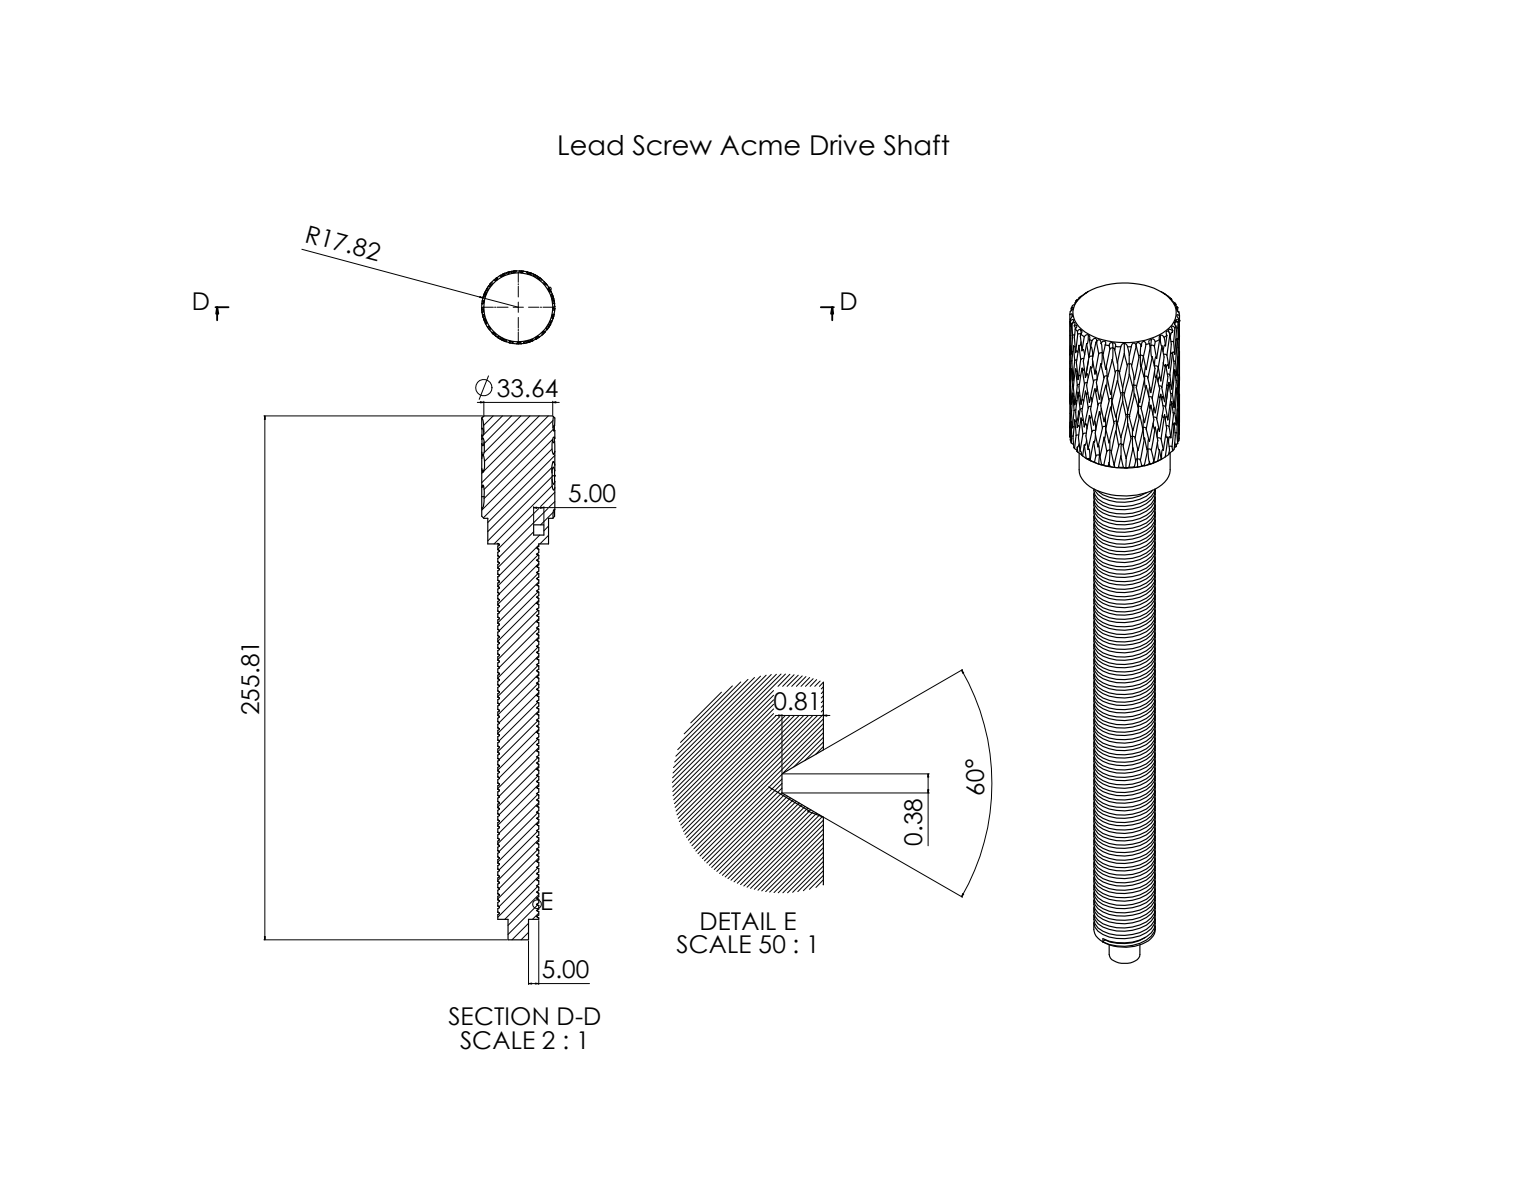
ISO-10303-21;
HEADER;
FILE_DESCRIPTION (('STEP AP214'),
    '1' );
FILE_NAME ('Lead Screw Acme Drive Shaft.step',
    '2026-10-24T22:31:37',
    ( '' ),
    ( '' ),
    'SwSTEP 2.0',
    'SolidWorks 2025',
    '' );
FILE_SCHEMA (( 'AUTOMOTIVE_DESIGN' ));
ENDSEC;

DATA;
#2=EDGE_CURVE ( 'NONE', #71353, #27127, #17244, .T. ) ;
#5=CARTESIAN_POINT ( 'NONE',  ( 165.5065167046122099, 285.3186853228385758, 0.5240180121679646197 ) ) ;
#6=CARTESIAN_POINT ( 'NONE',  ( 181.3318829485781976, 258.8378521386378566, -10.46588027007283017 ) ) ;
#8=ORIENTED_EDGE ( 'NONE', *, *, #76052, .F. ) ;
#9=CARTESIAN_POINT ( 'NONE',  ( 192.4853974341616549, 296.6629111496555424, 11.26379224701618398 ) ) ;
#12=CARTESIAN_POINT ( 'NONE',  ( 201.3053499423511425, 281.9759013948520874, -16.75960365258566398 ) ) ;
#15=CARTESIAN_POINT ( 'NONE',  ( 199.8044370756099966, 266.7412756917946695, 4.662294411209313871 ) ) ;
#16=CARTESIAN_POINT ( 'NONE',  ( 202.7688273210276293, 274.1343011241658587, 13.26872680179261366 ) ) ;
#19=CARTESIAN_POINT ( 'NONE',  ( 199.0151342380902406, 265.3454304162409585, 1.621217956766562551 ) ) ;
#20=CARTESIAN_POINT ( 'NONE',  ( 154.6973317394036940, 271.0068791071395253, 14.01324914462427174 ) ) ;
#21=VERTEX_POINT ( 'NONE', #91655 ) ;
#22=CARTESIAN_POINT ( 'NONE',  ( 146.8195026170398023, 276.3481572557323034, 4.765869558735466249 ) ) ;
#23=CARTESIAN_POINT ( 'NONE',  ( 202.2773826701151165, 280.2922913237452462, 16.62862787739668846 ) ) ;
#24=CARTESIAN_POINT ( 'NONE',  ( 164.2578067403839555, 246.1441285162624126, -2.322300236470859591 ) ) ;
#26=B_SPLINE_CURVE_WITH_KNOTS ( 'NONE', 3,
 ( #42002, #50106, #43488, #81061 ),
 .UNSPECIFIED., .F., .F.,
 ( 4, 4 ),
 ( 0.04462388129695979422, 0.04887120950165262795 ),
 .UNSPECIFIED. ) ;
#29=CARTESIAN_POINT ( 'NONE',  ( 171.0277932295235814, 274.5471866711665712, 17.25980421070102366 ) ) ;
#32=CARTESIAN_POINT ( 'NONE',  ( -22.42236680055709641, 157.8615022471902591, 0.000000000000000000 ) ) ;
#33=CARTESIAN_POINT ( 'NONE',  ( 149.7543087857887656, 247.2677522451417929, -5.000000000000041744 ) ) ;
#34=CARTESIAN_POINT ( 'NONE',  ( 82.20432729060253507, 208.2677522451417929, -5.000000000000041744 ) ) ;
#35=VERTEX_POINT ( 'NONE', #22220 ) ;
#41=CARTESIAN_POINT ( 'NONE',  ( 20.25662117580333899, 176.3768266524159856, -9.188101187500093303 ) ) ;
#42=FACE_OUTER_BOUND ( 'NONE', #88886, .T. ) ;
#43=ADVANCED_FACE ( 'NONE', ( #53119 ), #78501, .F. ) ;
#44=CARTESIAN_POINT ( 'NONE',  ( 181.8933809143826466, 275.6627081342313090, -16.43118812148207653 ) ) ;
#46=CARTESIAN_POINT ( 'NONE',  ( 119.5854454918513170, 251.3967562850347122, -4.648177544792955347E-16 ) ) ;
#48=DIRECTION ( 'NONE',  ( -0.8660254037844387076, -0.4999999999999998890, -0.000000000000000000 ) ) ;
#49=CARTESIAN_POINT ( 'NONE',  ( 176.0471099249906217, 252.5555583919553726, -3.347364798285545895 ) ) ;
#50=CARTESIAN_POINT ( 'NONE',  ( 190.7726985512088049, 261.9670508072832718, -0.9699378005772294475 ) ) ;
#51=CARTESIAN_POINT ( 'NONE',  ( 182.4467602783141729, 295.3384606270356585, 1.016252470355397008 ) ) ;
#52=CARTESIAN_POINT ( 'NONE',  ( 71.10837680816226225, 221.8615022471903160, 5.000000000000046185 ) ) ;
#55=CARTESIAN_POINT ( 'NONE',  ( 36.00728465925030974, 191.5958772461660544, -9.188101187500095079 ) ) ;
#57=ADVANCED_FACE ( 'NONE', ( #26227 ), #57103, .T. ) ;
#59=CARTESIAN_POINT ( 'NONE',  ( 72.04657099559547362, 205.7365022471902023, -10.00000000000009237 ) ) ;
#60=CARTESIAN_POINT ( 'NONE',  ( 198.6894790592683080, 286.5067226703918095, -17.06774375037124614 ) ) ;
#61=CARTESIAN_POINT ( 'NONE',  ( 164.2600772519394923, 246.1401958748887182, -2.110785484364219311 ) ) ;
#63=CARTESIAN_POINT ( 'NONE',  ( 159.8708946529933996, 278.4983629143405324, -9.843749539283454197 ) ) ;
#64=CARTESIAN_POINT ( 'NONE',  ( 160.1967185059513383, 280.0836358635930310, 9.265555704265979742 ) ) ;
#66=FACE_OUTER_BOUND ( 'NONE', #40596, .T. ) ;
#68=CARTESIAN_POINT ( 'NONE',  ( 188.9056787950111413, 270.0514309397178181, -14.11362088196558773 ) ) ;
#73=CARTESIAN_POINT ( 'NONE',  ( -4.101579717973121930, 179.9860189848785694, -2.679491924311240503 ) ) ;
#75=EDGE_LOOP ( 'NONE', ( #46929, #82112, #52955, #6832 ) ) ;
#79=CARTESIAN_POINT ( 'NONE',  ( 180.4501283053277803, 256.5846271277198412, -7.835696842545695873 ) ) ;
#81=ORIENTED_EDGE ( 'NONE', *, *, #67086, .T. ) ;
#83=ORIENTED_EDGE ( 'NONE', *, *, #17750, .F. ) ;
#84=CARTESIAN_POINT ( 'NONE',  ( 190.9907605556751093, 299.8412942717858414, 8.799173206188184437 ) ) ;
#85=DIRECTION ( 'NONE',  ( 0.4999999999999992784, -0.8660254037844390407, 0.000000000000000000 ) ) ;
#89=CARTESIAN_POINT ( 'NONE',  ( 148.3280470635002928, 273.7352816289870248, 9.058704604771318003 ) ) ;
#90=CARTESIAN_POINT ( 'NONE',  ( 196.4783028304046013, 290.3365922432724346, -16.37291435488387492 ) ) ;
#91=CARTESIAN_POINT ( 'NONE',  ( 173.2337249902883798, 270.7486416191997023, 17.82094672905207133 ) ) ;
#94=CARTESIAN_POINT ( 'NONE',  ( 159.3297396961336290, 265.7340194281295567, 16.79158499271843041 ) ) ;
#97=CARTESIAN_POINT ( 'NONE',  ( 149.4491471355718772, 271.7934793437897270, 11.43912701239353780 ) ) ;
#101=CARTESIAN_POINT ( 'NONE',  ( 159.7595800023532320, 255.3516961917271999, 16.21405881663931936 ) ) ;
#104=VERTEX_POINT ( 'NONE', #18635 ) ;
#106=CARTESIAN_POINT ( 'NONE',  ( 190.9402756120810523, 299.5005484933402613, 5.898581097966179243 ) ) ;
#108=CARTESIAN_POINT ( 'NONE',  ( 189.8480911035503880, 301.8204558191226283, -0.8992086515915015399 ) ) ;
#109=CARTESIAN_POINT ( 'NONE',  ( 190.2389970918280540, 301.1433867864428748, 4.601241515604689525 ) ) ;
#110=CARTESIAN_POINT ( 'NONE',  ( 173.6269293304046357, 276.7763204810394200, -15.65584202761720611 ) ) ;
#111=CARTESIAN_POINT ( 'NONE',  ( 146.5086121934486982, 276.8866352649785654, -0.04230388357226919777 ) ) ;
#113=CARTESIAN_POINT ( 'NONE',  ( 192.8011239859581849, 296.7056528303708660, -11.79847971295421694 ) ) ;
#114=CARTESIAN_POINT ( 'NONE',  ( 161.7445750920071816, 256.8061939151814386, 15.71254058960433397 ) ) ;
#116=DIRECTION ( 'NONE',  ( -0.8660254037844387076, -0.4999999999999998890, -0.000000000000000000 ) ) ;
#120=CARTESIAN_POINT ( 'NONE',  ( 105.9391831106087380, 219.7202760586659736, -5.415160957724236172E-17 ) ) ;
#122=CARTESIAN_POINT ( 'NONE',  ( 149.0943192338760070, 272.4080592974699471, -12.87526400066115606 ) ) ;
#126=CARTESIAN_POINT ( 'NONE',  ( 180.5399386764078997, 283.1336537301233420, -15.18944844307240238 ) ) ;
#130=VERTEX_POINT ( 'NONE', #94659 ) ;
#131=CARTESIAN_POINT ( 'NONE',  ( 163.0056347026689707, 248.3129541054019569, -11.27842346302751508 ) ) ;
#133=CARTESIAN_POINT ( 'NONE',  ( 45.39824762976388683, 187.0177522451417929, 5.000000000000051514 ) ) ;
#134=CARTESIAN_POINT ( 'NONE',  ( 124.5040820605901217, 248.8149278399160949, -9.188101187500095079 ) ) ;
#135=CARTESIAN_POINT ( 'NONE',  ( 180.7770252323854834, 294.0936096853982349, -2.952313513407788026 ) ) ;
#137=CARTESIAN_POINT ( 'NONE',  ( 157.6673516573649181, 257.5591315650518141, 16.79781451397666103 ) ) ;
#138=CARTESIAN_POINT ( 'NONE',  ( 175.3042518086594441, 253.4457403629180021, -3.880823026268251930 ) ) ;
#139=CARTESIAN_POINT ( 'NONE',  ( 46.23738328933649200, 191.3768266524159856, -9.188101187500091527 ) ) ;
#145=CARTESIAN_POINT ( 'NONE',  ( 146.8358616138309571, 276.3198226421291679, 4.054088818585255716 ) ) ;
#148=CARTESIAN_POINT ( 'NONE',  ( 17.25242200676963833, 170.7677522451417929, -5.000000000000041744 ) ) ;
#149=CARTESIAN_POINT ( 'NONE',  ( 102.9889369814289921, 240.2677522451419065, -5.000000000000047962 ) ) ;
#151=CARTESIAN_POINT ( 'NONE',  ( 163.3854574543125580, 247.6550818016845597, 10.82482370245618775 ) ) ;
#152=CARTESIAN_POINT ( 'NONE',  ( 163.3939361803663246, 247.6403962173759226, -10.78041711314006790 ) ) ;
#153=EDGE_CURVE ( 'NONE', #73023, #47320, #41466, .T. ) ;
#154=CARTESIAN_POINT ( 'NONE',  ( 29.56604717072103483, 194.0024278399160949, 9.188101187500095079 ) ) ;
#156=CARTESIAN_POINT ( 'NONE',  ( 195.4765535648738535, 273.5335777180424657, 14.55181105716135903 ) ) ;
#159=CARTESIAN_POINT ( 'NONE',  ( 194.7274671941087831, 275.0520795863097305, -15.83285290351333785 ) ) ;
#160=CARTESIAN_POINT ( 'NONE',  ( 69.07880331415105957, 204.5643266524160140, 9.188101187500095079 ) ) ;
#161=EDGE_CURVE ( 'NONE', #56410, #9864, #92298, .T. ) ;
#162=CARTESIAN_POINT ( 'NONE',  ( 161.4396252346964218, 251.0253620690641299, 14.51972485405798885 ) ) ;
#167=( BOUNDED_CURVE ( )  B_SPLINE_CURVE ( 2, ( #94120, #92619, #24674, #32772, #7471, #38365, #3886, #40856, #18091 ),
 .UNSPECIFIED., .F., .T. ) 
 B_SPLINE_CURVE_WITH_KNOTS ( ( 3, 2, 2, 2, 3 ),
 ( 0.1330645161290322509, 0.1344086021505376261, 0.1370967741935483764, 0.1397849462365591267, 0.1411290322580645296 ),
 .UNSPECIFIED. ) 
 CURVE ( )  GEOMETRIC_REPRESENTATION_ITEM ( )  RATIONAL_B_SPLINE_CURVE ( ( 0.9330127018922194093, 0.9330127018922194093, 1.000000000000000000, 0.8660254037844387076, 1.000000000000000000, 0.8660254037844387076, 1.000000000000000000, 0.9330127018922187432, 0.9330127018922194093 ) ) 
 REPRESENTATION_ITEM ( '' )  );
#168=CARTESIAN_POINT ( 'NONE',  ( 165.4887069070615269, 269.3414653546907402, 17.07898631664743405 ) ) ;
#169=CARTESIAN_POINT ( 'NONE',  ( 29.10614472461701752, 187.6115022471902591, 10.00000000000009592 ) ) ;
#170=CARTESIAN_POINT ( 'NONE',  ( 208.2175703429120688, 270.0035844679667889, 2.257951022351344150 ) ) ;
#171=CARTESIAN_POINT ( 'NONE',  ( -1.394013918807642360, 163.8768266524159856, 9.188101187500098632 ) ) ;
#173=CARTESIAN_POINT ( 'NONE',  ( 167.7163553651179768, 262.5077956943969753, -16.64284935447819791 ) ) ;
#175=CARTESIAN_POINT ( 'NONE',  ( 185.3704253846254346, 260.3657602090070782, 6.355839938251095944 ) ) ;
#176=CARTESIAN_POINT ( 'NONE',  ( 206.0627831668701901, 273.7357853363691902, 10.14454147593459687 ) ) ;
#181=CARTESIAN_POINT ( 'NONE',  ( 208.2813134324037492, 269.8931781983357041, -0.4511785827856357178 ) ) ;
#188=CARTESIAN_POINT ( 'NONE',  ( 84.96478326871331888, 219.8615022471902591, -10.00000000000009592 ) ) ;
#189=CARTESIAN_POINT ( 'NONE',  ( 173.0837253472800796, 264.8280141993791972, 17.07053884509587860 ) ) ;
#190=CARTESIAN_POINT ( 'NONE',  ( 162.6541320028305506, 248.9217746405196294, -10.16950121496441817 ) ) ;
#197=ORIENTED_EDGE ( 'NONE', *, *, #54268, .F. ) ;
#202=CARTESIAN_POINT ( 'NONE',  ( 171.2743479101317234, 254.4242377521371736, -11.94796457435898951 ) ) ;
#203=CARTESIAN_POINT ( 'NONE',  ( 164.2712161151136172, 246.1209027979328710, 7.276091357954241445 ) ) ;
#206=CARTESIAN_POINT ( 'NONE',  ( 155.6989589471585020, 260.9684877483775267, 17.28906573347438425 ) ) ;
#207=CARTESIAN_POINT ( 'NONE',  ( 151.2455280670316711, 268.6820563007532314, 14.35914944935941229 ) ) ;
#214=CARTESIAN_POINT ( 'NONE',  ( 159.9635946688021022, 268.7707599091479551, -17.14635356962945778 ) ) ;
#217=ORIENTED_EDGE ( 'NONE', *, *, #97229, .F. ) ;
#219=CARTESIAN_POINT ( 'NONE',  ( 207.5792673731680793, 271.1091576421853233, 2.359198794924813214 ) ) ;
#221=CARTESIAN_POINT ( 'NONE',  ( 167.3703162778506055, 281.6204983129350694, 11.41617640160279024 ) ) ;
#222=CARTESIAN_POINT ( 'NONE',  ( 194.9220242159064185, 293.0321458743159724, -14.92681063007793263 ) ) ;
#225=ADVANCED_FACE ( 'NONE', ( #75832 ), #98127, .T. ) ;
#228=CARTESIAN_POINT ( 'NONE',  ( 198.4408884114532725, 277.4403926908931908, -15.34803116808097023 ) ) ;
#232=EDGE_CURVE ( 'NONE', #38319, #90439, #71654, .T. ) ;
#233=CARTESIAN_POINT ( 'NONE',  ( 147.2256490141643042, 275.6446910606013603, -4.110658582098289493 ) ) ;
#236=CARTESIAN_POINT ( 'NONE',  ( 206.3018347371251195, 273.3217358710584790, -9.309724106897926177 ) ) ;
#239=CARTESIAN_POINT ( 'NONE',  ( 171.8224262749942852, 254.8926688302297521, 11.02064826558146748 ) ) ;
#240=CARTESIAN_POINT ( 'NONE',  ( 157.5687383428415274, 281.7222027203141579, 1.387399794590924440 ) ) ;
#242=CARTESIAN_POINT ( 'NONE',  ( 194.3044832453722677, 294.1017582110366106, -14.10778293554018603 ) ) ;
#244=CARTESIAN_POINT ( 'NONE',  ( 141.2767884429413243, 240.8262482093457777, 3.021315404115420679E-15 ) ) ;
#245=CARTESIAN_POINT ( 'NONE',  ( -0.9341114727036189391, 170.2677522451418781, 10.00000000000009592 ) ) ;
#246=CARTESIAN_POINT ( 'NONE',  ( 94.73480590126506229, 219.3768266524160140, 9.188101187500096856 ) ) ;
#247=CARTESIAN_POINT ( 'NONE',  ( 195.8651621160345542, 269.3302623707359658, -10.80388373675355851 ) ) ;
#250=CARTESIAN_POINT ( 'NONE',  ( 170.2105851965358738, 280.7371124046519526, -14.06690082814746390 ) ) ;
#252=CARTESIAN_POINT ( 'NONE',  ( 17.27983239817682559, 168.5327760586659736, 1.948934522072303157E-15 ) ) ;
#254=CARTESIAN_POINT ( 'NONE',  ( 200.4592688079413847, 283.4413569069752725, 18.39277739746426832 ) ) ;
#255=ORIENTED_EDGE ( 'NONE', *, *, #28716, .T. ) ;
#256=ORIENTED_EDGE ( 'NONE', *, *, #59561, .F. ) ;
#257=CARTESIAN_POINT ( 'NONE',  ( 167.4700212936181458, 285.1112495945437786, 9.221858443278774686 ) ) ;
#259=CARTESIAN_POINT ( 'NONE',  ( 157.8159121039657293, 257.3018173235443555, -17.05074702406642118 ) ) ;
#261=CARTESIAN_POINT ( 'NONE',  ( 201.9437967514558920, 280.8700790835527528, -16.67046097481324196 ) ) ;
#262=CARTESIAN_POINT ( 'NONE',  ( 113.9506338607584723, 225.0494855054051868, -2.679491924311248496 ) ) ;
#264=CARTESIAN_POINT ( 'NONE',  ( 23.34166312890287998, 184.2833772461660544, -9.188101187500095079 ) ) ;
#265=CARTESIAN_POINT ( 'NONE',  ( 130.0524911732904343, 236.7048013555409796, 4.594050593750051981 ) ) ;
#266=CARTESIAN_POINT ( 'NONE',  ( 183.1279196651564973, 257.7771318069471249, -2.489900343309737529 ) ) ;
#267=ORIENTED_EDGE ( 'NONE', *, *, #37270, .F. ) ;
#268=CARTESIAN_POINT ( 'NONE',  ( 179.8888715531147682, 274.4711782159853328, -17.82026667163308531 ) ) ;
#269=CARTESIAN_POINT ( 'NONE',  ( -8.863483026448420787, 159.5643266524160140, 9.188101187500095079 ) ) ;
#271=CARTESIAN_POINT ( 'NONE',  ( 194.5047661587782386, 293.7548580291293092, 14.86680123054176583 ) ) ;
#272=CARTESIAN_POINT ( 'NONE',  ( 177.2183068813167495, 256.3290312667157309, -10.31296860541032423 ) ) ;
#273=CARTESIAN_POINT ( 'NONE',  ( 190.1462790299653420, 284.8797699240140560, 17.00550891877788473 ) ) ;
#274=CARTESIAN_POINT ( 'NONE',  ( 147.6508870500795467, 274.9081571770856272, -8.950912509993816712 ) ) ;
#275=CARTESIAN_POINT ( 'NONE',  ( 189.2224370172964143, 262.6230431603515854, 8.075317388220659254 ) ) ;
#276=CARTESIAN_POINT ( 'NONE',  ( 167.7174649547847309, 278.2620246372183601, 14.62053864993239216 ) ) ;
#279=CARTESIAN_POINT ( 'NONE',  ( 148.3707431749605234, 273.6613297946520902, 8.912574527564540716 ) ) ;
#281=ORIENTED_EDGE ( 'NONE', *, *, #67790, .T. ) ;
#283=CARTESIAN_POINT ( 'NONE',  ( 184.9437015084479299, 269.6468049839930927, 15.52015019358652204 ) ) ;
#284=CARTESIAN_POINT ( 'NONE',  ( 109.0781781035623226, 233.7833772461660544, -9.188101187500095079 ) ) ;
#286=CARTESIAN_POINT ( 'NONE',  ( 190.9907605556751093, 299.8412942717858414, 8.799173206188184437 ) ) ;
#288=CYLINDRICAL_SURFACE ( 'NONE', #48455, 17.82106496071139645 ) ;
#290=CARTESIAN_POINT ( 'NONE',  ( 195.5685147139090816, 278.4936960503050045, 16.53693894814080423 ) ) ;
#291=CARTESIAN_POINT ( 'NONE',  ( 201.3138726815416817, 270.7303338844035352, -9.934698065831957692 ) ) ;
#292=CARTESIAN_POINT ( 'NONE',  ( 163.2031704490160848, 279.2514240946757695, 12.88724473550253258 ) ) ;
#293=CARTESIAN_POINT ( 'NONE',  ( 137.7719789713245291, 261.8967562850346553, -4.648177544792955347E-16 ) ) ;
#298=CARTESIAN_POINT ( 'NONE',  ( 163.8995163580303256, 256.4334289116373498, -14.90821826893867730 ) ) ;
#302=CARTESIAN_POINT ( 'NONE',  ( 149.5390997184345281, 271.6376768999995761, -11.52989534384373016 ) ) ;
#305=B_SPLINE_SURFACE_WITH_KNOTS ( 'NONE', 3, 1, ( 
 ( #12840, #43700 ),
 ( #74643, #5218 ),
 ( #82762, #13328 ),
 ( #36596, #67500 ),
 ( #98432, #29023 ),
 ( #59894, #44684 ),
 ( #39075, #60879 ),
 ( #91339, #6708 ),
 ( #61389, #92343 ),
 ( #76606, #22402 ),
 ( #37586, #53297 ),
 ( #7698, #46696 ),
 ( #602, #22892 ),
 ( #14308, #91841 ),
 ( #8206, #99420 ),
 ( #45194, #69988 ),
 ( #69496, #23889 ),
 ( #99915, #7192 ),
 ( #68496, #84250 ),
 ( #92834, #15789 ),
 ( #38077, #54790 ),
 ( #14798, #21899 ),
 ( #68004, #53777 ),
 ( #38590, #77621 ),
 ( #31486, #84740 ),
 ( #76133, #45680 ),
 ( #62378, #29997 ),
 ( #68990, #93335 ),
 ( #109, #85769 ),
 ( #30501, #15281 ),
 ( #46176, #77096 ),
 ( #83745, #30994 ),
 ( #61879, #16297 ),
 ( #23385, #54275 ) ),
 .UNSPECIFIED., .T., .F., .F.,
 ( 4, 2, 2, 2, 2, 2, 2, 2, 2, 2, 2, 2, 2, 2, 2, 2, 4 ),
 ( 2, 2 ),
 ( 0.000000000000000000, 0.06250000000000000000, 0.1250000000000000000, 0.1875000000000000000, 0.2500000000000000000, 0.3125000000000000000, 0.3750000000000000000, 0.4375000000000000000, 0.5000000000000000000, 0.5625000000000000000, 0.6250000000000000000, 0.6875000000000000000, 0.7500000000000000000, 0.8125000000000000000, 0.8750000000000000000, 0.9375000000000000000, 1.000000000000000000 ),
 ( 0.000000000000000000, 1.000000000000000000 ),
 .UNSPECIFIED. ) ;
#309=CARTESIAN_POINT ( 'NONE',  ( 183.6798712561491982, 264.4388490002158960, -13.51192819117503596 ) ) ;
#311=CARTESIAN_POINT ( 'NONE',  ( 152.6845319923753834, 266.1896283897672220, 17.20844521882669653 ) ) ;
#312=VERTEX_POINT ( 'NONE', #28205 ) ;
#316=CARTESIAN_POINT ( 'NONE',  ( 167.5102911960937320, 249.8330499937025309, 6.951336391313942542 ) ) ;
#318=B_SPLINE_CURVE_WITH_KNOTS ( 'NONE', 3,
 ( #32597, #24493, #55372, #7801 ),
 .UNSPECIFIED., .F., .F.,
 ( 4, 4 ),
 ( 0.02854077651451781411, 0.03771323773808555463 ),
 .UNSPECIFIED. ) ;
#321=CARTESIAN_POINT ( 'NONE',  ( 158.9773147466768819, 255.2902089383236159, 17.46634807813732237 ) ) ;
#322=CARTESIAN_POINT ( 'NONE',  ( 192.9115332263593814, 296.5144184163711429, -13.56440505672942898 ) ) ;
#323=CARTESIAN_POINT ( 'NONE',  ( 163.1062016187225936, 254.8584145212696228, 15.52417137768656019 ) ) ;
#327=ORIENTED_EDGE ( 'NONE', *, *, #3828, .T. ) ;
#328=CARTESIAN_POINT ( 'NONE',  ( 195.4130005142917241, 291.0508895501969846, 16.15472393341080348 ) ) ;
#331=ORIENTED_EDGE ( 'NONE', *, *, #16780, .F. ) ;
#332=CARTESIAN_POINT ( 'NONE',  ( 171.7871149756895761, 270.4574563033415870, 16.48193621075655102 ) ) ;
#334=EDGE_CURVE ( 'NONE', #85237, #99635, #55991, .T. ) ;
#338=CARTESIAN_POINT ( 'NONE',  ( 196.1025787785897307, 284.4507243824010629, -17.50425523595241017 ) ) ;
#340=CARTESIAN_POINT ( 'NONE',  ( 167.6634616256541790, 249.2278186638985744, -5.457181400944699057 ) ) ;
#341=DIRECTION ( 'NONE',  ( -0.8660254037844387076, -0.4999999999999998890, -0.000000000000000000 ) ) ;
#343=CARTESIAN_POINT ( 'NONE',  ( 186.8073520874924611, 287.1005927419247996, -15.84640929283254174 ) ) ;
#344=ADVANCED_FACE ( 'NONE', ( #31678 ), #99228, .T. ) ;
#345=CARTESIAN_POINT ( 'NONE',  ( 119.1457234225564008, 239.5958772461660544, -9.188101187500095079 ) ) ;
#346=VERTEX_POINT ( 'NONE', #7914 ) ;
#349=CARTESIAN_POINT ( 'NONE',  ( 189.4928799553373437, 274.7536700704093846, 17.18705487055967396 ) ) ;
#350=ORIENTED_EDGE ( 'NONE', *, *, #95990, .T. ) ;
#352=ORIENTED_EDGE ( 'NONE', *, *, #17619, .T. ) ;
#356=CARTESIAN_POINT ( 'NONE',  ( 171.0928659016861673, 287.7346803495887002, -4.756451642342891972 ) ) ;
#359=CARTESIAN_POINT ( 'NONE',  ( 153.1961624462112752, 265.3034584490234806, -16.19494717845262954 ) ) ;
#360=CARTESIAN_POINT ( 'NONE',  ( 177.2362443690770135, 288.8424983797139021, -9.276591687040479428 ) ) ;
#363=CARTESIAN_POINT ( 'NONE',  ( 164.5340810747928515, 246.5053760637088658, 4.244836759601243514 ) ) ;
#364=ORIENTED_EDGE ( 'NONE', *, *, #82612, .F. ) ;
#365=CARTESIAN_POINT ( 'NONE',  ( 147.9791529310278122, 274.3395839928920168, -7.789432462804474433 ) ) ;
#368=CARTESIAN_POINT ( 'NONE',  ( 188.2054311839045226, 266.2807901288332459, -11.82779421608511150 ) ) ;
#369=CARTESIAN_POINT ( 'NONE',  ( 156.9836120038223726, 276.6206255467238293, 10.24398227673275841 ) ) ;
#370=CARTESIAN_POINT ( 'NONE',  ( 195.6984238921373560, 265.3498530178097212, 4.338345965406653626 ) ) ;
#371=CARTESIAN_POINT ( 'NONE',  ( 179.8888715531147682, 274.4711782159853328, -17.82026667163308531 ) ) ;
#373=CARTESIAN_POINT ( 'NONE',  ( 153.4529711877194131, 270.0553744293359841, 14.23171068006870854 ) ) ;
#375=CARTESIAN_POINT ( 'NONE',  ( 200.7484899876179441, 282.9404111291507888, -16.88964748465601673 ) ) ;
#376=ORIENTED_EDGE ( 'NONE', *, *, #23774, .F. ) ;
#377=CARTESIAN_POINT ( 'NONE',  ( 147.4963928429778264, 275.1757489932608109, 4.929816573182678852 ) ) ;
#379=CARTESIAN_POINT ( 'NONE',  ( 187.3693387071396046, 263.1408467955632204, -9.037621127357647666 ) ) ;
#381=CARTESIAN_POINT ( 'NONE',  ( 173.8665542827094725, 250.6399523573830095, -0.9454928766311748722 ) ) ;
#382=B_SPLINE_CURVE_WITH_KNOTS ( 'NONE', 3,
 ( #16996, #47885, #78827, #78323 ),
 .UNSPECIFIED., .F., .F.,
 ( 4, 4 ),
 ( 0.003697259335896347244, 0.01166702794401381499 ),
 .UNSPECIFIED. ) ;
#383=CARTESIAN_POINT ( 'NONE',  ( 184.7157775894015117, 297.3647472220100099, -4.497232409310948142 ) ) ;
#386=CARTESIAN_POINT ( 'NONE',  ( 155.2419697281468416, 261.7600162942170527, 18.58580762350309357 ) ) ;
#387=CARTESIAN_POINT ( 'NONE',  ( 191.1424450985878138, 283.3691956586972083, -16.58317466969614173 ) ) ;
#389=CARTESIAN_POINT ( 'NONE',  ( 84.82981389336303835, 207.5327760586659167, 1.948934522072303157E-15 ) ) ;
#394=CARTESIAN_POINT ( 'NONE',  ( 202.8535267948003593, 279.2943804273081696, -15.36804658072946062 ) ) ;
#395=DIRECTION ( 'NONE',  ( 0.4999999999999992784, -0.8660254037844390407, 0.000000000000000000 ) ) ;
#397=CARTESIAN_POINT ( 'NONE',  ( 48.76667776935668996, 187.4155109091896065, 2.679491924311254714 ) ) ;
#400=FACE_OUTER_BOUND ( 'NONE', #98699, .T. ) ;
#401=CARTESIAN_POINT ( 'NONE',  ( 166.1592670111344887, 249.7066296865716311, -9.087955240109561572 ) ) ;
#402=CARTESIAN_POINT ( 'NONE',  ( 205.5338712131946863, 274.6518877128656868, -12.59077173197751343 ) ) ;
#403=CARTESIAN_POINT ( 'NONE',  ( 195.8248271798537417, 291.4684452715354155, 17.35175160929494709 ) ) ;
#404=CARTESIAN_POINT ( 'NONE',  ( 167.9211111253673323, 249.4040118433879627, 8.061254949035708606 ) ) ;
#405=CARTESIAN_POINT ( 'NONE',  ( 207.5785076975260779, 271.1104734389944042, -6.824813054587777650 ) ) ;
#406=CARTESIAN_POINT ( 'NONE',  ( 43.09804120061789945, 189.5643266524160140, 9.188101187500095079 ) ) ;
#407=CARTESIAN_POINT ( 'NONE',  ( 56.16917826928300883, 212.4244531367911577, -4.594050593750046652 ) ) ;
#408=CARTESIAN_POINT ( 'NONE',  ( 185.8626946602280441, 259.3471889805154547, 7.308832903665572367 ) ) ;
#411=CARTESIAN_POINT ( 'NONE',  ( 163.8983913010820572, 258.1275895590765685, 15.54516205773220250 ) ) ;
#412=CARTESIAN_POINT ( 'NONE',  ( -3.441976700948088386, 155.4865022471901455, 1.119607411625061291E-15 ) ) ;
#416=CARTESIAN_POINT ( 'NONE',  ( 132.8668134119921547, 247.5177522451418497, -10.00000000000009592 ) ) ;
#419=CARTESIAN_POINT ( 'NONE',  ( 70.29673831216418023, 202.2048013555409796, 4.594050593750051981 ) ) ;
#421=CARTESIAN_POINT ( 'NONE',  ( 155.2193237801463113, 261.7992402267395846, -18.58295809893692407 ) ) ;
#422=CARTESIAN_POINT ( 'NONE',  ( 159.6978881494930249, 254.0421391940632532, 15.34888828951022610 ) ) ;
#424=CARTESIAN_POINT ( 'NONE',  ( 153.3576077035983758, 276.7962943880863804, 7.310696788985877603 ) ) ;
#426=B_SPLINE_CURVE_WITH_KNOTS ( 'NONE', 3,
 ( #1225, #30627, #55888, #713 ),
 .UNSPECIFIED., .F., .F.,
 ( 4, 4 ),
 ( 0.04422796245080886507, 0.04887120950165270428 ),
 .UNSPECIFIED. ) ;
#427=EDGE_CURVE ( 'NONE', #15755, #20151, #43801, .T. ) ;
#429=CARTESIAN_POINT ( 'NONE',  ( 113.4714528099510744, 242.9865022471902876, -10.00000000000009415 ) ) ;
#430=CARTESIAN_POINT ( 'NONE',  ( 200.8828793852583203, 282.7076418644388696, 17.90302398138411633 ) ) ;
#431=CARTESIAN_POINT ( 'NONE',  ( 164.4440639631384045, 245.8215215431751233, -2.910115319305802029 ) ) ;
#432=ORIENTED_EDGE ( 'NONE', *, *, #46720, .F. ) ;
#436=CARTESIAN_POINT ( 'NONE',  ( 206.1405152101578437, 273.6011494880188479, -9.618815605734603480 ) ) ;
#437=CARTESIAN_POINT ( 'NONE',  ( 190.3113039736807934, 278.6935773923744364, -16.50932879894303085 ) ) ;
#439=EDGE_LOOP ( 'NONE', ( #58462, #85908, #2245, #41062 ) ) ;
#440=CARTESIAN_POINT ( 'NONE',  ( 173.3330552357551824, 251.5762317818503959, 0.1350323028907620126 ) ) ;
#441=VERTEX_POINT ( 'NONE', #51248 ) ;
#443=CARTESIAN_POINT ( 'NONE',  ( 147.8308140999695866, 274.5965143850199865, -7.866624397492971710 ) ) ;
#446=ORIENTED_EDGE ( 'NONE', *, *, #42908, .T. ) ;
#454=CARTESIAN_POINT ( 'NONE',  ( 206.7680519836501958, 272.5142239127119979, -10.57935479673322021 ) ) ;
#455=ORIENTED_EDGE ( 'NONE', *, *, #60528, .T. ) ;
#456=CARTESIAN_POINT ( 'NONE',  ( 174.8047606067528363, 286.1344884131184472, 10.79450168243746688 ) ) ;
#457=EDGE_CURVE ( 'NONE', #20349, #15680, #60827, .T. ) ;
#458=CARTESIAN_POINT ( 'NONE',  ( 162.5887743522035294, 284.9919049736276975, -2.844505511527740005 ) ) ;
#460=CARTESIAN_POINT ( 'NONE',  ( 163.4218292706009095, 247.5920839679097014, -10.44611490715852042 ) ) ;
#461=CARTESIAN_POINT ( 'NONE',  ( 204.9103773355753617, 275.7318107871104189, 13.62808820451859937 ) ) ;
#462=CARTESIAN_POINT ( 'NONE',  ( 185.4002507578896086, 292.6011188852542091, -10.72436994641770269 ) ) ;
#463=CARTESIAN_POINT ( 'NONE',  ( 164.3112807403088595, 265.7596940169248683, -17.57772941833111346 ) ) ;
#464=CARTESIAN_POINT ( 'NONE',  ( 141.8249372320439647, 246.5643266524160140, 9.188101187500095079 ) ) ;
#465=CARTESIAN_POINT ( 'NONE',  ( 165.2663344650013642, 263.6115507486170486, 17.68040007492823662 ) ) ;
#467=CARTESIAN_POINT ( 'NONE',  ( 181.8478599454992661, 260.3285582005539709, 9.484317556428793594 ) ) ;
#468=CARTESIAN_POINT ( 'NONE',  ( 71.08131351252005459, 211.8458772461660544, 9.188101187500095079 ) ) ;
#469=VERTEX_POINT ( 'NONE', #18019 ) ;
#470=CARTESIAN_POINT ( 'NONE',  ( 191.0900422946452011, 299.6693332556258724, 8.872191398975367349 ) ) ;
#473=CARTESIAN_POINT ( 'NONE',  ( 196.0559066898898379, 291.0682038195648715, -16.90522961251436485 ) ) ;
#474=ORIENTED_EDGE ( 'NONE', *, *, #73314, .T. ) ;
#476=EDGE_CURVE ( 'NONE', #86658, #66772, #15991, .T. ) ;
#480=CARTESIAN_POINT ( 'NONE',  ( 56.79295721098551297, 192.0494855054051868, -2.679491924311248496 ) ) ;
#481=CARTESIAN_POINT ( 'NONE',  ( 162.4279131726858623, 249.3135971479585464, 10.85034575916916921 ) ) ;
#482=CARTESIAN_POINT ( 'NONE',  ( 87.75264963113552596, 209.2202760586659167, -5.415160957724236172E-17 ) ) ;
#483=VERTEX_POINT ( 'NONE', #71220 ) ;
#487=CARTESIAN_POINT ( 'NONE',  ( 161.3271158790198001, 251.2202339894231216, -13.00083852162470244 ) ) ;
#490=CARTESIAN_POINT ( 'NONE',  ( 184.0117498620529659, 275.1892951444139612, 16.37277468287277671 ) ) ;
#491=ADVANCED_FACE ( 'NONE', ( #88467 ), #10916, .T. ) ;
#492=CARTESIAN_POINT ( 'NONE',  ( 206.4695239676918845, 273.0312896038346366, 10.41704154450801667 ) ) ;
#493=CARTESIAN_POINT ( 'NONE',  ( 161.9109773315472012, 284.6651530195127293, 0.5383145704399616704 ) ) ;
#495=CARTESIAN_POINT ( 'NONE',  ( 162.8949375270381665, 261.5393056731645061, 17.17550692532979895 ) ) ;
#499=CARTESIAN_POINT ( 'NONE',  ( 152.9251141908703175, 265.7729277985770864, -16.20110192949203309 ) ) ;
#503=CARTESIAN_POINT ( 'NONE',  ( 195.7907645185857461, 265.4364973583962524, 4.438536951565118294 ) ) ;
#504=CARTESIAN_POINT ( 'NONE',  ( 98.80083580102480312, 239.3967562850347122, -4.648177544792955347E-16 ) ) ;
#506=CARTESIAN_POINT ( 'NONE',  ( 187.8986993795193428, 266.2277010579576881, -11.94388868202539911 ) ) ;
#507=CARTESIAN_POINT ( 'NONE',  ( 198.6368176188399275, 266.0031191539155770, 1.462458297540865537 ) ) ;
#510=B_SPLINE_CURVE_WITH_KNOTS ( 'NONE', 3,
 ( #45409, #38802, #46912, #7929 ),
 .UNSPECIFIED., .F., .F.,
 ( 4, 4 ),
 ( 0.02277490244884483594, 0.03199231217593029308 ),
 .UNSPECIFIED. ) ;
#513=CARTESIAN_POINT ( 'NONE',  ( 202.5511585997265911, 279.8180975037686835, 17.12781264818056925 ) ) ;
#514=DIRECTION ( 'NONE',  ( -0.8660254037844359321, -0.5000000000000051070, -0.000000000000000000 ) ) ;
#517=CARTESIAN_POINT ( 'NONE',  ( 176.1295626651131556, 285.2769818187388751, -12.16386616229632800 ) ) ;
#520=CARTESIAN_POINT ( 'NONE',  ( 168.9255865893414921, 272.9744073663551376, 15.96626197445653261 ) ) ;
#522=CARTESIAN_POINT ( 'NONE',  ( 176.3945350884862933, 261.0281843545697029, -14.71337765310037504 ) ) ;
#523=CARTESIAN_POINT ( 'NONE',  ( 188.2324206269368858, 260.8148967101335529, 3.170919259758945952 ) ) ;
#524=CARTESIAN_POINT ( 'NONE',  ( 12.40843950188935629, 165.7202760586659736, -5.415160957724236172E-17 ) ) ;
#528=CARTESIAN_POINT ( 'NONE',  ( -22.42236680055709641, 157.8615022471902591, 0.000000000000000000 ) ) ;
#531=CARTESIAN_POINT ( 'NONE',  ( 25.61497981383703149, 185.5958772461660544, -9.188101187500095079 ) ) ;
#535=CARTESIAN_POINT ( 'NONE',  ( 191.7247331938518187, 298.5700163710982338, -9.650650827884682315 ) ) ;
#536=CARTESIAN_POINT ( 'NONE',  ( 142.5294721856450053, 241.5494855054051584, -2.679491924311248496 ) ) ;
#537=B_SPLINE_SURFACE_WITH_KNOTS ( 'NONE', 3, 1, ( 
 ( #25794, #64786 ),
 ( #41970, #96714 ),
 ( #10586, #19203 ),
 ( #57158, #3497 ),
 ( #88139, #43459 ),
 ( #50560, #42940 ),
 ( #41459, #81030 ),
 ( #96214, #56670 ),
 ( #73879, #4472 ),
 ( #26777, #57658 ),
 ( #11593, #11095 ),
 ( #34855, #82013 ),
 ( #66275, #97210 ),
 ( #89625, #74400 ),
 ( #87655, #49084 ),
 ( #80017, #72402 ),
 ( #3009, #33901 ),
 ( #95732, #26284 ),
 ( #18685, #49568 ),
 ( #72907, #14572 ),
 ( #75892, #28768 ),
 ( #22162, #29274 ),
 ( #15043, #76853 ),
 ( #5967, #43950 ),
 ( #98186, #30258 ),
 ( #82527, #74889 ),
 ( #84500, #22668 ),
 ( #59650, #97693 ),
 ( #98692, #37349 ),
 ( #28262, #45448 ),
 ( #90621, #44952 ),
 ( #92116, #36356 ),
 ( #76381, #21185 ),
 ( #14066, #60636 ) ),
 .UNSPECIFIED., .T., .F., .F.,
 ( 4, 2, 2, 2, 2, 2, 2, 2, 2, 2, 2, 2, 2, 2, 2, 2, 4 ),
 ( 2, 2 ),
 ( 0.000000000000000000, 0.06250000000000000000, 0.1250000000000000000, 0.1875000000000000000, 0.2500000000000000000, 0.3125000000000000000, 0.3750000000000000000, 0.4375000000000000000, 0.5000000000000000000, 0.5625000000000000000, 0.6250000000000000000, 0.6875000000000000000, 0.7500000000000000000, 0.8125000000000000000, 0.8750000000000000000, 0.9375000000000000000, 1.000000000000000000 ),
 ( 0.000000000000000000, 1.000000000000000000 ),
 .UNSPECIFIED. ) ;
#539=CARTESIAN_POINT ( 'NONE',  ( 174.3697573357644899, 277.1653490889620457, -17.12727634137145571 ) ) ;
#541=EDGE_CURVE ( 'NONE', #2236, #46058, #2271, .T. ) ;
#542=CARTESIAN_POINT ( 'NONE',  ( 183.0713581288837304, 295.8141884393991745, 1.453977782348063963 ) ) ;
#543=CARTESIAN_POINT ( 'NONE',  ( 64.97403019802248991, 214.9865022471903160, 10.00000000000009237 ) ) ;
#545=CARTESIAN_POINT ( 'NONE',  ( 205.7559715084180425, 271.1536124878838336, 6.114938359024117531 ) ) ;
#546=EDGE_CURVE ( 'NONE', #4549, #55003, #44142, .T. ) ;
#547=CARTESIAN_POINT ( 'NONE',  ( 24.66750420662404508, 194.2369531367911293, -4.594050593750048428 ) ) ;
#549=EDGE_CURVE ( 'NONE', #7391, #22636, #70359, .T. ) ;
#550=CARTESIAN_POINT ( 'NONE',  ( 73.72680694775513643, 201.8262482093457777, 3.021315404115420679E-15 ) ) ;
#551=CARTESIAN_POINT ( 'NONE',  ( 198.8570476668614049, 286.2164853282868080, -17.01721544293231858 ) ) ;
#554=CARTESIAN_POINT ( 'NONE',  ( 159.9770076892122006, 278.5918188642896212, -9.796288430209179054 ) ) ;
#556=SHAPE_DEFINITION_REPRESENTATION ( #17576, #88422 ) ;
#558=CARTESIAN_POINT ( 'NONE',  ( 190.5444288681022442, 300.6143634316900943, -1.000014190476072873 ) ) ;
#559=CARTESIAN_POINT ( 'NONE',  ( 100.0535195437283988, 240.1199935810941213, 2.679491924311251605 ) ) ;
#562=CARTESIAN_POINT ( 'NONE',  ( 185.5148080131019412, 290.8628339942631555, 13.12244952321606206 ) ) ;
#565=CARTESIAN_POINT ( 'NONE',  ( -3.532187684056978583, 178.7677522451419350, -5.000000000000047962 ) ) ;
#567=CARTESIAN_POINT ( 'NONE',  ( 174.1456200854750023, 291.7975269716956177, -2.042136877227955782 ) ) ;
#569=CARTESIAN_POINT ( 'NONE',  ( 150.8167050463783312, 269.4247995599803289, 14.38040671671637938 ) ) ;
#570=CARTESIAN_POINT ( 'NONE',  ( 180.2008674086625888, 256.3788900776044102, -7.862092545524210330 ) ) ;
#573=CARTESIAN_POINT ( 'NONE',  ( 189.0587110057432483, 273.8589833282692325, -15.65961006902252883 ) ) ;
#576=CARTESIAN_POINT ( 'NONE',  ( 191.3375250863502970, 299.2406804863936145, 8.828791580707859410 ) ) ;
#580=CARTESIAN_POINT ( 'NONE',  ( 190.5154909595809727, 300.6644853595138329, -0.04129855346138300298 ) ) ;
#584=CARTESIAN_POINT ( 'NONE',  ( 161.8159150606452670, 267.0902596021308568, 16.49972241951906327 ) ) ;
#585=ORIENTED_EDGE ( 'NONE', *, *, #42908, .F. ) ;
#587=CARTESIAN_POINT ( 'NONE',  ( 149.5593209768671841, 271.6026526530012575, 11.55487339793564949 ) ) ;
#592=CARTESIAN_POINT ( 'NONE',  ( 150.2494575935072874, 270.4073009688167986, 14.61449051812962985 ) ) ;
#598=AXIS2_PLACEMENT_3D ( 'NONE', #72578, #77279, #80192 ) ;
#600=CARTESIAN_POINT ( 'NONE',  ( 190.5444288681022442, 300.6143634316900943, -1.000014190476072873 ) ) ;
#602=CARTESIAN_POINT ( 'NONE',  ( 190.6023073677431512, 300.5141149296460981, 3.174888932019753973 ) ) ;
#603=CARTESIAN_POINT ( 'NONE',  ( 132.5758265486178971, 258.8967562850347122, -4.648177544792955347E-16 ) ) ;
#604=CARTESIAN_POINT ( 'NONE',  ( 191.0739205222354258, 299.6972569845476073, 8.800115285385583519 ) ) ;
#605=CARTESIAN_POINT ( 'NONE',  ( 147.4323331177958494, 275.2867036919951147, -5.064030047414062707 ) ) ;
#607=CARTESIAN_POINT ( 'NONE',  ( 163.5023530932012079, 257.7703811534142346, 15.52546879389397461 ) ) ;
#610=CARTESIAN_POINT ( 'NONE',  ( 205.7576124508049418, 274.2643565215761328, 10.88614016733041545 ) ) ;
#614=CARTESIAN_POINT ( 'NONE',  ( 115.2218061334819623, 228.1423013555409796, -4.594050593750043987 ) ) ;
#615=ORIENTED_EDGE ( 'NONE', *, *, #63474, .T. ) ;
#616=CARTESIAN_POINT ( 'NONE',  ( 190.0576675296552764, 301.4574588010404455, -4.282990501740621347 ) ) ;
#619=CARTESIAN_POINT ( 'NONE',  ( 203.1705638993064156, 278.7452560544191442, -15.08126533799095093 ) ) ;
#621=CARTESIAN_POINT ( 'NONE',  ( 192.6159067191336476, 296.6392389330721926, 11.36185169173896448 ) ) ;
#623=CARTESIAN_POINT ( 'NONE',  ( 198.6444633007815810, 284.5846922512318997, -17.80363864581810418 ) ) ;
#624=ORIENTED_EDGE ( 'NONE', *, *, #90672, .T. ) ;
#625=CARTESIAN_POINT ( 'NONE',  ( 162.9383752892161397, 248.4294508267893491, -11.25953730674605957 ) ) ;
#628=CARTESIAN_POINT ( 'NONE',  ( 206.3009434829942279, 272.9081483067511158, 8.547891559723822752 ) ) ;
#629=CARTESIAN_POINT ( 'NONE',  ( 124.8827946268633298, 255.1589784336661069, -6.496448406907676862E-16 ) ) ;
#630=CARTESIAN_POINT ( 'NONE',  ( 190.2913651263166628, 294.6875229615724265, -12.30047797060472803 ) ) ;
#632=CARTESIAN_POINT ( 'NONE',  ( 196.2609093297512857, 290.7131288316392670, 16.03897268885959448 ) ) ;
#635=CARTESIAN_POINT ( 'NONE',  ( 57.73936995728981714, 194.9548013555410080, -4.594050593750042211 ) ) ;
#637=ORIENTED_EDGE ( 'NONE', *, *, #87810, .T. ) ;
#640=CARTESIAN_POINT ( 'NONE',  ( 21.31191609055706593, 183.1115022471902591, 10.00000000000009592 ) ) ;
#641=CARTESIAN_POINT ( 'NONE',  ( 174.4676371989123140, 262.1820789082375995, 14.34376349448554144 ) ) ;
#643=CARTESIAN_POINT ( 'NONE',  ( 154.9528145190857344, 262.2608478075840708, -17.26679351315302213 ) ) ;
#644=CARTESIAN_POINT ( 'NONE',  ( 178.2689201652922861, 261.3463682195790625, 12.89043557696258979 ) ) ;
#645=CARTESIAN_POINT ( 'NONE',  ( 100.3908607700756619, 238.7677522451419065, -5.000000000000047962 ) ) ;
#647=ORIENTED_EDGE ( 'NONE', *, *, #96875, .T. ) ;
#648=CARTESIAN_POINT ( 'NONE',  ( 202.6070187115982719, 279.7213449518906145, 15.56322169823762280 ) ) ;
#650=CARTESIAN_POINT ( 'NONE',  ( 29.48529115882250551, 178.6423013555409796, -4.594050593750043987 ) ) ;
#655=CARTESIAN_POINT ( 'NONE',  ( 174.4019427205360842, 268.6781143085732992, 17.66204038257215458 ) ) ;
#656=CARTESIAN_POINT ( 'NONE',  ( 67.50895872190925218, 209.7833772461660544, -9.188101187500095079 ) ) ;
#657=CARTESIAN_POINT ( 'NONE',  ( 164.4817765375028102, 245.7562014482918755, -6.334578229142199035 ) ) ;
#659=CARTESIAN_POINT ( 'NONE',  ( 45.37789370152431445, 208.5530062829863027, -4.648177544792955347E-16 ) ) ;
#661=ORIENTED_EDGE ( 'NONE', *, *, #87113, .F. ) ;
#663=CARTESIAN_POINT ( 'NONE',  ( 164.0312634879877294, 268.4089602666911105, 16.55773273759760400 ) ) ;
#664=CARTESIAN_POINT ( 'NONE',  ( 22.68312297988236992, 197.2365022471903444, 2.944929066748280225E-16 ) ) ;
#665=CARTESIAN_POINT ( 'NONE',  ( 163.1008115941903895, 248.1481028935802442, 11.25332017433677834 ) ) ;
#666=CARTESIAN_POINT ( 'NONE',  ( -4.614459115189767147, 158.9548013555409796, -4.594050593750042211 ) ) ;
#668=CARTESIAN_POINT ( 'NONE',  ( 164.4039089034689027, 259.8557547647841943, -16.35869283172417710 ) ) ;
#669=CARTESIAN_POINT ( 'NONE',  ( 170.1430290936755227, 263.5485301713791841, 15.83574950237116141 ) ) ;
#671=CARTESIAN_POINT ( 'NONE',  ( 185.5569508314414406, 260.4628387231232409, 6.337775543338724837 ) ) ;
#672=CARTESIAN_POINT ( 'NONE',  ( 206.0691053506789387, 273.7248349927971844, 11.70564474658248422 ) ) ;
#674=CARTESIAN_POINT ( 'NONE',  ( 183.8314122675164981, 256.5947891462430448, -1.876126292579811894 ) ) ;
#677=CARTESIAN_POINT ( 'NONE',  ( 135.2899281637556896, 260.4637435831425023, 2.679491924311251605 ) ) ;
#679=CARTESIAN_POINT ( 'NONE',  ( 181.7952694153465245, 287.8449457046345970, 13.56394578825295305 ) ) ;
#680=CARTESIAN_POINT ( 'NONE',  ( 196.2127072044743272, 290.0836373517121274, 16.37479000986071398 ) ) ;
#682=ORIENTED_EDGE ( 'NONE', *, *, #27159, .T. ) ;
#683=CARTESIAN_POINT ( 'NONE',  ( 160.3856437025401931, 252.8509116329982191, 16.19741910828728493 ) ) ;
#684=CARTESIAN_POINT ( 'NONE',  ( 157.3029956111992362, 258.1902147490555421, -18.22269824972649843 ) ) ;
#686=CARTESIAN_POINT ( 'NONE',  ( 207.6477529416552557, 270.9905371579805546, 7.447146952410988341 ) ) ;
#687=CARTESIAN_POINT ( 'NONE',  ( 185.2057911854575138, 276.7165103822673586, 17.80337911918299909 ) ) ;
#688=CARTESIAN_POINT ( 'NONE',  ( 163.0056347026689707, 248.3129541054019569, -11.27842346302751508 ) ) ;
#689=CARTESIAN_POINT ( 'NONE',  ( 153.0444155045374544, 265.5662918618958201, -16.15173036748435109 ) ) ;
#690=VERTEX_POINT ( 'NONE', #63350 ) ;
#691=CARTESIAN_POINT ( 'NONE',  ( 190.8932553518572206, 280.9403775647153338, 16.64665765453319679 ) ) ;
#699=CARTESIAN_POINT ( 'NONE',  ( 149.7072529793668707, 271.3464269086063041, -11.98883662638834657 ) ) ;
#702=CARTESIAN_POINT ( 'NONE',  ( 200.6129772034685175, 283.1751261563724142, 18.36811917402039640 ) ) ;
#704=CARTESIAN_POINT ( 'NONE',  ( 151.2591548104722108, 274.8925958778597192, -8.633445779095369588 ) ) ;
#705=VERTEX_POINT ( 'NONE', #23335 ) ;
#711=ORIENTED_EDGE ( 'NONE', *, *, #24354, .F. ) ;
#712=CARTESIAN_POINT ( 'NONE',  ( 207.5215400641004351, 271.2091442744748520, 2.886080616848571534 ) ) ;
#713=CARTESIAN_POINT ( 'NONE',  ( 198.7045056313791633, 284.4806958840320021, 17.79791830837532274 ) ) ;
#715=CARTESIAN_POINT ( 'NONE',  ( 148.3025927079438304, 273.7793698660844939, -8.046026357031887954 ) ) ;
#716=CARTESIAN_POINT ( 'NONE',  ( 175.1828650004762267, 290.0278138422783627, 6.199890812727518075 ) ) ;
#721=CARTESIAN_POINT ( 'NONE',  ( 198.3666213183647926, 277.3917214242281375, -15.34159264812408452 ) ) ;
#723=CARTESIAN_POINT ( 'NONE',  ( 193.0512205562391159, 275.6825563886401369, -16.88465587640301280 ) ) ;
#725=CARTESIAN_POINT ( 'NONE',  ( 191.1159732739488106, 299.6244194819818745, 5.816361631709846769 ) ) ;
#727=CARTESIAN_POINT ( 'NONE',  ( 159.4491226731523454, 254.4730136382542582, -15.39140229921534520 ) ) ;
#732=CARTESIAN_POINT ( 'NONE',  ( 200.4116241316243645, 283.5238799070667142, 18.37703770054986663 ) ) ;
#734=VERTEX_POINT ( 'NONE', #24355 ) ;
#735=CARTESIAN_POINT ( 'NONE',  ( 193.8687075137383999, 294.8565439189318340, -14.51137100490168486 ) ) ;
#736=LINE ( 'NONE', #24036, #27376 ) ;
#737=EDGE_CURVE ( 'NONE', #53287, #48247, #79529, .T. ) ;
#738=CARTESIAN_POINT ( 'NONE',  ( 15.88121511744428282, 166.6427522451417644, 1.119607411625061291E-15 ) ) ;
#739=CARTESIAN_POINT ( 'NONE',  ( 85.91165145656357538, 232.6589784336661353, -6.496448406907676862E-16 ) ) ;
#741=CYLINDRICAL_SURFACE ( 'NONE', #85952, 17.82106496071139645 ) ;
#742=CARTESIAN_POINT ( 'NONE',  ( 166.9577072416738019, 278.1838835069849551, -13.42963054343457863 ) ) ;
#744=CARTESIAN_POINT ( 'NONE',  ( 9.079046938504149011, 185.2369531367911293, -4.594050593750048428 ) ) ;
#746=CARTESIAN_POINT ( 'NONE',  ( 161.4025183475459073, 251.0896330829197041, 14.50747140106038735 ) ) ;
#748=UNCERTAINTY_MEASURE_WITH_UNIT (LENGTH_MEASURE( 1.000000000000000082E-05 ), #95770, 'distance_accuracy_value', 'NONE');
#751=CARTESIAN_POINT ( 'NONE',  ( 197.6375537770108792, 265.0377995068387804, -2.979366280021975122 ) ) ;
#753=CARTESIAN_POINT ( 'NONE',  ( 202.6448056009234904, 279.6558961397194594, -17.13147024041661126 ) ) ;
#754=( BOUNDED_CURVE ( )  B_SPLINE_CURVE ( 2, ( #51590, #82036, #12612, #50581, #74420, #81531, #96236, #65295, #83027 ),
 .UNSPECIFIED., .F., .T. ) 
 B_SPLINE_CURVE_WITH_KNOTS ( ( 3, 2, 2, 2, 3 ),
 ( 0.3266129032258064391, 0.3279569892473118142, 0.3306451612903225645, 0.3333333333333333148, 0.3346774193548386900 ),
 .UNSPECIFIED. ) 
 CURVE ( )  GEOMETRIC_REPRESENTATION_ITEM ( )  RATIONAL_B_SPLINE_CURVE ( ( 0.9330127018922194093, 0.9330127018922194093, 1.000000000000000000, 0.8660254037844387076, 1.000000000000000000, 0.8660254037844387076, 1.000000000000000000, 0.9330127018922194093, 0.9330127018922194093 ) ) 
 REPRESENTATION_ITEM ( '' )  );
#755=CARTESIAN_POINT ( 'NONE',  ( 113.3812418268423414, 226.2677522451417929, -5.000000000000041744 ) ) ;
#757=CARTESIAN_POINT ( 'NONE',  ( 24.36989474801440636, 191.0024278399161233, 9.188101187500095079 ) ) ;
#758=CARTESIAN_POINT ( 'NONE',  ( 197.6585140451727511, 276.4987611936116423, 15.20518655683599896 ) ) ;
#759=VERTEX_POINT ( 'NONE', #25344 ) ;
#761=CARTESIAN_POINT ( 'NONE',  ( 182.6096789788834087, 260.7894769810658318, -10.76918927552311622 ) ) ;
#765=CARTESIAN_POINT ( 'NONE',  ( 59.77787777531585789, 211.9865022471903160, 10.00000000000009415 ) ) ;
#766=CARTESIAN_POINT ( 'NONE',  ( 186.1370921618058674, 283.3846817430978149, 17.26256540491417368 ) ) ;
#767=CARTESIAN_POINT ( 'NONE',  ( 194.2389208611690492, 294.2153155915419802, -15.75132567904764791 ) ) ;
#769=CARTESIAN_POINT ( 'NONE',  ( 192.5078993207126814, 265.1470235889372589, 7.748826881858292381 ) ) ;
#770=CARTESIAN_POINT ( 'NONE',  ( 168.9579038699606315, 279.3139280689009070, 15.08363371378442608 ) ) ;
#772=CARTESIAN_POINT ( 'NONE',  ( 146.8859094598974480, 276.2331372299326517, -0.7994986043261681496 ) ) ;
#773=CARTESIAN_POINT ( 'NONE',  ( 148.3997536239841679, 273.6110822229926498, 8.713694244701960301 ) ) ;
#776=CARTESIAN_POINT ( 'NONE',  ( 188.7267243920021542, 295.1910411013678299, 11.79826141631466463 ) ) ;
#777=CARTESIAN_POINT ( 'NONE',  ( 9.548404355818409073, 182.9865022471903160, -10.00000000000009592 ) ) ;
#778=CARTESIAN_POINT ( 'NONE',  ( 115.8441751185107478, 231.5643266524159856, 9.188101187500095079 ) ) ;
#780=CARTESIAN_POINT ( 'NONE',  ( -13.83428154636143503, 169.4865022471903160, -10.00000000000009592 ) ) ;
#781=EDGE_CURVE ( 'NONE', #55876, #18677, #11467, .T. ) ;
#784=CARTESIAN_POINT ( 'NONE',  ( 195.1938325246360364, 279.1028983798199761, 16.30285934901647238 ) ) ;
#785=CARTESIAN_POINT ( 'NONE',  ( 150.4341052900205682, 270.0874817769553147, -15.18648472748443368 ) ) ;
#786=CARTESIAN_POINT ( 'NONE',  ( 190.4856830296963039, 261.1280128588217622, -4.649057565560686278 ) ) ;
#787=CARTESIAN_POINT ( 'NONE',  ( 149.8050492866161392, 271.5723974896224604, -11.69608657949948061 ) ) ;
#788=CARTESIAN_POINT ( 'NONE',  ( 113.8864233123832577, 229.8927522451418213, 10.00000000000009948 ) ) ;
#789=CARTESIAN_POINT ( 'NONE',  ( 132.0211419364472363, 235.4824982072973683, 3.021315404115420679E-15 ) ) ;
#792=CARTESIAN_POINT ( 'NONE',  ( 192.9767279769529864, 266.9258724154651645, 11.43531444180136347 ) ) ;
#793=CARTESIAN_POINT ( 'NONE',  ( 178.9040352719350722, 280.8175526911114162, 16.40818605171233813 ) ) ;
#794=CARTESIAN_POINT ( 'NONE',  ( 199.8193483442802005, 270.0841922650383822, 9.248294916842718649 ) ) ;
#799=( GEOMETRIC_REPRESENTATION_CONTEXT ( 3 ) GLOBAL_UNCERTAINTY_ASSIGNED_CONTEXT ( ( #748 ) ) GLOBAL_UNIT_ASSIGNED_CONTEXT ( ( #95770, #27323, #35406 ) ) REPRESENTATION_CONTEXT ( 'NONE', 'WORKASPACE' ) );
#800=CARTESIAN_POINT ( 'NONE',  ( 182.6461938784695747, 263.4785373306806378, -13.90739657620127190 ) ) ;
#804=CARTESIAN_POINT ( 'NONE',  ( 187.3992198486085385, 278.8856332353482230, 17.56695100383910102 ) ) ;
#805=B_SPLINE_SURFACE_WITH_KNOTS ( 'NONE', 3, 1, ( 
 ( #39651, #16380 ),
 ( #76687, #85852 ),
 ( #46781, #683 ),
 ( #77179, #92421 ),
 ( #60970, #69577 ),
 ( #53858, #21983 ),
 ( #84821, #76212 ),
 ( #60465, #22971 ),
 ( #6788, #91420 ),
 ( #99503, #8286 ),
 ( #39152, #100002 ),
 ( #47271, #15359 ),
 ( #30586, #31068 ),
 ( #84329, #70065 ),
 ( #62455, #93422 ),
 ( #23973, #61959 ),
 ( #61473, #54353 ),
 ( #52877, #83828 ),
 ( #45764, #91930 ),
 ( #15871, #22485 ),
 ( #14875, #95446 ),
 ( #94418, #33589 ),
 ( #55848, #40665 ),
 ( #9805, #47760 ),
 ( #16875, #40161 ),
 ( #71602, #71103 ),
 ( #86843, #78699 ),
 ( #17899, #79233 ),
 ( #2698, #1701 ),
 ( #87852, #56868 ),
 ( #72610, #17378 ),
 ( #24971, #25997 ),
 ( #64485, #2198 ),
 ( #33081, #63481 ) ),
 .UNSPECIFIED., .T., .F., .F.,
 ( 4, 2, 2, 2, 2, 2, 2, 2, 2, 2, 2, 2, 2, 2, 2, 2, 4 ),
 ( 2, 2 ),
 ( 0.000000000000000000, 0.06250000000000000000, 0.1250000000000000000, 0.1875000000000000000, 0.2500000000000000000, 0.3125000000000000000, 0.3750000000000000000, 0.4375000000000000000, 0.5000000000000000000, 0.5625000000000000000, 0.6250000000000000000, 0.6875000000000000000, 0.7500000000000000000, 0.8125000000000000000, 0.8750000000000000000, 0.9375000000000000000, 1.000000000000000000 ),
 ( 0.000000000000000000, 1.000000000000000000 ),
 .UNSPECIFIED. ) ;
#807=ORIENTED_EDGE ( 'NONE', *, *, #26966, .F. ) ;
#808=B_SPLINE_CURVE_WITH_KNOTS ( 'NONE', 3,
 ( #93246, #8616, #85674, #37500, #16211, #70408, #16709, #68407, #29915, #60785, #91750, #22313, #53216, #84167, #2530, #71426, #19242, #65308, #78530, #33412, #95269, #18222, #32901, #2016, #17202, #49603, #70927, #56193, #64818, #94250, #49116, #80053, #3531, #94743, #1532, #48624, #10620, #55682, #86669, #41498, #42006, #32413, #63308, #72439, #3045, #48104, #26320, #34408, #79047, #57194 ),
 .UNSPECIFIED., .F., .F.,
 ( 4, 2, 2, 2, 2, 2, 2, 2, 2, 2, 2, 2, 2, 2, 2, 2, 2, 2, 2, 2, 2, 2, 2, 2, 4 ),
 ( 0.0001456936475078258835, 0.001156712366743216369, 0.001662221726360948787, 0.001788599066265381945, 0.001914976406169814887, 0.002041353746074247612, 0.002167731085978680770, 0.002420485765787583950, 0.002673240445596487564, 0.003178749805214391069, 0.004189768524450103969, 0.005200787243685817303, 0.005706296603303709532, 0.005959051283112655646, 0.006211805962921601761, 0.006274994632873879055, 0.006338183302826156350, 0.006401371972778433644, 0.006464560642730710939, 0.006717315322539938946, 0.007222824682158399297, 0.007475579361967629038, 0.007728334041776859648, 0.007981088721586090257, 0.008233843401395319131 ),
 .UNSPECIFIED. ) ;
#810=CARTESIAN_POINT ( 'NONE',  ( 147.8819534105757043, 274.5079385007862811, -9.338341377131436971 ) ) ;
#811=CARTESIAN_POINT ( 'NONE',  ( 156.7854950622006527, 259.0865519928661911, 18.17819951099994213 ) ) ;
#815=CARTESIAN_POINT ( 'NONE',  ( 205.9381235462180655, 273.9517021329910449, 12.32333910181129788 ) ) ;
#817=CARTESIAN_POINT ( 'NONE',  ( -22.42236680055709641, 157.8615022471902591, 0.000000000000000000 ) ) ;
#818=B_SPLINE_CURVE_WITH_KNOTS ( 'NONE', 3,
 ( #71729, #81351, #33203, #2834, #64103, #49904, #57488, #95053, #56499, #27618, #95568, #64613, #80862, #4294, #35196, #25614, #18022, #66102, #26113, #40781, #56991, #58484, #89460, #87973, #20015, #49403, #19032, #80351, #10921, #3332, #34210, #42288, #51391, #53382, #51903, #75711, #21021, #58967, #98011, #29109, #45282, #82844, #89937, #83331, #99507, #66599, #13415, #74728, #12417, #5793, #44284, #52388, #6792, #43284 ),
 .UNSPECIFIED., .F., .F.,
 ( 4, 2, 2, 2, 2, 2, 2, 2, 2, 2, 2, 2, 2, 2, 2, 2, 2, 2, 2, 2, 2, 2, 2, 2, 2, 2, 4 ),
 ( 0.0007884837803721018784, 0.0009911425274972654638, 0.001092471901059910953, 0.001193801274622556009, 0.001295130648185201499, 0.001396460021747846555, 0.001599118768873064025, 0.002004436263123498315, 0.002409753757373932822, 0.003220388745874802703, 0.004031023734375672150, 0.004841658722876542899, 0.005246976217126939242, 0.005449634964252138281, 0.005550964337814701804, 0.005601629024595986168, 0.005652293711377270533, 0.005702958398158554897, 0.005753623084939839261, 0.005854952458502437479, 0.006057611205627632181, 0.006260269952752827750, 0.006462928699878023320, 0.006665587447003218889, 0.006868246194128413591, 0.007070904941253609161, 0.007273563688378803863 ),
 .UNSPECIFIED. ) ;
#821=CARTESIAN_POINT ( 'NONE',  ( 121.6288370910339864, 229.4824982072973398, 3.021315404115420679E-15 ) ) ;
#823=ORIENTED_EDGE ( 'NONE', *, *, #34079, .T. ) ;
#825=CARTESIAN_POINT ( 'NONE',  ( 175.1988826894065312, 258.4881829066944192, 12.95490576022639928 ) ) ;
#828=ORIENTED_EDGE ( 'NONE', *, *, #42263, .F. ) ;
#829=CARTESIAN_POINT ( 'NONE',  ( 169.4845393771928173, 269.1455624229661225, 17.04989631985375453 ) ) ;
#834=CARTESIAN_POINT ( 'NONE',  ( 190.0226014859668453, 301.5181949703289774, 3.835066345245774500 ) ) ;
#835=CARTESIAN_POINT ( 'NONE',  ( 195.0987748510856647, 262.8777892843546056, 0.5876111608821336096 ) ) ;
#836=CARTESIAN_POINT ( 'NONE',  ( 171.4762298308916968, 250.4071321773194256, -5.778962900379556622 ) ) ;
#837=CARTESIAN_POINT ( 'NONE',  ( 44.24123536260515976, 207.8967562850346837, -4.648177544792955347E-16 ) ) ;
#838=CARTESIAN_POINT ( 'NONE',  ( 202.6998011068605194, 275.8073517492424571, -14.46034972092035531 ) ) ;
#839=CARTESIAN_POINT ( 'NONE',  ( 127.4544149619371609, 235.2048013555409796, 4.594050593750051981 ) ) ;
#842=ORIENTED_EDGE ( 'NONE', *, *, #99346, .F. ) ;
#846=ORIENTED_EDGE ( 'NONE', *, *, #5709, .T. ) ;
#847=CARTESIAN_POINT ( 'NONE',  ( 203.6154480045567254, 276.2142138887539886, 13.33356564682453893 ) ) ;
#848=CARTESIAN_POINT ( 'NONE',  ( 177.5663600863603904, 253.5925114390991553, 1.368723437027021594 ) ) ;
#850=CARTESIAN_POINT ( 'NONE',  ( 165.4781454232152953, 246.0304399151612245, -2.837517270351797016 ) ) ;
#851=DIRECTION ( 'NONE',  ( -0.8660254037844359321, -0.5000000000000051070, -0.000000000000000000 ) ) ;
#853=CARTESIAN_POINT ( 'NONE',  ( 153.2283961777204695, 265.2476279883323400, -17.66880461074566000 ) ) ;
#854=CARTESIAN_POINT ( 'NONE',  ( 174.2107584283791937, 288.2982359596526294, -10.05413864759180775 ) ) ;
#855=CARTESIAN_POINT ( 'NONE',  ( 173.2798715285074991, 281.8114527337138497, 15.08241540710736750 ) ) ;
#858=B_SPLINE_CURVE_WITH_KNOTS ( 'NONE', 3,
 ( #9139, #88196, #40012, #86692 ),
 .UNSPECIFIED., .F., .F.,
 ( 4, 4 ),
 ( 0.01500120671162206987, 0.02374886763876108906 ),
 .UNSPECIFIED. ) ;
#859=CARTESIAN_POINT ( 'NONE',  ( 194.9385458806846430, 293.0035295114944347, -15.70518692812489192 ) ) ;
#860=CARTESIAN_POINT ( 'NONE',  ( 152.7606255379852485, 273.9024957846719417, 12.20944343624798201 ) ) ;
#862=CARTESIAN_POINT ( 'NONE',  ( 190.7462944391682527, 267.5255109591399787, -12.03952247946680565 ) ) ;
#863=EDGE_CURVE ( 'NONE', #22269, #42801, #98193, .T. ) ;
#864=CARTESIAN_POINT ( 'NONE',  ( 159.4675140783279801, 279.0638630585228270, 10.93816975955046544 ) ) ;
#865=CARTESIAN_POINT ( 'NONE',  ( 194.1886218511698985, 264.4780071475063892, 4.425547236910387205 ) ) ;
#867=CARTESIAN_POINT ( 'NONE',  ( 6.290725127440143893, 185.9860189848785126, -2.679491924311252493 ) ) ;
#868=CARTESIAN_POINT ( 'NONE',  ( 164.7214155129279902, 283.9927988242368428, -6.830869372685311802 ) ) ;
#869=CARTESIAN_POINT ( 'NONE',  ( 160.8351940225509793, 281.7148115565385638, 6.356997412616704146 ) ) ;
#870=CARTESIAN_POINT ( 'NONE',  ( 200.6680263064462792, 283.0797783131037022, -17.21821073473145347 ) ) ;
#872=CARTESIAN_POINT ( 'NONE',  ( 204.7752845747214110, 272.8046689790122628, -9.561809439462201965 ) ) ;
#873=CARTESIAN_POINT ( 'NONE',  ( 190.3857086002435324, 265.7052621535535195, -12.18680232436801170 ) ) ;
#874=CARTESIAN_POINT ( 'NONE',  ( 188.8588437571793008, 263.8686956098205769, -9.115312588253704718 ) ) ;
#875=CARTESIAN_POINT ( 'NONE',  ( 191.8098186646358272, 275.3759357196170185, -15.83273902380079257 ) ) ;
#876=CARTESIAN_POINT ( 'NONE',  ( 33.29424590502123493, 178.4824982072973683, 3.021315404115420679E-15 ) ) ;
#878=CARTESIAN_POINT ( 'NONE',  ( 184.9851449735395192, 296.8426758125457354, -4.344182660386399775 ) ) ;
#881=CARTESIAN_POINT ( 'NONE',  ( 153.1745822862813498, 265.3408363824576668, 16.18092354043443493 ) ) ;
#884=CARTESIAN_POINT ( 'NONE',  ( 34.75566377745538205, 179.3262482093457493, 3.021315404115420679E-15 ) ) ;
#885=CARTESIAN_POINT ( 'NONE',  ( -2.801305199957352166, 163.0643266524160140, -9.188101187500093303 ) ) ;
#886=CARTESIAN_POINT ( 'NONE',  ( 88.99704050542813150, 228.3149278399160664, 9.188101187500093303 ) ) ;
#888=CARTESIAN_POINT ( 'NONE',  ( 147.2567621633200474, 275.5908015054806128, -3.647191014543873955 ) ) ;
#889=CARTESIAN_POINT ( 'NONE',  ( 187.7710022618638277, 277.0665775429750397, -17.72351784843695555 ) ) ;
#894=CARTESIAN_POINT ( 'NONE',  ( 158.3585752585947262, 263.3710999200782226, 17.79390465796247156 ) ) ;
#898=CARTESIAN_POINT ( 'NONE',  ( 161.8357418099448353, 250.3392680350139869, 14.17480975207680061 ) ) ;
#900=CARTESIAN_POINT ( 'NONE',  ( 169.4976558230340231, 251.7484151835147657, -9.940267045083754027 ) ) ;
#901=CARTESIAN_POINT ( 'NONE',  ( 161.8566033897550085, 252.0880471315855686, 14.23877116480228544 ) ) ;
#902=CARTESIAN_POINT ( 'NONE',  ( 157.6335212189247557, 257.6177276032722716, 16.76495363836117036 ) ) ;
#903=CARTESIAN_POINT ( 'NONE',  ( -22.42236680055709641, 157.8615022471902591, 0.000000000000000000 ) ) ;
#906=CARTESIAN_POINT ( 'NONE',  ( 37.36027580478099708, 198.5024278399160664, 9.188101187500095079 ) ) ;
#907=CARTESIAN_POINT ( 'NONE',  ( 78.84873917453550973, 207.1423013555409796, -4.594050593750043987 ) ) ;
#911=CARTESIAN_POINT ( 'NONE',  ( 167.2464745708191458, 259.8228882802526982, 16.05418551386606651 ) ) ;
#912=CARTESIAN_POINT ( 'NONE',  ( 147.5623555321158165, 249.8768266524159856, -9.188101187500091527 ) ) ;
#917=EDGE_CURVE ( 'NONE', #66866, #86172, #60293, .T. ) ;
#919=CARTESIAN_POINT ( 'NONE',  ( 150.7133245577828689, 269.6038598187387834, -14.58664962216439598 ) ) ;
#920=CARTESIAN_POINT ( 'NONE',  ( 196.2630260332681189, 290.7094625936034049, -17.43112004684450866 ) ) ;
#922=CARTESIAN_POINT ( 'NONE',  ( 68.13167480270307408, 200.9548013555409796, -4.594050593750042211 ) ) ;
#924=CARTESIAN_POINT ( 'NONE',  ( 203.1044072055706806, 278.8598428092302584, -16.67109798570195878 ) ) ;
#925=CARTESIAN_POINT ( 'NONE',  ( 198.5966822647444587, 286.6674514332866579, 17.25284514431582750 ) ) ;
#927=CARTESIAN_POINT ( 'NONE',  ( 153.3890631498689743, 264.9693446294729711, 16.84838431772464773 ) ) ;
#928=ADVANCED_FACE ( 'NONE', ( #98768 ), #28850, .T. ) ;
#929=AXIS2_PLACEMENT_3D ( 'NONE', #31113, #92953, #30634 ) ;
#931=CARTESIAN_POINT ( 'NONE',  ( 103.0791479645378104, 236.9865022471902876, -10.00000000000009415 ) ) ;
#932=CARTESIAN_POINT ( 'NONE',  ( 200.8769374536528858, 282.7179335918746688, 17.26928237494566787 ) ) ;
#933=CARTESIAN_POINT ( 'NONE',  ( 164.4781197247689306, 245.7625352337404649, -1.511762618280499515 ) ) ;
#936=CARTESIAN_POINT ( 'NONE',  ( 184.6950506501621021, 271.1962962339267165, 16.22049766843658603 ) ) ;
#938=CARTESIAN_POINT ( 'NONE',  ( 206.6912923161529818, 272.6471755567893638, -9.325620632947922317 ) ) ;
#939=CARTESIAN_POINT ( 'NONE',  ( 193.9232833982383113, 293.2909642926495621, 15.00674244883364139 ) ) ;
#941=VERTEX_POINT ( 'NONE', #98260 ) ;
#945=CARTESIAN_POINT ( 'NONE',  ( 194.3011251241114508, 294.1075746476782342, -14.76047579547631905 ) ) ;
#947=VERTEX_POINT ( 'NONE', #91178 ) ;
#951=CARTESIAN_POINT ( 'NONE',  ( 30.24280306353621128, 178.2677522451417929, -5.000000000000041744 ) ) ;
#955=CARTESIAN_POINT ( 'NONE',  ( 159.7132918459648181, 254.0154592091499239, -16.90058287995827158 ) ) ;
#957=ORIENTED_EDGE ( 'NONE', *, *, #62143, .T. ) ;
#958=CARTESIAN_POINT ( 'NONE',  ( 174.8110114269580606, 286.1294775324029160, 11.21431686804888983 ) ) ;
#959=CARTESIAN_POINT ( 'NONE',  ( 163.2766929973646484, 283.7647176037089594, -3.009406773168611604 ) ) ;
#962=CARTESIAN_POINT ( 'NONE',  ( 194.1493756275458793, 294.3704124857528655, 13.94613522129020744 ) ) ;
#964=CARTESIAN_POINT ( 'NONE',  ( 157.1539462478114615, 258.4483758192793061, -17.96006278656275867 ) ) ;
#965=CARTESIAN_POINT ( 'NONE',  ( 138.6852480475602931, 257.0024278399160949, 9.188101187500095079 ) ) ;
#966=CARTESIAN_POINT ( 'NONE',  ( 206.3049127377101968, 270.5357785998967870, 2.445900227168405383 ) ) ;
#967=CARTESIAN_POINT ( 'NONE',  ( 179.2020837305335306, 258.4857288146945962, 9.693322143454775386 ) ) ;
#968=CARTESIAN_POINT ( 'NONE',  ( 80.33678646758374953, 223.3149278399160949, -9.188101187500095079 ) ) ;
#970=CARTESIAN_POINT ( 'NONE',  ( 151.4327733764141612, 268.3577379114237829, 14.90862905801242100 ) ) ;
#972=EDGE_LOOP ( 'NONE', ( #1245, #99515, #43357, #14062, #15878 ) ) ;
#973=CARTESIAN_POINT ( 'NONE',  ( 157.2072737763903945, 258.3560098303381096, -16.87862088075553402 ) ) ;
#975=ORIENTED_EDGE ( 'NONE', *, *, #37146, .F. ) ;
#978=CARTESIAN_POINT ( 'NONE',  ( 146.6138605399200117, 276.7043397814778132, -0.5394499176159462950 ) ) ;
#979=CARTESIAN_POINT ( 'NONE',  ( 149.3545991938273971, 273.9572411826421217, -10.14243178476390028 ) ) ;
#982=CARTESIAN_POINT ( 'NONE',  ( 90.35072584248885619, 210.7202760586659736, -5.415160957724236172E-17 ) ) ;
#983=VERTEX_POINT ( 'NONE', #22234 ) ;
#985=CARTESIAN_POINT ( 'NONE',  ( 112.9278751967105450, 247.5530062829863311, -4.648177544792955347E-16 ) ) ;
#986=CARTESIAN_POINT ( 'NONE',  ( 161.2518619042614034, 251.3505776971759360, -13.56582882383257349 ) ) ;
#990=CARTESIAN_POINT ( 'NONE',  ( 183.6463619201787481, 275.7299020814296568, 17.02459170948687373 ) ) ;
#993=CARTESIAN_POINT ( 'NONE',  ( 155.8152618860606538, 260.7670451491295012, 0.000000000000000000 ) ) ;
#998=CARTESIAN_POINT ( 'NONE',  ( 185.2745384195171141, 260.2690603060960370, 6.274088207539249673 ) ) ;
#1000=CARTESIAN_POINT ( 'NONE',  ( 200.7694952279801157, 282.9040289856181403, -17.94628235092568502 ) ) ;
#1002=VECTOR ( 'NONE', #51820, 1000.000000000000000 ) ;
#1004=EDGE_CURVE ( 'NONE', #12032, #15116, #42515, .T. ) ;
#1007=CARTESIAN_POINT ( 'NONE',  ( 186.6806167748573273, 293.5666024053780916, -12.22359308779079079 ) ) ;
#1008=CARTESIAN_POINT ( 'NONE',  ( 200.8828793852583203, 282.7076418644388696, 17.90302398138411633 ) ) ;
#1010=CARTESIAN_POINT ( 'NONE',  ( 169.7276834213985239, 251.0855122629868106, 6.971127372306837877 ) ) ;
#1012=CARTESIAN_POINT ( 'NONE',  ( 156.9258225138436842, 272.6371026541438596, 14.45601229042061675 ) ) ;
#1013=CARTESIAN_POINT ( 'NONE',  ( 162.7561251957091031, 248.7451172484279027, 11.07313294959361194 ) ) ;
#1014=B_SPLINE_CURVE_WITH_KNOTS ( 'NONE', 3,
 ( #94462, #9852, #87416, #64532 ),
 .UNSPECIFIED., .F., .F.,
 ( 4, 4 ),
 ( 0.02269137219855666548, 0.03190570623119325794 ),
 .UNSPECIFIED. ) ;
#1017=CARTESIAN_POINT ( 'NONE',  ( 194.4889937320412230, 293.7821766735966662, 14.99892588346621380 ) ) ;
#1019=CARTESIAN_POINT ( 'NONE',  ( 200.1528453280087945, 282.4639923692292314, -16.67548112269998128 ) ) ;
#1021=CARTESIAN_POINT ( 'NONE',  ( 168.3381296007061678, 273.6507282997970947, 16.34367694402899573 ) ) ;
#1025=CARTESIAN_POINT ( 'NONE',  ( 188.8970709661001592, 261.1830301768237632, 2.866754512114129128 ) ) ;
#1026=CARTESIAN_POINT ( 'NONE',  ( 194.9663593620817892, 265.9656423931795644, -7.350908074652497071 ) ) ;
#1028=CARTESIAN_POINT ( 'NONE',  ( -6.184650803196579893, 176.4244531367911293, -4.594050593750046652 ) ) ;
#1029=CARTESIAN_POINT ( 'NONE',  ( 154.6982851380984130, 273.6571292083216349, -13.42362762759460892 ) ) ;
#1031=CARTESIAN_POINT ( 'NONE',  ( 161.1018488054811542, 253.0685122771756994, -14.87691902254530696 ) ) ;
#1032=ADVANCED_FACE ( 'NONE', ( #74961 ), #37422, .T. ) ;
#1034=CARTESIAN_POINT ( 'NONE',  ( 164.6063343576543048, 274.4739709976624908, 16.17759516952312637 ) ) ;
#1035=CARTESIAN_POINT ( 'NONE',  ( 22.47598482088345406, 171.5327760586659451, 1.948934522072302763E-15 ) ) ;
#1036=CARTESIAN_POINT ( 'NONE',  ( 71.24475614018626857, 200.3932355074535963, -2.679491924311248496 ) ) ;
#1038=CARTESIAN_POINT ( 'NONE',  ( 129.9981042655041392, 235.8615022471901739, 5.000000000000051514 ) ) ;
#1039=B_SPLINE_CURVE_WITH_KNOTS ( 'NONE', 3,
 ( #8432, #70727, #7943, #24129, #38316, #68726, #92091, #16026, #78345, #39300, #69722, #86490, #100153, #85996 ),
 .UNSPECIFIED., .F., .F.,
 ( 4, 2, 2, 2, 2, 2, 4 ),
 ( 0.000000000000000000, 0.0004397231552390210105, 0.0008794463104780420211, 0.001099307888097552418, 0.001319169465717063032, 0.001539031043336573645, 0.001758892620956084042 ),
 .UNSPECIFIED. ) ;
#1040=CARTESIAN_POINT ( 'NONE',  ( 173.3440299427151388, 273.3511298303828312, -17.59202441768653102 ) ) ;
#1041=CARTESIAN_POINT ( 'NONE',  ( 13.97105408662886461, 167.3262482093458061, -5.229199737892075682E-14 ) ) ;
#1043=DIRECTION ( 'NONE',  ( 0.8660254037844395958, 0.4999999999999985567, 0.000000000000000000 ) ) ;
#1044=CARTESIAN_POINT ( 'NONE',  ( 150.3996455637841621, 270.1471677736116703, 15.13740740754872327 ) ) ;
#1045=CARTESIAN_POINT ( 'NONE',  ( 64.10800479423805598, 214.4865022471902876, -10.00000000000009415 ) ) ;
#1049=CARTESIAN_POINT ( 'NONE',  ( 36.95476026646328194, 182.9548013555409796, -4.594050593750042211 ) ) ;
#1053=CARTESIAN_POINT ( 'NONE',  ( 199.1526122334580862, 285.7045524820243259, -17.32174362185583050 ) ) ;
#1056=CARTESIAN_POINT ( 'NONE',  ( 202.2006020915977729, 279.2500615382859905, -15.85648173203151323 ) ) ;
#1057=CARTESIAN_POINT ( 'NONE',  ( 163.9073938094922767, 282.0100812378155410, 10.03296392472801024 ) ) ;
#1059=CARTESIAN_POINT ( 'NONE',  ( 202.7599932440484451, 279.4563852894229967, 15.58249343055423353 ) ) ;
#1060=CARTESIAN_POINT ( 'NONE',  ( 100.8238734719678860, 239.0177522451419350, 5.000000000000046185 ) ) ;
#1062=CARTESIAN_POINT ( 'NONE',  ( 175.2559942677915785, 257.1225370724986874, 11.81907156814548365 ) ) ;
#1063=ORIENTED_EDGE ( 'NONE', *, *, #73652, .T. ) ;
#1070=( BOUNDED_CURVE ( )  B_SPLINE_CURVE ( 2, ( #26741, #78974, #33868, #55617, #95188, #32338, #25759, #50042, #86600 ),
 .UNSPECIFIED., .F., .T. ) 
 B_SPLINE_CURVE_WITH_KNOTS ( ( 3, 2, 2, 2, 3 ),
 ( 0.3588709677419354982, 0.3602150537634408733, 0.3629032258064516236, 0.3655913978494623739, 0.3669354838709677491 ),
 .UNSPECIFIED. ) 
 CURVE ( )  GEOMETRIC_REPRESENTATION_ITEM ( )  RATIONAL_B_SPLINE_CURVE ( ( 0.9330127018922194093, 0.9330127018922194093, 1.000000000000000000, 0.8660254037844387076, 1.000000000000000000, 0.8660254037844387076, 1.000000000000000000, 0.9330127018922194093, 0.9330127018922194093 ) ) 
 REPRESENTATION_ITEM ( '' )  );
#1071=CARTESIAN_POINT ( 'NONE',  ( 32.27361296988652128, 177.8932355074535678, -2.679491924311248496 ) ) ;
#1073=VECTOR ( 'NONE', #13467, 1000.000000000000000 ) ;
#1076=ORIENTED_EDGE ( 'NONE', *, *, #83228, .T. ) ;
#1077=VERTEX_POINT ( 'NONE', #76454 ) ;
#1078=DIRECTION ( 'NONE',  ( 0.4999999999999998890, -0.8660254037844385966, 0.000000000000000000 ) ) ;
#1081=CARTESIAN_POINT ( 'NONE',  ( 191.5766842709549280, 298.8264446275616137, 8.039910086100929831 ) ) ;
#1083=CYLINDRICAL_SURFACE ( 'NONE', #77437, 17.82106496071139645 ) ;
#1086=CARTESIAN_POINT ( 'NONE',  ( 147.6220714307702622, 274.9580672937808572, 8.392894244419288441 ) ) ;
#1087=CARTESIAN_POINT ( 'NONE',  ( 148.9194629746633893, 272.7109192224475009, -12.27648025871169679 ) ) ;
#1088=CARTESIAN_POINT ( 'NONE',  ( 180.5747241553744686, 287.0254358638467806, -13.54112932651550416 ) ) ;
#1089=ORIENTED_EDGE ( 'NONE', *, *, #73411, .F. ) ;
#1092=CARTESIAN_POINT ( 'NONE',  ( 161.9493756838661511, 266.9722091390776768, 16.54811282007660012 ) ) ;
#1093=ORIENTED_EDGE ( 'NONE', *, *, #65996, .T. ) ;
#1095=CARTESIAN_POINT ( 'NONE',  ( 157.1289238671306805, 259.1523436189365270, 17.02785937198905941 ) ) ;
#1097=CARTESIAN_POINT ( 'NONE',  ( 58.68649846873780263, 198.5643266524160140, 9.188101187500095079 ) ) ;
#1106=CARTESIAN_POINT ( 'NONE',  ( 190.1607982559816890, 301.2788311432216233, -4.972636536415983244 ) ) ;
#1107=CARTESIAN_POINT ( 'NONE',  ( 147.6207754342248961, 274.9603120256437592, 8.795690793376332195 ) ) ;
#1108=VERTEX_POINT ( 'NONE', #37915 ) ;
#1109=CARTESIAN_POINT ( 'NONE',  ( 175.3538927705540686, 261.0322813687463395, -14.65776196239626650 ) ) ;
#1110=CARTESIAN_POINT ( 'NONE',  ( 171.9695299662907360, 276.3046275190319534, -16.98996149290084645 ) ) ;
#1111=CARTESIAN_POINT ( 'NONE',  ( 207.8792014703394671, 270.5896565469619759, -5.780233892547864905 ) ) ;
#1112=CARTESIAN_POINT ( 'NONE',  ( 193.1169444172380167, 296.1586357973259283, -13.13373377033755318 ) ) ;
#1113=CARTESIAN_POINT ( 'NONE',  ( 163.8566702472313921, 257.1696457478908542, 15.67296822151954849 ) ) ;
#1114=CARTESIAN_POINT ( 'NONE',  ( 176.9230647991562364, 269.9553266851162334, 16.63264067541030755 ) ) ;
#1119=CARTESIAN_POINT ( 'NONE',  ( 109.2403843188893831, 240.0024278399160949, -9.188101187500093303 ) ) ;
#1121=CARTESIAN_POINT ( 'NONE',  ( 191.1000148935602567, 299.6520602076213891, -9.462302242170249400 ) ) ;
#1123=CARTESIAN_POINT ( 'NONE',  ( 155.6535436963908694, 261.0471492701456668, -17.87366571046205976 ) ) ;
#1124=EDGE_CURVE ( 'NONE', #7185, #31220, #63203, .T. ) ;
#1125=CARTESIAN_POINT ( 'NONE',  ( 192.3862142521138878, 296.3260726571497798, 12.05156688669263687 ) ) ;
#1127=CYLINDRICAL_SURFACE ( 'NONE', #11083, 17.82106496071139645 ) ;
#1133=CARTESIAN_POINT ( 'NONE',  ( 206.7044739906782809, 272.6243442267827959, -10.28926534613781030 ) ) ;
#1134=CARTESIAN_POINT ( 'NONE',  ( 126.4254891512956220, 252.9869531367911009, 4.594050593750046652 ) ) ;
#1135=CARTESIAN_POINT ( 'NONE',  ( 151.1126408083691501, 268.9122237844355254, -15.82705194100464396 ) ) ;
#1136=CARTESIAN_POINT ( 'NONE',  ( 185.5783427554117395, 297.2518047243089541, 4.097492125301632093 ) ) ;
#1138=CARTESIAN_POINT ( 'NONE',  ( 187.5093160991869752, 281.3588210269506931, -17.01637650260816059 ) ) ;
#1140=CARTESIAN_POINT ( 'NONE',  ( 46.39958950466356669, 197.5958772461660544, -9.188101187500095079 ) ) ;
#1145=CARTESIAN_POINT ( 'NONE',  ( 161.9461893331167914, 280.9078031139047198, -10.53061385661272276 ) ) ;
#1146=B_SPLINE_SURFACE_WITH_KNOTS ( 'NONE', 3, 1, ( 
 ( #89996, #5855 ),
 ( #51958, #82898 ),
 ( #84381, #98579 ),
 ( #52440, #59026 ),
 ( #83388, #20572 ),
 ( #13953, #22044 ),
 ( #44836, #83892 ),
 ( #37727, #15933 ),
 ( #92477, #45818 ),
 ( #23024, #38730 ),
 ( #92967, #93981 ),
 ( #47330, #76742 ),
 ( #1760, #77240 ),
 ( #242, #7335 ),
 ( #23521, #53917 ),
 ( #54412, #40216 ),
 ( #46838, #61534 ),
 ( #8344, #77761 ),
 ( #38217, #85387 ),
 ( #78256, #70122 ),
 ( #31123, #8836 ),
 ( #735, #25031 ),
 ( #24533, #55910 ),
 ( #39215, #32639 ),
 ( #69633, #100062 ),
 ( #7846, #31619 ),
 ( #86398, #69132 ),
 ( #63535, #84879 ),
 ( #62516, #93479 ),
 ( #62015, #15419 ),
 ( #55414, #1246 ),
 ( #94477, #24032 ),
 ( #54932, #30649 ),
 ( #85909, #16436 ) ),
 .UNSPECIFIED., .T., .F., .F.,
 ( 4, 2, 2, 2, 2, 2, 2, 2, 2, 2, 2, 2, 2, 2, 2, 2, 4 ),
 ( 2, 2 ),
 ( 0.000000000000000000, 0.06250000000000000000, 0.1250000000000000000, 0.1875000000000000000, 0.2500000000000000000, 0.3125000000000000000, 0.3750000000000000000, 0.4375000000000000000, 0.5000000000000000000, 0.5625000000000000000, 0.6250000000000000000, 0.6875000000000000000, 0.7500000000000000000, 0.8125000000000000000, 0.8750000000000000000, 0.9375000000000000000, 1.000000000000000000 ),
 ( 0.000000000000000000, 1.000000000000000000 ),
 .UNSPECIFIED. ) ;
#1148=CARTESIAN_POINT ( 'NONE',  ( 174.7088583562716053, 261.8961954955167357, 14.25351817334065530 ) ) ;
#1149=CARTESIAN_POINT ( 'NONE',  ( 151.2840067701813780, 278.5577605986394474, -1.687242923209387735 ) ) ;
#1151=CARTESIAN_POINT ( 'NONE',  ( 17.82181404068577635, 169.5494855054051868, -2.679491924311248496 ) ) ;
#1154=CARTESIAN_POINT ( 'NONE',  ( 119.0825757350898755, 232.8927522451418213, 10.00000000000009592 ) ) ;
#1155=CARTESIAN_POINT ( 'NONE',  ( 194.6014564220333511, 293.2009624057436099, -14.62462923522720715 ) ) ;
#1157=CARTESIAN_POINT ( 'NONE',  ( 147.6430623265936219, 274.9217099957185155, 8.258152514891218487 ) ) ;
#1158=CYLINDRICAL_SURFACE ( 'NONE', #83638, 10.00000000000010658 ) ;
#1159=CARTESIAN_POINT ( 'NONE',  ( 34.24843087963692767, 181.3923013555409796, 4.594050593750050204 ) ) ;
#1165=CARTESIAN_POINT ( 'NONE',  ( 55.05949644674294774, 214.8464784336661637, 1.353441290958777327E-15 ) ) ;
#1166=CARTESIAN_POINT ( 'NONE',  ( 172.5743551997954910, 287.3686559151746565, 7.484598097167019404 ) ) ;
#1167=CARTESIAN_POINT ( 'NONE',  ( 184.7346430054644770, 257.4289713573899689, 1.391138223594709178 ) ) ;
#1168=CARTESIAN_POINT ( 'NONE',  ( 204.6470611188870521, 276.1878878528713130, -13.02652554726987866 ) ) ;
#1171=CARTESIAN_POINT ( 'NONE',  ( 179.4155677608637802, 294.8372702107813552, 1.080509646882094721 ) ) ;
#1172=CARTESIAN_POINT ( 'NONE',  ( 33.07542782529571923, 183.2365022471902023, -10.00000000000009059 ) ) ;
#1175=CARTESIAN_POINT ( 'NONE',  ( 162.7644741734472120, 248.7306563947940958, 9.865755277559742353 ) ) ;
#1176=CARTESIAN_POINT ( 'NONE',  ( -5.724140937729833567, 161.3768266524159856, -9.188101187500091527 ) ) ;
#1179=CARTESIAN_POINT ( 'NONE',  ( 200.3640505997411481, 282.4509422428217249, 17.04400613106654561 ) ) ;
#1180=CARTESIAN_POINT ( 'NONE',  ( 185.7885272225882147, 259.4715261277827949, 7.392998191279108511 ) ) ;
#1181=CARTESIAN_POINT ( 'NONE',  ( 164.3090168944849836, 246.0554299274959931, 2.641760039552302430 ) ) ;
#1185=CARTESIAN_POINT ( 'NONE',  ( 177.8941590232256829, 264.7610587325321490, 16.13327920565182438 ) ) ;
#1187=CARTESIAN_POINT ( 'NONE',  ( 177.8185504528716194, 286.5248637125107507, 13.46785215458145935 ) ) ;
#1188=CARTESIAN_POINT ( 'NONE',  ( 167.1765958872485669, 286.3533408718084843, 0.5009160953947644490 ) ) ;
#1190=DIRECTION ( 'NONE',  ( -0.8660254037844387076, -0.4999999999999998890, -0.000000000000000000 ) ) ;
#1191=CARTESIAN_POINT ( 'NONE',  ( 206.0930919633010774, 273.6832889610345774, -9.866500005465628220 ) ) ;
#1192=CARTESIAN_POINT ( 'NONE',  ( 152.6656396574222754, 266.2223508737794759, 17.04346597795114349 ) ) ;
#1193=DIRECTION ( 'NONE',  ( 0.4999999999999992784, -0.8660254037844390407, 0.000000000000000000 ) ) ;
#1194=CARTESIAN_POINT ( 'NONE',  ( 191.3509382880371561, 298.5884961055737108, 8.308752174519279166 ) ) ;
#1195=CARTESIAN_POINT ( 'NONE',  ( 162.6257765080958677, 248.9708877980734485, -10.42859054881151160 ) ) ;
#1196=CARTESIAN_POINT ( 'NONE',  ( 155.2695601165254402, 261.7122283397445131, 16.98599069618989077 ) ) ;
#1198=ORIENTED_EDGE ( 'NONE', *, *, #96350, .T. ) ;
#1201=ORIENTED_EDGE ( 'NONE', *, *, #26302, .F. ) ;
#1207=CARTESIAN_POINT ( 'NONE',  ( 197.0226655822963551, 289.3937282992477549, -17.28982543158101493 ) ) ;
#1211=CARTESIAN_POINT ( 'NONE',  ( 203.1289230791707325, 278.8173800705629901, 16.48573034889792766 ) ) ;
#1212=AXIS2_PLACEMENT_3D ( 'NONE', #50050, #11070, #88611 ) ;
#1213=CARTESIAN_POINT ( 'NONE',  ( 179.7896684074626705, 294.5542936293851994, 4.419446707887151327 ) ) ;
#1214=CARTESIAN_POINT ( 'NONE',  ( 151.1926529451685326, 268.7736386982768408, 14.30343427984827365 ) ) ;
#1215=CARTESIAN_POINT ( 'NONE',  ( 170.8865616681041786, 262.8912071418242817, 16.88624067591380040 ) ) ;
#1222=ORIENTED_EDGE ( 'NONE', *, *, #62050, .F. ) ;
#1223=CARTESIAN_POINT ( 'NONE',  ( 164.4989226152910646, 245.7265035704120351, -6.575810094723514965 ) ) ;
#1225=CARTESIAN_POINT ( 'NONE',  ( 194.3413770922408617, 282.8930799310762723, 17.82077676852630077 ) ) ;
#1226=CARTESIAN_POINT ( 'NONE',  ( 167.8168677204402286, 281.0867839191200233, 11.63333370205274164 ) ) ;
#1227=CARTESIAN_POINT ( 'NONE',  ( 194.8708600166808651, 293.1207648669033006, -14.79199694356877970 ) ) ;
#1232=CARTESIAN_POINT ( 'NONE',  ( 198.5175125801355023, 277.4849542247185923, -15.35271413496788284 ) ) ;
#1233=CARTESIAN_POINT ( 'NONE',  ( 191.2828038517077687, 298.6283140572585921, -8.265843987895989287 ) ) ;
#1234=CARTESIAN_POINT ( 'NONE',  ( 159.3169041484411537, 254.7020228407560580, 16.67170756419672628 ) ) ;
#1236=CARTESIAN_POINT ( 'NONE',  ( 147.4638118793037336, 275.2321808777038541, -3.319864518316978597 ) ) ;
#1237=CARTESIAN_POINT ( 'NONE',  ( 168.5649949959667424, 256.9588418996493715, -14.86446260810648567 ) ) ;
#1238=CARTESIAN_POINT ( 'NONE',  ( 206.7408728089182546, 272.5612996242556960, -10.63134519248043475 ) ) ;
#1242=CARTESIAN_POINT ( 'NONE',  ( 200.4403816905005158, 283.4740703539914648, 16.81798557643505987 ) ) ;
#1244=CARTESIAN_POINT ( 'NONE',  ( 115.1800009256237729, 225.7592609112380160, 2.679491924311254714 ) ) ;
#1245=ORIENTED_EDGE ( 'NONE', *, *, #53442, .T. ) ;
#1246=CARTESIAN_POINT ( 'NONE',  ( 155.2417138354696817, 261.7604595133352063, -18.54054473025617966 ) ) ;
#1248=CARTESIAN_POINT ( 'NONE',  ( 128.6323578686148892, 256.6199935810940929, 2.679491924311251605 ) ) ;
#1250=CARTESIAN_POINT ( 'NONE',  ( 141.9699493749754140, 259.7505386000626686, -7.968025677899344572 ) ) ;
#1251=EDGE_CURVE ( 'NONE', #65280, #58155, #20847, .T. ) ;
#1252=CARTESIAN_POINT ( 'NONE',  ( 14.65434579541627969, 179.2677522451418497, 10.00000000000009592 ) ) ;
#1253=CARTESIAN_POINT ( 'NONE',  ( 94.11243691623624841, 215.9548013555409796, -4.594050593750042211 ) ) ;
#1255=CARTESIAN_POINT ( 'NONE',  ( 174.6020076113873358, 282.3130386525841686, -14.36087153468174904 ) ) ;
#1256=B_SPLINE_CURVE_WITH_KNOTS ( 'NONE', 3,
 ( #89072, #19623, #50977, #66193 ),
 .UNSPECIFIED., .F., .F.,
 ( 4, 4 ),
 ( 0.03792759114226184475, 0.04649815087312540729 ),
 .UNSPECIFIED. ) ;
#1258=CARTESIAN_POINT ( 'NONE',  ( 6.480970727150832111, 183.7369531367911009, -4.594050593750048428 ) ) ;
#1260=CARTESIAN_POINT ( 'NONE',  ( 200.6129772034685175, 283.1751261563724142, 18.36811917402039640 ) ) ;
#1263=CARTESIAN_POINT ( 'NONE',  ( 147.7840666256145425, 276.6774833857293174, 0.9737628777943441172 ) ) ;
#1264=CARTESIAN_POINT ( 'NONE',  ( 189.0469464145041911, 261.1622915045712148, -6.157471025067191128 ) ) ;
#1267=CARTESIAN_POINT ( 'NONE',  ( 207.7320178805681508, 270.8445860024863237, -5.379955943374661764 ) ) ;
#1268=CARTESIAN_POINT ( 'NONE',  ( 86.26382137438992004, 230.6115022471902876, -5.000000000000047962 ) ) ;
#1270=CARTESIAN_POINT ( 'NONE',  ( 30.10766014385131939, 182.0643266524160424, 9.188101187500095079 ) ) ;
#1271=CARTESIAN_POINT ( 'NONE',  ( 82.63733999249467388, 228.5177522451419350, 5.000000000000046185 ) ) ;
#1273=CARTESIAN_POINT ( 'NONE',  ( 199.5360113197090186, 277.4446805320934004, 15.14791943599612445 ) ) ;
#1275=CARTESIAN_POINT ( 'NONE',  ( 194.9499559406243918, 279.5747724307917679, 17.51673600049429780 ) ) ;
#1276=CARTESIAN_POINT ( 'NONE',  ( 182.5651185885155598, 260.5800487877630758, -10.89712475207159592 ) ) ;
#1278=CARTESIAN_POINT ( 'NONE',  ( 151.2671975087473015, 270.6445237267302559, 14.15418255155509542 ) ) ;
#1279=CARTESIAN_POINT ( 'NONE',  ( 157.1606030646430554, 258.4368458743103361, 17.96998724893680688 ) ) ;
#1282=LINE ( 'NONE', #32166, #20635 ) ;
#1283=CARTESIAN_POINT ( 'NONE',  ( 186.5814202129567434, 282.6718092406691767, 16.17431581196632706 ) ) ;
#1284=CARTESIAN_POINT ( 'NONE',  ( 194.7576540903134799, 293.3168432830895540, -14.62421624641040196 ) ) ;
#1285=CARTESIAN_POINT ( 'NONE',  ( 190.1907070792632624, 262.6060493502955637, 8.341994654895554362 ) ) ;
#1286=CARTESIAN_POINT ( 'NONE',  ( 163.7239493340838123, 247.0687966679708438, 6.286946239157660266 ) ) ;
#1287=CARTESIAN_POINT ( 'NONE',  ( 26.96143514339544467, 174.8262482093457777, 3.021315404115420679E-15 ) ) ;
#1289=CARTESIAN_POINT ( 'NONE',  ( 147.7978300115112233, 274.6536445020713018, 7.902890709649431855 ) ) ;
#1291=FACE_OUTER_BOUND ( 'NONE', #71938, .T. ) ;
#1292=AXIS2_PLACEMENT_3D ( 'NONE', #79941, #10501, #47984 ) ;
#1293=CARTESIAN_POINT ( 'NONE',  ( 162.0012282828890022, 251.8624688453083422, -14.05248242572528738 ) ) ;
#1294=CARTESIAN_POINT ( 'NONE',  ( 105.1810637865323628, 231.5333772461660828, 9.188101187500095079 ) ) ;
#1299=CARTESIAN_POINT ( 'NONE',  ( 196.2609093297512857, 290.7131288316392670, 16.03897268885959448 ) ) ;
#1301=CARTESIAN_POINT ( 'NONE',  ( 191.1669730766547275, 299.5360852325191559, -7.933564783864602177 ) ) ;
#1302=CARTESIAN_POINT ( 'NONE',  ( 190.2490083984490354, 261.0793145204391976, -4.628088261293119565 ) ) ;
#1305=CARTESIAN_POINT ( 'NONE',  ( 46.95533697774293103, 209.4637435831424455, 2.679491924311303119 ) ) ;
#1306=CARTESIAN_POINT ( 'NONE',  ( 146.9700173529739970, 276.0874580858064746, -5.099093031535578469 ) ) ;
#1309=CARTESIAN_POINT ( 'NONE',  ( -22.42236680055709641, 157.8615022471902591, 0.000000000000000000 ) ) ;
#1311=CARTESIAN_POINT ( 'NONE',  ( 199.9158968934949598, 270.1292180026705410, 9.240553224730840398 ) ) ;
#1312=ORIENTED_EDGE ( 'NONE', *, *, #9305, .T. ) ;
#1315=CARTESIAN_POINT ( 'NONE',  ( 180.9962514683335257, 255.6518059654043782, 5.281628127585873855 ) ) ;
#1317=CARTESIAN_POINT ( 'NONE',  ( 183.2138347319267950, 296.5967044714456620, -4.168135968712713968 ) ) ;
#1318=FACE_OUTER_BOUND ( 'NONE', #30711, .T. ) ;
#1325=CARTESIAN_POINT ( 'NONE',  ( 165.6005443753849420, 279.9182785130287243, 11.76136245517345991 ) ) ;
#1326=ADVANCED_FACE ( 'NONE', ( #76214 ), #13894, .T. ) ;
#1329=ORIENTED_EDGE ( 'NONE', *, *, #21958, .F. ) ;
#1331=CARTESIAN_POINT ( 'NONE',  ( 134.6192181478005523, 236.9824982072973967, 3.021315404115420679E-15 ) ) ;
#1332=CARTESIAN_POINT ( 'NONE',  ( 163.7729086741176161, 246.9839966035275438, 6.099406794390714204 ) ) ;
#1335=FACE_OUTER_BOUND ( 'NONE', #59028, .T. ) ;
#1338=CARTESIAN_POINT ( 'NONE',  ( 175.4214522509338678, 258.5208151414564668, 13.04691889165856011 ) ) ;
#1341=VERTEX_POINT ( 'NONE', #60468 ) ;
#1342=CARTESIAN_POINT ( 'NONE',  ( 173.3891276806938322, 270.4835184475072651, 17.26558241125811222 ) ) ;
#1345=CARTESIAN_POINT ( 'NONE',  ( 182.7854418666322545, 280.3108875730028444, -16.10961360330436065 ) ) ;
#1346=CARTESIAN_POINT ( 'NONE',  ( 164.2877295051262934, 246.0923007674255416, -1.726861278304287373 ) ) ;
#1347=CARTESIAN_POINT ( 'NONE',  ( 147.5830093564496224, 275.0257247911527543, -7.422490571551428218 ) ) ;
#1348=CARTESIAN_POINT ( 'NONE',  ( 186.1630411436486554, 296.9614825196608194, -7.488375694256206749 ) ) ;
#1351=CARTESIAN_POINT ( 'NONE',  ( 167.6436438581388870, 249.1749608028844705, -5.378307912567069415 ) ) ;
#1354=CARTESIAN_POINT ( 'NONE',  ( 154.0314627544081816, 279.5640916383285912, 2.169601216685385303 ) ) ;
#1355=CARTESIAN_POINT ( 'NONE',  ( 129.5380282679697075, 245.5958772461660544, -9.188101187500095079 ) ) ;
#1356=CARTESIAN_POINT ( 'NONE',  ( 186.6422722926715778, 262.8257398156653153, -9.173408779546029734 ) ) ;
#1364=CARTESIAN_POINT ( 'NONE',  ( 180.8417871952999860, 256.1704575049583354, 0.9644184763862307941 ) ) ;
#1365=CARTESIAN_POINT ( 'NONE',  ( 174.3162989310297633, 290.4431585964500755, -4.830845372109453528 ) ) ;
#1366=CARTESIAN_POINT ( 'NONE',  ( 192.2537778369132582, 297.6536841698438138, 12.51786810291793550 ) ) ;
#1370=CARTESIAN_POINT ( 'NONE',  ( 153.6596595523362794, 266.9882342533689439, 16.60685250298524807 ) ) ;
#1372=( BOUNDED_CURVE ( )  B_SPLINE_CURVE ( 1, ( #51079, #12106 ),
 .UNSPECIFIED., .F., .T. ) 
 B_SPLINE_CURVE_WITH_KNOTS ( ( 2, 2 ),
 ( 0.000000000000000000, 0.0003750000000000086272 ),
 .UNSPECIFIED. ) 
 CURVE ( )  GEOMETRIC_REPRESENTATION_ITEM ( )  RATIONAL_B_SPLINE_CURVE ( ( 0.9368410486966849415, 0.9368410486966849415 ) ) 
 REPRESENTATION_ITEM ( '' )  );
#1373=ORIENTED_EDGE ( 'NONE', *, *, #91745, .T. ) ;
#1374=CARTESIAN_POINT ( 'NONE',  ( 194.5252985417586729, 293.7192948986070178, -14.54632727629426370 ) ) ;
#1378=CARTESIAN_POINT ( 'NONE',  ( 191.0752600067845037, 266.8597520346529564, -12.80755884565359892 ) ) ;
#1381=CARTESIAN_POINT ( 'NONE',  ( 160.2722201351343472, 278.9910888498445729, 10.57498524561427367 ) ) ;
#1382=CARTESIAN_POINT ( 'NONE',  ( 151.9042993347139827, 267.5410309945612539, -16.88973072590943403 ) ) ;
#1383=CARTESIAN_POINT ( 'NONE',  ( 190.7862358025146534, 300.1955415356651429, 3.573119809004446257 ) ) ;
#1384=CARTESIAN_POINT ( 'NONE',  ( 204.7544901219449969, 272.8412540040631029, -10.83433605784845355 ) ) ;
#1385=CARTESIAN_POINT ( 'NONE',  ( 152.9741103202414081, 270.0357790464439063, 14.04803099111643760 ) ) ;
#1386=CARTESIAN_POINT ( 'NONE',  ( 160.8742158466989736, 281.6452003631559364, 6.228587064600521472 ) ) ;
#1387=CARTESIAN_POINT ( 'NONE',  ( 152.6621968174709991, 266.2283140474973493, -17.02835521334403168 ) ) ;
#1388=ORIENTED_EDGE ( 'NONE', *, *, #48703, .F. ) ;
#1389=CARTESIAN_POINT ( 'NONE',  ( 190.2648877593310317, 301.0985428348857340, -4.426259207433023590 ) ) ;
#1390=B_SPLINE_SURFACE_WITH_KNOTS ( 'NONE', 3, 1, ( 
 ( #13898, #71857 ),
 ( #79977, #98016 ),
 ( #41420, #36683 ),
 ( #67592, #59475 ),
 ( #80483, #34336 ),
 ( #2970, #2454 ),
 ( #33336, #96176 ),
 ( #70074, #45771 ),
 ( #83837, #37190 ),
 ( #100010, #91940 ),
 ( #22493, #6299 ),
 ( #39161, #84828 ),
 ( #30595, #22978 ),
 ( #14881, #61481 ),
 ( #7286, #689 ),
 ( #77710, #99510 ),
 ( #85334, #61964 ),
 ( #6795, #30094 ),
 ( #31571, #23982 ),
 ( #76219, #62463 ),
 ( #46265, #84336 ),
 ( #8296, #15367 ),
 ( #68092, #93429 ),
 ( #99013, #76693 ),
 ( #92431, #29600 ),
 ( #60472, #69085 ),
 ( #46790, #54879 ),
 ( #91429, #37676 ),
 ( #92917, #85860 ),
 ( #15877, #68587 ),
 ( #45285, #44778 ),
 ( #53867, #54361 ),
 ( #77186, #75714 ),
 ( #21992, #69583 ) ),
 .UNSPECIFIED., .T., .F., .F.,
 ( 4, 2, 2, 2, 2, 2, 2, 2, 2, 2, 2, 2, 2, 2, 2, 2, 4 ),
 ( 2, 2 ),
 ( 0.000000000000000000, 0.06250000000000000000, 0.1250000000000000000, 0.1875000000000000000, 0.2500000000000000000, 0.3125000000000000000, 0.3750000000000000000, 0.4375000000000000000, 0.5000000000000000000, 0.5625000000000000000, 0.6250000000000000000, 0.6875000000000000000, 0.7500000000000000000, 0.8125000000000000000, 0.8750000000000000000, 0.9375000000000000000, 1.000000000000000000 ),
 ( 0.000000000000000000, 1.000000000000000000 ),
 .UNSPECIFIED. ) ;
#1392=CARTESIAN_POINT ( 'NONE',  ( 128.5366863930700276, 235.0177522451417929, 5.000000000000051514 ) ) ;
#1393=CARTESIAN_POINT ( 'NONE',  ( 196.0587100571994483, 289.0633482449420626, -17.27351923437598913 ) ) ;
#1394=CARTESIAN_POINT ( 'NONE',  ( 199.1713105229414964, 278.4797133870983430, -16.65774537300400837 ) ) ;
#1396=CARTESIAN_POINT ( 'NONE',  ( 193.9204722154232741, 294.7668848255750049, 15.43855698596013859 ) ) ;
#1399=CARTESIAN_POINT ( 'NONE',  ( -12.00317221093202136, 170.0024278399160949, 9.188101187500095079 ) ) ;
#1400=CARTESIAN_POINT ( 'NONE',  ( 84.42325706775034178, 228.7369531367911293, -4.594050593750048428 ) ) ;
#1402=CARTESIAN_POINT ( 'NONE',  ( 146.7944005049231180, 276.3916353892955726, -4.243051111306586520 ) ) ;
#1403=CARTESIAN_POINT ( 'NONE',  ( 182.7907705717913416, 294.2845485110142363, -8.010541978009545261 ) ) ;
#1404=B_SPLINE_CURVE_WITH_KNOTS ( 'NONE', 3,
 ( #51844, #89875, #97463, #67524, #6224, #81777, #42715, #73650, #37120, #43720, #4230, #51321, #82288, #13349 ),
 .UNSPECIFIED., .F., .F.,
 ( 4, 2, 2, 2, 2, 2, 4 ),
 ( 8.079268757097385768E-15, 0.0005064305305122302706, 0.001012861061016381284, 0.001266076326268456790, 0.001519291591520532296, 0.001772506856772607803, 0.002025722122024683526 ),
 .UNSPECIFIED. ) ;
#1412=CARTESIAN_POINT ( 'NONE',  ( 161.9966032734278940, 250.0606478072812706, 13.86476480043075199 ) ) ;
#1413=CARTESIAN_POINT ( 'NONE',  ( 192.1779685593947420, 266.1842805242176269, 11.64530923862864142 ) ) ;
#1414=CARTESIAN_POINT ( 'NONE',  ( 161.5601416284384584, 251.9944088100220085, 13.91020052908825733 ) ) ;
#1417=CARTESIAN_POINT ( 'NONE',  ( 161.2133744761260061, 251.4172398781588811, -14.30368667312104058 ) ) ;
#1418=CARTESIAN_POINT ( 'NONE',  ( 39.09232661234986494, 199.5024278399160664, -9.188101187500093303 ) ) ;
#1419=CARTESIAN_POINT ( 'NONE',  ( 75.81765026128996965, 205.3923013555409796, 4.594050593750050204 ) ) ;
#1422=AXIS2_PLACEMENT_3D ( 'NONE', #52734, #21363, #76084 ) ;
#1423=CARTESIAN_POINT ( 'NONE',  ( 96.31878499345593525, 237.9637435831424739, 2.679491924311251605 ) ) ;
#1424=CARTESIAN_POINT ( 'NONE',  ( 198.2912749888956512, 286.5204237852628353, -17.12625248512345166 ) ) ;
#1426=AXIS2_PLACEMENT_3D ( 'NONE', #48202, #77624, #47685 ) ;
#1427=CARTESIAN_POINT ( 'NONE',  ( 196.5306890327151734, 269.6898905632888273, -10.81324570519863748 ) ) ;
#1430=CARTESIAN_POINT ( 'NONE',  ( 198.4522155198218059, 286.9176751754968109, -17.57438352224490075 ) ) ;
#1433=CARTESIAN_POINT ( 'NONE',  ( 65.88516108981343677, 208.8458772461660544, 9.188101187500095079 ) ) ;
#1435=CARTESIAN_POINT ( 'NONE',  ( 203.2369479875374623, 278.6302754407888074, -16.66242713208754367 ) ) ;
#1437=CARTESIAN_POINT ( 'NONE',  ( 197.8822014719394531, 287.9049684674569676, 17.88172308374019792 ) ) ;
#1439=CARTESIAN_POINT ( 'NONE',  ( 153.8601318185219782, 264.1534297615118021, 16.57777867432794139 ) ) ;
#1440=ADVANCED_FACE ( 'NONE', ( #52883 ), #76689, .T. ) ;
#1443=CARTESIAN_POINT ( 'NONE',  ( 104.4503548538631890, 231.1115022471902307, 10.00000000000009592 ) ) ;
#1444=CARTESIAN_POINT ( 'NONE',  ( 200.9111546617170916, 282.6586676490145464, 17.66063511622358106 ) ) ;
#1445=CARTESIAN_POINT ( 'NONE',  ( 207.4826643481121664, 271.2764789897469768, 7.783310782367018454 ) ) ;
#1448=CARTESIAN_POINT ( 'NONE',  ( 185.8974605661406940, 271.6370272364711127, 16.87882237039100275 ) ) ;
#1449=ORIENTED_EDGE ( 'NONE', *, *, #86391, .F. ) ;
#1450=CARTESIAN_POINT ( 'NONE',  ( 159.8732321751776624, 253.7384344327741132, -15.51998349828054202 ) ) ;
#1451=CARTESIAN_POINT ( 'NONE',  ( 189.2360998237118963, 278.0599140720760829, -16.51445267049493282 ) ) ;
#1452=EDGE_CURVE ( 'NONE', #483, #4766, #99437, .T. ) ;
#1456=VERTEX_POINT ( 'NONE', #82843 ) ;
#1458=CARTESIAN_POINT ( 'NONE',  ( 162.7595241543376972, 265.1439861438755088, -17.82152945942356226 ) ) ;
#1462=CARTESIAN_POINT ( 'NONE',  ( -27.42236680055714260, 166.5217562850347406, 1.224646799147364892E-15 ) ) ;
#1465=ORIENTED_EDGE ( 'NONE', *, *, #2974, .T. ) ;
#1469=EDGE_LOOP ( 'NONE', ( #89103, #33769, #36814, #35601 ) ) ;
#1470=CARTESIAN_POINT ( 'NONE',  ( 171.2347629857892457, 284.6507891007374269, 10.77592557674535279 ) ) ;
#1474=CARTESIAN_POINT ( 'NONE',  ( 155.5204415533959548, 261.2776889444089647, 17.19127227448963424 ) ) ;
#1475=CARTESIAN_POINT ( 'NONE',  ( 185.3860032077430162, 292.5766161388369255, -10.74141587811191911 ) ) ;
#1476=CARTESIAN_POINT ( 'NONE',  ( 157.1269483542914998, 258.4951375425532092, -17.15328932028234377 ) ) ;
#1477=CARTESIAN_POINT ( 'NONE',  ( 134.1114646098825176, 257.4244531367911577, -4.594050593750046652 ) ) ;
#1478=CARTESIAN_POINT ( 'NONE',  ( 205.3498812800093276, 270.0116018477241369, 2.442032521302731851 ) ) ;
#1480=CARTESIAN_POINT ( 'NONE',  ( 93.67942421434402434, 215.7048013555409796, 4.594050593750051981 ) ) ;
#1482=CARTESIAN_POINT ( 'NONE',  ( 151.4281781455628675, 268.3656970847310390, 15.24742929158552585 ) ) ;
#1485=CARTESIAN_POINT ( 'NONE',  ( 182.7264905230827878, 296.4309396610331078, 3.745374670362856762 ) ) ;
#1486=ORIENTED_EDGE ( 'NONE', *, *, #95684, .F. ) ;
#1490=CARTESIAN_POINT ( 'NONE',  ( 146.6834825911944620, 276.5837508513432681, 0.6716460511724984261 ) ) ;
#1492=CARTESIAN_POINT ( 'NONE',  ( 171.9695299662907360, 276.3046275190319534, -16.98996149290084645 ) ) ;
#1493=CARTESIAN_POINT ( 'NONE',  ( 207.5603179267596374, 271.1419790461399089, 2.162348062361596490 ) ) ;
#1494=CARTESIAN_POINT ( 'NONE',  ( 81.04025856027610075, 229.8464784336661353, 1.353441290958777327E-15 ) ) ;
#1498=CARTESIAN_POINT ( 'NONE',  ( 162.9111474110223412, 248.4766108952035211, -9.702990628959184960 ) ) ;
#1502=ADVANCED_FACE ( 'NONE', ( #1704 ), #40670, .T. ) ;
#1505=CARTESIAN_POINT ( 'NONE',  ( 162.2205785505892948, 283.9195354534895728, 0.5141653453796740658 ) ) ;
#1506=CARTESIAN_POINT ( 'NONE',  ( 186.2214199329484074, 263.1771180729978710, -12.06840420414929937 ) ) ;
#1511=CARTESIAN_POINT ( 'NONE',  ( 185.1628174925895678, 260.2253205732822039, 6.313110411375027375 ) ) ;
#1512=CARTESIAN_POINT ( 'NONE',  ( 206.3423291502491566, 273.2515974901050413, -10.76717883871977577 ) ) ;
#1514=CARTESIAN_POINT ( 'NONE',  ( 199.3359313799735162, 277.8054090533971134, 16.38672730308284997 ) ) ;
#1515=CARTESIAN_POINT ( 'NONE',  ( 174.6702674810315159, 283.6871151125846495, 13.51636394462591895 ) ) ;
#1516=CARTESIAN_POINT ( 'NONE',  ( -22.42236680055709641, 157.8615022471902591, 0.000000000000000000 ) ) ;
#1518=ORIENTED_EDGE ( 'NONE', *, *, #11686, .T. ) ;
#1519=CARTESIAN_POINT ( 'NONE',  ( -2.408111037970082968, 180.9637435831425307, 2.679491924311264039 ) ) ;
#1521=CARTESIAN_POINT ( 'NONE',  ( 161.1884843536000744, 251.4603508349806873, 13.21272898143761942 ) ) ;
#1523=CARTESIAN_POINT ( 'NONE',  ( 171.6205452999947738, 251.3949250676056977, 7.279205862586061393 ) ) ;
#1524=CARTESIAN_POINT ( 'NONE',  ( 198.8472845770790229, 265.6353728642903889, 1.646580097172975155 ) ) ;
#1525=CARTESIAN_POINT ( 'NONE',  ( 177.2779740990669666, 290.8998969752722701, -6.149525471840052937 ) ) ;
#1526=CARTESIAN_POINT ( 'NONE',  ( 153.4465587549918837, 270.2984085571182504, 14.02096340496593108 ) ) ;
#1528=FACE_OUTER_BOUND ( 'NONE', #61023, .T. ) ;
#1529=B_SPLINE_CURVE_WITH_KNOTS ( 'NONE', 3,
 ( #96845, #49698, #64407, #3141, #26909, #50685, #4601, #80651, #87781, #27413, #66398, #72019, #97325, #19817, #11229, #48719, #3621, #18317, #42095, #89268, #79650, #80149, #10715, #10216 ),
 .UNSPECIFIED., .F., .F.,
 ( 4, 2, 2, 2, 2, 2, 2, 2, 2, 2, 2, 4 ),
 ( 0.0002170125375182288085, 0.0007842342920218860289, 0.001067845169273751692, 0.001138747888586716644, 0.001174199248243124093, 0.001209650607899531542, 0.001245101967555938991, 0.001280553327212346441, 0.001351456046525128813, 0.001918677801027586635, 0.002202288678278833435, 0.002485899555530080886 ),
 .UNSPECIFIED. ) ;
#1532=CARTESIAN_POINT ( 'NONE',  ( 180.6402368737672646, 266.9317641007265252, -14.80827112732728779 ) ) ;
#1536=CARTESIAN_POINT ( 'NONE',  ( 170.0966408101324703, 273.6447761240920613, 15.99755975640291084 ) ) ;
#1537=CARTESIAN_POINT ( 'NONE',  ( 163.3213225887255078, 283.7535443778070317, -3.395488904438747735 ) ) ;
#1539=CARTESIAN_POINT ( 'NONE',  ( 188.8136734414513001, 259.8025127425751180, 3.692511016432421744 ) ) ;
#1540=CARTESIAN_POINT ( 'NONE',  ( 194.8451752635450021, 266.1831273802821443, -7.490151361129687935 ) ) ;
#1541=CARTESIAN_POINT ( 'NONE',  ( 2.557053438076354990, 172.2833772461660828, -9.188101187500095079 ) ) ;
#1543=VERTEX_POINT ( 'NONE', #85856 ) ;
#1544=CARTESIAN_POINT ( 'NONE',  ( 160.2740869459746023, 254.0686150970925610, -15.36085255641610914 ) ) ;
#1547=CARTESIAN_POINT ( 'NONE',  ( 198.7501991201633018, 286.4015524398827779, -18.58948563601804693 ) ) ;
#1548=CARTESIAN_POINT ( 'NONE',  ( 24.58674819472551931, 178.8768266524160140, 9.188101187500096856 ) ) ;
#1551=CARTESIAN_POINT ( 'NONE',  ( 180.8890834033174713, 294.3766012452771861, 6.559837412958372305 ) ) ;
#1552=CARTESIAN_POINT ( 'NONE',  ( 191.8000917695741805, 298.4394914891611847, -9.452573400474340914 ) ) ;
#1553=CARTESIAN_POINT ( 'NONE',  ( 12.29081813446918758, 171.2365022471902023, -10.00000000000009237 ) ) ;
#1556=CARTESIAN_POINT ( 'NONE',  ( 187.5517675740670427, 259.2187753813501558, -0.7877570970383018789 ) ) ;
#1557=CARTESIAN_POINT ( 'NONE',  ( 192.9518127100452034, 296.0217619941561793, -12.12386602825073645 ) ) ;
#1558=CARTESIAN_POINT ( 'NONE',  ( 63.31414817410230000, 217.3615022471903160, 5.000000000000046185 ) ) ;
#1560=CARTESIAN_POINT ( 'NONE',  ( 185.5756359364698085, 277.7569889279997142, -17.43085986457148806 ) ) ;
#1561=CYLINDRICAL_SURFACE ( 'NONE', #75770, 10.00000000000010658 ) ;
#1562=CARTESIAN_POINT ( 'NONE',  ( 29.86365662933068066, 197.2369531367911293, -4.594050593750048428 ) ) ;
#1563=CARTESIAN_POINT ( 'NONE',  ( 159.2077906806335932, 254.8910129107889588, 16.14624949541834553 ) ) ;
#1565=CARTESIAN_POINT ( 'NONE',  ( 198.7829547491859330, 286.3448180261817129, -18.59838968157616179 ) ) ;
#1567=AXIS2_PLACEMENT_3D ( 'NONE', #41270, #32183, #47869 ) ;
#1570=CARTESIAN_POINT ( 'NONE',  ( 89.31526421587503251, 210.8262482093457777, 3.021315404115420679E-15 ) ) ;
#1572=CARTESIAN_POINT ( 'NONE',  ( 162.8121824534329107, 280.4967882457603423, -9.952098035278266863 ) ) ;
#1573=CARTESIAN_POINT ( 'NONE',  ( 205.7045377653668936, 269.1581673421392793, -1.349048711920618926 ) ) ;
#1575=CARTESIAN_POINT ( 'NONE',  ( 203.0337691736598629, 278.9821914694464340, 16.08167820133810011 ) ) ;
#1576=CARTESIAN_POINT ( 'NONE',  ( 149.6191398986701415, 271.4990432411842676, -11.66821883946526839 ) ) ;
#1577=CARTESIAN_POINT ( 'NONE',  ( 186.1808859727878485, 268.2690591356716823, -14.28216311553996754 ) ) ;
#1584=ORIENTED_EDGE ( 'NONE', *, *, #68260, .F. ) ;
#1585=CARTESIAN_POINT ( 'NONE',  ( 32.15758756610207314, 177.8262482093457777, 3.021315404115420679E-15 ) ) ;
#1586=CARTESIAN_POINT ( 'NONE',  ( -22.42236680055709641, 157.8615022471902591, 0.000000000000000000 ) ) ;
#1587=DIRECTION ( 'NONE',  ( 0.5000000000000003331, -0.8660254037844384856, 0.000000000000000000 ) ) ;
#1588=ADVANCED_FACE ( 'NONE', ( #86345 ), #63107, .F. ) ;
#1589=CARTESIAN_POINT ( 'NONE',  ( 180.8238942241078178, 257.6885452376805574, -7.457973117650044337 ) ) ;
#1590=CARTESIAN_POINT ( 'NONE',  ( 190.0607312434325138, 301.4521522931182176, 3.538147641957853473 ) ) ;
#1593=CARTESIAN_POINT ( 'NONE',  ( 189.6631063493766760, 274.4263583876541475, -15.75412945656347041 ) ) ;
#1596=CARTESIAN_POINT ( 'NONE',  ( 200.6737073311291795, 283.0699384897140476, -17.61533935526990291 ) ) ;
#1600=CARTESIAN_POINT ( 'NONE',  ( 204.6470611188870521, 276.1878878528713130, -13.02652554726987866 ) ) ;
#1602=CARTESIAN_POINT ( 'NONE',  ( 100.2557178503908517, 222.5643266524160140, 9.188101187500095079 ) ) ;
#1604=CARTESIAN_POINT ( 'NONE',  ( 182.1881639437997933, 287.6810548547900908, -13.22834577702405490 ) ) ;
#1605=ORIENTED_EDGE ( 'NONE', *, *, #70139, .T. ) ;
#1606=CARTESIAN_POINT ( 'NONE',  ( 164.4578252119609090, 245.7976863610386999, -6.211333091911165560 ) ) ;
#1609=FACE_OUTER_BOUND ( 'NONE', #99954, .T. ) ;
#1611=CARTESIAN_POINT ( 'NONE',  ( 63.88265089144443465, 201.5643266524160140, 9.188101187500095079 ) ) ;
#1614=CARTESIAN_POINT ( 'NONE',  ( 150.6431064791187850, 269.7254810985950257, 15.11064854015152470 ) ) ;
#1616=CARTESIAN_POINT ( 'NONE',  ( 176.5838317420758870, 273.2463210208075566, 17.06958482087071260 ) ) ;
#1617=EDGE_LOOP ( 'NONE', ( #74533, #9087, #40422 ) ) ;
#1618=ADVANCED_FACE ( 'NONE', ( #89819 ), #64994, .T. ) ;
#1619=CARTESIAN_POINT ( 'NONE',  ( 183.1426684129219780, 267.5694331394444703, -16.03671021927237206 ) ) ;
#1620=CARTESIAN_POINT ( 'NONE',  ( 146.9376205018946848, 276.1435710778808925, 5.066564108429441937 ) ) ;
#1622=EDGE_LOOP ( 'NONE', ( #48162, #99884, #64854, #38345 ) ) ;
#1623=CARTESIAN_POINT ( 'NONE',  ( 175.2696475750532841, 261.2817613914389767, -14.26110703076659902 ) ) ;
#1625=CARTESIAN_POINT ( 'NONE',  ( 146.5068495316331791, 276.8896882847997176, 0.02371565180376856638 ) ) ;
#1626=CARTESIAN_POINT ( 'NONE',  ( 192.9523350703175311, 296.4437475495926719, -13.35611922184540923 ) ) ;
#1627=EDGE_CURVE ( 'NONE', #8540, #35319, #15977, .T. ) ;
#1629=CARTESIAN_POINT ( 'NONE',  ( 149.1903793729515257, 272.2416782560088677, 12.95958987445043675 ) ) ;
#1630=CARTESIAN_POINT ( 'NONE',  ( 179.7358607235859438, 270.8417515334642189, 16.28888456289437414 ) ) ;
#1631=CARTESIAN_POINT ( 'NONE',  ( 205.7829192689729325, 274.2205238267313234, 11.21202327925415254 ) ) ;
#1634=CARTESIAN_POINT ( 'NONE',  ( 208.3135187673106543, 269.8373969220020285, 2.829653198597726682 ) ) ;
#1635=CARTESIAN_POINT ( 'NONE',  ( 104.4229444624559733, 243.3464784336661353, 1.353441290958777327E-15 ) ) ;
#1637=CARTESIAN_POINT ( 'NONE',  ( 147.2229325088103735, 275.6493961858936927, -0.4918294119671829390 ) ) ;
#1641=CARTESIAN_POINT ( 'NONE',  ( 192.1146148663661393, 296.2687097199236632, 12.34145616421383984 ) ) ;
#1643=CARTESIAN_POINT ( 'NONE',  ( 178.0719526903251619, 255.3558746966477315, 4.708485374109758759 ) ) ;
#1645=CARTESIAN_POINT ( 'NONE',  ( 162.6396274730868186, 248.9468972229755082, -10.26162218571527518 ) ) ;
#1646=CARTESIAN_POINT ( 'NONE',  ( 157.9704523343261258, 276.0272599195727707, -12.71455051359169808 ) ) ;
#1647=CARTESIAN_POINT ( 'NONE',  ( 182.2170977436522605, 260.5581375984304486, 9.500862743582350944 ) ) ;
#1649=CARTESIAN_POINT ( 'NONE',  ( 119.6866422041566551, 252.1589784336661069, -6.496448406907676862E-16 ) ) ;
#1650=CARTESIAN_POINT ( 'NONE',  ( 151.0013883899287066, 269.1049186256390726, -14.25461351222133466 ) ) ;
#1652=CARTESIAN_POINT ( 'NONE',  ( 189.9224218318563260, 282.6927222767778858, -16.57155747260814849 ) ) ;
#1654=CARTESIAN_POINT ( 'NONE',  ( 45.88512659934279014, 206.4869531367911009, 4.594050593750046652 ) ) ;
#1658=CARTESIAN_POINT ( 'NONE',  ( 172.6568878728820948, 261.0847548073755320, 14.48626931307794763 ) ) ;
#1660=CARTESIAN_POINT ( 'NONE',  ( 178.8759581903709943, 291.7429665371036549, -6.258367371696258452 ) ) ;
#1661=CARTESIAN_POINT ( 'NONE',  ( 92.14326550588401687, 235.5530062829863027, -4.648177544792955347E-16 ) ) ;
#1662=CARTESIAN_POINT ( 'NONE',  ( 154.5654453936281811, 269.4902856693395279, -15.08148675096953717 ) ) ;
#1663=CARTESIAN_POINT ( 'NONE',  ( 115.9793180381956148, 237.7677522451418497, 10.00000000000009592 ) ) ;
#1668=CARTESIAN_POINT ( 'NONE',  ( 202.8499463704053198, 279.3005819042728604, 17.04674939340617001 ) ) ;
#1670=CARTESIAN_POINT ( 'NONE',  ( 21.77181853666109745, 189.5024278399160949, 9.188101187500095079 ) ) ;
#1672=CARTESIAN_POINT ( 'NONE',  ( 82.54166851694979812, 206.9155109091895781, 2.679491924311254714 ) ) ;
#1676=CARTESIAN_POINT ( 'NONE',  ( 60.19284827774804114, 198.8927522451417929, -10.00000000000009059 ) ) ;
#1677=CARTESIAN_POINT ( 'NONE',  ( 173.6627686280932039, 288.1531483176477764, 7.554607035878428967 ) ) ;
#1678=CARTESIAN_POINT ( 'NONE',  ( 163.1218343930725894, 256.2508100442478849, -16.13596270478102923 ) ) ;
#1679=FACE_OUTER_BOUND ( 'NONE', #67932, .T. ) ;
#1681=( BOUNDED_CURVE ( )  B_SPLINE_CURVE ( 2, ( #41156, #50264, #34092, #96411, #26979, #96917, #48791, #34568, #56365 ),
 .UNSPECIFIED., .F., .T. ) 
 B_SPLINE_CURVE_WITH_KNOTS ( ( 3, 2, 2, 2, 3 ),
 ( 0.5201612903225806273, 0.5215053763440860024, 0.5241935483870967527, 0.5268817204301075030, 0.5282258064516128782 ),
 .UNSPECIFIED. ) 
 CURVE ( )  GEOMETRIC_REPRESENTATION_ITEM ( )  RATIONAL_B_SPLINE_CURVE ( ( 0.9330127018922194093, 0.9330127018922194093, 1.000000000000000000, 0.8660254037844387076, 1.000000000000000000, 0.8660254037844387076, 1.000000000000000000, 0.9330127018922194093, 0.9330127018922194093 ) ) 
 REPRESENTATION_ITEM ( '' )  );
#1682=ORIENTED_EDGE ( 'NONE', *, *, #28240, .T. ) ;
#1683=CARTESIAN_POINT ( 'NONE',  ( 30.33301404664501888, 174.9865022471901739, 1.119607411625061291E-15 ) ) ;
#1684=CARTESIAN_POINT ( 'NONE',  ( 141.5809337175232940, 261.7369531367911009, -4.594050593750048428 ) ) ;
#1685=CARTESIAN_POINT ( 'NONE',  ( 162.8996025780091941, 248.4966071325470125, 11.23567065566008516 ) ) ;
#1686=CARTESIAN_POINT ( 'NONE',  ( 150.1064787036151245, 245.2202760586659736, -5.415160957724236172E-17 ) ) ;
#1689=CARTESIAN_POINT ( 'NONE',  ( 170.5027933921127214, 263.5424279318320941, 15.79580204150556710 ) ) ;
#1690=CARTESIAN_POINT ( 'NONE',  ( 190.5297895243285211, 290.4239949136141377, -15.76409704461241290 ) ) ;
#1692=EDGE_CURVE ( 'NONE', #25829, #86364, #82436, .T. ) ;
#1693=CARTESIAN_POINT ( 'NONE',  ( 183.4288420069315180, 257.9430297361450926, -2.297013850620948983 ) ) ;
#1698=CARTESIAN_POINT ( 'NONE',  ( 150.3237008197049249, 246.0494855054051868, -2.679491924311248496 ) ) ;
#1699=CARTESIAN_POINT ( 'NONE',  ( 153.3157916388551882, 277.7051378986778900, -5.233164379718747483 ) ) ;
#1701=CARTESIAN_POINT ( 'NONE',  ( 160.6498352449959555, 252.3933184585345657, 15.68867965355669192 ) ) ;
#1702=CARTESIAN_POINT ( 'NONE',  ( 206.8106726053982811, 272.4404028303941914, -10.47827087991598560 ) ) ;
#1703=EDGE_CURVE ( 'NONE', #82896, #73620, #37671, .T. ) ;
#1704=FACE_OUTER_BOUND ( 'NONE', #98531, .T. ) ;
#1705=CARTESIAN_POINT ( 'NONE',  ( 82.29453827371126806, 224.9865022471902876, -10.00000000000009592 ) ) ;
#1706=CARTESIAN_POINT ( 'NONE',  ( 93.72070878210261924, 236.4637435831425023, 2.679491924311251605 ) ) ;
#1708=CARTESIAN_POINT ( 'NONE',  ( 207.6555576926778883, 270.9770189326688410, -1.235081510489080436 ) ) ;
#1709=CARTESIAN_POINT ( 'NONE',  ( 193.7275870247597425, 295.1009717758319084, 14.48058678254265885 ) ) ;
#1710=ORIENTED_EDGE ( 'NONE', *, *, #10635, .F. ) ;
#1712=CARTESIAN_POINT ( 'NONE',  ( 155.8328110275561187, 276.9913226184394830, -10.28370083813354263 ) ) ;
#1717=VERTEX_POINT ( 'NONE', #76574 ) ;
#1718=CARTESIAN_POINT ( 'NONE',  ( 146.5310397537613483, 276.8477895910274356, -0.2793038414862049068 ) ) ;
#1720=B_SPLINE_CURVE_WITH_KNOTS ( 'NONE', 3,
 ( #31253, #17055, #62140, #71282 ),
 .UNSPECIFIED., .F., .F.,
 ( 4, 4 ),
 ( 0.003189740795969862874, 0.006687314450048887672 ),
 .UNSPECIFIED. ) ;
#1721=B_SPLINE_CURVE_WITH_KNOTS ( 'NONE', 3,
 ( #38117, #44236, #53821, #52839, #69035, #99962, #61432, #36639, #92385, #67045, #68046, #83788, #22933, #5748, #98475, #29068, #47724, #8251, #8743, #38630, #54316, #33037, #78659, #39613, #85286, #48242, #16835, #94380, #2158, #92873, #77664, #24444, #63937, #15831, #46736, #39116, #47237, #9247, #24934, #69541, #644, #56328, #32026, #23426, #61923, #62935 ),
 .UNSPECIFIED., .F., .F.,
 ( 4, 2, 2, 2, 2, 2, 2, 2, 2, 2, 2, 2, 2, 2, 2, 2, 2, 2, 2, 2, 2, 2, 4 ),
 ( 0.0004469933677433058803, 0.001460477987537453677, 0.001967220297434580430, 0.002093905874908885429, 0.002220591452383190428, 0.002347277029857495426, 0.002473962607331800859, 0.002727333762280489352, 0.002980704917229178279, 0.003487447227126506261, 0.004500931846921240286, 0.005514416466715974310, 0.006021158776613377318, 0.006274529931562079256, 0.006527901086510781194, 0.006591243875247919382, 0.006654586663985056702, 0.006717929452722194890, 0.006781272241459332210, 0.007034643396407847665, 0.007541385706304846483, 0.008048128016201843565, 0.008554870326098843250 ),
 .UNSPECIFIED. ) ;
#1722=B_SPLINE_CURVE_WITH_KNOTS ( 'NONE', 3,
 ( #93645, #23686, #24210, #69304 ),
 .UNSPECIFIED., .F., .F.,
 ( 4, 4 ),
 ( 0.008780835828182721042, 0.01389840247672927999 ),
 .UNSPECIFIED. ) ;
#1723=CARTESIAN_POINT ( 'NONE',  ( 149.3253462891332219, 272.0079086998416074, -12.99539319630191336 ) ) ;
#1726=CARTESIAN_POINT ( 'NONE',  ( 200.6129772034685175, 283.1751261563724142, 18.36811917402039640 ) ) ;
#1728=CARTESIAN_POINT ( 'NONE',  ( 150.6431064791187850, 269.7254810985950257, 15.11064854015152470 ) ) ;
#1730=ORIENTED_EDGE ( 'NONE', *, *, #38874, .F. ) ;
#1732=CARTESIAN_POINT ( 'NONE',  ( 163.4216610345155800, 247.5923753613567442, 10.58669027323842826 ) ) ;
#1736=ORIENTED_EDGE ( 'NONE', *, *, #93576, .T. ) ;
#1738=ORIENTED_EDGE ( 'NONE', *, *, #62645, .F. ) ;
#1742=CARTESIAN_POINT ( 'NONE',  ( 147.8505793332463725, 274.5622799967613332, -9.317516487097901035 ) ) ;
#1743=CARTESIAN_POINT ( 'NONE',  ( 174.9090629387510205, 290.7237071972734270, 6.492599126899565753 ) ) ;
#1744=CARTESIAN_POINT ( 'NONE',  ( -9.181706736895311138, 177.0530062829863027, -4.648177544792955347E-16 ) ) ;
#1746=CARTESIAN_POINT ( 'NONE',  ( 162.0192538899617318, 268.0510789565263394, -17.53028463913764057 ) ) ;
#1748=CARTESIAN_POINT ( 'NONE',  ( 206.0627831668701901, 273.7357853363691902, 10.14454147593459687 ) ) ;
#1749=CARTESIAN_POINT ( 'NONE',  ( 164.4494343874829099, 245.8122196953522121, 2.922779519406129456 ) ) ;
#1750=CARTESIAN_POINT ( 'NONE',  ( 194.7576052748250390, 276.3294723641358246, -16.78574826228364714 ) ) ;
#1752=CARTESIAN_POINT ( 'NONE',  ( 159.5180972751518595, 279.0588588540967976, -11.03979334413982016 ) ) ;
#1753=CYLINDRICAL_SURFACE ( 'NONE', #31801, 10.00000000000010658 ) ;
#1755=CARTESIAN_POINT ( 'NONE',  ( 206.4484807199597753, 273.0677375780628608, -9.220527398138528952 ) ) ;
#1757=CARTESIAN_POINT ( 'NONE',  ( 200.8828793852583203, 282.7076418644388696, 17.90302398138411633 ) ) ;
#1758=LINE ( 'NONE', #32637, #38511 ) ;
#1760=CARTESIAN_POINT ( 'NONE',  ( 194.4041250891751247, 293.9291734750100886, -14.17881196554796119 ) ) ;
#1761=CARTESIAN_POINT ( 'NONE',  ( 125.9182562534771677, 255.0530062829863311, -4.648177544792955347E-16 ) ) ;
#1762=FACE_OUTER_BOUND ( 'NONE', #78352, .T. ) ;
#1763=CARTESIAN_POINT ( 'NONE',  ( 22.01556172758404628, 173.5177522451417929, 5.000000000000051514 ) ) ;
#1764=CARTESIAN_POINT ( 'NONE',  ( 88.48327179163739231, 212.7048013555409796, 4.594050593750051981 ) ) ;
#1767=CARTESIAN_POINT ( 'NONE',  ( 208.1583869480885483, 270.1060931147653719, 3.025867354224990979 ) ) ;
#1769=CARTESIAN_POINT ( 'NONE',  ( 6.400214715252306341, 168.3768266524160140, 9.188101187500098632 ) ) ;
#1771=CARTESIAN_POINT ( 'NONE',  ( 161.8289209813647176, 250.3510820566641257, 13.28523796267037937 ) ) ;
#1774=EDGE_LOOP ( 'NONE', ( #22497, #18781, #42916, #60250, #80866, #21666, #96508 ) ) ;
#1775=CARTESIAN_POINT ( 'NONE',  ( 200.7721129302025247, 267.7114073205713112, -2.857155443757144031 ) ) ;
#1781=CARTESIAN_POINT ( 'NONE',  ( 43.58535403812915376, 183.7202760586659451, -5.415160957724236172E-17 ) ) ;
#1782=CARTESIAN_POINT ( 'NONE',  ( 200.0154776055639445, 276.6224788825257974, 15.58692471366793519 ) ) ;
#1784=CARTESIAN_POINT ( 'NONE',  ( 150.0080822439343535, 271.6737539543675553, -11.69383360110748526 ) ) ;
#1785=CARTESIAN_POINT ( 'NONE',  ( 173.8805019302338621, 250.6242863632701585, 0.4030408839048176262 ) ) ;
#1786=CARTESIAN_POINT ( 'NONE',  ( -15.08856125979659346, 174.3464784336661353, 1.353441290958777327E-15 ) ) ;
#1788=CARTESIAN_POINT ( 'NONE',  ( 191.3843761966370209, 282.8631020262318430, -17.76976768207862278 ) ) ;
#1790=CARTESIAN_POINT ( 'NONE',  ( 148.4083960970861256, 273.5961130204771052, -8.574185186226726429 ) ) ;
#1791=CARTESIAN_POINT ( 'NONE',  ( 186.0715527847238207, 298.7753624933060337, 1.084710433360843940 ) ) ;
#1792=CARTESIAN_POINT ( 'NONE',  ( 204.4325665793906524, 276.5594032932251594, 13.33817701435311598 ) ) ;
#1793=CARTESIAN_POINT ( 'NONE',  ( 147.2937583206075942, 275.5267222813735088, 0.1877253132609109920 ) ) ;
#1794=CARTESIAN_POINT ( 'NONE',  ( 147.9748066657072627, 274.3471119452502762, 9.387104374042873900 ) ) ;
#1796=CARTESIAN_POINT ( 'NONE',  ( 161.4297170363470570, 251.4317974835881273, -13.07316258580638291 ) ) ;
#1797=CARTESIAN_POINT ( 'NONE',  ( 105.5326262849960131, 240.9244531367911293, -4.594050593750046652 ) ) ;
#1799=CARTESIAN_POINT ( 'NONE',  ( 151.3883635558152321, 268.4346579770563608, 15.44343517165679103 ) ) ;
#1801=CARTESIAN_POINT ( 'NONE',  ( 157.2744851780909414, 258.2395962677452985, 18.17792129701959070 ) ) ;
#1803=CARTESIAN_POINT ( 'NONE',  ( -17.42236680055705023, 149.2012482093457777, 0.000000000000000000 ) ) ;
#1805=CARTESIAN_POINT ( 'NONE',  ( 149.4965729687386045, 271.7113353911534546, -11.48413836595348059 ) ) ;
#1806=CARTESIAN_POINT ( 'NONE',  ( 91.91334042722833431, 212.3262482093457493, 3.021315404115420679E-15 ) ) ;
#1807=CARTESIAN_POINT ( 'NONE',  ( 172.9595584307079434, 290.0517967578398384, -1.801039841358881066 ) ) ;
#1812=CARTESIAN_POINT ( 'NONE',  ( 199.9590217945695372, 270.1275301915071054, 9.211081333144562677 ) ) ;
#1819=CARTESIAN_POINT ( 'NONE',  ( 71.35865581505748878, 223.5530062829863027, -4.648177544792955347E-16 ) ) ;
#1820=CARTESIAN_POINT ( 'NONE',  ( 192.8325075361489382, 296.6512949269187516, 11.74553025762331515 ) ) ;
#1825=CARTESIAN_POINT ( 'NONE',  ( 193.9412999261856783, 289.2827323037661245, -16.07620684846729375 ) ) ;
#1826=ORIENTED_EDGE ( 'NONE', *, *, #7528, .F. ) ;
#1827=CARTESIAN_POINT ( 'NONE',  ( 164.0147331130573320, 279.8062665722855513, 12.46059690269307829 ) ) ;
#1829=CARTESIAN_POINT ( 'NONE',  ( 147.9500839974939197, 274.3899328626944225, -9.375093207164509224 ) ) ;
#1830=CARTESIAN_POINT ( 'NONE',  ( 160.2740869459746023, 254.0686150970925610, -15.36085255641610914 ) ) ;
#1833=CARTESIAN_POINT ( 'NONE',  ( 188.6020111787380529, 293.7306159932854825, 12.99143650644070824 ) ) ;
#1834=CARTESIAN_POINT ( 'NONE',  ( 163.7707306762541748, 246.9877690064858484, 7.021959502997312086 ) ) ;
#1838=CARTESIAN_POINT ( 'NONE',  ( 203.3205561747472814, 278.4854618126124706, -15.14439614831292147 ) ) ;
#1840=ORIENTED_EDGE ( 'NONE', *, *, #7938, .F. ) ;
#1841=CARTESIAN_POINT ( 'NONE',  ( 159.5606259118165724, 264.0648208006689401, -17.79391822139266566 ) ) ;
#1845=FACE_OUTER_BOUND ( 'NONE', #48421, .T. ) ;
#1846=CARTESIAN_POINT ( 'NONE',  ( 203.3684377202211522, 278.4025285431072803, -16.56116267537666076 ) ) ;
#1847=EDGE_LOOP ( 'NONE', ( #71468, #74257, #26944, #16905, #19567 ) ) ;
#1848=CARTESIAN_POINT ( 'NONE',  ( 185.9803440489478987, 282.4389606638047212, -17.18315826590863082 ) ) ;
#1850=CARTESIAN_POINT ( 'NONE',  ( 147.3086308153996242, 275.5009623647583226, -7.272174762944374038 ) ) ;
#1852=CARTESIAN_POINT ( 'NONE',  ( 192.5076277540105423, 297.2140032159341558, -13.10094381206144298 ) ) ;
#1853=CARTESIAN_POINT ( 'NONE',  ( 153.2283961777204695, 265.2476279883323400, -17.66880461074566000 ) ) ;
#1855=CARTESIAN_POINT ( 'NONE',  ( 154.7533266961937102, 279.6344470633707715, 2.131676877324898189 ) ) ;
#1856=CARTESIAN_POINT ( 'NONE',  ( 127.8874276638293850, 235.4548013555409796, -4.594050593750042211 ) ) ;
#1858=ORIENTED_EDGE ( 'NONE', *, *, #37574, .T. ) ;
#1859=CARTESIAN_POINT ( 'NONE',  ( 138.9086373102437051, 262.5530062829863027, -4.648177544792955347E-16 ) ) ;
#1861=CARTESIAN_POINT ( 'NONE',  ( 203.6309649086862237, 276.2215947889915810, 13.33342147041682502 ) ) ;
#1862=CARTESIAN_POINT ( 'NONE',  ( 180.7207050551674001, 256.2221533644915894, 1.285094096768985006 ) ) ;
#1863=CARTESIAN_POINT ( 'NONE',  ( 174.1986536150437246, 290.1369587316962679, -4.770100445387263299 ) ) ;
#1864=CARTESIAN_POINT ( 'NONE',  ( 192.5140213078438762, 297.2029292558541442, 12.60096557781599103 ) ) ;
#1865=CARTESIAN_POINT ( 'NONE',  ( 174.8696466734779449, 292.3029143586743430, -1.153856708368909967 ) ) ;
#1867=CARTESIAN_POINT ( 'NONE',  ( 174.1678698021581226, 287.3101935015571939, -9.481082537716513770 ) ) ;
#1868=CARTESIAN_POINT ( 'NONE',  ( 174.4948782939823104, 282.3355020129680497, 14.83901814079321824 ) ) ;
#1872=CARTESIAN_POINT ( 'NONE',  ( 194.1972774922283236, 294.2874440223457100, -15.09915398317898649 ) ) ;
#1873=B_SPLINE_CURVE_WITH_KNOTS ( 'NONE', 3,
 ( #86795, #64439, #19844, #89292, #50714, #49728, #72047, #96369 ),
 .UNSPECIFIED., .F., .F.,
 ( 4, 2, 2, 4 ),
 ( 0.001444873917495229261, 0.001841091017814789352, 0.002237308118134349443, 0.003029742318773326077 ),
 .UNSPECIFIED. ) ;
#1874=CARTESIAN_POINT ( 'NONE',  ( 152.1754162881449872, 273.0523641828442010, 11.78941638112353907 ) ) ;
#1875=ORIENTED_EDGE ( 'NONE', *, *, #26762, .F. ) ;
#1877=CARTESIAN_POINT ( 'NONE',  ( 191.0428398434177097, 283.3979691902844138, -16.57323166652324886 ) ) ;
#1878=CARTESIAN_POINT ( 'NONE',  ( 152.5148928264552524, 266.4834520440945198, -16.24327773663125640 ) ) ;
#1881=CARTESIAN_POINT ( 'NONE',  ( 162.8037981520209314, 248.6625452659484381, 9.809699077002424161 ) ) ;
#1882=CARTESIAN_POINT ( 'NONE',  ( 163.8036614586782207, 284.0923275947843081, -7.069034562687269485 ) ) ;
#1883=CARTESIAN_POINT ( 'NONE',  ( 160.9007617730179902, 281.5835503259689290, 5.800644519205480520 ) ) ;
#1884=CARTESIAN_POINT ( 'NONE',  ( 152.6692142062575499, 266.2161595735824449, -16.77985299603479419 ) ) ;
#1886=CARTESIAN_POINT ( 'NONE',  ( 164.4644309026115252, 280.9914584399565456, -11.74015880431011105 ) ) ;
#1887=CARTESIAN_POINT ( 'NONE',  ( 187.0781841533855641, 262.9812258568358629, -9.029666229471835948 ) ) ;
#1889=CARTESIAN_POINT ( 'NONE',  ( 173.8376058068382122, 250.6904955415916731, -0.9792276279091526314 ) ) ;
#1890=CARTESIAN_POINT ( 'NONE',  ( 198.6346039733307975, 275.4709485704699432, 15.56980991080272680 ) ) ;
#1892=CARTESIAN_POINT ( 'NONE',  ( 192.1396999271463812, 297.8512729055811974, 12.32430960859512403 ) ) ;
#1895=CARTESIAN_POINT ( 'NONE',  ( 193.0126352936363503, 264.4189281174865869, 8.906082567666748773 ) ) ;
#1897=CARTESIAN_POINT ( 'NONE',  ( 80.71549903385694336, 229.6589784336661637, -6.496448406907675876E-16 ) ) ;
#1901=EDGE_CURVE ( 'NONE', #82781, #91972, #39535, .T. ) ;
#1902=CARTESIAN_POINT ( 'NONE',  ( 202.9547455376043672, 279.1190644220934018, -15.19669173352461478 ) ) ;
#1904=DIRECTION ( 'NONE',  ( -0.8660254037844387076, -0.4999999999999998890, -0.000000000000000000 ) ) ;
#1908=CARTESIAN_POINT ( 'NONE',  ( 207.7802404240296141, 270.7610621071412424, 4.972114562312238029 ) ) ;
#1909=CARTESIAN_POINT ( 'NONE',  ( 169.2351887702091915, 252.1965608303764554, -9.016775029077457759 ) ) ;
#1910=CARTESIAN_POINT ( 'NONE',  ( 205.5937218600166432, 274.5482233517041095, -12.97537981636971338 ) ) ;
#1912=CARTESIAN_POINT ( 'NONE',  ( -14.49388456338638598, 173.9860189848785410, -2.679491924311249385 ) ) ;
#1913=CARTESIAN_POINT ( 'NONE',  ( 207.3874697692679945, 271.4413608369101780, -6.809237722377445401 ) ) ;
#1914=CARTESIAN_POINT ( 'NONE',  ( 43.96406660440233338, 190.0643266524159571, -9.188101187500093303 ) ) ;
#1916=CARTESIAN_POINT ( 'NONE',  ( 68.80799682758592439, 210.5333772461660544, 9.188101187500095079 ) ) ;
#1922=CARTESIAN_POINT ( 'NONE',  ( 175.2780979910569954, 269.4248474843194572, -16.41417513093275105 ) ) ;
#1925=CARTESIAN_POINT ( 'NONE',  ( 149.2765980486851731, 272.0923431290771646, -11.40617906909507973 ) ) ;
#1928=CARTESIAN_POINT ( 'NONE',  ( 60.41820218054165537, 211.8149278399160949, 9.188101187500093303 ) ) ;
#1931=CARTESIAN_POINT ( 'NONE',  ( 172.8484988039289476, 290.2287427593016673, -0.3445454264097566610 ) ) ;
#1933=CARTESIAN_POINT ( 'NONE',  ( 201.6381078894957852, 281.3995477237756404, 17.82831317141172889 ) ) ;
#1934=CARTESIAN_POINT ( 'NONE',  ( 121.3378502276597288, 240.8615022471902591, -10.00000000000009592 ) ) ;
#1936=CARTESIAN_POINT ( 'NONE',  ( 206.9377610035629118, 272.2202792677204002, 7.440532334334675646 ) ) ;
#1938=CARTESIAN_POINT ( 'NONE',  ( 149.1542970168542865, 273.4448608269726719, -9.883886189052034865 ) ) ;
#1940=EDGE_LOOP ( 'NONE', ( #364, #62575, #82433, #97940 ) ) ;
#1941=CARTESIAN_POINT ( 'NONE',  ( 162.8996025780091941, 248.4966071325470125, 11.23567065566008516 ) ) ;
#1942=CARTESIAN_POINT ( 'NONE',  ( 37.35373998880870516, 180.8262482093457493, 3.021315404115420679E-15 ) ) ;
#1944=EDGE_CURVE ( 'NONE', #21068, #20148, #50964, .T. ) ;
#1946=CARTESIAN_POINT ( 'NONE',  ( 176.5495440887839038, 253.2411848376090973, -0.2568067590575703329 ) ) ;
#1947=ORIENTED_EDGE ( 'NONE', *, *, #8996, .F. ) ;
#1949=CARTESIAN_POINT ( 'NONE',  ( 169.5363729319136610, 249.7081694927524040, 3.427481716433138814 ) ) ;
#1950=CARTESIAN_POINT ( 'NONE',  ( 161.1582366080876625, 264.6096096715138515, -17.81198817937834633 ) ) ;
#1954=DIRECTION ( 'NONE',  ( -0.8660254037844387076, -0.4999999999999998890, -0.000000000000000000 ) ) ;
#1957=CARTESIAN_POINT ( 'NONE',  ( 86.60116260073726835, 209.2592609112380160, 2.679491924311254714 ) ) ;
#1960=CARTESIAN_POINT ( 'NONE',  ( 180.8890834033174713, 294.3766012452771861, 6.559837412958372305 ) ) ;
#1961=( BOUNDED_CURVE ( )  B_SPLINE_CURVE ( 2, ( #31273, #15561, #30791, #76407, #8487, #15070, #23662, #38367, #37374 ),
 .UNSPECIFIED., .F., .T. ) 
 B_SPLINE_CURVE_WITH_KNOTS ( ( 3, 2, 2, 2, 3 ),
 ( 0.2782258064516128782, 0.2795698924731182533, 0.2822580645161290591, 0.2849462365591398094, 0.2862903225806451846 ),
 .UNSPECIFIED. ) 
 CURVE ( )  GEOMETRIC_REPRESENTATION_ITEM ( )  RATIONAL_B_SPLINE_CURVE ( ( 0.9330127018922194093, 0.9330127018922194093, 1.000000000000000000, 0.8660254037844387076, 1.000000000000000000, 0.8660254037844387076, 1.000000000000000000, 0.9330127018922194093, 0.9330127018922194093 ) ) 
 REPRESENTATION_ITEM ( '' )  );
#1963=CARTESIAN_POINT ( 'NONE',  ( 148.0346525705264469, 274.2434557974783615, -9.381294579651672905 ) ) ;
#1964=CARTESIAN_POINT ( 'NONE',  ( 208.2124092825819162, 270.0125236866795149, -2.339659020816897694 ) ) ;
#1965=CARTESIAN_POINT ( 'NONE',  ( 155.0303156110108489, 262.1266119787277944, 17.11986653161320859 ) ) ;
#1967=CARTESIAN_POINT ( 'NONE',  ( 205.2660270307054304, 275.1158074454486382, -13.97598661256119179 ) ) ;
#1968=CARTESIAN_POINT ( 'NONE',  ( 208.0280121190496629, 270.3319089426888127, -3.803189352412944757 ) ) ;
#1969=CARTESIAN_POINT ( 'NONE',  ( 206.4633727170604232, 270.6208656945399866, 2.462764060182144554 ) ) ;
#1971=CARTESIAN_POINT ( 'NONE',  ( 91.08134800299070832, 214.2048013555409796, 4.594050593750051981 ) ) ;
#1973=CARTESIAN_POINT ( 'NONE',  ( 151.0036289208911171, 269.1010379121764799, 14.24595189915657478 ) ) ;
#1976=ORIENTED_EDGE ( 'NONE', *, *, #55649, .F. ) ;
#1977=VECTOR ( 'NONE', #48677, 1000.000000000000114 ) ;
#1978=CARTESIAN_POINT ( 'NONE',  ( 195.3813422720796780, 292.2365836641902774, -16.04365517931749707 ) ) ;
#1979=ORIENTED_EDGE ( 'NONE', *, *, #89670, .F. ) ;
#1983=B_SPLINE_SURFACE_WITH_KNOTS ( 'NONE', 3, 1, ( 
 ( #70286, #13727 ),
 ( #31288, #62175 ),
 ( #54570, #898 ),
 ( #44604, #16095 ),
 ( #77913, #75538 ),
 ( #13252, #6123 ),
 ( #28421, #51216 ),
 ( #75048, #44109 ),
 ( #46999, #20345 ),
 ( #37020, #5137 ),
 ( #67419, #89772 ),
 ( #59300, #8502 ),
 ( #90280, #98348 ),
 ( #28938, #21332 ),
 ( #91260, #59815 ),
 ( #33818, #70804 ),
 ( #18611, #24691 ),
 ( #10499, #63194 ),
 ( #25711, #56072 ),
 ( #55573, #56590 ),
 ( #47981, #93633 ),
 ( #79444, #64195 ),
 ( #1908, #88062 ),
 ( #25190, #10009 ),
 ( #95146, #32293 ),
 ( #87065, #57083 ),
 ( #2928, #86557 ),
 ( #41890, #94633 ),
 ( #32789, #49489 ),
 ( #87579, #17089 ),
 ( #55081, #1412 ),
 ( #18104, #17597 ),
 ( #64705, #33293 ),
 ( #80446, #8995 ) ),
 .UNSPECIFIED., .T., .F., .F.,
 ( 4, 2, 2, 2, 2, 2, 2, 2, 2, 2, 2, 2, 2, 2, 2, 2, 4 ),
 ( 2, 2 ),
 ( 0.000000000000000000, 0.06250000000000000000, 0.1250000000000000000, 0.1875000000000000000, 0.2500000000000000000, 0.3125000000000000000, 0.3750000000000000000, 0.4375000000000000000, 0.5000000000000000000, 0.5625000000000000000, 0.6250000000000000000, 0.6875000000000000000, 0.7500000000000000000, 0.8125000000000000000, 0.8750000000000000000, 0.9375000000000000000, 1.000000000000000000 ),
 ( 0.000000000000000000, 1.000000000000000000 ),
 .UNSPECIFIED. ) ;
#1986=CARTESIAN_POINT ( 'NONE',  ( 162.6859166034911652, 248.8667220972772611, 10.26171246773997758 ) ) ;
#1987=CARTESIAN_POINT ( 'NONE',  ( 75.46539357129627490, 220.5024278399160664, -9.188101187500093303 ) ) ;
#1988=ORIENTED_EDGE ( 'NONE', *, *, #92550, .F. ) ;
#1990=CARTESIAN_POINT ( 'NONE',  ( 200.7664336291577172, 282.9093318303307569, -18.32876612325386034 ) ) ;
#1991=ORIENTED_EDGE ( 'NONE', *, *, #49837, .F. ) ;
#1993=EDGE_CURVE ( 'NONE', #19180, #39829, #83364, .T. ) ;
#1994=CARTESIAN_POINT ( 'NONE',  ( 165.4345553874274799, 285.6554192157983039, 1.183051567514476599 ) ) ;
#1998=CARTESIAN_POINT ( 'NONE',  ( 188.6991936886695953, 294.9304948621235667, 11.61111646670225106 ) ) ;
#1999=CARTESIAN_POINT ( 'NONE',  ( 156.7504469567443550, 274.0276245742728634, 13.42060143992435428 ) ) ;
#2000=CARTESIAN_POINT ( 'NONE',  ( 159.9531724557437826, 253.5999738052623229, -15.71074128491364874 ) ) ;
#2001=CARTESIAN_POINT ( 'NONE',  ( 155.6583371091562640, 262.5339888893300895, -17.25629704915573015 ) ) ;
#2002=CARTESIAN_POINT ( 'NONE',  ( 175.2754180912867241, 284.4784848018189223, 14.01285901753186458 ) ) ;
#2003=FACE_OUTER_BOUND ( 'NONE', #31225, .T. ) ;
#2004=CARTESIAN_POINT ( 'NONE',  ( 195.4167945326838378, 279.6122101856814197, -17.17760159917481744 ) ) ;
#2007=CARTESIAN_POINT ( 'NONE',  ( 161.1089126327036354, 251.5981730984191529, 13.95161017039218976 ) ) ;
#2009=CARTESIAN_POINT ( 'NONE',  ( 170.9817807944941137, 251.5856905545531959, 7.058976180640677001 ) ) ;
#2011=CARTESIAN_POINT ( 'NONE',  ( 202.4721870783228894, 268.0718720055712083, 5.348787301547115902 ) ) ;
#2012=EDGE_CURVE ( 'NONE', #64801, #80515, #62589, .T. ) ;
#2013=CARTESIAN_POINT ( 'NONE',  ( 153.2026299055073650, 270.4964049230587761, 13.90442887244355497 ) ) ;
#2014=ORIENTED_EDGE ( 'NONE', *, *, #42285, .T. ) ;
#2016=CARTESIAN_POINT ( 'NONE',  ( 179.8355924322922590, 266.3652243622770470, -14.78567419157851504 ) ) ;
#2018=CARTESIAN_POINT ( 'NONE',  ( 185.0402102251197789, 257.2940728988994579, 2.699890041601303192 ) ) ;
#2020=DIRECTION ( 'NONE',  ( -0.8660254037844387076, -0.4999999999999998890, -0.000000000000000000 ) ) ;
#2021=EDGE_CURVE ( 'NONE', #87939, #4112, #98188, .T. ) ;
#2022=CARTESIAN_POINT ( 'NONE',  ( 172.3175038124396110, 275.1038600624426067, 16.61276981194052738 ) ) ;
#2023=CARTESIAN_POINT ( 'NONE',  ( 183.7733247487505253, 274.9862421907877206, 16.36274383044956693 ) ) ;
#2025=CARTESIAN_POINT ( 'NONE',  ( 192.1810643495398665, 262.2731238949148178, 2.987946743577344133 ) ) ;
#2026=CARTESIAN_POINT ( 'NONE',  ( 207.8792014703394671, 270.5896565469619759, -5.780233892547864905 ) ) ;
#2027=CARTESIAN_POINT ( 'NONE',  ( -9.892408837089961438, 177.3464784336661637, 1.353441290958777327E-15 ) ) ;
#2029=ORIENTED_EDGE ( 'NONE', *, *, #232, .F. ) ;
#2030=CARTESIAN_POINT ( 'NONE',  ( 174.9122443831272165, 255.2793860169833522, 8.300717241462230334 ) ) ;
#2032=CARTESIAN_POINT ( 'NONE',  ( 208.3117541397001844, 269.8404533466799080, 2.895672523916592578 ) ) ;
#2034=CARTESIAN_POINT ( 'NONE',  ( 15.38488118375084390, 185.8149278399160949, -9.188101187500095079 ) ) ;
#2036=FACE_OUTER_BOUND ( 'NONE', #13697, .T. ) ;
#2038=B_SPLINE_CURVE_WITH_KNOTS ( 'NONE', 3,
 ( #95873, #2133, #9746, #48219, #25414, #86781, #56306, #87795, #86278, #18337, #16814, #93865, #10230, #17835, #24422, #33016, #49231, #47701, #9222, #64422, #25937, #63915, #40099, #26430, #48735, #80165, #40605, #79668, #10732, #57310, #42109, #41606, #71040, #95385, #32527, #32004, #88280, #18833, #80669, #1643, #94360, #24914, #55788, #17315, #44087, #28921, #52193, #5119, #19353, #35999, #90764, #51199 ),
 .UNSPECIFIED., .F., .F.,
 ( 4, 2, 2, 2, 2, 2, 2, 2, 2, 2, 2, 2, 2, 2, 2, 2, 2, 2, 2, 2, 2, 2, 2, 2, 2, 4 ),
 ( 0.0004155875641910399465, 0.0008752706911513232803, 0.001105112254631483758, 0.001334953818111644236, 0.001449874599851724150, 0.001564795381591804063, 0.001679716163331883977, 0.001794636945071964324, 0.002024478508552008792, 0.002254320072032053261, 0.003173686325952355166, 0.004093052579872656638, 0.005012418833792958543, 0.005472101960753063959, 0.005701943524233080672, 0.005816864305973089462, 0.005874324696843134623, 0.005931785087713179784, 0.005989245478583224945, 0.006046705869453270106, 0.006161626651193358693, 0.006391468214673476020, 0.006851151341633709806, 0.007310834468593942724, 0.007540676032074041836, 0.007770517595554140081 ),
 .UNSPECIFIED. ) ;
#2039=CARTESIAN_POINT ( 'NONE',  ( 199.5313597256959781, 267.4056706038007292, -6.663851089317214260 ) ) ;
#2040=CARTESIAN_POINT ( 'NONE',  ( 173.5268431453002620, 273.0267676714563549, -16.40558794790413444 ) ) ;
#2044=ADVANCED_FACE ( 'NONE', ( #94305 ), #46909, .F. ) ;
#2045=CARTESIAN_POINT ( 'NONE',  ( 186.8369214609370488, 295.7978260411641713, -8.160117540320300122 ) ) ;
#2046=AXIS2_PLACEMENT_3D ( 'NONE', #13651, #66837, #83081 ) ;
#2049=CARTESIAN_POINT ( 'NONE',  ( 182.6352093130429068, 296.5685661505265784, 1.834901431546525297 ) ) ;
#2050=CARTESIAN_POINT ( 'NONE',  ( 85.83080867249778123, 210.3615022471902023, 5.000000000000051514 ) ) ;
#2052=CARTESIAN_POINT ( 'NONE',  ( 161.8935460472482930, 280.0887632390822546, 11.41936692958946509 ) ) ;
#2053=CARTESIAN_POINT ( 'NONE',  ( 170.2529524909020324, 288.7139002527517277, 5.426736320396455149 ) ) ;
#2054=CARTESIAN_POINT ( 'NONE',  ( 47.96943409690536697, 192.3768266524160140, 9.188101187500098632 ) ) ;
#2056=CARTESIAN_POINT ( 'NONE',  ( 203.7093853360854894, 270.4153380413875993, -6.448685755690142685 ) ) ;
#2057=CARTESIAN_POINT ( 'NONE',  ( 147.5498377207569263, 275.0831797495432056, 4.097967709737811326 ) ) ;
#2060=ORIENTED_EDGE ( 'NONE', *, *, #27585, .T. ) ;
#2064=CARTESIAN_POINT ( 'NONE',  ( 147.1674053649995528, 275.7455720201731424, 6.878590988502374159 ) ) ;
#2067=CARTESIAN_POINT ( 'NONE',  ( 162.8996025780091941, 248.4966071325470125, 11.23567065566008516 ) ) ;
#2068=CARTESIAN_POINT ( 'NONE',  ( 149.1486417047969155, 272.3139700178423368, -11.47583619705022606 ) ) ;
#2069=CARTESIAN_POINT ( 'NONE',  ( 188.9913214560809536, 269.9620198908939415, -15.45701251956971944 ) ) ;
#2071=B_SPLINE_CURVE_WITH_KNOTS ( 'NONE', 3,
 ( #43014, #33970, #96281, #50142, #11662, #66341, #42524, #73458, #4041, #65826, #73952, #27841, #48660, #3080, #98762, #14639, #67332, #66832, #59725, #91667, #36424, #84088, #45519, #97760, #35930, #82090, #14138, #98256, #6543, #6034, #28330, #75450, #68821, #36929, #60210, #37418, #59207, #90691, #76450, #68324, #20757, #99250, #60706, #90182, #29345, #7027, #28845, #51645 ),
 .UNSPECIFIED., .F., .F.,
 ( 4, 2, 2, 2, 2, 2, 2, 2, 2, 2, 2, 2, 2, 2, 2, 2, 2, 2, 2, 2, 2, 2, 2, 4 ),
 ( 0.0007362855887611816693, 0.0009426974782739958644, 0.001149109367786810059, 0.001252315312543195690, 0.001355521257299581537, 0.001561933146812410911, 0.001974756925838208003, 0.002387580704864005095, 0.003213228262915446623, 0.004038875820966888151, 0.004864523379018329680, 0.005277347158044092511, 0.005483759047556896297, 0.005586964992313334620, 0.005638567964691484392, 0.005690170937069634165, 0.005793376881825774115, 0.005896582826581914065, 0.006102994716094055187, 0.006515818495118457995, 0.006722230384630654629, 0.006928642274142851262, 0.007135054163655047896, 0.007341466053167244529 ),
 .UNSPECIFIED. ) ;
#2074=CARTESIAN_POINT ( 'NONE',  ( 198.4226516368227067, 264.7884397865803408, 0.06761542484275395726 ) ) ;
#2077=ADVANCED_FACE ( 'NONE', ( #39367 ), #10005, .T. ) ;
#2079=FACE_OUTER_BOUND ( 'NONE', #90824, .T. ) ;
#2080=CARTESIAN_POINT ( 'NONE',  ( 150.6487462746963502, 269.7157126861102370, 15.18501655901553704 ) ) ;
#2082=CARTESIAN_POINT ( 'NONE',  ( 190.0896302098338424, 301.4020978150248311, 3.433521196325825642 ) ) ;
#2084=CARTESIAN_POINT ( 'NONE',  ( 186.2533614392526715, 272.0223876180238562, -16.20928411658415769 ) ) ;
#2085=CARTESIAN_POINT ( 'NONE',  ( 183.4553195968295256, 297.0403188216897661, -2.838562726794640056 ) ) ;
#2087=CARTESIAN_POINT ( 'NONE',  ( 152.7295469705997277, 266.1116601603806657, -17.40211458100010589 ) ) ;
#2088=CARTESIAN_POINT ( 'NONE',  ( 175.3074307085254020, 254.5436327766159650, 9.407465564047683415 ) ) ;
#2092=CARTESIAN_POINT ( 'NONE',  ( 157.4211152037729562, 257.9856256133486454, -16.71526195140576831 ) ) ;
#2093=CARTESIAN_POINT ( 'NONE',  ( 98.52366704282199805, 221.5643266524159856, -9.188101187500093303 ) ) ;
#2094=B_SPLINE_CURVE_WITH_KNOTS ( 'NONE', 3,
 ( #88328, #34559, #34083, #88831, #89322, #81699 ),
 .UNSPECIFIED., .F., .F.,
 ( 4, 2, 4 ),
 ( 0.001541644710436317414, 0.001826678494032424977, 0.002111712277628532541 ),
 .UNSPECIFIED. ) ;
#2095=CARTESIAN_POINT ( 'NONE',  ( 184.0096797657860179, 289.1861371066262905, -13.00318607164890494 ) ) ;
#2100=CARTESIAN_POINT ( 'NONE',  ( 159.4574711498080433, 254.4585536525209477, 16.86100557095418395 ) ) ;
#2102=CARTESIAN_POINT ( 'NONE',  ( 65.42534541587671981, 199.3923013555409796, 4.594050593750050204 ) ) ;
#2104=CARTESIAN_POINT ( 'NONE',  ( 150.7226148805041817, 269.5877685077668957, 15.52819754351937576 ) ) ;
#2105=CARTESIAN_POINT ( 'NONE',  ( 150.4319008355389542, 270.0913000041206260, 13.83804576328048697 ) ) ;
#2106=CARTESIAN_POINT ( 'NONE',  ( 172.6732692711807147, 271.7370492138056761, 16.73332340419656461 ) ) ;
#2107=EDGE_LOOP ( 'NONE', ( #36555, #33108, #78838, #5603, #26273, #97174, #217, #80248, #20760, #70554, #64523, #79355, #35597, #90155, #96285, #63008, #99410, #19525, #46811, #50604 ) ) ;
#2110=CARTESIAN_POINT ( 'NONE',  ( 177.1723795352289130, 288.8195398279596589, 11.30650638855078327 ) ) ;
#2111=DIRECTION ( 'NONE',  ( -0.8660254037844359321, -0.5000000000000051070, -0.000000000000000000 ) ) ;
#2113=CARTESIAN_POINT ( 'NONE',  ( 172.1042385749445032, 259.7490272540697447, -13.86291087914393039 ) ) ;
#2114=CARTESIAN_POINT ( 'NONE',  ( 174.0496840832364569, 277.6969804377837931, -15.67051255850419444 ) ) ;
#2116=CARTESIAN_POINT ( 'NONE',  ( 193.0142717932987182, 296.3364699985351081, -13.30037542329744937 ) ) ;
#2117=CARTESIAN_POINT ( 'NONE',  ( 190.4841013044967042, 300.7188538369516095, 4.682298117523464143 ) ) ;
#2118=AXIS2_PLACEMENT_3D ( 'NONE', #61696, #17102, #69309 ) ;
#2119=CARTESIAN_POINT ( 'NONE',  ( 177.3509020185674103, 269.5276210205321945, 16.09886373478537180 ) ) ;
#2120=ADVANCED_FACE ( 'NONE', ( #62170 ), #8990, .T. ) ;
#2121=CARTESIAN_POINT ( 'NONE',  ( -22.42236680055709641, 157.8615022471902591, 0.000000000000000000 ) ) ;
#2125=CARTESIAN_POINT ( 'NONE',  ( 102.9345500736427113, 239.4244531367911293, -4.594050593750046652 ) ) ;
#2127=CARTESIAN_POINT ( 'NONE',  ( 191.0862225170008628, 299.6759493045793192, -9.402218231374108726 ) ) ;
#2130=CARTESIAN_POINT ( 'NONE',  ( 155.3513572141771704, 261.5705516107003064, -17.00592413546589299 ) ) ;
#2131=CARTESIAN_POINT ( 'NONE',  ( 164.0741338217690668, 246.4622593432776796, 7.359073626423302983 ) ) ;
#2133=CARTESIAN_POINT ( 'NONE',  ( 175.7490893856983689, 252.6561874605901608, 5.270972134136622245 ) ) ;
#2136=B_SPLINE_CURVE_WITH_KNOTS ( 'NONE', 3,
 ( #3952, #18667, #96194, #40927, #95713, #57137 ),
 .UNSPECIFIED., .F., .F.,
 ( 4, 2, 4 ),
 ( 0.0007689256722880135090, 0.001136985650662513314, 0.001505045629037013010 ),
 .UNSPECIFIED. ) ;
#2138=CARTESIAN_POINT ( 'NONE',  ( 181.9589692923136113, 260.5425098207756491, 9.737347583194500444 ) ) ;
#2139=CARTESIAN_POINT ( 'NONE',  ( 206.5266458972945429, 272.9323515195362120, -9.802257691457246125 ) ) ;
#2140=CARTESIAN_POINT ( 'NONE',  ( 146.0739611433025686, 245.9548013555409796, -4.594050593750042211 ) ) ;
#2142=CARTESIAN_POINT ( 'NONE',  ( 150.8247211172754589, 269.4109153179094278, -14.37608026040300402 ) ) ;
#2143=CIRCLE ( 'NONE', #15053, 17.82106496071138224 ) ;
#2144=CARTESIAN_POINT ( 'NONE',  ( 189.1275178940386752, 299.7030702647930411, 4.939670191479129890 ) ) ;
#2146=CARTESIAN_POINT ( 'NONE',  ( 62.50250967810423930, 197.7048013555409796, 4.594050593750051981 ) ) ;
#2148=CARTESIAN_POINT ( 'NONE',  ( 205.2414727015710412, 275.1583367910551488, -12.71338796362297963 ) ) ;
#2150=EDGE_CURVE ( 'NONE', #39162, #45893, #11517, .T. ) ;
#2151=B_SPLINE_CURVE_WITH_KNOTS ( 'NONE', 3,
 ( #21256, #60218, #75459, #36940, #91182, #21743, #52627, #45034, #32339, #56638, #79489, #62724, #71864, #86601, #31823, #86109 ),
 .UNSPECIFIED., .F., .F.,
 ( 4, 2, 2, 2, 2, 2, 2, 4 ),
 ( 0.0005595848447356708590, 0.0008683227071104232054, 0.001177060569485175552, 0.001485798431859928007, 0.001794536294234680245, 0.002103274156609432483, 0.002412012018984184721, 0.003029487743733707845 ),
 .UNSPECIFIED. ) ;
#2154=CARTESIAN_POINT ( 'NONE',  ( 174.3956825652301461, 262.1553256887494854, 14.35235884442154308 ) ) ;
#2155=CARTESIAN_POINT ( 'NONE',  ( 155.1820006974310218, 279.5632244157534387, -1.579113261361717369 ) ) ;
#2156=CARTESIAN_POINT ( 'NONE',  ( 178.8091420268403908, 291.8339325867452771, -6.888020678422202003 ) ) ;
#2157=CARTESIAN_POINT ( 'NONE',  ( 155.6569868912636991, 261.0411854816857158, -17.75433477650897984 ) ) ;
#2158=CARTESIAN_POINT ( 'NONE',  ( 178.6208630460672282, 261.2445556773918156, 12.21686540733617754 ) ) ;
#2159=CARTESIAN_POINT ( 'NONE',  ( 128.9696990949622659, 235.2677522451417929, -5.000000000000041744 ) ) ;
#2162=CARTESIAN_POINT ( 'NONE',  ( 189.9457600613112902, 301.6512882219586800, 0.04117870562599101891 ) ) ;
#2163=CARTESIAN_POINT ( 'NONE',  ( -15.79203335248894469, 167.8149278399160949, -9.188101187500095079 ) ) ;
#2164=CARTESIAN_POINT ( 'NONE',  ( 46.56214281575564939, 191.5643266524159856, -9.188101187500093303 ) ) ;
#2166=CARTESIAN_POINT ( 'NONE',  ( 32.38751264475774860, 201.0530062829863027, -4.648177544792955347E-16 ) ) ;
#2168=CARTESIAN_POINT ( 'NONE',  ( 190.4976253092930278, 300.6954295735222900, -5.764807383508308902 ) ) ;
#2170=ADVANCED_FACE ( 'NONE', ( #58089 ), #90025, .T. ) ;
#2171=CARTESIAN_POINT ( 'NONE',  ( 198.0787076940555949, 277.7817408258703722, -16.06897465026475658 ) ) ;
#2172=CARTESIAN_POINT ( 'NONE',  ( 64.52297529667023923, 201.3927522451418213, 10.00000000000009592 ) ) ;
#2174=CARTESIAN_POINT ( 'NONE',  ( 184.5677135434892193, 257.8300269524731334, 1.356526893385950006 ) ) ;
#2175=CARTESIAN_POINT ( 'NONE',  ( 157.8159121039657293, 257.3018173235443555, -17.05074702406642118 ) ) ;
#2177=ORIENTED_EDGE ( 'NONE', *, *, #46472, .F. ) ;
#2179=CARTESIAN_POINT ( 'NONE',  ( 34.80747863286459420, 184.2365022471902023, 10.00000000000009592 ) ) ;
#2181=CARTESIAN_POINT ( 'NONE',  ( 202.4323889586180201, 280.0238125565655878, 15.69595176008160919 ) ) ;
#2182=CARTESIAN_POINT ( 'NONE',  ( 142.3387059458346755, 262.1744531367911009, 4.594050593750047540 ) ) ;
#2184=CARTESIAN_POINT ( 'NONE',  ( 164.3186433446439878, 252.3970802647851315, 13.58250517929732659 ) ) ;
#2185=CARTESIAN_POINT ( 'NONE',  ( 170.3204754281883879, 263.6398627415188116, 15.82658840592242022 ) ) ;
#2188=CARTESIAN_POINT ( 'NONE',  ( 205.8379285891498682, 274.1252448892948905, 10.44730901608240181 ) ) ;
#2189=CARTESIAN_POINT ( 'NONE',  ( 185.7240582157602091, 259.0518005378353337, -2.331041323071082250 ) ) ;
#2193=CARTESIAN_POINT ( 'NONE',  ( 188.1018771210319471, 260.4230313274653099, 6.875771660441075461 ) ) ;
#2194=CARTESIAN_POINT ( 'NONE',  ( 195.2495212664957194, 275.1290853193528392, -16.26662379558266380 ) ) ;
#2196=CARTESIAN_POINT ( 'NONE',  ( 166.1085421714060431, 285.6684600996341032, 0.4957535612788783186 ) ) ;
#2198=CARTESIAN_POINT ( 'NONE',  ( 160.4797372417389454, 252.6879368424417294, 16.11078530976836731 ) ) ;
#2201=CARTESIAN_POINT ( 'NONE',  ( 152.9031728309432765, 274.9703759552688780, 10.73379579711528820 ) ) ;
#2202=CARTESIAN_POINT ( 'NONE',  ( 159.9770824720811220, 253.5585604421560788, -16.42166711341322483 ) ) ;
#2205=CARTESIAN_POINT ( 'NONE',  ( 207.6209998424140792, 271.0368748851258260, 6.610167240481342965 ) ) ;
#2207=CARTESIAN_POINT ( 'NONE',  ( 162.7738416911812180, 248.7144313781379310, -11.09964294874192525 ) ) ;
#2208=CARTESIAN_POINT ( 'NONE',  ( 154.8596847415876994, 262.4221533139083817, 17.65401077761399762 ) ) ;
#2209=ORIENTED_EDGE ( 'NONE', *, *, #23725, .T. ) ;
#2211=CARTESIAN_POINT ( 'NONE',  ( 156.0423484674798829, 277.4799991307274922, -10.51687751763815726 ) ) ;
#2216=CARTESIAN_POINT ( 'NONE',  ( 155.3895351254020625, 262.3183883289777896, -17.15772230249129393 ) ) ;
#2217=ORIENTED_EDGE ( 'NONE', *, *, #99968, .F. ) ;
#2222=ORIENTED_EDGE ( 'NONE', *, *, #85455, .T. ) ;
#2223=CARTESIAN_POINT ( 'NONE',  ( 200.4775477985258760, 283.4096967665721536, 16.80647240730505487 ) ) ;
#2224=CARTESIAN_POINT ( 'NONE',  ( 166.1020561509257902, 274.0512672971645429, -15.22686407272243336 ) ) ;
#2225=CARTESIAN_POINT ( 'NONE',  ( 164.2059258710715994, 246.2339888178522926, 7.329631442356459914 ) ) ;
#2226=CARTESIAN_POINT ( 'NONE',  ( 151.4086371529806740, 275.0624268371906282, -8.516296556100446224 ) ) ;
#2229=CARTESIAN_POINT ( 'NONE',  ( 170.9015845831005436, 255.7403565480592533, -11.60269983186427467 ) ) ;
#2231=EDGE_LOOP ( 'NONE', ( #47227, #68601, #60703, #89435 ) ) ;
#2234=ORIENTED_EDGE ( 'NONE', *, *, #80199, .F. ) ;
#2235=CARTESIAN_POINT ( 'NONE',  ( 160.9377252177449975, 270.8987565486240783, 15.95750095843152039 ) ) ;
#2236=VERTEX_POINT ( 'NONE', #79936 ) ;
#2238=CARTESIAN_POINT ( 'NONE',  ( 168.5704745160775246, 272.7448807985149415, 15.97903247022720485 ) ) ;
#2240=DIRECTION ( 'NONE',  ( -0.8660254037844387076, -0.4999999999999998890, -0.000000000000000000 ) ) ;
#2243=CARTESIAN_POINT ( 'NONE',  ( 174.5780023577881082, 290.2779860773731002, 6.405149012862879410 ) ) ;
#2245=ORIENTED_EDGE ( 'NONE', *, *, #94471, .F. ) ;
#2246=CARTESIAN_POINT ( 'NONE',  ( 157.9225728654248257, 276.1116997103654285, -12.95724163227552239 ) ) ;
#2249=CARTESIAN_POINT ( 'NONE',  ( 197.9952413503812352, 287.7091776547143809, 17.17611241386010690 ) ) ;
#2250=VERTEX_POINT ( 'NONE', #35286 ) ;
#2251=ORIENTED_EDGE ( 'NONE', *, *, #23354, .F. ) ;
#2254=CARTESIAN_POINT ( 'NONE',  ( 159.3995226465659982, 254.5589234043588078, -16.81133486613867234 ) ) ;
#2256=CARTESIAN_POINT ( 'NONE',  ( 200.5621507313343557, 283.2631601884785368, 16.81037192529623425 ) ) ;
#2258=ORIENTED_EDGE ( 'NONE', *, *, #93815, .T. ) ;
#2259=CARTESIAN_POINT ( 'NONE',  ( 153.0051671234592163, 269.7671913317512917, 15.26340949627251042 ) ) ;
#2263=CARTESIAN_POINT ( 'NONE',  ( 6.860117161356284576, 184.7677522451419065, -5.000000000000047962 ) ) ;
#2264=CARTESIAN_POINT ( 'NONE',  ( 90.72909131299699936, 229.3149278399160949, -9.188101187500095079 ) ) ;
#2265=EDGE_CURVE ( 'NONE', #61940, #28329, #66575, .T. ) ;
#2268=FACE_OUTER_BOUND ( 'NONE', #2590, .T. ) ;
#2269=CARTESIAN_POINT ( 'NONE',  ( 4.992576338337581632, 179.8149278399160949, -9.188101187500095079 ) ) ;
#2271=CIRCLE ( 'NONE', #89654, 17.82106496071138935 ) ;
#2272=CARTESIAN_POINT ( 'NONE',  ( 200.1103929410127762, 284.0456276340304953, 17.67835211026828901 ) ) ;
#2274=ORIENTED_EDGE ( 'NONE', *, *, #36758, .F. ) ;
#2275=CARTESIAN_POINT ( 'NONE',  ( 200.8494367518017611, 267.7546157101949689, -2.866440153229757648 ) ) ;
#2277=( BOUNDED_CURVE ( )  B_SPLINE_CURVE ( 2, ( #72348, #57102, #10529, #63216, #41404, #17110, #97508, #32315, #25213 ),
 .UNSPECIFIED., .F., .T. ) 
 B_SPLINE_CURVE_WITH_KNOTS ( ( 3, 2, 2, 2, 3 ),
 ( 0.6653225806451612545, 0.6666666666666666297, 0.6693548387096773800, 0.6720430107526881303, 0.6733870967741935054 ),
 .UNSPECIFIED. ) 
 CURVE ( )  GEOMETRIC_REPRESENTATION_ITEM ( )  RATIONAL_B_SPLINE_CURVE ( ( 0.9330127018922194093, 0.9330127018922194093, 1.000000000000000000, 0.8660254037844387076, 1.000000000000000000, 0.8660254037844387076, 1.000000000000000000, 0.9330127018922194093, 0.9330127018922194093 ) ) 
 REPRESENTATION_ITEM ( '' )  );
#2279=EDGE_CURVE ( 'NONE', #8428, #64780, #93724, .T. ) ;
#2283=CARTESIAN_POINT ( 'NONE',  ( 185.8590724889926378, 286.6100872548933012, 15.79318560268085037 ) ) ;
#2284=CARTESIAN_POINT ( 'NONE',  ( 174.9671601572613326, 281.6994072225486434, -15.63500919100072473 ) ) ;
#2285=CARTESIAN_POINT ( 'NONE',  ( 32.16412338207434374, 195.5024278399160949, 9.188101187500095079 ) ) ;
#2286=CARTESIAN_POINT ( 'NONE',  ( 73.18322933451453594, 226.3927522451419350, 2.944929066748280225E-16 ) ) ;
#2288=CARTESIAN_POINT ( 'NONE',  ( 93.02964483790795214, 234.5177522451419350, 5.000000000000046185 ) ) ;
#2292=CARTESIAN_POINT ( 'NONE',  ( 175.5827251679224617, 251.6158941198623040, 0.7410290085531462401 ) ) ;
#2293=CARTESIAN_POINT ( 'NONE',  ( -5.399381411310668177, 161.5643266524160140, -9.188101187500093303 ) ) ;
#2295=DIRECTION ( 'NONE',  ( -0.4330127018922184656, -0.2499999999999943934, -0.8660254037844407060 ) ) ;
#2296=CARTESIAN_POINT ( 'NONE',  ( 186.7612184996281144, 282.7283756238621777, 16.18745214556588863 ) ) ;
#2297=CARTESIAN_POINT ( 'NONE',  ( 194.3541845315608612, 294.0156730581561533, -14.67567721756631016 ) ) ;
#2299=CARTESIAN_POINT ( 'NONE',  ( 204.7610021263893429, 275.9905362388115577, 13.36619428527026976 ) ) ;
#2300=CARTESIAN_POINT ( 'NONE',  ( 147.2784190576484491, 275.5532906641692534, 0.2793038414862047958 ) ) ;
#2301=CARTESIAN_POINT ( 'NONE',  ( 148.3280470635002928, 273.7352816289870248, 9.058704604771318003 ) ) ;
#2302=ORIENTED_EDGE ( 'NONE', *, *, #92503, .F. ) ;
#2303=EDGE_CURVE ( 'NONE', #30511, #19593, #61709, .T. ) ;
#2304=CARTESIAN_POINT ( 'NONE',  ( 8.321535033790441460, 185.6115022471903160, -5.000000000000047962 ) ) ;
#2305=CARTESIAN_POINT ( 'NONE',  ( 108.0499464844507997, 227.0643266524160424, 9.188101187500095079 ) ) ;
#2308=CARTESIAN_POINT ( 'NONE',  ( 40.63510790894943625, 194.2677522451418781, 10.00000000000009592 ) ) ;
#2309=CARTESIAN_POINT ( 'NONE',  ( 195.9713281756800427, 291.2146981034049418, 17.52210387885178022 ) ) ;
#2310=CARTESIAN_POINT ( 'NONE',  ( 162.1227137712282342, 251.8422180177273901, -14.11218862277787345 ) ) ;
#2312=CARTESIAN_POINT ( 'NONE',  ( 150.8963010474469684, 269.2869352420495943, -15.14557988994318016 ) ) ;
#2313=DIRECTION ( 'NONE',  ( 0.4999999999999998890, -0.8660254037844385966, 0.000000000000000000 ) ) ;
#2314=CARTESIAN_POINT ( 'NONE',  ( 149.1939152435731728, 272.2355539484436235, -11.44223522189843933 ) ) ;
#2316=CARTESIAN_POINT ( 'NONE',  ( 204.0100964097678968, 276.7670827000571876, 13.67351780134896266 ) ) ;
#2319=CARTESIAN_POINT ( 'NONE',  ( 189.3522642941718743, 265.7560121150649479, 10.75527977382243527 ) ) ;
#2320=CARTESIAN_POINT ( 'NONE',  ( 177.7074169911321349, 279.7993272485674652, 15.60716354588072718 ) ) ;
#2321=CARTESIAN_POINT ( 'NONE',  ( 165.7666411575162329, 269.9458407505568402, -16.28142105735056333 ) ) ;
#2322=EDGE_CURVE ( 'NONE', #76205, #22170, #43600, .T. ) ;
#2327=CARTESIAN_POINT ( 'NONE',  ( 152.8134625983922490, 265.9663140294953791, 17.57333028169644251 ) ) ;
#2328=CARTESIAN_POINT ( 'NONE',  ( -22.42236680055709641, 157.8615022471902591, 0.000000000000000000 ) ) ;
#2330=CARTESIAN_POINT ( 'NONE',  ( 187.4322965893034905, 284.5321960278562301, 17.17379807122665625 ) ) ;
#2331=VERTEX_POINT ( 'NONE', #7882 ) ;
#2332=CARTESIAN_POINT ( 'NONE',  ( 167.8081459420055523, 280.8398059720881861, 11.95526808680748942 ) ) ;
#2333=CARTESIAN_POINT ( 'NONE',  ( 148.3625667886952044, 273.6754917110858401, -8.960758510948144462 ) ) ;
#2337=CARTESIAN_POINT ( 'NONE',  ( 188.6646623341742668, 293.7383209822070285, 12.96511213459449863 ) ) ;
#2340=CARTESIAN_POINT ( 'NONE',  ( 202.8535267948003593, 279.2943804273081696, -15.36804658072946062 ) ) ;
#2342=B_SPLINE_CURVE_WITH_KNOTS ( 'NONE', 3,
 ( #81861, #2853, #33743, #87507, #18040, #57012, #87991, #18539, #89958, #45304 ),
 .UNSPECIFIED., .F., .F.,
 ( 4, 2, 2, 2, 4 ),
 ( 0.001222343323482912199, 0.001313399527160096208, 0.001404455730837280217, 0.001586568138191648235, 0.001950792952900384488 ),
 .UNSPECIFIED. ) ;
#2343=VERTEX_POINT ( 'NONE', #85938 ) ;
#2345=ORIENTED_EDGE ( 'NONE', *, *, #52749, .T. ) ;
#2353=CARTESIAN_POINT ( 'NONE',  ( 185.7214944442812907, 282.3173832595768431, -17.29588648652288185 ) ) ;
#2354=CARTESIAN_POINT ( 'NONE',  ( 164.5379227956242687, 245.6589532765702870, -2.440899697315300987 ) ) ;
#2355=CARTESIAN_POINT ( 'NONE',  ( 147.1970330202780701, 275.6942554159216456, -7.017118315561711839 ) ) ;
#2357=CARTESIAN_POINT ( 'NONE',  ( 192.9523350703175311, 296.4437475495926719, -13.35611922184540923 ) ) ;
#2358=B_SPLINE_CURVE_WITH_KNOTS ( 'NONE', 3,
 ( #3094, #55728, #86717, #79100 ),
 .UNSPECIFIED., .F., .F.,
 ( 4, 4 ),
 ( 0.04814469201508995294, 0.04887120950165273203 ),
 .UNSPECIFIED. ) ;
#2359=CARTESIAN_POINT ( 'NONE',  ( 152.9251141908703175, 265.7729277985770864, -16.20110192949203309 ) ) ;
#2363=CARTESIAN_POINT ( 'NONE',  ( 157.7753659096992180, 281.3564795509028613, 2.871017466566028187 ) ) ;
#2364=CARTESIAN_POINT ( 'NONE',  ( 120.1739550416679378, 246.3149278399160949, 9.188101187500093303 ) ) ;
#2365=ORIENTED_EDGE ( 'NONE', *, *, #11432, .F. ) ;
#2367=DIRECTION ( 'NONE',  ( 0.5000000000000048850, -0.8660254037844358210, 0.000000000000000000 ) ) ;
#2369=ORIENTED_EDGE ( 'NONE', *, *, #47652, .F. ) ;
#2372=CARTESIAN_POINT ( 'NONE',  ( 203.5267646298421482, 276.4525192296148930, 13.67989786268708308 ) ) ;
#2373=CARTESIAN_POINT ( 'NONE',  ( 177.9747879117682317, 253.3556439134052027, 1.401624406440116877 ) ) ;
#2374=CARTESIAN_POINT ( 'NONE',  ( 171.2053697672408816, 287.8281772831969647, -4.637733492338565355 ) ) ;
#2375=CARTESIAN_POINT ( 'NONE',  ( 192.6815422931747435, 296.9127743979267962, 12.45400196617769595 ) ) ;
#2378=CARTESIAN_POINT ( 'NONE',  ( 173.5110880923138836, 287.6292713490308302, -9.896673617075110840 ) ) ;
#2379=CARTESIAN_POINT ( 'NONE',  ( 174.4023533683497362, 281.7821760571821983, 14.15141610718057485 ) ) ;
#2382=CARTESIAN_POINT ( 'NONE',  ( 194.3442947553755005, 294.0328026529847421, -15.97648891113594871 ) ) ;
#2383=CARTESIAN_POINT ( 'NONE',  ( 5.488910272030937065, 180.6427522451419350, -10.00000000000009592 ) ) ;
#2385=CARTESIAN_POINT ( 'NONE',  ( 164.0628648187332885, 278.0734779406835173, 13.23368607355390481 ) ) ;
#2386=CARTESIAN_POINT ( 'NONE',  ( 205.1070740870186455, 269.0972391188071242, -3.016557977693823389 ) ) ;
#2387=CARTESIAN_POINT ( 'NONE',  ( 151.9037511824772082, 267.5419804220855440, -15.52605960223452186 ) ) ;
#2388=CARTESIAN_POINT ( 'NONE',  ( 190.3572031550745294, 300.9386478791372497, 3.093832330100951378 ) ) ;
#2389=CARTESIAN_POINT ( 'NONE',  ( 163.2835940097493790, 247.8315144631017404, 11.08416305054517359 ) ) ;
#2390=CARTESIAN_POINT ( 'NONE',  ( 153.1733743200604181, 270.1408812147403751, 14.03834090807932888 ) ) ;
#2391=CARTESIAN_POINT ( 'NONE',  ( 152.8134590189604580, 275.7618923605953114, -8.624218497726184651 ) ) ;
#2392=CARTESIAN_POINT ( 'NONE',  ( 200.6583719735737645, 283.0965001081523269, -17.35266956530146132 ) ) ;
#2394=CARTESIAN_POINT ( 'NONE',  ( 166.7135982584813405, 281.2722395198167646, -10.95386632010279193 ) ) ;
#2395=CARTESIAN_POINT ( 'NONE',  ( 1.326623512302396168, 183.1199935810941213, 2.679491924311264039 ) ) ;
#2396=CARTESIAN_POINT ( 'NONE',  ( 42.54989241151534429, 183.8262482093457493, 3.021315404115420679E-15 ) ) ;
#2397=EDGE_CURVE ( 'NONE', #36600, #21409, #76285, .T. ) ;
#2400=ADVANCED_FACE ( 'NONE', ( #8867 ), #55484, .T. ) ;
#2404=CARTESIAN_POINT ( 'NONE',  ( -9.134289513013563067, 165.5333772461660828, 9.188101187500095079 ) ) ;
#2405=EDGE_CURVE ( 'NONE', #34725, #23455, #44181, .T. ) ;
#2406=CARTESIAN_POINT ( 'NONE',  ( 85.91165145656356117, 232.6589784336661637, -6.496448406907675876E-16 ) ) ;
#2408=CARTESIAN_POINT ( 'NONE',  ( 147.8927139526707606, 275.3200074130446637, 4.767002118840804492 ) ) ;
#2410=FACE_OUTER_BOUND ( 'NONE', #81383, .T. ) ;
#2412=CARTESIAN_POINT ( 'NONE',  ( 164.1968994398425536, 284.1293336553245581, 5.791912491216440806 ) ) ;
#2415=CARTESIAN_POINT ( 'NONE',  ( 177.8607531624229523, 289.9922794532071180, 9.730199643517920549 ) ) ;
#2417=CARTESIAN_POINT ( 'NONE',  ( 164.6890007341313265, 245.3972786111733626, -5.485860350477558711 ) ) ;
#2421=CARTESIAN_POINT ( 'NONE',  ( 207.2683629543511756, 271.6476598918739001, -6.694388351944108528 ) ) ;
#2423=CARTESIAN_POINT ( 'NONE',  ( 51.37958267218910891, 188.2202760586659451, -5.415160957724236172E-17 ) ) ;
#2424=EDGE_CURVE ( 'NONE', #77804, #11947, #65853, .T. ) ;
#2425=CARTESIAN_POINT ( 'NONE',  ( 175.5502453897478574, 265.0413399349590691, -16.57660258381358531 ) ) ;
#2426=CARTESIAN_POINT ( 'NONE',  ( 65.85835811776894388, 199.6423013555410080, -4.594050593750043987 ) ) ;
#2427=CARTESIAN_POINT ( 'NONE',  ( 207.1158949475991164, 271.9117422260973740, -5.823035679195911918 ) ) ;
#2431=CARTESIAN_POINT ( 'NONE',  ( 167.6502826215564994, 287.3877002845107995, 4.891367078714356609 ) ) ;
#2432=CARTESIAN_POINT ( 'NONE',  ( 200.2066897919534938, 283.8788365955923609, 16.98287317603211477 ) ) ;
#2433=CARTESIAN_POINT ( 'NONE',  ( 176.6519481562020246, 270.0898229012302068, -17.23250062992003606 ) ) ;
#2437=VERTEX_POINT ( 'NONE', #70557 ) ;
#2439=CARTESIAN_POINT ( 'NONE',  ( 73.67938972387338481, 213.3458772461660544, 9.188101187500095079 ) ) ;
#2441=CARTESIAN_POINT ( 'NONE',  ( 172.5631314460892156, 290.7196233979062754, -0.4289259863806654249 ) ) ;
#2443=CARTESIAN_POINT ( 'NONE',  ( 153.7538396745889031, 264.3375331552495027, 18.11269671319490371 ) ) ;
#2446=CARTESIAN_POINT ( 'NONE',  ( 189.7817514553160834, 286.5108602900515393, 16.56304429735581962 ) ) ;
#2447=CARTESIAN_POINT ( 'NONE',  ( 124.8019518427975356, 232.8615022471901739, 5.000000000000051514 ) ) ;
#2449=ORIENTED_EDGE ( 'NONE', *, *, #87057, .T. ) ;
#2451=ORIENTED_EDGE ( 'NONE', *, *, #14087, .F. ) ;
#2452=CARTESIAN_POINT ( 'NONE',  ( 202.9216520459657147, 279.1763840310111391, 15.75371595331685803 ) ) ;
#2454=CARTESIAN_POINT ( 'NONE',  ( 153.4361244163197000, 264.8878321249116539, -17.23169627811277493 ) ) ;
#2456=CARTESIAN_POINT ( 'NONE',  ( 173.3140550308864078, 251.6862458793178234, -0.2129259167810379494 ) ) ;
#2459=CARTESIAN_POINT ( 'NONE',  ( 170.6745590487207096, 250.4173498944666107, 3.281460215579040884 ) ) ;
#2460=CARTESIAN_POINT ( 'NONE',  ( 148.4682235075532901, 274.1715865626006803, 7.806811515100825716 ) ) ;
#2468=CARTESIAN_POINT ( 'NONE',  ( 168.1001124519679877, 276.8241359285356111, 15.41633075000079423 ) ) ;
#2470=EDGE_LOOP ( 'NONE', ( #75576, #27975, #83260, #5207 ) ) ;
#2472=CARTESIAN_POINT ( 'NONE',  ( 183.1096229524326020, 295.7703253833122403, 0.8402911052648339707 ) ) ;
#2476=CARTESIAN_POINT ( 'NONE',  ( 194.4459411895494725, 293.8567458645873103, 14.31012567920753042 ) ) ;
#2477=CARTESIAN_POINT ( 'NONE',  ( 185.3991843159095367, 292.5114241635241115, -11.58673315860843189 ) ) ;
#2478=CARTESIAN_POINT ( 'NONE',  ( 122.1835217032046330, 252.8967562850346553, -4.648177544792955347E-16 ) ) ;
#2479=CARTESIAN_POINT ( 'NONE',  ( 206.7587669622944304, 270.1143081540075173, 3.338494309489741241 ) ) ;
#2481=CARTESIAN_POINT ( 'NONE',  ( 86.31820828217628616, 211.4548013555409796, -4.594050593750042211 ) ) ;
#2482=ORIENTED_EDGE ( 'NONE', *, *, #56346, .F. ) ;
#2483=CARTESIAN_POINT ( 'NONE',  ( 149.9428439900298144, 271.4018792907216380, 11.96959320080079259 ) ) ;
#2486=CARTESIAN_POINT ( 'NONE',  ( 164.9747645813434644, 264.6250227286296877, -16.82035684215298232 ) ) ;
#2489=DIRECTION ( 'NONE',  ( 0.8660254037844395958, 0.4999999999999985567, 0.000000000000000000 ) ) ;
#2490=CARTESIAN_POINT ( 'NONE',  ( 147.0721334091522294, 275.9105878882373304, 0.7242168585908188572 ) ) ;
#2493=CARTESIAN_POINT ( 'NONE',  ( 207.5573902749007971, 271.1470498879065190, 2.528158314636208548 ) ) ;
#2494=CARTESIAN_POINT ( 'NONE',  ( 86.23641098298274699, 232.8464784336661353, 1.353441290958777327E-15 ) ) ;
#2496=CIRCLE ( 'NONE', #12172, 17.82106496071138224 ) ;
#2500=CARTESIAN_POINT ( 'NONE',  ( 208.3226489551340990, 269.8215829728092103, -1.240262689467544366 ) ) ;
#2509=CARTESIAN_POINT ( 'NONE',  ( 157.0808507922293131, 258.5749808621497436, 16.84357500595720580 ) ) ;
#2510=CARTESIAN_POINT ( 'NONE',  ( 157.5154073855773902, 274.2076768598925582, 13.14496121706235598 ) ) ;
#2511=CARTESIAN_POINT ( 'NONE',  ( 159.8732321751776624, 253.7384344327741132, -15.51998349828054202 ) ) ;
#2512=CARTESIAN_POINT ( 'NONE',  ( 191.4622417012445226, 271.4753688487222689, 14.17392657159957103 ) ) ;
#2513=CARTESIAN_POINT ( 'NONE',  ( 177.7195682713364988, 285.0153326636437896, 13.03457619952185098 ) ) ;
#2515=CARTESIAN_POINT ( 'NONE',  ( 198.8010046576729337, 284.7357643445890290, -17.59468233100604806 ) ) ;
#2518=EDGE_CURVE ( 'NONE', #22379, #61940, #42592, .T. ) ;
#2519=CARTESIAN_POINT ( 'NONE',  ( 0.02212491418958350761, 177.4865022471903160, 10.00000000000009415 ) ) ;
#2520=FACE_OUTER_BOUND ( 'NONE', #32195, .T. ) ;
#2522=CARTESIAN_POINT ( 'NONE',  ( 187.6695521735992997, 265.9902340032063535, -11.83501235947671404 ) ) ;
#2524=CARTESIAN_POINT ( 'NONE',  ( 178.7342092137616305, 291.7075392037597226, -6.124219736295335004 ) ) ;
#2529=CARTESIAN_POINT ( 'NONE',  ( 206.9878665138179770, 272.1334939782196329, 6.566295309274049252 ) ) ;
#2530=CARTESIAN_POINT ( 'NONE',  ( 177.3863179211383567, 264.6869915026061335, -15.25279286059338624 ) ) ;
#2531=CARTESIAN_POINT ( 'NONE',  ( 183.7457943646905676, 265.5583575750509908, 13.24080542652859904 ) ) ;
#2532=CARTESIAN_POINT ( 'NONE',  ( 199.1563789199090877, 281.8025795620720260, -16.58559166199236756 ) ) ;
#2535=CARTESIAN_POINT ( 'NONE',  ( 168.5628821761766289, 273.2637907955208902, 15.98574214255321380 ) ) ;
#2536=CARTESIAN_POINT ( 'NONE',  ( 180.9278271019973374, 273.2195462377731019, 17.49290913295951100 ) ) ;
#2539=CARTESIAN_POINT ( 'NONE',  ( 178.3571982967953602, 292.6181790745828835, -7.174879954037646002 ) ) ;
#2540=CARTESIAN_POINT ( 'NONE',  ( 190.8429499865819707, 278.0757709512191695, -17.64141544901220371 ) ) ;
#2541=CARTESIAN_POINT ( 'NONE',  ( 2.042590532755589994, 181.1744531367911577, 4.594050593750047540 ) ) ;
#2544=CARTESIAN_POINT ( 'NONE',  ( 177.7380108946867665, 256.6765468135970423, 8.337886873569251733 ) ) ;
#2547=CARTESIAN_POINT ( 'NONE',  ( 26.64321143294854721, 192.3149278399161233, 9.188101187500093303 ) ) ;
#2548=CARTESIAN_POINT ( 'NONE',  ( 181.6779114849496466, 276.3290641470016453, -17.56019397242378588 ) ) ;
#2550=CARTESIAN_POINT ( 'NONE',  ( 179.5516160758070612, 292.2552566163012671, 6.096423350851510214 ) ) ;
#2553=CARTESIAN_POINT ( 'NONE',  ( 196.3214660117057235, 290.6082415817560332, 16.86635188982479860 ) ) ;
#2556=CARTESIAN_POINT ( 'NONE',  ( 186.8161249571872133, 295.8581466444864532, -7.749471023126312197 ) ) ;
#2558=CARTESIAN_POINT ( 'NONE',  ( 91.96515528263753936, 217.2365022471902307, 10.00000000000009592 ) ) ;
#2562=CARTESIAN_POINT ( 'NONE',  ( 42.85403768609726427, 204.7369531367911293, -4.594050593750048428 ) ) ;
#2566=CARTESIAN_POINT ( 'NONE',  ( 190.9380839614473473, 299.9325328093580652, -5.232187664503159752 ) ) ;
#2567=DIRECTION ( 'NONE',  ( 0.5000000000000048850, -0.8660254037844358210, 0.000000000000000000 ) ) ;
#2568=ORIENTED_EDGE ( 'NONE', *, *, #28791, .F. ) ;
#2569=CARTESIAN_POINT ( 'NONE',  ( 167.6379738498630729, 285.0209819684473018, 7.709156655479272757 ) ) ;
#2574=CARTESIAN_POINT ( 'NONE',  ( 162.9466247808429102, 248.4151622881552441, 11.25765811906727443 ) ) ;
#2575=CARTESIAN_POINT ( 'NONE',  ( 196.6288634187112052, 290.0758136547079289, -16.31544900032282186 ) ) ;
#2576=EDGE_CURVE ( 'NONE', #60705, #8540, #71704, .T. ) ;
#2577=CARTESIAN_POINT ( 'NONE',  ( 175.2796639585627361, 257.3526018093201060, 11.64661369289347448 ) ) ;
#2580=CARTESIAN_POINT ( 'NONE',  ( 199.1041333440138317, 265.1832257255362038, 0.2027868546939186056 ) ) ;
#2581=CARTESIAN_POINT ( 'NONE',  ( 24.47938433582656259, 173.3932355074535963, -2.679491924311248496 ) ) ;
#2586=CARTESIAN_POINT ( 'NONE',  ( 177.4968317130364994, 256.2040971538554004, -7.264605064380178057 ) ) ;
#2590=EDGE_LOOP ( 'NONE', ( #64056, #58020, #66053 ) ) ;
#2591=CARTESIAN_POINT ( 'NONE',  ( 188.2427339305948522, 273.3740536669656649, -15.69085291912274549 ) ) ;
#2592=ORIENTED_EDGE ( 'NONE', *, *, #72741, .T. ) ;
#2593=CARTESIAN_POINT ( 'NONE',  ( 200.6583719735737645, 283.0965001081523269, -17.35266956530146132 ) ) ;
#2597=EDGE_CURVE ( 'NONE', #31958, #82127, #99240, .T. ) ;
#2598=CARTESIAN_POINT ( 'NONE',  ( 157.8159121039657293, 257.3018173235443555, -17.05074702406642118 ) ) ;
#2599=CARTESIAN_POINT ( 'NONE',  ( 110.1064097226738312, 240.5024278399161233, 9.188101187500095079 ) ) ;
#2600=CARTESIAN_POINT ( 'NONE',  ( 181.9173911336421270, 287.5464557181833243, -13.25301832635643429 ) ) ;
#2603=CARTESIAN_POINT ( 'NONE',  ( 161.2652686759580831, 266.8029729739616869, 16.52606187695826989 ) ) ;
#2606=CARTESIAN_POINT ( 'NONE',  ( 197.8809552785519656, 287.9071269377202498, 17.61728046362068412 ) ) ;
#2608=CARTESIAN_POINT ( 'NONE',  ( 69.56611615166229967, 198.7202760586659736, -5.415160957724236172E-17 ) ) ;
#2610=CARTESIAN_POINT ( 'NONE',  ( 151.4327733764141612, 268.3577379114237829, 14.90862905801242100 ) ) ;
#2611=CARTESIAN_POINT ( 'NONE',  ( 198.4383541551818553, 286.9416837633153250, 16.97133247567711578 ) ) ;
#2615=DIRECTION ( 'NONE',  ( -0.4999999999999987788, 0.8660254037844392627, 0.000000000000000000 ) ) ;
#2617=CARTESIAN_POINT ( 'NONE',  ( 177.7333452155622524, 288.3950663957488700, 10.76829023525657725 ) ) ;
#2620=CARTESIAN_POINT ( 'NONE',  ( 175.4672344667806385, 261.1926118659519602, -14.53162499237264704 ) ) ;
#2622=CARTESIAN_POINT ( 'NONE',  ( 207.8575108622103755, 270.6272257822888037, -6.381720258959569847 ) ) ;
#2624=CARTESIAN_POINT ( 'NONE',  ( 149.0802055316563326, 272.4325049467973940, 12.84384348890831085 ) ) ;
#2625=CARTESIAN_POINT ( 'NONE',  ( 186.7554075434758545, 282.3000898601083577, 17.53539547572453827 ) ) ;
#2626=DIRECTION ( 'NONE',  ( 0.8660254037844395958, 0.4999999999999985567, 0.000000000000000000 ) ) ;
#2627=CARTESIAN_POINT ( 'NONE',  ( 168.0509104211369333, 255.6975718937168267, 13.75861284036475851 ) ) ;
#2629=CARTESIAN_POINT ( 'NONE',  ( 113.7598676209481994, 245.6744531367911293, 4.594050593750047540 ) ) ;
#2630=ORIENTED_EDGE ( 'NONE', *, *, #20845, .T. ) ;
#2634=ADVANCED_FACE ( 'NONE', ( #20367 ), #27947, .T. ) ;
#2637=CARTESIAN_POINT ( 'NONE',  ( 183.2034608524758994, 284.9060971692327939, -14.93137950553607673 ) ) ;
#2639=ORIENTED_EDGE ( 'NONE', *, *, #24673, .F. ) ;
#2641=CARTESIAN_POINT ( 'NONE',  ( 157.6038783220860466, 274.4889219920046344, -12.58265736104147159 ) ) ;
#2642=CARTESIAN_POINT ( 'NONE',  ( -0.04208563418565033909, 182.3297689869269504, -2.679491924311240503 ) ) ;
#2643=CARTESIAN_POINT ( 'NONE',  ( 185.0449151060633142, 261.9026404081322994, 9.668537895844421470 ) ) ;
#2644=CARTESIAN_POINT ( 'NONE',  ( 206.6093111437328957, 272.7891711126852101, -9.934261249647553527 ) ) ;
#2645=CARTESIAN_POINT ( 'NONE',  ( 145.1264855360895751, 254.5958772461660544, -9.188101187500095079 ) ) ;
#2649=CARTESIAN_POINT ( 'NONE',  ( 56.95410056540389832, 209.8149278399160949, -9.188101187500095079 ) ) ;
#2651=CARTESIAN_POINT ( 'NONE',  ( 176.6604108716779820, 252.5228158049957017, 3.079518071111189137 ) ) ;
#2653=CARTESIAN_POINT ( 'NONE',  ( 172.0910100529608258, 260.0785035667472584, 15.53398388876759206 ) ) ;
#2656=CARTESIAN_POINT ( 'NONE',  ( 203.2187760522547819, 278.6617501559703101, -15.08675642319914978 ) ) ;
#2657=CARTESIAN_POINT ( 'NONE',  ( 193.0813327359068126, 289.3713108709676476, 16.53843723896193652 ) ) ;
#2658=CARTESIAN_POINT ( 'NONE',  ( 125.0004159942835571, 229.6427522451417360, 1.119607411625061291E-15 ) ) ;
#2660=ORIENTED_EDGE ( 'NONE', *, *, #81375, .T. ) ;
#2662=CARTESIAN_POINT ( 'NONE',  ( -16.46870247313679059, 170.4869531367911293, 4.594050593750046652 ) ) ;
#2663=B_SPLINE_CURVE_WITH_KNOTS ( 'NONE', 3,
 ( #70677, #40263, #24575, #77805, #47862, #15979, #38772, #61571, #94023, #77285, #54453, #23067, #32175, #100107, #24079, #16971 ),
 .UNSPECIFIED., .F., .F.,
 ( 4, 2, 2, 2, 2, 2, 2, 4 ),
 ( 0.000000000000000000, 0.0003786681000628006294, 0.0007573362001256012587, 0.001136004300188401834, 0.001514672400251202517, 0.001893340500314003418, 0.002272008600376803668, 0.003029344800502417178 ),
 .UNSPECIFIED. ) ;
#2665=CARTESIAN_POINT ( 'NONE',  ( 44.28847903505648986, 202.5024278399160949, -9.188101187500093303 ) ) ;
#2667=CARTESIAN_POINT ( 'NONE',  ( 42.80017141841058503, 185.5177522451417929, 5.000000000000051514 ) ) ;
#2669=LINE ( 'NONE', #94886, #41900 ) ;
#2670=CIRCLE ( 'NONE', #59247, 10.00000000000011369 ) ;
#2671=CARTESIAN_POINT ( 'NONE',  ( 190.3791419447713906, 300.9006487807255326, -5.688668718458480988 ) ) ;
#2674=CARTESIAN_POINT ( 'NONE',  ( 70.44081555586392085, 198.1427522451417644, 1.119607411625061291E-15 ) ) ;
#2675=CARTESIAN_POINT ( 'NONE',  ( 119.5854454918513170, 251.3967562850347122, -4.648177544792955347E-16 ) ) ;
#2676=CARTESIAN_POINT ( 'NONE',  ( 183.9856954830609936, 257.7508274558034032, 1.338685087526031658 ) ) ;
#2677=CARTESIAN_POINT ( 'NONE',  ( 4.496589500409242213, 166.7365022471902023, -10.00000000000009237 ) ) ;
#2680=CARTESIAN_POINT ( 'NONE',  ( 161.4046941692269002, 267.9362656474927462, 17.36169958451479189 ) ) ;
#2681=CARTESIAN_POINT ( 'NONE',  ( 35.67350403664894998, 204.7365022471903160, 2.944929066748280225E-16 ) ) ;
#2682=CARTESIAN_POINT ( 'NONE',  ( 184.9788321220551381, 294.4173266759285070, 9.914855298944029727 ) ) ;
#2683=CARTESIAN_POINT ( 'NONE',  ( 163.0171530587457767, 248.2930037274571191, 9.677214176418313940 ) ) ;
#2684=CARTESIAN_POINT ( 'NONE',  ( 0.6624493194153854292, 177.3149278399160664, 9.188101187500093303 ) ) ;
#2686=CARTESIAN_POINT ( 'NONE',  ( 161.5266078408477597, 251.3399204103630211, 13.01505764280997468 ) ) ;
#2688=CARTESIAN_POINT ( 'NONE',  ( 192.7507137768506880, 296.7929658737652971, 11.30364540927242345 ) ) ;
#2690=CARTESIAN_POINT ( 'NONE',  ( 75.87151652897667020, 224.6115022471903160, -5.000000000000047962 ) ) ;
#2692=CARTESIAN_POINT ( 'NONE',  ( 154.8838596469624349, 262.3802811495310152, 18.07457254681616021 ) ) ;
#2694=FACE_OUTER_BOUND ( 'NONE', #12221, .T. ) ;
#2696=CARTESIAN_POINT ( 'NONE',  ( 153.3042509968460934, 277.6952823349280948, -5.244408299408142682 ) ) ;
#2698=CARTESIAN_POINT ( 'NONE',  ( 207.2051200232459962, 271.7571998617677309, 9.213853433517439129 ) ) ;
#2701=CARTESIAN_POINT ( 'NONE',  ( 193.9204722154232741, 294.7668848255750049, 15.43855698596013859 ) ) ;
#2704=CARTESIAN_POINT ( 'NONE',  ( 159.8732321751776624, 253.7384344327741132, -15.51998349828054202 ) ) ;
#2707=CARTESIAN_POINT ( 'NONE',  ( 152.3854270389657586, 267.1361007204005205, 15.42493684955348066 ) ) ;
#2708=CARTESIAN_POINT ( 'NONE',  ( 164.6460902696047128, 245.4716017159096566, -3.036414139157908476 ) ) ;
#2709=AXIS2_PLACEMENT_3D ( 'NONE', #26703, #42381, #19128 ) ;
#2712=CARTESIAN_POINT ( 'NONE',  ( 155.5888570658010508, 261.1591898008976500, 17.34682632352454945 ) ) ;
#2713=VERTEX_POINT ( 'NONE', #64972 ) ;
#2715=CARTESIAN_POINT ( 'NONE',  ( 159.5339686208487535, 278.3616057620046149, -9.790299535603285364 ) ) ;
#2720=ORIENTED_EDGE ( 'NONE', *, *, #89108, .F. ) ;
#2721=ADVANCED_FACE ( 'NONE', ( #88327 ), #26969, .F. ) ;
#2724=CARTESIAN_POINT ( 'NONE',  ( 198.2505066714982149, 285.2670451491296149, 0.000000000000000000 ) ) ;
#2727=CARTESIAN_POINT ( 'NONE',  ( 161.7587802986029999, 250.4725692828850754, 14.33336164792646450 ) ) ;
#2728=CARTESIAN_POINT ( 'NONE',  ( 169.5281517825888500, 276.4612764335079191, -15.85450656213009601 ) ) ;
#2729=CARTESIAN_POINT ( 'NONE',  ( 191.1489696025915919, 299.5672681643093256, 8.892130899335590755 ) ) ;
#2730=CARTESIAN_POINT ( 'NONE',  ( 151.0597526782644309, 274.7879323711273400, -8.642014759372267818 ) ) ;
#2732=CARTESIAN_POINT ( 'NONE',  ( 173.2764727202423387, 256.9869438812573321, -11.70977877276238921 ) ) ;
#2738=EDGE_LOOP ( 'NONE', ( #28327, #90071, #29281, #27735 ) ) ;
#2740=ORIENTED_EDGE ( 'NONE', *, *, #13889, .F. ) ;
#2742=CARTESIAN_POINT ( 'NONE',  ( 147.9036042187065618, 274.4704382010785935, 6.970551717703401984 ) ) ;
#2745=CARTESIAN_POINT ( 'NONE',  ( 152.6845319923753834, 266.1896283897672220, 17.20844521882669653 ) ) ;
#2747=CARTESIAN_POINT ( 'NONE',  ( 158.6106834916122068, 255.9252328997384609, -16.08117073480969239 ) ) ;
#2749=CARTESIAN_POINT ( 'NONE',  ( 174.3506819931331506, 286.9267872025895940, 11.76311152586403885 ) ) ;
#2752=CARTESIAN_POINT ( 'NONE',  ( 164.6869624841032191, 245.4008089637804346, 1.435659848726088317 ) ) ;
#2753=FACE_OUTER_BOUND ( 'NONE', #46864, .T. ) ;
#2754=CARTESIAN_POINT ( 'NONE',  ( 206.2520115784021471, 273.4080321133600933, 11.69992874350409018 ) ) ;
#2755=CARTESIAN_POINT ( 'NONE',  ( 198.2114954873088948, 287.3346145022089786, 18.52864136173620935 ) ) ;
#2759=CARTESIAN_POINT ( 'NONE',  ( 187.5021553793853002, 277.0230319745485872, 17.44130860609008948 ) ) ;
#2761=CARTESIAN_POINT ( 'NONE',  ( 171.5618304431668548, 259.5850279847709885, -13.97585501171604427 ) ) ;
#2762=CARTESIAN_POINT ( 'NONE',  ( 164.4568492923521887, 247.7993767033852919, 8.703614106482779889 ) ) ;
#2765=CARTESIAN_POINT ( 'NONE',  ( 161.5875797534026219, 250.7690973254556468, 12.95526170413129030 ) ) ;
#2766=CARTESIAN_POINT ( 'NONE',  ( 191.2423980897042100, 261.1760977627640159, -0.01336292133867102681 ) ) ;
#2767=ORIENTED_EDGE ( 'NONE', *, *, #22716, .F. ) ;
#2768=CARTESIAN_POINT ( 'NONE',  ( 153.4232513496498598, 270.1086993216917449, 15.21047082690287588 ) ) ;
#2769=ADVANCED_FACE ( 'NONE', ( #45136 ), #22342, .T. ) ;
#2770=CARTESIAN_POINT ( 'NONE',  ( 178.9714194486930694, 253.6239517424200187, 1.422777586239305059 ) ) ;
#2771=CARTESIAN_POINT ( 'NONE',  ( 207.6477529416552557, 270.9905371579805546, 7.447146952410988341 ) ) ;
#2772=CARTESIAN_POINT ( 'NONE',  ( 17.68543470866176648, 191.0177522451419065, 5.000000000000046185 ) ) ;
#2773=CARTESIAN_POINT ( 'NONE',  ( 92.65049840370248546, 233.4869531367911293, 4.594050593750046652 ) ) ;
#2775=ADVANCED_FACE ( 'NONE', ( #98370 ), #38529, .T. ) ;
#2777=CARTESIAN_POINT ( 'NONE',  ( 162.8493988834005677, 248.5835624823365322, 11.81438570587263470 ) ) ;
#2778=CARTESIAN_POINT ( 'NONE',  ( 25.45277359850996390, 179.3768266524160140, -9.188101187500091527 ) ) ;
#2782=VERTEX_POINT ( 'NONE', #14741 ) ;
#2783=CIRCLE ( 'NONE', #38311, 17.82106496071138224 ) ;
#2785=VERTEX_POINT ( 'NONE', #99854 ) ;
#2787=CARTESIAN_POINT ( 'NONE',  ( 188.1316680866631543, 261.3724935531064375, -5.915372741867520823 ) ) ;
#2793=CARTESIAN_POINT ( 'NONE',  ( 42.66591781529977823, 183.8932355074535963, -2.679491924311248496 ) ) ;
#2795=CARTESIAN_POINT ( 'NONE',  ( 98.22579726061456995, 237.5177522451419350, 5.000000000000046185 ) ) ;
#2796=CARTESIAN_POINT ( 'NONE',  ( 35.38456857845647363, 200.4244531367911293, -4.594050593750046652 ) ) ;
#2797=CARTESIAN_POINT ( 'NONE',  ( 80.83312040127708542, 224.1427522451419065, -10.00000000000009415 ) ) ;
#2798=ORIENTED_EDGE ( 'NONE', *, *, #60201, .T. ) ;
#2800=CARTESIAN_POINT ( 'NONE',  ( 1.032487885271483163, 164.7365022471902307, 10.00000000000009948 ) ) ;
#2801=CARTESIAN_POINT ( 'NONE',  ( -11.38080322590321281, 173.4244531367911293, -4.594050593750046652 ) ) ;
#2803=CARTESIAN_POINT ( 'NONE',  ( 199.1944722252943905, 285.6320488493591938, -18.17555833707144686 ) ) ;
#2805=CARTESIAN_POINT ( 'NONE',  ( 147.5118896528469179, 275.1489077312122049, -3.975523961781759930 ) ) ;
#2807=CARTESIAN_POINT ( 'NONE',  ( 163.9704062730716032, 246.6419207277664327, 7.317582738093436845 ) ) ;
#2808=CARTESIAN_POINT ( 'NONE',  ( 191.0933613939813540, 299.6635844069401173, -8.689828987424775164 ) ) ;
#2809=CARTESIAN_POINT ( 'NONE',  ( 207.1601050488701503, 271.8351680844880889, 6.320235450527015075 ) ) ;
#2810=VERTEX_POINT ( 'NONE', #30937 ) ;
#2811=CARTESIAN_POINT ( 'NONE',  ( 5.723458822437210713, 164.1115022471902023, -5.000000000000041744 ) ) ;
#2812=CARTESIAN_POINT ( 'NONE',  ( 16.11576366785047654, 170.1115022471901739, -5.000000000000041744 ) ) ;
#2813=CARTESIAN_POINT ( 'NONE',  ( 121.1210835531159091, 249.9244531367911293, -4.594050593750046652 ) ) ;
#2816=CARTESIAN_POINT ( 'NONE',  ( 151.2076104553919151, 269.2233279204718883, 14.08327307015630225 ) ) ;
#2817=CARTESIAN_POINT ( 'NONE',  ( 195.8248271798537417, 291.4684452715354155, 17.35175160929494709 ) ) ;
#2818=CARTESIAN_POINT ( 'NONE',  ( 185.9608592076092464, 288.5956984647530703, 15.36535719480430018 ) ) ;
#2819=CARTESIAN_POINT ( 'NONE',  ( 190.7790613819595080, 300.2079679965814876, -6.533365802463900529 ) ) ;
#2821=CARTESIAN_POINT ( 'NONE',  ( 193.4292346840946379, 262.9787757345689556, -5.315308200742018485 ) ) ;
#2822=CARTESIAN_POINT ( 'NONE',  ( 149.6230451358742926, 271.4922791719315001, -12.72565967355361671 ) ) ;
#2823=AXIS2_PLACEMENT_3D ( 'NONE', #62040, #46345, #46865 ) ;
#2824=CARTESIAN_POINT ( 'NONE',  ( 96.20275958967147290, 237.8967562850346837, -4.648177544792955347E-16 ) ) ;
#2825=CARTESIAN_POINT ( 'NONE',  ( 172.9948194558320438, 289.9929851553021081, -1.758069817448381977 ) ) ;
#2828=CARTESIAN_POINT ( 'NONE',  ( 189.1399679817465938, 265.6558378727139029, 10.77106915762913353 ) ) ;
#2829=CARTESIAN_POINT ( 'NONE',  ( 175.2876851193108223, 279.0504642908932738, 15.49633333057976259 ) ) ;
#2831=CARTESIAN_POINT ( 'NONE',  ( 168.7163198393688788, 271.7405862636877600, -16.69663154779234304 ) ) ;
#2833=B_SPLINE_SURFACE_WITH_KNOTS ( 'NONE', 3, 1, ( 
 ( #98216, #43978 ),
 ( #4004, #81059 ),
 ( #74920, #66796 ),
 ( #88668, #51084 ),
 ( #27311, #58197 ),
 ( #5502, #19724 ),
 ( #81539, #11622 ),
 ( #73417, #65304 ),
 ( #90653, #28800 ),
 ( #67289, #21211 ),
 ( #5014, #82554 ),
 ( #58679, #34890 ),
 ( #73913, #97721 ),
 ( #82046, #44481 ),
 ( #89177, #13119 ),
 ( #89651, #50589 ),
 ( #83037, #96246 ),
 ( #26807, #59165 ),
 ( #20212, #13608 ),
 ( #35396, #43486 ),
 ( #12111, #66305 ),
 ( #97238, #75412 ),
 ( #57690, #19235 ),
 ( #27806, #74430 ),
 ( #30293, #92148 ),
 ( #30798, #92627 ),
 ( #100212, #44982 ),
 ( #8005, #6504 ),
 ( #77907, #53089 ),
 ( #61677, #16086 ),
 ( #99705, #84533 ),
 ( #60170, #61181 ),
 ( #15077, #14100 ),
 ( #37381, #22701 ) ),
 .UNSPECIFIED., .T., .F., .F.,
 ( 4, 2, 2, 2, 2, 2, 2, 2, 2, 2, 2, 2, 2, 2, 2, 2, 4 ),
 ( 2, 2 ),
 ( 0.000000000000000000, 0.06250000000000000000, 0.1250000000000000000, 0.1875000000000000000, 0.2500000000000000000, 0.3125000000000000000, 0.3750000000000000000, 0.4375000000000000000, 0.5000000000000000000, 0.5625000000000000000, 0.6250000000000000000, 0.6875000000000000000, 0.7500000000000000000, 0.8125000000000000000, 0.8750000000000000000, 0.9375000000000000000, 1.000000000000000000 ),
 ( 0.000000000000000000, 1.000000000000000000 ),
 .UNSPECIFIED. ) ;
#2834=CARTESIAN_POINT ( 'NONE',  ( 200.2436573053165034, 272.2885561403415977, 12.78478541099706156 ) ) ;
#2837=CARTESIAN_POINT ( 'NONE',  ( 153.1973045377566507, 265.3014802884401320, 17.70608187426261892 ) ) ;
#2839=CARTESIAN_POINT ( 'NONE',  ( 197.9901163037401943, 272.1418500761980681, -13.83221381771805625 ) ) ;
#2841=CARTESIAN_POINT ( 'NONE',  ( 191.8915949969537564, 288.0041433326085780, -15.85806419801627598 ) ) ;
#2844=CARTESIAN_POINT ( 'NONE',  ( 194.2223991963907963, 294.2439319543634610, -14.97294938100067441 ) ) ;
#2845=CARTESIAN_POINT ( 'NONE',  ( 164.4429246715887416, 246.1956853373532681, -1.592092674508304384 ) ) ;
#2849=CARTESIAN_POINT ( 'NONE',  ( 188.2744984008364497, 292.9879626925077218, 12.47922449114265042 ) ) ;
#2853=CARTESIAN_POINT ( 'NONE',  ( 189.4220206103759381, 300.3593688522817615, 3.300941728658063568 ) ) ;
#2854=CARTESIAN_POINT ( 'NONE',  ( 25.47966334272171807, 195.5177522451419350, 5.000000000000046185 ) ) ;
#2855=ORIENTED_EDGE ( 'NONE', *, *, #29398, .F. ) ;
#2858=CARTESIAN_POINT ( 'NONE',  ( 178.0571612022058048, 260.8998630075552683, 12.21430617061977486 ) ) ;
#2860=ORIENTED_EDGE ( 'NONE', *, *, #96342, .T. ) ;
#2861=CARTESIAN_POINT ( 'NONE',  ( 192.8902927049463472, 294.0135136195178802, 14.17129879840491391 ) ) ;
#2864=CARTESIAN_POINT ( 'NONE',  ( 203.5629025532486196, 278.0657055720176913, -15.85226727704602823 ) ) ;
#2865=( BOUNDED_CURVE ( )  B_SPLINE_CURVE ( 2, ( #96602, #72278, #11485, #89034, #19583, #42337, #73267, #20068, #10973 ),
 .UNSPECIFIED., .F., .T. ) 
 B_SPLINE_CURVE_WITH_KNOTS ( ( 3, 2, 2, 2, 3 ),
 ( 0.8508064516129032473, 0.8521505376344086224, 0.8548387096774193727, 0.8575268817204301230, 0.8588709677419354982 ),
 .UNSPECIFIED. ) 
 CURVE ( )  GEOMETRIC_REPRESENTATION_ITEM ( )  RATIONAL_B_SPLINE_CURVE ( ( 0.9330127018922194093, 0.9330127018922194093, 1.000000000000000000, 0.8660254037844387076, 1.000000000000000000, 0.8660254037844387076, 1.000000000000000000, 0.9330127018922194093, 0.9330127018922194093 ) ) 
 REPRESENTATION_ITEM ( '' )  );
#2866=VERTEX_POINT ( 'NONE', #79082 ) ;
#2869=CARTESIAN_POINT ( 'NONE',  ( 190.6501024053443132, 300.4313314961713672, 3.138638463324308514 ) ) ;
#2870=CARTESIAN_POINT ( 'NONE',  ( 162.0312816687286386, 277.4338305391307244, -12.97134983198379210 ) ) ;
#2871=CARTESIAN_POINT ( 'NONE',  ( 192.6789561813392595, 296.9172536750198219, -11.84591848451790952 ) ) ;
#2872=CARTESIAN_POINT ( 'NONE',  ( 153.3506059258413643, 265.0359544954067132, -16.39100908615009899 ) ) ;
#2874=B_SPLINE_CURVE_WITH_KNOTS ( 'NONE', 3,
 ( #32869, #26776, #57657, #73385, #17168, #48068, #26283, #57157, #79009, #94707, #71394, #63775, #74399, #50559, #12080, #51567, #5966, #20679, #97209, #44951, #13088, #89143 ),
 .UNSPECIFIED., .F., .F.,
 ( 4, 2, 2, 2, 2, 2, 2, 2, 2, 2, 4 ),
 ( 0.0002504268395162665534, 0.0009777574624113120373, 0.001705088085306357467, 0.001796004413168241940, 0.001841462577099220715, 0.001886920741030199706, 0.001977837068892119524, 0.002068753396754039343, 0.002432418708201630145, 0.002796084019649220515, 0.003159749331096811317 ),
 .UNSPECIFIED. ) ;
#2875=CARTESIAN_POINT ( 'NONE',  ( 183.4283023828987211, 284.5394489297055429, -16.36380929643289406 ) ) ;
#2876=CARTESIAN_POINT ( 'NONE',  ( 134.7341806906763395, 248.5958772461660544, -9.188101187500095079 ) ) ;
#2880=ORIENTED_EDGE ( 'NONE', *, *, #13843, .F. ) ;
#2881=CARTESIAN_POINT ( 'NONE',  ( 176.1016924857606796, 254.5150318770701290, -8.700168781860330824 ) ) ;
#2883=CARTESIAN_POINT ( 'NONE',  ( 105.1336465626505969, 243.0530062829863027, -4.648177544792955347E-16 ) ) ;
#2884=CARTESIAN_POINT ( 'NONE',  ( 192.0681310285980032, 297.9752338741087101, 12.08674140724503054 ) ) ;
#2885=CARTESIAN_POINT ( 'NONE',  ( 155.2046175752080615, 277.9469667126091394, 7.179509265143448893 ) ) ;
#2887=DIRECTION ( 'NONE',  ( 0.4999999999999998890, -0.8660254037844385966, 0.000000000000000000 ) ) ;
#2888=( BOUNDED_CURVE ( )  B_SPLINE_CURVE ( 2, ( #3403, #2395, #11000, #80426, #57564, #71798, #41873, #33275, #34277 ),
 .UNSPECIFIED., .F., .T. ) 
 B_SPLINE_CURVE_WITH_KNOTS ( ( 3, 2, 2, 2, 3 ),
 ( 0.1169354838709677491, 0.1182795698924731242, 0.1209677419354838745, 0.1236559139784946248, 0.1250000000000000000 ),
 .UNSPECIFIED. ) 
 CURVE ( )  GEOMETRIC_REPRESENTATION_ITEM ( )  RATIONAL_B_SPLINE_CURVE ( ( 0.9330127018922192983, 0.9330127018922196314, 1.000000000000000000, 0.8660254037844387076, 1.000000000000000000, 0.8660254037844387076, 1.000000000000000000, 0.9330127018922194093, 0.9330127018922194093 ) ) 
 REPRESENTATION_ITEM ( '' )  );
#2889=CARTESIAN_POINT ( 'NONE',  ( 171.0049078633470856, 280.9014079933706967, 14.16035466535159415 ) ) ;
#2891=CARTESIAN_POINT ( 'NONE',  ( 177.2243378689070710, 256.1247485821839405, -7.470792856032248075 ) ) ;
#2892=ORIENTED_EDGE ( 'NONE', *, *, #90641, .T. ) ;
#2893=CARTESIAN_POINT ( 'NONE',  ( 147.8163551302855296, 274.6215580551378821, -9.286329195885331345 ) ) ;
#2894=EDGE_CURVE ( 'NONE', #39791, #63243, #19419, .T. ) ;
#2900=CARTESIAN_POINT ( 'NONE',  ( 204.9603142014765353, 269.2154079871559702, -2.986001317163250235 ) ) ;
#2901=CARTESIAN_POINT ( 'NONE',  ( 152.3236346572827813, 266.8147209104637909, -16.89516215687428158 ) ) ;
#2902=CARTESIAN_POINT ( 'NONE',  ( 196.0997760050400416, 263.6366458471133569, -2.478146138921373254 ) ) ;
#2904=CARTESIAN_POINT ( 'NONE',  ( 163.2919429874875448, 247.8170536094679903, 9.876785378511263147 ) ) ;
#2906=CARTESIAN_POINT ( 'NONE',  ( 151.4835516929774712, 274.9458191638564131, -9.335966666621812848 ) ) ;
#2907=CARTESIAN_POINT ( 'NONE',  ( 199.9887875258707197, 267.3737047273518783, 6.263774817124060590 ) ) ;
#2911=CARTESIAN_POINT ( 'NONE',  ( 193.5554883805989164, 276.0937916413638504, -16.57716084711649174 ) ) ;
#2913=CARTESIAN_POINT ( 'NONE',  ( 153.3127735718713609, 265.1014820546527631, 17.57722645152040641 ) ) ;
#2917=CARTESIAN_POINT ( 'NONE',  ( -5.074968980656518802, 174.0024278399161233, -9.188101187500093303 ) ) ;
#2918=CARTESIAN_POINT ( 'NONE',  ( 98.87557663705065636, 218.7048013555409796, 4.594050593750051981 ) ) ;
#2919=CARTESIAN_POINT ( 'NONE',  ( 192.5076277540105423, 297.2140032159341558, -13.10094381206144298 ) ) ;
#2923=CARTESIAN_POINT ( 'NONE',  ( 194.4175321639488629, 282.9566666730594307, 17.82086732188745870 ) ) ;
#2925=CARTESIAN_POINT ( 'NONE',  ( 160.9346792447446717, 281.6669817926451174, 5.574211404230215550 ) ) ;
#2927=CARTESIAN_POINT ( 'NONE',  ( 163.4178923001155681, 247.5989030008181260, -10.38047187240561442 ) ) ;
#2928=CARTESIAN_POINT ( 'NONE',  ( 207.9683050836422069, 270.4353245615839114, 5.627704969255242773 ) ) ;
#2932=CARTESIAN_POINT ( 'NONE',  ( 143.2591182574054187, 253.5177522451418497, -10.00000000000009592 ) ) ;
#2933=CARTESIAN_POINT ( 'NONE',  ( 183.1207986101861138, 294.8225010653632694, -8.165837621905515320 ) ) ;
#2935=CARTESIAN_POINT ( 'NONE',  ( 55.03304057046344866, 193.3923013555409796, 4.594050593750050204 ) ) ;
#2939=CARTESIAN_POINT ( 'NONE',  ( 68.04987750350953490, 222.3464784336661637, 1.353441290958777327E-15 ) ) ;
#2940=CARTESIAN_POINT ( 'NONE',  ( 207.3874697692679945, 271.4413608369101780, -6.809237722377445401 ) ) ;
#2941=B_SPLINE_CURVE_WITH_KNOTS ( 'NONE', 3,
 ( #40943, #58526, #64269, #10580, #35239, #74274, #18177, #5344, #90491, #95222, #97566, #82399, #35740, #56665, #4858, #75253, #42819, #66636, #4343, #10079, #50931, #29145, #28135, #36225, #80011, #59513, #89975, #20555, #81881, #51433, #67130, #21064, #51941, #82880, #13455, #5833, #67626, #60016, #48578, #79517, #2486, #99051, #83370, #37225, #60506, #13934, #52423, #68123, #21540, #44814 ),
 .UNSPECIFIED., .F., .F.,
 ( 4, 2, 2, 2, 2, 2, 2, 2, 2, 2, 2, 2, 2, 2, 2, 2, 2, 2, 2, 2, 2, 2, 2, 2, 4 ),
 ( 0.001883115646984252940, 0.002330946116002702642, 0.002554861350511887595, 0.002778776585021072547, 0.002890734202275699934, 0.003002691819530327322, 0.003114649436784954276, 0.003226607054039581229, 0.003450522288548780493, 0.003674437523057979757, 0.004570098461094487113, 0.005465759399130996204, 0.006361420337167503561, 0.006809250806185799740, 0.007257081275204095051, 0.007369038892458601442, 0.007425017701085824713, 0.007480996509713047984, 0.007592954126967495394, 0.007704911744221941937, 0.008152742213239631830, 0.008376657447748478078, 0.008600572682257322590, 0.008824487916766168838, 0.009048403151275013351 ),
 .UNSPECIFIED. ) ;
#2943=CARTESIAN_POINT ( 'NONE',  ( 163.2522125179119996, 258.2236914498371334, 15.93854035083980669 ) ) ;
#2945=DIRECTION ( 'NONE',  ( -0.8660254037844387076, -0.4999999999999998890, -0.000000000000000000 ) ) ;
#2946=CARTESIAN_POINT ( 'NONE',  ( 196.8489777528309048, 268.3839510415193104, -10.94460251732624023 ) ) ;
#2952=CARTESIAN_POINT ( 'NONE',  ( 80.17458025225667484, 217.0958772461660544, -9.188101187500095079 ) ) ;
#2954=CARTESIAN_POINT ( 'NONE',  ( 169.1905967623088145, 288.2264484338115835, -1.107241701029636038 ) ) ;
#2955=CARTESIAN_POINT ( 'NONE',  ( 147.1125781744767949, 275.8405354997948962, -5.216646253929903665 ) ) ;
#2956=CARTESIAN_POINT ( 'NONE',  ( 201.9589676041426003, 280.8438023959050156, 17.68527200368066943 ) ) ;
#2959=CARTESIAN_POINT ( 'NONE',  ( 193.8272087209040251, 288.0738267443611562, 16.53761133020671181 ) ) ;
#2961=CARTESIAN_POINT ( 'NONE',  ( 136.8541387121310038, 236.4865022471901455, 1.119607411625061291E-15 ) ) ;
#2962=CARTESIAN_POINT ( 'NONE',  ( 21.88130812447325368, 171.8932355074535678, -2.679491924311248496 ) ) ;
#2966=CARTESIAN_POINT ( 'NONE',  ( 188.3087462637927842, 273.2467909115973157, 15.60395914083236946 ) ) ;
#2968=CARTESIAN_POINT ( 'NONE',  ( 202.6560281492536717, 279.6364581158209717, 17.15553667345918853 ) ) ;
#2970=CARTESIAN_POINT ( 'NONE',  ( 201.3715986869907510, 281.8611552031986776, -17.89433714524984964 ) ) ;
#2971=ORIENTED_EDGE ( 'NONE', *, *, #13120, .F. ) ;
#2973=VERTEX_POINT ( 'NONE', #81577 ) ;
#2974=EDGE_CURVE ( 'NONE', #88081, #4549, #42478, .T. ) ;
#2976=CARTESIAN_POINT ( 'NONE',  ( 170.3932416883117753, 250.2835119183525308, 3.409375801508330639 ) ) ;
#2977=CARTESIAN_POINT ( 'NONE',  ( 201.4520623681621316, 281.7217880192456505, -17.56577389517433119 ) ) ;
#2978=AXIS2_PLACEMENT_3D ( 'NONE', #44180, #4720, #5205 ) ;
#2984=CARTESIAN_POINT ( 'NONE',  ( 85.83080867249778123, 210.3615022471902023, 5.000000000000051514 ) ) ;
#2988=CARTESIAN_POINT ( 'NONE',  ( 183.2998219562535667, 295.8549255701772154, 1.009210091351407490 ) ) ;
#2991=CARTESIAN_POINT ( 'NONE',  ( 194.7576540903134799, 293.3168432830895540, -14.62421624641040196 ) ) ;
#2993=CARTESIAN_POINT ( 'NONE',  ( 194.4889937320412230, 293.7821766735966662, 14.99892588346621380 ) ) ;
#2995=CARTESIAN_POINT ( 'NONE',  ( 157.7847820078105201, 257.3557362317297361, -18.02899742403477035 ) ) ;
#2996=CARTESIAN_POINT ( 'NONE',  ( 164.5591015285399408, 245.6222706351205147, 4.316513966039805084 ) ) ;
#2997=CARTESIAN_POINT ( 'NONE',  ( 169.3663320018198988, 267.2185400183821002, 16.84669842072003476 ) ) ;
#2998=AXIS2_PLACEMENT_3D ( 'NONE', #23502, #46822, #87414 ) ;
#3000=CARTESIAN_POINT ( 'NONE',  ( 78.60473566001486745, 222.3149278399160664, 9.188101187500093303 ) ) ;
#3002=CARTESIAN_POINT ( 'NONE',  ( 150.4606192027571581, 271.6476180253717416, 12.81392864905067874 ) ) ;
#3003=CARTESIAN_POINT ( 'NONE',  ( 163.1660300598458377, 276.5360652196470710, -13.90274221281887534 ) ) ;
#3007=CARTESIAN_POINT ( 'NONE',  ( 191.0604813119340690, 299.7205343796033503, -9.270812881586136811 ) ) ;
#3009=CARTESIAN_POINT ( 'NONE',  ( 206.2041691044954348, 273.4908977089264113, -9.455375957961031474 ) ) ;
#3011=CARTESIAN_POINT ( 'NONE',  ( 85.85769841670953895, 226.5024278399160664, -9.188101187500093303 ) ) ;
#3016=CARTESIAN_POINT ( 'NONE',  ( 207.9328781051891042, 270.4966858882232259, -0.8820402142964423042 ) ) ;
#3017=ORIENTED_EDGE ( 'NONE', *, *, #70166, .T. ) ;
#3019=AXIS2_PLACEMENT_3D ( 'NONE', #44601, #98345, #28936 ) ;
#3022=CARTESIAN_POINT ( 'NONE',  ( -11.32641631811692662, 174.2677522451419350, -5.000000000000047962 ) ) ;
#3025=CARTESIAN_POINT ( 'NONE',  ( 156.6938127249734976, 259.2453504591003934, 17.44495368413245728 ) ) ;
#3026=CARTESIAN_POINT ( 'NONE',  ( 160.7333616651760622, 275.5160038079451397, 13.07907024587930245 ) ) ;
#3027=CARTESIAN_POINT ( 'NONE',  ( 191.2827847134780654, 298.6246597018299553, 8.274781095337747416 ) ) ;
#3028=CARTESIAN_POINT ( 'NONE',  ( 152.2788729538580696, 278.4366366002627160, 5.141355727269526277 ) ) ;
#3029=CARTESIAN_POINT ( 'NONE',  ( 174.8134674376002522, 283.6915436203280478, 13.42846482262391028 ) ) ;
#3034=CARTESIAN_POINT ( 'NONE',  ( 200.7079229450794173, 283.0106753079404029, 16.90512463913211505 ) ) ;
#3037=CARTESIAN_POINT ( 'NONE',  ( 167.6339060968662977, 249.9402736688152515, 7.007630826504156474 ) ) ;
#3039=CARTESIAN_POINT ( 'NONE',  ( 109.0771152426536190, 245.3297689869269220, -2.679491924311252493 ) ) ;
#3040=CARTESIAN_POINT ( 'NONE',  ( 163.1454208480229511, 248.0708373994541773, -10.54743435624756742 ) ) ;
#3044=CARTESIAN_POINT ( 'NONE',  ( 206.8986117509267899, 272.2880877623646825, 6.975890063856878598 ) ) ;
#3045=CARTESIAN_POINT ( 'NONE',  ( 180.5523533409438812, 267.1348689491979371, -15.92591746638905015 ) ) ;
#3046=CARTESIAN_POINT ( 'NONE',  ( 181.9612031435554229, 264.0215097815707281, 13.83388833630109183 ) ) ;
#3047=CARTESIAN_POINT ( 'NONE',  ( 199.7141866094727334, 282.2205715192249613, -16.63415621045345105 ) ) ;
#3050=DIRECTION ( 'NONE',  ( -0.8660254037844387076, -0.4999999999999998890, -0.000000000000000000 ) ) ;
#3052=CARTESIAN_POINT ( 'NONE',  ( 161.0804023394942988, 273.4036736971156074, -15.32506370326049705 ) ) ;
#3055=CARTESIAN_POINT ( 'NONE',  ( 9.052243966459650792, 176.0333772461660828, 9.188101187500095079 ) ) ;
#3058=B_SPLINE_CURVE_WITH_KNOTS ( 'NONE', 3,
 ( #41803, #57000, #57501, #49914, #40292, #1827, #88480, #72750, #72237, #9931, #17513, #87982, #19042, #71235, #24609, #55490, #80871, #32710, #33214, #64623, #1325, #55985, #86476, #63610, #3343, #95578, #34219, #70711, #47893, #26123, #17004, #86982, #78835, #94549, #25104, #48418, #2332, #64112, #95064, #18031, #65605, #44292, #83339, #90955 ),
 .UNSPECIFIED., .F., .F.,
 ( 4, 2, 2, 2, 2, 2, 2, 2, 2, 2, 2, 2, 2, 2, 2, 2, 2, 2, 2, 2, 2, 4 ),
 ( 0.0002033711871256132782, 0.0006869211536439505947, 0.001170471120162287857, 0.001412246103421541544, 0.001654021086680795448, 0.001774908578310349216, 0.001895796069939902984, 0.002137571053198942216, 0.002621121019716995959, 0.003104670986235049703, 0.004071770919271142444, 0.005038870852307235186, 0.005522420818825281123, 0.005764195802084304959, 0.006005970785343327928, 0.006066414531158064588, 0.006126858276972801248, 0.006247745768602325743, 0.006489520751861375600, 0.006973070718379464905, 0.007456620684897553343, 0.007940170651415641781 ),
 .UNSPECIFIED. ) ;
#3062=CARTESIAN_POINT ( 'NONE',  ( 39.11982377592438809, 184.2048013555409796, 4.594050593750051981 ) ) ;
#3065=CARTESIAN_POINT ( 'NONE',  ( 146.8058449195592061, 276.3718130816831149, 4.181814292810413392 ) ) ;
#3067=CARTESIAN_POINT ( 'NONE',  ( 177.8525236415347024, 292.7868308833215565, 5.877363187741069694 ) ) ;
#3068=CARTESIAN_POINT ( 'NONE',  ( 176.3456817854797691, 291.4259432939911107, 2.560940383191315561 ) ) ;
#3069=CARTESIAN_POINT ( 'NONE',  ( 196.7881396906236944, 289.7999390593150224, 16.36925548999025537 ) ) ;
#3070=CARTESIAN_POINT ( 'NONE',  ( 182.4930781751271240, 280.1738083852680461, -16.09858767428634607 ) ) ;
#3072=B_SPLINE_SURFACE_WITH_KNOTS ( 'NONE', 3, 1, ( 
 ( #8719, #63417 ),
 ( #77638, #8223 ),
 ( #17830, #40094 ),
 ( #32523, #47209 ),
 ( #32001, #71037 ),
 ( #85785, #1123 ),
 ( #16315, #71537 ),
 ( #94356, #62393 ),
 ( #31009, #39091 ),
 ( #93350, #86777 ),
 ( #23908, #40601 ),
 ( #9743, #2130 ),
 ( #55785, #70005 ),
 ( #23400, #86275 ),
 ( #619, #33011 ),
 ( #24911, #48731 ),
 ( #63912, #78132 ),
 ( #17312, #39589 ),
 ( #56303, #94850 ),
 ( #54808, #70510 ),
 ( #62912, #93862 ),
 ( #25411, #46711 ),
 ( #41096, #61899 ),
 ( #92849, #24418 ),
 ( #54290, #55294 ),
 ( #16811, #47698 ),
 ( #42593, #3151 ),
 ( #43599, #10727 ),
 ( #34036, #58302 ),
 ( #64924, #12224 ),
 ( #19827, #50698 ),
 ( #42106, #35508 ),
 ( #58785, #95868 ),
 ( #4615, #18829 ) ),
 .UNSPECIFIED., .T., .F., .F.,
 ( 4, 2, 2, 2, 2, 2, 2, 2, 2, 2, 2, 2, 2, 2, 2, 2, 4 ),
 ( 2, 2 ),
 ( 0.000000000000000000, 0.06250000000000000000, 0.1250000000000000000, 0.1875000000000000000, 0.2500000000000000000, 0.3125000000000000000, 0.3750000000000000000, 0.4375000000000000000, 0.5000000000000000000, 0.5625000000000000000, 0.6250000000000000000, 0.6875000000000000000, 0.7500000000000000000, 0.8125000000000000000, 0.8750000000000000000, 0.9375000000000000000, 1.000000000000000000 ),
 ( 0.000000000000000000, 1.000000000000000000 ),
 .UNSPECIFIED. ) ;
#3073=CARTESIAN_POINT ( 'NONE',  ( 167.0943254138853717, 257.9640194188826285, -15.42997351562387642 ) ) ;
#3075=CARTESIAN_POINT ( 'NONE',  ( 91.45997379709665154, 213.6115022471902023, -5.000000000000041744 ) ) ;
#3077=CARTESIAN_POINT ( 'NONE',  ( 45.85867072306329817, 185.0327760586659451, 1.948934522072303157E-15 ) ) ;
#3078=CARTESIAN_POINT ( 'NONE',  ( -22.42236680055709641, 157.8615022471902591, 0.000000000000000000 ) ) ;
#3080=CARTESIAN_POINT ( 'NONE',  ( 163.1015652178793403, 263.5875002883286129, 17.00931977151094188 ) ) ;
#3081=CARTESIAN_POINT ( 'NONE',  ( 147.5634954182374372, 275.0595239235922236, 4.682022975662822439 ) ) ;
#3083=VERTEX_POINT ( 'NONE', #41528 ) ;
#3084=CARTESIAN_POINT ( 'NONE',  ( 168.2938362192519435, 285.1573150202705165, 7.602421082290971910 ) ) ;
#3085=CARTESIAN_POINT ( 'NONE',  ( 207.2383675728608239, 271.6996134166075763, 7.873592648726489784 ) ) ;
#3086=CARTESIAN_POINT ( 'NONE',  ( -27.42236680055714260, 166.5217562850347406, 1.224646799147364892E-15 ) ) ;
#3087=CARTESIAN_POINT ( 'NONE',  ( 191.0083787145144925, 298.9706005401350808, -7.573825802859819767 ) ) ;
#3089=CARTESIAN_POINT ( 'NONE',  ( 202.3139361598622372, 280.2289788223093865, 15.93832709035092421 ) ) ;
#3090=CARTESIAN_POINT ( 'NONE',  ( 148.9504735598738137, 272.6572073132907690, -11.88406006066344744 ) ) ;
#3091=CARTESIAN_POINT ( 'NONE',  ( 157.0482715255472215, 258.6314098073167997, 18.43444315619183271 ) ) ;
#3094=CARTESIAN_POINT ( 'NONE',  ( 189.0720805967732758, 299.7343203868808246, 4.955419684386629164 ) ) ;
#3095=CARTESIAN_POINT ( 'NONE',  ( 172.9532272929666306, 253.9275976348661743, 8.329286765949929006 ) ) ;
#3097=ORIENTED_EDGE ( 'NONE', *, *, #26150, .T. ) ;
#3100=CARTESIAN_POINT ( 'NONE',  ( 151.3560786774222322, 268.4905770267490652, 15.54402364351346932 ) ) ;
#3102=B_SPLINE_CURVE_WITH_KNOTS ( 'NONE', 3,
 ( #7657, #76096, #75579, #23344 ),
 .UNSPECIFIED., .F., .F.,
 ( 4, 4 ),
 ( 0.001104354452915805437, 0.009031582544426527970 ),
 .UNSPECIFIED. ) ;
#3103=CARTESIAN_POINT ( 'NONE',  ( -22.42236680055709641, 157.8615022471902591, 0.000000000000000000 ) ) ;
#3105=VERTEX_POINT ( 'NONE', #27346 ) ;
#3106=ORIENTED_EDGE ( 'NONE', *, *, #73261, .T. ) ;
#3107=CARTESIAN_POINT ( 'NONE',  ( 207.1432938686257046, 271.8642859028066141, -6.405155839440290322 ) ) ;
#3109=CARTESIAN_POINT ( 'NONE',  ( 149.4965729687386045, 271.7113353911534546, -11.48413836595348059 ) ) ;
#3111=CARTESIAN_POINT ( 'NONE',  ( 152.9273493951901628, 265.7690563111299298, -17.70273273795505631 ) ) ;
#3117=CARTESIAN_POINT ( 'NONE',  ( 205.2937235227012707, 275.0678357141204629, -12.80017165135291535 ) ) ;
#3118=EDGE_CURVE ( 'NONE', #33408, #39284, #47180, .T. ) ;
#3119=AXIS2_PLACEMENT_3D ( 'NONE', #10889, #11890, #12386 ) ;
#3121=CARTESIAN_POINT ( 'NONE',  ( 86.17361039128121547, 213.8927522451417929, -10.00000000000009237 ) ) ;
#3123=CARTESIAN_POINT ( 'NONE',  ( 164.0854748117396582, 246.4426161724408928, -5.757837433625331514 ) ) ;
#3126=CARTESIAN_POINT ( 'NONE',  ( 159.2876523829509665, 254.7526883847961017, 15.64395448151312351 ) ) ;
#3128=CARTESIAN_POINT ( 'NONE',  ( 59.87693630317638593, 211.5024278399160949, -9.188101187500093303 ) ) ;
#3130=CARTESIAN_POINT ( 'NONE',  ( 191.3638605175971747, 299.1950661814348678, 7.382965314423603154 ) ) ;
#3131=CARTESIAN_POINT ( 'NONE',  ( 198.0788209437629916, 287.5644135525011507, 18.31867165462247726 ) ) ;
#3132=CARTESIAN_POINT ( 'NONE',  ( 172.7371573690596449, 271.6299009131761864, 17.79590902495428040 ) ) ;
#3137=VERTEX_POINT ( 'NONE', #61715 ) ;
#3138=CARTESIAN_POINT ( 'NONE',  ( 171.7735634000264895, 259.5473476820295673, -13.86153561918547261 ) ) ;
#3140=CARTESIAN_POINT ( 'NONE',  ( 161.7412967960748915, 250.5028515975580774, -14.36228887024421041 ) ) ;
#3141=CARTESIAN_POINT ( 'NONE',  ( 206.7630081259394785, 270.7710843149401967, 2.449322393346784033 ) ) ;
#3143=CARTESIAN_POINT ( 'NONE',  ( 42.43386700773090325, 183.7592609112380444, 2.679491924311254714 ) ) ;
#3144=CARTESIAN_POINT ( 'NONE',  ( 152.2107918078027637, 269.9234269244417987, -14.46751604775859690 ) ) ;
#3145=CARTESIAN_POINT ( 'NONE',  ( 164.1289849693733913, 253.9388421045659072, 14.48896490727248043 ) ) ;
#3146=CARTESIAN_POINT ( 'NONE',  ( 164.2090401137261892, 246.2285947913476889, -5.787448100099915393 ) ) ;
#3147=CARTESIAN_POINT ( 'NONE',  ( 119.6326891643026471, 246.0024278399160949, -9.188101187500093303 ) ) ;
#3151=CARTESIAN_POINT ( 'NONE',  ( 155.0453531195792038, 262.1005662498678817, -18.46987289964740953 ) ) ;
#3153=CARTESIAN_POINT ( 'NONE',  ( -7.772103719870364635, 172.9865022471903160, 10.00000000000009415 ) ) ;
#3157=CARTESIAN_POINT ( 'NONE',  ( 158.3970702420060945, 275.2847853859153133, -12.36479235985845904 ) ) ;
#3158=CARTESIAN_POINT ( 'NONE',  ( 147.6970978007492761, 275.3689941975056286, 3.616184303788550825 ) ) ;
#3159=CARTESIAN_POINT ( 'NONE',  ( 182.0448786185565950, 260.4843149835525082, 9.534127780721211920 ) ) ;
#3160=CARTESIAN_POINT ( 'NONE',  ( 154.5391432594492755, 279.1751768281744717, -6.541910729268716196 ) ) ;
#3161=CARTESIAN_POINT ( 'NONE',  ( 149.7817191771959244, 245.0327760586659451, 1.948934522072302763E-15 ) ) ;
#3162=CARTESIAN_POINT ( 'NONE',  ( 18.26047324907200675, 192.8967562850347122, -4.648177544792955347E-16 ) ) ;
#3164=CARTESIAN_POINT ( 'NONE',  ( 65.61435460324827318, 214.8149278399160664, 9.188101187500093303 ) ) ;
#3165=ADVANCED_FACE ( 'NONE', ( #90686 ), #61218, .T. ) ;
#3166=CARTESIAN_POINT ( 'NONE',  ( 170.6732825991835796, 250.4417675700726420, 3.839369570936610021 ) ) ;
#3168=CARTESIAN_POINT ( 'NONE',  ( 149.6700657135140489, 271.4108371424580355, 12.58635654151485284 ) ) ;
#3169=CARTESIAN_POINT ( 'NONE',  ( 190.3081770915147217, 296.7547009589226832, -11.12978463209281799 ) ) ;
#3171=CARTESIAN_POINT ( 'NONE',  ( 203.1526193585190470, 278.7763369107815379, -16.67658907091021447 ) ) ;
#3172=CARTESIAN_POINT ( 'NONE',  ( 195.8377875905904659, 289.9203488409928013, 16.32594698151886092 ) ) ;
#3174=CARTESIAN_POINT ( 'NONE',  ( 115.4741365526546275, 244.1427522451419350, 10.00000000000009237 ) ) ;
#3177=EDGE_CURVE ( 'NONE', #45420, #31691, #65313, .T. ) ;
#3178=CARTESIAN_POINT ( 'NONE',  ( 196.2048238403250764, 290.8102717488927169, 17.53926796892840656 ) ) ;
#3179=CARTESIAN_POINT ( 'NONE',  ( 190.4750160083620472, 300.7345900314585947, -1.159659205620361400 ) ) ;
#3181=CARTESIAN_POINT ( 'NONE',  ( -0.9067010812963882671, 158.0327760586659451, 1.948934522072302763E-15 ) ) ;
#3182=CARTESIAN_POINT ( 'NONE',  ( 46.18343024948246978, 185.2202760586659736, -5.415160957724236172E-17 ) ) ;
#3184=CARTESIAN_POINT ( 'NONE',  ( 192.7218293306584656, 264.9217214401847400, 8.853126855886975122 ) ) ;
#3186=CYLINDRICAL_SURFACE ( 'NONE', #6046, 17.82106496071139645 ) ;
#3188=CARTESIAN_POINT ( 'NONE',  ( 192.5691088913182796, 292.3284985076070939, -14.35085839917381101 ) ) ;
#3189=CARTESIAN_POINT ( 'NONE',  ( 147.5498377207569263, 275.0831797495432056, 4.097967709737811326 ) ) ;
#3191=CARTESIAN_POINT ( 'NONE',  ( 170.9108195568088888, 258.2889562468841973, 13.94820864694325202 ) ) ;
#3192=CARTESIAN_POINT ( 'NONE',  ( 53.62548896571598078, 211.7677522451419350, -5.000000000000047962 ) ) ;
#3193=CARTESIAN_POINT ( 'NONE',  ( 163.0642942239685738, 256.3512231501143219, -15.96636853477880003 ) ) ;
#3194=CARTESIAN_POINT ( 'NONE',  ( 205.2414727015710412, 275.1583367910551488, -12.71338796362297963 ) ) ;
#3195=CARTESIAN_POINT ( 'NONE',  ( 150.3996455637841621, 270.1471677736116703, 15.13740740754872327 ) ) ;
#3197=CARTESIAN_POINT ( 'NONE',  ( 48.66388509341562241, 192.2365022471902023, -10.00000000000009059 ) ) ;
#3198=CARTESIAN_POINT ( 'NONE',  ( 185.1034421103952923, 294.2212680083668488, 9.756692795348159919 ) ) ;
#3199=CARTESIAN_POINT ( 'NONE',  ( 163.1008115941903895, 248.1481028935802442, 11.25332017433677834 ) ) ;
#3200=CARTESIAN_POINT ( 'NONE',  ( -0.8802452050168975139, 179.4869531367911293, 4.594050593750046652 ) ) ;
#3202=CARTESIAN_POINT ( 'NONE',  ( 164.3036517873781008, 252.3706336020835579, 13.60069832213670082 ) ) ;
#3203=CARTESIAN_POINT ( 'NONE',  ( 192.5712965840290849, 297.1037255674836501, 11.03742858512898906 ) ) ;
#3206=CARTESIAN_POINT ( 'NONE',  ( 183.2977132992604368, 278.9993326301736261, 16.98963108586711712 ) ) ;
#3207=CARTESIAN_POINT ( 'NONE',  ( 191.5520471495731840, 262.7669810543075641, 7.572277432245083872 ) ) ;
#3208=CARTESIAN_POINT ( 'NONE',  ( 178.3071527192634562, 261.8922108035372389, -12.91157669021449195 ) ) ;
#3210=CARTESIAN_POINT ( 'NONE',  ( 167.0271109968743417, 287.8086958075197686, 0.5416428030073258126 ) ) ;
#3213=CARTESIAN_POINT ( 'NONE',  ( 67.50789586100057704, 221.3297689869269504, -2.679491924311252493 ) ) ;
#3214=CARTESIAN_POINT ( 'NONE',  ( 153.0539157576005209, 277.5780052395393795, -5.206865708505814538 ) ) ;
#3215=CARTESIAN_POINT ( 'NONE',  ( 156.8874040700877117, 276.4568989644782278, 10.40147400811322420 ) ) ;
#3216=CARTESIAN_POINT ( 'NONE',  ( 159.4491226731523454, 254.4730136382542582, -15.39140229921534520 ) ) ;
#3219=CARTESIAN_POINT ( 'NONE',  ( 152.7314557461996571, 266.1083540640618708, 17.39314074348802208 ) ) ;
#3222=ORIENTED_EDGE ( 'NONE', *, *, #9052, .T. ) ;
#3224=CARTESIAN_POINT ( 'NONE',  ( 156.0916382163451601, 277.5285333452508212, -10.52960063827285886 ) ) ;
#3228=CARTESIAN_POINT ( 'NONE',  ( 178.3112482654562996, 264.0450902665834860, 14.95807064277194698 ) ) ;
#3229=EDGE_LOOP ( 'NONE', ( #70706, #95231, #49675, #30782 ) ) ;
#3231=ADVANCED_FACE ( 'NONE', ( #44008 ), #70377, .F. ) ;
#3232=CARTESIAN_POINT ( 'NONE',  ( 162.9821135744430478, 258.3369963296131004, -16.89381123770511195 ) ) ;
#3235=CARTESIAN_POINT ( 'NONE',  ( 174.0669043376117600, 267.5140543244703508, 16.51994157467699509 ) ) ;
#3236=CARTESIAN_POINT ( 'NONE',  ( 168.8717317207870963, 276.2693029408995358, -16.23631712967058860 ) ) ;
#3239=CARTESIAN_POINT ( 'NONE',  ( 171.2643466405970401, 254.4411532906372599, -11.87753971852902701 ) ) ;
#3242=CARTESIAN_POINT ( 'NONE',  ( 160.3032094352624597, 268.8024171257220587, -16.64298077618573757 ) ) ;
#3244=CARTESIAN_POINT ( 'NONE',  ( 176.1640045926653499, 252.3529155287689321, -3.563159428949892682 ) ) ;
#3245=ORIENTED_EDGE ( 'NONE', *, *, #52583, .T. ) ;
#3246=CARTESIAN_POINT ( 'NONE',  ( 166.0416043136671931, 271.3796547996244612, 16.27046467588942846 ) ) ;
#3247=CARTESIAN_POINT ( 'NONE',  ( 147.2754198212952303, 275.5584854939172601, 7.218566409973668385 ) ) ;
#3248=CARTESIAN_POINT ( 'NONE',  ( 177.3417901484068295, 288.7674540264798111, -9.484566118077653485 ) ) ;
#3253=CARTESIAN_POINT ( 'NONE',  ( 197.1461414061409130, 289.1798618988426597, -16.76433772241966835 ) ) ;
#3255=CARTESIAN_POINT ( 'NONE',  ( 160.3083099072513846, 277.9173855857870308, -12.60700862289685809 ) ) ;
#3260=ORIENTED_EDGE ( 'NONE', *, *, #41666, .T. ) ;
#3261=CARTESIAN_POINT ( 'NONE',  ( 190.3538263673709423, 300.9444966470061900, 5.721980729251035847 ) ) ;
#3265=CARTESIAN_POINT ( 'NONE',  ( 199.4166651881534449, 285.2471993486035444, -17.96931216571487511 ) ) ;
#3268=EDGE_LOOP ( 'NONE', ( #42673, #98072, #9177, #22911 ) ) ;
#3269=CARTESIAN_POINT ( 'NONE',  ( 181.1374228341973662, 274.2894623748312597, -17.79777986536515755 ) ) ;
#3271=CARTESIAN_POINT ( 'NONE',  ( 44.46005344233068257, 203.1427522451419350, -10.00000000000009592 ) ) ;
#3272=CARTESIAN_POINT ( 'NONE',  ( -10.31836507581447471, 176.3967562850347406, -4.648177544792955347E-16 ) ) ;
#3273=CARTESIAN_POINT ( 'NONE',  ( 25.04665064082954729, 185.2677522451418497, 10.00000000000009592 ) ) ;
#3274=CARTESIAN_POINT ( 'NONE',  ( 109.7008941843561445, 224.9548013555409796, -4.594050593750042211 ) ) ;
#3276=CARTESIAN_POINT ( 'NONE',  ( 171.0056477905797863, 288.0889058818636386, -7.731614188742962135 ) ) ;
#3277=CARTESIAN_POINT ( 'NONE',  ( 162.2049812978500540, 253.7488527073383864, -15.21977816412132611 ) ) ;
#3278=CARTESIAN_POINT ( 'NONE',  ( 14.27519936121077926, 188.2369531367911293, -4.594050593750048428 ) ) ;
#3281=CARTESIAN_POINT ( 'NONE',  ( 168.2356071464602962, 248.8554872198452301, 6.669745218284529820 ) ) ;
#3282=ORIENTED_EDGE ( 'NONE', *, *, #41263, .T. ) ;
#3284=CARTESIAN_POINT ( 'NONE',  ( 187.3379511102435799, 261.0847295920454485, -5.858954167403199520 ) ) ;
#3287=CARTESIAN_POINT ( 'NONE',  ( 172.2467550100553808, 258.4300157609564508, -14.58559033337875377 ) ) ;
#3289=CARTESIAN_POINT ( 'NONE',  ( 207.3646600298985447, 271.4808684644054324, -5.284084612275558257 ) ) ;
#3291=CARTESIAN_POINT ( 'NONE',  ( 108.6384560342674064, 221.9824982072974251, 3.021315404115420679E-15 ) ) ;
#3292=CARTESIAN_POINT ( 'NONE',  ( 44.12627281972940807, 196.2833772461660828, -9.188101187500095079 ) ) ;
#3293=CARTESIAN_POINT ( 'NONE',  ( 70.58515312316123413, 224.8927522451419350, 2.944929066748280225E-16 ) ) ;
#3294=ORIENTED_EDGE ( 'NONE', *, *, #56721, .T. ) ;
#3297=CARTESIAN_POINT ( 'NONE',  ( -2.070769811622779510, 169.6115022471902591, 10.00000000000009592 ) ) ;
#3298=CARTESIAN_POINT ( 'NONE',  ( -8.349714312657674498, 175.1744531367911293, 4.594050593750047540 ) ) ;
#3300=CARTESIAN_POINT ( 'NONE',  ( 198.7136873185829984, 286.4647927352960437, -18.57144721070432070 ) ) ;
#3302=CARTESIAN_POINT ( 'NONE',  ( 147.2089949622447875, 275.6735367246781720, -3.633014386235353221 ) ) ;
#3304=CARTESIAN_POINT ( 'NONE',  ( 163.8670932201372352, 246.8208641845333773, 5.912697114930636211 ) ) ;
#3305=DIRECTION ( 'NONE',  ( 0.8660254037844395958, 0.4999999999999985567, 0.000000000000000000 ) ) ;
#3306=CARTESIAN_POINT ( 'NONE',  ( 207.3062152119541679, 271.5820978585240368, 7.879821064966149535 ) ) ;
#3309=CARTESIAN_POINT ( 'NONE',  ( 207.6932907333322191, 270.9116633891313199, 2.120963121341169710 ) ) ;
#3310=CARTESIAN_POINT ( 'NONE',  ( -5.895715345004106211, 180.7365022471903444, 2.944929066748280225E-16 ) ) ;
#3312=CARTESIAN_POINT ( 'NONE',  ( 127.2647115830355347, 244.2833772461660544, -9.188101187500095079 ) ) ;
#3316=CARTESIAN_POINT ( 'NONE',  ( 151.1268740129666526, 270.4373661374733615, 13.95431671769892823 ) ) ;
#3317=CARTESIAN_POINT ( 'NONE',  ( 157.7233946900069839, 257.4620621851055375, 16.86796251324260254 ) ) ;
#3320=CARTESIAN_POINT ( 'NONE',  ( 190.8001679306945277, 300.1714103817999444, 7.815449226872675403 ) ) ;
#3321=CARTESIAN_POINT ( 'NONE',  ( 149.7072529793668707, 271.3464269086063041, -11.98883662638834657 ) ) ;
#3322=CARTESIAN_POINT ( 'NONE',  ( 193.0126352936363503, 264.4189281174865869, 8.906082567666748773 ) ) ;
#3323=CARTESIAN_POINT ( 'NONE',  ( 175.8552468537395725, 291.6480507690039872, -1.084866266826680192 ) ) ;
#3327=B_SPLINE_CURVE_WITH_KNOTS ( 'NONE', 3,
 ( #31912, #84180, #62817, #14730 ),
 .UNSPECIFIED., .F., .F.,
 ( 4, 4 ),
 ( 0.03150042049964920515, 0.04052083632573695582 ),
 .UNSPECIFIED. ) ;
#3328=CARTESIAN_POINT ( 'NONE',  ( 175.9876842035281186, 278.7540883045039095, 15.46622700675096240 ) ) ;
#3329=CARTESIAN_POINT ( 'NONE',  ( 168.9176169510960506, 271.9055336743668363, -16.92632823138126952 ) ) ;
#3332=CARTESIAN_POINT ( 'NONE',  ( 196.3460172103508228, 270.8952704866825343, 12.02876777916156570 ) ) ;
#3334=CARTESIAN_POINT ( 'NONE',  ( 175.0809028706871118, 261.2525943152746208, 15.25527675994286092 ) ) ;
#3336=CARTESIAN_POINT ( 'NONE',  ( 153.3127735718713609, 265.1014820546527631, 17.57722645152040641 ) ) ;
#3337=EDGE_CURVE ( 'NONE', #51615, #45796, #52840, .T. ) ;
#3339=DIRECTION ( 'NONE',  ( 0.4999999999999992784, -0.8660254037844390407, 0.000000000000000000 ) ) ;
#3341=CARTESIAN_POINT ( 'NONE',  ( 191.8232983172789261, 287.9405117321300054, -15.86170699942114659 ) ) ;
#3342=EDGE_LOOP ( 'NONE', ( #59544, #46564 ) ) ;
#3343=CARTESIAN_POINT ( 'NONE',  ( 167.0385653880582311, 280.6345426807069998, 11.66514859715476859 ) ) ;
#3344=CARTESIAN_POINT ( 'NONE',  ( 194.5252985417586729, 293.7192948986070178, -14.54632727629426370 ) ) ;
#3346=CARTESIAN_POINT ( 'NONE',  ( 107.7317227740038987, 244.5530062829863311, -4.648177544792955347E-16 ) ) ;
#3349=EDGE_CURVE ( 'NONE', #49368, #37697, #77535, .T. ) ;
#3352=CARTESIAN_POINT ( 'NONE',  ( 198.1679321590325458, 277.6257778925182720, -16.56331389466651061 ) ) ;
#3361=B_SPLINE_CURVE_WITH_KNOTS ( 'NONE', 3,
 ( #37476, #15679, #99312, #61282 ),
 .UNSPECIFIED., .F., .F.,
 ( 4, 4 ),
 ( 0.001425702847953698189, 0.001426788465073381296 ),
 .UNSPECIFIED. ) ;
#3364=CARTESIAN_POINT ( 'NONE',  ( 154.8579861482817535, 262.4250953638155011, -17.69813260923097786 ) ) ;
#3367=CARTESIAN_POINT ( 'NONE',  ( 189.9707338884078638, 301.6080322845677415, 2.301871164863099395 ) ) ;
#3368=CARTESIAN_POINT ( 'NONE',  ( 161.9937702561999515, 277.3490201517574292, -12.90888215145142937 ) ) ;
#3369=CARTESIAN_POINT ( 'NONE',  ( 193.1028332910263998, 296.1830769848763225, -12.04975758233223893 ) ) ;
#3373=CARTESIAN_POINT ( 'NONE',  ( 135.2750994722765654, 261.1589784336661637, -6.496448406907675876E-16 ) ) ;
#3374=B_SPLINE_CURVE_WITH_KNOTS ( 'NONE', 3,
 ( #30001, #39080, #62382, #69992, #77626, #31991, #16303, #85773, #93852, #15793, #114, #61396, #30505, #38081, #92347, #38595, #99920, #22896, #8708, #39575, #47196, #91846, #15285, #7197, #61884, #607, #14313, #53781, #22408, #31490, #45198, #1113, #46181, #46699, #76138, #93339 ),
 .UNSPECIFIED., .F., .F.,
 ( 4, 2, 2, 2, 2, 2, 2, 2, 2, 2, 2, 2, 2, 2, 2, 2, 2, 4 ),
 ( 0.001074311027334474630, 0.001255084196826616264, 0.001435857366318757898, 0.001797403705303101448, 0.002520496383271696172, 0.003966681739208911643, 0.004689774417177518945, 0.005051320756161901092, 0.005232093925654099538, 0.005322480510400157128, 0.005412867095146215585, 0.005458060387519308998, 0.005503253679892403279, 0.005593640264638590105, 0.005774413434130967228, 0.006135959773115820352, 0.006497506112100673477, 0.006859052451085527469 ),
 .UNSPECIFIED. ) ;
#3376=B_SPLINE_CURVE_WITH_KNOTS ( 'NONE', 3,
 ( #74850, #43413, #36813, #5922, #51014, #81965, #28220, #12541, #90067, #56748, #67723, #72485, #3087, #33978, #5431, #20637 ),
 .UNSPECIFIED., .F., .F.,
 ( 4, 2, 2, 2, 2, 2, 2, 4 ),
 ( 2.934965519869990483E-17, 0.0003787177898467209997, 0.0007574355796934127260, 0.001136153369540104235, 0.001514871159386795962, 0.001893588949233487688, 0.002272306739080179414, 0.003029742318773616643 ),
 .UNSPECIFIED. ) ;
#3378=EDGE_LOOP ( 'NONE', ( #28357, #63527, #37847, #4040 ) ) ;
#3379=CARTESIAN_POINT ( 'NONE',  ( 204.0723286345250926, 271.5096690584438761, 9.850150987350732024 ) ) ;
#3382=CARTESIAN_POINT ( 'NONE',  ( 202.3421728196210552, 280.1800714929709670, 16.85915999540957344 ) ) ;
#3384=LINE ( 'NONE', #28020, #56298 ) ;
#3385=CARTESIAN_POINT ( 'NONE',  ( 157.8501323257721083, 280.8042112442767007, -7.123878780571343050 ) ) ;
#3386=CYLINDRICAL_SURFACE ( 'NONE', #48073, 10.00000000000010658 ) ;
#3387=CARTESIAN_POINT ( 'NONE',  ( 172.0111262547279125, 280.2166085468118126, 13.88871956038429190 ) ) ;
#3389=CARTESIAN_POINT ( 'NONE',  ( 177.2202596218039048, 256.1409925865689843, -7.582792283667149746 ) ) ;
#3391=CARTESIAN_POINT ( 'NONE',  ( 194.6050500505458842, 285.5465367126718093, -17.70104686455487553 ) ) ;
#3393=CARTESIAN_POINT ( 'NONE',  ( 163.8398204947978627, 278.2177931945711862, 13.52153232863776289 ) ) ;
#3394=CARTESIAN_POINT ( 'NONE',  ( 200.9826050441883183, 267.6805681769415060, -2.536256614860724845 ) ) ;
#3395=CARTESIAN_POINT ( 'NONE',  ( 164.0110128646736598, 246.5715880479891382, -7.582345067072046696 ) ) ;
#3397=CARTESIAN_POINT ( 'NONE',  ( 162.6937333994314656, 248.8531830095558632, 10.02305144031113926 ) ) ;
#3398=CARTESIAN_POINT ( 'NONE',  ( 161.1867049071889824, 281.8197337930336630, -7.641306719448324181 ) ) ;
#3400=EDGE_CURVE ( 'NONE', #82839, #79646, #73568, .T. ) ;
#3402=ORIENTED_EDGE ( 'NONE', *, *, #67790, .F. ) ;
#3403=CARTESIAN_POINT ( 'NONE',  ( 1.210598108517954463, 183.0530062829863596, 2.649461200531984646E-14 ) ) ;
#3407=CIRCLE ( 'NONE', #69677, 17.82106496071138935 ) ;
#3410=B_SPLINE_CURVE_WITH_KNOTS ( 'NONE', 3,
 ( #47051, #94193, #70346, #38436, #69351, #39925, #9057, #70861, #16649, #76469, #31347, #47544, #24747, #1470, #62230, #32351, #54630, #15636, #77965, #22760, #7049, #84108, #92206, #69844, #78471, #85611, #68843, #14661, #63252, #8560, #37930, #77471, #53638, #54127, #45537, #84593, #456, #30354, #958, #61240, #76945, #93182, #7545, #23239, #31834, #100270, #23736, #30855 ),
 .UNSPECIFIED., .F., .F.,
 ( 4, 2, 2, 2, 2, 2, 2, 2, 2, 2, 2, 2, 2, 2, 2, 2, 2, 2, 2, 2, 2, 2, 2, 4 ),
 ( 0.0003844728647056017330, 0.001402722206477688372, 0.001911846877363706674, 0.002166409212806677878, 0.002293690380528164673, 0.002420971548249651467, 0.002675533883692692710, 0.002930096219135733520, 0.003439220890021694576, 0.004457470231793539926, 0.005475719573565384843, 0.005984844244451306867, 0.006239406579894231017, 0.006493968915337156034, 0.006557609499197887722, 0.006621250083058618542, 0.006684890666919349363, 0.006748531250780081051, 0.007003093586223157856, 0.007512218257109299323, 0.007766780592552338831, 0.008021342927995377473, 0.008275905263438416981, 0.008530467598881454755 ),
 .UNSPECIFIED. ) ;
#3411=CARTESIAN_POINT ( 'NONE',  ( 202.6560281492536717, 279.6364581158209717, 17.15553667345918853 ) ) ;
#3412=CARTESIAN_POINT ( 'NONE',  ( 3.097972219676621730, 184.8464784336661637, 1.353441290958777525E-15 ) ) ;
#3413=CARTESIAN_POINT ( 'NONE',  ( 111.8659576938172364, 226.2048013555410080, 4.594050593750051981 ) ) ;
#3414=CARTESIAN_POINT ( 'NONE',  ( 203.1705638993064156, 278.7452560544191442, -15.08126533799095093 ) ) ;
#3415=CARTESIAN_POINT ( 'NONE',  ( 162.8386403195304410, 249.0994062285972461, 10.29435687412694911 ) ) ;
#3416=CARTESIAN_POINT ( 'NONE',  ( 179.9997804975865563, 255.3430733840098696, -2.381954882531521100 ) ) ;
#3417=ADVANCED_FACE ( 'NONE', ( #42406 ), #90580, .F. ) ;
#3419=CARTESIAN_POINT ( 'NONE',  ( 197.1346277874646375, 285.2336655192412991, 17.81342416061711376 ) ) ;
#3420=CARTESIAN_POINT ( 'NONE',  ( 160.2798150919779232, 282.6907811372386163, 5.236356400565768787 ) ) ;
#3422=CARTESIAN_POINT ( 'NONE',  ( 181.8525389448113287, 291.4924873961389267, 9.560256996614759473 ) ) ;
#3424=CARTESIAN_POINT ( 'NONE',  ( 205.3532617248650922, 274.9647125229813582, -13.76587875506490199 ) ) ;
#3426=CARTESIAN_POINT ( 'NONE',  ( 166.2132108024410400, 253.5770524951610412, -13.49425642745076459 ) ) ;
#3429=CARTESIAN_POINT ( 'NONE',  ( 84.66726058227095564, 213.5643266524160140, 9.188101187500095079 ) ) ;
#3430=CARTESIAN_POINT ( 'NONE',  ( 207.6357208050208101, 271.0113774299547913, -6.790259683043212036 ) ) ;
#3433=CARTESIAN_POINT ( 'NONE',  ( -22.42236680055709641, 157.8615022471902591, 0.000000000000000000 ) ) ;
#3435=CARTESIAN_POINT ( 'NONE',  ( 176.7763917151297903, 270.1915396991327043, -17.04233178615594113 ) ) ;
#3441=CARTESIAN_POINT ( 'NONE',  ( 74.81622161422296813, 207.8768266524159856, -9.188101187500093303 ) ) ;
#3442=CARTESIAN_POINT ( 'NONE',  ( 170.5832237462292085, 288.4275712266821756, -1.073378329848412305 ) ) ;
#3443=CARTESIAN_POINT ( 'NONE',  ( 192.8301672656986341, 296.6553483942417415, -13.40355799340913556 ) ) ;
#3444=CARTESIAN_POINT ( 'NONE',  ( 201.9921138689924476, 280.7863913811041812, 16.46984661270056804 ) ) ;
#3447=CARTESIAN_POINT ( 'NONE',  ( 123.8637576553643100, 248.9865022471902876, -10.00000000000009415 ) ) ;
#3448=( BOUNDED_CURVE ( )  B_SPLINE_CURVE ( 2, ( #29303, #60165, #22189, #44978, #6499, #30287, #61174, #92142, #884 ),
 .UNSPECIFIED., .F., .T. ) 
 B_SPLINE_CURVE_WITH_KNOTS ( ( 3, 2, 2, 2, 3 ),
 ( 0.2620967741935483764, 0.2634408602150537515, 0.2661290322580645018, 0.2688172043010752521, 0.2701612903225806273 ),
 .UNSPECIFIED. ) 
 CURVE ( )  GEOMETRIC_REPRESENTATION_ITEM ( )  RATIONAL_B_SPLINE_CURVE ( ( 0.9330127018922194093, 0.9330127018922194093, 1.000000000000000000, 0.8660254037844387076, 1.000000000000000000, 0.8660254037844387076, 1.000000000000000000, 0.9330127018922194093, 0.9330127018922194093 ) ) 
 REPRESENTATION_ITEM ( '' )  );
#3450=EDGE_CURVE ( 'NONE', #81863, #33648, #99027, .T. ) ;
#3452=VERTEX_POINT ( 'NONE', #7278 ) ;
#3453=CARTESIAN_POINT ( 'NONE',  ( 169.5334234935042730, 248.6278552856955457, -1.925906227684481609 ) ) ;
#3455=CARTESIAN_POINT ( 'NONE',  ( 202.3894997978090373, 280.0980987621804275, 16.95659012541789323 ) ) ;
#3456=CARTESIAN_POINT ( 'NONE',  ( 207.4268178751038079, 270.9325979257727681, -1.158184821002688158 ) ) ;
#3461=ORIENTED_EDGE ( 'NONE', *, *, #74575, .F. ) ;
#3462=CARTESIAN_POINT ( 'NONE',  ( 189.3986374548728406, 289.9821967149230204, 14.43509327751535132 ) ) ;
#3464=CARTESIAN_POINT ( 'NONE',  ( 167.9378326867459919, 248.4084500838292797, 3.496453975134492076 ) ) ;
#3465=CARTESIAN_POINT ( 'NONE',  ( 157.8493099884071285, 257.7921011362392392, -16.71337817344635468 ) ) ;
#3468=ADVANCED_FACE ( 'NONE', ( #94920 ), #31530, .F. ) ;
#3477=CARTESIAN_POINT ( 'NONE',  ( 186.2976226307126524, 298.7307822690146395, 1.075632280427271992 ) ) ;
#3478=CARTESIAN_POINT ( 'NONE',  ( 204.3574891606595827, 276.6894411969685166, 13.41627538812899978 ) ) ;
#3479=CARTESIAN_POINT ( 'NONE',  ( 194.4666154385731431, 293.8209370148700827, -14.56896502715340702 ) ) ;
#3483=CARTESIAN_POINT ( 'NONE',  ( 187.6361772789746567, 291.3791347085116854, -13.85621784405196166 ) ) ;
#3484=CARTESIAN_POINT ( 'NONE',  ( 208.1115139972721977, 270.1872794470800159, -4.030174891007424876 ) ) ;
#3485=CARTESIAN_POINT ( 'NONE',  ( 165.9640472274821263, 265.7646867401422242, 16.70851906738806392 ) ) ;
#3486=CARTESIAN_POINT ( 'NONE',  ( 169.5007657120409874, 248.2156828994837099, -1.963647642838588503 ) ) ;
#3487=CARTESIAN_POINT ( 'NONE',  ( 109.7008941843561445, 224.9548013555409796, -4.594050593750042211 ) ) ;
#3489=CARTESIAN_POINT ( 'NONE',  ( 150.6655900823359389, 269.6865383554857090, 15.31288044136207205 ) ) ;
#3491=CARTESIAN_POINT ( 'NONE',  ( 166.7548757565938047, 278.1757261261363396, -13.35741561976894154 ) ) ;
#3492=VERTEX_POINT ( 'NONE', #96423 ) ;
#3497=CARTESIAN_POINT ( 'NONE',  ( 160.0081047537594543, 253.5048282741223602, -16.11956848123596941 ) ) ;
#3498=CARTESIAN_POINT ( 'NONE',  ( 163.1306191313178431, 248.0964747248268338, 10.50682697533535048 ) ) ;
#3499=CARTESIAN_POINT ( 'NONE',  ( 87.77910550741502504, 230.6744531367911293, 4.594050593750047540 ) ) ;
#3504=ORIENTED_EDGE ( 'NONE', *, *, #53633, .F. ) ;
#3507=CARTESIAN_POINT ( 'NONE',  ( 153.4475728592434791, 265.3059609131843217, 16.25445176718542584 ) ) ;
#3509=CARTESIAN_POINT ( 'NONE',  ( 142.3662031094091844, 246.8768266524159856, -9.188101187500091527 ) ) ;
#3511=CARTESIAN_POINT ( 'NONE',  ( -14.42967401501114999, 169.1427522451419065, 10.00000000000009237 ) ) ;
#3513=VERTEX_POINT ( 'NONE', #27496 ) ;
#3514=CARTESIAN_POINT ( 'NONE',  ( 204.6244483240926400, 276.2270543623566255, 13.10813453876796864 ) ) ;
#3515=CARTESIAN_POINT ( 'NONE',  ( 159.6438702623246968, 275.1686529806921158, 12.86435351470504962 ) ) ;
#3517=CARTESIAN_POINT ( 'NONE',  ( 192.3297092044942076, 271.8923391751263239, 14.13782850498305699 ) ) ;
#3518=CARTESIAN_POINT ( 'NONE',  ( 178.0095323540602124, 285.1773387558561694, 13.03190070314914628 ) ) ;
#3520=CARTESIAN_POINT ( 'NONE',  ( -22.42236680055709641, 157.8615022471902591, 0.000000000000000000 ) ) ;
#3522=CARTESIAN_POINT ( 'NONE',  ( 200.6129772034685175, 283.1751261563724142, 18.36811917402039640 ) ) ;
#3523=B_SPLINE_CURVE_WITH_KNOTS ( 'NONE', 3,
 ( #35166, #36156, #37643, #90423 ),
 .UNSPECIFIED., .F., .F.,
 ( 4, 4 ),
 ( 0.005280122280043920285, 0.01026413765061139072 ),
 .UNSPECIFIED. ) ;
#3524=CARTESIAN_POINT ( 'NONE',  ( 200.2093391412865060, 269.7417714514684803, 10.46510648850140157 ) ) ;
#3525=CARTESIAN_POINT ( 'NONE',  ( 159.9997000813754084, 253.5193855937126841, -16.28798248637880519 ) ) ;
#3527=CARTESIAN_POINT ( 'NONE',  ( 174.8675334118165665, 290.2565163415771394, -6.409605830264317738 ) ) ;
#3530=CARTESIAN_POINT ( 'NONE',  ( 207.6918009085542849, 270.9142438413412037, 7.009114282139513818 ) ) ;
#3531=CARTESIAN_POINT ( 'NONE',  ( 180.6314016098794184, 266.8740464315611121, -14.78152555368366272 ) ) ;
#3532=CARTESIAN_POINT ( 'NONE',  ( 192.7790337852146081, 267.5346380212243389, -12.58653425593504593 ) ) ;
#3537=CARTESIAN_POINT ( 'NONE',  ( 155.4495868485232108, 261.4004128932040203, -18.48326470492642315 ) ) ;
#3538=CARTESIAN_POINT ( 'NONE',  ( 181.8336903648691134, 273.8601736245342408, 16.48343320725793149 ) ) ;
#3539=CARTESIAN_POINT ( 'NONE',  ( 161.0616241103177515, 273.2725257209350502, -15.13342039239440240 ) ) ;
#3542=CARTESIAN_POINT ( 'NONE',  ( 22.31343150979137846, 177.5643266524160424, 9.188101187500095079 ) ) ;
#3546=CARTESIAN_POINT ( 'NONE',  ( 175.5746833524315775, 278.5347786252573314, 16.94864957847115505 ) ) ;
#3548=CARTESIAN_POINT ( 'NONE',  ( 40.17520546284541894, 187.8768266524160140, 9.188101187500096856 ) ) ;
#3550=CARTESIAN_POINT ( 'NONE',  ( 190.2236813008869660, 301.1699145145108218, -5.401374690107298093 ) ) ;
#3552=CARTESIAN_POINT ( 'NONE',  ( 178.6162270217735681, 291.6660180747913387, 6.059679334779388249 ) ) ;
#3553=CARTESIAN_POINT ( 'NONE',  ( 191.2211340522693774, 299.4422756709672626, -8.405362570633277741 ) ) ;
#3556=CARTESIAN_POINT ( 'NONE',  ( 165.3037345041042840, 257.2179537824439421, -14.95315835255182613 ) ) ;
#3558=CARTESIAN_POINT ( 'NONE',  ( 79.84079962965532218, 230.2365022471903444, 2.944929066748280225E-16 ) ) ;
#3560=EDGE_CURVE ( 'NONE', #68558, #43956, #83961, .T. ) ;
#3561=CARTESIAN_POINT ( 'NONE',  ( 161.7665152264152937, 267.7794624542035535, -16.93321476133663239 ) ) ;
#3562=CARTESIAN_POINT ( 'NONE',  ( 55.14129374593650113, 193.4548013555410080, -4.594050593750042211 ) ) ;
#3565=CARTESIAN_POINT ( 'NONE',  ( 146.8729474948188454, 276.2555880120147549, 3.934020695290606273 ) ) ;
#3568=CARTESIAN_POINT ( 'NONE',  ( 168.5910505471324257, 286.4687829538495976, 8.106709794022206594 ) ) ;
#3569=CARTESIAN_POINT ( 'NONE',  ( 206.9258336080761183, 272.2409381227055292, 6.776000910836894597 ) ) ;
#3573=CARTESIAN_POINT ( 'NONE',  ( 196.4170778717353585, 290.4426369823788718, -17.78762421190030452 ) ) ;
#3578=CARTESIAN_POINT ( 'NONE',  ( 173.6495897994842323, 254.4294486916353151, 8.278733075952791509 ) ) ;
#3581=ORIENTED_EDGE ( 'NONE', *, *, #32602, .F. ) ;
#3583=CARTESIAN_POINT ( 'NONE',  ( 191.4922467593309250, 298.9726946877590876, 7.604184559945784017 ) ) ;
#3584=CARTESIAN_POINT ( 'NONE',  ( 177.3608330322163908, 256.1156063845999711, -7.251559029670058720 ) ) ;
#3587=CARTESIAN_POINT ( 'NONE',  ( 207.8431546909062320, 270.6520914003897360, -6.441273666418043220 ) ) ;
#3589=CARTESIAN_POINT ( 'NONE',  ( 62.42776884207837895, 218.3967562850346837, -4.648177544792955347E-16 ) ) ;
#3592=CARTESIAN_POINT ( 'NONE',  ( 198.1230806404959139, 287.4877535090322453, 17.00698319228197164 ) ) ;
#3595=CARTESIAN_POINT ( 'NONE',  ( 204.8385597977314490, 275.8562024115307167, -12.64672659107585240 ) ) ;
#3596=CARTESIAN_POINT ( 'NONE',  ( 119.4704829489755724, 239.7833772461660544, -9.188101187500095079 ) ) ;
#3599=CARTESIAN_POINT ( 'NONE',  ( 66.04647798856640861, 220.4860189848785694, -2.679491924311252493 ) ) ;
#3601=CARTESIAN_POINT ( 'NONE',  ( 164.1146561143383167, 246.3920726737087534, -7.362905700427413436 ) ) ;
#3602=ORIENTED_EDGE ( 'NONE', *, *, #79291, .T. ) ;
#3604=CARTESIAN_POINT ( 'NONE',  ( 198.2414483977475754, 287.2827345394944700, 16.94931984969033678 ) ) ;
#3605=CARTESIAN_POINT ( 'NONE',  ( 204.7121744066665201, 275.6653527038535572, -12.51300999821487459 ) ) ;
#3606=CARTESIAN_POINT ( 'NONE',  ( 70.62149783858335184, 202.3923013555409796, 4.594050593750050204 ) ) ;
#3608=CARTESIAN_POINT ( 'NONE',  ( 190.8443993347725325, 300.0947993426467519, 8.522468760355437212 ) ) ;
#3609=CARTESIAN_POINT ( 'NONE',  ( 150.9158774466703221, 269.2530279239659308, 15.11407781020157515 ) ) ;
#3610=CARTESIAN_POINT ( 'NONE',  ( 175.7525910197133214, 278.2325559912325730, 16.72575950286108082 ) ) ;
#3617=CARTESIAN_POINT ( 'NONE',  ( 173.8847286580779326, 277.9849265731808146, -16.77224647300125326 ) ) ;
#3619=EDGE_CURVE ( 'NONE', #23455, #58437, #95818, .T. ) ;
#3620=CARTESIAN_POINT ( 'NONE',  ( 160.4332679175176963, 258.1579911225197179, -17.11564559875521141 ) ) ;
#3621=CARTESIAN_POINT ( 'NONE',  ( 206.4797064717481305, 270.5928626827364383, 2.315921482892212779 ) ) ;
#3623=CARTESIAN_POINT ( 'NONE',  ( 164.8537203408104972, 245.1119758834023230, 2.926011033004258355 ) ) ;
#3626=CARTESIAN_POINT ( 'NONE',  ( 167.2877554666358435, 256.3763460065391087, 13.71623913248891036 ) ) ;
#3628=CARTESIAN_POINT ( 'NONE',  ( 1.663964738649655661, 181.7677522451419350, -5.000000000000047962 ) ) ;
#3629=CARTESIAN_POINT ( 'NONE',  ( 122.5830220656496579, 232.3923013555409796, 4.594050593750050204 ) ) ;
#3631=CARTESIAN_POINT ( 'NONE',  ( 191.0933613939813540, 299.6635844069401173, -8.689828987424775164 ) ) ;
#3632=CARTESIAN_POINT ( 'NONE',  ( 15.66239703771868719, 191.3967562850346837, -4.648177544792955347E-16 ) ) ;
#3636=CARTESIAN_POINT ( 'NONE',  ( 174.2379957965557651, 251.2590728793752248, 3.639292605338433795 ) ) ;
#3639=CARTESIAN_POINT ( 'NONE',  ( 157.9225728654248257, 276.1116997103654285, -12.95724163227552239 ) ) ;
#3641=CARTESIAN_POINT ( 'NONE',  ( 206.9349434189263661, 269.8064106017384916, 1.784245431258210113 ) ) ;
#3642=CARTESIAN_POINT ( 'NONE',  ( 206.7074763235984562, 272.6191440336236838, -10.69202547607624609 ) ) ;
#3643=CARTESIAN_POINT ( 'NONE',  ( 142.3662031094092129, 246.8768266524159856, -9.188101187500093303 ) ) ;
#3644=CARTESIAN_POINT ( 'NONE',  ( 190.2236813008869660, 301.1699145145108218, -5.401374690107298093 ) ) ;
#3646=CARTESIAN_POINT ( 'NONE',  ( 174.6784134397683488, 251.9041659443967376, 3.568609730242054301 ) ) ;
#3647=B_SPLINE_SURFACE_WITH_KNOTS ( 'NONE', 3, 1, ( 
 ( #86992, #57013 ),
 ( #80373, #18041 ),
 ( #16520, #17014 ),
 ( #95588, #26134 ),
 ( #47906, #78848 ),
 ( #56520, #9429 ),
 ( #87992, #72761 ),
 ( #55997, #95074 ),
 ( #18540, #48934 ),
 ( #78342, #40305 ),
 ( #49423, #10944 ),
 ( #41814, #71243 ),
 ( #1838, #8924 ),
 ( #39790, #31699 ),
 ( #62606, #32719 ),
 ( #63623, #94560 ),
 ( #25115, #17522 ),
 ( #79873, #48429 ),
 ( #40802, #79377 ),
 ( #9939, #71748 ),
 ( #2340, #33223 ),
 ( #24224, #31310 ),
 ( #17111, #69811 ),
 ( #70826, #86091 ),
 ( #93659, #71338 ),
 ( #16615, #54595 ),
 ( #8525, #9019 ),
 ( #54097, #55104 ),
 ( #63217, #421 ),
 ( #924, #70311 ),
 ( #31800, #47511 ),
 ( #1435, #32316 ),
 ( #78438, #78952 ),
 ( #85577, #63721 ) ),
 .UNSPECIFIED., .T., .F., .F.,
 ( 4, 2, 2, 2, 2, 2, 2, 2, 2, 2, 2, 2, 2, 2, 2, 2, 4 ),
 ( 2, 2 ),
 ( 0.000000000000000000, 0.06250000000000000000, 0.1250000000000000000, 0.1875000000000000000, 0.2500000000000000000, 0.3125000000000000000, 0.3750000000000000000, 0.4375000000000000000, 0.5000000000000000000, 0.5625000000000000000, 0.6250000000000000000, 0.6875000000000000000, 0.7500000000000000000, 0.8125000000000000000, 0.8750000000000000000, 0.9375000000000000000, 1.000000000000000000 ),
 ( 0.000000000000000000, 1.000000000000000000 ),
 .UNSPECIFIED. ) ;
#3648=EDGE_CURVE ( 'NONE', #88304, #99270, #74813, .T. ) ;
#3650=CARTESIAN_POINT ( 'NONE',  ( 175.0864214957619822, 292.0986614963166517, -3.428571861336215054 ) ) ;
#3652=CARTESIAN_POINT ( 'NONE',  ( 169.8838196135249348, 285.4608273923216188, -7.965848187381914691 ) ) ;
#3653=CARTESIAN_POINT ( 'NONE',  ( 154.9067123643522734, 262.3406990819208886, -18.18534662427576265 ) ) ;
#3655=CARTESIAN_POINT ( 'NONE',  ( 193.6272073153312476, 288.5543963742453570, 16.06608169681408782 ) ) ;
#3656=CARTESIAN_POINT ( 'NONE',  ( 144.1251436611898953, 244.0177522451417644, 5.000000000000051514 ) ) ;
#3661=AXIS2_PLACEMENT_3D ( 'NONE', #53912, #75264, #76263 ) ;
#3662=CARTESIAN_POINT ( 'NONE',  ( 196.1241105319816143, 290.9500712997905794, 15.97146679939154268 ) ) ;
#3663=CARTESIAN_POINT ( 'NONE',  ( 190.4281805785508084, 300.8157113754859893, -1.233909217199055774 ) ) ;
#3664=CARTESIAN_POINT ( 'NONE',  ( -10.75808714510939090, 164.5958772461660544, -9.188101187500095079 ) ) ;
#3665=CARTESIAN_POINT ( 'NONE',  ( 33.89617418964321871, 196.5024278399160949, -9.188101187500093303 ) ) ;
#3666=CARTESIAN_POINT ( 'NONE',  ( 178.4777856415780946, 273.6615857960989047, -17.31426804045896617 ) ) ;
#3668=FACE_OUTER_BOUND ( 'NONE', #77964, .T. ) ;
#3669=CARTESIAN_POINT ( 'NONE',  ( 157.1965120183049578, 258.3746497421212780, -18.06591467563559306 ) ) ;
#3671=CARTESIAN_POINT ( 'NONE',  ( 146.8000281410530192, 276.3818880375922049, 4.652863924796177386 ) ) ;
#3673=CARTESIAN_POINT ( 'NONE',  ( 167.5121282280925925, 256.6568260522151945, 13.80861252335286515 ) ) ;
#3674=CARTESIAN_POINT ( 'NONE',  ( 67.98707691180791812, 223.3927522451419350, 2.944929066748280225E-16 ) ) ;
#3678=CARTESIAN_POINT ( 'NONE',  ( 43.39556388706024848, 195.8615022471902591, -10.00000000000009592 ) ) ;
#3679=CARTESIAN_POINT ( 'NONE',  ( -22.42236680055709641, 157.8615022471902591, 0.000000000000000000 ) ) ;
#3681=CARTESIAN_POINT ( 'NONE',  ( 4.668163907683432257, 167.3768266524159856, -9.188101187500091527 ) ) ;
#3683=CYLINDRICAL_SURFACE ( 'NONE', #20134, 17.82106496071139645 ) ;
#3684=CARTESIAN_POINT ( 'NONE',  ( 33.29424590502123493, 178.4824982072973683, 3.021315404115420679E-15 ) ) ;
#3686=CARTESIAN_POINT ( 'NONE',  ( 206.4943150373521803, 272.9883502116088039, 11.34100825923693101 ) ) ;
#3687=CARTESIAN_POINT ( 'NONE',  ( 180.1994282899806592, 277.1211297568123086, 16.31084869235452217 ) ) ;
#3688=CARTESIAN_POINT ( 'NONE',  ( 193.7999837595647250, 294.9755769528473479, 15.24609078262870199 ) ) ;
#3689=CARTESIAN_POINT ( 'NONE',  ( 196.2878005184348353, 290.6665519265632724, -16.69183432842427806 ) ) ;
#3690=CARTESIAN_POINT ( 'NONE',  ( 179.6275593323862267, 262.7184705051237188, -12.85240121697976612 ) ) ;
#3693=CARTESIAN_POINT ( 'NONE',  ( 172.3986314675530309, 263.7922717222033384, -16.89442142407995107 ) ) ;
#3697=ORIENTED_EDGE ( 'NONE', *, *, #51113, .F. ) ;
#3698=CARTESIAN_POINT ( 'NONE',  ( 155.8897943095830954, 276.0389231161490784, 10.29249315839296663 ) ) ;
#3701=PRODUCT_DEFINITION ( 'UNKNOWN', '', #60799, #41236 ) ;
#3702=CARTESIAN_POINT ( 'NONE',  ( 192.7944000592152634, 296.7172990131160759, 11.44860011299869740 ) ) ;
#3703=CARTESIAN_POINT ( 'NONE',  ( 206.9878665138179770, 272.1334939782196329, 6.566295309274049252 ) ) ;
#3707=CARTESIAN_POINT ( 'NONE',  ( 159.1993561622898596, 279.5966400365493882, -9.758000324901335176 ) ) ;
#3708=CARTESIAN_POINT ( 'NONE',  ( 72.26538907532096800, 200.9824982072973967, 3.021315404115420679E-15 ) ) ;
#3716=CARTESIAN_POINT ( 'NONE',  ( 196.9976074755333286, 289.4371302133026802, -16.79549473444794216 ) ) ;
#3721=CARTESIAN_POINT ( 'NONE',  ( 200.9110265982630779, 282.6588894614233141, 17.52479721249226685 ) ) ;
#3722=CARTESIAN_POINT ( 'NONE',  ( 166.5515458049821973, 274.4079129713531415, -15.18104102794923982 ) ) ;
#3725=CARTESIAN_POINT ( 'NONE',  ( 174.5155504680193417, 276.9095236141292844, -16.96454991327265205 ) ) ;
#3729=CARTESIAN_POINT ( 'NONE',  ( 156.6812872898450735, 261.2670451491295012, 0.000000000000000000 ) ) ;
#3731=CYLINDRICAL_SURFACE ( 'NONE', #89747, 17.82106496071139645 ) ;
#3732=ORIENTED_EDGE ( 'NONE', *, *, #73853, .F. ) ;
#3733=CARTESIAN_POINT ( 'NONE',  ( 168.6570739278365068, 272.7872155009642370, 15.97839558931424975 ) ) ;
#3734=CARTESIAN_POINT ( 'NONE',  ( 194.0793808334966570, 294.4916470253114085, 14.16320079385157626 ) ) ;
#3735=CYLINDRICAL_SURFACE ( 'NONE', #52900, 10.00000000000010658 ) ;
#3737=EDGE_CURVE ( 'NONE', #14175, #86029, #76396, .T. ) ;
#3740=CARTESIAN_POINT ( 'NONE',  ( 197.6052335461745599, 288.3846909869485557, -16.86014524025736350 ) ) ;
#3744=B_SPLINE_CURVE_WITH_KNOTS ( 'NONE', 3,
 ( #68238, #37335, #59122, #29259, #67245, #51040, #76367, #44439, #5952, #51552, #22148, #90606, #99161, #13568, #12570, #75371, #5459, #52537, #90095, #53039, #36343, #81997, #91090, #14054, #21655, #60127, #83994, #29749, #60621, #20663, #82991, #91576, #13076, #82514, #43937, #74876, #21172, #98175, #28754, #14558, #45433, #97196, #43446, #59633, #52053, #36846, #83488, #6939, #67754, #74388, #44933, #27763 ),
 .UNSPECIFIED., .F., .F.,
 ( 4, 2, 2, 2, 2, 2, 2, 2, 2, 2, 2, 2, 2, 2, 2, 2, 2, 2, 2, 2, 2, 2, 2, 2, 2, 4 ),
 ( 0.0002156964707596482531, 0.001236790380387270492, 0.001747337335201052094, 0.002002610812607897358, 0.002130247551311319557, 0.002257884290014742189, 0.002385521028718164387, 0.002513157767421587020, 0.002768431244828421876, 0.003278978199642059495, 0.004300072109269333434, 0.005321166018896607806, 0.005831712973710208130, 0.006086986451116970995, 0.006342259928523734727, 0.006406078297875446477, 0.006469896667227158227, 0.006533715036578869977, 0.006597533405930581726, 0.006725170144634006961, 0.006852806883337431328, 0.007363353838151069815, 0.007618627315557889058, 0.007873900792964709169, 0.008129174270371528413, 0.008384447747778347657 ),
 .UNSPECIFIED. ) ;
#3746=CARTESIAN_POINT ( 'NONE',  ( 178.3810821012210113, 281.7766761570669587, -16.43735388118292917 ) ) ;
#3747=FACE_OUTER_BOUND ( 'NONE', #68337, .T. ) ;
#3749=CARTESIAN_POINT ( 'NONE',  ( 187.3225772020536795, 276.9076140642868609, 17.54334712858875989 ) ) ;
#3750=CARTESIAN_POINT ( 'NONE',  ( 171.7154418923348942, 259.3365693118849435, -15.26938553599716641 ) ) ;
#3752=CARTESIAN_POINT ( 'NONE',  ( 130.8844835975280887, 234.8262482093457493, 3.021315404115420679E-15 ) ) ;
#3753=CARTESIAN_POINT ( 'NONE',  ( 198.6303137791167330, 286.6091999416584599, -17.67087462607727488 ) ) ;
#3754=CARTESIAN_POINT ( 'NONE',  ( 190.0302884585784398, 301.5048807432094122, -1.372174654977964536 ) ) ;
#3758=CARTESIAN_POINT ( 'NONE',  ( 155.4341113147262945, 261.7935976400785876, 16.97053765338380771 ) ) ;
#3759=CARTESIAN_POINT ( 'NONE',  ( 38.03703169759612734, 192.7677522451418781, 10.00000000000009592 ) ) ;
#3760=CARTESIAN_POINT ( 'NONE',  ( 104.8563042601131770, 231.3458772461660544, 9.188101187500095079 ) ) ;
#3762=FACE_OUTER_BOUND ( 'NONE', #47597, .T. ) ;
#3764=CARTESIAN_POINT ( 'NONE',  ( 20.41882739113040302, 182.5958772461660544, -9.188101187500095079 ) ) ;
#3765=CARTESIAN_POINT ( 'NONE',  ( 170.8463542321686077, 287.4393069310528972, -8.645854640182026429 ) ) ;
#3768=CARTESIAN_POINT ( 'NONE',  ( 187.6513412634644169, 261.2126229280032135, -5.876874455337775416 ) ) ;
#3769=B_SPLINE_CURVE_WITH_KNOTS ( 'NONE', 3,
 ( #25085, #57480, #71723, #26107, #34689, #9400, #87480, #87967, #72733, #33714, #18511, #49897, #42279, #49397, #80344, #10912, #88463, #41787, #18015, #3323, #33196, #86459, #96047, #65094, #64097, #48907, #55473, #65590, #95043, #79842, #9914, #10408, #19024, #78814, #80855, #40275, #79348, #16984, #47875, #25606, #56493, #11427, #71216, #2825, #1807, #32691, #41278, #55966, #86961, #17496, #48401, #35693 ),
 .UNSPECIFIED., .F., .F.,
 ( 4, 2, 2, 2, 2, 2, 2, 2, 2, 2, 2, 2, 2, 2, 2, 2, 2, 2, 2, 2, 2, 2, 2, 2, 2, 4 ),
 ( 0.0001612845407840359966, 0.0006508920563406033269, 0.001140499571897170793, 0.001385303329675468620, 0.001507705208564656891, 0.001630107087453845595, 0.001752508966343033865, 0.001874910845232222135, 0.002119714603010437563, 0.002609322118566773877, 0.003098929634123110191, 0.004078144665235782819, 0.005057359696348456314, 0.005546967211904781786, 0.005791770969682908526, 0.005914172848572016132, 0.006036574727461122870, 0.006097775666905676240, 0.006158976606350230476, 0.006281378485239340684, 0.006526182243017528140, 0.006770986000795716463, 0.007015789758573903918, 0.007260593516352092242, 0.007505397274130279697, 0.007995004789686802060 ),
 .UNSPECIFIED. ) ;
#3772=CARTESIAN_POINT ( 'NONE',  ( 192.9739757011855659, 263.8060229890649566, -4.212473007787504997 ) ) ;
#3773=CYLINDRICAL_SURFACE ( 'NONE', #38163, 5.000000000000058620 ) ;
#3775=CARTESIAN_POINT ( 'NONE',  ( 167.6119263830523778, 251.7459577958838679, 10.36624589958357490 ) ) ;
#3776=CARTESIAN_POINT ( 'NONE',  ( 41.52819660837609916, 194.7833772461660544, -9.188101187500095079 ) ) ;
#3777=CARTESIAN_POINT ( 'NONE',  ( 87.83349241520130590, 231.5177522451419350, 5.000000000000046185 ) ) ;
#3778=ORIENTED_EDGE ( 'NONE', *, *, #15190, .F. ) ;
#3781=CARTESIAN_POINT ( 'NONE',  ( -7.604263460676718545, 177.9637435831425023, 2.679491924311251605 ) ) ;
#3782=CARTESIAN_POINT ( 'NONE',  ( 3.071516343397128423, 163.3923013555410080, 4.594050593750050204 ) ) ;
#3784=CARTESIAN_POINT ( 'NONE',  ( 150.9584389135710865, 269.1793093008492406, -15.82751450793727699 ) ) ;
#3786=CARTESIAN_POINT ( 'NONE',  ( 146.9700173529739970, 276.0874580858064746, -5.099093031535578469 ) ) ;
#3787=AXIS2_PLACEMENT_3D ( 'NONE', #20599, #28182, #12003 ) ;
#3789=CARTESIAN_POINT ( 'NONE',  ( 164.4761815919938215, 245.7658921781788592, 6.833796894895563412 ) ) ;
#3790=CARTESIAN_POINT ( 'NONE',  ( 147.2999496562918296, 275.5159985734018164, -0.1418322875769767455 ) ) ;
#3791=CARTESIAN_POINT ( 'NONE',  ( 207.1059763530604698, 271.9289217357780899, 6.370907250589925575 ) ) ;
#3792=ORIENTED_EDGE ( 'NONE', *, *, #7604, .F. ) ;
#3793=CARTESIAN_POINT ( 'NONE',  ( -4.668846022976095966, 168.1115022471902591, 10.00000000000009592 ) ) ;
#3796=CARTESIAN_POINT ( 'NONE',  ( 121.0403275412173656, 234.5643266524160140, 9.188101187500095079 ) ) ;
#3798=CARTESIAN_POINT ( 'NONE',  ( 193.5005633302724277, 262.8551920378705518, -5.236817587991198231 ) ) ;
#3801=CARTESIAN_POINT ( 'NONE',  ( 157.3025066944120454, 258.1910615777721887, 18.21299529665260053 ) ) ;
#3802=CARTESIAN_POINT ( 'NONE',  ( 149.3166057054752400, 247.0244633538772234, 5.014128649969458174 ) ) ;
#3803=CARTESIAN_POINT ( 'NONE',  ( 150.2762856237821438, 270.3608334573137881, -14.20317525964708061 ) ) ;
#3804=ORIENTED_EDGE ( 'NONE', *, *, #12922, .F. ) ;
#3805=CARTESIAN_POINT ( 'NONE',  ( 151.3560786774222322, 268.4905770267490652, 15.54402364351346932 ) ) ;
#3806=CARTESIAN_POINT ( 'NONE',  ( 207.9405038940993222, 270.4834776343830640, -0.2435786705607262403 ) ) ;
#3808=CARTESIAN_POINT ( 'NONE',  ( 180.6066648745947134, 283.7006809008031496, -16.18202752516933174 ) ) ;
#3811=CARTESIAN_POINT ( 'NONE',  ( 139.3620039403755015, 241.2677522451417929, -5.000000000000041744 ) ) ;
#3812=CARTESIAN_POINT ( 'NONE',  ( 165.3884017376936129, 269.6430054510781815, -16.30567925014516817 ) ) ;
#3815=CARTESIAN_POINT ( 'NONE',  ( 180.7877299985295565, 263.4844111323488960, 14.67210611338813919 ) ) ;
#3817=ORIENTED_EDGE ( 'NONE', *, *, #84109, .T. ) ;
#3820=CARTESIAN_POINT ( 'NONE',  ( 174.4355206875066813, 273.1373033844686802, -16.36721432446067936 ) ) ;
#3823=CARTESIAN_POINT ( 'NONE',  ( 148.3025927079438304, 273.7793698660844939, -8.046026357031887954 ) ) ;
#3824=CARTESIAN_POINT ( 'NONE',  ( 156.3384060043484567, 261.3563118228615849, -17.44929643486769777 ) ) ;
#3827=CARTESIAN_POINT ( 'NONE',  ( 184.9118810634971339, 291.9181506604203378, 12.13670245241820567 ) ) ;
#3828=EDGE_CURVE ( 'NONE', #759, #13192, #59173, .T. ) ;
#3833=CARTESIAN_POINT ( 'NONE',  ( 184.2569950528642551, 259.4484375049545406, -5.816461788221651830 ) ) ;
#3836=CARTESIAN_POINT ( 'NONE',  ( 175.1230978711317618, 258.7486093689314544, 12.66210094468590697 ) ) ;
#3837=ORIENTED_EDGE ( 'NONE', *, *, #61776, .T. ) ;
#3842=CARTESIAN_POINT ( 'NONE',  ( 154.8833801513861772, 262.3811116602312268, -17.49275566389638215 ) ) ;
#3846=CARTESIAN_POINT ( 'NONE',  ( 151.6442999004562751, 268.6057199523998520, 14.65032303984580686 ) ) ;
#3847=CARTESIAN_POINT ( 'NONE',  ( 159.3761195245467377, 275.4568327680622701, -12.53322028322178916 ) ) ;
#3848=CARTESIAN_POINT ( 'NONE',  ( 153.3859906278383676, 264.9746663937372091, -17.41799046551451013 ) ) ;
#3851=CARTESIAN_POINT ( 'NONE',  ( 157.6439063144099180, 281.5864387313514499, 2.957906020347658593 ) ) ;
#3852=CARTESIAN_POINT ( 'NONE',  ( 131.1886288721100300, 255.7369531367911293, -4.594050593750048428 ) ) ;
#3855=ORIENTED_EDGE ( 'NONE', *, *, #89326, .T. ) ;
#3858=CARTESIAN_POINT ( 'NONE',  ( 3.578749241215597010, 161.3262482093458061, 3.021315404115420679E-15 ) ) ;
#3859=CARTESIAN_POINT ( 'NONE',  ( -9.065681333110875428, 177.1199935810941213, 2.679491924311251605 ) ) ;
#3860=CARTESIAN_POINT ( 'NONE',  ( 170.8526566076953088, 288.1261369771856948, -5.563456055268631850 ) ) ;
#3861=CARTESIAN_POINT ( 'NONE',  ( 156.7700855017945401, 279.3500026499473279, 7.384081754847029444 ) ) ;
#3862=CARTESIAN_POINT ( 'NONE',  ( 120.7221038307704788, 252.0530062829862743, -4.648177544792955347E-16 ) ) ;
#3863=CARTESIAN_POINT ( 'NONE',  ( 173.7893683034945411, 252.1476285642659150, 6.872699842875177545 ) ) ;
#3864=AXIS2_PLACEMENT_3D ( 'NONE', #49789, #66483, #80752 ) ;
#3865=CARTESIAN_POINT ( 'NONE',  ( 168.1011763779767989, 253.1388740643201629, 11.70041143357935631 ) ) ;
#3873=CARTESIAN_POINT ( 'NONE',  ( 204.8003314451236463, 269.2376841632477635, -2.968733614000913068 ) ) ;
#3876=CARTESIAN_POINT ( 'NONE',  ( 202.5245888501533216, 279.8641176599742266, 15.60152447840272494 ) ) ;
#3877=CARTESIAN_POINT ( 'NONE',  ( 152.3249143222120381, 268.8125044657937792, -15.54600960379902297 ) ) ;
#3879=CARTESIAN_POINT ( 'NONE',  ( 203.3440828345331965, 270.0445236297473457, 6.009308755609846564 ) ) ;
#3882=EDGE_CURVE ( 'NONE', #44895, #75103, #68521, .T. ) ;
#3884=CARTESIAN_POINT ( 'NONE',  ( 119.5336306364421404, 246.4865022471903160, 10.00000000000009415 ) ) ;
#3886=CARTESIAN_POINT ( 'NONE',  ( 14.22133309352410002, 169.0177522451418213, 5.000000000000051514 ) ) ;
#3887=CARTESIAN_POINT ( 'NONE',  ( 149.0247308281161622, 274.5285899518638075, 9.115861392502811356 ) ) ;
#3888=DIRECTION ( 'NONE',  ( -0.8660254037844387076, -0.4999999999999998890, -0.000000000000000000 ) ) ;
#3890=CARTESIAN_POINT ( 'NONE',  ( 8.781437479894508513, 182.0024278399160949, 9.188101187500095079 ) ) ;
#3891=CARTESIAN_POINT ( 'NONE',  ( 106.3175485811169239, 238.3149278399160949, -9.188101187500095079 ) ) ;
#3892=CARTESIAN_POINT ( 'NONE',  ( 154.8786460229866577, 262.3893114111486398, -18.06164891362396929 ) ) ;
#3893=DIRECTION ( 'NONE',  ( -0.8660254037844387076, -0.4999999999999998890, -0.000000000000000000 ) ) ;
#3894=CARTESIAN_POINT ( 'NONE',  ( 180.7705417327010196, 254.9826106211711192, -2.480839038887178827 ) ) ;
#3898=CYLINDRICAL_SURFACE ( 'NONE', #59853, 10.00000000000010658 ) ;
#3899=CARTESIAN_POINT ( 'NONE',  ( 147.6508870500795467, 274.9081571770856272, -8.950912509993816712 ) ) ;
#3900=EDGE_CURVE ( 'NONE', #37554, #75967, #11186, .T. ) ;
#3903=CARTESIAN_POINT ( 'NONE',  ( 205.5958069356747728, 274.5446118947268701, -13.04136175932365305 ) ) ;
#3906=CARTESIAN_POINT ( 'NONE',  ( 172.6644317266046471, 263.3511091774913098, -15.41941820294944421 ) ) ;
#3907=CARTESIAN_POINT ( 'NONE',  ( 92.94880205384217220, 212.2202760586659736, -5.415160957724236172E-17 ) ) ;
#3908=CARTESIAN_POINT ( 'NONE',  ( 161.1150691641480535, 251.5875096731584506, -13.48836942566120101 ) ) ;
#3910=CARTESIAN_POINT ( 'NONE',  ( 163.2179886388746013, 258.2814482063444075, 16.13245504067606007 ) ) ;
#3911=CARTESIAN_POINT ( 'NONE',  ( 196.4994169513186364, 290.3000215130921902, 16.82935102260526961 ) ) ;
#3912=CARTESIAN_POINT ( 'NONE',  ( 199.6892316128565028, 284.7751004525801477, 18.03507624704203494 ) ) ;
#3913=CARTESIAN_POINT ( 'NONE',  ( 198.8570476668614049, 286.2164853282868080, -17.01721544293231858 ) ) ;
#3914=CARTESIAN_POINT ( 'NONE',  ( 176.7122878561889365, 270.1790051031098869, -16.88799780853275578 ) ) ;
#3916=CARTESIAN_POINT ( 'NONE',  ( 172.8210543149999978, 253.0650713199155177, -9.347212986753337560 ) ) ;
#3919=CARTESIAN_POINT ( 'NONE',  ( 72.92127039979698111, 225.1589784336661353, -6.496448406907676862E-16 ) ) ;
#3920=CARTESIAN_POINT ( 'NONE',  ( 173.1254351131793499, 289.7002511501680715, -0.9735186482341396941 ) ) ;
#3922=CARTESIAN_POINT ( 'NONE',  ( 191.2712410773971499, 288.8438557170641729, -16.41810066034774707 ) ) ;
#3925=CARTESIAN_POINT ( 'NONE',  ( 190.4756535880310651, 286.7931554109379135, 16.24365846582493589 ) ) ;
#3927=CARTESIAN_POINT ( 'NONE',  ( 126.5340026503663466, 243.8615022471902591, -10.00000000000009592 ) ) ;
#3928=CARTESIAN_POINT ( 'NONE',  ( 205.2660270307054304, 275.1158074454486382, -13.97598661256119179 ) ) ;
#3930=ORIENTED_EDGE ( 'NONE', *, *, #59767, .T. ) ;
#3931=CARTESIAN_POINT ( 'NONE',  ( 169.4751163247794921, 248.6553299212260413, -1.920092548325727844 ) ) ;
#3933=CARTESIAN_POINT ( 'NONE',  ( 163.1484656051875106, 248.0655637253488806, 9.714247672444804138 ) ) ;
#3934=CARTESIAN_POINT ( 'NONE',  ( 185.1491161497484370, 292.9437783688060222, -11.97406807593424993 ) ) ;
#3935=ORIENTED_EDGE ( 'NONE', *, *, #49800, .T. ) ;
#3938=EDGE_LOOP ( 'NONE', ( #39237, #94553, #45036, #75603 ) ) ;
#3939=CARTESIAN_POINT ( 'NONE',  ( 190.5002508066484097, 290.6439963610214363, 14.51933001755366881 ) ) ;
#3940=CARTESIAN_POINT ( 'NONE',  ( 158.7734878439422630, 255.6432474898095393, 16.04789767506137466 ) ) ;
#3941=CARTESIAN_POINT ( 'NONE',  ( 151.5948730924283723, 249.1423013555410080, -4.594050593750043987 ) ) ;
#3942=CARTESIAN_POINT ( 'NONE',  ( 153.9854481409094547, 263.9363755241191711, -17.91143416251955856 ) ) ;
#3943=CARTESIAN_POINT ( 'NONE',  ( 192.8645107159946122, 296.1983763133186471, -11.90925672746789310 ) ) ;
#3944=EDGE_CURVE ( 'NONE', #45874, #69600, #13297, .T. ) ;
#3948=DIRECTION ( 'NONE',  ( -0.8660254037844387076, -0.4999999999999998890, -0.000000000000000000 ) ) ;
#3949=CARTESIAN_POINT ( 'NONE',  ( -22.42236680055709641, 157.8615022471902591, 0.000000000000000000 ) ) ;
#3950=VERTEX_POINT ( 'NONE', #83590 ) ;
#3952=CARTESIAN_POINT ( 'NONE',  ( 198.2391837281077756, 286.3575794386269422, 17.25947343406376078 ) ) ;
#3954=CARTESIAN_POINT ( 'NONE',  ( 147.6512387128590262, 274.9075480792844246, -8.209968531507987777 ) ) ;
#3956=CARTESIAN_POINT ( 'NONE',  ( 201.3693897336875693, 274.8123126220266386, -14.20577604999000698 ) ) ;
#3959=CARTESIAN_POINT ( 'NONE',  ( 207.9353140363083128, 270.4924667317612830, -5.099483218880686231 ) ) ;
#3961=CARTESIAN_POINT ( 'NONE',  ( 169.8458979940169229, 267.4598849057458096, 17.28316019494766209 ) ) ;
#3962=CARTESIAN_POINT ( 'NONE',  ( 156.6812872898450735, 261.2670451491295012, 0.000000000000000000 ) ) ;
#3963=CARTESIAN_POINT ( 'NONE',  ( 100.4447270377624477, 237.9869531367911293, 4.594050593750046652 ) ) ;
#3964=ORIENTED_EDGE ( 'NONE', *, *, #16416, .T. ) ;
#3966=CARTESIAN_POINT ( 'NONE',  ( 166.5240211178292782, 278.8801525804102539, -13.25163146027725425 ) ) ;
#3971=CARTESIAN_POINT ( 'NONE',  ( 177.2663517457237106, 293.3853303008062312, -2.825851527699106303 ) ) ;
#3973=CARTESIAN_POINT ( 'NONE',  ( 161.9974668067621622, 270.5451527692481477, -16.99912248473486187 ) ) ;
#3974=CARTESIAN_POINT ( 'NONE',  ( 206.9436690247072193, 270.9240130450578476, -4.881398567238052877 ) ) ;
#3976=CARTESIAN_POINT ( 'NONE',  ( 87.34609280552280097, 230.4244531367911009, -4.594050593750046652 ) ) ;
#3978=VERTEX_POINT ( 'NONE', #15628 ) ;
#3982=CARTESIAN_POINT ( 'NONE',  ( 153.9627345078393716, 265.2571514742093655, 16.78486123779136463 ) ) ;
#3984=CARTESIAN_POINT ( 'NONE',  ( 122.2847184155099995, 253.6589784336661069, -6.496448406907675876E-16 ) ) ;
#3986=CARTESIAN_POINT ( 'NONE',  ( -8.728340106763567974, 165.7677522451418781, 10.00000000000009592 ) ) ;
#3989=CARTESIAN_POINT ( 'NONE',  ( 205.0302908362115772, 275.5241145114948154, 13.44798751587103425 ) ) ;
#3991=EDGE_CURVE ( 'NONE', #2782, #41802, #80977, .T. ) ;
#3992=CARTESIAN_POINT ( 'NONE',  ( 206.7680519836501958, 272.5142239127119979, -10.57935479673322021 ) ) ;
#3994=CARTESIAN_POINT ( 'NONE',  ( 168.5554356917367045, 285.0925123692317129, 10.08420881268239455 ) ) ;
#3997=CARTESIAN_POINT ( 'NONE',  ( 89.54518929453067244, 234.0530062829863027, -4.648177544792955347E-16 ) ) ;
#3999=EDGE_CURVE ( 'NONE', #5430, #2810, #90662, .T. ) ;
#4002=CARTESIAN_POINT ( 'NONE',  ( 167.6224482745345767, 249.9459711549417591, 7.039320684982598664 ) ) ;
#4004=CARTESIAN_POINT ( 'NONE',  ( 208.3829315663354862, 269.7171704273955015, -1.768817828503133072 ) ) ;
#4005=CARTESIAN_POINT ( 'NONE',  ( 202.7005662011214042, 279.5593159471158629, -16.25860390100328345 ) ) ;
#4008=ADVANCED_FACE ( 'NONE', ( #14653 ), #76462, .T. ) ;
#4009=CARTESIAN_POINT ( 'NONE',  ( 182.4036492637225138, 264.0684302237640395, 14.07752408005863920 ) ) ;
#4010=ADVANCED_FACE ( 'NONE', ( #38431 ), #68837, .T. ) ;
#4011=CARTESIAN_POINT ( 'NONE',  ( 79.17323837735700920, 206.5177522451417929, 5.000000000000051514 ) ) ;
#4018=CARTESIAN_POINT ( 'NONE',  ( 18.65997361151702449, 172.3923013555409796, 4.594050593750050204 ) ) ;
#4019=CYLINDRICAL_SURFACE ( 'NONE', #45230, 17.82106496071139645 ) ;
#4022=CARTESIAN_POINT ( 'NONE',  ( 183.8274263638271577, 281.3324037098167310, 17.41033114534894111 ) ) ;
#4024=CARTESIAN_POINT ( 'NONE',  ( 42.77328167419872074, 189.3768266524160424, 9.188101187500096856 ) ) ;
#4025=CARTESIAN_POINT ( 'NONE',  ( 200.6449165581618956, 283.1198055712825976, 18.35107460171532523 ) ) ;
#4026=CARTESIAN_POINT ( 'NONE',  ( 190.6954410837624607, 300.3528026016029457, -5.728531842148099962 ) ) ;
#4028=CARTESIAN_POINT ( 'NONE',  ( 178.5837403247565192, 291.6510475641956646, 6.049951385461257658 ) ) ;
#4029=CARTESIAN_POINT ( 'NONE',  ( 191.7934382699952494, 298.4510156884799699, -8.680100145728863126 ) ) ;
#4030=CARTESIAN_POINT ( 'NONE',  ( 178.9534601940523260, 278.3064132268250432, -16.87083665727369919 ) ) ;
#4032=CARTESIAN_POINT ( 'NONE',  ( 118.9147354758962081, 227.9155109091896065, 2.679491924311254714 ) ) ;
#4034=CARTESIAN_POINT ( 'NONE',  ( 192.3926678149021825, 295.4131196713046847, -13.42882169270698256 ) ) ;
#4035=CARTESIAN_POINT ( 'NONE',  ( 79.84079962965540744, 210.2365022471902023, -10.00000000000009059 ) ) ;
#4037=DIRECTION ( 'NONE',  ( -0.8660254037844387076, -0.4999999999999998890, -0.000000000000000000 ) ) ;
#4038=ORIENTED_EDGE ( 'NONE', *, *, #97659, .F. ) ;
#4039=CARTESIAN_POINT ( 'NONE',  ( 38.09089796528284211, 201.9869531367911293, 4.594050593750046652 ) ) ;
#4040=ORIENTED_EDGE ( 'NONE', *, *, #49837, .T. ) ;
#4041=CARTESIAN_POINT ( 'NONE',  ( 162.5350674691047459, 263.2285193240729768, 17.40336567648585131 ) ) ;
#4042=CARTESIAN_POINT ( 'NONE',  ( 147.4317198359019301, 275.2877659273946733, 3.797273160043843188 ) ) ;
#4046=CARTESIAN_POINT ( 'NONE',  ( 206.8968397926183229, 272.2911568841838061, 7.145103750817420440 ) ) ;
#4049=CARTESIAN_POINT ( 'NONE',  ( 186.1775172130778344, 263.6544597137042274, 10.94427764037104822 ) ) ;
#4051=CARTESIAN_POINT ( 'NONE',  ( 174.8699766508015330, 257.3397558657187574, 11.46886032790315646 ) ) ;
#4052=ORIENTED_EDGE ( 'NONE', *, *, #24922, .F. ) ;
#4055=CARTESIAN_POINT ( 'NONE',  ( 174.7032039963333716, 255.1089386847479830, 8.234442070018992865 ) ) ;
#4057=EDGE_LOOP ( 'NONE', ( #75868, #62612, #50767, #29149 ) ) ;
#4059=CARTESIAN_POINT ( 'NONE',  ( 150.8888667059421209, 269.2998118992572927, 15.79021133717968617 ) ) ;
#4060=LINE ( 'NONE', #19782, #90121 ) ;
#4064=CARTESIAN_POINT ( 'NONE',  ( 207.6357208050208101, 271.0113774299547913, -6.790259683043212036 ) ) ;
#4067=ORIENTED_EDGE ( 'NONE', *, *, #53027, .F. ) ;
#4069=FACE_OUTER_BOUND ( 'NONE', #8900, .T. ) ;
#4072=CARTESIAN_POINT ( 'NONE',  ( 198.1847055346428590, 286.9842163890704683, 16.95145238430053070 ) ) ;
#4073=AXIS2_PLACEMENT_3D ( 'NONE', #14389, #85321, #99499 ) ;
#4074=CARTESIAN_POINT ( 'NONE',  ( 107.0210206738092609, 244.8464784336661353, 1.353441290958777525E-15 ) ) ;
#4076=CARTESIAN_POINT ( 'NONE',  ( 27.07533481826667554, 197.9860189848785694, -2.679491924311252493 ) ) ;
#4077=CARTESIAN_POINT ( 'NONE',  ( 207.5583741822599393, 271.1453457103705205, 3.140867606700001424 ) ) ;
#4080=CARTESIAN_POINT ( 'NONE',  ( 160.0105735053945182, 253.5005522708592594, 16.10371386499367929 ) ) ;
#4081=CARTESIAN_POINT ( 'NONE',  ( 204.6785851723931557, 274.1332865905380913, -12.34137688749581407 ) ) ;
#4082=CARTESIAN_POINT ( 'NONE',  ( 81.01380268399661588, 208.3923013555409796, 4.594050593750050204 ) ) ;
#4083=EDGE_CURVE ( 'NONE', #72864, #14672, #77333, .T. ) ;
#4085=CARTESIAN_POINT ( 'NONE',  ( 151.1926529451685326, 268.7736386982768408, 14.30343427984827365 ) ) ;
#4086=CARTESIAN_POINT ( 'NONE',  ( 154.9683083969241011, 262.2340116239618055, 18.33261662430134109 ) ) ;
#4087=CARTESIAN_POINT ( 'NONE',  ( 175.4922833695144959, 278.4365452609995373, 15.47038347327790220 ) ) ;
#4088=ADVANCED_FACE ( 'NONE', ( #41813 ), #89005, .T. ) ;
#4091=CARTESIAN_POINT ( 'NONE',  ( 203.2187760522547819, 278.6617501559703101, -15.08675642319914978 ) ) ;
#4092=VERTEX_POINT ( 'NONE', #3352 ) ;
#4093=CARTESIAN_POINT ( 'NONE',  ( 148.4286446168608791, 273.5610415554491510, 8.864897967665541501 ) ) ;
#4094=CARTESIAN_POINT ( 'NONE',  ( 174.2665823609021913, 277.1739101417822440, -15.63194565161007610 ) ) ;
#4095=CARTESIAN_POINT ( 'NONE',  ( 207.7666684749232786, 270.7845694125510931, -6.630926507062123498 ) ) ;
#4097=CARTESIAN_POINT ( 'NONE',  ( 176.6128493493775693, 293.2828690831819927, -1.507349561191283493 ) ) ;
#4100=CARTESIAN_POINT ( 'NONE',  ( 165.0308887387863876, 244.8051112166122891, 1.948365933089477808 ) ) ;
#4102=CARTESIAN_POINT ( 'NONE',  ( 153.8480465357228013, 265.0660884932569843, -16.61306390558784685 ) ) ;
#4103=CARTESIAN_POINT ( 'NONE',  ( 163.7595992360150490, 247.0070492265414828, -6.976205010573520049 ) ) ;
#4104=CARTESIAN_POINT ( 'NONE',  ( 132.9753269110629503, 238.3923013555409796, 4.594050593750050204 ) ) ;
#4105=ORIENTED_EDGE ( 'NONE', *, *, #47542, .F. ) ;
#4109=CARTESIAN_POINT ( 'NONE',  ( 204.3276935076901850, 276.7410487817560920, 13.46217427333259309 ) ) ;
#4112=VERTEX_POINT ( 'NONE', #26629 ) ;
#4115=CARTESIAN_POINT ( 'NONE',  ( 167.5938299737844943, 249.2181452600659952, -5.555151102822903475 ) ) ;
#4116=CARTESIAN_POINT ( 'NONE',  ( 206.7182525013508041, 272.6004791462452204, -10.42767927275168205 ) ) ;
#4117=CARTESIAN_POINT ( 'NONE',  ( 143.4758849319492526, 244.4548013555409796, -4.594050593750042211 ) ) ;
#4118=CARTESIAN_POINT ( 'NONE',  ( 196.1506231955608257, 263.5440226259423753, 0.8792856859939570668 ) ) ;
#4119=CARTESIAN_POINT ( 'NONE',  ( 190.2510882691990730, 301.1224442529128851, -5.480893437181090455 ) ) ;
#4122=CARTESIAN_POINT ( 'NONE',  ( 179.0678258594554677, 253.8070992628930753, 2.501565655556938772 ) ) ;
#4123=EDGE_CURVE ( 'NONE', #78500, #61239, #2342, .T. ) ;
#4125=CARTESIAN_POINT ( 'NONE',  ( 172.7003033961413223, 290.5754134926764891, -4.014267798627228601 ) ) ;
#4127=CARTESIAN_POINT ( 'NONE',  ( 169.4354079512919213, 285.1812872968449710, -7.984367431210777966 ) ) ;
#4129=DIRECTION ( 'NONE',  ( 0.4999999999999992784, -0.8660254037844390407, 0.000000000000000000 ) ) ;
#4130=CARTESIAN_POINT ( 'NONE',  ( 193.5950831135630494, 288.5422439134695765, 16.06279111291604877 ) ) ;
#4131=CARTESIAN_POINT ( 'NONE',  ( 130.1965684169901181, 252.6427522451419634, -10.00000000000009415 ) ) ;
#4132=CARTESIAN_POINT ( 'NONE',  ( 175.9490061063565349, 285.5465045145652425, -11.89368724642156572 ) ) ;
#4133=EDGE_LOOP ( 'NONE', ( #89229, #65845, #74782, #84473 ) ) ;
#4134=ADVANCED_FACE ( 'NONE', ( #7270 ), #75697, .T. ) ;
#4135=CARTESIAN_POINT ( 'NONE',  ( 157.8562613713738472, 257.2319303423452652, 17.81420683562559404 ) ) ;
#4136=CARTESIAN_POINT ( 'NONE',  ( 189.8147415777049218, 301.8782188922952514, -0.5019643756309712934 ) ) ;
#4137=CARTESIAN_POINT ( 'NONE',  ( -12.32793173735119652, 169.8149278399161233, 9.188101187500093303 ) ) ;
#4138=CARTESIAN_POINT ( 'NONE',  ( 38.93012039702277605, 193.2833772461660544, -9.188101187500095079 ) ) ;
#4139=CARTESIAN_POINT ( 'NONE',  ( 178.6079043543401781, 259.1547383593973564, -10.33114907980992925 ) ) ;
#4142=CARTESIAN_POINT ( 'NONE',  ( 205.4103625296683617, 274.8658110279089897, -13.38953657917851814 ) ) ;
#4143=CARTESIAN_POINT ( 'NONE',  ( 192.4574196167241382, 292.2611441422025109, -14.34643084275922043 ) ) ;
#4144=CARTESIAN_POINT ( 'NONE',  ( 146.8358616138309571, 276.3198226421291679, 4.054088818585255716 ) ) ;
#4146=CARTESIAN_POINT ( 'NONE',  ( 170.5175754660751011, 258.1364974620091175, 13.85570805355783897 ) ) ;
#4148=CARTESIAN_POINT ( 'NONE',  ( 204.7242223814549504, 276.0542406257275161, -13.93608974681376189 ) ) ;
#4149=CARTESIAN_POINT ( 'NONE',  ( 193.1030321335636586, 294.1827325794992021, -14.54662778306917481 ) ) ;
#4150=CARTESIAN_POINT ( 'NONE',  ( 39.06543686813810012, 183.3615022471902023, 5.000000000000051514 ) ) ;
#4153=CARTESIAN_POINT ( 'NONE',  ( 0.9332558059805314832, 171.3458772461660544, 9.188101187500095079 ) ) ;
#4154=CARTESIAN_POINT ( 'NONE',  ( 168.2351335216934558, 286.3770512125953474, 4.694921679824968663 ) ) ;
#4156=EDGE_CURVE ( 'NONE', #61069, #28867, #25290, .T. ) ;
#4157=CARTESIAN_POINT ( 'NONE',  ( 192.8323852661406761, 296.6515067047851062, 11.86505947732313615 ) ) ;
#4159=CARTESIAN_POINT ( 'NONE',  ( -27.42236680055714260, 166.5217562850347406, 1.224646799147364892E-15 ) ) ;
#4160=CARTESIAN_POINT ( 'NONE',  ( 179.6127186018034649, 277.1388513108101961, 16.32392918091530376 ) ) ;
#4161=CARTESIAN_POINT ( 'NONE',  ( 193.7114073116034945, 295.1289958610702797, 14.86160832869823345 ) ) ;
#4163=CARTESIAN_POINT ( 'NONE',  ( 179.7546709676660726, 262.8207191251350423, -12.87104168322583497 ) ) ;
#4165=CARTESIAN_POINT ( 'NONE',  ( 115.6419768118483091, 249.1199935810940929, 2.679491924311251605 ) ) ;
#4168=CARTESIAN_POINT ( 'NONE',  ( 154.9455285025717615, 262.2734675583710100, 18.28470720339922551 ) ) ;
#4172=CARTESIAN_POINT ( 'NONE',  ( 159.5221561062548972, 254.3465160214695118, -16.91023001054109542 ) ) ;
#4174=DIRECTION ( 'NONE',  ( 0.4999999999999992784, -0.8660254037844390407, 0.000000000000000000 ) ) ;
#4175=CARTESIAN_POINT ( 'NONE',  ( 164.2723164851102808, 246.1189969011916503, -1.993789335506892302 ) ) ;
#4179=ORIENTED_EDGE ( 'NONE', *, *, #47907, .F. ) ;
#4182=CARTESIAN_POINT ( 'NONE',  ( 163.9149533033796047, 246.7379680887036670, 7.273005089308705706 ) ) ;
#4183=CARTESIAN_POINT ( 'NONE',  ( 192.1149248854976861, 297.8941845364767005, 12.26771790733441314 ) ) ;
#4185=CARTESIAN_POINT ( 'NONE',  ( 193.8212943487757514, 292.9386659295947197, 15.46346239154970625 ) ) ;
#4186=CARTESIAN_POINT ( 'NONE',  ( 167.0957737472305666, 246.8272050136007749, 1.963998143010642128 ) ) ;
#4188=CYLINDRICAL_SURFACE ( 'NONE', #60388, 17.82106496071139645 ) ;
#4189=CARTESIAN_POINT ( 'NONE',  ( 77.00817486789581778, 225.2677522451419350, -5.000000000000047962 ) ) ;
#4190=CARTESIAN_POINT ( 'NONE',  ( 149.5796913320911870, 271.5673701627850960, -12.80793412251569841 ) ) ;
#4192=ORIENTED_EDGE ( 'NONE', *, *, #38570, .F. ) ;
#4193=CARTESIAN_POINT ( 'NONE',  ( 203.0765383200355245, 267.8773628719704334, 2.545970250563589943 ) ) ;
#4194=CARTESIAN_POINT ( 'NONE',  ( 166.1815834339950015, 273.8822376155316078, -15.37734293452891876 ) ) ;
#4196=DIRECTION ( 'NONE',  ( -0.8660254037844387076, -0.4999999999999998890, -0.000000000000000000 ) ) ;
#4197=VERTEX_POINT ( 'NONE', #74748 ) ;
#4198=CARTESIAN_POINT ( 'NONE',  ( 148.9266665119372703, 272.6984423298952152, 12.06339424062075061 ) ) ;
#4199=CARTESIAN_POINT ( 'NONE',  ( 169.2748951493203151, 261.4352243401077658, -16.54128482989432314 ) ) ;
#4202=CARTESIAN_POINT ( 'NONE',  ( 159.2204200025353487, 268.0642290086452704, -16.29750726868432409 ) ) ;
#4204=ORIENTED_EDGE ( 'NONE', *, *, #68344, .F. ) ;
#4209=CARTESIAN_POINT ( 'NONE',  ( 194.0244658732981122, 294.5867625264709204, 13.70898399957177283 ) ) ;
#4211=CARTESIAN_POINT ( 'NONE',  ( 135.1220879045620507, 255.4865022471903160, 10.00000000000009415 ) ) ;
#4212=CARTESIAN_POINT ( 'NONE',  ( 193.7483724793648037, 294.3783421859641862, 13.84800572152474807 ) ) ;
#4213=CARTESIAN_POINT ( 'NONE',  ( 162.0489775477180387, 249.9699329032011406, -13.37069569336162012 ) ) ;
#4214=CARTESIAN_POINT ( 'NONE',  ( 166.2786698706664765, 279.3007919285489606, -14.16120680810289301 ) ) ;
#4215=CARTESIAN_POINT ( 'NONE',  ( 197.4070200448009587, 288.7280068420738530, -18.25155942860170910 ) ) ;
#4216=ORIENTED_EDGE ( 'NONE', *, *, #49738, .T. ) ;
#4219=CARTESIAN_POINT ( 'NONE',  ( 205.7867067512454184, 274.2139637150027056, 10.62737868262404106 ) ) ;
#4220=CARTESIAN_POINT ( 'NONE',  ( 160.0105735053945182, 253.5005522708592594, 16.10371386499367929 ) ) ;
#4222=CARTESIAN_POINT ( 'NONE',  ( 185.4126573565306444, 275.9338992703376903, 16.44638672139682711 ) ) ;
#4226=CARTESIAN_POINT ( 'NONE',  ( 199.2788941474133253, 285.4858257909769463, -18.43300471952202813 ) ) ;
#4227=CARTESIAN_POINT ( 'NONE',  ( 148.3870282890677288, 273.6331231496113787, -8.845975465985159047 ) ) ;
#4228=VERTEX_POINT ( 'NONE', #47787 ) ;
#4230=CARTESIAN_POINT ( 'NONE',  ( 205.6418006816680304, 274.0625766808819890, 10.49905374274900893 ) ) ;
#4232=CARTESIAN_POINT ( 'NONE',  ( 134.6192181478005523, 236.9824982072973967, 3.021315404115420679E-15 ) ) ;
#4233=CARTESIAN_POINT ( 'NONE',  ( 155.3480338107684986, 262.6013740870448601, 17.23779241981489463 ) ) ;
#4234=CARTESIAN_POINT ( 'NONE',  ( 39.26390101962412871, 180.1427522451417644, 1.119607411625061291E-15 ) ) ;
#4235=CARTESIAN_POINT ( 'NONE',  ( 98.52331994705697582, 233.8149278399160949, -9.188101187500095079 ) ) ;
#4236=CARTESIAN_POINT ( 'NONE',  ( 183.8352931141344300, 296.4858501351076825, -2.730139885982957093 ) ) ;
#4237=CARTESIAN_POINT ( 'NONE',  ( 167.2877005011474694, 283.1435899044605549, -11.30941513220499850 ) ) ;
#4239=CARTESIAN_POINT ( 'NONE',  ( 163.2189713653645242, 247.9434441664957944, 10.97120828841990914 ) ) ;
#4240=CARTESIAN_POINT ( 'NONE',  ( 23.01690360248371903, 184.0958772461660544, -9.188101187500095079 ) ) ;
#4241=CIRCLE ( 'NONE', #5903, 17.82106496071138935 ) ;
#4242=CARTESIAN_POINT ( 'NONE',  ( 173.9076247008792393, 277.9417859016587045, -16.84130823774900776 ) ) ;
#4243=ORIENTED_EDGE ( 'NONE', *, *, #90245, .T. ) ;
#4245=ORIENTED_EDGE ( 'NONE', *, *, #38649, .F. ) ;
#4247=CARTESIAN_POINT ( 'NONE',  ( 185.5580716964178407, 259.1746232884236747, -5.314944570831372950 ) ) ;
#4250=CARTESIAN_POINT ( 'NONE',  ( 190.3286155001717930, 300.9881631498979004, -5.624828231725103045 ) ) ;
#4252=CARTESIAN_POINT ( 'NONE',  ( 207.2683629543511756, 271.6476598918739001, -6.694388351944108528 ) ) ;
#4253=CARTESIAN_POINT ( 'NONE',  ( 182.4155610542803458, 284.2376793896972345, 14.93425214775039223 ) ) ;
#4255=CARTESIAN_POINT ( 'NONE',  ( 52.86797706100236383, 192.1423013555410080, -4.594050593750043987 ) ) ;
#4256=CARTESIAN_POINT ( 'NONE',  ( 92.09145065047481182, 230.6427522451419065, 10.00000000000009237 ) ) ;
#4257=ADVANCED_FACE ( 'NONE', ( #31587 ), #21784, .F. ) ;
#4260=CARTESIAN_POINT ( 'NONE',  ( -7.720288864461156919, 177.8967562850347122, -4.648177544792955347E-16 ) ) ;
#4262=CARTESIAN_POINT ( 'NONE',  ( -7.673045192009834814, 172.5024278399160664, -9.188101187500093303 ) ) ;
#4264=CARTESIAN_POINT ( 'NONE',  ( 176.9878821292914211, 283.3466992399841615, -15.40003107629192769 ) ) ;
#4265=VECTOR ( 'NONE', #17081, 1000.000000000000000 ) ;
#4266=CARTESIAN_POINT ( 'NONE',  ( 176.4425850253208523, 252.1586887174202616, -1.458368723655519394 ) ) ;
#4267=CARTESIAN_POINT ( 'NONE',  ( 193.0761489135300906, 296.2292956824684893, -11.99675185248219655 ) ) ;
#4269=CARTESIAN_POINT ( 'NONE',  ( 164.4272222519600746, 245.8506922426221593, 7.021336339662529902 ) ) ;
#4271=CARTESIAN_POINT ( 'NONE',  ( 164.3774690880109119, 245.9368672504194819, -2.805681983503304000 ) ) ;
#4273=CARTESIAN_POINT ( 'NONE',  ( -2.575951297163730835, 175.9865022471903160, 10.00000000000009237 ) ) ;
#4275=CARTESIAN_POINT ( 'NONE',  ( 120.0114017305758551, 252.3464784336661353, 1.353441290958777327E-15 ) ) ;
#4280=CARTESIAN_POINT ( 'NONE',  ( 186.1630411436486554, 296.9614825196608194, -7.488375694256206749 ) ) ;
#4284=CARTESIAN_POINT ( 'NONE',  ( 191.4044787581200069, 299.1247133251352466, 7.435199718141230818 ) ) ;
#4285=CARTESIAN_POINT ( 'NONE',  ( 163.8402264623212545, 246.8673987741056237, 8.938446005630277469 ) ) ;
#4287=CARTESIAN_POINT ( 'NONE',  ( 164.3036517873781008, 252.3706336020835579, 13.60069832213670082 ) ) ;
#4291=CARTESIAN_POINT ( 'NONE',  ( 168.9073988155618053, 271.9158883140793250, -17.00354098114102896 ) ) ;
#4294=CARTESIAN_POINT ( 'NONE',  ( 199.7995805052075866, 272.4254932667536764, 12.42849113847113252 ) ) ;
#4295=CARTESIAN_POINT ( 'NONE',  ( 185.5553639007409004, 297.2884567403993969, 5.667419552555970519 ) ) ;
#4297=DIRECTION ( 'NONE',  ( 0.4999999999999998890, -0.8660254037844385966, 0.000000000000000000 ) ) ;
#4298=EDGE_LOOP ( 'NONE', ( #14769, #3930, #20433, #36614 ) ) ;
#4301=DIRECTION ( 'NONE',  ( 0.4999999999999992784, -0.8660254037844390407, 0.000000000000000000 ) ) ;
#4304=CARTESIAN_POINT ( 'NONE',  ( 194.2389208611690492, 294.2153155915419802, -15.75132567904764791 ) ) ;
#4305=CARTESIAN_POINT ( 'NONE',  ( 156.3084473884123042, 262.1325509154355018, -16.95104440301710014 ) ) ;
#4306=ORIENTED_EDGE ( 'NONE', *, *, #98151, .T. ) ;
#4310=VECTOR ( 'NONE', #39859, 1000.000000000000000 ) ;
#4311=CARTESIAN_POINT ( 'NONE',  ( 188.5410240070633563, 293.7196559869043426, 13.01390607220156248 ) ) ;
#4313=CARTESIAN_POINT ( 'NONE',  ( 81.79837788435251866, 218.0333772461660544, 9.188101187500095079 ) ) ;
#4315=CIRCLE ( 'NONE', #28611, 17.82106496071138224 ) ;
#4318=CARTESIAN_POINT ( 'NONE',  ( 185.5169003523186859, 259.2275736936089743, -6.864738593364268837 ) ) ;
#4320=( BOUNDED_CURVE ( )  B_SPLINE_CURVE ( 2, ( #8637, #536, #56216, #31422, #15722, #62823, #93267, #40517, #39504 ),
 .UNSPECIFIED., .F., .T. ) 
 B_SPLINE_CURVE_WITH_KNOTS ( ( 3, 2, 2, 2, 3 ),
 ( 0.9314516129032257563, 0.9327956989247311315, 0.9354838709677418818, 0.9381720430107527431, 0.9395161290322581182 ),
 .UNSPECIFIED. ) 
 CURVE ( )  GEOMETRIC_REPRESENTATION_ITEM ( )  RATIONAL_B_SPLINE_CURVE ( ( 0.9330127018922194093, 0.9330127018922194093, 1.000000000000000000, 0.8660254037844387076, 1.000000000000000000, 0.8660254037844387076, 1.000000000000000000, 0.9330127018922194093, 0.9330127018922194093 ) ) 
 REPRESENTATION_ITEM ( '' )  );
#4323=CARTESIAN_POINT ( 'NONE',  ( -14.37785915960194494, 174.0530062829862743, 6.972266317189433612E-15 ) ) ;
#4325=VERTEX_POINT ( 'NONE', #65865 ) ;
#4331=CARTESIAN_POINT ( 'NONE',  ( 203.1044072055706806, 278.8598428092302584, -16.67109798570195878 ) ) ;
#4332=ORIENTED_EDGE ( 'NONE', *, *, #78318, .F. ) ;
#4333=CARTESIAN_POINT ( 'NONE',  ( 206.7834510497742713, 272.4875519477961348, -7.518391375580527836 ) ) ;
#4337=EDGE_CURVE ( 'NONE', #32549, #90499, #61991, .T. ) ;
#4339=ADVANCED_FACE ( 'NONE', ( #90218 ), #90724, .T. ) ;
#4341=CARTESIAN_POINT ( 'NONE',  ( 0.9603191016227148324, 181.3615022471903444, 5.000000000000046185 ) ) ;
#4342=CARTESIAN_POINT ( 'NONE',  ( 143.8274474304129171, 253.8458772461660260, 9.188101187500095079 ) ) ;
#4343=CARTESIAN_POINT ( 'NONE',  ( 167.9796227970851703, 267.0069495776506301, -16.94467948695188397 ) ) ;
#4347=CARTESIAN_POINT ( 'NONE',  ( 164.1398834480021378, 281.6669933700340493, 8.767707422804397410 ) ) ;
#4352=CARTESIAN_POINT ( 'NONE',  ( 202.7865629936218284, 279.4103651332174536, 17.10878160033216133 ) ) ;
#4353=CARTESIAN_POINT ( 'NONE',  ( 170.6105105942687032, 288.5462187197699109, -5.627715764860385050 ) ) ;
#4354=CARTESIAN_POINT ( 'NONE',  ( 153.3397897684428131, 276.8807737960509598, 7.109465309109985753 ) ) ;
#4355=LINE ( 'NONE', #81399, #90694 ) ;
#4356=CARTESIAN_POINT ( 'NONE',  ( 171.2776707721998264, 280.4287170469435750, 13.77496485982851304 ) ) ;
#4357=CARTESIAN_POINT ( 'NONE',  ( 168.0584336595957211, 252.9231910825713214, 11.85262793608598031 ) ) ;
#4363=CARTESIAN_POINT ( 'NONE',  ( 194.3518562708335651, 293.5167449611453208, -14.44919933576977122 ) ) ;
#4364=CARTESIAN_POINT ( 'NONE',  ( 201.0458349605253545, 267.5706676224597800, -2.392963673958802939 ) ) ;
#4368=CARTESIAN_POINT ( 'NONE',  ( 160.9155581428462085, 282.2930683307629920, -7.657675304491033508 ) ) ;
#4370=CARTESIAN_POINT ( 'NONE',  ( 203.2529752088261716, 269.9999405576584763, 6.016569300217926575 ) ) ;
#4372=VERTEX_POINT ( 'NONE', #74988 ) ;
#4374=CARTESIAN_POINT ( 'NONE',  ( 189.8703400361598312, 274.0992181554749436, -15.62282287125612434 ) ) ;
#4376=CARTESIAN_POINT ( 'NONE',  ( 171.6704389044023458, 289.7300494326029252, 2.700906889728273086 ) ) ;
#4377=CARTESIAN_POINT ( 'NONE',  ( 192.6797324865049745, 296.9159090750308110, 12.42053959885222625 ) ) ;
#4379=CARTESIAN_POINT ( 'NONE',  ( 52.82617185314417441, 189.7592609112379876, 2.679491924311254714 ) ) ;
#4380=CARTESIAN_POINT ( 'NONE',  ( -2.476892769303202790, 175.5024278399161233, -9.188101187500093303 ) ) ;
#4381=CARTESIAN_POINT ( 'NONE',  ( 116.0067284296028589, 225.5327760586659451, 1.948934522072303157E-15 ) ) ;
#4382=CARTESIAN_POINT ( 'NONE',  ( 40.79748767570693246, 194.3615022471902591, -10.00000000000009592 ) ) ;
#4383=CARTESIAN_POINT ( 'NONE',  ( 184.1809134956363607, 294.4725012015020411, -7.735934973952240945 ) ) ;
#4389=CARTESIAN_POINT ( 'NONE',  ( 160.8590558562208912, 281.7049668674798681, 5.440820967619280246 ) ) ;
#4390=CARTESIAN_POINT ( 'NONE',  ( 148.3874010092782498, 273.6324775792697892, -8.328854486678444857 ) ) ;
#4392=CARTESIAN_POINT ( 'NONE',  ( 85.03695205236203947, 213.2365022471901739, -10.00000000000009237 ) ) ;
#4393=CARTESIAN_POINT ( 'NONE',  ( 139.3620039403753879, 261.2677522451419350, -5.000000000000047962 ) ) ;
#4397=ADVANCED_FACE ( 'NONE', ( #34964 ), #82488, .F. ) ;
#4398=CARTESIAN_POINT ( 'NONE',  ( 71.75763553740291911, 221.4244531367911293, -4.594050593750046652 ) ) ;
#4399=CARTESIAN_POINT ( 'NONE',  ( 161.8935665241663457, 250.2391126920490194, -13.69501063978231770 ) ) ;
#4401=CARTESIAN_POINT ( 'NONE',  ( 163.2100640172580199, 258.2939446478983427, 16.33648908913500364 ) ) ;
#4402=CARTESIAN_POINT ( 'NONE',  ( 195.6974783896144174, 291.6890198465123945, 16.70600479393688431 ) ) ;
#4403=CARTESIAN_POINT ( 'NONE',  ( 199.6580449488688771, 284.8291173391253892, 17.61636456357554437 ) ) ;
#4405=CARTESIAN_POINT ( 'NONE',  ( 198.9225589249066957, 286.1030165008847916, -17.03502353404871883 ) ) ;
#4406=CARTESIAN_POINT ( 'NONE',  ( 203.7690284654797210, 275.7086850192775955, -13.99192714286714612 ) ) ;
#4408=CARTESIAN_POINT ( 'NONE',  ( 193.2140586456748679, 295.9904290195353269, -12.67640480829088823 ) ) ;
#4415=CARTESIAN_POINT ( 'NONE',  ( 188.3152126950631100, 286.0690311334317357, -16.15890536769158459 ) ) ;
#4418=CARTESIAN_POINT ( 'NONE',  ( 153.6596595523362794, 266.9882342533689439, 16.60685250298524807 ) ) ;
#4420=CARTESIAN_POINT ( 'NONE',  ( 141.3286032983506004, 245.7365022471902307, 10.00000000000009592 ) ) ;
#4421=CARTESIAN_POINT ( 'NONE',  ( 205.4029933437358295, 274.8785748323546159, -13.50815392427034922 ) ) ;
#4425=CARTESIAN_POINT ( 'NONE',  ( 165.6439160563409416, 246.9868693674390840, -1.864321359011917867 ) ) ;
#4427=CARTESIAN_POINT ( 'NONE',  ( 196.7817283509550919, 264.7241178856941701, -4.656590905670582536 ) ) ;
#4432=CARTESIAN_POINT ( 'NONE',  ( 189.3260947096056839, 290.0486036062610538, 14.38962922108246900 ) ) ;
#4434=CARTESIAN_POINT ( 'NONE',  ( 157.5367219092377695, 258.1941064437173168, -16.74304786559553904 ) ) ;
#4440=EDGE_CURVE ( 'NONE', #73330, #20729, #53097, .T. ) ;
#4443=ORIENTED_EDGE ( 'NONE', *, *, #72309, .F. ) ;
#4444=ORIENTED_EDGE ( 'NONE', *, *, #48746, .F. ) ;
#4447=CARTESIAN_POINT ( 'NONE',  ( 147.6508870500795467, 274.9081571770856272, -8.950912509993816712 ) ) ;
#4449=CARTESIAN_POINT ( 'NONE',  ( 155.2419697281468416, 261.7600162942170527, 18.58580762350309357 ) ) ;
#4450=CARTESIAN_POINT ( 'NONE',  ( 120.8381292345549127, 252.1199935810940929, 2.679491924311251605 ) ) ;
#4451=CARTESIAN_POINT ( 'NONE',  ( 187.3067335226663772, 291.4160526537789906, -14.11360718373232359 ) ) ;
#4452=ADVANCED_FACE ( 'NONE', ( #87134 ), #16184, .F. ) ;
#4453=DIRECTION ( 'NONE',  ( -0.8660254037844387076, -0.4999999999999998890, -0.000000000000000000 ) ) ;
#4454=EDGE_CURVE ( 'NONE', #50641, #2713, #84542, .T. ) ;
#4455=CARTESIAN_POINT ( 'NONE',  ( 190.1758200331204876, 279.2204749713225169, -17.78067544974210890 ) ) ;
#4457=CARTESIAN_POINT ( 'NONE',  ( 105.1271107466783121, 225.3768266524159856, 9.188101187500098632 ) ) ;
#4459=CARTESIAN_POINT ( 'NONE',  ( 150.6571681785161445, 269.7011255207979730, 15.24894850018880454 ) ) ;
#4462=CARTESIAN_POINT ( 'NONE',  ( 163.0336413175346877, 276.6660547541027881, -14.15222362243524046 ) ) ;
#4464=ORIENTED_EDGE ( 'NONE', *, *, #3944, .T. ) ;
#4467=ORIENTED_EDGE ( 'NONE', *, *, #75237, .F. ) ;
#4468=CARTESIAN_POINT ( 'NONE',  ( -22.42236680055709641, 157.8615022471902591, 0.000000000000000000 ) ) ;
#4470=B_SPLINE_SURFACE_WITH_KNOTS ( 'NONE', 3, 1, ( 
 ( #31610, #63526 ),
 ( #48336, #25019 ),
 ( #2755, #70623 ),
 ( #63027, #87420 ),
 ( #77750, #1234 ),
 ( #9855, #93470 ),
 ( #55403, #93971 ),
 ( #86388, #78745 ),
 ( #48847, #79282 ),
 ( #32117, #71658 ),
 ( #16920, #17948 ),
 ( #47809, #9333 ),
 ( #2249, #55899 ),
 ( #64030, #94972 ),
 ( #39201, #8333 ),
 ( #25536, #79779 ),
 ( #64536, #70113 ),
 ( #95495, #26046 ),
 ( #15922, #65034 ),
 ( #82277, #43709 ),
 ( #12338, #96976 ),
 ( #11847, #80788 ),
 ( #5228, #96472 ),
 ( #11362, #4220 ),
 ( #18951, #34623 ),
 ( #97936, #42216 ),
 ( #89389, #49830 ),
 ( #50815, #4739 ),
 ( #27040, #73153 ),
 ( #88903, #74651 ),
 ( #36106, #35623 ),
 ( #19464, #95981 ),
 ( #67011, #56917 ),
 ( #43203, #27544 ) ),
 .UNSPECIFIED., .T., .F., .F.,
 ( 4, 2, 2, 2, 2, 2, 2, 2, 2, 2, 2, 2, 2, 2, 2, 2, 4 ),
 ( 2, 2 ),
 ( 0.000000000000000000, 0.06250000000000000000, 0.1250000000000000000, 0.1875000000000000000, 0.2500000000000000000, 0.3125000000000000000, 0.3750000000000000000, 0.4375000000000000000, 0.5000000000000000000, 0.5625000000000000000, 0.6250000000000000000, 0.6875000000000000000, 0.7500000000000000000, 0.8125000000000000000, 0.8750000000000000000, 0.9375000000000000000, 1.000000000000000000 ),
 ( 0.000000000000000000, 1.000000000000000000 ),
 .UNSPECIFIED. ) ;
#4471=CARTESIAN_POINT ( 'NONE',  ( 157.7233946900069839, 257.4620621851055375, 16.86796251324260254 ) ) ;
#4472=CARTESIAN_POINT ( 'NONE',  ( 159.8188415394622268, 253.8326417772889840, -15.43862849427313222 ) ) ;
#4473=CARTESIAN_POINT ( 'NONE',  ( 208.3490404761574553, 269.7758715175073689, 2.423947743236856578 ) ) ;
#4475=AXIS2_PLACEMENT_3D ( 'NONE', #15081, #1904, #25186 ) ;
#4476=ORIENTED_EDGE ( 'NONE', *, *, #11776, .T. ) ;
#4477=CARTESIAN_POINT ( 'NONE',  ( 208.3699316049496133, 269.7396870210121733, -1.898463622294385811 ) ) ;
#4479=CARTESIAN_POINT ( 'NONE',  ( 195.1474640768281290, 265.6393084148356252, -8.887799905196541062 ) ) ;
#4480=CARTESIAN_POINT ( 'NONE',  ( 153.2151911666999808, 266.1153816512735943, 16.19125425417644948 ) ) ;
#4482=CARTESIAN_POINT ( 'NONE',  ( 130.8370663736463655, 246.3458772461660544, 9.188101187500095079 ) ) ;
#4485=ORIENTED_EDGE ( 'NONE', *, *, #23194, .T. ) ;
#4487=CARTESIAN_POINT ( 'NONE',  ( 204.7088172315186512, 276.0809231281156144, 13.09496711537969027 ) ) ;
#4490=CARTESIAN_POINT ( 'NONE',  ( 192.1705252917600433, 271.8754300319524191, 14.16870868845061082 ) ) ;
#4491=CARTESIAN_POINT ( 'NONE',  ( 159.5180972751518595, 279.0588588540967976, -11.03979334413982016 ) ) ;
#4493=CARTESIAN_POINT ( 'NONE',  ( 199.0946232933934539, 281.9005678297153850, -16.60409553737443034 ) ) ;
#4497=CARTESIAN_POINT ( 'NONE',  ( 206.3023480738090996, 271.3208467458289874, 7.632938913807082670 ) ) ;
#4498=CARTESIAN_POINT ( 'NONE',  ( 167.6421291605131785, 249.9379862031578625, 6.991320327740723428 ) ) ;
#4500=CARTESIAN_POINT ( 'NONE',  ( 178.4479030810299207, 292.4469683173247176, -5.630510813558092131 ) ) ;
#4503=ADVANCED_FACE ( 'NONE', ( #18671 ), #51037, .T. ) ;
#4507=CARTESIAN_POINT ( 'NONE',  ( 161.0794898748901858, 273.2957853699189172, -15.15413963670030739 ) ) ;
#4509=CARTESIAN_POINT ( 'NONE',  ( 17.19803509898326510, 189.9244531367911293, -4.594050593750046652 ) ) ;
#4513=EDGE_CURVE ( 'NONE', #99632, #46611, #92611, .T. ) ;
#4515=CARTESIAN_POINT ( 'NONE',  ( 194.2158379711820544, 277.1301694417633712, 17.09965426914677167 ) ) ;
#4517=CARTESIAN_POINT ( 'NONE',  ( 38.09089796528284211, 201.9869531367911293, 4.594050593750046652 ) ) ;
#4520=CARTESIAN_POINT ( 'NONE',  ( 174.2509005389064498, 289.3797888277572952, 7.946914131557713645 ) ) ;
#4521=CARTESIAN_POINT ( 'NONE',  ( 147.0670278774466908, 275.9194309285509235, 3.666898409139099257 ) ) ;
#4523=CARTESIAN_POINT ( 'NONE',  ( 199.8626824144776606, 267.9900519737070113, -6.523113416085821292 ) ) ;
#4524=CARTESIAN_POINT ( 'NONE',  ( 178.7159350970735261, 293.8993888918343487, 2.713728331163343555 ) ) ;
#4525=CARTESIAN_POINT ( 'NONE',  ( 179.1784693145256142, 278.4914505192345473, -17.09466235216729402 ) ) ;
#4526=CARTESIAN_POINT ( 'NONE',  ( 149.0358100033410267, 277.1350342654116048, 3.013846530473550445 ) ) ;
#4527=CARTESIAN_POINT ( 'NONE',  ( 167.0744888229918956, 257.9696763678884963, -15.40152651063776013 ) ) ;
#4528=EDGE_CURVE ( 'NONE', #89364, #31208, #95884, .T. ) ;
#4532=CARTESIAN_POINT ( 'NONE',  ( 104.4503548538632316, 221.1115022471901739, -5.000000000000041744 ) ) ;
#4534=CARTESIAN_POINT ( 'NONE',  ( 161.7453106966084704, 267.8664946259053181, -17.40444035468481943 ) ) ;
#4535=ORIENTED_EDGE ( 'NONE', *, *, #59772, .T. ) ;
#4536=CARTESIAN_POINT ( 'NONE',  ( 64.04520420253651025, 195.5327760586659736, 1.948934522072303157E-15 ) ) ;
#4539=CARTESIAN_POINT ( 'NONE',  ( 147.3984236761635884, 275.3454365677582700, 5.108566646342994844 ) ) ;
#4542=CARTESIAN_POINT ( 'NONE',  ( 171.1315556791619770, 286.9288989291006828, 8.543482685092364193 ) ) ;
#4543=CARTESIAN_POINT ( 'NONE',  ( 206.9059968923335475, 272.2752963222270068, 6.902135944297345560 ) ) ;
#4544=CARTESIAN_POINT ( 'NONE',  ( 193.1459436135753833, 292.3487159552965409, -15.56164613900618754 ) ) ;
#4546=CARTESIAN_POINT ( 'NONE',  ( 188.2179220736648233, 265.0898711547592370, 10.74980725069386978 ) ) ;
#4549=VERTEX_POINT ( 'NONE', #12567 ) ;
#4557=CARTESIAN_POINT ( 'NONE',  ( 182.4527117421103526, 284.0689693941391738, 15.01769654107919116 ) ) ;
#4558=CARTESIAN_POINT ( 'NONE',  ( 191.5694344253287511, 298.8390017285333897, 8.250976118904059575 ) ) ;
#4564=CARTESIAN_POINT ( 'NONE',  ( 161.2977680094314223, 251.2710659906439616, -13.03191437619249982 ) ) ;
#4566=CARTESIAN_POINT ( 'NONE',  ( 196.2421909983451940, 290.7455499326673021, -17.31908925000307065 ) ) ;
#4569=CYLINDRICAL_SURFACE ( 'NONE', #75553, 17.82106496071139645 ) ;
#4574=CARTESIAN_POINT ( 'NONE',  ( 118.4422513298640638, 233.0643266524159856, 9.188101187500095079 ) ) ;
#4575=EDGE_CURVE ( 'NONE', #32378, #29964, #82228, .T. ) ;
#4576=CARTESIAN_POINT ( 'NONE',  ( 150.8359915840788688, 269.3913942967808453, 15.73449616766854575 ) ) ;
#4577=CARTESIAN_POINT ( 'NONE',  ( 109.1413257910288479, 240.4865022471902876, 10.00000000000009415 ) ) ;
#4578=ORIENTED_EDGE ( 'NONE', *, *, #23692, .T. ) ;
#4580=CARTESIAN_POINT ( 'NONE',  ( 163.7323023463233937, 247.0543288263758086, -6.244751637846886361 ) ) ;
#4581=VERTEX_POINT ( 'NONE', #77342 ) ;
#4582=ORIENTED_EDGE ( 'NONE', *, *, #93275, .T. ) ;
#4586=EDGE_CURVE ( 'NONE', #6702, #28883, #37482, .T. ) ;
#4587=CARTESIAN_POINT ( 'NONE',  ( 74.78872445064843077, 223.1744531367911293, 4.594050593750047540 ) ) ;
#4590=CARTESIAN_POINT ( 'NONE',  ( 150.4572752258758612, 270.0473502708459250, 15.21885120838634187 ) ) ;
#4591=CARTESIAN_POINT ( 'NONE',  ( 171.8543870755469243, 276.6897476962967630, 16.27073464812542980 ) ) ;
#4595=CARTESIAN_POINT ( 'NONE',  ( 155.6048174803203210, 261.1315455520403361, -17.38645169541727498 ) ) ;
#4598=CARTESIAN_POINT ( 'NONE',  ( 195.4228050201512303, 292.1647680779090024, 16.44344289977338391 ) ) ;
#4600=CARTESIAN_POINT ( 'NONE',  ( 207.6357208050208101, 271.0113774299547913, -6.790259683043212036 ) ) ;
#4601=CARTESIAN_POINT ( 'NONE',  ( 206.5523081671381931, 270.6640731400667050, 2.446578107278855274 ) ) ;
#4603=CARTESIAN_POINT ( 'NONE',  ( 200.1505510372172694, 283.2820884176684899, -16.95936656477399396 ) ) ;
#4604=B_SPLINE_CURVE_WITH_KNOTS ( 'NONE', 3,
 ( #79775, #25532, #3255, #2246 ),
 .UNSPECIFIED., .F., .F.,
 ( 4, 4 ),
 ( 0.03120710976339495860, 0.04024459120465366524 ),
 .UNSPECIFIED. ) ;
#4606=CARTESIAN_POINT ( 'NONE',  ( 156.2224770818481545, 267.4677849582849376, -16.91854127892884208 ) ) ;
#4607=CARTESIAN_POINT ( 'NONE',  ( 164.5259176133158689, 246.1953198488120051, 1.882264443804981813 ) ) ;
#4609=CARTESIAN_POINT ( 'NONE',  ( 164.4989226152910646, 245.7265035704120351, -6.575810094723514965 ) ) ;
#4611=CARTESIAN_POINT ( 'NONE',  ( 118.9560200436548314, 248.6744531367911293, 4.594050593750047540 ) ) ;
#4614=CARTESIAN_POINT ( 'NONE',  ( 183.7243390097106328, 259.3199907679909870, 6.356928255902579039 ) ) ;
#4615=CARTESIAN_POINT ( 'NONE',  ( 203.3041373168503299, 278.5139001086923827, -16.61929732091214973 ) ) ;
#4616=CARTESIAN_POINT ( 'NONE',  ( 204.9608076533459950, 275.6444629144898499, 14.31488288944633069 ) ) ;
#4618=CYLINDRICAL_SURFACE ( 'NONE', #72911, 17.82106496071139645 ) ;
#4619=VERTEX_POINT ( 'NONE', #53035 ) ;
#4623=CARTESIAN_POINT ( 'NONE',  ( 182.4292202362132116, 275.0433250554996221, -17.33419130812088582 ) ) ;
#4624=CARTESIAN_POINT ( 'NONE',  ( 167.5904688695373750, 249.2039005190006549, -5.515356433798250357 ) ) ;
#4626=CARTESIAN_POINT ( 'NONE',  ( 198.5413888763568195, 266.2629941491867953, 0.8512800372524856884 ) ) ;
#4627=CARTESIAN_POINT ( 'NONE',  ( 190.6954410837624607, 300.3528026016029457, -5.728531842148099962 ) ) ;
#4629=CARTESIAN_POINT ( 'NONE',  ( 157.2104826425669728, 258.3504519110855995, -16.92635148710569482 ) ) ;
#4630=CARTESIAN_POINT ( 'NONE',  ( 170.7941491505363842, 250.2313031156421914, 4.188098645002056308 ) ) ;
#4631=B_SPLINE_CURVE_WITH_KNOTS ( 'NONE', 3,
 ( #53069, #84024, #7983, #1385, #8969, #47953, #2390, #38859, #25163, #87552, #70260, #55548, #9986, #62148, #71289, #78896, #79420, #373, #17571, #33270, #94608, #32763, #40846, #77889, #93604, #48478 ),
 .UNSPECIFIED., .F., .F.,
 ( 4, 2, 2, 2, 2, 2, 2, 2, 2, 2, 2, 2, 4 ),
 ( 0.0003107992373423731349, 0.002113324222800152651, 0.002338639845982365319, 0.002451297657573469919, 0.002563955469164574084, 0.002592119922062337441, 0.002620284374960100797, 0.002676613280755630545, 0.002789271092346726905, 0.003014586715528822913, 0.003465217961892969826, 0.003690533585075043716, 0.003915849208257117173 ),
 .UNSPECIFIED. ) ;
#4633=CARTESIAN_POINT ( 'NONE',  ( 190.3572031550745294, 300.9386478791372497, 3.093832330100951378 ) ) ;
#4636=CARTESIAN_POINT ( 'NONE',  ( 155.0453531195792038, 262.1005662498678817, -18.46987289964740953 ) ) ;
#4637=CARTESIAN_POINT ( 'NONE',  ( 194.9146483705927153, 289.3315033412051207, 16.17650949137597749 ) ) ;
#4638=B_SPLINE_CURVE_WITH_KNOTS ( 'NONE', 3,
 ( #14535, #70204, #31693, #37806, #100142, #84957, #14031, #75855, #6437, #61607, #53996, #68215, #29727, #60601, #57007, #16515 ),
 .UNSPECIFIED., .F., .F.,
 ( 4, 2, 2, 2, 2, 2, 2, 4 ),
 ( 3.925231146709437917E-17, 0.0003558565760979790437, 0.0007117131521959188393, 0.001067569728293858581, 0.001423426304391798430, 0.001779282880489738280, 0.002135139456587678130, 0.002846852608783629387 ),
 .UNSPECIFIED. ) ;
#4639=CARTESIAN_POINT ( 'NONE',  ( 133.7328388157766312, 238.0177522451417929, 5.000000000000051514 ) ) ;
#4640=CARTESIAN_POINT ( 'NONE',  ( 172.6748435171904532, 283.7256293223668422, -12.33524359727445763 ) ) ;
#4644=CARTESIAN_POINT ( 'NONE',  ( 198.7829547491859330, 286.3448180261817129, -18.59838968157616179 ) ) ;
#4645=CARTESIAN_POINT ( 'NONE',  ( -14.92600794870450898, 168.3149278399161233, 9.188101187500093303 ) ) ;
#4647=CARTESIAN_POINT ( 'NONE',  ( 45.77687342386973057, 206.4244531367911293, -4.594050593750046652 ) ) ;
#4648=CARTESIAN_POINT ( 'NONE',  ( 178.6152369244925637, 259.3283413532399777, -10.64205949810462926 ) ) ;
#4651=CARTESIAN_POINT ( 'NONE',  ( 204.6470611188870521, 276.1878878528713130, -13.02652554726987866 ) ) ;
#4652=CARTESIAN_POINT ( 'NONE',  ( 192.6054495295585696, 292.3993297283804509, -14.32894417406807364 ) ) ;
#4653=CARTESIAN_POINT ( 'NONE',  ( 150.0179852530401092, 276.4561033902535883, 3.706981700497388843 ) ) ;
#4654=CARTESIAN_POINT ( 'NONE',  ( 74.91528014208350328, 207.3927522451418213, 10.00000000000009948 ) ) ;
#4655=CARTESIAN_POINT ( 'NONE',  ( 76.57516216600367898, 205.0177522451417929, 5.000000000000051514 ) ) ;
#4656=CARTESIAN_POINT ( 'NONE',  ( 179.0862785926605341, 254.3646952837514448, -4.132455289343337945 ) ) ;
#4657=ADVANCED_FACE ( 'NONE', ( #85487 ), #14528, .F. ) ;
#4658=CARTESIAN_POINT ( 'NONE',  ( 157.1965120183049578, 258.3746497421212780, -18.06591467563559306 ) ) ;
#4659=CARTESIAN_POINT ( 'NONE',  ( 198.1444248750829047, 287.4507842102791528, 18.42558436659502519 ) ) ;
#4660=EDGE_CURVE ( 'NONE', #76868, #60705, #9517, .T. ) ;
#4661=CARTESIAN_POINT ( 'NONE',  ( 36.39519187313601378, 198.4865022471902876, 10.00000000000009237 ) ) ;
#4662=CARTESIAN_POINT ( 'NONE',  ( 181.7016834730597736, 291.7820365442338471, 9.111168900057094788 ) ) ;
#4663=FACE_OUTER_BOUND ( 'NONE', #68106, .T. ) ;
#4665=CARTESIAN_POINT ( 'NONE',  ( -1.313257906909115480, 179.2369531367911293, -4.594050593750048428 ) ) ;
#4669=CARTESIAN_POINT ( 'NONE',  ( 79.76863084600667264, 216.8615022471902591, -10.00000000000009592 ) ) ;
#4671=CARTESIAN_POINT ( 'NONE',  ( 164.3706594650489023, 245.9486618633701482, -1.665857659249071698 ) ) ;
#4673=CARTESIAN_POINT ( 'NONE',  ( 153.5916109235682541, 265.1562792198043326, -16.36868264138671591 ) ) ;
#4674=CARTESIAN_POINT ( 'NONE',  ( 176.4634627281214421, 260.3851565349380053, -13.39184936855075136 ) ) ;
#4681=CARTESIAN_POINT ( 'NONE',  ( 193.7706395672514645, 295.0264025848412075, 15.16938698680137065 ) ) ;
#4683=CIRCLE ( 'NONE', #98485, 17.82106496071138224 ) ;
#4684=CARTESIAN_POINT ( 'NONE',  ( 156.7410793263471760, 276.7253777054597208, 11.42669515405709646 ) ) ;
#4687=CARTESIAN_POINT ( 'NONE',  ( 168.0561721676931199, 250.9850586709442837, -10.23605044211346105 ) ) ;
#4689=CARTESIAN_POINT ( 'NONE',  ( 192.7259387352017939, 296.8358775046606297, 11.24705370801146209 ) ) ;
#4692=CARTESIAN_POINT ( 'NONE',  ( 155.2922060645262263, 261.6730044072216401, -16.98884022075611355 ) ) ;
#4697=CARTESIAN_POINT ( 'NONE',  ( 159.7794170132337683, 278.5358178951433956, -9.739126798237956351 ) ) ;
#4699=CARTESIAN_POINT ( 'NONE',  ( 192.7944000592152634, 296.7172990131160759, 11.44860011299869740 ) ) ;
#4701=CARTESIAN_POINT ( 'NONE',  ( 191.5281967176683509, 298.9104275333885994, 7.715154960566919407 ) ) ;
#4704=VERTEX_POINT ( 'NONE', #35735 ) ;
#4708=EDGE_CURVE ( 'NONE', #79972, #88994, #85629, .T. ) ;
#4711=ORIENTED_EDGE ( 'NONE', *, *, #58928, .F. ) ;
#4712=CARTESIAN_POINT ( 'NONE',  ( 177.5778721735796069, 268.8026387624398694, 16.30278465327989323 ) ) ;
#4713=CARTESIAN_POINT ( 'NONE',  ( 205.8030308266901898, 274.1856895869457844, 10.55961490432110317 ) ) ;
#4716=B_SPLINE_SURFACE_WITH_KNOTS ( 'NONE', 3, 1, ( 
 ( #71471, #2064 ),
 ( #63848, #94787 ),
 ( #87729, #80097 ),
 ( #10663, #88213 ),
 ( #41539, #33977 ),
 ( #95808, #26362 ),
 ( #49642, #80600 ),
 ( #56905, #49326 ),
 ( #42204, #87891 ),
 ( #64525, #95969 ),
 ( #25524, #65512 ),
 ( #57405, #10333 ),
 ( #58402, #73624 ),
 ( #4209, #96461 ),
 ( #56412, #41708 ),
 ( #41199, #81261 ),
 ( #48835, #73139 ),
 ( #3734, #18436 ),
 ( #72652, #80265 ),
 ( #35106, #10828 ),
 ( #79768, #88386 ),
 ( #72137, #2742 ),
 ( #87407, #34612 ),
 ( #27027, #94959 ),
 ( #88890, #34130 ),
 ( #57911, #96965 ),
 ( #19452, #17937 ),
 ( #33631, #95482 ),
 ( #26034, #18940 ),
 ( #64019, #3247 ),
 ( #66016, #49817 ),
 ( #65023, #26532 ),
 ( #27531, #80776 ),
 ( #19930, #11348 ) ),
 .UNSPECIFIED., .T., .F., .F.,
 ( 4, 2, 2, 2, 2, 2, 2, 2, 2, 2, 2, 2, 2, 2, 2, 2, 4 ),
 ( 2, 2 ),
 ( 0.000000000000000000, 0.06250000000000000000, 0.1250000000000000000, 0.1875000000000000000, 0.2500000000000000000, 0.3125000000000000000, 0.3750000000000000000, 0.4375000000000000000, 0.5000000000000000000, 0.5625000000000000000, 0.6250000000000000000, 0.6875000000000000000, 0.7500000000000000000, 0.8125000000000000000, 0.8750000000000000000, 0.9375000000000000000, 1.000000000000000000 ),
 ( 0.000000000000000000, 1.000000000000000000 ),
 .UNSPECIFIED. ) ;
#4719=CARTESIAN_POINT ( 'NONE',  ( 190.0607312434325138, 301.4521522931182176, 3.538147641957853473 ) ) ;
#4720=DIRECTION ( 'NONE',  ( -0.8660254037844387076, -0.4999999999999998890, -0.000000000000000000 ) ) ;
#4721=EDGE_CURVE ( 'NONE', #84236, #56021, #54148, .T. ) ;
#4724=ORIENTED_EDGE ( 'NONE', *, *, #56609, .F. ) ;
#4725=CARTESIAN_POINT ( 'NONE',  ( 157.2786326963988586, 269.2986199873796522, 15.63648806844084405 ) ) ;
#4728=CARTESIAN_POINT ( 'NONE',  ( 190.3286155001717930, 300.9881631498979004, -5.624828231725103045 ) ) ;
#4731=CARTESIAN_POINT ( 'NONE',  ( 153.0070714074088016, 265.6309737354857248, 17.74442213480098474 ) ) ;
#4733=CARTESIAN_POINT ( 'NONE',  ( 197.4537186060251486, 288.6471225613934166, -18.22696722856148455 ) ) ;
#4734=VERTEX_POINT ( 'NONE', #13267 ) ;
#4735=B_SPLINE_CURVE_WITH_KNOTS ( 'NONE', 3,
 ( #99023, #98026, #82858, #67602 ),
 .UNSPECIFIED., .F., .F.,
 ( 4, 4 ),
 ( 0.003963300069783955853, 0.01194164548429975728 ),
 .UNSPECIFIED. ) ;
#4736=CARTESIAN_POINT ( 'NONE',  ( 164.9617201910520237, 244.9249146555742414, 2.745022583679548767 ) ) ;
#4737=CARTESIAN_POINT ( 'NONE',  ( 196.6800254274587019, 289.9871984561398222, -17.90749311895638129 ) ) ;
#4739=CARTESIAN_POINT ( 'NONE',  ( 159.8416255366773839, 253.7931787365127434, 16.77980437810719394 ) ) ;
#4743=CARTESIAN_POINT ( 'NONE',  ( 186.9332467140213794, 276.6677885244452000, 17.67048876257000600 ) ) ;
#4744=CARTESIAN_POINT ( 'NONE',  ( 200.5039526449628795, 267.3497397166782434, 6.370409075474873006 ) ) ;
#4745=CARTESIAN_POINT ( 'NONE',  ( 164.0532584536765626, 247.8859213503266972, 8.571009476567882146 ) ) ;
#4747=CARTESIAN_POINT ( 'NONE',  ( 199.3272761551183692, 285.4020256954596562, -18.33026947811089258 ) ) ;
#4748=CARTESIAN_POINT ( 'NONE',  ( 148.0167748296930199, 274.2744209529264481, -10.15233092020212347 ) ) ;
#4750=CARTESIAN_POINT ( 'NONE',  ( 170.3593749743948536, 255.4184166931929951, -11.62125758648799057 ) ) ;
#4751=CARTESIAN_POINT ( 'NONE',  ( 183.3634088509504352, 284.6525016221286251, -16.42631288611494256 ) ) ;
#4752=CARTESIAN_POINT ( 'NONE',  ( 125.8664413980679342, 250.1427522451419350, 10.00000000000009415 ) ) ;
#4753=CARTESIAN_POINT ( 'NONE',  ( 207.6209998424140792, 271.0368748851258260, 6.610167240481342965 ) ) ;
#4755=CARTESIAN_POINT ( 'NONE',  ( 38.54221318313706490, 186.3927522451418213, 10.00000000000009592 ) ) ;
#4756=CARTESIAN_POINT ( 'NONE',  ( 94.19319292813476352, 231.3149278399160949, 9.188101187500093303 ) ) ;
#4757=CARTESIAN_POINT ( 'NONE',  ( 182.4111744044705006, 295.1865784113461473, -2.664051097989806660 ) ) ;
#4758=CIRCLE ( 'NONE', #61336, 17.82106496071138935 ) ;
#4759=CARTESIAN_POINT ( 'NONE',  ( 167.6233549396688147, 282.5614550147377031, -10.64682312388593211 ) ) ;
#4760=CARTESIAN_POINT ( 'NONE',  ( 195.8627871995700502, 291.4026965887302936, 17.41145040657729481 ) ) ;
#4761=CARTESIAN_POINT ( 'NONE',  ( 163.1968603775171118, 247.9817415208531202, 11.27455733958931994 ) ) ;
#4762=CARTESIAN_POINT ( 'NONE',  ( 13.65283037618196893, 184.8149278399160664, 9.188101187500093303 ) ) ;
#4764=VERTEX_POINT ( 'NONE', #97866 ) ;
#4766=VERTEX_POINT ( 'NONE', #96396 ) ;
#4767=DIRECTION ( 'NONE',  ( -0.8660254037844387076, -0.4999999999999998890, -0.000000000000000000 ) ) ;
#4768=CARTESIAN_POINT ( 'NONE',  ( 185.1461160444276004, 259.9246127725722886, -5.696222747182419610 ) ) ;
#4770=FACE_OUTER_BOUND ( 'NONE', #56164, .T. ) ;
#4774=CARTESIAN_POINT ( 'NONE',  ( 168.1671718393196500, 251.7577310522514153, 10.56854090917195421 ) ) ;
#4775=CARTESIAN_POINT ( 'NONE',  ( 49.48463145776311478, 205.5024278399160949, -9.188101187500093303 ) ) ;
#4776=CARTESIAN_POINT ( 'NONE',  ( 90.50373741020339935, 216.3927522451417929, 10.00000000000009592 ) ) ;
#4781=CARTESIAN_POINT ( 'NONE',  ( 162.6257765080958677, 248.9708877980734485, -10.42859054881151160 ) ) ;
#4783=CARTESIAN_POINT ( 'NONE',  ( -0.9884983804899494242, 179.4244531367911577, -4.594050593750046652 ) ) ;
#4784=CARTESIAN_POINT ( 'NONE',  ( 150.7691137448031213, 269.5072301123068428, -15.63821625702598084 ) ) ;
#4786=CARTESIAN_POINT ( 'NONE',  ( 147.1125781744767949, 275.8405354997948962, -5.216646253929903665 ) ) ;
#4788=CARTESIAN_POINT ( 'NONE',  ( 51.40603854846860798, 209.6744531367911293, 4.594050593750047540 ) ) ;
#4789=CARTESIAN_POINT ( 'NONE',  ( 208.0692320075777957, 270.2605140014760536, 2.043861372130216569 ) ) ;
#4791=EDGE_CURVE ( 'NONE', #44920, #79399, #51857, .T. ) ;
#4795=EDGE_CURVE ( 'NONE', #45744, #75611, #74883, .T. ) ;
#4796=CARTESIAN_POINT ( 'NONE',  ( 3.125382611083852957, 172.6115022471902591, 10.00000000000009592 ) ) ;
#4798=CARTESIAN_POINT ( 'NONE',  ( 125.9656734773588767, 243.5333772461660544, 9.188101187500095079 ) ) ;
#4800=CARTESIAN_POINT ( 'NONE',  ( 164.6112646021906869, 245.5319215412782796, 0.9047594026039291748 ) ) ;
#4804=CARTESIAN_POINT ( 'NONE',  ( 189.3785535910650424, 289.8996385724929041, 14.46956945346604861 ) ) ;
#4806=ORIENTED_EDGE ( 'NONE', *, *, #51075, .F. ) ;
#4808=CARTESIAN_POINT ( 'NONE',  ( 151.0715479399129606, 268.9833987204304435, 14.24612252017116987 ) ) ;
#4809=CARTESIAN_POINT ( 'NONE',  ( 208.4115645851568388, 269.6675765840226973, -1.114383557117654133 ) ) ;
#4810=CARTESIAN_POINT ( 'NONE',  ( 151.3433504153738909, 269.1997824268871113, -14.27012659247592730 ) ) ;
#4811=CARTESIAN_POINT ( 'NONE',  ( 172.7592676337296211, 268.7804561342234138, -17.20143128700372159 ) ) ;
#4817=CARTESIAN_POINT ( 'NONE',  ( 182.2606358067372412, 295.0231671335754982, 4.761058120652655212 ) ) ;
#4819=CARTESIAN_POINT ( 'NONE',  ( 148.6181070846184866, 274.7356907660122260, -7.901608801242418600 ) ) ;
#4822=FACE_OUTER_BOUND ( 'NONE', #53550, .T. ) ;
#4824=CYLINDRICAL_SURFACE ( 'NONE', #62737, 10.00000000000010658 ) ;
#4825=ORIENTED_EDGE ( 'NONE', *, *, #6143, .F. ) ;
#4828=CARTESIAN_POINT ( 'NONE',  ( 158.7054080432568526, 263.5240239109023150, -17.05492894054507147 ) ) ;
#4832=CARTESIAN_POINT ( 'NONE',  ( 184.9393937902272853, 291.8736057701431719, 12.09585067037464690 ) ) ;
#4833=CARTESIAN_POINT ( 'NONE',  ( 204.3276935076901850, 276.7410487817560920, 13.46217427333259309 ) ) ;
#4836=CARTESIAN_POINT ( 'NONE',  ( 81.52757139778736928, 224.0024278399161233, 9.188101187500095079 ) ) ;
#4838=CARTESIAN_POINT ( 'NONE',  ( 203.4656741260425861, 278.2341101478789369, 15.04751411186255794 ) ) ;
#4841=CARTESIAN_POINT ( 'NONE',  ( 185.0661581905127946, 259.9867678767801067, -5.962180284922311557 ) ) ;
#4844=VERTEX_POINT ( 'NONE', #38524 ) ;
#4846=ORIENTED_EDGE ( 'NONE', *, *, #78162, .F. ) ;
#4847=DIRECTION ( 'NONE',  ( 0.8660254037844387076, 0.4999999999999998890, 0.000000000000000000 ) ) ;
#4850=CARTESIAN_POINT ( 'NONE',  ( 155.0619429961492983, 262.0718317407570339, -17.08853361476647592 ) ) ;
#4852=CARTESIAN_POINT ( 'NONE',  ( 166.1309782654906257, 249.2029336093187339, -9.347746458946922132 ) ) ;
#4854=CARTESIAN_POINT ( 'NONE',  ( 152.0427391285763008, 268.8460936103824679, 15.18634991826209379 ) ) ;
#4856=CARTESIAN_POINT ( 'NONE',  ( 194.3708539535661259, 293.9868007723104029, -16.01585187499628304 ) ) ;
#4857=CARTESIAN_POINT ( 'NONE',  ( 133.1643360984345179, 253.8149278399160949, 9.188101187500093303 ) ) ;
#4858=CARTESIAN_POINT ( 'NONE',  ( 168.2960286251776836, 267.1807326767980157, -17.13187780290563822 ) ) ;
#4865=CARTESIAN_POINT ( 'NONE',  ( 167.4640555680685452, 284.2325975850394570, 9.238334356205527342 ) ) ;
#4867=ORIENTED_EDGE ( 'NONE', *, *, #61947, .T. ) ;
#4870=CARTESIAN_POINT ( 'NONE',  ( 159.4915328267279904, 280.5121072581201247, -6.654986942288538820 ) ) ;
#4875=ORIENTED_EDGE ( 'NONE', *, *, #50491, .T. ) ;
#4876=CARTESIAN_POINT ( 'NONE',  ( 182.2370137474378282, 271.6850240291627188, -16.00081368563178330 ) ) ;
#4879=CARTESIAN_POINT ( 'NONE',  ( 161.4789001435202636, 276.1860666989730362, 12.81388631890260932 ) ) ;
#4880=CARTESIAN_POINT ( 'NONE',  ( 174.2334270921930113, 280.9505671044033761, -14.19419622416070048 ) ) ;
#4882=CARTESIAN_POINT ( 'NONE',  ( 149.4539134692060145, 271.7852238117696402, 12.95627816374690688 ) ) ;
#4883=CARTESIAN_POINT ( 'NONE',  ( 163.3241744239597040, 273.7201536836278706, 14.82517280019972361 ) ) ;
#4887=ORIENTED_EDGE ( 'NONE', *, *, #66450, .T. ) ;
#4888=B_SPLINE_CURVE_WITH_KNOTS ( 'NONE', 3,
 ( #51577, #90629, #13585, #75391, #36870, #43958, #59144, #73395, #27290, #27786, #5973, #34867, #73889, #43465, #12598, #51063, #35871, #20688, #82534, #13097, #67776, #19211, #50569, #96724, #88647, #74408, #58172, #65766, #20193, #42950, #50083, #81039, #66284, #89157, #11602, #35371, #83015, #81519, #90114, #59657, #89631, #19703, #4994, #12088, #74896, #4479 ),
 .UNSPECIFIED., .F., .F.,
 ( 4, 2, 2, 2, 2, 2, 2, 2, 2, 2, 2, 2, 2, 2, 2, 2, 2, 2, 2, 2, 2, 2, 4 ),
 ( 0.001330336800848096928, 0.001796201410264788162, 0.002262066019681479179, 0.002494998324389811895, 0.002611464476743977168, 0.002727930629098142441, 0.002844396781452308148, 0.002960862933806473855, 0.003193795238514659553, 0.003659659847931111612, 0.004125524457347563671, 0.005057253676180531975, 0.005988982895013501145, 0.006454847504429985297, 0.006920712113846468581, 0.007037178266200548420, 0.007095411342377589206, 0.007153644418554628258, 0.007270110570908708963, 0.007386576723262788802, 0.007852441332679101216, 0.008318305942095415365, 0.008784170551511727779 ),
 .UNSPECIFIED. ) ;
#4889=ORIENTED_EDGE ( 'NONE', *, *, #78442, .T. ) ;
#4893=CARTESIAN_POINT ( 'NONE',  ( 173.4201897355620474, 289.8359727321131913, 2.578270883801049518 ) ) ;
#4894=CARTESIAN_POINT ( 'NONE',  ( 152.8134625983922490, 265.9663140294953791, 17.57333028169644251 ) ) ;
#4896=CARTESIAN_POINT ( 'NONE',  ( 41.75918455503629190, 206.4637435831424739, 2.679491924311251605 ) ) ;
#4897=CARTESIAN_POINT ( 'NONE',  ( 5.155129649429669669, 173.7833772461660828, -9.188101187500095079 ) ) ;
#4898=CARTESIAN_POINT ( 'NONE',  ( 97.41363812451689341, 236.2369531367911009, -4.594050593750048428 ) ) ;
#4900=CARTESIAN_POINT ( 'NONE',  ( 180.4454643261772731, 254.9133515654937696, -2.466473243201257937 ) ) ;
#4901=AXIS2_PLACEMENT_3D ( 'NONE', #25113, #76823, #92566 ) ;
#4904=CARTESIAN_POINT ( 'NONE',  ( 155.0898745997320134, 262.0234527842152374, 17.05457557403769542 ) ) ;
#4905=CARTESIAN_POINT ( 'NONE',  ( 194.2389208611690492, 294.2153155915419802, -15.75132567904764791 ) ) ;
#4907=CARTESIAN_POINT ( 'NONE',  ( 187.3930124382416693, 298.9285105704863668, -0.5915368864456632680 ) ) ;
#4908=EDGE_CURVE ( 'NONE', #9648, #3492, #58643, .T. ) ;
#4909=CARTESIAN_POINT ( 'NONE',  ( 200.1294354126899009, 267.3366221627135246, -6.812218948514619399 ) ) ;
#4910=CARTESIAN_POINT ( 'NONE',  ( 162.3094458652978744, 251.7674390756731668, -12.89874854057887354 ) ) ;
#4911=CARTESIAN_POINT ( 'NONE',  ( 176.5750811079351763, 290.0661888821730372, -9.631901365267058424 ) ) ;
#4915=EDGE_CURVE ( 'NONE', #47930, #93599, #83277, .T. ) ;
#4917=CARTESIAN_POINT ( 'NONE',  ( 82.14994038281616895, 227.4244531367911293, -4.594050593750046652 ) ) ;
#4921=CARTESIAN_POINT ( 'NONE',  ( 157.6286460899086137, 257.6261715744221306, 18.25526781158026779 ) ) ;
#4922=CARTESIAN_POINT ( 'NONE',  ( 152.2859909530489517, 266.8799217187815884, 16.93598397993736882 ) ) ;
#4923=B_SPLINE_CURVE_WITH_KNOTS ( 'NONE', 3,
 ( #74458, #66331, #26839, #5038, #50132, #41522, #57715, #4525, #58707, #81084, #19265, #58222, #4030, #72465, #64335, #73446, #89201, #42028, #11650, #42510, #34918, #18745, #96776, #97264, #80583, #89681, #20242, #95295, #64842, #95789, #25854, #3070, #56730, #26344, #87713, #33956, #57220, #49142, #88195, #53120, #84076, #7016, #75439, #68809, #99237, #92178, #28833, #74945 ),
 .UNSPECIFIED., .F., .F.,
 ( 4, 2, 2, 2, 2, 2, 2, 2, 2, 2, 2, 2, 2, 2, 2, 2, 2, 2, 2, 2, 2, 2, 2, 4 ),
 ( 0.0008144580099773583498, 0.001301468210863030231, 0.001788478411748702004, 0.002031983512191493438, 0.002275488612634284872, 0.002397241162855693383, 0.002518993713077101460, 0.002640746263298509536, 0.002762498813519918047, 0.003006003913962740706, 0.003249509014405562932, 0.003736519215291275037, 0.004710539617062700982, 0.005684560018834127794, 0.006171570219719800868, 0.006658580420605473074, 0.006780332970826863370, 0.006841209245937644387, 0.006902085521048426271, 0.007145590621491398550, 0.007632600822377442855, 0.008119611023263488894, 0.008363116123706508878, 0.008606621224149532332 ),
 .UNSPECIFIED. ) ;
#4924=CARTESIAN_POINT ( 'NONE',  ( 197.0943835026307056, 289.2695092174155889, 17.13247302375833669 ) ) ;
#4928=CARTESIAN_POINT ( 'NONE',  ( 193.1649355862271591, 296.0755126543221536, -12.21556774862162698 ) ) ;
#4930=ORIENTED_EDGE ( 'NONE', *, *, #25360, .F. ) ;
#4933=CARTESIAN_POINT ( 'NONE',  ( 193.1569697810063531, 296.0893098336876506, -13.02398914535779539 ) ) ;
#4935=ORIENTED_EDGE ( 'NONE', *, *, #76767, .F. ) ;
#4938=CARTESIAN_POINT ( 'NONE',  ( 198.0006249058153003, 287.6998530631771587, 18.31850453277666801 ) ) ;
#4939=CARTESIAN_POINT ( 'NONE',  ( 157.8154903851704205, 268.3609324989079710, 16.38998070839103249 ) ) ;
#4941=CARTESIAN_POINT ( 'NONE',  ( 136.1324508756439400, 242.7365022471902307, 10.00000000000009592 ) ) ;
#4945=CARTESIAN_POINT ( 'NONE',  ( 165.5459811318285972, 246.9046815158575328, -1.768130512343973226 ) ) ;
#4946=EDGE_LOOP ( 'NONE', ( #84609, #14073, #50650, #71398 ) ) ;
#4949=ORIENTED_EDGE ( 'NONE', *, *, #10768, .T. ) ;
#4952=CARTESIAN_POINT ( 'NONE',  ( 189.3510599963105960, 290.0131996961930554, 14.40846774032805300 ) ) ;
#4953=CARTESIAN_POINT ( 'NONE',  ( 158.5534433844464104, 256.0243756735802094, 16.12506798773286221 ) ) ;
#4954=CARTESIAN_POINT ( 'NONE',  ( 147.0210896547505399, 249.5643266524160140, 9.188101187500095079 ) ) ;
#4956=CARTESIAN_POINT ( 'NONE',  ( 192.2836406301186685, 296.5693283646611462, -11.72525413493355373 ) ) ;
#4959=CARTESIAN_POINT ( 'NONE',  ( 164.9592205905213973, 274.6244470290632194, 14.74651761685257512 ) ) ;
#4965=CARTESIAN_POINT ( 'NONE',  ( 194.3442947553755005, 294.0328026529847421, -15.97648891113594871 ) ) ;
#4968=CARTESIAN_POINT ( 'NONE',  ( 158.7507817778773074, 280.7662553832301455, -8.161742422992587009 ) ) ;
#4969=CARTESIAN_POINT ( 'NONE',  ( 147.6121581866023007, 274.9752375363476631, 8.700660424766859080 ) ) ;
#4972=EDGE_CURVE ( 'NONE', #38611, #37700, #26531, .T. ) ;
#4974=CARTESIAN_POINT ( 'NONE',  ( 96.30395630197683943, 238.6589784336661637, -6.496448406907675876E-16 ) ) ;
#4976=CARTESIAN_POINT ( 'NONE',  ( 171.7154418923348942, 259.3365693118849435, -15.26938553599716641 ) ) ;
#4978=CARTESIAN_POINT ( 'NONE',  ( 164.8623370068202689, 277.1737403023538491, -13.48993746920329073 ) ) ;
#4984=CARTESIAN_POINT ( 'NONE',  ( 157.7529601300917363, 257.4108533407307959, 16.91445305439664892 ) ) ;
#4986=CARTESIAN_POINT ( 'NONE',  ( 208.1583869480885483, 270.1060931147653719, 3.025867354224990979 ) ) ;
#4990=CARTESIAN_POINT ( 'NONE',  ( 162.8223739550644211, 248.6303710312858186, -11.16939803179192658 ) ) ;
#4991=ORIENTED_EDGE ( 'NONE', *, *, #22539, .F. ) ;
#4992=EDGE_CURVE ( 'NONE', #35225, #15906, #23827, .T. ) ;
#4993=B_SPLINE_CURVE_WITH_KNOTS ( 'NONE', 3,
 ( #55173, #85652, #54167, #76985 ),
 .UNSPECIFIED., .F., .F.,
 ( 4, 4 ),
 ( 0.000000000000000000, 0.001252170427096359296 ),
 .UNSPECIFIED. ) ;
#4994=CARTESIAN_POINT ( 'NONE',  ( 194.8450826448002715, 266.1639313023655973, -8.766057580558177520 ) ) ;
#4997=CARTESIAN_POINT ( 'NONE',  ( 123.3944002380500677, 251.2369531367911293, -4.594050593750048428 ) ) ;
#5001=CARTESIAN_POINT ( 'NONE',  ( 147.3154503175461514, 275.4891506405583073, 3.671329888160011823 ) ) ;
#5002=CARTESIAN_POINT ( 'NONE',  ( 60.78824074639776143, 199.2365022471902307, 10.00000000000009948 ) ) ;
#5003=CARTESIAN_POINT ( 'NONE',  ( 159.9470087484377814, 253.6106496594791508, -16.54933891566789939 ) ) ;
#5004=CARTESIAN_POINT ( 'NONE',  ( 192.4273719102352800, 271.7576443049806585, 14.08159452427905300 ) ) ;
#5005=CARTESIAN_POINT ( 'NONE',  ( 178.2382707639212356, 285.7843550335422833, 14.43266090959460435 ) ) ;
#5007=CARTESIAN_POINT ( 'NONE',  ( 198.9728866542080823, 282.1116337930695295, -16.69484273823314879 ) ) ;
#5011=CARTESIAN_POINT ( 'NONE',  ( 61.98804677278346986, 206.5958772461660828, -9.188101187500095079 ) ) ;
#5012=CARTESIAN_POINT ( 'NONE',  ( 206.1408608592916494, 273.6005508061571732, -10.42739367433323494 ) ) ;
#5013=CARTESIAN_POINT ( 'NONE',  ( -22.42236680055709641, 157.8615022471902591, 0.000000000000000000 ) ) ;
#5014=CARTESIAN_POINT ( 'NONE',  ( 207.9328781051891042, 270.4966858882232259, -0.8820402142964423042 ) ) ;
#5018=CARTESIAN_POINT ( 'NONE',  ( 185.8639835793372583, 267.1203966262607992, -15.06692291552070273 ) ) ;
#5022=CARTESIAN_POINT ( 'NONE',  ( 205.9652721086518739, 272.7100367737629085, -9.293361325695892461 ) ) ;
#5023=CARTESIAN_POINT ( 'NONE',  ( 24.28913873611587348, 175.6423013555409796, -4.594050593750043987 ) ) ;
#5026=EDGE_CURVE ( 'NONE', #52618, #83827, #17955, .T. ) ;
#5030=CARTESIAN_POINT ( 'NONE',  ( 53.65289935712326042, 189.5327760586659167, 1.948934522072302763E-15 ) ) ;
#5031=CARTESIAN_POINT ( 'NONE',  ( 200.9110265982630779, 282.6588894614233141, 17.52479721249226685 ) ) ;
#5032=CARTESIAN_POINT ( 'NONE',  ( 171.2443824779643080, 286.7566234589221494, 7.224323052557026337 ) ) ;
#5033=CARTESIAN_POINT ( 'NONE',  ( 147.4317198359019301, 275.2877659273946733, 3.797273160043843188 ) ) ;
#5035=CARTESIAN_POINT ( 'NONE',  ( 202.9457411048790618, 270.0800994776229800, -6.926181921767012639 ) ) ;
#5036=CARTESIAN_POINT ( 'NONE',  ( 178.7320898300308727, 293.3905527527083450, 2.643181550327659668 ) ) ;
#5037=CARTESIAN_POINT ( 'NONE',  ( 176.5744236666108691, 275.1798363790605322, 17.44874769457867458 ) ) ;
#5038=CARTESIAN_POINT ( 'NONE',  ( 179.6882155687777356, 278.8364783109157088, -17.29851916968328140 ) ) ;
#5040=CARTESIAN_POINT ( 'NONE',  ( 167.1114647352963232, 257.9194854303543138, -15.52048492569388038 ) ) ;
#5041=ADVANCED_FACE ( 'NONE', ( #46375 ), #24590, .T. ) ;
#5043=CARTESIAN_POINT ( 'NONE',  ( 149.0710170770012724, 245.3262482093457777, 3.021315404115420679E-15 ) ) ;
#5044=CARTESIAN_POINT ( 'NONE',  ( 91.45997379709655206, 233.6115022471902876, -5.000000000000047962 ) ) ;
#5046=CARTESIAN_POINT ( 'NONE',  ( 165.2187654623328683, 269.8677273813709121, -16.27684390681923432 ) ) ;
#5047=ORIENTED_EDGE ( 'NONE', *, *, #52016, .T. ) ;
#5048=CARTESIAN_POINT ( 'NONE',  ( 60.33744616864313315, 196.4548013555410080, -4.594050593750042211 ) ) ;
#5050=DIRECTION ( 'NONE',  ( -0.4999999999999987788, 0.8660254037844392627, 0.000000000000000000 ) ) ;
#5051=CARTESIAN_POINT ( 'NONE',  ( 146.7845206192450007, 276.4087478532630939, 4.443586170796542945 ) ) ;
#5054=CARTESIAN_POINT ( 'NONE',  ( 71.01270533261738649, 200.2592609112379591, 2.679491924311254714 ) ) ;
#5055=CARTESIAN_POINT ( 'NONE',  ( 164.2953672501826929, 246.0790718049323687, -2.576662677987826111 ) ) ;
#5058=CARTESIAN_POINT ( 'NONE',  ( 185.7415151600560819, 263.1377994056483089, 11.14276090414980480 ) ) ;
#5059=CARTESIAN_POINT ( 'NONE',  ( 149.1004267900891307, 272.3974806997987343, -12.86882154300063341 ) ) ;
#5060=CARTESIAN_POINT ( 'NONE',  ( 156.8296764551412537, 259.0100275755436883, 18.25869368615038013 ) ) ;
#5061=ORIENTED_EDGE ( 'NONE', *, *, #98017, .F. ) ;
#5069=CARTESIAN_POINT ( 'NONE',  ( 159.3586121662929713, 254.6297824347537642, -15.50090345830412630 ) ) ;
#5070=ORIENTED_EDGE ( 'NONE', *, *, #24480, .T. ) ;
#5072=CARTESIAN_POINT ( 'NONE',  ( 207.3874697692679945, 271.4413608369101780, -6.809237722377445401 ) ) ;
#5074=CARTESIAN_POINT ( 'NONE',  ( 182.3700640764176342, 263.2847133751610045, -13.94439451147478337 ) ) ;
#5075=ORIENTED_EDGE ( 'NONE', *, *, #18319, .T. ) ;
#5077=CARTESIAN_POINT ( 'NONE',  ( 159.3767386493506137, 254.5983864451355032, 15.47015898230477760 ) ) ;
#5078=CARTESIAN_POINT ( 'NONE',  ( 182.6784043417008263, 256.7666309132076776, 5.682484670743590094 ) ) ;
#5080=CARTESIAN_POINT ( 'NONE',  ( 137.4948102131217240, 244.0643266524160424, -9.188101187500093303 ) ) ;
#5082=CARTESIAN_POINT ( 'NONE',  ( -22.42236680055709641, 157.8615022471902591, 0.000000000000000000 ) ) ;
#5088=CARTESIAN_POINT ( 'NONE',  ( 159.5573297132660002, 254.2855935470410031, 16.91607698584599007 ) ) ;
#5090=CARTESIAN_POINT ( 'NONE',  ( 77.90126356732251622, 215.7833772461660544, -9.188101187500095079 ) ) ;
#5093=CARTESIAN_POINT ( 'NONE',  ( 198.2860450010354043, 287.2054909567549430, 18.54284983329501557 ) ) ;
#5095=CARTESIAN_POINT ( 'NONE',  ( 182.3414255478350299, 257.1538671092444588, -6.203902589603837114 ) ) ;
#5096=ORIENTED_EDGE ( 'NONE', *, *, #92773, .F. ) ;
#5099=CARTESIAN_POINT ( 'NONE',  ( 153.2283961777204695, 265.2476279883323400, -17.66880461074566000 ) ) ;
#5102=CARTESIAN_POINT ( 'NONE',  ( 206.8217325168575371, 270.0045844243117017, 3.350393751014514532 ) ) ;
#5103=EDGE_CURVE ( 'NONE', #29135, #35604, #72326, .T. ) ;
#5105=CARTESIAN_POINT ( 'NONE',  ( 165.1399196574946018, 246.6162641258139843, 5.603258891903981187 ) ) ;
#5107=CARTESIAN_POINT ( 'NONE',  ( 176.9050207115652711, 269.9844065969573990, 16.88525275472998288 ) ) ;
#5108=CARTESIAN_POINT ( 'NONE',  ( 148.9322735291567597, 272.6887306911919495, -12.40988026045598858 ) ) ;
#5109=CARTESIAN_POINT ( 'NONE',  ( 199.0131399161024035, 281.1222020366274137, 17.22481283254653306 ) ) ;
#5110=CARTESIAN_POINT ( 'NONE',  ( 207.5792673731680793, 271.1091576421853233, 2.359198794924813214 ) ) ;
#5111=CARTESIAN_POINT ( 'NONE',  ( 116.3579438323015012, 247.1744531367911293, 4.594050593750047540 ) ) ;
#5112=ORIENTED_EDGE ( 'NONE', *, *, #70437, .F. ) ;
#5116=CARTESIAN_POINT ( 'NONE',  ( 204.9427641582406636, 275.6757151647582305, 14.40446820030680897 ) ) ;
#5119=CARTESIAN_POINT ( 'NONE',  ( 178.6379759496232111, 254.3921254701204759, 4.464154310029138983 ) ) ;
#5125=CARTESIAN_POINT ( 'NONE',  ( 201.2290932460805948, 267.4596528866035783, 0.8384362464926046199 ) ) ;
#5126=CARTESIAN_POINT ( 'NONE',  ( 199.0733432591706276, 265.2368624245646060, 0.1624720798152879120 ) ) ;
#5127=CARTESIAN_POINT ( 'NONE',  ( 190.1693911629507738, 301.2639477917662703, -5.112716700269980485 ) ) ;
#5129=CARTESIAN_POINT ( 'NONE',  ( 193.3516273516660533, 268.9799088949432075, 12.17662679305565909 ) ) ;
#5133=CARTESIAN_POINT ( 'NONE',  ( 190.5477107455830321, 300.6086790531491033, 3.126266616601216963 ) ) ;
#5135=CARTESIAN_POINT ( 'NONE',  ( -27.42236680055714260, 166.5217562850347406, 1.224646799147364892E-15 ) ) ;
#5136=CARTESIAN_POINT ( 'NONE',  ( 201.3911183001464451, 266.9640362439821502, -3.754059931952923534 ) ) ;
#5137=CARTESIAN_POINT ( 'NONE',  ( 161.2966333957525933, 251.2730311991824408, 13.85068866972710744 ) ) ;
#5139=CARTESIAN_POINT ( 'NONE',  ( 142.4652616372697480, 246.3927522451418497, 10.00000000000009592 ) ) ;
#5140=CARTESIAN_POINT ( 'NONE',  ( 182.7403103768833432, 278.7531403573107127, 17.53058794496005390 ) ) ;
#5141=ORIENTED_EDGE ( 'NONE', *, *, #41856, .F. ) ;
#5143=CARTESIAN_POINT ( 'NONE',  ( 157.5042325173297684, 257.8416622032797818, 16.70595240278738203 ) ) ;
#5144=CARTESIAN_POINT ( 'NONE',  ( 150.6815632051821581, 269.6588720951601772, -14.68790257316217307 ) ) ;
#5145=CARTESIAN_POINT ( 'NONE',  ( -13.87062626178347813, 171.9869531367911293, 4.594050593750046652 ) ) ;
#5146=CARTESIAN_POINT ( 'NONE',  ( 61.77188751760236585, 194.2202760586659736, -5.415160957724236172E-17 ) ) ;
#5150=FACE_OUTER_BOUND ( 'NONE', #96864, .T. ) ;
#5154=CARTESIAN_POINT ( 'NONE',  ( 171.4364880475070265, 258.3207074781752794, 14.28679915105377241 ) ) ;
#5155=CARTESIAN_POINT ( 'NONE',  ( 67.91490812815924016, 210.0177522451418497, -10.00000000000009592 ) ) ;
#5156=EDGE_CURVE ( 'NONE', #2331, #55485, #27122, .T. ) ;
#5158=CARTESIAN_POINT ( 'NONE',  ( 150.3737790450080354, 270.1919698983467697, 15.09624067603409969 ) ) ;
#5159=CARTESIAN_POINT ( 'NONE',  ( 55.08690683815017763, 202.6115022471902591, 10.00000000000009592 ) ) ;
#5160=CARTESIAN_POINT ( 'NONE',  ( 181.8512048739169700, 291.6361654578719254, 9.308531600642181658 ) ) ;
#5161=CARTESIAN_POINT ( 'NONE',  ( 202.9216520459657147, 279.1763840310111391, 15.75371595331685803 ) ) ;
#5162=CARTESIAN_POINT ( 'NONE',  ( 18.84898279888859918, 187.8149278399161233, 9.188101187500093303 ) ) ;
#5164=CARTESIAN_POINT ( 'NONE',  ( 2.788041384736548611, 183.9637435831425307, 2.679491924311251605 ) ) ;
#5166=CARTESIAN_POINT ( 'NONE',  ( 201.2846070193694175, 280.3231637734562582, -16.68660556726656807 ) ) ;
#5167=CARTESIAN_POINT ( 'NONE',  ( 179.3828213106868077, 277.5311947685291329, 17.51078081574469536 ) ) ;
#5169=CARTESIAN_POINT ( 'NONE',  ( 153.4176784699686777, 265.3156473403554969, -16.22513339788883968 ) ) ;
#5176=CARTESIAN_POINT ( 'NONE',  ( 194.0672051292551430, 294.5127359636757660, 15.53337744471869364 ) ) ;
#5177=ORIENTED_EDGE ( 'NONE', *, *, #25032, .F. ) ;
#5179=CARTESIAN_POINT ( 'NONE',  ( 103.9969882237314351, 242.3967562850347122, -4.648177544792955347E-16 ) ) ;
#5186=CARTESIAN_POINT ( 'NONE',  ( 201.5931001570695571, 271.8169877960688723, -11.84458199429158931 ) ) ;
#5187=CARTESIAN_POINT ( 'NONE',  ( 203.1526193585190470, 278.7763369107815379, -16.67658907091021447 ) ) ;
#5188=ORIENTED_EDGE ( 'NONE', *, *, #40157, .F. ) ;
#5189=CARTESIAN_POINT ( 'NONE',  ( 164.4077444581934060, 246.8171098232803047, -5.536143951676388397 ) ) ;
#5190=CARTESIAN_POINT ( 'NONE',  ( 164.4990934228277411, 245.7262077230798809, 6.470820838822735510 ) ) ;
#5191=CARTESIAN_POINT ( 'NONE',  ( 192.7693357657653053, 296.7607116428271183, 12.22606306887835714 ) ) ;
#5192=ORIENTED_EDGE ( 'NONE', *, *, #4721, .T. ) ;
#5195=CARTESIAN_POINT ( 'NONE',  ( 174.5400248142499890, 262.3018208131371125, 14.37995792819177154 ) ) ;
#5197=LINE ( 'NONE', #75598, #96114 ) ;
#5200=ORIENTED_EDGE ( 'NONE', *, *, #4454, .T. ) ;
#5201=CARTESIAN_POINT ( 'NONE',  ( 206.4229368915142686, 273.1119807867502800, 10.31819530520674810 ) ) ;
#5202=CARTESIAN_POINT ( 'NONE',  ( 151.0534475874070779, 275.6857711074018766, -8.249277203261174307 ) ) ;
#5203=ORIENTED_EDGE ( 'NONE', *, *, #58316, .T. ) ;
#5204=CARTESIAN_POINT ( 'NONE',  ( 177.4590209526847389, 279.3686772430251608, -16.70803785899330762 ) ) ;
#5205=DIRECTION ( 'NONE',  ( 0.4999999999999992784, -0.8660254037844390407, 0.000000000000000000 ) ) ;
#5206=EDGE_CURVE ( 'NONE', #94561, #86855, #57060, .T. ) ;
#5207=ORIENTED_EDGE ( 'NONE', *, *, #93109, .F. ) ;
#5209=CARTESIAN_POINT ( 'NONE',  ( 193.2053309019613891, 296.0055459150826778, -12.79465285318189061 ) ) ;
#5211=CARTESIAN_POINT ( 'NONE',  ( 157.3127155075455050, 269.2413269589708307, 15.61457394689876388 ) ) ;
#5213=( BOUNDED_CURVE ( )  B_SPLINE_CURVE ( 2, ( #58570, #64189, #17592, #71813, #95138, #10494, #11516, #64699, #73304 ),
 .UNSPECIFIED., .F., .T. ) 
 B_SPLINE_CURVE_WITH_KNOTS ( ( 3, 2, 2, 2, 3 ),
 ( 0.03629032258064516375, 0.03763440860215053890, 0.04032258064516128920, 0.04301075268817204644, 0.04435483870967742159 ),
 .UNSPECIFIED. ) 
 CURVE ( )  GEOMETRIC_REPRESENTATION_ITEM ( )  RATIONAL_B_SPLINE_CURVE ( ( 0.9330127018922194093, 0.9330127018922195203, 1.000000000000000000, 0.8660254037844387076, 1.000000000000000000, 0.8660254037844387076, 1.000000000000000000, 0.9330127018922194093, 0.9330127018922194093 ) ) 
 REPRESENTATION_ITEM ( '' )  );
#5214=CARTESIAN_POINT ( 'NONE',  ( 156.5650439790640860, 266.5144819405009571, -16.22741892766980953 ) ) ;
#5215=CARTESIAN_POINT ( 'NONE',  ( 169.0688750560406675, 272.3726058702321779, 16.94514216011815932 ) ) ;
#5216=CARTESIAN_POINT ( 'NONE',  ( 190.2236813008869660, 301.1699145145108218, -5.401374690107298093 ) ) ;
#5218=CARTESIAN_POINT ( 'NONE',  ( 148.9228818358559749, 272.7049975811580680, 12.13823097167056275 ) ) ;
#5219=CARTESIAN_POINT ( 'NONE',  ( 192.3401793061076717, 297.5040324353506094, 12.56432540404525611 ) ) ;
#5221=CARTESIAN_POINT ( 'NONE',  ( 177.2398528310001495, 290.8784864842746174, 6.085034101453419275 ) ) ;
#5222=CARTESIAN_POINT ( 'NONE',  ( 146.5095091551180815, 276.8850816817948726, 0.1418322875769769398 ) ) ;
#5225=AXIS2_PLACEMENT_3D ( 'NONE', #7540, #98778, #60719 ) ;
#5226=CARTESIAN_POINT ( 'NONE',  ( 149.6230451358742926, 271.4922791719315001, -12.72565967355361671 ) ) ;
#5227=CARTESIAN_POINT ( 'NONE',  ( 164.9356397357043704, 244.9700873293209042, 2.799217332519396972 ) ) ;
#5228=CARTESIAN_POINT ( 'NONE',  ( 198.5966822647444587, 286.6674514332866579, 17.25284514431582750 ) ) ;
#5229=CARTESIAN_POINT ( 'NONE',  ( 171.2304119843477963, 289.1496298482710472, 4.331491222947584596 ) ) ;
#5237=CARTESIAN_POINT ( 'NONE',  ( 199.0619536713871582, 285.8615777176725032, -18.61677200412056976 ) ) ;
#5238=ORIENTED_EDGE ( 'NONE', *, *, #35698, .F. ) ;
#5239=CARTESIAN_POINT ( 'NONE',  ( 207.9328781051891042, 270.4966858882232259, -0.8820402142964423042 ) ) ;
#5241=CARTESIAN_POINT ( 'NONE',  ( 201.0468719883840265, 282.4235983437597497, -16.59631526626950659 ) ) ;
#5242=CARTESIAN_POINT ( 'NONE',  ( 165.0532575723395041, 244.7663672603923715, -2.144843157699870773 ) ) ;
#5243=CARTESIAN_POINT ( 'NONE',  ( 27.64472685218285264, 186.7677522451418497, 10.00000000000009592 ) ) ;
#5244=CARTESIAN_POINT ( 'NONE',  ( 117.4951228184160783, 229.4548013555409796, -4.594050593750042211 ) ) ;
#5246=CARTESIAN_POINT ( 'NONE',  ( 180.8047931442907270, 294.0922736414096903, -2.692425206983429131 ) ) ;
#5247=CARTESIAN_POINT ( 'NONE',  ( 162.8839686824157127, 249.6387011324054015, -11.33670648097108113 ) ) ;
#5249=CARTESIAN_POINT ( 'NONE',  ( 163.1177074157340030, 248.1188384722309195, 11.53923137679231026 ) ) ;
#5250=CARTESIAN_POINT ( 'NONE',  ( 30.81113223654366706, 188.5958772461660544, -9.188101187500095079 ) ) ;
#5253=CYLINDRICAL_SURFACE ( 'NONE', #52742, 10.00000000000010658 ) ;
#5256=DIRECTION ( 'NONE',  ( 0.4999999999999992784, -0.8660254037844390407, 0.000000000000000000 ) ) ;
#5259=CARTESIAN_POINT ( 'NONE',  ( 179.0026682949594488, 287.9522070891227941, -12.87249257965389759 ) ) ;
#5261=EDGE_CURVE ( 'NONE', #53287, #82871, #57996, .T. ) ;
#5263=CARTESIAN_POINT ( 'NONE',  ( 95.19470834736912934, 215.7677522451417929, -5.000000000000041744 ) ) ;
#5264=ORIENTED_EDGE ( 'NONE', *, *, #71455, .F. ) ;
#5266=ADVANCED_FACE ( 'NONE', ( #30083 ), #8781, .T. ) ;
#5267=EDGE_CURVE ( 'NONE', #34753, #63230, #62581, .T. ) ;
#5268=CARTESIAN_POINT ( 'NONE',  ( 202.4943568615953779, 279.9164810001701085, 17.09064351659286984 ) ) ;
#5269=CARTESIAN_POINT ( 'NONE',  ( 208.0006710756887287, 270.3792650189220126, -0.8737665032493013850 ) ) ;
#5270=CARTESIAN_POINT ( 'NONE',  ( 9.403806464923315289, 185.4244531367911293, -4.594050593750046652 ) ) ;
#5276=CARTESIAN_POINT ( 'NONE',  ( 56.95444766116892055, 197.5643266524159856, -9.188101187500093303 ) ) ;
#5277=CARTESIAN_POINT ( 'NONE',  ( 163.7595992360150490, 247.0070492265414828, -6.976205010573520049 ) ) ;
#5278=CARTESIAN_POINT ( 'NONE',  ( 203.6731738038005517, 276.2319078309685096, 13.32647105319332326 ) ) ;
#5282=B_SPLINE_CURVE_WITH_KNOTS ( 'NONE', 3,
 ( #18556, #87522, #18054, #79884 ),
 .UNSPECIFIED., .F., .F.,
 ( 4, 4 ),
 ( 0.009818966555397349791, 0.01814036154117733973 ),
 .UNSPECIFIED. ) ;
#5283=CARTESIAN_POINT ( 'NONE',  ( 16.11576366785043746, 180.1115022471902591, 10.00000000000009592 ) ) ;
#5285=CARTESIAN_POINT ( 'NONE',  ( 146.3987206697217403, 246.1423013555409796, -4.594050593750043987 ) ) ;
#5287=CARTESIAN_POINT ( 'NONE',  ( 188.7923053583308217, 259.7687708077174307, -4.103412599247693748 ) ) ;
#5288=CARTESIAN_POINT ( 'NONE',  ( -27.42236680055714260, 166.5217562850347406, 1.224646799147364892E-15 ) ) ;
#5289=CARTESIAN_POINT ( 'NONE',  ( 197.3711752247862705, 281.8738618512871881, -17.64585401704185941 ) ) ;
#5293=ORIENTED_EDGE ( 'NONE', *, *, #21840, .F. ) ;
#5294=CARTESIAN_POINT ( 'NONE',  ( 191.4922467593309250, 298.9726946877590876, 7.604184559945784017 ) ) ;
#5295=CARTESIAN_POINT ( 'NONE',  ( 208.1052924987534425, 270.1980553986139171, -0.2554279711716039847 ) ) ;
#5296=CARTESIAN_POINT ( 'NONE',  ( 152.2397443934144690, 268.7033665454236484, -15.42800614587808461 ) ) ;
#5298=CARTESIAN_POINT ( 'NONE',  ( 170.6178593158246315, 266.5408558992322696, -17.65857870869936974 ) ) ;
#5299=LINE ( 'NONE', #91928, #66907 ) ;
#5303=CARTESIAN_POINT ( 'NONE',  ( 168.7064118984686161, 282.3780792379856166, -10.92572408344284440 ) ) ;
#5304=B_SPLINE_SURFACE_WITH_KNOTS ( 'NONE', 3, 1, ( 
 ( #58821, #73558 ),
 ( #12260, #82198 ),
 ( #49751, #18868 ),
 ( #57838, #43118 ),
 ( #90294, #96390 ),
 ( #74572, #97373 ),
 ( #4142, #65942 ),
 ( #81687, #13262 ),
 ( #26954, #36031 ),
 ( #19865, #50732 ),
 ( #96895, #44122 ),
 ( #80703, #88818 ),
 ( #11279, #51229 ),
 ( #74063, #66931 ),
 ( #27939, #19384 ),
 ( #89783, #88314 ),
 ( #81197, #28432 ),
 ( #59314, #11766 ),
 ( #26464, #20359 ),
 ( #35037, #20863 ),
 ( #4651, #73071 ),
 ( #51754, #27465 ),
 ( #82696, #75059 ),
 ( #66445, #12768 ),
 ( #43633, #3669 ),
 ( #5636, #36529 ),
 ( #95906, #57340 ),
 ( #98862, #46110 ),
 ( #30431, #90793 ),
 ( #38521, #67941 ),
 ( #54208, #7630 ),
 ( #68922, #14242 ),
 ( #13736, #29932 ),
 ( #99354, #92765 ) ),
 .UNSPECIFIED., .T., .F., .F.,
 ( 4, 2, 2, 2, 2, 2, 2, 2, 2, 2, 2, 2, 2, 2, 2, 2, 4 ),
 ( 2, 2 ),
 ( 0.000000000000000000, 0.06250000000000000000, 0.1250000000000000000, 0.1875000000000000000, 0.2500000000000000000, 0.3125000000000000000, 0.3750000000000000000, 0.4375000000000000000, 0.5000000000000000000, 0.5625000000000000000, 0.6250000000000000000, 0.6875000000000000000, 0.7500000000000000000, 0.8125000000000000000, 0.8750000000000000000, 0.9375000000000000000, 1.000000000000000000 ),
 ( 0.000000000000000000, 1.000000000000000000 ),
 .UNSPECIFIED. ) ;
#5307=CARTESIAN_POINT ( 'NONE',  ( 181.8596306508903524, 295.2094889523889378, 4.865735665145750843 ) ) ;
#5308=CARTESIAN_POINT ( 'NONE',  ( 146.5247557210571756, 248.7365022471902023, 10.00000000000009948 ) ) ;
#5312=CARTESIAN_POINT ( 'NONE',  ( 159.1344352748853055, 279.7114264697810313, -10.00621538743078354 ) ) ;
#5318=CARTESIAN_POINT ( 'NONE',  ( 159.3149481673140144, 263.8852099524119126, -17.20139123423869520 ) ) ;
#5319=VERTEX_POINT ( 'NONE', #99005 ) ;
#5320=CARTESIAN_POINT ( 'NONE',  ( 146.7818291168261453, 276.4134096722012828, -0.7617065417431535534 ) ) ;
#5321=CARTESIAN_POINT ( 'NONE',  ( 186.0392071921917534, 291.3832317854910343, 12.18629431491837600 ) ) ;
#5323=CARTESIAN_POINT ( 'NONE',  ( 204.8523313866422484, 275.8323493198358847, 14.65426965484541100 ) ) ;
#5324=CARTESIAN_POINT ( 'NONE',  ( 51.11762373747147592, 206.9865022471902876, -10.00000000000009592 ) ) ;
#5325=ORIENTED_EDGE ( 'NONE', *, *, #20648, .T. ) ;
#5326=CARTESIAN_POINT ( 'NONE',  ( 88.45577462806285496, 228.0024278399160949, -9.188101187500093303 ) ) ;
#5327=CARTESIAN_POINT ( 'NONE',  ( 155.3184171719837252, 261.6276054373827833, 18.58354126389791361 ) ) ;
#5329=CARTESIAN_POINT ( 'NONE',  ( 185.1433062948085251, 259.8750339556800100, -6.566076700648285858 ) ) ;
#5332=CARTESIAN_POINT ( 'NONE',  ( 192.9672696936424074, 283.3911346215554659, -17.79517654261226767 ) ) ;
#5337=CARTESIAN_POINT ( 'NONE',  ( 203.1705638993064156, 278.7452560544191442, -15.08126533799095093 ) ) ;
#5339=CARTESIAN_POINT ( 'NONE',  ( 182.7224642469025468, 280.1677561527186526, -16.13469908156701393 ) ) ;
#5340=FACE_OUTER_BOUND ( 'NONE', #3268, .T. ) ;
#5341=CARTESIAN_POINT ( 'NONE',  ( 81.75096066047075283, 229.5530062829863027, -4.648177544792955347E-16 ) ) ;
#5344=CARTESIAN_POINT ( 'NONE',  ( 168.2829851573790165, 267.1582986060611802, -17.45266922015316879 ) ) ;
#5349=CARTESIAN_POINT ( 'NONE',  ( 167.2946170330464497, 284.3018367931351804, 9.330332355628671692 ) ) ;
#5350=CARTESIAN_POINT ( 'NONE',  ( 203.9579186766783891, 271.6971408411359334, 9.704203457501737518 ) ) ;
#5353=CARTESIAN_POINT ( 'NONE',  ( 163.1008115941903895, 248.1481028935802442, 11.25332017433677834 ) ) ;
#5354=CARTESIAN_POINT ( 'NONE',  ( 188.9068162171112419, 259.6246725331779999, 2.484684062397731097 ) ) ;
#5355=CARTESIAN_POINT ( 'NONE',  ( 160.7119030392097727, 282.6337468314966372, -6.452778162566800368 ) ) ;
#5356=ADVANCED_FACE ( 'NONE', ( #37668 ), #805, .F. ) ;
#5357=CARTESIAN_POINT ( 'NONE',  ( 174.5432515410337544, 282.4104588529930311, -15.15290805577315680 ) ) ;
#5363=CARTESIAN_POINT ( 'NONE',  ( 102.4216706764260465, 218.3932355074535678, -2.679491924311248496 ) ) ;
#5365=ORIENTED_EDGE ( 'NONE', *, *, #96234, .F. ) ;
#5366=CARTESIAN_POINT ( 'NONE',  ( 11.48900327905998431, 165.8932355074535678, -2.679491924311248496 ) ) ;
#5367=CARTESIAN_POINT ( 'NONE',  ( 171.4037692059896472, 279.8853805441466420, -15.04371018346111377 ) ) ;
#5370=CARTESIAN_POINT ( 'NONE',  ( 162.5447505464307483, 273.3239273621815073, 14.91589735394761007 ) ) ;
#5371=CARTESIAN_POINT ( 'NONE',  ( -16.90171517502901466, 170.2369531367911293, -4.594050593750048428 ) ) ;
#5373=CARTESIAN_POINT ( 'NONE',  ( 188.3993081743329014, 296.6400551805262467, 8.121699605044829795 ) ) ;
#5377=CARTESIAN_POINT ( 'NONE',  ( 189.8395658503075367, 274.1636632147208843, -15.63209073522486214 ) ) ;
#5378=AXIS2_PLACEMENT_3D ( 'NONE', #72081, #16858, #72592 ) ;
#5380=CARTESIAN_POINT ( 'NONE',  ( 171.6531670106267029, 289.5256590595021748, 2.674700294240007103 ) ) ;
#5385=CARTESIAN_POINT ( 'NONE',  ( 0.4998960083233069396, 183.3464784336661637, 1.353441290958777525E-15 ) ) ;
#5386=CARTESIAN_POINT ( 'NONE',  ( 100.9591899430832029, 229.0958772461660260, -9.188101187500095079 ) ) ;
#5387=CARTESIAN_POINT ( 'NONE',  ( 44.53222222597941027, 196.5177522451418781, -10.00000000000009592 ) ) ;
#5388=CARTESIAN_POINT ( 'NONE',  ( 186.7556369116643680, 295.8656198945773781, -7.669303673011643063 ) ) ;
#5392=CARTESIAN_POINT ( 'NONE',  ( 177.4587666978972322, 282.9167551205503628, -14.35547426222066925 ) ) ;
#5394=CARTESIAN_POINT ( 'NONE',  ( 193.8603219414924013, 294.8710681561126989, 15.36476279452078586 ) ) ;
#5395=CARTESIAN_POINT ( 'NONE',  ( 183.2664581031647231, 274.6986942775652665, 16.36951637877005084 ) ) ;
#5396=CARTESIAN_POINT ( 'NONE',  ( 147.8819534105757043, 274.5079385007862811, -9.338341377131436971 ) ) ;
#5397=EDGE_CURVE ( 'NONE', #79979, #87041, #68336, .T. ) ;
#5399=CARTESIAN_POINT ( 'NONE',  ( 193.1215250612204102, 265.4992790482471605, 7.789832503989316592 ) ) ;
#5401=CARTESIAN_POINT ( 'NONE',  ( 184.4954910655095546, 268.6554621394339506, -15.49256567782061467 ) ) ;
#5402=B_SPLINE_CURVE_WITH_KNOTS ( 'NONE', 3,
 ( #72318, #11016, #19120, #60805, #91765, #84669, #37259, #13001, #60047, #50967, #4376, #13974, #98598, #5380, #51975, #51470, #52960, #81919, #21575, #6376, #82915, #11994, #60543, #29180, #4893, #13489, #68157, #91012, #66182, #52459, #27693, #12495, #82438, #67668, #43860, #74802, #35775, #66670, #44359, #90015, #97606, #43362, #28173, #99084, #29666, #75292, #36266, #59045, #83404, #91498, #22061, #42851 ),
 .UNSPECIFIED., .F., .F.,
 ( 4, 2, 2, 2, 2, 2, 2, 2, 2, 2, 2, 2, 2, 2, 2, 2, 2, 2, 2, 2, 2, 2, 2, 2, 2, 4 ),
 ( 0.0007237080175806911249, 0.001215060144269388548, 0.001706412270958085863, 0.001952088334302373371, 0.002197764397646660879, 0.002320602429318732209, 0.002443440460990803538, 0.002566278492662874867, 0.002689116524334946197, 0.002934792587679060667, 0.003180468651023176004, 0.003671820777711521169, 0.004654525031088134306, 0.005637229284464748309, 0.006128581411153092608, 0.006374257474497301186, 0.006619933537841508897, 0.006681352553677620022, 0.006742771569513730280, 0.006804190585349841405, 0.006865609601185951663, 0.007111285664530410909, 0.007602637791219313788, 0.008093989917908217535, 0.008339665981252667240, 0.008585342044597118680 ),
 .UNSPECIFIED. ) ;
#5404=CARTESIAN_POINT ( 'NONE',  ( 157.7632566947985708, 282.3764601569879460, -1.694678876849560645 ) ) ;
#5405=CARTESIAN_POINT ( 'NONE',  ( 85.85769841670953895, 226.5024278399160664, -9.188101187500093303 ) ) ;
#5407=CARTESIAN_POINT ( 'NONE',  ( 190.8264243556038195, 300.1259329198319961, 8.466983560044813117 ) ) ;
#5408=CARTESIAN_POINT ( 'NONE',  ( 47.74604483422196921, 186.8262482093457777, 3.021315404115420679E-15 ) ) ;
#5409=CARTESIAN_POINT ( 'NONE',  ( 157.6673516573649181, 257.5591315650518141, 16.79781451397666103 ) ) ;
#5410=CARTESIAN_POINT ( 'NONE',  ( 152.4958592292019830, 266.5164192015877234, 16.46101990066986431 ) ) ;
#5411=CARTESIAN_POINT ( 'NONE',  ( 149.0651262117185354, 272.4586230950732784, 12.81403047969042319 ) ) ;
#5412=CARTESIAN_POINT ( 'NONE',  ( 199.2205425252482200, 285.5868937652708155, -18.05012564782189344 ) ) ;
#5415=CARTESIAN_POINT ( 'NONE',  ( 147.3236643320416022, 275.4749235501183193, -5.185334239426818037 ) ) ;
#5416=CARTESIAN_POINT ( 'NONE',  ( 176.8917175299031896, 289.5346434493817469, -10.53293604869262978 ) ) ;
#5417=ORIENTED_EDGE ( 'NONE', *, *, #92946, .F. ) ;
#5420=CARTESIAN_POINT ( 'NONE',  ( 147.3715240516018810, 275.3920280842035595, -3.728968767617475866 ) ) ;
#5421=CARTESIAN_POINT ( 'NONE',  ( 191.1350110915517462, 287.5662594520668449, -15.83302594719356371 ) ) ;
#5422=ORIENTED_EDGE ( 'NONE', *, *, #34996, .F. ) ;
#5425=CARTESIAN_POINT ( 'NONE',  ( 157.5967295993894481, 268.7214701990851609, 15.68487696739332193 ) ) ;
#5426=EDGE_CURVE ( 'NONE', #91683, #85466, #47798, .T. ) ;
#5428=CARTESIAN_POINT ( 'NONE',  ( 147.2464435575442110, 242.4865022471901455, 1.119607411625061291E-15 ) ) ;
#5430=VERTEX_POINT ( 'NONE', #64987 ) ;
#5431=CARTESIAN_POINT ( 'NONE',  ( 190.5496216836923224, 298.9665820173917155, -8.014846329333149555 ) ) ;
#5433=CARTESIAN_POINT ( 'NONE',  ( 196.7937303734090904, 265.3195474433538266, -4.517652853299265026 ) ) ;
#5435=EDGE_CURVE ( 'NONE', #79763, #15038, #57746, .T. ) ;
#5437=CARTESIAN_POINT ( 'NONE',  ( 181.8097039409798299, 290.8543075322054392, -10.92870535220637684 ) ) ;
#5438=ORIENTED_EDGE ( 'NONE', *, *, #93934, .F. ) ;
#5439=CARTESIAN_POINT ( 'NONE',  ( 41.59134429584264581, 201.4865022471903160, 10.00000000000009415 ) ) ;
#5441=CARTESIAN_POINT ( 'NONE',  ( 157.6621077668482087, 257.9721149867314125, -16.69158026131348294 ) ) ;
#5449=VERTEX_POINT ( 'NONE', #50269 ) ;
#5453=CARTESIAN_POINT ( 'NONE',  ( 162.4144876147732077, 272.5436428348735944, -16.23799951425711185 ) ) ;
#5454=CYLINDRICAL_SURFACE ( 'NONE', #82197, 10.00000000000010658 ) ;
#5456=AXIS2_PLACEMENT_3D ( 'NONE', #15973, #45855, #54449 ) ;
#5459=CARTESIAN_POINT ( 'NONE',  ( 167.5902884827328023, 286.2268049185996688, -4.744512013060059097 ) ) ;
#5463=CARTESIAN_POINT ( 'NONE',  ( 98.52331994705694740, 233.8149278399160949, -9.188101187500095079 ) ) ;
#5465=CARTESIAN_POINT ( 'NONE',  ( 148.5272680744187141, 275.3902207161408455, -7.185975151065171929 ) ) ;
#5466=CARTESIAN_POINT ( 'NONE',  ( 191.7774707643941667, 275.0877732711670092, 16.73782656324233642 ) ) ;
#5470=CARTESIAN_POINT ( 'NONE',  ( 196.5452668095620368, 286.2544686769650752, -17.73926526098317069 ) ) ;
#5471=CARTESIAN_POINT ( 'NONE',  ( 157.5042325173297684, 257.8416622032797818, 16.70595240278738203 ) ) ;
#5473=EDGE_CURVE ( 'NONE', #99839, #36195, #16670, .T. ) ;
#5477=VERTEX_POINT ( 'NONE', #12795 ) ;
#5482=CARTESIAN_POINT ( 'NONE',  ( 153.3409266555433703, 265.4419702791891496, 16.17400560137409116 ) ) ;
#5484=CARTESIAN_POINT ( 'NONE',  ( 139.7681268980558968, 245.3768266524160140, -9.188101187500091527 ) ) ;
#5485=CARTESIAN_POINT ( 'NONE',  ( 199.2082368456953532, 284.5671209592410946, 17.30778797021233828 ) ) ;
#5491=CARTESIAN_POINT ( 'NONE',  ( 172.9708666340684999, 251.4732952470851615, -0.2584728925942609279 ) ) ;
#5495=DIRECTION ( 'NONE',  ( 0.4999999999999992784, -0.8660254037844390407, 0.000000000000000000 ) ) ;
#5499=CARTESIAN_POINT ( 'NONE',  ( 61.44712799118319424, 194.0327760586659451, 1.948934522072303157E-15 ) ) ;
#5500=CARTESIAN_POINT ( 'NONE',  ( 206.3454060440500086, 273.2462681537123785, -9.268083217908118954 ) ) ;
#5502=CARTESIAN_POINT ( 'NONE',  ( 208.3226489551340990, 269.8215829728092103, -1.240262689467544366 ) ) ;
#5507=CARTESIAN_POINT ( 'NONE',  ( 79.94359230559648211, 205.4155109091896065, 2.679491924311254714 ) ) ;
#5511=CARTESIAN_POINT ( 'NONE',  ( 157.6831565925140239, 270.7739412695440819, -15.91244755415583612 ) ) ;
#5514=CARTESIAN_POINT ( 'NONE',  ( 24.99226373304320958, 194.4244531367911293, -4.594050593750046652 ) ) ;
#5515=CARTESIAN_POINT ( 'NONE',  ( 196.0727848089514964, 291.0389700598140621, 17.56388901715066808 ) ) ;
#5516=VECTOR ( 'NONE', #51919, 1000.000000000000000 ) ;
#5520=CARTESIAN_POINT ( 'NONE',  ( 53.16558651961199899, 195.3768266524160140, 9.188101187500096856 ) ) ;
#5523=CARTESIAN_POINT ( 'NONE',  ( 199.0756812798354645, 285.8378008023734083, -18.45377816087746936 ) ) ;
#5524=CARTESIAN_POINT ( 'NONE',  ( 196.9098758191317700, 289.5890858996224324, -16.54412079817003800 ) ) ;
#5526=CARTESIAN_POINT ( 'NONE',  ( 202.9510194980842641, 270.0555581978532587, -6.495183321546498689 ) ) ;
#5527=CARTESIAN_POINT ( 'NONE',  ( 174.9787010148468767, 292.1454046610912769, 2.108760379847960387 ) ) ;
#5528=CARTESIAN_POINT ( 'NONE',  ( 179.7724920804510873, 276.7831429704333459, 16.31391713246987862 ) ) ;
#5531=B_SPLINE_SURFACE_WITH_KNOTS ( 'NONE', 3, 1, ( 
 ( #48658, #79591 ),
 ( #74350, #10155 ),
 ( #88205, #63344 ),
 ( #78562, #33968 ),
 ( #64853, #24837 ),
 ( #4938, #40022 ),
 ( #41021, #70962 ),
 ( #41531, #1563 ),
 ( #49153, #71959 ),
 ( #80088, #33446 ),
 ( #55711, #17235 ),
 ( #48142, #64343 ),
 ( #79086, #95307 ),
 ( #40529, #71464 ),
 ( #10655, #29712 ),
 ( #51513, #60588 ),
 ( #91544, #75334 ),
 ( #91057, #5917 ),
 ( #53498, #29225 ),
 ( #37794, #84452 ),
 ( #98135, #28720 ),
 ( #67211, #22112 ),
 ( #53005, #83956 ),
 ( #90571, #43904 ),
 ( #68697, #99628 ),
 ( #36806, #45881 ),
 ( #97646, #36306 ),
 ( #13532, #37302 ),
 ( #82479, #60093 ),
 ( #22612, #75838 ),
 ( #13043, #14993 ),
 ( #21622, #59594 ),
 ( #67718, #44898 ),
 ( #38291, #21139 ) ),
 .UNSPECIFIED., .T., .F., .F.,
 ( 4, 2, 2, 2, 2, 2, 2, 2, 2, 2, 2, 2, 2, 2, 2, 2, 4 ),
 ( 2, 2 ),
 ( 0.000000000000000000, 0.06250000000000000000, 0.1250000000000000000, 0.1875000000000000000, 0.2500000000000000000, 0.3125000000000000000, 0.3750000000000000000, 0.4375000000000000000, 0.5000000000000000000, 0.5625000000000000000, 0.6250000000000000000, 0.6875000000000000000, 0.7500000000000000000, 0.8125000000000000000, 0.8750000000000000000, 0.9375000000000000000, 1.000000000000000000 ),
 ( 0.000000000000000000, 1.000000000000000000 ),
 .UNSPECIFIED. ) ;
#5532=CARTESIAN_POINT ( 'NONE',  ( 163.2883354864554519, 256.0504063331084694, -14.91619366091854282 ) ) ;
#5534=CARTESIAN_POINT ( 'NONE',  ( 90.16093569141993669, 222.8615022471902591, -10.00000000000009592 ) ) ;
#5535=CARTESIAN_POINT ( 'NONE',  ( 184.6894110187365641, 293.7322318964822330, -10.88359728165448814 ) ) ;
#5536=CARTESIAN_POINT ( 'NONE',  ( 163.5869523275859763, 268.7237500424058680, -16.42576965565886482 ) ) ;
#5538=CARTESIAN_POINT ( 'NONE',  ( 59.90443346675090908, 196.2048013555409796, 4.594050593750051981 ) ) ;
#5539=ORIENTED_EDGE ( 'NONE', *, *, #75864, .F. ) ;
#5541=CARTESIAN_POINT ( 'NONE',  ( 147.0538900202505488, 275.9421863647172017, 5.192507380313251986 ) ) ;
#5547=CARTESIAN_POINT ( 'NONE',  ( 186.3306027636789679, 263.0363486839914913, 11.47262423782134277 ) ) ;
#5549=CARTESIAN_POINT ( 'NONE',  ( 205.0722772166587902, 275.4513919673344731, 14.18415804594472185 ) ) ;
#5554=CARTESIAN_POINT ( 'NONE',  ( 7.816353548249534100, 181.9865022471903160, 10.00000000000009415 ) ) ;
#5556=CARTESIAN_POINT ( 'NONE',  ( 181.5631808996132008, 283.6781476641766631, 14.96027398286517496 ) ) ;
#5557=CARTESIAN_POINT ( 'NONE',  ( 167.6885389621171782, 262.0286974587709210, 16.15245462749480154 ) ) ;
#5558=CARTESIAN_POINT ( 'NONE',  ( 206.4484807199597753, 273.0677375780628608, -9.220527398138528952 ) ) ;
#5560=CARTESIAN_POINT ( 'NONE',  ( 162.1541172097854826, 283.1473020987244809, -3.122785026967457966 ) ) ;
#5562=CARTESIAN_POINT ( 'NONE',  ( 181.7882433779857081, 293.0516533115879270, -9.677455024747617429 ) ) ;
#5564=CARTESIAN_POINT ( 'NONE',  ( 159.8416255366773839, 253.7931787365127434, 16.77980437810719394 ) ) ;
#5565=CARTESIAN_POINT ( 'NONE',  ( -22.42236680055709641, 157.8615022471902591, 0.000000000000000000 ) ) ;
#5566=CARTESIAN_POINT ( 'NONE',  ( -22.42236680055709641, 157.8615022471902591, 0.000000000000000000 ) ) ;
#5567=CARTESIAN_POINT ( 'NONE',  ( 118.5230073417626073, 248.4244531367911293, -4.594050593750046652 ) ) ;
#5570=CARTESIAN_POINT ( 'NONE',  ( 173.3549678798564742, 265.3355617639286379, 16.05511268515816781 ) ) ;
#5576=CARTESIAN_POINT ( 'NONE',  ( 159.7897726928491409, 253.8829904965402875, 16.83923858130328810 ) ) ;
#5578=CARTESIAN_POINT ( 'NONE',  ( 68.04987750350953490, 222.3464784336661637, 1.353441290958777525E-15 ) ) ;
#5579=CARTESIAN_POINT ( 'NONE',  ( 16.74724052122864393, 187.1427522451419350, 10.00000000000009415 ) ) ;
#5581=CARTESIAN_POINT ( 'NONE',  ( 155.6126298223767890, 261.1180141786725244, 18.15400560664037855 ) ) ;
#5583=CARTESIAN_POINT ( 'NONE',  ( 171.9941656342203089, 276.8346263436580443, 16.42768944293989719 ) ) ;
#5586=EDGE_CURVE ( 'NONE', #88849, #19800, #34782, .T. ) ;
#5588=CARTESIAN_POINT ( 'NONE',  ( 152.8328714238065515, 265.9326969577624027, -16.29536156676786263 ) ) ;
#5589=CARTESIAN_POINT ( 'NONE',  ( 155.1865148098964937, 261.8560670301561686, -16.99758927948949605 ) ) ;
#5594=CARTESIAN_POINT ( 'NONE',  ( 174.2386054419784784, 253.2136311291264690, -7.745944249412784366 ) ) ;
#5596=CARTESIAN_POINT ( 'NONE',  ( 174.8696466734779449, 292.3029143586743430, -1.153856708368909967 ) ) ;
#5601=CARTESIAN_POINT ( 'NONE',  ( 164.4963285489318991, 245.7309966251440301, -6.672251175510283794 ) ) ;
#5602=CARTESIAN_POINT ( 'NONE',  ( 147.5084024922618084, 243.7202760586659736, -5.415160957724236172E-17 ) ) ;
#5603=ORIENTED_EDGE ( 'NONE', *, *, #97462, .T. ) ;
#5605=CARTESIAN_POINT ( 'NONE',  ( 182.0573489978566215, 257.5803797228366534, 6.639334650236212276 ) ) ;
#5611=CARTESIAN_POINT ( 'NONE',  ( 182.4299782848027291, 275.0440474321702595, -17.09684782076308807 ) ) ;
#5612=CARTESIAN_POINT ( 'NONE',  ( 167.5444266783159435, 249.1640122146770011, -5.486574941136140637 ) ) ;
#5615=CARTESIAN_POINT ( 'NONE',  ( 198.3653284636346541, 266.1659536649856932, 0.8111552996551663064 ) ) ;
#5616=CARTESIAN_POINT ( 'NONE',  ( 147.5492216329511166, 275.0842468449245644, 4.751613690710122739 ) ) ;
#5617=CARTESIAN_POINT ( 'NONE',  ( 182.8710648154623186, 280.6231348432476125, 16.78699077144874252 ) ) ;
#5622=CARTESIAN_POINT ( 'NONE',  ( 178.7600897929267774, 254.1784503161647706, 4.743017227330367014 ) ) ;
#5623=CARTESIAN_POINT ( 'NONE',  ( 159.6978881494930249, 254.0421391940632532, 15.34888828951022610 ) ) ;
#5625=CARTESIAN_POINT ( 'NONE',  ( 135.5370584069941060, 262.3927522451419350, 2.944929066748280225E-16 ) ) ;
#5626=B_SPLINE_CURVE_WITH_KNOTS ( 'NONE', 3,
 ( #52457, #82913, #257, #99574 ),
 .UNSPECIFIED., .F., .F.,
 ( 4, 4 ),
 ( 0.008863162062248396492, 0.01509767807619737633 ),
 .UNSPECIFIED. ) ;
#5627=CARTESIAN_POINT ( 'NONE',  ( 174.4421927399967842, 284.4761513374891706, -12.08263559617888916 ) ) ;
#5628=ORIENTED_EDGE ( 'NONE', *, *, #46192, .F. ) ;
#5630=CARTESIAN_POINT ( 'NONE',  ( 150.6386650955079176, 269.7331738006648720, -15.06054658539322766 ) ) ;
#5631=CARTESIAN_POINT ( 'NONE',  ( 3.531332017333847606, 172.8458772461660828, 9.188101187500095079 ) ) ;
#5633=CARTESIAN_POINT ( 'NONE',  ( 178.5281950170523544, 259.0983513684005288, -10.32239201220430225 ) ) ;
#5636=CARTESIAN_POINT ( 'NONE',  ( 204.7242223814549504, 276.0542406257275161, -13.93608974681376189 ) ) ;
#5639=CARTESIAN_POINT ( 'NONE',  ( 196.2956918591910664, 269.5555983294441376, -10.79850100103040944 ) ) ;
#5640=CARTESIAN_POINT ( 'NONE',  ( 66.11068853694163749, 215.6427522451419065, 10.00000000000009237 ) ) ;
#5642=CARTESIAN_POINT ( 'NONE',  ( 150.8613910702043768, 269.3474010963252567, 15.19517615056406612 ) ) ;
#5645=CARTESIAN_POINT ( 'NONE',  ( 179.5028650301413791, 294.0833190536570214, 1.038326004487517551 ) ) ;
#5646=CARTESIAN_POINT ( 'NONE',  ( 63.38631695775107033, 200.7365022471902023, 10.00000000000009592 ) ) ;
#5648=CARTESIAN_POINT ( 'NONE',  ( 181.7815785431583038, 276.1505370498239813, -17.81783396216490445 ) ) ;
#5649=CARTESIAN_POINT ( 'NONE',  ( 17.27983239817682559, 168.5327760586659736, 1.948934522072303157E-15 ) ) ;
#5650=CARTESIAN_POINT ( 'NONE',  ( 164.2838888460686064, 285.0926974262010276, 4.322335904415723462 ) ) ;
#5651=EDGE_CURVE ( 'NONE', #82532, #52858, #64690, .T. ) ;
#5652=CARTESIAN_POINT ( 'NONE',  ( 11.42479273068475010, 170.7365022471902307, 10.00000000000009948 ) ) ;
#5654=CARTESIAN_POINT ( 'NONE',  ( 201.9062777989876452, 280.4778359209939254, -15.96862433567465622 ) ) ;
#5655=CARTESIAN_POINT ( 'NONE',  ( 206.9408877595175511, 272.2148635675444552, 6.707071080545934372 ) ) ;
#5656=CARTESIAN_POINT ( 'NONE',  ( 193.9401685343300699, 294.7327698005063326, 14.01047396938887069 ) ) ;
#5657=CARTESIAN_POINT ( 'NONE',  ( 188.3428823685774489, 267.3304898084075489, 14.27533445868386508 ) ) ;
#5662=CARTESIAN_POINT ( 'NONE',  ( 165.2720705891711930, 285.9514678962245853, -0.2691863636319293818 ) ) ;
#5665=CARTESIAN_POINT ( 'NONE',  ( 194.3562588153086779, 294.0120802933159325, 14.11474987148825200 ) ) ;
#5670=CARTESIAN_POINT ( 'NONE',  ( 155.5995420464182644, 262.6346450740109617, -17.48312782858739567 ) ) ;
#5671=VERTEX_POINT ( 'NONE', #47143 ) ;
#5673=CARTESIAN_POINT ( 'NONE',  ( 71.10837680816226225, 221.8615022471903160, 5.000000000000046185 ) ) ;
#5675=CARTESIAN_POINT ( 'NONE',  ( 202.9881971861223917, 279.0611244672630278, -15.16231470264511927 ) ) ;
#5679=CARTESIAN_POINT ( 'NONE',  ( 204.5831314780710954, 276.2986172388744421, 13.28075685133257089 ) ) ;
#5680=CARTESIAN_POINT ( 'NONE',  ( 192.5712965840290849, 297.1037255674836501, 11.03742858512898906 ) ) ;
#5682=CARTESIAN_POINT ( 'NONE',  ( 190.9061255863007318, 299.9878863388391892, 7.497146773253707153 ) ) ;
#5686=CARTESIAN_POINT ( 'NONE',  ( 149.6890529486499872, 271.3779502865075983, -12.51465682618088593 ) ) ;
#5689=CARTESIAN_POINT ( 'NONE',  ( 164.3493441216711517, 245.9855811210807417, 1.722120810491653664 ) ) ;
#5692=ADVANCED_FACE ( 'NONE', ( #8655 ), #44410, .F. ) ;
#5693=CARTESIAN_POINT ( 'NONE',  ( 174.6178695879432041, 276.7332269073218072, -16.18563341224413676 ) ) ;
#5694=CARTESIAN_POINT ( 'NONE',  ( 172.3630404188492662, 263.8283741867592198, -15.51507169348583304 ) ) ;
#5696=CARTESIAN_POINT ( 'NONE',  ( 161.4666507344003605, 276.8280471058072294, -12.69379384225013219 ) ) ;
#5698=CARTESIAN_POINT ( 'NONE',  ( 192.8301672656986341, 296.6553483942417415, -13.40355799340913556 ) ) ;
#5701=B_SPLINE_CURVE_WITH_KNOTS ( 'NONE', 3,
 ( #47796, #16410, #93957, #78231 ),
 .UNSPECIFIED., .F., .F.,
 ( 4, 4 ),
 ( 0.01771268258920854696, 0.02667042995983895728 ),
 .UNSPECIFIED. ) ;
#5703=CARTESIAN_POINT ( 'NONE',  ( 190.5653282632609091, 300.5781646174276602, -5.775635208185608604 ) ) ;
#5705=FACE_OUTER_BOUND ( 'NONE', #26331, .T. ) ;
#5706=CARTESIAN_POINT ( 'NONE',  ( 192.1883190596398094, 297.7670620978826150, 12.41391288785556668 ) ) ;
#5708=CARTESIAN_POINT ( 'NONE',  ( 146.6344723850759522, 276.6686390184297579, -0.5903044561608344898 ) ) ;
#5709=EDGE_CURVE ( 'NONE', #38470, #53225, #43211, .T. ) ;
#5710=CARTESIAN_POINT ( 'NONE',  ( 191.3413020738616410, 299.2341385521244774, -8.295023558158421295 ) ) ;
#5711=ORIENTED_EDGE ( 'NONE', *, *, #4513, .T. ) ;
#5713=CARTESIAN_POINT ( 'NONE',  ( 164.9171241593586217, 245.0021572482830550, 1.622680932994367220 ) ) ;
#5714=CARTESIAN_POINT ( 'NONE',  ( 206.5117639185820906, 272.9581278627833285, 11.28485531511759099 ) ) ;
#5716=CARTESIAN_POINT ( 'NONE',  ( 171.4584946453171597, 288.7452855169624399, 4.212295942657065417 ) ) ;
#5717=CARTESIAN_POINT ( 'NONE',  ( 203.9648368022151601, 269.0477214045654364, 5.644613064108824574 ) ) ;
#5718=CARTESIAN_POINT ( 'NONE',  ( 99.22679203974932705, 240.3464784336661637, 1.353441290958777327E-15 ) ) ;
#5719=VERTEX_POINT ( 'NONE', #42534 ) ;
#5720=CARTESIAN_POINT ( 'NONE',  ( 149.1807793072240997, 272.2583060576048979, -11.58584517200773867 ) ) ;
#5724=CARTESIAN_POINT ( 'NONE',  ( 179.5668846297247683, 282.8373499615596529, -15.68793421486103945 ) ) ;
#5726=VERTEX_POINT ( 'NONE', #88716 ) ;
#5727=CARTESIAN_POINT ( 'NONE',  ( 163.4055107321044318, 247.6203485056908846, -10.24153090796238530 ) ) ;
#5729=CARTESIAN_POINT ( 'NONE',  ( 164.6460902696047128, 245.4716017159096566, -3.036414139157908476 ) ) ;
#5730=CARTESIAN_POINT ( 'NONE',  ( 55.79055247517715799, 193.0177522451417929, 5.000000000000051514 ) ) ;
#5731=CARTESIAN_POINT ( 'NONE',  ( 118.6048046409561465, 227.0327760586659451, 1.948934522072302763E-15 ) ) ;
#5733=CARTESIAN_POINT ( 'NONE',  ( 151.3898985249405200, 268.4319993325432847, -14.65018536945715510 ) ) ;
#5735=DIRECTION ( 'NONE',  ( -0.8660254037844387076, -0.4999999999999998890, -0.000000000000000000 ) ) ;
#5737=CARTESIAN_POINT ( 'NONE',  ( 27.26558041797736465, 195.7369531367911293, -4.594050593750048428 ) ) ;
#5739=B_SPLINE_CURVE_WITH_KNOTS ( 'NONE', 3,
 ( #55637, #78480, #94696, #3486 ),
 .UNSPECIFIED., .F., .F.,
 ( 4, 4 ),
 ( 0.008210304326597597790, 0.01330689658320593181 ),
 .UNSPECIFIED. ) ;
#5741=B_SPLINE_CURVE_WITH_KNOTS ( 'NONE', 3,
 ( #22597, #70178, #292, #91043 ),
 .UNSPECIFIED., .F., .F.,
 ( 4, 4 ),
 ( 0.01080220131554398416, 0.01688746497888054740 ),
 .UNSPECIFIED. ) ;
#5746=CARTESIAN_POINT ( 'NONE',  ( -22.42236680055709641, 157.8615022471902591, 0.000000000000000000 ) ) ;
#5747=CARTESIAN_POINT ( 'NONE',  ( 179.0788045520370702, 287.9706957157609963, -12.84865443290734888 ) ) ;
#5748=CARTESIAN_POINT ( 'NONE',  ( 182.0889153921933143, 262.8220885373254418, 12.61422020207666073 ) ) ;
#5749=CARTESIAN_POINT ( 'NONE',  ( 95.19470834736908671, 225.7677522451418497, 10.00000000000009592 ) ) ;
#5750=EDGE_LOOP ( 'NONE', ( #75965, #64656, #12072, #53852 ) ) ;
#5751=CARTESIAN_POINT ( 'NONE',  ( 198.6608371149412733, 267.8789152959208195, -8.090336142662009067 ) ) ;
#5752=CARTESIAN_POINT ( 'NONE',  ( 155.4640109849479472, 279.7078215382471171, -1.643371934387127808 ) ) ;
#5753=CARTESIAN_POINT ( 'NONE',  ( 155.0568450317760494, 264.0806616740677555, 17.52241723436104337 ) ) ;
#5754=AXIS2_PLACEMENT_3D ( 'NONE', #66039, #73164, #88407 ) ;
#5756=CARTESIAN_POINT ( 'NONE',  ( 12.78715206816254302, 172.0643266524160140, -9.188101187500093303 ) ) ;
#5758=CARTESIAN_POINT ( 'NONE',  ( 195.8612935349768520, 273.6653920451291242, 14.68105839524987744 ) ) ;
#5761=CARTESIAN_POINT ( 'NONE',  ( 52.86797706100236383, 192.1423013555410080, -4.594050593750043987 ) ) ;
#5763=CARTESIAN_POINT ( 'NONE',  ( 207.5290616128274337, 271.1961165699281651, 2.604679844609484984 ) ) ;
#5766=CARTESIAN_POINT ( 'NONE',  ( 165.0532575723395041, 244.7663672603923715, -2.144843157699870773 ) ) ;
#5767=ORIENTED_EDGE ( 'NONE', *, *, #1944, .F. ) ;
#5769=CARTESIAN_POINT ( 'NONE',  ( 15.61058218230948036, 186.4865022471903160, 10.00000000000009237 ) ) ;
#5770=CARTESIAN_POINT ( 'NONE',  ( 208.3057440179679531, 269.8508631828800617, 2.969924427282375046 ) ) ;
#5771=CARTESIAN_POINT ( 'NONE',  ( 138.6044920356617922, 241.6423013555409796, -4.594050593750043987 ) ) ;
#5773=CARTESIAN_POINT ( 'NONE',  ( 164.3075360873267527, 246.0579947607303097, 1.438421213066341187 ) ) ;
#5774=EDGE_CURVE ( 'NONE', #37486, #92061, #84354, .T. ) ;
#5777=CARTESIAN_POINT ( 'NONE',  ( 157.6286460899086137, 257.6261715744221306, 18.25526781158026779 ) ) ;
#5778=CARTESIAN_POINT ( 'NONE',  ( 185.9978760885800853, 288.1611571412556714, 14.69368409826119404 ) ) ;
#5781=CARTESIAN_POINT ( 'NONE',  ( 150.8888667059421209, 269.2998118992572927, 15.79021133717968617 ) ) ;
#5782=CARTESIAN_POINT ( 'NONE',  ( 208.2011561505922828, 270.0320146830300132, -1.742225264168492771 ) ) ;
#5783=CARTESIAN_POINT ( 'NONE',  ( 181.6780919045320672, 288.0220715738037711, 13.83910407665415931 ) ) ;
#5784=CARTESIAN_POINT ( 'NONE',  ( 170.4610070438220930, 266.6194390815376210, -16.58348635212187361 ) ) ;
#5785=CARTESIAN_POINT ( 'NONE',  ( 197.2730491841539617, 273.3678195921213501, -13.56865045505698575 ) ) ;
#5792=CARTESIAN_POINT ( 'NONE',  ( 200.7867161642997758, 282.5082135784035131, -16.60672201385608204 ) ) ;
#5793=CARTESIAN_POINT ( 'NONE',  ( 196.2709069678370497, 270.8137320491818514, 13.18132365197871358 ) ) ;
#5794=VECTOR ( 'NONE', #58198, 1000.000000000000000 ) ;
#5795=DIRECTION ( 'NONE',  ( -0.4999999999999987788, 0.8660254037844392627, 0.000000000000000000 ) ) ;
#5796=CARTESIAN_POINT ( 'NONE',  ( 208.3829315663354862, 269.7171704273955015, -1.768817828503133072 ) ) ;
#5798=( BOUNDED_CURVE ( )  B_SPLINE_CURVE ( 2, ( #26099, #87472, #25597, #19014, #2308, #57983, #12400, #88455, #42271 ),
 .UNSPECIFIED., .F., .T. ) 
 B_SPLINE_CURVE_WITH_KNOTS ( ( 3, 2, 2, 2, 3 ),
 ( 0.3266129032258064391, 0.3279569892473118142, 0.3306451612903225645, 0.3333333333333333148, 0.3346774193548386900 ),
 .UNSPECIFIED. ) 
 CURVE ( )  GEOMETRIC_REPRESENTATION_ITEM ( )  RATIONAL_B_SPLINE_CURVE ( ( 0.9330127018922194093, 0.9330127018922194093, 1.000000000000000000, 0.8660254037844387076, 1.000000000000000000, 0.8660254037844387076, 1.000000000000000000, 0.9330127018922194093, 0.9330127018922194093 ) ) 
 REPRESENTATION_ITEM ( '' )  );
#5802=CARTESIAN_POINT ( 'NONE',  ( 85.23541620384800410, 230.0177522451419350, 5.000000000000046185 ) ) ;
#5809=CARTESIAN_POINT ( 'NONE',  ( 205.8889072768004951, 273.5716727396786041, -9.812782715980612025 ) ) ;
#5810=CARTESIAN_POINT ( 'NONE',  ( 204.2133777088835700, 276.9390495533970693, 13.75768580338462144 ) ) ;
#5811=CARTESIAN_POINT ( 'NONE',  ( 58.13834967963523326, 192.8262482093458061, 3.021315404115420679E-15 ) ) ;
#5813=CARTESIAN_POINT ( 'NONE',  ( 90.35072584248885619, 210.7202760586659167, -5.415160957724236172E-17 ) ) ;
#5814=CARTESIAN_POINT ( 'NONE',  ( 203.4046850588284485, 278.3397463110001695, 14.99647135965170897 ) ) ;
#5815=CARTESIAN_POINT ( 'NONE',  ( 177.8917589780327546, 269.0032800508485593, -16.65457745387491073 ) ) ;
#5817=ORIENTED_EDGE ( 'NONE', *, *, #73326, .F. ) ;
#5818=ADVANCED_FACE ( 'NONE', ( #68831 ), #30341, .T. ) ;
#5824=CARTESIAN_POINT ( 'NONE',  ( 173.4026771546767804, 273.2456497557084845, -17.70700034978624515 ) ) ;
#5828=B_SPLINE_CURVE_WITH_KNOTS ( 'NONE', 3,
 ( #16096, #71316, #39868, #1413 ),
 .UNSPECIFIED., .F., .F.,
 ( 4, 4 ),
 ( 0.008174317677677851723, 0.01411586822901593832 ),
 .UNSPECIFIED. ) ;
#5833=CARTESIAN_POINT ( 'NONE',  ( 164.7649989079121156, 265.0053717114169558, -16.62870243764915656 ) ) ;
#5834=ORIENTED_EDGE ( 'NONE', *, *, #9246, .F. ) ;
#5841=FACE_OUTER_BOUND ( 'NONE', #91048, .T. ) ;
#5843=ADVANCED_FACE ( 'NONE', ( #15623 ), #91676, .T. ) ;
#5845=CARTESIAN_POINT ( 'NONE',  ( 202.2773826701151165, 280.2922913237452462, 16.62862787739668846 ) ) ;
#5847=CARTESIAN_POINT ( 'NONE',  ( 188.0130000780826265, 260.6906737763359274, 2.852620083407500395 ) ) ;
#5848=CARTESIAN_POINT ( 'NONE',  ( 161.0174131639706161, 281.2532803613611918, -6.597337978638083911 ) ) ;
#5852=CARTESIAN_POINT ( 'NONE',  ( 168.4162858537046645, 252.9027699456641187, 12.03307035579989126 ) ) ;
#5853=CARTESIAN_POINT ( 'NONE',  ( 158.1077839419051827, 281.0782939731791998, 2.063989399413418191 ) ) ;
#5855=CARTESIAN_POINT ( 'NONE',  ( 155.3935616475962149, 261.4974513877137952, -18.59422973016237890 ) ) ;
#5858=CARTESIAN_POINT ( 'NONE',  ( 160.6427889144519554, 275.7530518071173447, 12.78665216319188858 ) ) ;
#5859=CARTESIAN_POINT ( 'NONE',  ( -7.429302001086912632, 166.5177522451418781, -10.00000000000009592 ) ) ;
#5860=CARTESIAN_POINT ( 'NONE',  ( 196.1510318622376872, 269.5623502998935805, -10.89412449686265560 ) ) ;
#5862=CARTESIAN_POINT ( 'NONE',  ( 169.3092427493755281, 280.4792478331783059, -14.38416588291234000 ) ) ;
#5864=CARTESIAN_POINT ( 'NONE',  ( 160.8606767143015759, 272.6466877113235228, 15.42252470312289248 ) ) ;
#5865=CARTESIAN_POINT ( 'NONE',  ( 0.1486806056246424423, 161.7048013555410080, 4.594050593750051981 ) ) ;
#5867=CARTESIAN_POINT ( 'NONE',  ( 185.0971745880719936, 295.3200165845683500, 8.402215535322445916 ) ) ;
#5877=CARTESIAN_POINT ( 'NONE',  ( 153.2507058676394536, 279.2988129818712650, 3.890835714306057458 ) ) ;
#5878=CARTESIAN_POINT ( 'NONE',  ( 17.11727908708474288, 174.5643266524160424, 9.188101187500095079 ) ) ;
#5879=CARTESIAN_POINT ( 'NONE',  ( 120.0931990297694085, 230.9548013555409796, -4.594050593750042211 ) ) ;
#5881=CARTESIAN_POINT ( 'NONE',  ( 183.1420952819525780, 257.7645371039402562, -2.611028994885449261 ) ) ;
#5882=CARTESIAN_POINT ( 'NONE',  ( 206.2084181172874651, 271.6286034143743677, -8.104356745948360086 ) ) ;
#5883=CARTESIAN_POINT ( 'NONE',  ( 178.5070354113733231, 283.8968948738306608, -14.91322718153175053 ) ) ;
#5885=CARTESIAN_POINT ( 'NONE',  ( 166.2015897840689149, 251.7888940817747425, -12.22707897765162599 ) ) ;
#5886=CARTESIAN_POINT ( 'NONE',  ( 183.8863552858182118, 275.0393761356287996, 16.36257040815191388 ) ) ;
#5887=CARTESIAN_POINT ( 'NONE',  ( 147.7785919239399846, 274.6869658471848652, -7.924750738206837397 ) ) ;
#5890=CARTESIAN_POINT ( 'NONE',  ( 196.3622566498499111, 266.7229801469659947, 8.086874854287275483 ) ) ;
#5891=CARTESIAN_POINT ( 'NONE',  ( -22.42236680055709641, 157.8615022471902591, 0.000000000000000000 ) ) ;
#5892=CARTESIAN_POINT ( 'NONE',  ( 183.6708288585361686, 268.4310204149097103, -15.04327638771743381 ) ) ;
#5894=CARTESIAN_POINT ( 'NONE',  ( 174.0300771628572818, 264.6284561815462553, -15.49364447767913866 ) ) ;
#5895=CARTESIAN_POINT ( 'NONE',  ( 96.25000326212280299, 232.5024278399160664, -9.188101187500093303 ) ) ;
#5898=CARTESIAN_POINT ( 'NONE',  ( 157.5520850189458884, 257.7587792392113215, 16.71892742266126319 ) ) ;
#5899=CARTESIAN_POINT ( 'NONE',  ( 152.3887669668241074, 266.7019084411238623, 16.79563195480379534 ) ) ;
#5900=CARTESIAN_POINT ( 'NONE',  ( 201.3105023133114173, 270.3128416713978481, -10.18795719577549796 ) ) ;
#5901=CARTESIAN_POINT ( 'NONE',  ( 198.8533049117289977, 286.2229679703367538, -18.60939981449148561 ) ) ;
#5903=AXIS2_PLACEMENT_3D ( 'NONE', #2724, #63500, #26020 ) ;
#5911=CARTESIAN_POINT ( 'NONE',  ( 193.1169444172380167, 296.1586357973259283, -13.13373377033755318 ) ) ;
#5917=CARTESIAN_POINT ( 'NONE',  ( 159.7608930362198407, 253.9330115291272421, 15.38895778945778581 ) ) ;
#5918=CARTESIAN_POINT ( 'NONE',  ( 154.3836164983932804, 267.1724063083494229, 16.08677479740975969 ) ) ;
#5920=CARTESIAN_POINT ( 'NONE',  ( 140.3904091109174317, 241.8615022471902023, 5.000000000000051514 ) ) ;
#5921=EDGE_LOOP ( 'NONE', ( #85265, #71901, #35711, #55489 ) ) ;
#5922=CARTESIAN_POINT ( 'NONE',  ( 190.4606495512497304, 299.4734402352337383, -6.528258444144710460 ) ) ;
#5924=CARTESIAN_POINT ( 'NONE',  ( 197.0096825693687776, 265.1139848888072379, -4.595851537931033626 ) ) ;
#5927=CARTESIAN_POINT ( 'NONE',  ( 185.2453734934235570, 292.5319340899530971, -10.69469963830730919 ) ) ;
#5930=CARTESIAN_POINT ( 'NONE',  ( 205.8843284829576987, 274.0448779157541708, 10.73475218247099683 ) ) ;
#5932=CARTESIAN_POINT ( 'NONE',  ( 204.1793134244172734, 273.0455815889928886, 10.99258542199709154 ) ) ;
#5936=AXIS2_PLACEMENT_3D ( 'NONE', #79896, #94094, #78876 ) ;
#5938=B_SPLINE_CURVE_WITH_KNOTS ( 'NONE', 3,
 ( #23528, #76747, #53922, #24540 ),
 .UNSPECIFIED., .F., .F.,
 ( 4, 4 ),
 ( 0.000000000000000000, 0.003871553614270288081 ),
 .UNSPECIFIED. ) ;
#5940=CARTESIAN_POINT ( 'NONE',  ( 73.72680694775513643, 201.8262482093457777, 3.021315404115420679E-15 ) ) ;
#5945=EDGE_CURVE ( 'NONE', #60977, #25883, #2151, .T. ) ;
#5946=CARTESIAN_POINT ( 'NONE',  ( 174.4157552818196848, 257.3257494145293549, -11.97941750818477757 ) ) ;
#5947=CARTESIAN_POINT ( 'NONE',  ( 165.4717973444044503, 273.8037661123966586, -15.20093003926469066 ) ) ;
#5948=CARTESIAN_POINT ( 'NONE',  ( 206.6829130365991034, 272.6616888947074244, -10.15488415123734001 ) ) ;
#5952=CARTESIAN_POINT ( 'NONE',  ( 167.0625938901047789, 286.3493216121294154, -4.853271414194278321 ) ) ;
#5954=EDGE_CURVE ( 'NONE', #31208, #97695, #66196, .T. ) ;
#5955=CARTESIAN_POINT ( 'NONE',  ( 178.1108306389469647, 255.4780320608604995, 4.908464522874967706 ) ) ;
#5956=EDGE_CURVE ( 'NONE', #44657, #62092, #20388, .T. ) ;
#5957=CARTESIAN_POINT ( 'NONE',  ( 109.7816501962546454, 240.3149278399160949, 9.188101187500093303 ) ) ;
#5959=CARTESIAN_POINT ( 'NONE',  ( 148.1162654905123190, 275.3898513388497804, -5.688393309263520159 ) ) ;
#5961=CARTESIAN_POINT ( 'NONE',  ( 191.9772060522040533, 275.3178886761277226, 16.43916042812731249 ) ) ;
#5964=EDGE_CURVE ( 'NONE', #51310, #49046, #25092, .T. ) ;
#5966=CARTESIAN_POINT ( 'NONE',  ( 164.3720776498103646, 249.6648944244760173, 9.933307626539082946 ) ) ;
#5967=CARTESIAN_POINT ( 'NONE',  ( 206.1408608592916494, 273.6005508061571732, -10.42739367433323494 ) ) ;
#5968=CARTESIAN_POINT ( 'NONE',  ( 97.22551825371941447, 215.3932355074535394, -2.679491924311248496 ) ) ;
#5971=CARTESIAN_POINT ( 'NONE',  ( 199.7327534409123189, 266.0852835921289170, -4.070366225034659280 ) ) ;
#5973=CARTESIAN_POINT ( 'NONE',  ( 191.4684674121631076, 263.6719838314244271, -8.116905096791009910 ) ) ;
#5974=CARTESIAN_POINT ( 'NONE',  ( 174.1019790828183034, 269.4634721183348915, -17.75005378496514297 ) ) ;
#5979=DIRECTION ( 'NONE',  ( -0.8660254037844387076, -0.4999999999999998890, -0.000000000000000000 ) ) ;
#5982=CARTESIAN_POINT ( 'NONE',  ( 147.4317198359019301, 275.2877659273946733, 3.797273160043843188 ) ) ;
#5983=CARTESIAN_POINT ( 'NONE',  ( 52.03546399666511491, 212.3967562850347122, -4.648177544792955347E-16 ) ) ;
#5985=CARTESIAN_POINT ( 'NONE',  ( 172.1240434037265743, 250.9065000376095043, -0.2557444706756556996 ) ) ;
#5986=CARTESIAN_POINT ( 'NONE',  ( 189.3359066111170534, 270.2222636373566047, -14.08322114487687848 ) ) ;
#5990=CARTESIAN_POINT ( 'NONE',  ( -22.42236680055709641, 157.8615022471902591, 0.000000000000000000 ) ) ;
#5993=CARTESIAN_POINT ( 'NONE',  ( 75.14063404487711750, 220.3149278399160664, -9.188101187500095079 ) ) ;
#5994=CARTESIAN_POINT ( 'NONE',  ( 159.2536436069973718, 254.8115933126508992, -15.76697951715411250 ) ) ;
#5995=CARTESIAN_POINT ( 'NONE',  ( 197.0121621852902933, 287.4119207165142029, 17.64812647472269092 ) ) ;
#5998=CARTESIAN_POINT ( 'NONE',  ( 197.3665944960539491, 288.3056451486161222, -16.78855881086668234 ) ) ;
#5999=CARTESIAN_POINT ( 'NONE',  ( 161.2977680094314223, 251.2710659906439616, -13.03191437619249982 ) ) ;
#6001=CIRCLE ( 'NONE', #59342, 17.82106496071138935 ) ;
#6008=CARTESIAN_POINT ( 'NONE',  ( 20.90579313287664576, 189.0024278399160949, -9.188101187500093303 ) ) ;
#6009=CARTESIAN_POINT ( 'NONE',  ( 157.8763546842245376, 257.1971277035954699, 17.68444922773363004 ) ) ;
#6014=CARTESIAN_POINT ( 'NONE',  ( 45.88512659934279014, 206.4869531367911009, 4.594050593750046652 ) ) ;
#6016=CARTESIAN_POINT ( 'NONE',  ( 170.7424494536428483, 287.6183357598478665, 7.193943569343137057 ) ) ;
#6017=CARTESIAN_POINT ( 'NONE',  ( -17.99656830608997993, 171.9637435831424739, 2.679491924311252049 ) ) ;
#6019=CARTESIAN_POINT ( 'NONE',  ( 203.1504851873393136, 269.7283529643794395, -7.434428718697961180 ) ) ;
#6020=CARTESIAN_POINT ( 'NONE',  ( 175.6726996453791685, 291.0189004104380501, 2.504403466513535736 ) ) ;
#6021=ORIENTED_EDGE ( 'NONE', *, *, #63552, .F. ) ;
#6022=CARTESIAN_POINT ( 'NONE',  ( 157.1614910081131882, 264.8482722167576071, 17.59091970785239667 ) ) ;
#6024=CARTESIAN_POINT ( 'NONE',  ( 163.4107516284163637, 256.1401433533470708, -14.91842279323626030 ) ) ;
#6025=EDGE_CURVE ( 'NONE', #63549, #77820, #88730, .T. ) ;
#6028=CARTESIAN_POINT ( 'NONE',  ( 101.8522786425099156, 219.6115022471901739, -5.000000000000041744 ) ) ;
#6029=CARTESIAN_POINT ( 'NONE',  ( -22.42236680055709641, 157.8615022471902591, 0.000000000000000000 ) ) ;
#6030=CARTESIAN_POINT ( 'NONE',  ( 165.1531489442545535, 269.9894434971714077, -16.29722773533296731 ) ) ;
#6032=CARTESIAN_POINT ( 'NONE',  ( 61.44712799118319424, 194.0327760586659451, 1.948934522072303157E-15 ) ) ;
#6034=CARTESIAN_POINT ( 'NONE',  ( 166.1405104867327793, 265.3397484891177101, 16.55385694601057978 ) ) ;
#6035=B_SPLINE_CURVE_WITH_KNOTS ( 'NONE', 3,
 ( #88827, #49760, #81205, #65453 ),
 .UNSPECIFIED., .F., .F.,
 ( 4, 4 ),
 ( 0.006807249740348602328, 0.01254308171105925247 ),
 .UNSPECIFIED. ) ;
#6036=CARTESIAN_POINT ( 'NONE',  ( 147.1199024702499969, 275.8278494473859723, 5.224467159276165340 ) ) ;
#6041=CARTESIAN_POINT ( 'NONE',  ( 157.8444045675000496, 264.5910462210627543, -17.67892232388873097 ) ) ;
#6042=CARTESIAN_POINT ( 'NONE',  ( 175.3129199032210295, 273.6512861356621329, -16.42196374976860440 ) ) ;
#6045=VERTEX_POINT ( 'NONE', #54617 ) ;
#6046=AXIS2_PLACEMENT_3D ( 'NONE', #26463, #11765, #65940 ) ;
#6058=CARTESIAN_POINT ( 'NONE',  ( 159.3180704616806906, 282.3194142970525604, -3.259201431328204723 ) ) ;
#6059=DIRECTION ( 'NONE',  ( -0.8660254037844387076, -0.4999999999999998890, -0.000000000000000000 ) ) ;
#6060=CARTESIAN_POINT ( 'NONE',  ( 207.7837159184916231, 270.7550423741513441, -2.369602332675663448 ) ) ;
#6061=CARTESIAN_POINT ( 'NONE',  ( 163.8147431267737204, 246.9115372060205118, 7.125417796469586840 ) ) ;
#6062=CARTESIAN_POINT ( 'NONE',  ( 159.6898930778639283, 254.0559870643349143, 16.90891900388599822 ) ) ;
#6064=CARTESIAN_POINT ( 'NONE',  ( 164.4177597422757060, 265.5742877017660817, -16.83945066787966383 ) ) ;
#6065=CARTESIAN_POINT ( 'NONE',  ( 128.8345561752773278, 239.0643266524160424, 9.188101187500095079 ) ) ;
#6066=CARTESIAN_POINT ( 'NONE',  ( 73.32782722540972031, 203.9548013555409796, -4.594050593750042211 ) ) ;
#6068=CARTESIAN_POINT ( 'NONE',  ( 170.3588773579726308, 263.8410958083132982, 15.88277590726158017 ) ) ;
#6073=B_SPLINE_CURVE_WITH_KNOTS ( 'NONE', 3,
 ( #81995, #12568, #4968, #74386 ),
 .UNSPECIFIED., .F., .F.,
 ( 4, 4 ),
 ( 0.006379106832508525497, 0.01446904724182691837 ),
 .UNSPECIFIED. ) ;
#6074=CARTESIAN_POINT ( 'NONE',  ( 160.6481820402849792, 253.1006006086905984, 14.59193497169809284 ) ) ;
#6076=VERTEX_POINT ( 'NONE', #11062 ) ;
#6080=CARTESIAN_POINT ( 'NONE',  ( 191.8210230231139803, 298.4032374945642232, -8.800268167321144475 ) ) ;
#6082=CARTESIAN_POINT ( 'NONE',  ( 155.0197698005585494, 262.1448778582381465, 18.42918111182112284 ) ) ;
#6087=CARTESIAN_POINT ( 'NONE',  ( 200.8251833487811666, 282.8075743310126882, -16.74393672780000131 ) ) ;
#6088=CARTESIAN_POINT ( 'NONE',  ( 201.0740630776729745, 282.3765019955979483, -17.86148837378524590 ) ) ;
#6089=ORIENTED_EDGE ( 'NONE', *, *, #6261, .T. ) ;
#6092=CARTESIAN_POINT ( 'NONE',  ( 174.1320578672132626, 253.2284290848832313, -7.713315856054966169 ) ) ;
#6093=EDGE_CURVE ( 'NONE', #11051, #69971, #88085, .T. ) ;
#6094=CARTESIAN_POINT ( 'NONE',  ( 164.9617201910520237, 244.9249146555742414, 2.745022583679548767 ) ) ;
#6095=CARTESIAN_POINT ( 'NONE',  ( 47.63001943043753528, 186.7592609112380160, 2.679491924311254714 ) ) ;
#6096=CARTESIAN_POINT ( 'NONE',  ( 159.3282873775263795, 259.5781396707945987, 16.68337382483777276 ) ) ;
#6097=CARTESIAN_POINT ( 'NONE',  ( 138.6852480475602931, 257.0024278399161517, 9.188101187500095079 ) ) ;
#6098=ORIENTED_EDGE ( 'NONE', *, *, #36457, .F. ) ;
#6102=( BOUNDED_CURVE ( )  B_SPLINE_CURVE ( 2, ( #69220, #7419, #31214, #93048, #30733, #23604, #39296, #24617, #821 ),
 .UNSPECIFIED., .F., .F. ) 
 B_SPLINE_CURVE_WITH_KNOTS ( ( 3, 2, 2, 2, 3 ),
 ( 0.7943548387096773800, 0.7956989247311827551, 0.7983870967741935054, 0.8010752688172042557, 0.8024193548387096309 ),
 .UNSPECIFIED. ) 
 CURVE ( )  GEOMETRIC_REPRESENTATION_ITEM ( )  RATIONAL_B_SPLINE_CURVE ( ( 0.9330127018922194093, 0.9330127018922194093, 1.000000000000000000, 0.8660254037844387076, 1.000000000000000000, 0.8660254037844387076, 1.000000000000000000, 0.9330127018922194093, 0.9330127018922194093 ) ) 
 REPRESENTATION_ITEM ( '' )  );
#6107=CARTESIAN_POINT ( 'NONE',  ( 184.0420290590031414, 276.8802109191442469, -16.58438063308576105 ) ) ;
#6112=CARTESIAN_POINT ( 'NONE',  ( 196.3062046258999658, 264.8785121205631299, 0.8257428584848626185 ) ) ;
#6113=CARTESIAN_POINT ( 'NONE',  ( 190.9498149295421570, 299.9122141765958531, -5.138500224925297566 ) ) ;
#6114=CARTESIAN_POINT ( 'NONE',  ( 186.7005128325694727, 282.3869391950191812, 16.28400853260290759 ) ) ;
#6116=CARTESIAN_POINT ( 'NONE',  ( 196.6791268423878307, 270.0974108068855344, 11.84491577176450861 ) ) ;
#6117=B_SPLINE_SURFACE_WITH_KNOTS ( 'NONE', 3, 1, ( 
 ( #29536, #92369 ),
 ( #21928, #51848 ),
 ( #84768, #44219 ),
 ( #60909, #60409 ),
 ( #45710, #91365 ),
 ( #59921, #36620 ),
 ( #99449, #7726 ),
 ( #30025, #38615 ),
 ( #91874, #69016 ),
 ( #22429, #76634 ),
 ( #30529, #5733 ),
 ( #7219, #53803 ),
 ( #15304, #69521 ),
 ( #59411, #90391 ),
 ( #82789, #13354 ),
 ( #75156, #67529 ),
 ( #86285, #1650 ),
 ( #78141, #47219 ),
 ( #8728, #93872 ),
 ( #71547, #2142 ),
 ( #40108, #63429 ),
 ( #16821, #92858 ),
 ( #8234, #23918 ),
 ( #39600, #61909 ),
 ( #17322, #33024 ),
 ( #54302, #55305 ),
 ( #55796, #47708 ),
 ( #24921, #70520 ),
 ( #9753, #23412 ),
 ( #62922, #39101 ),
 ( #56314, #17843 ),
 ( #40613, #86788 ),
 ( #78646, #54816 ),
 ( #79676, #1135 ) ),
 .UNSPECIFIED., .T., .F., .F.,
 ( 4, 2, 2, 2, 2, 2, 2, 2, 2, 2, 2, 2, 2, 2, 2, 2, 4 ),
 ( 2, 2 ),
 ( 0.000000000000000000, 0.06250000000000000000, 0.1250000000000000000, 0.1875000000000000000, 0.2500000000000000000, 0.3125000000000000000, 0.3750000000000000000, 0.4375000000000000000, 0.5000000000000000000, 0.5625000000000000000, 0.6250000000000000000, 0.6875000000000000000, 0.7500000000000000000, 0.8125000000000000000, 0.8750000000000000000, 0.9375000000000000000, 1.000000000000000000 ),
 ( 0.000000000000000000, 1.000000000000000000 ),
 .UNSPECIFIED. ) ;
#6120=CARTESIAN_POINT ( 'NONE',  ( 205.4948664586259497, 274.1576266782160474, 10.82119204727489326 ) ) ;
#6122=CARTESIAN_POINT ( 'NONE',  ( 198.3075590527773784, 287.1682275260610027, 16.94807365630277118 ) ) ;
#6123=CARTESIAN_POINT ( 'NONE',  ( 161.6043392661310065, 250.7400689978998685, 14.26332272462310691 ) ) ;
#6125=CARTESIAN_POINT ( 'NONE',  ( -1.691623377417284635, 160.6423013555410080, -4.594050593750043987 ) ) ;
#6126=CARTESIAN_POINT ( 'NONE',  ( 175.4155855648062357, 286.4771596746830937, -12.38400456956481577 ) ) ;
#6129=CARTESIAN_POINT ( 'NONE',  ( 177.9714937548455680, 255.7189482022137383, 8.882064279750110813 ) ) ;
#6131=CARTESIAN_POINT ( 'NONE',  ( 199.1867231605587278, 285.6454706231928071, -17.41989184023605475 ) ) ;
#6132=CARTESIAN_POINT ( 'NONE',  ( 4.830370123010505168, 173.5958772461660828, -9.188101187500095079 ) ) ;
#6133=CARTESIAN_POINT ( 'NONE',  ( 181.9452575149977065, 275.8400803543989355, -16.44639771376654735 ) ) ;
#6138=CARTESIAN_POINT ( 'NONE',  ( 171.3928239984006723, 250.3015599828365509, -5.796133048607560845 ) ) ;
#6139=B_SPLINE_SURFACE_WITH_KNOTS ( 'NONE', 3, 1, ( 
 ( #40049, #32476 ),
 ( #94312, #79113 ),
 ( #12175, #19301 ),
 ( #26379, #74494 ),
 ( #43036, #89235 ),
 ( #26876, #96815 ),
 ( #57755, #50653 ),
 ( #81120, #88731 ),
 ( #57257, #90207 ),
 ( #27864, #59231 ),
 ( #18783, #73980 ),
 ( #19785, #4564 ),
 ( #41558, #64880 ),
 ( #49662, #49181 ),
 ( #34954, #12688 ),
 ( #33996, #80117 ),
 ( #66365, #88232 ),
 ( #95826, #11687 ),
 ( #80619, #73480 ),
 ( #35953, #20277 ),
 ( #28354, #81605 ),
 ( #11194, #35460 ),
 ( #3107, #50168 ),
 ( #10679, #42547 ),
 ( #97297, #43555 ),
 ( #5072, #65854 ),
 ( #58743, #51151 ),
 ( #89716, #82115 ),
 ( #4064, #27372 ),
 ( #58257, #66855 ),
 ( #97784, #72501 ),
 ( #42063, #72997 ),
 ( #3587, #34468 ),
 ( #65366, #96308 ) ),
 .UNSPECIFIED., .T., .F., .F.,
 ( 4, 2, 2, 2, 2, 2, 2, 2, 2, 2, 2, 2, 2, 2, 2, 2, 4 ),
 ( 2, 2 ),
 ( 0.000000000000000000, 0.06250000000000000000, 0.1250000000000000000, 0.1875000000000000000, 0.2500000000000000000, 0.3125000000000000000, 0.3750000000000000000, 0.4375000000000000000, 0.5000000000000000000, 0.5625000000000000000, 0.6250000000000000000, 0.6875000000000000000, 0.7500000000000000000, 0.8125000000000000000, 0.8750000000000000000, 0.9375000000000000000, 1.000000000000000000 ),
 ( 0.000000000000000000, 1.000000000000000000 ),
 .UNSPECIFIED. ) ;
#6140=CARTESIAN_POINT ( 'NONE',  ( 177.5863610073459427, 254.6759042037001848, -3.887113448368675339 ) ) ;
#6141=CARTESIAN_POINT ( 'NONE',  ( 150.8360166798673561, 269.3913508296000145, 13.81437070545826806 ) ) ;
#6142=EDGE_CURVE ( 'NONE', #67236, #17408, #46923, .T. ) ;
#6143=EDGE_CURVE ( 'NONE', #2866, #32378, #15387, .T. ) ;
#6144=CARTESIAN_POINT ( 'NONE',  ( 57.68498304950345812, 214.1115022471903444, -5.000000000000047962 ) ) ;
#6146=CIRCLE ( 'NONE', #51428, 2.471954595299370006 ) ;
#6147=CARTESIAN_POINT ( 'NONE',  ( 148.0427192501136062, 274.2294838985851015, 9.385226820296049155 ) ) ;
#6149=CARTESIAN_POINT ( 'NONE',  ( 12.62459875707045143, 178.0958772461660544, -9.188101187500095079 ) ) ;
#6150=CARTESIAN_POINT ( 'NONE',  ( 168.1939926483296972, 286.2578356360547218, 4.106630047314361320 ) ) ;
#6155=CARTESIAN_POINT ( 'NONE',  ( 207.6826438088389750, 270.9301044032979462, 7.252082088659585146 ) ) ;
#6156=CARTESIAN_POINT ( 'NONE',  ( 185.3916143550522122, 266.4269361941668990, 14.53728910407776098 ) ) ;
#6158=CARTESIAN_POINT ( 'NONE',  ( 164.1824377412969511, 281.5202305190522338, 9.046750956103593921 ) ) ;
#6160=CARTESIAN_POINT ( 'NONE',  ( 148.4016473149517594, 273.6078022540229426, 8.470066617688926769 ) ) ;
#6162=CARTESIAN_POINT ( 'NONE',  ( 186.8624879592976811, 268.0158595129609580, -15.20275046462360713 ) ) ;
#6164=CARTESIAN_POINT ( 'NONE',  ( 185.3078095671113772, 290.9215328420979176, 12.16701217945218083 ) ) ;
#6165=CARTESIAN_POINT ( 'NONE',  ( 177.5636530406916620, 258.7959717445368142, 12.62758304280528066 ) ) ;
#6168=VERTEX_POINT ( 'NONE', #12054 ) ;
#6172=CARTESIAN_POINT ( 'NONE',  ( 155.6328838216860220, 261.0829332228125850, -17.51014940606912518 ) ) ;
#6174=ORIENTED_EDGE ( 'NONE', *, *, #21173, .T. ) ;
#6175=CARTESIAN_POINT ( 'NONE',  ( 186.7746357155629084, 272.1319419735754082, -16.70060704968626553 ) ) ;
#6176=CARTESIAN_POINT ( 'NONE',  ( 170.8054577101068219, 287.4915981561377976, 8.526299399445241178 ) ) ;
#6185=CARTESIAN_POINT ( 'NONE',  ( 149.6191398986701415, 271.4990432411842676, -11.66821883946526839 ) ) ;
#6188=CARTESIAN_POINT ( 'NONE',  ( 164.5348324038273518, 245.6643059921780718, 1.473102934610569958 ) ) ;
#6189=AXIS2_PLACEMENT_3D ( 'NONE', #64785, #95731, #79524 ) ;
#6190=CARTESIAN_POINT ( 'NONE',  ( 150.1462219700033813, 275.7016199270512402, -8.305148579817409171 ) ) ;
#6192=CARTESIAN_POINT ( 'NONE',  ( 190.2935937139882299, 301.0488226629397559, 4.649863831023156813 ) ) ;
#6193=CARTESIAN_POINT ( 'NONE',  ( 172.2407488011533871, 263.6222815918252422, -15.46399472876365344 ) ) ;
#6195=CARTESIAN_POINT ( 'NONE',  ( 158.6969344861375077, 274.7767743472534221, -13.28740588576491533 ) ) ;
#6197=CARTESIAN_POINT ( 'NONE',  ( 164.9280325499431115, 267.7146836723554202, 17.76834957580831187 ) ) ;
#6203=CARTESIAN_POINT ( 'NONE',  ( 147.5177358149801421, 275.1387818813681179, 4.867883209065928085 ) ) ;
#6205=CARTESIAN_POINT ( 'NONE',  ( 192.7507137768506880, 296.7929658737652971, 11.30364540927242345 ) ) ;
#6206=CARTESIAN_POINT ( 'NONE',  ( 191.3292802282752803, 299.2549609994807724, 8.303257185644898897 ) ) ;
#6207=CARTESIAN_POINT ( 'NONE',  ( 191.1747001918821525, 299.5227014763493116, -9.654804683100723040 ) ) ;
#6210=ADVANCED_FACE ( 'NONE', ( #42906 ), #83287, .F. ) ;
#6211=CARTESIAN_POINT ( 'NONE',  ( 167.0957737472305666, 246.8272050136007749, 1.963998143010642128 ) ) ;
#6213=CARTESIAN_POINT ( 'NONE',  ( 171.4797962540974652, 288.7824835811317143, 4.217883281193715028 ) ) ;
#6216=CARTESIAN_POINT ( 'NONE',  ( 149.7298672153112591, 271.3072579029764029, -11.96904942057522270 ) ) ;
#6218=CARTESIAN_POINT ( 'NONE',  ( 202.7749754141538006, 277.6906214767087704, 15.33344055037920128 ) ) ;
#6220=CARTESIAN_POINT ( 'NONE',  ( 180.9602365206295929, 283.3372604617935622, -15.11549797918817895 ) ) ;
#6221=CARTESIAN_POINT ( 'NONE',  ( 147.9312304387540564, 274.4225881843351544, -9.820174179285407590 ) ) ;
#6222=VERTEX_POINT ( 'NONE', #84469 ) ;
#6223=CARTESIAN_POINT ( 'NONE',  ( 163.3473224498206093, 247.7211335670114352, -10.00320358166632850 ) ) ;
#6224=CARTESIAN_POINT ( 'NONE',  ( 205.7544487159363769, 273.3880016642347073, 10.04406142612960728 ) ) ;
#6227=EDGE_CURVE ( 'NONE', #48184, #31958, #42076, .T. ) ;
#6228=CARTESIAN_POINT ( 'NONE',  ( 40.12992642340848448, 200.6427522451419065, 10.00000000000009237 ) ) ;
#6229=CARTESIAN_POINT ( 'NONE',  ( 117.8466853168797428, 238.8458772461660544, 9.188101187500095079 ) ) ;
#6230=CARTESIAN_POINT ( 'NONE',  ( 180.5626108788783313, 294.4595582549500250, -3.477258678576252482 ) ) ;
#6231=CARTESIAN_POINT ( 'NONE',  ( 193.9979983253333842, 262.2552985615510579, -0.8131695963413709816 ) ) ;
#6232=CARTESIAN_POINT ( 'NONE',  ( 104.4503548538632316, 221.1115022471901739, -5.000000000000041744 ) ) ;
#6233=CARTESIAN_POINT ( 'NONE',  ( 175.4310824030733613, 253.5328469009434684, -3.918382160889689381 ) ) ;
#6234=B_SPLINE_CURVE_WITH_KNOTS ( 'NONE', 3,
 ( #71408, #32884, #39967, #24297, #38479, #23278, #23784, #1998, #69393, #69884, #39463, #78006, #47086, #31877, #16691, #78510, #47582, #63787, #92728, #79024, #25285, #84631, #8598, #85132, #9, #16194 ),
 .UNSPECIFIED., .F., .F.,
 ( 4, 2, 2, 2, 2, 2, 2, 2, 2, 2, 2, 2, 4 ),
 ( 0.003565812906164105359, 0.003712674125762171519, 0.003786104735561204599, 0.003859535345360237679, 0.004006396564958202358, 0.004153257784556166170, 0.004446980223752116344, 0.004740702662948066519, 0.005915592419731927065, 0.007090482176515788479, 0.007677927054907681889, 0.007971649494103592165, 0.008265371933299504176 ),
 .UNSPECIFIED. ) ;
#6235=CARTESIAN_POINT ( 'NONE',  ( 25.10051690851626560, 194.4869531367911293, 4.594050593750046652 ) ) ;
#6237=CARTESIAN_POINT ( 'NONE',  ( 147.7638709860940764, 275.5540662940547350, -3.738940778976949098 ) ) ;
#6240=CARTESIAN_POINT ( 'NONE',  ( 181.2586407163293813, 267.7608388338027225, 14.99160397322970972 ) ) ;
#6241=CYLINDRICAL_SURFACE ( 'NONE', #14161, 10.00000000000010658 ) ;
#6242=CARTESIAN_POINT ( 'NONE',  ( 146.8058449195592061, 276.3718130816831149, 4.181814292810413392 ) ) ;
#6244=DIRECTION ( 'NONE',  ( 0.4999999999999992784, -0.8660254037844390407, 0.000000000000000000 ) ) ;
#6245=CARTESIAN_POINT ( 'NONE',  ( 176.6906187182376300, 285.7386481342455795, -12.05608563264864763 ) ) ;
#6246=CARTESIAN_POINT ( 'NONE',  ( 203.3286960320409094, 267.8359400968079171, 2.569349860321338941 ) ) ;
#6247=CARTESIAN_POINT ( 'NONE',  ( 104.2158063034569579, 237.6427522451419065, -10.00000000000009415 ) ) ;
#6252=CARTESIAN_POINT ( 'NONE',  ( 202.2576150004249200, 280.3265299319959354, 16.24828394350762295 ) ) ;
#6255=CARTESIAN_POINT ( 'NONE',  ( 4.640666744108908226, 182.6744531367911577, 4.594050593750047540 ) ) ;
#6258=CARTESIAN_POINT ( 'NONE',  ( 192.1966557276483911, 272.1854317587748255, 14.40833446829215347 ) ) ;
#6261=EDGE_CURVE ( 'NONE', #33698, #27127, #94044, .T. ) ;
#6262=CARTESIAN_POINT ( 'NONE',  ( 198.1602621822531773, 277.2937910998977600, -15.34043159284401092 ) ) ;
#6263=CARTESIAN_POINT ( 'NONE',  ( 48.02338713675939630, 198.5333772461660828, 9.188101187500095079 ) ) ;
#6267=CARTESIAN_POINT ( 'NONE',  ( 207.3502731283117555, 271.5057873089173768, 6.280625384230454245 ) ) ;
#6270=CARTESIAN_POINT ( 'NONE',  ( 165.3402721949960892, 269.3030652250268417, 17.34759000155790432 ) ) ;
#6271=CARTESIAN_POINT ( 'NONE',  ( 5.723458822437122784, 184.1115022471903160, -5.000000000000047962 ) ) ;
#6272=CARTESIAN_POINT ( 'NONE',  ( 163.7012083107868534, 247.1081852757374975, -6.544933039329257518 ) ) ;
#6273=CARTESIAN_POINT ( 'NONE',  ( 138.9560545341254851, 251.0333772461660260, 9.188101187500095079 ) ) ;
#6281=CARTESIAN_POINT ( 'NONE',  ( 170.0812506307862009, 258.7503018971702318, -15.45556229382616031 ) ) ;
#6282=ORIENTED_EDGE ( 'NONE', *, *, #46472, .T. ) ;
#6283=B_SPLINE_CURVE_WITH_KNOTS ( 'NONE', 3,
 ( #49577, #19704, #58660, #74409, #12089, #4480, #73396, #89632, #67269, #5482, #66285, #3507, #27787, #57667, #72916, #50570, #3982, #18695, #80530, #27291 ),
 .UNSPECIFIED., .F., .F.,
 ( 4, 2, 2, 2, 2, 2, 2, 2, 2, 4 ),
 ( 3.403994264753323137E-15, 0.0003780139803775907554, 0.0007560279607517774413, 0.001134041941125964181, 0.001512055921500150921, 0.001701062911687225643, 0.001890069901874300799, 0.002268083882248450676, 0.002646097862622600987, 0.003024111842996750864 ),
 .UNSPECIFIED. ) ;
#6284=CARTESIAN_POINT ( 'NONE',  ( 154.1583213311439238, 272.3229918181682478, 14.15140380722988667 ) ) ;
#6285=CARTESIAN_POINT ( 'NONE',  ( 189.9686529740312153, 299.6116365339944423, 6.575253125843024016 ) ) ;
#6287=CARTESIAN_POINT ( 'NONE',  ( 169.7674466671218738, 266.1787835990222106, -16.83623305646149149 ) ) ;
#6290=ORIENTED_EDGE ( 'NONE', *, *, #14645, .F. ) ;
#6295=CARTESIAN_POINT ( 'NONE',  ( 148.8368245119552284, 273.2444610639298617, -9.231145687738527172 ) ) ;
#6296=CARTESIAN_POINT ( 'NONE',  ( 32.04156216231763210, 177.7592609112380444, 2.679491924311254714 ) ) ;
#6299=CARTESIAN_POINT ( 'NONE',  ( 153.3506059258413643, 265.0359544954067132, -16.39100908615009899 ) ) ;
#6300=CARTESIAN_POINT ( 'NONE',  ( 195.4625579292164161, 281.9119700028093689, -17.76036160681684350 ) ) ;
#6304=CARTESIAN_POINT ( 'NONE',  ( 190.4249800432324662, 300.8212548652687133, 3.085047376053959400 ) ) ;
#6306=CARTESIAN_POINT ( 'NONE',  ( 189.1071431715656104, 297.0811097836661361, 8.130666790968703594 ) ) ;
#6307=B_SPLINE_CURVE_WITH_KNOTS ( 'NONE', 3,
 ( #62557, #76781, #53960, #93007 ),
 .UNSPECIFIED., .F., .F.,
 ( 4, 4 ),
 ( 0.04511453035517336979, 0.04887066958154941826 ),
 .UNSPECIFIED. ) ;
#6311=CARTESIAN_POINT ( 'NONE',  ( 163.7707306762541748, 246.9877690064858484, 7.021959502997312086 ) ) ;
#6315=CARTESIAN_POINT ( 'NONE',  ( 91.91987624320061911, 230.0024278399160949, 9.188101187500095079 ) ) ;
#6317=CARTESIAN_POINT ( 'NONE',  ( 178.0062659503225859, 269.1087611653143199, -16.50835682451741349 ) ) ;
#6319=B_SPLINE_CURVE_WITH_KNOTS ( 'NONE', 3,
 ( #68142, #82422, #29164, #59029 ),
 .UNSPECIFIED., .F., .F.,
 ( 4, 4 ),
 ( 0.008739769553074294359, 0.01698173572311750812 ),
 .UNSPECIFIED. ) ;
#6323=CARTESIAN_POINT ( 'NONE',  ( 160.6734846709049691, 282.6943762970620924, -6.583290857611773461 ) ) ;
#6325=CARTESIAN_POINT ( 'NONE',  ( 151.1998204792857052, 278.0139405208182097, -4.510343437356565843 ) ) ;
#6328=CARTESIAN_POINT ( 'NONE',  ( 207.9622466093905189, 270.4458181468041289, 3.586592550214158681 ) ) ;
#6330=CARTESIAN_POINT ( 'NONE',  ( 153.1627746953036535, 265.3612877299463548, -17.72069958822647351 ) ) ;
#6335=ORIENTED_EDGE ( 'NONE', *, *, #69634, .T. ) ;
#6336=DIRECTION ( 'NONE',  ( 0.4999999999999992784, -0.8660254037844390407, 0.000000000000000000 ) ) ;
#6341=CARTESIAN_POINT ( 'NONE',  ( 164.0584767703456066, 281.7763263192914565, 8.638174457797754613 ) ) ;
#6344=CARTESIAN_POINT ( 'NONE',  ( 177.5337925685473408, 280.1858537220425092, 16.79564202278857721 ) ) ;
#6345=VERTEX_POINT ( 'NONE', #70718 ) ;
#6346=CARTESIAN_POINT ( 'NONE',  ( 163.3543347837650686, 247.7089878483399730, 10.92686688779373405 ) ) ;
#6348=CARTESIAN_POINT ( 'NONE',  ( 185.0156182622852441, 258.0389674772235935, 3.001315489709461382 ) ) ;
#6349=CARTESIAN_POINT ( 'NONE',  ( 159.2202160840655552, 280.3973568208431288, -6.670942047025803845 ) ) ;
#6352=CARTESIAN_POINT ( 'NONE',  ( 169.5542383065973695, 254.4246916622037133, 11.34482188162280636 ) ) ;
#6356=CARTESIAN_POINT ( 'NONE',  ( 181.6129181475825760, 270.8901633951155077, -15.97990793206353821 ) ) ;
#6358=CARTESIAN_POINT ( 'NONE',  ( 193.7547917776226427, 294.1291474128820482, -14.15125599393966205 ) ) ;
#6360=CARTESIAN_POINT ( 'NONE',  ( -3.532187684056978583, 178.7677522451419350, -5.000000000000047962 ) ) ;
#6362=B_SPLINE_CURVE_WITH_KNOTS ( 'NONE', 3,
 ( #90244, #43590, #21304, #52674, #52180, #20816, #5594, #6092, #23640, #46959, #83129, #51708, #60268, #77879, #74525, #13215, #54531, #13700, #44074, #14197, #36483, #45083, #77368, #7973, #85512, #39828, #88028, #49456, #71781, #41346, #64160, #78884, #33260, #63657, #9976, #48969, #17052, #32753, #17560, #47943, #2891, #3389, #24161, #72288, #72799, #10469, #64672, #55536, #79904, #33787, #95110, #70759 ),
 .UNSPECIFIED., .F., .F.,
 ( 4, 2, 2, 2, 2, 2, 2, 2, 2, 2, 2, 2, 2, 2, 2, 2, 2, 2, 2, 2, 2, 2, 2, 2, 2, 4 ),
 ( 0.0004385394321953336636, 0.0008914911018940902855, 0.001117966936743468569, 0.001344442771592846853, 0.001457680689017575894, 0.001570918606442304718, 0.001684156523867033758, 0.001797394441291762799, 0.002023870276141257959, 0.002250346110990753771, 0.003156249450389033220, 0.004062152789787312236, 0.004968056129185591252, 0.005421007798884741602, 0.005647483633734396574, 0.005760721551159234469, 0.005817340509871571884, 0.005873959468583910166, 0.005930578427296248449, 0.005987197386008586732, 0.006100435303433209520, 0.006326911138282458567, 0.006779862807980959263, 0.007232814477679459959, 0.007459290312528710741, 0.007685766147377961523 ),
 .UNSPECIFIED. ) ;
#6364=CARTESIAN_POINT ( 'NONE',  ( 203.4701571373468028, 278.2263453445292498, -15.29907731156314377 ) ) ;
#6367=CARTESIAN_POINT ( 'NONE',  ( 3.179769518870181777, 163.4548013555410080, -4.594050593750042211 ) ) ;
#6370=CARTESIAN_POINT ( 'NONE',  ( 185.9351731181741059, 295.4263767797440892, 8.222620372872301076 ) ) ;
#6371=ORIENTED_EDGE ( 'NONE', *, *, #34742, .F. ) ;
#6376=CARTESIAN_POINT ( 'NONE',  ( 172.1580654244187087, 289.4298437067981240, 2.621979037154522629 ) ) ;
#6378=CARTESIAN_POINT ( 'NONE',  ( 202.5254408350308495, 279.8626419788790827, -17.32378363213250694 ) ) ;
#6380=CARTESIAN_POINT ( 'NONE',  ( 150.5904159330389405, 276.7600202670964791, 3.696576208654118290 ) ) ;
#6381=CARTESIAN_POINT ( 'NONE',  ( 17.98330449086917682, 175.0643266524160140, -9.188101187500093303 ) ) ;
#6382=CARTESIAN_POINT ( 'NONE',  ( 118.6312605172356598, 248.4869531367911293, 4.594050593750046652 ) ) ;
#6383=CARTESIAN_POINT ( 'NONE',  ( 181.5281128488287834, 294.6324445685692126, -6.595065418016686110 ) ) ;
#6385=CARTESIAN_POINT ( 'NONE',  ( 206.6548133100257587, 272.3286174528128072, -7.213596576582502529 ) ) ;
#6387=CARTESIAN_POINT ( 'NONE',  ( 69.78333826775208593, 199.5494855054051868, -2.679491924311248496 ) ) ;
#6388=CARTESIAN_POINT ( 'NONE',  ( 193.8365934467825298, 294.9121671145370556, 14.14845633038902584 ) ) ;
#6389=CARTESIAN_POINT ( 'NONE',  ( 161.4143265314674522, 251.0691807084224365, -12.94469757303959234 ) ) ;
#6393=CARTESIAN_POINT ( 'NONE',  ( 164.8175787598647162, 249.8649966127220807, -10.54131631236613664 ) ) ;
#6394=CARTESIAN_POINT ( 'NONE',  ( 194.4774025889061591, 266.1532203706993869, 7.847259440529423813 ) ) ;
#6395=CARTESIAN_POINT ( 'NONE',  ( 55.54027346828191725, 191.3262482093457777, 3.021315404115420679E-15 ) ) ;
#6396=CARTESIAN_POINT ( 'NONE',  ( 66.18285732059042914, 199.0177522451417929, 5.000000000000051514 ) ) ;
#6398=( BOUNDED_CURVE ( )  B_SPLINE_CURVE ( 2, ( #77425, #1423, #86080, #9008, #16603, #25202, #33306, #64207, #93647 ),
 .UNSPECIFIED., .F., .T. ) 
 B_SPLINE_CURVE_WITH_KNOTS ( ( 3, 2, 2, 2, 3 ),
 ( 0.7137096774193548709, 0.7150537634408602461, 0.7177419354838709964, 0.7204301075268817467, 0.7217741935483871218 ),
 .UNSPECIFIED. ) 
 CURVE ( )  GEOMETRIC_REPRESENTATION_ITEM ( )  RATIONAL_B_SPLINE_CURVE ( ( 0.9330127018922194093, 0.9330127018922194093, 1.000000000000000000, 0.8660254037844387076, 1.000000000000000000, 0.8660254037844387076, 1.000000000000000000, 0.9330127018922194093, 0.9330127018922194093 ) ) 
 REPRESENTATION_ITEM ( '' )  );
#6399=CARTESIAN_POINT ( 'NONE',  ( 181.4945938287030742, 267.9359334561378887, 15.00701915070772507 ) ) ;
#6400=CARTESIAN_POINT ( 'NONE',  ( 95.57333414147498729, 235.1744531367911293, 4.594050593750047540 ) ) ;
#6403=CARTESIAN_POINT ( 'NONE',  ( 190.7851866479434761, 300.1973587246873194, 7.931162401707728016 ) ) ;
#6405=EDGE_CURVE ( 'NONE', #18290, #20047, #79522, .T. ) ;
#6409=CARTESIAN_POINT ( 'NONE',  ( 203.9678271304799750, 272.5810641093525533, -9.740920016785768354 ) ) ;
#6410=CARTESIAN_POINT ( 'NONE',  ( 150.6438662863770332, 269.7241650738195631, -14.92510732909997628 ) ) ;
#6413=CARTESIAN_POINT ( 'NONE',  ( 193.1569697810063531, 296.0893098336876506, -13.02398914535779539 ) ) ;
#6418=CARTESIAN_POINT ( 'NONE',  ( 154.8238461974347615, 274.8835241144952874, -12.48494116114558672 ) ) ;
#6419=CARTESIAN_POINT ( 'NONE',  ( 146.8868584395697781, 276.2314935489248455, -3.891417269505058396 ) ) ;
#6420=CARTESIAN_POINT ( 'NONE',  ( 65.81655290991075447, 197.2592609112379876, 2.679491924311254714 ) ) ;
#6423=VERTEX_POINT ( 'NONE', #43678 ) ;
#6425=CARTESIAN_POINT ( 'NONE',  ( 39.95181620016202118, 182.3262482093457493, 3.021315404115420679E-15 ) ) ;
#6426=CARTESIAN_POINT ( 'NONE',  ( 156.5742463479611786, 268.2652725409449204, 15.70701561319111406 ) ) ;
#6427=CARTESIAN_POINT ( 'NONE',  ( 173.2415407040283242, 253.7903840043475441, -9.089862982380825684 ) ) ;
#6429=CARTESIAN_POINT ( 'NONE',  ( 132.5240116932087062, 253.9865022471903160, 10.00000000000009237 ) ) ;
#6430=ORIENTED_EDGE ( 'NONE', *, *, #62643, .F. ) ;
#6434=CARTESIAN_POINT ( 'NONE',  ( 181.4091070389452511, 290.9398227325178823, -11.15856678108262123 ) ) ;
#6437=CARTESIAN_POINT ( 'NONE',  ( 158.7169418325966888, 256.1484519720124240, 16.12901909612147477 ) ) ;
#6438=CARTESIAN_POINT ( 'NONE',  ( 190.5500686693750083, 278.8001826294041621, -16.51372018954678111 ) ) ;
#6440=CARTESIAN_POINT ( 'NONE',  ( 152.8721808860877616, 265.8646109718731623, -17.65676496037632504 ) ) ;
#6444=CARTESIAN_POINT ( 'NONE',  ( 184.7157775894015117, 297.3647472220100099, -4.497232409310948142 ) ) ;
#6446=ORIENTED_EDGE ( 'NONE', *, *, #78162, .T. ) ;
#6447=VERTEX_POINT ( 'NONE', #97413 ) ;
#6451=CARTESIAN_POINT ( 'NONE',  ( 204.9103773355753617, 275.7318107871104189, 13.62808820451859937 ) ) ;
#6452=CARTESIAN_POINT ( 'NONE',  ( 163.3721123024899100, 272.7106123632322578, -15.45002922943936952 ) ) ;
#6456=CARTESIAN_POINT ( 'NONE',  ( 190.4744901378711290, 300.7355008658671522, 0.04566709859947504224 ) ) ;
#6457=CARTESIAN_POINT ( 'NONE',  ( 185.6331528164076019, 275.1493494416136514, -17.66137984873601496 ) ) ;
#6459=CARTESIAN_POINT ( 'NONE',  ( 178.4479938518580866, 254.7379757184021685, 5.915197645450990471 ) ) ;
#6460=CARTESIAN_POINT ( 'NONE',  ( 113.0020953926368037, 245.2369531367911009, -4.594050593750048428 ) ) ;
#6462=CARTESIAN_POINT ( 'NONE',  ( 183.3861558808938810, 260.1507132443945238, -9.436288690551128511 ) ) ;
#6464=CARTESIAN_POINT ( 'NONE',  ( 187.8353234249231321, 291.6460669958726157, -14.22777192653921041 ) ) ;
#6465=ORIENTED_EDGE ( 'NONE', *, *, #31210, .F. ) ;
#6466=ADVANCED_FACE ( 'NONE', ( #51274 ), #55001, .F. ) ;
#6467=CARTESIAN_POINT ( 'NONE',  ( 163.1192251533336162, 248.6989372057958576, -9.692595118822335820 ) ) ;
#6468=ADVANCED_FACE ( 'NONE', ( #77593 ), #97815, .F. ) ;
#6470=CARTESIAN_POINT ( 'NONE',  ( 196.0355168007595523, 291.1035201434990540, 17.55377893960077884 ) ) ;
#6472=CARTESIAN_POINT ( 'NONE',  ( 95.42925689777531773, 219.2365022471902023, -10.00000000000009237 ) ) ;
#6474=CARTESIAN_POINT ( 'NONE',  ( 148.6802791471854448, 273.1251977639880693, 9.299514254131516111 ) ) ;
#6478=CARTESIAN_POINT ( 'NONE',  ( 152.3360070569975449, 270.2436951681156643, -14.78697292633622951 ) ) ;
#6481=CARTESIAN_POINT ( 'NONE',  ( 196.2834844919150612, 264.3817122522384579, 3.934541318863804094 ) ) ;
#6485=CARTESIAN_POINT ( 'NONE',  ( 157.0825463324651707, 280.7710845550788576, 6.027187208097937621 ) ) ;
#6486=CARTESIAN_POINT ( 'NONE',  ( 201.3505934466285510, 281.8975373467312693, -16.83770227898004279 ) ) ;
#6488=CARTESIAN_POINT ( 'NONE',  ( 157.4729130248890954, 257.8959091554543761, 17.83439074639795052 ) ) ;
#6489=FACE_OUTER_BOUND ( 'NONE', #87749, .T. ) ;
#6490=CARTESIAN_POINT ( 'NONE',  ( 190.6636931378345992, 264.2239263948314374, -9.507720587469599138 ) ) ;
#6491=CARTESIAN_POINT ( 'NONE',  ( 171.6851387733911167, 250.5862967750797736, -0.2559814552254628395 ) ) ;
#6492=CARTESIAN_POINT ( 'NONE',  ( 189.1666306803385282, 269.6788385675433233, -13.95880351805504382 ) ) ;
#6499=CARTESIAN_POINT ( 'NONE',  ( 29.10614472461701752, 187.6115022471902591, 10.00000000000009592 ) ) ;
#6501=CARTESIAN_POINT ( 'NONE',  ( 82.77265646360999085, 218.5958772461660544, -9.188101187500095079 ) ) ;
#6502=CARTESIAN_POINT ( 'NONE',  ( 159.9770824720811220, 253.5585604421560788, -16.42166711341322483 ) ) ;
#6504=CARTESIAN_POINT ( 'NONE',  ( 163.3020905273760093, 247.7994775548095845, -11.05431316445765155 ) ) ;
#6505=B_SPLINE_CURVE_WITH_KNOTS ( 'NONE', 3,
 ( #53653, #98800, #52659, #92226 ),
 .UNSPECIFIED., .F., .F.,
 ( 4, 4 ),
 ( 0.03592842450685154038, 0.04464100137491056747 ),
 .UNSPECIFIED. ) ;
#6506=CARTESIAN_POINT ( 'NONE',  ( 196.9526636073363477, 287.5149752765084941, -17.63101726665603053 ) ) ;
#6507=CARTESIAN_POINT ( 'NONE',  ( 207.3874697692679945, 271.4413608369101780, -6.809237722377445401 ) ) ;
#6508=CYLINDRICAL_SURFACE ( 'NONE', #69176, 17.82106496071139645 ) ;
#6509=CARTESIAN_POINT ( 'NONE',  ( 108.1850894041357094, 223.2677522451417929, -5.000000000000041744 ) ) ;
#6510=CARTESIAN_POINT ( 'NONE',  ( 185.9530610298360216, 265.4397761326690670, 13.93956406728625375 ) ) ;
#6511=CARTESIAN_POINT ( 'NONE',  ( 188.1065894726285990, 258.8392727029177536, -0.5366119281032075694 ) ) ;
#6517=CARTESIAN_POINT ( 'NONE',  ( 29.83685365728618066, 188.0333772461660544, 9.188101187500095079 ) ) ;
#6518=CARTESIAN_POINT ( 'NONE',  ( 157.7365441389748923, 257.4392866714015895, 18.13124212464487073 ) ) ;
#6519=CARTESIAN_POINT ( 'NONE',  ( 199.3165775953382024, 277.8358694028592595, 15.47252840930216067 ) ) ;
#6520=ADVANCED_FACE ( 'NONE', ( #19788 ), #39615, .F. ) ;
#6523=CARTESIAN_POINT ( 'NONE',  ( 39.14627965220388006, 205.6589784336661637, -6.496448406907676862E-16 ) ) ;
#6525=CARTESIAN_POINT ( 'NONE',  ( 151.1451503555562113, 268.8559155969762742, -15.81507177720227553 ) ) ;
#6526=CARTESIAN_POINT ( 'NONE',  ( 196.9976074755333286, 289.4371302133026802, -16.79549473444794216 ) ) ;
#6528=CARTESIAN_POINT ( 'NONE',  ( 157.4893260420801653, 257.8674809757739013, -18.30842125257398223 ) ) ;
#6529=CARTESIAN_POINT ( 'NONE',  ( 202.9014212808193918, 270.0062346898790793, -6.438034076772497727 ) ) ;
#6530=CARTESIAN_POINT ( 'NONE',  ( 174.9358745049650565, 292.2217799751211942, 2.235529367806339263 ) ) ;
#6531=ADVANCED_FACE ( 'NONE', ( #57618 ), #61434, .F. ) ;
#6532=CARTESIAN_POINT ( 'NONE',  ( 179.2582380156520401, 276.5659109761746777, 16.30564618147165845 ) ) ;
#6534=CARTESIAN_POINT ( 'NONE',  ( 153.3384820949992502, 276.8128241755385943, 7.236455069745591828 ) ) ;
#6535=B_SPLINE_CURVE_WITH_KNOTS ( 'NONE', 3,
 ( #36354, #88635, #3971, #50558, #34853, #19201, #96212, #12585, #89623, #80517, #11591, #28260, #51051, #35363, #65757, #96711, #95730, #27279, #89142, #81509, #59134, #26281, #20184, #82011, #43457, #11093, #65269, #12079, #42938, #73877, #45446, #76379, #99174, #37347, #45933, #36857, #67259, #6954, #21183, #90619, #91589, #92114, #22160, #7966, #61141, #44950, #30256, #75890 ),
 .UNSPECIFIED., .F., .F.,
 ( 4, 2, 2, 2, 2, 2, 2, 2, 2, 2, 2, 2, 2, 2, 2, 2, 2, 2, 2, 2, 2, 2, 2, 4 ),
 ( 0.001614394524384737788, 0.002072026746786071599, 0.002529658969187404977, 0.002758475080388071883, 0.002872883135988325322, 0.002987291191588578761, 0.003101699247188831766, 0.003216107302789084771, 0.003444923413989510116, 0.003902555636390277975, 0.004360187858791046700, 0.005275452303592720327, 0.006190716748394393953, 0.006648348970795231634, 0.007105981193196068448, 0.007220389248796255967, 0.007277593276596350594, 0.007334797304396444353, 0.007449205359996691721, 0.007563613415596938221, 0.008021245637998029171, 0.008478877860399122723, 0.008707693971599577559, 0.008936510082800030660 ),
 .UNSPECIFIED. ) ;
#6537=CARTESIAN_POINT ( 'NONE',  ( 103.2234855318352373, 223.7365022471902023, -10.00000000000009059 ) ) ;
#6541=CARTESIAN_POINT ( 'NONE',  ( 60.95981515367195414, 199.8768266524160140, 9.188101187500098632 ) ) ;
#6542=ORIENTED_EDGE ( 'NONE', *, *, #92994, .T. ) ;
#6543=CARTESIAN_POINT ( 'NONE',  ( 166.1065669591089886, 265.3346322838461333, 16.55527594901084854 ) ) ;
#6544=CARTESIAN_POINT ( 'NONE',  ( 162.7414887829580721, 250.5555091418873985, 12.74047579032432687 ) ) ;
#6546=DIRECTION ( 'NONE',  ( -0.8660254037844387076, -0.4999999999999998890, -0.000000000000000000 ) ) ;
#6553=CARTESIAN_POINT ( 'NONE',  ( 204.3227106360847927, 276.7496793685443208, 13.60086062244164573 ) ) ;
#6554=ORIENTED_EDGE ( 'NONE', *, *, #7512, .F. ) ;
#6559=ORIENTED_EDGE ( 'NONE', *, *, #13796, .F. ) ;
#6561=CARTESIAN_POINT ( 'NONE',  ( 206.3018347371251195, 273.3217358710584790, -9.309724106897926177 ) ) ;
#6564=ORIENTED_EDGE ( 'NONE', *, *, #23596, .F. ) ;
#6566=CARTESIAN_POINT ( 'NONE',  ( 161.3004582353723322, 282.7615572226706604, -3.141450372068092634 ) ) ;
#6568=CARTESIAN_POINT ( 'NONE',  ( 189.7726967107949747, 264.4065126852114531, 11.24316165915873000 ) ) ;
#6569=CARTESIAN_POINT ( 'NONE',  ( 163.7707306762541748, 246.9877690064858484, 7.021959502997312086 ) ) ;
#6572=CARTESIAN_POINT ( 'NONE',  ( 161.2003520097632929, 263.0782596298864178, -17.28377924258164455 ) ) ;
#6574=CARTESIAN_POINT ( 'NONE',  ( 135.5734031224162663, 239.8923013555409796, 4.594050593750050204 ) ) ;
#6575=CARTESIAN_POINT ( 'NONE',  ( 198.2505066714982149, 285.2670451491296149, 0.000000000000000000 ) ) ;
#6576=CARTESIAN_POINT ( 'NONE',  ( 195.7755322585767317, 290.7755156195648851, -16.12766413607943150 ) ) ;
#6577=CARTESIAN_POINT ( 'NONE',  ( 78.09096694622414248, 206.7048013555409796, 4.594050593750051981 ) ) ;
#6579=CARTESIAN_POINT ( 'NONE',  ( 170.2456429460595757, 264.0157069346884668, 17.14554996422683431 ) ) ;
#6583=CARTESIAN_POINT ( 'NONE',  ( 160.2064895855051248, 253.7921695486214446, 15.02796977922756838 ) ) ;
#6584=ORIENTED_EDGE ( 'NONE', *, *, #82033, .F. ) ;
#6588=CARTESIAN_POINT ( 'NONE',  ( 190.0667283601964357, 259.9641452334862493, -5.090329199819447104E-14 ) ) ;
#6591=CARTESIAN_POINT ( 'NONE',  ( 193.0512205562391159, 275.6825563886401369, -16.88465587640301280 ) ) ;
#6595=CARTESIAN_POINT ( 'NONE',  ( 206.8711744556208885, 269.6661967102621702, -5.660351959544826712E-12 ) ) ;
#6599=CARTESIAN_POINT ( 'NONE',  ( 183.7168947869212161, 275.6071481288901168, 16.66324111737131730 ) ) ;
#6600=CARTESIAN_POINT ( 'NONE',  ( 206.5318754762992910, 272.9232936229979032, 10.63244694018452741 ) ) ;
#6601=CARTESIAN_POINT ( 'NONE',  ( 169.5608680270499917, 283.3855602016760713, -12.49222823364715040 ) ) ;
#6603=CARTESIAN_POINT ( 'NONE',  ( 162.8296681715975467, 261.5150638136722137, 17.10512620579534726 ) ) ;
#6604=CARTESIAN_POINT ( 'NONE',  ( 145.9657079678295020, 245.8923013555409511, 4.594050593750050204 ) ) ;
#6605=ORIENTED_EDGE ( 'NONE', *, *, #77001, .F. ) ;
#6608=CARTESIAN_POINT ( 'NONE',  ( 166.5303610463213602, 284.3444823442944767, -9.543174262395664798 ) ) ;
#6614=CARTESIAN_POINT ( 'NONE',  ( 199.5606914717536711, 266.8596729079026204, 4.600230128018988118 ) ) ;
#6615=CARTESIAN_POINT ( 'NONE',  ( 204.0884846259506276, 275.1553707185394728, 13.46337290381501717 ) ) ;
#6617=CARTESIAN_POINT ( 'NONE',  ( 185.1897086401880586, 263.6483258020415974, -12.64245034936682721 ) ) ;
#6619=CARTESIAN_POINT ( 'NONE',  ( 195.1395877695788670, 263.6489633415297931, 0.8500072188313321231 ) ) ;
#6620=B_SPLINE_CURVE_WITH_KNOTS ( 'NONE', 3,
 ( #31688, #23101, #15496, #54488 ),
 .UNSPECIFIED., .F., .F.,
 ( 4, 4 ),
 ( 0.008185375094193318019, 0.01430533136218472591 ),
 .UNSPECIFIED. ) ;
#6621=VERTEX_POINT ( 'NONE', #90582 ) ;
#6623=CARTESIAN_POINT ( 'NONE',  ( 186.4575292785845022, 282.5265642665722794, 16.18250184841760841 ) ) ;
#6624=CARTESIAN_POINT ( 'NONE',  ( 207.1122325394003951, 271.9180857031755636, 7.794245785756032774 ) ) ;
#6625=CARTESIAN_POINT ( 'NONE',  ( 155.0197698005585494, 262.1448778582381465, 18.42918111182112284 ) ) ;
#6626=CARTESIAN_POINT ( 'NONE',  ( 196.2721503905644056, 270.7675346716773106, 11.95883742778919157 ) ) ;
#6629=FACE_OUTER_BOUND ( 'NONE', #37555, .T. ) ;
#6631=CARTESIAN_POINT ( 'NONE',  ( 160.0072461633487535, 253.5063153963366744, 16.23938890643736244 ) ) ;
#6635=CARTESIAN_POINT ( 'NONE',  ( 150.9811781078167598, 244.6427522451417360, 1.119607411625061291E-15 ) ) ;
#6640=CARTESIAN_POINT ( 'NONE',  ( 202.5477177782173897, 274.2023237505306383, -12.92955543092264215 ) ) ;
#6641=CARTESIAN_POINT ( 'NONE',  ( 198.9590707264871412, 286.0397762054715827, -17.05306195936250191 ) ) ;
#6642=CARTESIAN_POINT ( 'NONE',  ( 1.717831006336420607, 180.9869531367911293, 4.594050593750046652 ) ) ;
#6643=CARTESIAN_POINT ( 'NONE',  ( 178.4244581223062767, 273.6332221299129515, -17.11712909880773736 ) ) ;
#6646=CARTESIAN_POINT ( 'NONE',  ( 70.58515312316130519, 204.8927522451418213, -10.00000000000009237 ) ) ;
#6650=CARTESIAN_POINT ( 'NONE',  ( 175.5929596258776542, 253.6151216998191558, -3.855483475996990705 ) ) ;
#6651=CARTESIAN_POINT ( 'NONE',  ( 198.6416989287814943, 286.5894802839873137, 18.33538993684147300 ) ) ;
#6652=CARTESIAN_POINT ( 'NONE',  ( 48.66388509341553714, 212.2365022471903444, 2.944929066748280225E-16 ) ) ;
#6654=CARTESIAN_POINT ( 'NONE',  ( 190.6071113721798156, 300.5057941498820924, -0.4754021072632813594 ) ) ;
#6655=CARTESIAN_POINT ( 'NONE',  ( 21.71786549680706102, 183.3458772461660544, 9.188101187500095079 ) ) ;
#6658=CARTESIAN_POINT ( 'NONE',  ( 201.3991315993686158, 280.4374122447417790, -16.53561221323570862 ) ) ;
#6659=DIRECTION ( 'NONE',  ( -0.8660254037844387076, -0.4999999999999998890, -0.000000000000000000 ) ) ;
#6660=CARTESIAN_POINT ( 'NONE',  ( 188.9655998164360824, 267.8375115036470220, 14.10301077631414302 ) ) ;
#6661=CARTESIAN_POINT ( 'NONE',  ( 153.7843434526567989, 265.0750476961756590, -16.54915785148878271 ) ) ;
#6662=CARTESIAN_POINT ( 'NONE',  ( 164.0803995805677573, 281.7114191920252892, 9.860144147819550398 ) ) ;
#6665=CARTESIAN_POINT ( 'NONE',  ( 190.5726849661229210, 300.5654224342945326, -0.2192718484028965964 ) ) ;
#6667=CARTESIAN_POINT ( 'NONE',  ( 154.9683083969241011, 262.2340116239618055, 18.33261662430134109 ) ) ;
#6669=CARTESIAN_POINT ( 'NONE',  ( 184.2544554321892747, 290.3215093552799999, 12.16168713926963996 ) ) ;
#6671=CARTESIAN_POINT ( 'NONE',  ( 0.3649266329730349034, 171.0177522451418781, -10.00000000000009592 ) ) ;
#6672=ORIENTED_EDGE ( 'NONE', *, *, #87563, .T. ) ;
#6676=CARTESIAN_POINT ( 'NONE',  ( 203.3684377202211522, 278.4025285431072803, -16.56116267537666076 ) ) ;
#6677=ADVANCED_FACE ( 'NONE', ( #35826 ), #58607, .T. ) ;
#6678=( BOUNDED_CURVE ( )  B_SPLINE_CURVE ( 2, ( #78273, #2793, #8857, #17458, #78777, #55930, #72695, #9362, #16948 ),
 .UNSPECIFIED., .F., .F. ) 
 B_SPLINE_CURVE_WITH_KNOTS ( ( 3, 2, 2, 2, 3 ),
 ( 0.3185483870967741882, 0.3198924731182795633, 0.3225806451612903136, 0.3252688172043010639, 0.3266129032258064391 ),
 .UNSPECIFIED. ) 
 CURVE ( )  GEOMETRIC_REPRESENTATION_ITEM ( )  RATIONAL_B_SPLINE_CURVE ( ( 0.9330127018922194093, 0.9330127018922194093, 1.000000000000000000, 0.8660254037844387076, 1.000000000000000000, 0.8660254037844387076, 1.000000000000000000, 0.9330127018922194093, 0.9330127018922194093 ) ) 
 REPRESENTATION_ITEM ( '' )  );
#6680=CARTESIAN_POINT ( 'NONE',  ( 67.62392126478502519, 221.3967562850346837, -4.648177544792955347E-16 ) ) ;
#6683=CARTESIAN_POINT ( 'NONE',  ( 191.4941427383744781, 298.9694107557253346, 8.584406880462095657 ) ) ;
#6684=DIRECTION ( 'NONE',  ( -0.8660254037844387076, -0.4999999999999998890, -0.000000000000000000 ) ) ;
#6686=CARTESIAN_POINT ( 'NONE',  ( 135.1739027599712131, 260.3967562850347122, -4.648177544792955347E-16 ) ) ;
#6687=EDGE_CURVE ( 'NONE', #26873, #85118, #74658, .T. ) ;
#6691=CARTESIAN_POINT ( 'NONE',  ( 164.4494343874829099, 245.8122196953522121, 2.922779519406129456 ) ) ;
#6694=CARTESIAN_POINT ( 'NONE',  ( 190.1190668544949460, 301.3511120508678118, 4.410340539513557090 ) ) ;
#6696=EDGE_LOOP ( 'NONE', ( #24877, #24488, #66344, #65999 ) ) ;
#6698=( BOUNDED_CURVE ( )  B_SPLINE_CURVE ( 2, ( #54420, #77769, #85397, #70130, #39223, #93487, #24045, #2642, #43093 ),
 .UNSPECIFIED., .F., .F. ) 
 B_SPLINE_CURVE_WITH_KNOTS ( ( 3, 2, 2, 2, 3 ),
 ( 0.1088709677419354843, 0.1102150537634408595, 0.1129032258064516098, 0.1155913978494623601, 0.1169354838709677491 ),
 .UNSPECIFIED. ) 
 CURVE ( )  GEOMETRIC_REPRESENTATION_ITEM ( )  RATIONAL_B_SPLINE_CURVE ( ( 0.9330127018922194093, 0.9330127018922194093, 1.000000000000000000, 0.8660254037844387076, 1.000000000000000000, 0.8660254037844387076, 1.000000000000000000, 0.9330127018922189652, 0.9330127018922192983 ) ) 
 REPRESENTATION_ITEM ( '' )  );
#6699=CARTESIAN_POINT ( 'NONE',  ( 149.0247308281161622, 274.5285899518638075, 9.115861392502811356 ) ) ;
#6702=VERTEX_POINT ( 'NONE', #57953 ) ;
#6704=ORIENTED_EDGE ( 'NONE', *, *, #76526, .F. ) ;
#6705=CARTESIAN_POINT ( 'NONE',  ( 156.2256614230932428, 267.4609830032940181, -16.82359569179483216 ) ) ;
#6706=CARTESIAN_POINT ( 'NONE',  ( 146.8358616138309571, 276.3198226421291679, 4.054088818585255716 ) ) ;
#6707=CARTESIAN_POINT ( 'NONE',  ( 148.4016473149517594, 273.6078022540229426, 8.470066617688926769 ) ) ;
#6708=CARTESIAN_POINT ( 'NONE',  ( 149.1856130393175306, 272.2499337880290682, 11.44243872309708188 ) ) ;
#6709=CARTESIAN_POINT ( 'NONE',  ( 157.4500450658088937, 258.5180226767713521, -16.88753703094210579 ) ) ;
#6710=CARTESIAN_POINT ( 'NONE',  ( 191.7833554288250184, 298.4684796816713970, 8.633437946248736949 ) ) ;
#6711=CARTESIAN_POINT ( 'NONE',  ( 146.6647111637776106, 276.6162639173599587, -0.6373001129109082674 ) ) ;
#6712=CARTESIAN_POINT ( 'NONE',  ( 148.9498507103374152, 272.6582861203333437, 11.90061892622094852 ) ) ;
#6714=CARTESIAN_POINT ( 'NONE',  ( 149.7109319212262051, 271.3400547943878109, -12.38605961032017433 ) ) ;
#6717=CARTESIAN_POINT ( 'NONE',  ( 168.2645477972932326, 286.3693708646730443, 3.929190110370803790 ) ) ;
#6719=CARTESIAN_POINT ( 'NONE',  ( 99.71410487726056715, 234.5024278399160949, 9.188101187500095079 ) ) ;
#6720=ORIENTED_EDGE ( 'NONE', *, *, #37203, .F. ) ;
#6721=CARTESIAN_POINT ( 'NONE',  ( 190.2890464677749662, 301.0566987244154120, -4.760511403740203207 ) ) ;
#6725=ADVANCED_FACE ( 'NONE', ( #50351 ), #87933, .T. ) ;
#6726=CARTESIAN_POINT ( 'NONE',  ( 180.4782130350719171, 283.6118113979034661, -16.15436706920364074 ) ) ;
#6729=CARTESIAN_POINT ( 'NONE',  ( 166.3623252550682423, 283.7353191977674101, -8.107535353489314645 ) ) ;
#6730=ORIENTED_EDGE ( 'NONE', *, *, #65631, .T. ) ;
#6731=CARTESIAN_POINT ( 'NONE',  ( 170.5698107352472732, 255.6068603507982289, -11.67185973913825769 ) ) ;
#6732=CARTESIAN_POINT ( 'NONE',  ( 159.2186641046529303, 254.8721795879351646, -15.96198087403305443 ) ) ;
#6735=ADVANCED_FACE ( 'NONE', ( #4770 ), #48874, .T. ) ;
#6736=CARTESIAN_POINT ( 'NONE',  ( 47.20246722098145398, 191.3927522451417929, -10.00000000000009059 ) ) ;
#6737=CARTESIAN_POINT ( 'NONE',  ( 108.9156247924702114, 239.8149278399160949, -9.188101187500095079 ) ) ;
#6738=CARTESIAN_POINT ( 'NONE',  ( 174.3575034883137391, 273.0034624690363216, 17.77573060583294762 ) ) ;
#6740=FACE_OUTER_BOUND ( 'NONE', #57022, .T. ) ;
#6741=CARTESIAN_POINT ( 'NONE',  ( 175.3489461370708398, 253.4744944187259819, -3.884895130763601490 ) ) ;
#6742=CARTESIAN_POINT ( 'NONE',  ( 41.71789998727770410, 185.7048013555409796, 4.594050593750051981 ) ) ;
#6744=ORIENTED_EDGE ( 'NONE', *, *, #457, .T. ) ;
#6749=CARTESIAN_POINT ( 'NONE',  ( 190.1696443193688708, 301.2635093119881162, -4.804312979389741223 ) ) ;
#6753=CARTESIAN_POINT ( 'NONE',  ( 105.5870131927823508, 231.7677522451418497, 10.00000000000009592 ) ) ;
#6755=FACE_OUTER_BOUND ( 'NONE', #56232, .T. ) ;
#6756=CARTESIAN_POINT ( 'NONE',  ( 155.4495112628364097, 279.7055087804715754, -1.752144325060382535 ) ) ;
#6757=CARTESIAN_POINT ( 'NONE',  ( 162.9383752892161397, 248.4294508267893491, -11.25953730674605957 ) ) ;
#6758=CARTESIAN_POINT ( 'NONE',  ( 22.80074434730262567, 171.7202760586659736, -5.415160957724236172E-17 ) ) ;
#6760=CARTESIAN_POINT ( 'NONE',  ( 196.1615410976813507, 273.7113085403182140, 14.86458732197895216 ) ) ;
#6763=CARTESIAN_POINT ( 'NONE',  ( 174.7229882116660065, 286.3465783895868526, 10.42342695070571601 ) ) ;
#6764=CARTESIAN_POINT ( 'NONE',  ( 73.65258675182887771, 204.1423013555409796, -4.594050593750043987 ) ) ;
#6765=CARTESIAN_POINT ( 'NONE',  ( 164.1821508476733698, 246.2751683663292397, -7.347745041495428175 ) ) ;
#6771=CARTESIAN_POINT ( 'NONE',  ( 12.29081813446918758, 171.2365022471902023, -10.00000000000009059 ) ) ;
#6772=CARTESIAN_POINT ( 'NONE',  ( 208.3135187673106543, 269.8373969220020285, 2.829653198597726682 ) ) ;
#6773=CARTESIAN_POINT ( 'NONE',  ( 135.0589402170954827, 248.7833772461660544, -9.188101187500095079 ) ) ;
#6775=CARTESIAN_POINT ( 'NONE',  ( 207.5551753531803172, 271.1508862448613399, -7.290975649195053698 ) ) ;
#6781=ORIENTED_EDGE ( 'NONE', *, *, #59421, .F. ) ;
#6782=CARTESIAN_POINT ( 'NONE',  ( 64.01779381112933720, 197.7677522451418213, -5.000000000000041744 ) ) ;
#6785=CARTESIAN_POINT ( 'NONE',  ( 196.6039295022987972, 289.7324168733214833, 16.35530466314298437 ) ) ;
#6786=CARTESIAN_POINT ( 'NONE',  ( 196.9474029239601975, 272.9819407449171536, -13.37321390883489691 ) ) ;
#6788=CARTESIAN_POINT ( 'NONE',  ( 206.5002523963886176, 272.9780664040949318, 9.017141309861059995 ) ) ;
#6791=CARTESIAN_POINT ( 'NONE',  ( 148.8112445470583225, 273.2837754581220793, -9.153596929589264519 ) ) ;
#6792=CARTESIAN_POINT ( 'NONE',  ( 196.3844087422174596, 270.6169231452851704, 13.31990624255254474 ) ) ;
#6794=CARTESIAN_POINT ( 'NONE',  ( 208.1912724900461740, 270.0491336852600170, -0.9856800448607289100 ) ) ;
#6795=CARTESIAN_POINT ( 'NONE',  ( 200.9812045408918380, 282.5373376992193926, -16.61165062382494284 ) ) ;
#6797=CARTESIAN_POINT ( 'NONE',  ( 190.6828093349753317, 281.2089909899326585, 16.73330534773390710 ) ) ;
#6805=CARTESIAN_POINT ( 'NONE',  ( 191.3041230083617563, 299.2985345825480863, -9.819045872446528378 ) ) ;
#6807=CARTESIAN_POINT ( 'NONE',  ( 164.4294002498235159, 245.8469198396639399, 6.098783631055905374 ) ) ;
#6811=CARTESIAN_POINT ( 'NONE',  ( 106.3178956768819319, 226.0643266524159856, -9.188101187500093303 ) ) ;
#6813=CARTESIAN_POINT ( 'NONE',  ( 180.5397319334442159, 270.7127871342991625, -15.99547242021038329 ) ) ;
#6815=ORIENTED_EDGE ( 'NONE', *, *, #62143, .F. ) ;
#6818=CARTESIAN_POINT ( 'NONE',  ( 157.4991920912938497, 281.1666361535517353, -5.886997319559604591 ) ) ;
#6819=ORIENTED_EDGE ( 'NONE', *, *, #99531, .T. ) ;
#6820=CARTESIAN_POINT ( 'NONE',  ( 159.5903462228227738, 257.4064654884239758, -17.16338673343565446 ) ) ;
#6822=CARTESIAN_POINT ( 'NONE',  ( 163.8111161534324935, 246.9178193081252743, -7.110480325054721717 ) ) ;
#6823=CYLINDRICAL_SURFACE ( 'NONE', #12371, 17.82106496071139645 ) ;
#6829=CARTESIAN_POINT ( 'NONE',  ( 198.7242481644049121, 277.5995992023655958, -15.36478769293520941 ) ) ;
#6832=ORIENTED_EDGE ( 'NONE', *, *, #55561, .T. ) ;
#6833=CARTESIAN_POINT ( 'NONE',  ( 162.9796882977680639, 248.3578945969637743, 9.683801903336119565 ) ) ;
#6834=CARTESIAN_POINT ( 'NONE',  ( 185.0543536129055155, 258.0163728256403033, 3.008362416367333925 ) ) ;
#6836=DIRECTION ( 'NONE',  ( -0.5000000000000006661, 0.8660254037844382635, -1.877843081442121204E-16 ) ) ;
#6837=CARTESIAN_POINT ( 'NONE',  ( 171.8532966785767258, 254.8378052108570273, 11.04733308641842804 ) ) ;
#6839=CARTESIAN_POINT ( 'NONE',  ( 157.7886504734048003, 281.3435236914132815, 1.490504832958681636 ) ) ;
#6840=ORIENTED_EDGE ( 'NONE', *, *, #99780, .F. ) ;
#6841=CARTESIAN_POINT ( 'NONE',  ( 97.95516432547988472, 227.3615022471902591, -10.00000000000009592 ) ) ;
#6844=EDGE_CURVE ( 'NONE', #73983, #2236, #33669, .T. ) ;
#6845=CARTESIAN_POINT ( 'NONE',  ( 4.262040950003053830, 163.2677522451418213, -5.000000000000041744 ) ) ;
#6846=CARTESIAN_POINT ( 'NONE',  ( 195.7350119871117329, 269.2567921979494372, -10.80356350091597761 ) ) ;
#6847=CARTESIAN_POINT ( 'NONE',  ( 175.0457569121529389, 281.4923175861599134, -14.14130193385072154 ) ) ;
#6848=CARTESIAN_POINT ( 'NONE',  ( 203.4748520814800088, 278.2182134627518053, -14.85237232639370575 ) ) ;
#6851=CARTESIAN_POINT ( 'NONE',  ( -11.27255005043015856, 173.4869531367911293, 4.594050593750046652 ) ) ;
#6853=CARTESIAN_POINT ( 'NONE',  ( 186.3020778951789111, 295.5636472136135922, 8.187152758880353431 ) ) ;
#6859=CYLINDRICAL_SURFACE ( 'NONE', #77663, 17.82106496071139645 ) ;
#6860=CARTESIAN_POINT ( 'NONE',  ( 202.1549692867851888, 280.5043175231993473, -17.32512590000773045 ) ) ;
#6862=CARTESIAN_POINT ( 'NONE',  ( 149.9300743764016488, 276.9001158938398817, 3.155267742367139139 ) ) ;
#6863=CARTESIAN_POINT ( 'NONE',  ( 25.77753312492912841, 179.5643266524160140, -9.188101187500093303 ) ) ;
#6864=CARTESIAN_POINT ( 'NONE',  ( 110.8370318831756975, 243.9869531367911009, 4.594050593750046652 ) ) ;
#6868=DIRECTION ( 'NONE',  ( -0.8660254037844387076, -0.4999999999999998890, -0.000000000000000000 ) ) ;
#6870=CARTESIAN_POINT ( 'NONE',  ( 62.64658692180388755, 213.6427522451419065, -10.00000000000009592 ) ) ;
#6871=CARTESIAN_POINT ( 'NONE',  ( 195.6974783896144174, 291.6890198465123945, 16.70600479393688431 ) ) ;
#6873=CARTESIAN_POINT ( 'NONE',  ( 184.3718295276511583, 274.4586611926505952, 17.53799969959756311 ) ) ;
#6876=CARTESIAN_POINT ( 'NONE',  ( 171.1613143928009606, 279.7166738654231040, 13.89588308401470051 ) ) ;
#6877=CARTESIAN_POINT ( 'NONE',  ( 186.9944938751388861, 298.8788464850996434, -0.5967753998689386830 ) ) ;
#6881=ORIENTED_EDGE ( 'NONE', *, *, #68874, .F. ) ;
#6884=CARTESIAN_POINT ( 'NONE',  ( 184.2750561946413654, 269.3830903805491630, 15.28138810499674349 ) ) ;
#6885=CARTESIAN_POINT ( 'NONE',  ( 94.03063961704269502, 237.3464784336661637, 1.353441290958777327E-15 ) ) ;
#6889=CARTESIAN_POINT ( 'NONE',  ( 196.0034224882197975, 291.1591091234520263, 17.53794140922627776 ) ) ;
#6891=CARTESIAN_POINT ( 'NONE',  ( 149.5742366896305668, 271.5768178806638957, 12.98651753098913098 ) ) ;
#6892=CARTESIAN_POINT ( 'NONE',  ( 150.9584389135710865, 269.1793093008492406, -15.82751450793727699 ) ) ;
#6893=CARTESIAN_POINT ( 'NONE',  ( 149.8928472635447804, 271.6201905152058771, -11.69094866835029656 ) ) ;
#6896=CARTESIAN_POINT ( 'NONE',  ( 123.2041546383393751, 253.4860189848785126, -2.679491924311252493 ) ) ;
#6901=CARTESIAN_POINT ( 'NONE',  ( 193.1977289678065404, 296.0187128512746995, -12.37159405312863925 ) ) ;
#6902=CARTESIAN_POINT ( 'NONE',  ( 149.7200635338602410, 271.3242383773507527, -12.12223662813266500 ) ) ;
#6903=VERTEX_POINT ( 'NONE', #67541 ) ;
#6906=CARTESIAN_POINT ( 'NONE',  ( 182.0647779265614190, 264.0180564602412119, -12.95455995337640864 ) ) ;
#6908=CARTESIAN_POINT ( 'NONE',  ( 173.1578642404289496, 253.8352349280846738, -9.039979433292165467 ) ) ;
#6909=CARTESIAN_POINT ( 'NONE',  ( 192.0963028965829551, 297.9264387674147656, 11.34530024772836754 ) ) ;
#6911=CARTESIAN_POINT ( 'NONE',  ( 187.3516457461684297, 278.8611292493811789, 17.07296404786917066 ) ) ;
#6914=CARTESIAN_POINT ( 'NONE',  ( 167.7292734088323130, 249.7294130688958376, 6.677680936074735563 ) ) ;
#6915=EDGE_CURVE ( 'NONE', #88465, #45893, #41290, .T. ) ;
#6916=CARTESIAN_POINT ( 'NONE',  ( 185.2856931816752990, 292.6844727045286731, -10.59087788492901971 ) ) ;
#6918=CARTESIAN_POINT ( 'NONE',  ( 166.1321135059490359, 260.4694391397057416, 16.98093069965871038 ) ) ;
#6920=CARTESIAN_POINT ( 'NONE',  ( 191.0757748809261045, 279.1147246841564993, -16.54284077524308927 ) ) ;
#6921=CARTESIAN_POINT ( 'NONE',  ( 192.6674894974040058, 296.9371145541902592, -12.11795536761400882 ) ) ;
#6922=CARTESIAN_POINT ( 'NONE',  ( 153.2513309553138470, 265.2079037882803618, -16.24091495603130397 ) ) ;
#6926=ORIENTED_EDGE ( 'NONE', *, *, #12641, .T. ) ;
#6927=CARTESIAN_POINT ( 'NONE',  ( 198.8683739244561082, 276.4215138120039796, -15.93986209720707414 ) ) ;
#6930=CARTESIAN_POINT ( 'NONE',  ( 205.0520875136525376, 275.4863615587311756, -14.16385635411862509 ) ) ;
#6931=CARTESIAN_POINT ( 'NONE',  ( 169.4094010280188911, 269.1046630455843456, 17.13746518211817360 ) ) ;
#6933=CARTESIAN_POINT ( 'NONE',  ( 174.0704149835363808, 256.6406572203894711, -12.38982705157956410 ) ) ;
#6938=CARTESIAN_POINT ( 'NONE',  ( 190.1730848958311810, 301.2575500587478814, 0.2415986433272204748 ) ) ;
#6939=CARTESIAN_POINT ( 'NONE',  ( 170.4449418037447970, 288.8185950528904300, -4.219811512460142744 ) ) ;
#6941=CARTESIAN_POINT ( 'NONE',  ( 178.6026051973306323, 254.4708812555809345, 5.813106864979912913 ) ) ;
#6942=CARTESIAN_POINT ( 'NONE',  ( 117.0621101165238542, 229.2048013555409796, 4.594050593750051981 ) ) ;
#6943=ORIENTED_EDGE ( 'NONE', *, *, #58563, .F. ) ;
#6946=CARTESIAN_POINT ( 'NONE',  ( 191.8258794905848674, 275.2947431816082258, 16.27196167175203811 ) ) ;
#6954=CARTESIAN_POINT ( 'NONE',  ( 180.7266824466902904, 294.1535421663213015, -2.386762920861517312 ) ) ;
#6955=FACE_OUTER_BOUND ( 'NONE', #85981, .T. ) ;
#6956=CARTESIAN_POINT ( 'NONE',  ( 190.3528479301325262, 300.4287509476951641, -0.1680789796435935290 ) ) ;
#6959=CARTESIAN_POINT ( 'NONE',  ( 147.9323189423145664, 274.4207028408641804, 9.430423372208688093 ) ) ;
#6961=B_SPLINE_CURVE_WITH_KNOTS ( 'NONE', 3,
 ( #202, #83344, #76702, #13910 ),
 .UNSPECIFIED., .F., .F.,
 ( 4, 4 ),
 ( 0.009355697899887138388, 0.01532099559381962239 ),
 .UNSPECIFIED. ) ;
#6963=EDGE_LOOP ( 'NONE', ( #62124, #48302, #96931, #83288 ) ) ;
#6964=CARTESIAN_POINT ( 'NONE',  ( 191.8890130564416552, 267.7039900243542547, -12.47167058615804258 ) ) ;
#6968=CARTESIAN_POINT ( 'NONE',  ( 192.4683202118899885, 263.0335775797599922, 4.534414443811968454 ) ) ;
#6969=CARTESIAN_POINT ( 'NONE',  ( 204.6209114679778338, 273.0706743954793296, -9.999413212032170151 ) ) ;
#6970=CARTESIAN_POINT ( 'NONE',  ( 184.2825131821604430, 288.8156619643899035, -13.20009111789595480 ) ) ;
#6971=CARTESIAN_POINT ( 'NONE',  ( 159.8157848413643762, 281.0678040903168267, 5.628117109850034439 ) ) ;
#6972=CARTESIAN_POINT ( 'NONE',  ( 153.3544108199959908, 265.0293642254135307, -17.49105661178601423 ) ) ;
#6974=CARTESIAN_POINT ( 'NONE',  ( 146.9709166616330549, 276.0859004375172390, 3.755270622130282732 ) ) ;
#6978=CARTESIAN_POINT ( 'NONE',  ( 192.4470566622854903, 271.7249251123275826, 14.07432190622019874 ) ) ;
#6979=CARTESIAN_POINT ( 'NONE',  ( 192.5309820353861312, 271.7291774915358360, -14.57346003379339727 ) ) ;
#6982=CARTESIAN_POINT ( 'NONE',  ( 67.06923665261433598, 197.9824982072973683, 3.021315404115420679E-15 ) ) ;
#6984=CARTESIAN_POINT ( 'NONE',  ( 80.17458025225667484, 217.0958772461660544, -9.188101187500095079 ) ) ;
#6985=DIRECTION ( 'NONE',  ( -0.8660254037844387076, -0.4999999999999998890, -0.000000000000000000 ) ) ;
#6986=CARTESIAN_POINT ( 'NONE',  ( 193.2100161762185735, 295.9974307820218087, -12.46499585622781758 ) ) ;
#6988=B_SPLINE_CURVE_WITH_KNOTS ( 'NONE', 3,
 ( #43229, #28040, #80297, #3281 ),
 .UNSPECIFIED., .F., .F.,
 ( 4, 4 ),
 ( 0.03632738840161289090, 0.04501103663793783877 ),
 .UNSPECIFIED. ) ;
#6989=CARTESIAN_POINT ( 'NONE',  ( 161.1093323826042933, 251.5974460702646809, -13.93502574894237078 ) ) ;
#6991=CARTESIAN_POINT ( 'NONE',  ( 99.82146873615951677, 239.9860189848785410, -2.679491924311252493 ) ) ;
#6995=CARTESIAN_POINT ( 'NONE',  ( 185.6713631041849055, 258.9584525764907426, -6.747383155299178092 ) ) ;
#6996=CARTESIAN_POINT ( 'NONE',  ( 161.9775247817796924, 252.0936927241524472, 14.33142805341373283 ) ) ;
#6997=CARTESIAN_POINT ( 'NONE',  ( 195.7578697689113199, 291.5844189092309193, 17.18796537138345215 ) ) ;
#6999=CARTESIAN_POINT ( 'NONE',  ( 26.45420224557697608, 176.8923013555409796, 4.594050593750050204 ) ) ;
#7000=CARTESIAN_POINT ( 'NONE',  ( 59.17381130624904273, 192.7202760586659736, -5.415160957724236172E-17 ) ) ;
#7001=CARTESIAN_POINT ( 'NONE',  ( 157.6335212189247557, 257.6177276032722716, 16.76495363836117036 ) ) ;
#7004=CARTESIAN_POINT ( 'NONE',  ( -5.895715345004023611, 160.7365022471901739, -10.00000000000009059 ) ) ;
#7005=CARTESIAN_POINT ( 'NONE',  ( 52.89478003304684250, 201.3458772461660260, 9.188101187500095079 ) ) ;
#7009=CARTESIAN_POINT ( 'NONE',  ( 151.2646864780760723, 268.6488729594320830, -14.38346604407754548 ) ) ;
#7010=CARTESIAN_POINT ( 'NONE',  ( 149.4965729687386045, 271.7113353911534546, -11.48413836595348059 ) ) ;
#7012=CARTESIAN_POINT ( 'NONE',  ( 157.7593757092099906, 257.3997412317380054, -18.08445832352326121 ) ) ;
#7014=CARTESIAN_POINT ( 'NONE',  ( 193.0622221429366050, 289.4054684591471300, 16.71589558189321778 ) ) ;
#7016=CARTESIAN_POINT ( 'NONE',  ( 182.2103161154203406, 281.0079499109055519, -16.50159754525817135 ) ) ;
#7017=CARTESIAN_POINT ( 'NONE',  ( 153.3639763765071677, 265.0127961955333262, 17.70482533658931956 ) ) ;
#7019=DIRECTION ( 'NONE',  ( -0.8660254037844359321, -0.5000000000000051070, -0.000000000000000000 ) ) ;
#7020=CARTESIAN_POINT ( 'NONE',  ( 110.8733765985977300, 241.4865022471902876, -10.00000000000009415 ) ) ;
#7021=CARTESIAN_POINT ( 'NONE',  ( 161.1238074876215478, 251.5723744529297505, 13.42537408252843179 ) ) ;
#7026=VERTEX_POINT ( 'NONE', #47235 ) ;
#7027=CARTESIAN_POINT ( 'NONE',  ( 166.5700286350222541, 264.7009711577636608, 17.59451997628320541 ) ) ;
#7028=CARTESIAN_POINT ( 'NONE',  ( 190.2971537673054456, 279.0018434785596924, -16.59784016563796172 ) ) ;
#7030=DIRECTION ( 'NONE',  ( 0.4999999999999992784, -0.8660254037844390407, 0.000000000000000000 ) ) ;
#7034=CARTESIAN_POINT ( 'NONE',  ( 164.9971748156432056, 244.8635054444190757, -1.825016704039769788 ) ) ;
#7036=CARTESIAN_POINT ( 'NONE',  ( 194.8067605455144076, 293.2317884077015151, -16.00245909155922774 ) ) ;
#7037=CARTESIAN_POINT ( 'NONE',  ( -17.42236680055705023, 149.2012482093457777, 0.000000000000000000 ) ) ;
#7041=CARTESIAN_POINT ( 'NONE',  ( 175.4168809732710201, 254.3420697835979638, 7.923593415617963487 ) ) ;
#7044=VERTEX_POINT ( 'NONE', #85284 ) ;
#7045=CARTESIAN_POINT ( 'NONE',  ( 181.1156277128715431, 292.7914473640799997, 9.490545386343454126 ) ) ;
#7046=ADVANCED_FACE ( 'NONE', ( #92382 ), #30545, .T. ) ;
#7047=CARTESIAN_POINT ( 'NONE',  ( 159.9531724557437826, 253.5999738052623229, -15.71074128491364874 ) ) ;
#7049=CARTESIAN_POINT ( 'NONE',  ( 173.4043485434340823, 285.5429356164705723, 10.51786951157661143 ) ) ;
#7050=CARTESIAN_POINT ( 'NONE',  ( 163.1916290246161054, 283.6901710720853771, -3.096747601227128666 ) ) ;
#7052=CARTESIAN_POINT ( 'NONE',  ( 208.3226489551340990, 269.8215829728092103, -1.240262689467544366 ) ) ;
#7053=CARTESIAN_POINT ( 'NONE',  ( 163.9149533033796047, 246.7379680887036670, 7.273005089308705706 ) ) ;
#7054=CARTESIAN_POINT ( 'NONE',  ( 198.4706398937704819, 286.8857632237200619, 17.04020736381253798 ) ) ;
#7056=CARTESIAN_POINT ( 'NONE',  ( 130.0249940097159254, 252.0024278399161517, -9.188101187500093303 ) ) ;
#7057=CARTESIAN_POINT ( 'NONE',  ( 176.3695042043887327, 268.9327831528794945, 16.12022517601484850 ) ) ;
#7058=CARTESIAN_POINT ( 'NONE',  ( 182.0444953139967197, 260.3474170450806469, 9.385908224742504302 ) ) ;
#7059=CARTESIAN_POINT ( 'NONE',  ( 74.43750904794977430, 201.5327760586659167, 1.948934522072303157E-15 ) ) ;
#7060=ORIENTED_EDGE ( 'NONE', *, *, #6142, .F. ) ;
#7061=CARTESIAN_POINT ( 'NONE',  ( 173.8505786369982786, 250.7855131160717121, 2.429319715737904950 ) ) ;
#7062=CARTESIAN_POINT ( 'NONE',  ( 161.9461893331167914, 280.9078031139047198, -10.53061385661272276 ) ) ;
#7066=EDGE_CURVE ( 'NONE', #19179, #66781, #32390, .T. ) ;
#7067=CARTESIAN_POINT ( 'NONE',  ( 68.76057960370418698, 222.0530062829863027, -4.648177544792955347E-16 ) ) ;
#7069=CARTESIAN_POINT ( 'NONE',  ( 194.2311797008547103, 284.7782822170849499, 17.68315500314775335 ) ) ;
#7070=CARTESIAN_POINT ( 'NONE',  ( 146.6363376198206652, 276.6654083370839885, -0.5879280619134327202 ) ) ;
#7072=CARTESIAN_POINT ( 'NONE',  ( 194.3799873100184641, 293.9709813348915191, 15.33105633561973669 ) ) ;
#7074=VERTEX_POINT ( 'NONE', #56325 ) ;
#7076=CARTESIAN_POINT ( 'NONE',  ( 161.7135578690656246, 250.5508968284854063, -12.67518793468364002 ) ) ;
#7084=CARTESIAN_POINT ( 'NONE',  ( 194.8918758260624315, 279.6717792136230401, 17.28916287495260917 ) ) ;
#7085=CARTESIAN_POINT ( 'NONE',  ( 162.9141107278308880, 261.5451400836783478, 17.20276467470873172 ) ) ;
#7086=CARTESIAN_POINT ( 'NONE',  ( 138.1979352100490530, 262.8464784336661637, 1.353441290958777327E-15 ) ) ;
#7089=EDGE_CURVE ( 'NONE', #50774, #99290, #39529, .T. ) ;
#7093=CARTESIAN_POINT ( 'NONE',  ( 153.0444155045374544, 265.5662918618958201, -16.15173036748435109 ) ) ;
#7098=CARTESIAN_POINT ( 'NONE',  ( 198.5871620011634491, 266.6819785607618769, 4.508239282148444715 ) ) ;
#7101=CARTESIAN_POINT ( 'NONE',  ( 184.5883480666688286, 263.6785044138370040, -12.30340380393476707 ) ) ;
#7102=CARTESIAN_POINT ( 'NONE',  ( 198.8150538021965588, 265.6931018340174546, 1.636156699923587254 ) ) ;
#7106=CARTESIAN_POINT ( 'NONE',  ( 183.6995465130360117, 281.2503605932585060, 17.37810211150572570 ) ) ;
#7108=CARTESIAN_POINT ( 'NONE',  ( 165.3498924805469414, 258.0561931571047580, -16.34667607723879001 ) ) ;
#7109=CARTESIAN_POINT ( 'NONE',  ( 196.9080397933726942, 269.7016881256661804, 12.39056067425276630 ) ) ;
#7112=CARTESIAN_POINT ( 'NONE',  ( 165.7002536143517091, 285.3157116585052222, -3.145807942481822828 ) ) ;
#7115=CARTESIAN_POINT ( 'NONE',  ( -8.863483026448420787, 159.5643266524160140, 9.188101187500095079 ) ) ;
#7120=CARTESIAN_POINT ( 'NONE',  ( 202.7163547726785282, 274.3787297666792711, -12.85394322792611632 ) ) ;
#7122=CARTESIAN_POINT ( 'NONE',  ( 14.68175618682351136, 167.0327760586659451, 1.948934522072302763E-15 ) ) ;
#7125=B_SPLINE_CURVE_WITH_KNOTS ( 'NONE', 3,
 ( #90677, #58704, #21233, #97746, #52605, #28314 ),
 .UNSPECIFIED., .F., .F.,
 ( 4, 2, 4 ),
 ( 0.001525191237219494008, 0.001894091869566394458, 0.002262992501913294908 ),
 .UNSPECIFIED. ) ;
#7126=CARTESIAN_POINT ( 'NONE',  ( 170.0564342972344321, 270.6948931233863505, -17.19293478356221883 ) ) ;
#7127=CARTESIAN_POINT ( 'NONE',  ( 150.1215823127449198, 276.5650925005066938, 4.233095963711685172 ) ) ;
#7128=CARTESIAN_POINT ( 'NONE',  ( 179.4321052950799356, 255.0977940521856340, -4.021643327155957515 ) ) ;
#7129=CARTESIAN_POINT ( 'NONE',  ( 188.1673108261343543, 259.1851068472254269, -0.8032118547848330348 ) ) ;
#7130=CARTESIAN_POINT ( 'NONE',  ( 56.38594494382682853, 203.3615022471902307, -10.00000000000009592 ) ) ;
#7132=CARTESIAN_POINT ( 'NONE',  ( 189.8238368927809745, 301.8624653444729802, -0.3620111495846872751 ) ) ;
#7133=CARTESIAN_POINT ( 'NONE',  ( 19.11978928545374501, 181.8458772461660544, 9.188101187500095079 ) ) ;
#7135=CARTESIAN_POINT ( 'NONE',  ( 125.6679772465819127, 253.3615022471903444, 5.000000000000046185 ) ) ;
#7139=CARTESIAN_POINT ( 'NONE',  ( 164.7694554770609159, 245.2579269087094076, -3.003635650077957742 ) ) ;
#7140=CARTESIAN_POINT ( 'NONE',  ( 189.1957819607296187, 268.1245522628738627, 13.92255382446146150 ) ) ;
#7141=CARTESIAN_POINT ( 'NONE',  ( 202.5650245025327081, 277.7940810556053179, -15.59262966521933791 ) ) ;
#7142=CARTESIAN_POINT ( 'NONE',  ( 179.6677993555305477, 263.0935507050606930, -13.53422970562010974 ) ) ;
#7147=CARTESIAN_POINT ( 'NONE',  ( 155.6435836392643637, 261.0644005951349982, 17.58841156286628049 ) ) ;
#7149=CARTESIAN_POINT ( 'NONE',  ( 181.6976215744686556, 289.2235858052403614, 12.51094214070181465 ) ) ;
#7155=CARTESIAN_POINT ( 'NONE',  ( 157.3525109086878899, 264.5174536549614572, 17.64881377233731641 ) ) ;
#7158=ADVANCED_FACE ( 'NONE', ( #74046 ), #20341, .T. ) ;
#7159=CARTESIAN_POINT ( 'NONE',  ( 179.4449360448816719, 257.2231220042240238, -7.316974778047405259 ) ) ;
#7163=CARTESIAN_POINT ( 'NONE',  ( 164.4864504671816690, 245.7481059646165704, 6.337356894698421783 ) ) ;
#7165=CARTESIAN_POINT ( 'NONE',  ( 190.8443993347725325, 300.0947993426467519, 8.522468760355437212 ) ) ;
#7169=B_SPLINE_CURVE_WITH_KNOTS ( 'NONE', 3,
 ( #54201, #76061, #85169, #98857, #83674, #46614, #29433, #75545, #21830, #6640, #14729, #45610, #7120, #18238, #63324, #17215, #87704, #17739 ),
 .UNSPECIFIED., .F., .F.,
 ( 4, 2, 2, 2, 2, 2, 2, 2, 4 ),
 ( 0.003007356136897285266, 0.003103104521746957896, 0.003198852906596630959, 0.003294601291446303589, 0.003390349676295976653, 0.003581846445995281580, 0.003773343215694586941, 0.004539330294491807950, 0.006071304452086345380 ),
 .UNSPECIFIED. ) ;
#7170=VERTEX_POINT ( 'NONE', #52213 ) ;
#7171=CARTESIAN_POINT ( 'NONE',  ( 189.9925954911225290, 301.5701668779311717, 0.1154287172046158938 ) ) ;
#7174=CARTESIAN_POINT ( 'NONE',  ( 157.1135969804030310, 258.5182628004787944, 17.19660297500358226 ) ) ;
#7175=CARTESIAN_POINT ( 'NONE',  ( 158.0882106229127828, 265.1277990769271469, 17.41991095839799542 ) ) ;
#7176=B_SPLINE_CURVE_WITH_KNOTS ( 'NONE', 3,
 ( #91327, #21887, #54775, #84238 ),
 .UNSPECIFIED., .F., .F.,
 ( 4, 4 ),
 ( 0.008222014946565199198, 0.01444170924531920988 ),
 .UNSPECIFIED. ) ;
#7177=VERTEX_POINT ( 'NONE', #59811 ) ;
#7178=CARTESIAN_POINT ( 'NONE',  ( 148.9275518150011806, 272.6969089400084272, 12.34519124974546500 ) ) ;
#7182=CARTESIAN_POINT ( 'NONE',  ( 160.0710471321888235, 254.2385718108182573, 15.38664727912921926 ) ) ;
#7185=VERTEX_POINT ( 'NONE', #20849 ) ;
#7186=ORIENTED_EDGE ( 'NONE', *, *, #8917, .F. ) ;
#7190=CARTESIAN_POINT ( 'NONE',  ( 190.1693911629507738, 301.2639477917662703, -5.112716700269980485 ) ) ;
#7192=CARTESIAN_POINT ( 'NONE',  ( 149.7166446726674565, 271.3301600186404698, 12.26048591517335495 ) ) ;
#7193=CARTESIAN_POINT ( 'NONE',  ( 133.0291931787496367, 257.6115022471902876, -5.000000000000047962 ) ) ;
#7194=CARTESIAN_POINT ( 'NONE',  ( 191.7416542989093671, 298.5407081574186350, 9.608469308039788714 ) ) ;
#7195=CARTESIAN_POINT ( 'NONE',  ( 191.5893301551938350, 298.8045413135534432, -8.323356515452589477 ) ) ;
#7197=CARTESIAN_POINT ( 'NONE',  ( 163.4623095168547025, 257.8152101734419261, 15.54367929412465976 ) ) ;
#7199=CARTESIAN_POINT ( 'NONE',  ( 149.0598351764325002, 272.4677874370131576, -11.59078276432863674 ) ) ;
#7200=CARTESIAN_POINT ( 'NONE',  ( 162.0192538899617318, 268.0510789565263394, -17.53028463913764057 ) ) ;
#7201=DIRECTION ( 'NONE',  ( -0.8660254037844387076, -0.4999999999999998890, -0.000000000000000000 ) ) ;
#7202=CARTESIAN_POINT ( 'NONE',  ( 171.4770449210933236, 289.0940507889877722, 4.287227504194440542 ) ) ;
#7204=ORIENTED_EDGE ( 'NONE', *, *, #62645, .T. ) ;
#7205=CARTESIAN_POINT ( 'NONE',  ( 190.7661460928718498, 300.2303379334758233, -3.568894913151918313 ) ) ;
#7208=CARTESIAN_POINT ( 'NONE',  ( 202.9521567073010146, 278.0333832980851412, 15.07843176052885781 ) ) ;
#7211=CARTESIAN_POINT ( 'NONE',  ( 147.9974455564266691, 274.3079002362971437, -10.09869768668086820 ) ) ;
#7212=CARTESIAN_POINT ( 'NONE',  ( 167.7560327080170453, 284.3066376844275283, -7.994707968029326928 ) ) ;
#7215=CARTESIAN_POINT ( 'NONE',  ( 159.3586121662929713, 254.6297824347537642, -15.50090345830412630 ) ) ;
#7217=CARTESIAN_POINT ( 'NONE',  ( 35.87196818813498567, 201.5177522451419350, 5.000000000000046185 ) ) ;
#7218=CARTESIAN_POINT ( 'NONE',  ( 114.8970466070627907, 227.9548013555409796, -4.594050593750042211 ) ) ;
#7219=CARTESIAN_POINT ( 'NONE',  ( 199.1867231605587278, 285.6454706231928071, -17.41989184023605475 ) ) ;
#7223=CARTESIAN_POINT ( 'NONE',  ( 33.24700223256990483, 183.8768266524160140, -9.188101187500091527 ) ) ;
#7225=CARTESIAN_POINT ( 'NONE',  ( -27.42236680055714260, 166.5217562850347406, 1.224646799147364892E-15 ) ) ;
#7228=CARTESIAN_POINT ( 'NONE',  ( 178.4621772040343899, 265.6203404136728068, 16.07317361885528584 ) ) ;
#7229=CARTESIAN_POINT ( 'NONE',  ( 26.96143514339544467, 174.8262482093457777, 3.021315404115420679E-15 ) ) ;
#7230=CARTESIAN_POINT ( 'NONE',  ( 190.1607982559816890, 301.2788311432216233, -4.972636536415983244 ) ) ;
#7234=CARTESIAN_POINT ( 'NONE',  ( 151.2546443255573934, 275.3395117651207897, -9.775857568146751220 ) ) ;
#7236=CARTESIAN_POINT ( 'NONE',  ( 101.7620676594010405, 242.8927522451419634, 2.944929066748280225E-16 ) ) ;
#7237=CARTESIAN_POINT ( 'NONE',  ( 194.6626581126282929, 293.0278785836280235, -14.76912774068482292 ) ) ;
#7238=ORIENTED_EDGE ( 'NONE', *, *, #25961, .F. ) ;
#7239=EDGE_CURVE ( 'NONE', #1456, #11457, #92521, .T. ) ;
#7241=CARTESIAN_POINT ( 'NONE',  ( 163.0309151244508712, 248.2691671304387739, 11.27270415168660200 ) ) ;
#7242=CARTESIAN_POINT ( 'NONE',  ( 154.9082074166165910, 263.9767827779738241, 17.34157506132131488 ) ) ;
#7243=CARTESIAN_POINT ( 'NONE',  ( 14.24839638916628459, 179.0333772461660544, 9.188101187500095079 ) ) ;
#7245=CARTESIAN_POINT ( 'NONE',  ( 192.2881851781887406, 272.0424645381762048, 14.23089303299685149 ) ) ;
#7248=CARTESIAN_POINT ( 'NONE',  ( 174.8809725116003619, 286.3757395011697326, 10.48282596314093063 ) ) ;
#7249=CARTESIAN_POINT ( 'NONE',  ( 77.36034478572226192, 203.2202760586659736, -5.415160957724236172E-17 ) ) ;
#7250=CARTESIAN_POINT ( 'NONE',  ( 200.4592688079413847, 283.4413569069752725, 18.39277739746426832 ) ) ;
#7255=( BOUNDED_CURVE ( )  B_SPLINE_CURVE ( 2, ( #14900, #45790, #76710, #100029, #30615, #61500, #31095, #22996, #15385 ),
 .UNSPECIFIED., .F., .T. ) 
 B_SPLINE_CURVE_WITH_KNOTS ( ( 3, 2, 2, 2, 3 ),
 ( 0.9233870967741935054, 0.9247311827956988806, 0.9274193548387096309, 0.9301075268817203812, 0.9314516129032257563 ),
 .UNSPECIFIED. ) 
 CURVE ( )  GEOMETRIC_REPRESENTATION_ITEM ( )  RATIONAL_B_SPLINE_CURVE ( ( 0.9330127018922194093, 0.9330127018922194093, 1.000000000000000000, 0.8660254037844387076, 1.000000000000000000, 0.8660254037844387076, 1.000000000000000000, 0.9330127018922194093, 0.9330127018922194093 ) ) 
 REPRESENTATION_ITEM ( '' )  );
#7256=CARTESIAN_POINT ( 'NONE',  ( 162.2803608993413320, 267.3877610371002902, 16.48173369095244567 ) ) ;
#7257=CARTESIAN_POINT ( 'NONE',  ( 14.02286894203806433, 172.2365022471902307, 10.00000000000009592 ) ) ;
#7258=CARTESIAN_POINT ( 'NONE',  ( 163.8111161534324935, 246.9178193081252743, -7.110480325054721717 ) ) ;
#7259=CARTESIAN_POINT ( 'NONE',  ( 140.0928864244750685, 245.5643266524160424, -9.188101187500093303 ) ) ;
#7261=CARTESIAN_POINT ( 'NONE',  ( 164.0665640930923246, 260.4805839323781811, -16.15133822266555441 ) ) ;
#7263=CARTESIAN_POINT ( 'NONE',  ( 196.4338619668326942, 281.5298852278613140, -17.66916360587062584 ) ) ;
#7269=CARTESIAN_POINT ( 'NONE',  ( 190.9907605556751093, 299.8412942717858414, 8.799173206188184437 ) ) ;
#7270=FACE_OUTER_BOUND ( 'NONE', #9816, .T. ) ;
#7272=CARTESIAN_POINT ( 'NONE',  ( 196.5433769452094737, 289.0926436443681382, 16.88005588253986033 ) ) ;
#7275=CARTESIAN_POINT ( 'NONE',  ( 165.9969153545198708, 246.1123342570000716, -1.176638740111072723 ) ) ;
#7277=CARTESIAN_POINT ( 'NONE',  ( -16.08955603893133812, 171.5177522451419350, 5.000000000000046185 ) ) ;
#7278=CARTESIAN_POINT ( 'NONE',  ( 29.78943643340442549, 199.5530062829863027, -4.648177544792955347E-16 ) ) ;
#7280=EDGE_CURVE ( 'NONE', #72868, #26607, #98799, .T. ) ;
#7281=CARTESIAN_POINT ( 'NONE',  ( 200.7975900406536596, 281.6935573902783858, -16.84479620147121537 ) ) ;
#7283=CARTESIAN_POINT ( 'NONE',  ( 96.56591523669446531, 219.8927522451417929, -10.00000000000009237 ) ) ;
#7284=ADVANCED_FACE ( 'NONE', ( #6629 ), #63314, .T. ) ;
#7285=CARTESIAN_POINT ( 'NONE',  ( 148.1846377449773513, 246.3615022471901739, 5.000000000000051514 ) ) ;
#7286=CARTESIAN_POINT ( 'NONE',  ( 201.1679199471075492, 282.2139371290980989, -16.62385308864941535 ) ) ;
#7290=CARTESIAN_POINT ( 'NONE',  ( 190.0274641710971082, 301.5097725526222803, 3.738976720635653450 ) ) ;
#7291=DIRECTION ( 'NONE',  ( -0.8660254037844387076, -0.4999999999999998890, -0.000000000000000000 ) ) ;
#7293=B_SPLINE_CURVE_WITH_KNOTS ( 'NONE', 3,
 ( #39344, #46969, #31746, #93093, #99686, #16067, #100193, #70769, #6969, #30778, #7982, #24172, #38858, #77888, #1384, #92608 ),
 .UNSPECIFIED., .F., .F.,
 ( 4, 2, 2, 2, 2, 2, 2, 4 ),
 ( -9.572876425213601166E-06, 3.117184193876883545E-05, 7.191656030275126528E-05, 0.0001534059970307206650, 0.0003163848704866175331, 0.0006423426173984245506, 0.0009683003643102314597, 0.001294258111222038260 ),
 .UNSPECIFIED. ) ;
#7297=B_SPLINE_CURVE_WITH_KNOTS ( 'NONE', 3,
 ( #15027, #92583, #836, #84975, #86009, #61128, #30246, #7435, #15520, #84485, #92104, #39808, #8941, #23125, #24143, #38827, #22649, #47924, #16039, #77857, #54018, #45919, #70739, #76837, #39314, #94082, #38328, #69734, #46422, #31231, #100165, #77347, #340, #55028, #16535, #47432, #1351, #86503, #63137, #17031, #62117, #93064, #23619, #54512, #78863, #85491, #46940, #37829 ),
 .UNSPECIFIED., .F., .F.,
 ( 4, 2, 2, 2, 2, 2, 2, 2, 2, 2, 2, 2, 2, 2, 2, 2, 2, 2, 2, 2, 2, 2, 2, 4 ),
 ( 0.002769618252134798449, 0.002972599584400432374, 0.003175580916666066733, 0.003277071582798824281, 0.003378562248931581830, 0.003480052915064339378, 0.003581543581197097360, 0.003784524913462612456, 0.003987506245728127986, 0.004393468910259121750, 0.005205394239320976571, 0.006017319568382830525, 0.006829244897444684478, 0.007641170226506538432, 0.007742660892639252612, 0.007793406225705632254, 0.007844151558772011895, 0.007894896891838391537, 0.007945642224904771178, 0.008047132891037544339, 0.008250114223303045558, 0.008453095555568546776, 0.008859058220099485029, 0.009265020884630421547 ),
 .UNSPECIFIED. ) ;
#7298=CARTESIAN_POINT ( 'NONE',  ( 149.7200635338602410, 271.3242383773507527, -12.12223662813266500 ) ) ;
#7300=ORIENTED_EDGE ( 'NONE', *, *, #3882, .T. ) ;
#7301=CARTESIAN_POINT ( 'NONE',  ( 102.5829875751790468, 230.0333772461660828, 9.188101187500095079 ) ) ;
#7302=CARTESIAN_POINT ( 'NONE',  ( 203.6711767524177219, 277.8781691579084736, 15.55577513624845132 ) ) ;
#7304=CARTESIAN_POINT ( 'NONE',  ( 181.1220979881137794, 271.7127838054424274, -16.46451683054539927 ) ) ;
#7312=CARTESIAN_POINT ( 'NONE',  ( 149.7489224357368869, 277.2657599369866830, -4.201129737586335011 ) ) ;
#7313=ORIENTED_EDGE ( 'NONE', *, *, #40123, .T. ) ;
#7314=CARTESIAN_POINT ( 'NONE',  ( 207.7655736232174206, 270.7864657513322300, 3.530742899761726949 ) ) ;
#7315=EDGE_CURVE ( 'NONE', #21409, #30521, #17866, .T. ) ;
#7317=CARTESIAN_POINT ( 'NONE',  ( 169.3571508527084291, 283.0956279022483955, 12.63651818596384935 ) ) ;
#7323=CARTESIAN_POINT ( 'NONE',  ( 200.3935147155627305, 278.4751539331289223, -15.53795961942556936 ) ) ;
#7325=CARTESIAN_POINT ( 'NONE',  ( 122.5466773502276254, 234.8927522451417360, -10.00000000000009237 ) ) ;
#7326=ORIENTED_EDGE ( 'NONE', *, *, #41107, .T. ) ;
#7327=B_SPLINE_CURVE_WITH_KNOTS ( 'NONE', 3,
 ( #29257, #67752, #91088, #44930 ),
 .UNSPECIFIED., .F., .F.,
 ( 4, 4 ),
 ( 0.000000000000000000, 0.0003654356002692110196 ),
 .UNSPECIFIED. ) ;
#7328=CARTESIAN_POINT ( 'NONE',  ( 202.6551236945213361, 279.6380246773706517, 15.55476940527561425 ) ) ;
#7329=CARTESIAN_POINT ( 'NONE',  ( 186.6492374970252683, 259.8286487250865662, 2.870770739009044004 ) ) ;
#7332=CARTESIAN_POINT ( 'NONE',  ( 169.7764802368346295, 254.5828642248548874, 11.32100359419826141 ) ) ;
#7333=CARTESIAN_POINT ( 'NONE',  ( 158.4097777638608875, 281.2458747730524919, 2.072559225148736584 ) ) ;
#7335=CARTESIAN_POINT ( 'NONE',  ( 155.5849683057210768, 261.1659253309343853, -17.10048217785023539 ) ) ;
#7337=CARTESIAN_POINT ( 'NONE',  ( 2.096977440541873516, 182.0177522451419350, 5.000000000000046185 ) ) ;
#7338=CARTESIAN_POINT ( 'NONE',  ( 193.0018192671613519, 266.8968850134971262, -11.37984971561561842 ) ) ;
#7341=CARTESIAN_POINT ( 'NONE',  ( 203.5339801188816580, 278.1158006978202479, -14.61497198938462105 ) ) ;
#7344=CARTESIAN_POINT ( 'NONE',  ( 162.1569020246023456, 250.8293869144198140, -12.73294256043488026 ) ) ;
#7345=CARTESIAN_POINT ( 'NONE',  ( -10.75808714510939090, 164.5958772461660544, -9.188101187500095079 ) ) ;
#7347=ORIENTED_EDGE ( 'NONE', *, *, #70785, .F. ) ;
#7349=CARTESIAN_POINT ( 'NONE',  ( 165.7655117394099591, 246.1853102806505831, -2.777750405961522784 ) ) ;
#7351=CYLINDRICAL_SURFACE ( 'NONE', #11418, 17.82106496071139645 ) ;
#7354=CARTESIAN_POINT ( 'NONE',  ( 158.4485968073939546, 275.2084588272041401, -13.86993402366507944 ) ) ;
#7356=CARTESIAN_POINT ( 'NONE',  ( 150.2414568861867679, 276.5756577973505728, 3.692317353432758242 ) ) ;
#7357=CARTESIAN_POINT ( 'NONE',  ( 19.71535529843806245, 176.0643266524160424, 9.188101187500095079 ) ) ;
#7358=CARTESIAN_POINT ( 'NONE',  ( 114.4904897814500515, 249.1589784336661069, -6.496448406907675876E-16 ) ) ;
#7360=CARTESIAN_POINT ( 'NONE',  ( 196.2076153567640517, 275.2112971549272515, 16.01702815084858855 ) ) ;
#7361=CARTESIAN_POINT ( 'NONE',  ( 153.5108272444703630, 274.2076890947117818, -12.10491928328822020 ) ) ;
#7362=CARTESIAN_POINT ( 'NONE',  ( 178.5305822085327350, 283.8616835467783517, -14.84070646491336554 ) ) ;
#7363=CARTESIAN_POINT ( 'NONE',  ( 190.5307517086160942, 299.7706353115473235, -5.301913143154168395 ) ) ;
#7366=CARTESIAN_POINT ( 'NONE',  ( 207.2337123599961899, 271.7076764818092443, -5.443417788256701861 ) ) ;
#7369=CARTESIAN_POINT ( 'NONE',  ( 189.2674249387218595, 262.5240697966969492, 8.133003587096190756 ) ) ;
#7370=CARTESIAN_POINT ( 'NONE',  ( 168.2540853406581789, 278.3014265215951468, 14.24901084982592891 ) ) ;
#7371=CARTESIAN_POINT ( 'NONE',  ( 175.4112849191630232, 256.5165010529896676, -10.85204326945974174 ) ) ;
#7374=CARTESIAN_POINT ( 'NONE',  ( 181.0085414047549932, 266.3579488787440255, -14.72432788045776242 ) ) ;
#7375=ORIENTED_EDGE ( 'NONE', *, *, #55972, .T. ) ;
#7378=CARTESIAN_POINT ( 'NONE',  ( 185.0762662215304601, 269.6689080139000225, 15.62688583476976056 ) ) ;
#7379=CARTESIAN_POINT ( 'NONE',  ( 88.45577462806285496, 228.0024278399160664, -9.188101187500093303 ) ) ;
#7382=CARTESIAN_POINT ( 'NONE',  ( 159.0906380018002153, 259.2649656523443582, -17.57712761084927067 ) ) ;
#7384=CARTESIAN_POINT ( 'NONE',  ( 195.2852648346649005, 278.9764887875277850, 16.29283862267904226 ) ) ;
#7385=CARTESIAN_POINT ( 'NONE',  ( -22.42236680055709641, 157.8615022471902591, 0.000000000000000000 ) ) ;
#7386=FACE_OUTER_BOUND ( 'NONE', #4057, .T. ) ;
#7387=CARTESIAN_POINT ( 'NONE',  ( 149.8377514179171328, 271.8685197739567343, -11.50488653483219537 ) ) ;
#7391=VERTEX_POINT ( 'NONE', #69906 ) ;
#7393=CARTESIAN_POINT ( 'NONE',  ( 178.3972326700113911, 280.2571014150069004, 15.75398658722560974 ) ) ;
#7394=CARTESIAN_POINT ( 'NONE',  ( 199.1702776998127433, 269.7223802865422613, 9.247749995336496553 ) ) ;
#7395=CARTESIAN_POINT ( 'NONE',  ( 196.6288634187112052, 290.0758136547079289, -16.31544900032282186 ) ) ;
#7399=CARTESIAN_POINT ( 'NONE',  ( 183.6390766470569247, 264.5367329039647757, -13.38022241395614387 ) ) ;
#7401=CARTESIAN_POINT ( 'NONE',  ( 172.2491325584012998, 253.6515925324379737, -8.857966409642921590 ) ) ;
#7402=CARTESIAN_POINT ( 'NONE',  ( 152.9920137376499838, 265.6570543845515431, 16.15798175643282164 ) ) ;
#7408=CARTESIAN_POINT ( 'NONE',  ( 166.8517212214031815, 249.4051957966311193, 6.977118993877414965 ) ) ;
#7415=CARTESIAN_POINT ( 'NONE',  ( 192.9271913386342021, 296.4872977703604420, -11.97251109041730288 ) ) ;
#7416=CARTESIAN_POINT ( 'NONE',  ( 200.6985908945154335, 283.0268388936558495, -17.74173253065502820 ) ) ;
#7417=CARTESIAN_POINT ( 'NONE',  ( -27.42236680055714260, 166.5217562850347406, 1.224646799147364892E-15 ) ) ;
#7419=CARTESIAN_POINT ( 'NONE',  ( 110.4458243891416487, 246.1199935810941213, 2.679491924311251605 ) ) ;
#7421=CARTESIAN_POINT ( 'NONE',  ( 154.3830968479286980, 271.8928371781024680, -14.51477723473457360 ) ) ;
#7422=ORIENTED_EDGE ( 'NONE', *, *, #31757, .F. ) ;
#7423=CARTESIAN_POINT ( 'NONE',  ( -22.42236680055709641, 157.8615022471902591, 0.000000000000000000 ) ) ;
#7426=ORIENTED_EDGE ( 'NONE', *, *, #65463, .F. ) ;
#7427=CARTESIAN_POINT ( 'NONE',  ( 172.5528256599575911, 270.8946351329052504, 16.43625532445414805 ) ) ;
#7429=CARTESIAN_POINT ( 'NONE',  ( 170.7847687409972366, 255.2762072239008830, -11.40120098929249437 ) ) ;
#7430=CARTESIAN_POINT ( 'NONE',  ( 185.2570508126727873, 282.0811717828997303, -17.42469797758589678 ) ) ;
#7431=CARTESIAN_POINT ( 'NONE',  ( 206.2849804695184446, 273.3509283188774930, -9.687080623179198824 ) ) ;
#7432=CARTESIAN_POINT ( 'NONE',  ( 197.9901163037401943, 272.1418500761980681, -13.83221381771805625 ) ) ;
#7435=CARTESIAN_POINT ( 'NONE',  ( 171.6432221199900141, 250.7645099467145542, -5.701615499911769191 ) ) ;
#7437=CARTESIAN_POINT ( 'NONE',  ( 178.0376065834567498, 255.4657367285703060, 5.065382276933755534 ) ) ;
#7438=CARTESIAN_POINT ( 'NONE',  ( 111.8924135700967355, 247.6589784336661069, -6.496448406907675876E-16 ) ) ;
#7440=CARTESIAN_POINT ( 'NONE',  ( 186.6478515376321070, 262.8385383458236788, -9.776049215535964620 ) ) ;
#7442=CARTESIAN_POINT ( 'NONE',  ( 187.9511160036650779, 273.8878269306266020, 16.63997191726063463 ) ) ;
#7448=CARTESIAN_POINT ( 'NONE',  ( 192.1298366743677946, 297.8683565605218746, 11.31374600872841008 ) ) ;
#7458=CARTESIAN_POINT ( 'NONE',  ( 188.5893119661470223, 266.4960058560010339, -11.84220618477010767 ) ) ;
#7463=CARTESIAN_POINT ( 'NONE',  ( 184.1240780222136095, 289.0015729834078684, -14.54488561116068901 ) ) ;
#7464=DIRECTION ( 'NONE',  ( 0.4999999999999998890, -0.8660254037844385966, 0.000000000000000000 ) ) ;
#7465=CARTESIAN_POINT ( 'NONE',  ( 201.4066285247549786, 281.8004817444100354, -17.79749223817309201 ) ) ;
#7467=CARTESIAN_POINT ( 'NONE',  ( 190.8907028847385448, 300.0145992415348815, -5.421341690443150618 ) ) ;
#7468=CARTESIAN_POINT ( 'NONE',  ( 192.1379539184286216, 266.4068991655999525, -11.89392551111776619 ) ) ;
#7470=CARTESIAN_POINT ( 'NONE',  ( 192.8090185325462471, 271.7505329995509555, -14.77105383832748942 ) ) ;
#7471=CARTESIAN_POINT ( 'NONE',  ( 9.458193372709645885, 176.2677522451418497, 10.00000000000009592 ) ) ;
#7474=CARTESIAN_POINT ( 'NONE',  ( 192.2414585986055897, 284.0409920799691008, -16.66054451170961315 ) ) ;
#7476=CARTESIAN_POINT ( 'NONE',  ( 67.72511797709034909, 222.1589784336661637, -6.496448406907675876E-16 ) ) ;
#7477=CARTESIAN_POINT ( 'NONE',  ( 28.60096323907606219, 193.9865022471902876, 10.00000000000009415 ) ) ;
#7478=CARTESIAN_POINT ( 'NONE',  ( 147.5749398328735822, 275.0397016159798227, -4.620786157167191099 ) ) ;
#7481=B_SPLINE_CURVE_WITH_KNOTS ( 'NONE', 3,
 ( #38563, #14776, #30969, #70469 ),
 .UNSPECIFIED., .F., .F.,
 ( 4, 4 ),
 ( 0.03663086090994036731, 0.04529359754877385069 ),
 .UNSPECIFIED. ) ;
#7484=CARTESIAN_POINT ( 'NONE',  ( 207.7666684749232786, 270.7845694125510931, -6.630926507062123498 ) ) ;
#7489=CARTESIAN_POINT ( 'NONE',  ( 144.6270795744234476, 268.7413018095040798, -2.761272660171008000E-15 ) ) ;
#7491=CARTESIAN_POINT ( 'NONE',  ( 164.7073188963636028, 245.3655506234856034, -4.606661621890939529 ) ) ;
#7492=CARTESIAN_POINT ( 'NONE',  ( 157.3025066944120454, 258.1910615777721887, 18.21299529665260053 ) ) ;
#7493=CARTESIAN_POINT ( 'NONE',  ( -19.92236680055706088, 153.5313752282680184, 0.000000000000000000 ) ) ;
#7494=CARTESIAN_POINT ( 'NONE',  ( 47.75258065019424691, 204.5024278399160949, 9.188101187500095079 ) ) ;
#7495=CARTESIAN_POINT ( 'NONE',  ( 163.9488516144422192, 247.0953858819488005, -6.080757577568762784 ) ) ;
#7497=CYLINDRICAL_SURFACE ( 'NONE', #30383, 17.82106496071139645 ) ;
#7498=CARTESIAN_POINT ( 'NONE',  ( 144.9642793207625004, 248.3768266524159856, -9.188101187500091527 ) ) ;
#7499=CYLINDRICAL_SURFACE ( 'NONE', #2118, 10.00000000000010658 ) ;
#7500=CARTESIAN_POINT ( 'NONE',  ( 200.2187516388992492, 271.0431823872724522, -11.39384425366991493 ) ) ;
#7503=CARTESIAN_POINT ( 'NONE',  ( 151.1126408083691501, 268.9122237844355254, -15.82705194100464396 ) ) ;
#7504=CARTESIAN_POINT ( 'NONE',  ( 146.8358616138309571, 276.3198226421291679, 4.054088818585255716 ) ) ;
#7506=CARTESIAN_POINT ( 'NONE',  ( 56.95410056540391253, 209.8149278399160949, -9.188101187500095079 ) ) ;
#7508=CARTESIAN_POINT ( 'NONE',  ( 175.7685826524176491, 291.0674233232674624, 2.543747227769448394 ) ) ;
#7509=CARTESIAN_POINT ( 'NONE',  ( 198.3150362131025588, 287.1552767044814800, 18.53472937702030521 ) ) ;
#7511=CARTESIAN_POINT ( 'NONE',  ( 201.4689129737137989, 281.6926019142917994, 17.66990927715608706 ) ) ;
#7512=EDGE_CURVE ( 'NONE', #51824, #20349, #95241, .T. ) ;
#7513=B_SPLINE_CURVE_WITH_KNOTS ( 'NONE', 3,
 ( #68668, #53467, #24073, #52978, #84420, #68175, #77800, #46354, #14966, #69169, #6393, #54966, #93003, #99593, #77278, #70161, #23556, #60558 ),
 .UNSPECIFIED., .F., .F.,
 ( 4, 2, 2, 2, 2, 2, 2, 2, 4 ),
 ( 0.002569504393709426404, 0.002648854729461323342, 0.002728205065213220280, 0.002807555400965117652, 0.002886905736717014590, 0.003045606408220883927, 0.003204307079724752830, 0.003839109765740250126, 0.005108715137771275075 ),
 .UNSPECIFIED. ) ;
#7517=CARTESIAN_POINT ( 'NONE',  ( 109.6465072765698636, 224.1115022471901739, -5.000000000000041744 ) ) ;
#7518=CARTESIAN_POINT ( 'NONE',  ( 161.0952649348064938, 251.6218116045831437, 13.81854265722852482 ) ) ;
#7519=CARTESIAN_POINT ( 'NONE',  ( 207.0548180518391916, 272.0175305127218053, 7.721676452263806389 ) ) ;
#7525=CARTESIAN_POINT ( 'NONE',  ( 159.8946522441011382, 253.7013337850969492, -16.68230890105693121 ) ) ;
#7526=CARTESIAN_POINT ( 'NONE',  ( 186.8357760858314975, 276.5851586346784075, -17.24064928530544094 ) ) ;
#7527=CARTESIAN_POINT ( 'NONE',  ( -17.42236680055705023, 149.2012482093457777, 0.000000000000000000 ) ) ;
#7528=EDGE_CURVE ( 'NONE', #83021, #81006, #13504, .T. ) ;
#7529=ORIENTED_EDGE ( 'NONE', *, *, #61826, .F. ) ;
#7531=CARTESIAN_POINT ( 'NONE',  ( 207.6918009085542849, 270.9142438413412037, 7.009114282139513818 ) ) ;
#7532=CARTESIAN_POINT ( 'NONE',  ( 147.9311236323648870, 274.4227731784279172, -7.799459659034405412 ) ) ;
#7533=ADVANCED_FACE ( 'NONE', ( #23055 ), #47726, .F. ) ;
#7536=EDGE_LOOP ( 'NONE', ( #43758, #94952, #84107, #75164 ) ) ;
#7539=CARTESIAN_POINT ( 'NONE',  ( 188.1018771210319471, 260.4230313274653099, 6.875771660441075461 ) ) ;
#7540=CARTESIAN_POINT ( 'NONE',  ( -22.42236680055709641, 157.8615022471902591, 0.000000000000000000 ) ) ;
#7541=ORIENTED_EDGE ( 'NONE', *, *, #93952, .F. ) ;
#7543=CARTESIAN_POINT ( 'NONE',  ( 206.4640281786353171, 273.0408085897082060, -10.81921452789957883 ) ) ;
#7544=VERTEX_POINT ( 'NONE', #94013 ) ;
#7545=CARTESIAN_POINT ( 'NONE',  ( 174.6338837768408609, 286.4401551613050856, 11.66525039651988749 ) ) ;
#7546=CARTESIAN_POINT ( 'NONE',  ( 159.2472135755374154, 282.4118482373870052, -3.281722807136270958 ) ) ;
#7548=CARTESIAN_POINT ( 'NONE',  ( 162.6257765080958677, 248.9708877980734485, -10.42859054881151160 ) ) ;
#7549=CARTESIAN_POINT ( 'NONE',  ( 163.7729086741176161, 246.9839966035275438, 6.099406794390714204 ) ) ;
#7550=CARTESIAN_POINT ( 'NONE',  ( 188.5838923881401001, 295.0354966342055718, -11.12588321966210714 ) ) ;
#7551=CARTESIAN_POINT ( 'NONE',  ( 164.3625597711517230, 265.6729452914248668, -17.82104740451561753 ) ) ;
#7552=B_SPLINE_CURVE_WITH_KNOTS ( 'NONE', 3,
 ( #7354, #77779, #100081, #23539 ),
 .UNSPECIFIED., .F., .F.,
 ( 4, 4 ),
 ( 0.008629964147991740775, 0.01453130706412321220 ),
 .UNSPECIFIED. ) ;
#7553=CARTESIAN_POINT ( 'NONE',  ( 135.5998589986957370, 261.3464784336661637, 1.353441290958777525E-15 ) ) ;
#7555=CARTESIAN_POINT ( 'NONE',  ( 178.9693536223838635, 258.2551845487027435, 9.752734003342059310 ) ) ;
#7556=CARTESIAN_POINT ( 'NONE',  ( 74.81622161422296813, 207.8768266524159856, -9.188101187500091527 ) ) ;
#7557=ORIENTED_EDGE ( 'NONE', *, *, #35687, .T. ) ;
#7560=CARTESIAN_POINT ( 'NONE',  ( 181.4954090331713417, 255.0423029034424189, 0.9094182891644410072 ) ) ;
#7564=ORIENTED_EDGE ( 'NONE', *, *, #90388, .F. ) ;
#7566=CARTESIAN_POINT ( 'NONE',  ( 90.33589715100974615, 211.4155109091896065, 2.679491924311254714 ) ) ;
#7568=CARTESIAN_POINT ( 'NONE',  ( 197.9225324884813801, 286.9052520424737622, 16.93390111457149416 ) ) ;
#7569=CARTESIAN_POINT ( 'NONE',  ( 191.4852287632733123, 298.9848502134979071, -9.870565261052552941 ) ) ;
#7570=B_SPLINE_SURFACE_WITH_KNOTS ( 'NONE', 3, 1, ( 
 ( #88917, #30396 ),
 ( #22298, #67024 ),
 ( #84634, #29898 ),
 ( #92251, #14699 ),
 ( #53198, #15685 ),
 ( #22801, #15175 ),
 ( #61288, #78009 ),
 ( #92730, #84153 ),
 ( #82291, #97951 ),
 ( #53680, #76510 ),
 ( #68884, #45582 ),
 ( #58907, #46077 ),
 ( #12, #38981 ),
 ( #93227, #76988 ),
 ( #7594, #7093 ),
 ( #23788, #91735 ),
 ( #5241, #499 ),
 ( #61784, #16197 ),
 ( #46579, #37975 ),
 ( #38482, #74664 ),
 ( #36121, #99811 ),
 ( #8601, #62271 ),
 ( #69396, #69887 ),
 ( #30896, #23281 ),
 ( #54170, #31387 ),
 ( #77516, #60770 ),
 ( #54673, #85137 ),
 ( #1000, #8107 ),
 ( #12862, #85657 ),
 ( #47089, #39466 ),
 ( #43721, #51322 ),
 ( #70391, #89876 ),
 ( #20451, #94235 ),
 ( #94729, #33396 ) ),
 .UNSPECIFIED., .T., .F., .F.,
 ( 4, 2, 2, 2, 2, 2, 2, 2, 2, 2, 2, 2, 2, 2, 2, 2, 4 ),
 ( 2, 2 ),
 ( 0.000000000000000000, 0.06250000000000000000, 0.1250000000000000000, 0.1875000000000000000, 0.2500000000000000000, 0.3125000000000000000, 0.3750000000000000000, 0.4375000000000000000, 0.5000000000000000000, 0.5625000000000000000, 0.6250000000000000000, 0.6875000000000000000, 0.7500000000000000000, 0.8125000000000000000, 0.8750000000000000000, 0.9375000000000000000, 1.000000000000000000 ),
 ( 0.000000000000000000, 1.000000000000000000 ),
 .UNSPECIFIED. ) ;
#7573=CARTESIAN_POINT ( 'NONE',  ( 193.7706395672514645, 295.0264025848412075, 15.16938698680137065 ) ) ;
#7576=CARTESIAN_POINT ( 'NONE',  ( 81.44681538588882574, 208.6423013555409796, -4.594050593750043987 ) ) ;
#7583=EDGE_CURVE ( 'NONE', #14234, #64644, #73493, .T. ) ;
#7584=CARTESIAN_POINT ( 'NONE',  ( 165.3478801264585627, 285.2307890726268056, 0.5090311687081423564 ) ) ;
#7586=PLANE ( 'NONE',  #73644 ) ;
#7587=CARTESIAN_POINT ( 'NONE',  ( 99.70756906128829655, 216.8262482093457493, 3.021315404115420679E-15 ) ) ;
#7588=ORIENTED_EDGE ( 'NONE', *, *, #22472, .F. ) ;
#7592=EDGE_CURVE ( 'NONE', #47832, #42238, #49255, .T. ) ;
#7594=CARTESIAN_POINT ( 'NONE',  ( 201.1679199471075492, 282.2139371290980989, -16.62385308864941535 ) ) ;
#7599=CARTESIAN_POINT ( 'NONE',  ( 197.7849526899220223, 266.3861572259672243, 4.467793449146438611 ) ) ;
#7600=CARTESIAN_POINT ( 'NONE',  ( 181.4735074999749145, 292.1586133693310785, 10.55809797880889001 ) ) ;
#7603=CARTESIAN_POINT ( 'NONE',  ( 198.5109395995180535, 266.2319359199144060, 1.007832260215294928 ) ) ;
#7604=EDGE_CURVE ( 'NONE', #31824, #5449, #85433, .T. ) ;
#7605=CARTESIAN_POINT ( 'NONE',  ( 156.8938808821919793, 272.5684933834573940, 14.39157411223618688 ) ) ;
#7606=ORIENTED_EDGE ( 'NONE', *, *, #82998, .T. ) ;
#7607=CARTESIAN_POINT ( 'NONE',  ( 190.9335643195044838, 299.9403610588350944, -4.692880224846124548 ) ) ;
#7608=CARTESIAN_POINT ( 'NONE',  ( 202.7865629936218284, 279.4103651332174536, 17.10878160033216133 ) ) ;
#7610=CARTESIAN_POINT ( 'NONE',  ( 155.6435836392643637, 261.0644005951349982, 17.58841156286628049 ) ) ;
#7613=EDGE_CURVE ( 'NONE', #23003, #5719, #1282, .T. ) ;
#7615=CARTESIAN_POINT ( 'NONE',  ( 164.6292270401010853, 284.5473998418419797, -3.121378508483925174 ) ) ;
#7617=CARTESIAN_POINT ( 'NONE',  ( 198.6562788533279615, 286.5642271139020636, 17.47134757795404525 ) ) ;
#7618=CARTESIAN_POINT ( 'NONE',  ( 142.3930928536209422, 263.0177522451418781, 5.000000000000046185 ) ) ;
#7620=ORIENTED_EDGE ( 'NONE', *, *, #62851, .T. ) ;
#7621=CARTESIAN_POINT ( 'NONE',  ( 178.5504536548465353, 256.2493563142403445, 8.783846101583462129 ) ) ;
#7624=CARTESIAN_POINT ( 'NONE',  ( 31.32559514186443295, 179.7048013555409796, 4.594050593750051981 ) ) ;
#7627=CARTESIAN_POINT ( 'NONE',  ( 181.1531766136657495, 275.2180700950633536, -16.44407546173127344 ) ) ;
#7630=CARTESIAN_POINT ( 'NONE',  ( 157.6921299354026189, 257.5162143285667753, -18.18720974599499840 ) ) ;
#7632=ADVANCED_FACE ( 'NONE', ( #64075 ), #99465, .F. ) ;
#7633=CARTESIAN_POINT ( 'NONE',  ( 175.6261675056671550, 253.6354083681499105, -3.856844943141242155 ) ) ;
#7634=CARTESIAN_POINT ( 'NONE',  ( 187.5747766728329964, 259.5710330847772411, -0.7742262142532535529 ) ) ;
#7635=EDGE_CURVE ( 'NONE', #49046, #64894, #34712, .T. ) ;
#7637=CARTESIAN_POINT ( 'NONE',  ( 61.65426615018211010, 219.7365022471903160, 2.944929066748280225E-16 ) ) ;
#7639=CARTESIAN_POINT ( 'NONE',  ( 147.6140518775699491, 274.9719575673779559, 8.457032797753797126 ) ) ;
#7640=CARTESIAN_POINT ( 'NONE',  ( 25.77718602916411683, 191.8149278399160949, -9.188101187500095079 ) ) ;
#7643=CARTESIAN_POINT ( 'NONE',  ( 203.0652949094600501, 269.8798128736668218, -6.158547683694125752 ) ) ;
#7644=CARTESIAN_POINT ( 'NONE',  ( 151.0388915836658725, 269.0399611886400635, -14.24896787280406585 ) ) ;
#7645=CARTESIAN_POINT ( 'NONE',  ( 207.6508796976096107, 270.9851214578045528, 6.713685698622268383 ) ) ;
#7647=CARTESIAN_POINT ( 'NONE',  ( 188.9965416891025995, 268.2223090079140206, 13.67363464215795865 ) ) ;
#7648=CARTESIAN_POINT ( 'NONE',  ( 162.0898649156316935, 280.9600800141846548, -10.51109445094396833 ) ) ;
#7649=CARTESIAN_POINT ( 'NONE',  ( 179.6688721834134412, 263.0910175821119878, -13.35864055896102620 ) ) ;
#7654=CARTESIAN_POINT ( 'NONE',  ( 188.9004165423950212, 270.0841463155638849, -14.13780846912426448 ) ) ;
#7657=CARTESIAN_POINT ( 'NONE',  ( 159.0906380018002153, 259.2649656523443582, -17.57712761084927067 ) ) ;
#7662=CARTESIAN_POINT ( 'NONE',  ( 155.7054361929259301, 262.7846159439811800, -17.64293531980526808 ) ) ;
#7670=ORIENTED_EDGE ( 'NONE', *, *, #44948, .F. ) ;
#7672=CARTESIAN_POINT ( 'NONE',  ( 201.3911183001464451, 266.9640362439821502, -3.754059931952923534 ) ) ;
#7675=CARTESIAN_POINT ( 'NONE',  ( 153.2583947049096764, 265.1956690150883560, -17.64103123457563882 ) ) ;
#7680=CARTESIAN_POINT ( 'NONE',  ( 189.8314329296643450, 301.8493086226544619, -0.8085564604676659384 ) ) ;
#7681=CARTESIAN_POINT ( 'NONE',  ( 149.1486417047969155, 272.3139700178423368, -11.47583619705022606 ) ) ;
#7684=CARTESIAN_POINT ( 'NONE',  ( 158.8801886266397787, 265.4961833764209018, 16.91276571221451164 ) ) ;
#7686=CARTESIAN_POINT ( 'NONE',  ( 190.5477107455830321, 300.6086790531491033, 3.126266616601216963 ) ) ;
#7694=ORIENTED_EDGE ( 'NONE', *, *, #40866, .F. ) ;
#7695=CARTESIAN_POINT ( 'NONE',  ( 190.0914054637564163, 299.5768487891093628, 6.564776197388576762 ) ) ;
#7696=CARTESIAN_POINT ( 'NONE',  ( 75.78130554586792300, 207.8927522451418213, -10.00000000000009237 ) ) ;
#7697=CARTESIAN_POINT ( 'NONE',  ( 148.2159754900428936, 273.9293952882992471, 9.267836332806297150 ) ) ;
#7698=CARTESIAN_POINT ( 'NONE',  ( 190.5477107455830321, 300.6086790531491033, 3.126266616601216963 ) ) ;
#7699=CARTESIAN_POINT ( 'NONE',  ( 172.7484569319901482, 276.2894592982432869, -15.71612304295510043 ) ) ;
#7700=CARTESIAN_POINT ( 'NONE',  ( 146.8598618121150423, 276.2782530793093656, -0.7992850717744983680 ) ) ;
#7701=CARTESIAN_POINT ( 'NONE',  ( 147.5540328368684300, 275.0759135952944234, -4.750028533202499403 ) ) ;
#7703=VECTOR ( 'NONE', #88792, 1000.000000000000000 ) ;
#7704=DIRECTION ( 'NONE',  ( 0.4999999999999998890, -0.8660254037844385966, 0.000000000000000000 ) ) ;
#7705=FACE_OUTER_BOUND ( 'NONE', #59598, .T. ) ;
#7710=ORIENTED_EDGE ( 'NONE', *, *, #51836, .T. ) ;
#7711=CARTESIAN_POINT ( 'NONE',  ( 149.7662956631658631, 271.2441619804512243, -12.26682131771685036 ) ) ;
#7715=B_SPLINE_CURVE_WITH_KNOTS ( 'NONE', 3,
 ( #54312, #33543, #94375, #73914 ),
 .UNSPECIFIED., .F., .F.,
 ( 4, 4 ),
 ( 0.0008745192274822840206, 0.006137245505070649740 ),
 .UNSPECIFIED. ) ;
#7716=CARTESIAN_POINT ( 'NONE',  ( 43.39556388706024848, 195.8615022471902591, -10.00000000000009592 ) ) ;
#7718=CARTESIAN_POINT ( 'NONE',  ( 165.4078582752671878, 283.6377208367567846, -8.325660689787278912 ) ) ;
#7720=CARTESIAN_POINT ( 'NONE',  ( 162.8480293090835005, 248.5859346546387769, -9.753154585358942086 ) ) ;
#7723=CARTESIAN_POINT ( 'NONE',  ( 38.03703169759608471, 202.7677522451419350, -5.000000000000047962 ) ) ;
#7724=CARTESIAN_POINT ( 'NONE',  ( 121.9060058492368483, 247.3149278399160949, -9.188101187500095079 ) ) ;
#7726=CARTESIAN_POINT ( 'NONE',  ( 151.3999564459286375, 268.4145785023736153, -15.40574304386609050 ) ) ;
#7728=CARTESIAN_POINT ( 'NONE',  ( -22.42236680055709641, 157.8615022471902591, 0.000000000000000000 ) ) ;
#7729=CARTESIAN_POINT ( 'NONE',  ( 157.8763546842245376, 257.1971277035954699, 17.68444922773363004 ) ) ;
#7730=CARTESIAN_POINT ( 'NONE',  ( 172.6900760593800044, 250.5973497951363811, -4.149042267653843652 ) ) ;
#7731=CARTESIAN_POINT ( 'NONE',  ( 50.29670382169353360, 199.8458772461660260, 9.188101187500095079 ) ) ;
#7732=CARTESIAN_POINT ( 'NONE',  ( 178.7655400679708464, 291.8864583725769535, -5.901772721150448042 ) ) ;
#7734=DIRECTION ( 'NONE',  ( -0.8660254037844387076, -0.4999999999999998890, -0.000000000000000000 ) ) ;
#7735=ORIENTED_EDGE ( 'NONE', *, *, #9431, .F. ) ;
#7738=EDGE_CURVE ( 'NONE', #60977, #12604, #75831, .T. ) ;
#7741=CARTESIAN_POINT ( 'NONE',  ( 190.9335643195044838, 299.9403610588350944, -4.692880224846124548 ) ) ;
#7743=CARTESIAN_POINT ( 'NONE',  ( 191.2104420009116836, 280.2857515794617598, 17.80337293751487593 ) ) ;
#7744=CARTESIAN_POINT ( 'NONE',  ( 156.3864393596315381, 270.3627023744734856, -14.79408036704170470 ) ) ;
#7746=CARTESIAN_POINT ( 'NONE',  ( 109.4119587261636752, 220.6427522451417644, 1.119607411625061291E-15 ) ) ;
#7749=CARTESIAN_POINT ( 'NONE',  ( 163.4260108471723640, 247.5848412648317662, 10.45113099391573108 ) ) ;
#7751=CARTESIAN_POINT ( 'NONE',  ( 32.70573635520464251, 183.5643266524160140, 9.188101187500095079 ) ) ;
#7753=CARTESIAN_POINT ( 'NONE',  ( 195.9351945738247309, 273.3307776679702670, 15.22350882708002118 ) ) ;
#7754=CARTESIAN_POINT ( 'NONE',  ( 146.9709166616330549, 276.0859004375172390, 3.755270622130282732 ) ) ;
#7756=CARTESIAN_POINT ( 'NONE',  ( 198.2782625130438987, 277.4159975312159645, -15.37005889760090405 ) ) ;
#7757=CARTESIAN_POINT ( 'NONE',  ( 65.85835811776894388, 199.6423013555410080, -4.594050593750043987 ) ) ;
#7758=CARTESIAN_POINT ( 'NONE',  ( 164.4414259850711915, 245.8260906552167171, -6.983224448873608381 ) ) ;
#7760=CARTESIAN_POINT ( 'NONE',  ( 182.0338464029501040, 278.3680066549227945, 17.69288446120480174 ) ) ;
#7762=VERTEX_POINT ( 'NONE', #16244 ) ;
#7764=CARTESIAN_POINT ( 'NONE',  ( 23.90999230191038549, 184.6115022471902591, 10.00000000000009592 ) ) ;
#7765=B_SPLINE_CURVE_WITH_KNOTS ( 'NONE', 3,
 ( #38243, #61051, #6383, #37266, #84407, #14480, #77265, #45361, #14952, #22570, #76764, #91507, #24932, #69158, #100088, #76293, #99091, #45842, #22072, #52967, #71559, #30675, #92024, #9244, #37755, #92501, #68660, #99583, #23047, #79185, #53944, #84902, #40119, #71059, #94873, #1660, #63443, #94378, #55806, #86799, #48239, #40622, #2156, #29675, #33035, #63934, #25435, #56326 ),
 .UNSPECIFIED., .F., .F.,
 ( 4, 2, 2, 2, 2, 2, 2, 2, 2, 2, 2, 2, 2, 2, 2, 2, 2, 2, 2, 2, 2, 2, 2, 4 ),
 ( 0.0005154968519531658369, 0.0009585995601737966462, 0.001180150914284111997, 0.001290926591339269618, 0.001401702268394427239, 0.001512477945449584643, 0.001623253622504742264, 0.001844804976615087430, 0.002287907684835912420, 0.003174113101277619645, 0.004060318517719327738, 0.004946523934161035398, 0.005389626642381843691, 0.005611177996492257812, 0.005721953673547463572, 0.005777341512075067319, 0.005832729350602670199, 0.005888117189130273946, 0.005943505027657876826, 0.006054280704713086055, 0.006275832058823504513, 0.006718934767044361378, 0.007162037475265219111, 0.007605140183486076844 ),
 .UNSPECIFIED. ) ;
#7766=CARTESIAN_POINT ( 'NONE',  ( 163.7085541710205234, 247.0954618725873217, -6.713544974106887331 ) ) ;
#7768=CARTESIAN_POINT ( 'NONE',  ( 150.4851912698882757, 251.5643266524160424, -9.188101187500093303 ) ) ;
#7771=CARTESIAN_POINT ( 'NONE',  ( 188.8015641287956612, 261.8435057067845833, 6.507177985326441316 ) ) ;
#7772=EDGE_CURVE ( 'NONE', #46269, #82418, #65276, .T. ) ;
#7773=CARTESIAN_POINT ( 'NONE',  ( 206.3907062969896060, 273.1678058140250300, 11.56942460516550675 ) ) ;
#7780=CARTESIAN_POINT ( 'NONE',  ( 181.4396949203754161, 287.4694724887078223, 13.37274027909958640 ) ) ;
#7787=CARTESIAN_POINT ( 'NONE',  ( 205.0994677818405023, 275.4042965269534307, -14.14519517703424789 ) ) ;
#7789=CARTESIAN_POINT ( 'NONE',  ( 200.8812236821030126, 282.2243460117538234, -16.60069316942784567 ) ) ;
#7790=CARTESIAN_POINT ( 'NONE',  ( 189.2654362934434289, 294.2704508525881693, 12.90651062627435053 ) ) ;
#7792=CARTESIAN_POINT ( 'NONE',  ( 163.1369207721744772, 248.0855599626920593, -11.24692769914530110 ) ) ;
#7796=ORIENTED_EDGE ( 'NONE', *, *, #91300, .F. ) ;
#7797=CARTESIAN_POINT ( 'NONE',  ( 190.5361265807717359, 281.4599470083306869, 16.99703021481662191 ) ) ;
#7800=CARTESIAN_POINT ( 'NONE',  ( 190.7705347155322499, 300.2227366160529414, 3.504769718465625239 ) ) ;
#7801=CARTESIAN_POINT ( 'NONE',  ( 157.4068442735347446, 281.9945091197541274, 2.874377194828706905 ) ) ;
#7807=CARTESIAN_POINT ( 'NONE',  ( 149.6890529486499872, 271.3779502865075983, -12.51465682618088593 ) ) ;
#7809=ORIENTED_EDGE ( 'NONE', *, *, #98151, .F. ) ;
#7810=CARTESIAN_POINT ( 'NONE',  ( 93.65192705076950119, 231.0024278399160949, -9.188101187500093303 ) ) ;
#7811=CARTESIAN_POINT ( 'NONE',  ( 155.3841941879665853, 261.5136763037301648, 18.59686659711820411 ) ) ;
#7812=CARTESIAN_POINT ( 'NONE',  ( 191.4685399627163633, 299.0137560639802814, 7.545791216288330716 ) ) ;
#7813=CARTESIAN_POINT ( 'NONE',  ( 166.7187202459675746, 278.5591580196478958, -14.78021074750266273 ) ) ;
#7814=B_SPLINE_SURFACE_WITH_KNOTS ( 'NONE', 3, 1, ( 
 ( #63290, #99940 ),
 ( #52813, #71910 ),
 ( #14818, #94233 ),
 ( #9617, #76157 ),
 ( #37609, #99443 ),
 ( #30020, #24784 ),
 ( #39969, #2000 ),
 ( #79544, #2511 ),
 ( #76629, #17702 ),
 ( #55666, #62782 ),
 ( #40479, #48605 ),
 ( #64296, #38099 ),
 ( #45218, #40964 ),
 ( #70904, #7215 ),
 ( #69010, #71410 ),
 ( #94727, #32886 ),
 ( #30524, #83770 ),
 ( #79026, #86653 ),
 ( #32394, #6732 ),
 ( #93739, #25287 ),
 ( #56173, #14330 ),
 ( #17184, #68522 ),
 ( #87169, #48086 ),
 ( #24299, #55175 ),
 ( #86159, #78512 ),
 ( #16693, #47584 ),
 ( #1512, #12609 ),
 ( #50579, #10603 ),
 ( #73406, #89640 ),
 ( #43474, #34393 ),
 ( #41475, #72424 ),
 ( #74418, #5003 ),
 ( #3992, #56688 ),
 ( #82034, #11119 ) ),
 .UNSPECIFIED., .T., .F., .F.,
 ( 4, 2, 2, 2, 2, 2, 2, 2, 2, 2, 2, 2, 2, 2, 2, 2, 4 ),
 ( 2, 2 ),
 ( 0.000000000000000000, 0.06250000000000000000, 0.1250000000000000000, 0.1875000000000000000, 0.2500000000000000000, 0.3125000000000000000, 0.3750000000000000000, 0.4375000000000000000, 0.5000000000000000000, 0.5625000000000000000, 0.6250000000000000000, 0.6875000000000000000, 0.7500000000000000000, 0.8125000000000000000, 0.8750000000000000000, 0.9375000000000000000, 1.000000000000000000 ),
 ( 0.000000000000000000, 1.000000000000000000 ),
 .UNSPECIFIED. ) ;
#7815=EDGE_LOOP ( 'NONE', ( #2630, #20932, #91451, #80762 ) ) ;
#7819=ORIENTED_EDGE ( 'NONE', *, *, #79029, .F. ) ;
#7820=CARTESIAN_POINT ( 'NONE',  ( 152.6547697591180111, 278.7515079535921814, -4.825746761778547445 ) ) ;
#7822=ORIENTED_EDGE ( 'NONE', *, *, #17356, .T. ) ;
#7823=CARTESIAN_POINT ( 'NONE',  ( 208.3117541397001844, 269.8404533466799080, 2.895672523916592578 ) ) ;
#7826=CARTESIAN_POINT ( 'NONE',  ( 165.1189985546704975, 271.0502085123236498, 16.97077559774535871 ) ) ;
#7831=VERTEX_POINT ( 'NONE', #65343 ) ;
#7836=CARTESIAN_POINT ( 'NONE',  ( -22.42236680055709641, 157.8615022471902591, 0.000000000000000000 ) ) ;
#7839=CARTESIAN_POINT ( 'NONE',  ( 170.9828833598360234, 259.0842644313817686, -13.89840066965689758 ) ) ;
#7840=CARTESIAN_POINT ( 'NONE',  ( 206.6268150440956504, 272.7588534679261443, -10.76664753678610609 ) ) ;
#7843=CARTESIAN_POINT ( 'NONE',  ( 171.1494736412307418, 255.4807717095144994, 11.23012609300629450 ) ) ;
#7844=CARTESIAN_POINT ( 'NONE',  ( 194.0472512474883047, 263.4056162429215533, -0.7688519765262188388 ) ) ;
#7846=CARTESIAN_POINT ( 'NONE',  ( 193.8618999797658091, 294.8683349136467200, -15.25219021621163051 ) ) ;
#7849=CARTESIAN_POINT ( 'NONE',  ( 163.1218343930725894, 256.2508100442478849, -16.13596270478102923 ) ) ;
#7850=CARTESIAN_POINT ( 'NONE',  ( -0.9341114727036623488, 180.2677522451419350, -5.000000000000047962 ) ) ;
#7851=CARTESIAN_POINT ( 'NONE',  ( 87.42789010471635436, 209.0327760586659451, 1.948934522072302763E-15 ) ) ;
#7852=EDGE_CURVE ( 'NONE', #36064, #16265, #2071, .T. ) ;
#7853=CARTESIAN_POINT ( 'NONE',  ( 192.8523012050875707, 267.1932176075470124, -11.09616388545629384 ) ) ;
#7856=CARTESIAN_POINT ( 'NONE',  ( 203.5365106480763018, 278.1114176926849382, -15.57541962905212252 ) ) ;
#7858=CARTESIAN_POINT ( 'NONE',  ( 176.0164579604465018, 289.8288593268874251, 9.535015465809415502 ) ) ;
#7859=CARTESIAN_POINT ( 'NONE',  ( 7.266240119036749157, 168.8768266524159856, -9.188101187500091527 ) ) ;
#7860=CARTESIAN_POINT ( 'NONE',  ( 200.9110265982630779, 282.6588894614233141, 17.52479721249226685 ) ) ;
#7862=VECTOR ( 'NONE', #7291, 1000.000000000000000 ) ;
#7864=CARTESIAN_POINT ( 'NONE',  ( 155.5995420464182644, 262.6346450740109617, -17.48312782858739567 ) ) ;
#7865=CARTESIAN_POINT ( 'NONE',  ( 198.1306167967736940, 265.0230878689690144, -3.023881929457708395 ) ) ;
#7866=ADVANCED_FACE ( 'NONE', ( #52126 ), #83076, .T. ) ;
#7868=CARTESIAN_POINT ( 'NONE',  ( 205.4029933437358295, 274.8785748323546159, -13.50815392427034922 ) ) ;
#7872=( BOUNDED_CURVE ( )  B_SPLINE_CURVE ( 2, ( #18600, #94125, #55070, #40861, #8490, #72310, #70789, #79434, #39360, #9999, #33809, #8983, #39854, #71808, #88052, #87052, #79929, #1399, #2404, #17587, #63182, #57071, #24679, #77904, #95645, #56579, #86546, #87566, #33283, #94622, #25179, #17077, #48493, #86055, #70274, #885, #78913, #64185, #95134, #56059, #47478, #47967, #18095, #48993, #31764, #9499, #16582, #10489, #62668, #2917, #40365, #41370, #93620, #26192, #24187, #71304, #78402, #81923, #59554, #58567, #51475, #4380, #43865, #74807, #50473, #28671, #34772, #49479, #67170, #28177, #80943, #59048, #43368, #73791, #35280, #73299, #89539, #26685, #41882, #11009, #81426, #97132, #12499, #74315, #4897, #90531, #57573, #5385, #80435, #36271, #97609, #49988, #72820, #66186, #98093, #35781, #20592, #42365, #66675, #3412, #11998, #34286, #58083, #42855, #65183, #90020, #27699, #20100, #19112, #96131, #96628, #88546, #11511, #3890, #82442, #50971, #65673, #13005, #27194, #89063, #19615, #13494, #23044, #92499, #13980, #84405, #22070, #5878, #31145, #99581, #61049, #6381, #77263, #45359, #53941, #68658, #67674, #30165, #60548, #7357, #44855, #21580, #75795, #36764, #45839, #69156, #76762, #14950, #38752, #84900, #15441, #37264, #37752, #46340, #68163, #99089, #29672, #91505, #76291, #52965, #83916, #62036, #7875, #51980, #98603, #14478, #21102, #6863, #264, #92022, #100086, #82919, #69655, #22568, #44365, #29186, #53454, #75297, #61553, #52465, #38241, #60054, #91017, #30673, #83410, #757, #24556, #1270, #86425, #93500, #47354, #8370, #17461, #40744, #48371, #55933, #10377, #95011, #25571, #78276, #9365, #32155, #63062, #33677, #94005, #40244, #86931, #8860, #71689, #92989, #56460, #23543, #70144, #55436, #85933, #78780, #79319, #54434, #39727, #31641, #9887, #2285, #15958, #85409, #62541, #79813, #47840, #48878, #24060, #33163, #54954, #64067, #16951, #94500, #71185, #87451, #17984, #1781, #72186, #70658, #46861, #41247, #2796, #77783, #32660, #39235, #16458, #63560, #25057, #87937, #57451, #65558, #3776, #73184, #57956, #81310, #42738, #11881, #35658, #41754, #81800, #10877, #64574, #96506, #3292, #49366, #34658, #88430, #95530, #56951, #80826, #72700, #18480, #11395, #43242, #42248, #27075, #34172, #58448, #88942, #19501, #80310, #65064, #49861, #50355, #73674, #4255, #35155, #18990, #66062, #96014, #26575, #97012, #27581, #26075, #19973, #89419, #97486, #12376, #50850, #74184, #4775, #66558, #79636, #25910, #47673, #48188, #78100, #93837, #71009, #79134, #9714, #32498, #63388, #9192, #87272, #24391, #40067, #94329, #1097, #47178, #64898, #87765, #40571, #41578, #31974, #78606, #8690, #95355, #86246, #24882, #62879, #56782, #39559, #56275, #10700, #55265, #86750, #55758, #71511, #16783, #70483, #17284, #1611, #2102, #32983, #63887, #72519, #94823, #3128, #25387, #17803, #48702, #10203, #95844, #41066, #72004, #2608, #33496, #64391, #54777, #18304, #49203, #80136, #85755, #34013, #16285, #80638, #3606, #19322, #89733, #73499, #74511, #49683, #18800, #96327, #13201, #81623, #82643, #34484, #12706, #36470, #35480, #28374, #50185, #20294, #66384, #57775, #26399, #58763, #74001, #51693, #44059, #74999, #82134, #97314, #11215, #65384, #65877, #5578, #42082, #73014, #88253, #27396, #27881, #51171, #50671, #26897, #88750, #96832, #57276, #81139, #11705, #42565, #12196, #67374, #4082, #20800, #34974, #58278, #5090, #89254, #19804, #43055, #4587, #43577, #35970, #66872, #97805, #59252, #90231, #29128, #43303, #35717, #50413, #82863, #97546, #66616, #4313, #27136, #81859, #28112, #58987, #12436, #74251, #89477, #67107, #35217, #20036, #4836, #81371, #58021, #36699, #5813, #27639, #98032, #89956, #19553, #44794, #12945, #74746, #20534, #11939, #75231, #89002, #36203, #90964, #42795, #51412, #82375, #43805, #66119, #50909, #73729, #59492, #13436, #90471, #28609, #52405, #67608, #98538, #5326, #59995, #21041, #51923, #58504, #44302, #21522, #83350, #13916, #75730, #34714, #65614, #97067, #96569, #48693, #52903, #6315, #60487, #83854, #99526, #70998, #37206, #2093, #30109, #7810, #68107, #40058, #63879, #37692, #68602, #1602, #17794, #15382, #9703, #60992, #32485, #46279, #91959, #99029, #63380, #29615, #25377, #86740, #22507, #17275, #94319, #30611, #61496, #53401, #77205, #14420, #91446, #22007, #7301, #24874, #55748, #92447, #76236, #6811, #22993, #45302, #48178, #94814, #84350, #38182, #14897, #100025, #45786, #76707, #69098, #79123, #40563, #71500, #32971, #56267, #87260, #53884, #84844, #96318, #43045, #88242, #20285, #49672, #26885, #73490, #34004, #58268, #79628, #81614, #10192, #56774, #80629, #72510, #65375, #42556, #41057, #95836, #87755, #4074, #71994, #2599, #33484, #49190, #66373, #34477, #35469, #18296, #65863, #41567, #19795, #42075, #81131, #57764, #73989, #4574, #11204, #58753, #64889, #64383, #97305, #27872, #34963, #19312, #95344, #80127, #18792, #89724, #25901, #26388, #88740, #73007, #3596, #50177, #11697, #96823, #27381, #10688, #57267, #89244, #50662, #12186, #75482, #20788, #35962, #83104, #5567, #82123, #12696, #28877, #59239, #43564, #98288, #45546, #59752, #52155, #66863, #99280, #13675, #44548, #51679, #90217, #67360, #6065, #36959, #90723, #21278, #36459, #83604, #82628, #67871, #98792, #97793, #74502, #53162, #22258, #44046, #14171, #29374, #28363, #61247, #91696, #13190, #60240, #91201, #21761, #45056, #75996, #6574, #30363, #74987, #76477, #92215, #7056, #29863, #52650, #51160, #37445, #37937, #68355, #84116, #60734, #14668, #5080, #68850, #99771, #31354, #23744, #38444, #70869, #85617, #54638, #92696, #15138, #69852, #69359, #100277, #17154, #1477, #16160, #46036, #23247, #8073, #464, #30864, #76952, #24754, #94200, #15643, #86127, #47059, #7553, #32853, #965, #62744, #38947, #78994, #77972, #55635, #70353, #61747, #54134, #8568, #62237, #39434, #85097, #77477, #46540, #47551, #32358, #78478, #16656, #40444, #86620, #48052 ),
 .UNSPECIFIED., .F., .T. ) 
 B_SPLINE_CURVE_WITH_KNOTS ( ( 3, 2, 2, 2, 2, 2, 2, 2, 2, 2, 2, 2, 2, 2, 2, 2, 2, 2, 2, 2, 2, 2, 2, 2, 2, 2, 2, 2, 2, 2, 2, 2, 2, 2, 2, 2, 2, 2, 2, 2, 2, 2, 2, 2, 2, 2, 2, 2, 2, 2, 2, 2, 2, 2, 2, 2, 2, 2, 2, 2, 2, 2, 2, 2, 2, 2, 2, 2, 2, 2, 2, 2, 2, 2, 2, 2, 2, 2, 2, 2, 2, 2, 2, 2, 2, 2, 2, 2, 2, 2, 2, 2, 2, 2, 2, 2, 2, 2, 2, 2, 2, 2, 2, 2, 2, 2, 2, 2, 2, 2, 2, 2, 2, 2, 2, 2, 2, 2, 2, 2, 2, 2, 2, 2, 2, 2, 2, 2, 2, 2, 2, 2, 2, 2, 2, 2, 2, 2, 2, 2, 2, 2, 2, 2, 2, 2, 2, 2, 2, 2, 2, 2, 2, 2, 2, 2, 2, 2, 2, 2, 2, 2, 2, 2, 2, 2, 2, 2, 2, 2, 2, 2, 2, 2, 2, 2, 2, 2, 2, 2, 2, 2, 2, 2, 2, 2, 2, 2, 2, 2, 2, 2, 2, 2, 2, 2, 2, 2, 2, 2, 2, 2, 2, 2, 2, 2, 2, 2, 2, 2, 2, 2, 2, 2, 2, 2, 2, 2, 2, 2, 2, 2, 2, 2, 2, 2, 2, 2, 2, 2, 2, 2, 2, 2, 2, 2, 2, 2, 2, 2, 2, 2, 2, 2, 2, 2, 2, 2, 2, 2, 2, 2, 2, 2, 2, 2, 2, 2, 2, 2, 2, 2, 2, 2, 2, 2, 2, 2, 2, 2, 2, 2, 2, 2, 2, 2, 2, 2, 2, 2, 2, 2, 2, 2, 2, 2, 2, 2, 2, 2, 2, 2, 2, 2, 2, 2, 2, 2, 2, 2, 2, 2, 2, 2, 2, 2, 2, 2, 2, 2, 2, 2, 2, 2, 2, 2, 2, 2, 2, 2, 2, 2, 2, 2, 2, 2, 2, 2, 2, 2, 2, 2, 2, 2, 2, 2, 2, 2, 2, 2, 2, 2, 2, 2, 2, 2, 2, 2, 2, 2, 2, 2, 2, 2, 2, 2, 2, 2, 2, 2, 2, 2, 2, 2, 2, 2, 2, 3 ),
 ( 0.000000000000000000, 0.002688172043010752903, 0.005376344086021505805, 0.008064516129032257841, 0.01075268817204301161, 0.01344086021505376365, 0.01612903225806451568, 0.01881720430107526945, 0.02150537634408602322, 0.02419354838709677352, 0.02688172043010752729, 0.02956989247311828106, 0.03225806451612903136, 0.03494623655913978166, 0.03763440860215053890, 0.04032258064516128920, 0.04301075268817204644, 0.04569892473118279674, 0.04838709677419354704, 0.05107526881720430428, 0.05376344086021505458, 0.05645161290322580488, 0.05913978494623656212, 0.06182795698924731242, 0.06451612903225806273, 0.06720430107526881303, 0.06989247311827956333, 0.07258064516129032751, 0.07526881720430107781, 0.07795698924731182811, 0.08064516129032257841, 0.08333333333333332871, 0.08602150537634409289, 0.08870967741935484319, 0.09139784946236559349, 0.09408602150537634379, 0.09677419354838709409, 0.09946236559139784439, 0.1021505376344086086, 0.1048387096774193589, 0.1075268817204301092, 0.1102150537634408595, 0.1129032258064516098, 0.1155913978494623601, 0.1182795698924731242, 0.1209677419354838745, 0.1236559139784946248, 0.1263440860215053752, 0.1290322580645161255, 0.1317204301075268758, 0.1344086021505376261, 0.1370967741935483764, 0.1397849462365591267, 0.1424731182795699047, 0.1451612903225806550, 0.1478494623655914053, 0.1505376344086021556, 0.1532258064516129059, 0.1559139784946236562, 0.1586021505376344065, 0.1612903225806451568, 0.1639784946236559071, 0.1666666666666666574, 0.1693548387096774077, 0.1720430107526881858, 0.1747311827956989361, 0.1774193548387096864, 0.1801075268817204367, 0.1827956989247311870, 0.1854838709677419373, 0.1881720430107526876, 0.1908602150537634379, 0.1935483870967741882, 0.1962365591397849385, 0.1989247311827956888, 0.2016129032258064391, 0.2043010752688172171, 0.2069892473118279674, 0.2096774193548387177, 0.2123655913978494680, 0.2150537634408602183, 0.2177419354838709686, 0.2204301075268817189, 0.2231182795698924692, 0.2258064516129032195, 0.2284946236559139698, 0.2311827956989247201, 0.2338709677419354704, 0.2365591397849462485, 0.2392473118279569988, 0.2419354838709677491, 0.2446236559139784994, 0.2473118279569892497, 0.2500000000000000000, 0.2526881720430107503, 0.2553763440860215006, 0.2580645161290322509, 0.2607526881720430012, 0.2634408602150537515, 0.2661290322580645018, 0.2688172043010752521, 0.2715053763440860024, 0.2741935483870967527, 0.2768817204301075030, 0.2795698924731182533, 0.2822580645161290591, 0.2849462365591398094, 0.2876344086021505597, 0.2903225806451613100, 0.2930107526881720603, 0.2956989247311828106, 0.2983870967741935609, 0.3010752688172043112, 0.3037634408602150615, 0.3064516129032258118, 0.3091397849462365621, 0.3118279569892473124, 0.3145161290322580627, 0.3172043010752688130, 0.3198924731182795633, 0.3225806451612903136, 0.3252688172043010639, 0.3279569892473118142, 0.3306451612903225645, 0.3333333333333333148, 0.3360215053763440651, 0.3387096774193548154, 0.3413978494623655657, 0.3440860215053763715, 0.3467741935483871218, 0.3494623655913978721, 0.3521505376344086224, 0.3548387096774193727, 0.3575268817204301230, 0.3602150537634408733, 0.3629032258064516236, 0.3655913978494623739, 0.3682795698924731242, 0.3709677419354838745, 0.3736559139784946248, 0.3763440860215053752, 0.3790322580645161255, 0.3817204301075268758, 0.3844086021505376261, 0.3870967741935483764, 0.3897849462365591267, 0.3924731182795698770, 0.3951612903225806273, 0.3978494623655913776, 0.4005376344086021279, 0.4032258064516128782, 0.4059139784946236285, 0.4086021505376344343, 0.4112903225806451846, 0.4139784946236559349, 0.4166666666666666852, 0.4193548387096774355, 0.4220430107526881858, 0.4247311827956989361, 0.4274193548387096864, 0.4301075268817204367, 0.4327956989247311870, 0.4354838709677419373, 0.4381720430107526876, 0.4408602150537634379, 0.4435483870967741882, 0.4462365591397849385, 0.4489247311827956888, 0.4516129032258064391, 0.4543010752688171894, 0.4569892473118279397, 0.4596774193548386900, 0.4623655913978494403, 0.4650537634408601906, 0.4677419354838709409, 0.4704301075268817467, 0.4731182795698924970, 0.4758064516129032473, 0.4784946236559139976, 0.4811827956989247479, 0.4838709677419354982, 0.4865591397849462485, 0.4892473118279569988, 0.4919354838709677491, 0.4946236559139784994, 0.4973118279569892497, 0.5000000000000000000, 0.5026881720430107503, 0.5053763440860215006, 0.5080645161290322509, 0.5107526881720430012, 0.5134408602150537515, 0.5161290322580645018, 0.5188172043010752521, 0.5215053763440860024, 0.5241935483870967527, 0.5268817204301075030, 0.5295698924731182533, 0.5322580645161290036, 0.5349462365591397539, 0.5376344086021505042, 0.5403225806451612545, 0.5430107526881720048, 0.5456989247311827551, 0.5483870967741935054, 0.5510752688172042557, 0.5537634408602150060, 0.5564516129032257563, 0.5591397849462365066, 0.5618279569892472569, 0.5645161290322581182, 0.5672043010752688685, 0.5698924731182796188, 0.5725806451612903691, 0.5752688172043011194, 0.5779569892473118697, 0.5806451612903226200, 0.5833333333333333703, 0.5860215053763441206, 0.5887096774193548709, 0.5913978494623656212, 0.5940860215053763715, 0.5967741935483871218, 0.5994623655913978721, 0.6021505376344086224, 0.6048387096774193727, 0.6075268817204301230, 0.6102150537634408733, 0.6129032258064516236, 0.6155913978494623739, 0.6182795698924731242, 0.6209677419354838745, 0.6236559139784946248, 0.6263440860215053752, 0.6290322580645161255, 0.6317204301075268758, 0.6344086021505376261, 0.6370967741935483764, 0.6397849462365591267, 0.6424731182795698770, 0.6451612903225806273, 0.6478494623655913776, 0.6505376344086021279, 0.6532258064516128782, 0.6559139784946236285, 0.6586021505376343788, 0.6612903225806451291, 0.6639784946236558794, 0.6666666666666666297, 0.6693548387096773800, 0.6720430107526881303, 0.6747311827956988806, 0.6774193548387096309, 0.6801075268817203812, 0.6827956989247311315, 0.6854838709677418818, 0.6881720430107527431, 0.6908602150537634934, 0.6935483870967742437, 0.6962365591397849940, 0.6989247311827957443, 0.7016129032258064946, 0.7043010752688172449, 0.7069892473118279952, 0.7096774193548387455, 0.7123655913978494958, 0.7150537634408602461, 0.7177419354838709964, 0.7204301075268817467, 0.7231182795698924970, 0.7258064516129032473, 0.7284946236559139976, 0.7311827956989247479, 0.7338709677419354982, 0.7365591397849462485, 0.7392473118279569988, 0.7419354838709677491, 0.7446236559139784994, 0.7473118279569892497, 0.7500000000000000000, 0.7526881720430107503, 0.7553763440860215006, 0.7580645161290322509, 0.7607526881720430012, 0.7634408602150537515, 0.7661290322580645018, 0.7688172043010752521, 0.7715053763440860024, 0.7741935483870967527, 0.7768817204301075030, 0.7795698924731182533, 0.7822580645161290036, 0.7849462365591397539, 0.7876344086021505042, 0.7903225806451612545, 0.7930107526881720048, 0.7956989247311827551, 0.7983870967741935054, 0.8010752688172042557, 0.8037634408602150060, 0.8064516129032257563, 0.8091397849462365066, 0.8118279569892472569, 0.8145161290322581182, 0.8172043010752688685, 0.8198924731182796188, 0.8225806451612903691, 0.8252688172043011194, 0.8279569892473118697, 0.8306451612903226200, 0.8333333333333333703, 0.8360215053763441206, 0.8387096774193548709, 0.8413978494623656212, 0.8440860215053763715, 0.8467741935483871218, 0.8494623655913978721, 0.8521505376344086224, 0.8548387096774193727, 0.8575268817204301230, 0.8602150537634408733, 0.8629032258064516236, 0.8655913978494623739, 0.8682795698924731242, 0.8709677419354838745, 0.8736559139784946248, 0.8763440860215053752, 0.8790322580645161255, 0.8817204301075268758, 0.8844086021505376261, 0.8870967741935483764, 0.8897849462365591267, 0.8924731182795698770, 0.8951612903225806273, 0.8978494623655913776, 0.9005376344086021279, 0.9032258064516128782, 0.9059139784946236285, 0.9086021505376343788, 0.9112903225806451291, 0.9139784946236558794, 0.9166666666666666297, 0.9193548387096773800, 0.9220430107526881303, 0.9247311827956988806, 0.9274193548387096309, 0.9301075268817203812, 0.9327956989247311315, 0.9354838709677418818, 0.9381720430107527431, 0.9408602150537634934, 0.9435483870967742437, 0.9462365591397849940, 0.9489247311827957443, 0.9516129032258064946, 0.9543010752688172449, 0.9569892473118279952, 0.9596774193548387455, 0.9623655913978494958, 0.9650537634408602461, 0.9677419354838709964, 0.9704301075268817467, 0.9731182795698924970, 0.9758064516129032473, 0.9784946236559139976, 0.9811827956989247479, 0.9838709677419354982, 0.9855363728105643872 ),
 .UNSPECIFIED. ) 
 CURVE ( )  GEOMETRIC_REPRESENTATION_ITEM ( )  RATIONAL_B_SPLINE_CURVE ( ( 1.000000000000000000, 0.8660254037844387076, 1.000000000000000000, 0.8660254037844387076, 1.000000000000000000, 0.8660254037844387076, 1.000000000000000000, 0.8660254037844387076, 1.000000000000000000, 0.8660254037844387076, 1.000000000000000000, 0.8660254037844387076, 1.000000000000000000, 0.8660254037844387076, 1.000000000000000000, 0.8660254037844387076, 1.000000000000000000, 0.8660254037844387076, 1.000000000000000000, 0.8660254037844387076, 1.000000000000000000, 0.8660254037844387076, 1.000000000000000000, 0.8660254037844387076, 1.000000000000000000, 0.8660254037844387076, 1.000000000000000000, 0.8660254037844387076, 1.000000000000000000, 0.8660254037844387076, 1.000000000000000000, 0.8660254037844387076, 1.000000000000000000, 0.8660254037844387076, 1.000000000000000000, 0.8660254037844387076, 1.000000000000000000, 0.8660254037844387076, 1.000000000000000000, 0.8660254037844387076, 1.000000000000000000, 0.8660254037844387076, 1.000000000000000000, 0.8660254037844387076, 1.000000000000000000, 0.8660254037844387076, 1.000000000000000000, 0.8660254037844387076, 1.000000000000000000, 0.8660254037844387076, 1.000000000000000000, 0.8660254037844387076, 1.000000000000000000, 0.8660254037844387076, 1.000000000000000000, 0.8660254037844387076, 1.000000000000000000, 0.8660254037844387076, 1.000000000000000000, 0.8660254037844387076, 1.000000000000000000, 0.8660254037844387076, 1.000000000000000000, 0.8660254037844387076, 1.000000000000000000, 0.8660254037844387076, 1.000000000000000000, 0.8660254037844387076, 1.000000000000000000, 0.8660254037844387076, 1.000000000000000000, 0.8660254037844387076, 1.000000000000000000, 0.8660254037844387076, 1.000000000000000000, 0.8660254037844387076, 1.000000000000000000, 0.8660254037844387076, 1.000000000000000000, 0.8660254037844387076, 1.000000000000000000, 0.8660254037844387076, 1.000000000000000000, 0.8660254037844387076, 1.000000000000000000, 0.8660254037844387076, 1.000000000000000000, 0.8660254037844387076, 1.000000000000000000, 0.8660254037844387076, 1.000000000000000000, 0.8660254037844387076, 1.000000000000000000, 0.8660254037844387076, 1.000000000000000000, 0.8660254037844387076, 1.000000000000000000, 0.8660254037844387076, 1.000000000000000000, 0.8660254037844387076, 1.000000000000000000, 0.8660254037844387076, 1.000000000000000000, 0.8660254037844387076, 1.000000000000000000, 0.8660254037844387076, 1.000000000000000000, 0.8660254037844387076, 1.000000000000000000, 0.8660254037844387076, 1.000000000000000000, 0.8660254037844387076, 1.000000000000000000, 0.8660254037844387076, 1.000000000000000000, 0.8660254037844387076, 1.000000000000000000, 0.8660254037844387076, 1.000000000000000000, 0.8660254037844387076, 1.000000000000000000, 0.8660254037844387076, 1.000000000000000000, 0.8660254037844387076, 1.000000000000000000, 0.8660254037844387076, 1.000000000000000000, 0.8660254037844387076, 1.000000000000000000, 0.8660254037844387076, 1.000000000000000000, 0.8660254037844387076, 1.000000000000000000, 0.8660254037844387076, 1.000000000000000000, 0.8660254037844387076, 1.000000000000000000, 0.8660254037844387076, 1.000000000000000000, 0.8660254037844387076, 1.000000000000000000, 0.8660254037844387076, 1.000000000000000000, 0.8660254037844387076, 1.000000000000000000, 0.8660254037844387076, 1.000000000000000000, 0.8660254037844387076, 1.000000000000000000, 0.8660254037844387076, 1.000000000000000000, 0.8660254037844387076, 1.000000000000000000, 0.8660254037844387076, 1.000000000000000000, 0.8660254037844387076, 1.000000000000000000, 0.8660254037844387076, 1.000000000000000000, 0.8660254037844387076, 1.000000000000000000, 0.8660254037844387076, 1.000000000000000000, 0.8660254037844387076, 1.000000000000000000, 0.8660254037844387076, 1.000000000000000000, 0.8660254037844387076, 1.000000000000000000, 0.8660254037844387076, 1.000000000000000000, 0.8660254037844387076, 1.000000000000000000, 0.8660254037844387076, 1.000000000000000000, 0.8660254037844387076, 1.000000000000000000, 0.8660254037844387076, 1.000000000000000000, 0.8660254037844387076, 1.000000000000000000, 0.8660254037844387076, 1.000000000000000000, 0.8660254037844387076, 1.000000000000000000, 0.8660254037844387076, 1.000000000000000000, 0.8660254037844387076, 1.000000000000000000, 0.8660254037844387076, 1.000000000000000000, 0.8660254037844387076, 1.000000000000000000, 0.8660254037844387076, 1.000000000000000000, 0.8660254037844387076, 1.000000000000000000, 0.8660254037844387076, 1.000000000000000000, 0.8660254037844387076, 1.000000000000000000, 0.8660254037844387076, 1.000000000000000000, 0.8660254037844387076, 1.000000000000000000, 0.8660254037844387076, 1.000000000000000000, 0.8660254037844387076, 1.000000000000000000, 0.8660254037844387076, 1.000000000000000000, 0.8660254037844387076, 1.000000000000000000, 0.8660254037844387076, 1.000000000000000000, 0.8660254037844387076, 1.000000000000000000, 0.8660254037844387076, 1.000000000000000000, 0.8660254037844387076, 1.000000000000000000, 0.8660254037844387076, 1.000000000000000000, 0.8660254037844387076, 1.000000000000000000, 0.8660254037844387076, 1.000000000000000000, 0.8660254037844387076, 1.000000000000000000, 0.8660254037844387076, 1.000000000000000000, 0.8660254037844387076, 1.000000000000000000, 0.8660254037844387076, 1.000000000000000000, 0.8660254037844387076, 1.000000000000000000, 0.8660254037844387076, 1.000000000000000000, 0.8660254037844387076, 1.000000000000000000, 0.8660254037844387076, 1.000000000000000000, 0.8660254037844387076, 1.000000000000000000, 0.8660254037844387076, 1.000000000000000000, 0.8660254037844387076, 1.000000000000000000, 0.8660254037844387076, 1.000000000000000000, 0.8660254037844387076, 1.000000000000000000, 0.8660254037844387076, 1.000000000000000000, 0.8660254037844387076, 1.000000000000000000, 0.8660254037844387076, 1.000000000000000000, 0.8660254037844387076, 1.000000000000000000, 0.8660254037844387076, 1.000000000000000000, 0.8660254037844387076, 1.000000000000000000, 0.8660254037844387076, 1.000000000000000000, 0.8660254037844387076, 1.000000000000000000, 0.8660254037844387076, 1.000000000000000000, 0.8660254037844387076, 1.000000000000000000, 0.8660254037844387076, 1.000000000000000000, 0.8660254037844387076, 1.000000000000000000, 0.8660254037844387076, 1.000000000000000000, 0.8660254037844387076, 1.000000000000000000, 0.8660254037844387076, 1.000000000000000000, 0.8660254037844387076, 1.000000000000000000, 0.8660254037844387076, 1.000000000000000000, 0.8660254037844387076, 1.000000000000000000, 0.8660254037844387076, 1.000000000000000000, 0.8660254037844387076, 1.000000000000000000, 0.8660254037844387076, 1.000000000000000000, 0.8660254037844387076, 1.000000000000000000, 0.8660254037844387076, 1.000000000000000000, 0.8660254037844387076, 1.000000000000000000, 0.8660254037844387076, 1.000000000000000000, 0.8660254037844387076, 1.000000000000000000, 0.8660254037844387076, 1.000000000000000000, 0.8660254037844387076, 1.000000000000000000, 0.8660254037844387076, 1.000000000000000000, 0.8660254037844387076, 1.000000000000000000, 0.8660254037844387076, 1.000000000000000000, 0.8660254037844387076, 1.000000000000000000, 0.8660254037844387076, 1.000000000000000000, 0.8660254037844387076, 1.000000000000000000, 0.8660254037844387076, 1.000000000000000000, 0.8660254037844387076, 1.000000000000000000, 0.8660254037844387076, 1.000000000000000000, 0.8660254037844387076, 1.000000000000000000, 0.8660254037844387076, 1.000000000000000000, 0.8660254037844387076, 1.000000000000000000, 0.8660254037844387076, 1.000000000000000000, 0.8660254037844387076, 1.000000000000000000, 0.8660254037844387076, 1.000000000000000000, 0.8660254037844387076, 1.000000000000000000, 0.8660254037844387076, 1.000000000000000000, 0.8660254037844387076, 1.000000000000000000, 0.8660254037844387076, 1.000000000000000000, 0.8660254037844387076, 1.000000000000000000, 0.8660254037844387076, 1.000000000000000000, 0.8660254037844387076, 1.000000000000000000, 0.8660254037844387076, 1.000000000000000000, 0.8660254037844387076, 1.000000000000000000, 0.8660254037844387076, 1.000000000000000000, 0.8660254037844387076, 1.000000000000000000, 0.8660254037844387076, 1.000000000000000000, 0.8660254037844387076, 1.000000000000000000, 0.8660254037844387076, 1.000000000000000000, 0.8660254037844387076, 1.000000000000000000, 0.8660254037844387076, 1.000000000000000000, 0.8660254037844387076, 1.000000000000000000, 0.8660254037844387076, 1.000000000000000000, 0.8660254037844387076, 1.000000000000000000, 0.8660254037844387076, 1.000000000000000000, 0.8660254037844387076, 1.000000000000000000, 0.8660254037844387076, 1.000000000000000000, 0.8660254037844387076, 1.000000000000000000, 0.8660254037844387076, 1.000000000000000000, 0.8660254037844387076, 1.000000000000000000, 0.8660254037844387076, 1.000000000000000000, 0.8660254037844387076, 1.000000000000000000, 0.8660254037844387076, 1.000000000000000000, 0.8660254037844387076, 1.000000000000000000, 0.8660254037844387076, 1.000000000000000000, 0.8660254037844387076, 1.000000000000000000, 0.8660254037844387076, 1.000000000000000000, 0.8660254037844387076, 1.000000000000000000, 0.8660254037844387076, 1.000000000000000000, 0.8660254037844387076, 1.000000000000000000, 0.8660254037844387076, 1.000000000000000000, 0.8660254037844387076, 1.000000000000000000, 0.8660254037844387076, 1.000000000000000000, 0.8660254037844387076, 1.000000000000000000, 0.8660254037844387076, 1.000000000000000000, 0.8660254037844387076, 1.000000000000000000, 0.8660254037844387076, 1.000000000000000000, 0.8660254037844387076, 1.000000000000000000, 0.8660254037844387076, 1.000000000000000000, 0.8660254037844387076, 1.000000000000000000, 0.8660254037844387076, 1.000000000000000000, 0.8660254037844387076, 1.000000000000000000, 0.8660254037844387076, 1.000000000000000000, 0.8660254037844387076, 1.000000000000000000, 0.8660254037844387076, 1.000000000000000000, 0.8660254037844387076, 1.000000000000000000, 0.8660254037844387076, 1.000000000000000000, 0.8660254037844387076, 1.000000000000000000, 0.8660254037844387076, 1.000000000000000000, 0.8660254037844387076, 1.000000000000000000, 0.8660254037844387076, 1.000000000000000000, 0.8660254037844387076, 1.000000000000000000, 0.8660254037844387076, 1.000000000000000000, 0.8660254037844387076, 1.000000000000000000, 0.8660254037844387076, 1.000000000000000000, 0.8660254037844387076, 1.000000000000000000, 0.8660254037844387076, 1.000000000000000000, 0.8660254037844387076, 1.000000000000000000, 0.8660254037844387076, 1.000000000000000000, 0.8660254037844387076, 1.000000000000000000, 0.8660254037844387076, 1.000000000000000000, 0.8660254037844387076, 1.000000000000000000, 0.8660254037844387076, 1.000000000000000000, 0.8660254037844387076, 1.000000000000000000, 0.8660254037844387076, 1.000000000000000000, 0.8660254037844387076, 1.000000000000000000, 0.8660254037844387076, 1.000000000000000000, 0.8660254037844387076, 1.000000000000000000, 0.8660254037844387076, 1.000000000000000000, 0.8660254037844387076, 1.000000000000000000, 0.8660254037844387076, 1.000000000000000000, 0.8660254037844387076, 1.000000000000000000, 0.8660254037844387076, 1.000000000000000000, 0.8660254037844387076, 1.000000000000000000, 0.8660254037844387076, 1.000000000000000000, 0.8660254037844387076, 1.000000000000000000, 0.8660254037844387076, 1.000000000000000000, 0.8660254037844387076, 1.000000000000000000, 0.8660254037844387076, 1.000000000000000000, 0.8660254037844387076, 1.000000000000000000, 0.8660254037844387076, 1.000000000000000000, 0.8660254037844387076, 1.000000000000000000, 0.8660254037844387076, 1.000000000000000000, 0.8660254037844387076, 1.000000000000000000, 0.8660254037844387076, 1.000000000000000000, 0.8660254037844387076, 1.000000000000000000, 0.8660254037844387076, 1.000000000000000000, 0.8660254037844387076, 1.000000000000000000, 0.8660254037844387076, 1.000000000000000000, 0.8660254037844387076, 1.000000000000000000, 0.8660254037844387076, 1.000000000000000000, 0.8660254037844387076, 1.000000000000000000, 0.8660254037844387076, 1.000000000000000000, 0.8660254037844387076, 1.000000000000000000, 0.8660254037844387076, 1.000000000000000000, 0.8660254037844387076, 1.000000000000000000, 0.8660254037844387076, 1.000000000000000000, 0.8660254037844387076, 1.000000000000000000, 0.8660254037844387076, 1.000000000000000000, 0.8660254037844387076, 1.000000000000000000, 0.8660254037844387076, 1.000000000000000000, 0.8660254037844387076, 1.000000000000000000, 0.8660254037844387076, 1.000000000000000000, 0.8660254037844387076, 1.000000000000000000, 0.8660254037844387076, 1.000000000000000000, 0.8660254037844387076, 1.000000000000000000, 0.8660254037844387076, 1.000000000000000000, 0.8660254037844387076, 1.000000000000000000, 0.8660254037844387076, 1.000000000000000000, 0.8660254037844387076, 1.000000000000000000, 0.8660254037844387076, 1.000000000000000000, 0.8660254037844387076, 1.000000000000000000, 0.8660254037844387076, 1.000000000000000000, 0.8660254037844387076, 1.000000000000000000, 0.8660254037844387076, 1.000000000000000000, 0.8660254037844387076, 1.000000000000000000, 0.8660254037844387076, 1.000000000000000000, 0.8660254037844387076, 1.000000000000000000, 0.8660254037844387076, 1.000000000000000000, 0.8660254037844387076, 1.000000000000000000, 0.8660254037844387076, 1.000000000000000000, 0.8660254037844387076, 1.000000000000000000, 0.8660254037844387076, 1.000000000000000000, 0.8660254037844387076, 1.000000000000000000, 0.8660254037844387076, 1.000000000000000000, 0.8660254037844387076, 1.000000000000000000, 0.8660254037844387076, 1.000000000000000000, 0.8660254037844387076, 1.000000000000000000, 0.8660254037844387076, 1.000000000000000000, 0.8660254037844387076, 1.000000000000000000, 0.8660254037844387076, 1.000000000000000000, 0.8660254037844387076, 1.000000000000000000, 0.8660254037844387076, 1.000000000000000000, 0.8660254037844387076, 1.000000000000000000, 0.8660254037844387076, 1.000000000000000000, 0.8660254037844387076, 1.000000000000000000, 0.8660254037844387076, 1.000000000000000000, 0.8660254037844387076, 1.000000000000000000, 0.8660254037844387076, 1.000000000000000000, 0.8660254037844387076, 1.000000000000000000, 0.8660254037844387076, 1.000000000000000000, 0.8660254037844387076, 1.000000000000000000, 0.8660254037844387076, 1.000000000000000000, 0.8660254037844387076, 1.000000000000000000, 0.8660254037844387076, 1.000000000000000000, 0.8660254037844387076, 1.000000000000000000, 0.8660254037844387076, 1.000000000000000000, 0.8660254037844387076, 1.000000000000000000, 0.8660254037844387076, 1.000000000000000000, 0.8660254037844387076, 1.000000000000000000, 0.8660254037844387076, 1.000000000000000000, 0.8660254037844387076, 1.000000000000000000, 0.8660254037844387076, 1.000000000000000000, 0.8660254037844387076, 1.000000000000000000, 0.8660254037844387076, 1.000000000000000000, 0.8660254037844387076, 1.000000000000000000, 0.8660254037844387076, 1.000000000000000000, 0.8660254037844387076, 1.000000000000000000, 0.8660254037844387076, 1.000000000000000000, 0.8660254037844387076, 1.000000000000000000, 0.8660254037844387076, 1.000000000000000000, 0.8660254037844387076, 1.000000000000000000, 0.8660254037844387076, 1.000000000000000000, 0.8660254037844387076, 1.000000000000000000, 0.8660254037844387076, 1.000000000000000000, 0.8660254037844387076, 1.000000000000000000, 0.8660254037844387076, 1.000000000000000000, 0.8660254037844387076, 1.000000000000000000, 0.8660254037844387076, 1.000000000000000000, 0.8660254037844387076, 1.000000000000000000, 0.8660254037844387076, 1.000000000000000000, 0.8660254037844387076, 1.000000000000000000, 0.8660254037844387076, 1.000000000000000000, 0.8660254037844387076, 1.000000000000000000, 0.8660254037844387076, 1.000000000000000000, 0.8660254037844387076, 1.000000000000000000, 0.8660254037844387076, 1.000000000000000000, 0.8660254037844387076, 1.000000000000000000, 0.8660254037844387076, 1.000000000000000000, 0.8660254037844387076, 1.000000000000000000, 0.8660254037844387076, 1.000000000000000000, 0.8660254037844387076, 1.000000000000000000, 0.8660254037844387076, 1.000000000000000000, 0.8660254037844387076, 1.000000000000000000, 0.8660254037844387076, 1.000000000000000000, 0.8660254037844387076, 1.000000000000000000, 0.8660254037844387076, 1.000000000000000000, 0.8660254037844387076, 1.000000000000000000, 0.8660254037844387076, 1.000000000000000000, 0.8660254037844387076, 1.000000000000000000, 0.8660254037844387076, 1.000000000000000000, 0.8660254037844387076, 1.000000000000000000, 0.9169986265629754829, 0.9368410486966849415 ) ) 
 REPRESENTATION_ITEM ( '' )  );
#7874=CARTESIAN_POINT ( 'NONE',  ( 153.6043694648998894, 279.0369973721463452, 3.800317288925857628 ) ) ;
#7875=CARTESIAN_POINT ( 'NONE',  ( 22.04262502322622908, 183.5333772461660544, 9.188101187500095079 ) ) ;
#7876=CARTESIAN_POINT ( 'NONE',  ( 113.4351080945290278, 245.4869531367911009, 4.594050593750046652 ) ) ;
#7877=CARTESIAN_POINT ( 'NONE',  ( 183.1556239524084333, 257.7435932540183217, -2.690512520808968411 ) ) ;
#7878=VERTEX_POINT ( 'NONE', #12662 ) ;
#7879=CARTESIAN_POINT ( 'NONE',  ( 34.87168918123982309, 179.3932355074535394, -2.679491924311248496 ) ) ;
#7880=CARTESIAN_POINT ( 'NONE',  ( 175.3097973626215662, 281.1046532212878901, -14.83871771951074692 ) ) ;
#7882=CARTESIAN_POINT ( 'NONE',  ( 139.8153705705071843, 239.9824982072973967, 3.021315404115420679E-15 ) ) ;
#7883=CARTESIAN_POINT ( 'NONE',  ( 200.6117230619925635, 269.0360104864248001, 9.242361455687714056 ) ) ;
#7884=CARTESIAN_POINT ( 'NONE',  ( 155.2419697281468416, 261.7600162942170527, 18.58580762350309357 ) ) ;
#7885=CARTESIAN_POINT ( 'NONE',  ( 207.1158949475991164, 271.9117422260973740, -5.823035679195911918 ) ) ;
#7887=CARTESIAN_POINT ( 'NONE',  ( 147.9500839974939197, 274.3899328626944225, -9.375093207164509224 ) ) ;
#7888=CARTESIAN_POINT ( 'NONE',  ( 190.4677317829447247, 263.8822203009034411, 7.824480301607388277 ) ) ;
#7889=CARTESIAN_POINT ( 'NONE',  ( 167.8570435341544567, 278.4618103485150868, 14.78497630034688726 ) ) ;
#7890=CARTESIAN_POINT ( 'NONE',  ( 176.5481980778163518, 256.7330344388156504, -11.15910957749502330 ) ) ;
#7892=CARTESIAN_POINT ( 'NONE',  ( 189.8763472015711216, 301.7715148217271803, -0.1184663095182975079 ) ) ;
#7893=CARTESIAN_POINT ( 'NONE',  ( 181.1200065746923826, 266.1666110466232453, -14.84348402710393877 ) ) ;
#7894=ORIENTED_EDGE ( 'NONE', *, *, #59618, .F. ) ;
#7897=CARTESIAN_POINT ( 'NONE',  ( 163.7423057141168385, 247.0370024851108610, -6.909410042141566066 ) ) ;
#7899=CARTESIAN_POINT ( 'NONE',  ( 91.43256340568937901, 235.8464784336661353, 1.353441290958777327E-15 ) ) ;
#7901=CARTESIAN_POINT ( 'NONE',  ( -6.813555604197667037, 155.3262482093457777, -6.972266317189433020E-16 ) ) ;
#7904=CARTESIAN_POINT ( 'NONE',  ( 195.0772487819253911, 279.0847438180149993, 16.30750567507551096 ) ) ;
#7905=CARTESIAN_POINT ( 'NONE',  ( 155.0898067732971697, 280.3139227198241201, -4.343794903066061863 ) ) ;
#7907=CARTESIAN_POINT ( 'NONE',  ( 146.0195742355162452, 245.1115022471902023, -5.000000000000041744 ) ) ;
#7909=CARTESIAN_POINT ( 'NONE',  ( 204.2143397907769611, 276.5280330293650195, 13.36303585211030054 ) ) ;
#7910=LINE ( 'NONE', #55967, #53942 ) ;
#7911=ORIENTED_EDGE ( 'NONE', *, *, #99719, .T. ) ;
#7912=CARTESIAN_POINT ( 'NONE',  ( 192.7785635360272352, 266.6923795695631156, 11.52468468594655526 ) ) ;
#7914=CARTESIAN_POINT ( 'NONE',  ( 196.1370092075112268, 290.1209220278959720, 16.40156295354631411 ) ) ;
#7915=CARTESIAN_POINT ( 'NONE',  ( 200.6117230619925635, 269.0360104864248001, 9.242361455687714056 ) ) ;
#7918=ORIENTED_EDGE ( 'NONE', *, *, #59421, .T. ) ;
#7921=CARTESIAN_POINT ( 'NONE',  ( 179.9071714477294961, 262.8436713092991113, -12.82472271075318737 ) ) ;
#7923=CARTESIAN_POINT ( 'NONE',  ( 152.7153488183568300, 266.1362520814392951, 17.33540622643059237 ) ) ;
#7929=CARTESIAN_POINT ( 'NONE',  ( 163.7166294601506991, 282.3380383384618995, 10.03031969300557513 ) ) ;
#7933=CARTESIAN_POINT ( 'NONE',  ( 206.1014820340073186, 273.6687569322920126, 12.23319432534553108 ) ) ;
#7935=CARTESIAN_POINT ( 'NONE',  ( 193.1476055184262464, 296.1055292122517244, -12.13892458995638535 ) ) ;
#7938=EDGE_CURVE ( 'NONE', #9864, #22636, #50502, .T. ) ;
#7943=CARTESIAN_POINT ( 'NONE',  ( 163.2237683175472398, 249.5215337783042173, 11.38175491140649598 ) ) ;
#7949=CARTESIAN_POINT ( 'NONE',  ( 165.4922176576098138, 275.0575853646175233, -16.02269507257410908 ) ) ;
#7950=CARTESIAN_POINT ( 'NONE',  ( 206.7044739906782809, 272.6243442267827959, -10.28926534613781030 ) ) ;
#7951=CARTESIAN_POINT ( 'NONE',  ( 148.4832040919255292, 276.1351389192656143, -5.425582376124524764 ) ) ;
#7954=CARTESIAN_POINT ( 'NONE',  ( 182.0016526522884135, 263.2485514694740800, 14.07076055901416112 ) ) ;
#7956=CARTESIAN_POINT ( 'NONE',  ( 183.4628397030323015, 284.7042858584374017, -15.01390401402201213 ) ) ;
#7957=CARTESIAN_POINT ( 'NONE',  ( 122.2582625392304863, 232.2048013555409796, 4.594050593750051981 ) ) ;
#7958=CARTESIAN_POINT ( 'NONE',  ( 186.4788919898187203, 262.6505567889508370, -9.037439985774382123 ) ) ;
#7960=CARTESIAN_POINT ( 'NONE',  ( 177.3572886147324823, 288.7233493041218821, -9.936058525762780036 ) ) ;
#7961=ORIENTED_EDGE ( 'NONE', *, *, #43432, .T. ) ;
#7966=CARTESIAN_POINT ( 'NONE',  ( 180.2794780956456293, 294.9385830392915864, -2.005224010670390022 ) ) ;
#7967=CARTESIAN_POINT ( 'NONE',  ( 203.5726949774746117, 269.0034548673361883, -6.096665150295551783 ) ) ;
#7969=CARTESIAN_POINT ( 'NONE',  ( 201.3053499423511425, 281.9759013948520874, -16.75960365258566398 ) ) ;
#7970=CARTESIAN_POINT ( 'NONE',  ( 173.8410576106227552, 287.9787963164463918, -9.990854418439887752 ) ) ;
#7971=ORIENTED_EDGE ( 'NONE', *, *, #96808, .F. ) ;
#7973=CARTESIAN_POINT ( 'NONE',  ( 175.9428832018305400, 255.2228740406303871, -7.310609490979488534 ) ) ;
#7974=ORIENTED_EDGE ( 'NONE', *, *, #37580, .T. ) ;
#7975=CARTESIAN_POINT ( 'NONE',  ( 148.1632261683078013, 274.0207597936089883, -7.853210555358286271 ) ) ;
#7976=CARTESIAN_POINT ( 'NONE',  ( 200.1294354126899009, 267.3366221627135246, -6.812218948514619399 ) ) ;
#7977=ORIENTED_EDGE ( 'NONE', *, *, #11020, .F. ) ;
#7978=CARTESIAN_POINT ( 'NONE',  ( 191.4451218093941804, 267.1586281749990235, -12.73097342071060289 ) ) ;
#7979=CARTESIAN_POINT ( 'NONE',  ( 160.0225884613553262, 278.6577504188115881, 10.44739908625478186 ) ) ;
#7980=CARTESIAN_POINT ( 'NONE',  ( 193.6750207660124374, 264.1248559586345550, 4.439471659852311625 ) ) ;
#7981=CARTESIAN_POINT ( 'NONE',  ( 158.4419986971542471, 263.4018671416569077, 17.51825679525311230 ) ) ;
#7982=CARTESIAN_POINT ( 'NONE',  ( 204.6046391762972689, 273.0979756738785795, -10.26949011951421298 ) ) ;
#7983=CARTESIAN_POINT ( 'NONE',  ( 152.3764452470134358, 269.7209059243594993, 14.08360062969545368 ) ) ;
#7984=CARTESIAN_POINT ( 'NONE',  ( 160.2115073521705710, 281.2659082526984662, 5.619886021066055726 ) ) ;
#7985=CARTESIAN_POINT ( 'NONE',  ( 200.8251833487811666, 282.8075743310126882, -16.74393672780000131 ) ) ;
#7987=CARTESIAN_POINT ( 'NONE',  ( 147.4368675721658519, 275.2788497866417288, 5.050119523016719292 ) ) ;
#7989=CARTESIAN_POINT ( 'NONE',  ( 163.9293054476912630, 248.0008627108990993, -8.754753442298728316 ) ) ;
#7992=EDGE_CURVE ( 'NONE', #63243, #33752, #91810, .T. ) ;
#7993=CARTESIAN_POINT ( 'NONE',  ( 188.5978122785818414, 298.5986698468521467, -4.210741860408480974 ) ) ;
#7995=ADVANCED_FACE ( 'NONE', ( #53131 ), #12885, .F. ) ;
#7996=CARTESIAN_POINT ( 'NONE',  ( 57.59477206639473224, 197.3927522451417929, -10.00000000000009237 ) ) ;
#7997=CARTESIAN_POINT ( 'NONE',  ( 194.2199708651012600, 294.2481379475345875, 15.50834247347371253 ) ) ;
#8001=CARTESIAN_POINT ( 'NONE',  ( 69.94448162217048548, 217.3149278399160949, -9.188101187500095079 ) ) ;
#8003=B_SPLINE_CURVE_WITH_KNOTS ( 'NONE', 3,
 ( #70684, #86452, #94527, #10401 ),
 .UNSPECIFIED., .F., .F.,
 ( 4, 4 ),
 ( 0.01296045245666641033, 0.01919682551789810704 ),
 .UNSPECIFIED. ) ;
#8005=CARTESIAN_POINT ( 'NONE',  ( 208.1612901671020381, 270.1010645919285480, -2.401583477149568768 ) ) ;
#8008=CARTESIAN_POINT ( 'NONE',  ( 202.8874463667715133, 279.2356300052831557, -15.29930322226033468 ) ) ;
#8012=CARTESIAN_POINT ( 'NONE',  ( 43.23318412030275226, 195.7677522451418781, 10.00000000000009592 ) ) ;
#8015=CARTESIAN_POINT ( 'NONE',  ( 169.2469165748500188, 252.1036659777226703, -8.798953830286828648 ) ) ;
#8016=CARTESIAN_POINT ( 'NONE',  ( 164.0701913188777041, 246.4690879585942866, -4.479195405916993167 ) ) ;
#8017=CARTESIAN_POINT ( 'NONE',  ( 196.0395593785976018, 291.0965181932902510, 15.97855489120023087 ) ) ;
#8018=CARTESIAN_POINT ( 'NONE',  ( 172.3741624485570867, 252.4865239976215037, 8.880853820034850798 ) ) ;
#8021=CARTESIAN_POINT ( 'NONE',  ( 30.62142885764206568, 197.6744531367911293, 4.594050593750047540 ) ) ;
#8022=CARTESIAN_POINT ( 'NONE',  ( 62.82726920452340380, 197.8923013555409796, 4.594050593750050204 ) ) ;
#8023=CARTESIAN_POINT ( 'NONE',  ( 58.91185237153143106, 211.4865022471902876, -10.00000000000009592 ) ) ;
#8025=CARTESIAN_POINT ( 'NONE',  ( -6.761740748788464650, 160.2365022471902023, 10.00000000000009592 ) ) ;
#8027=CARTESIAN_POINT ( 'NONE',  ( 196.4711259686879146, 269.6575937712059385, -10.81078490099711864 ) ) ;
#8030=CARTESIAN_POINT ( 'NONE',  ( 149.0164813726494799, 272.5428784278667536, -11.67305721329070423 ) ) ;
#8032=CARTESIAN_POINT ( 'NONE',  ( 62.50250967810423930, 197.7048013555409796, 4.594050593750051981 ) ) ;
#8035=CARTESIAN_POINT ( 'NONE',  ( 198.3075590527773784, 287.1682275260610027, 16.94807365630277118 ) ) ;
#8036=CARTESIAN_POINT ( 'NONE',  ( 185.8492146212669240, 258.6745004276652935, -5.862532207920108540 ) ) ;
#8037=CARTESIAN_POINT ( 'NONE',  ( 153.3739204864665169, 276.7760111581692399, 7.465203695501545056 ) ) ;
#8040=CARTESIAN_POINT ( 'NONE',  ( 112.2445834879231086, 235.6115022471902307, 10.00000000000009592 ) ) ;
#8041=CARTESIAN_POINT ( 'NONE',  ( 11.48687755014677947, 188.9860189848785410, -2.679491924311252493 ) ) ;
#8042=CARTESIAN_POINT ( 'NONE',  ( 207.6209998424140792, 271.0368748851258260, 6.610167240481342965 ) ) ;
#8043=VERTEX_POINT ( 'NONE', #38647 ) ;
#8047=CARTESIAN_POINT ( 'NONE',  ( 206.5237403681858552, 272.9373840435757188, -10.81420335655575116 ) ) ;
#8048=CARTESIAN_POINT ( 'NONE',  ( 194.0630436426056633, 294.0785447019548542, 13.99500891659908852 ) ) ;
#8052=ORIENTED_EDGE ( 'NONE', *, *, #15658, .F. ) ;
#8054=CARTESIAN_POINT ( 'NONE',  ( 194.4032909867620447, 293.9306181827685123, -16.05392006271526384 ) ) ;
#8059=CARTESIAN_POINT ( 'NONE',  ( 179.4408063581041688, 277.4340371255875652, 17.62723233342114071 ) ) ;
#8061=CARTESIAN_POINT ( 'NONE',  ( 182.4832887632573488, 293.7996546558092632, 9.189678001673824426 ) ) ;
#8062=CARTESIAN_POINT ( 'NONE',  ( -3.027006198515987734, 162.3927522451418213, 10.00000000000009948 ) ) ;
#8063=ORIENTED_EDGE ( 'NONE', *, *, #79934, .F. ) ;
#8067=CARTESIAN_POINT ( 'NONE',  ( 207.6837091943624785, 270.9282591014416539, -1.156610046911421552 ) ) ;
#8068=CARTESIAN_POINT ( 'NONE',  ( 204.5133713884061706, 276.4194452585140311, 14.87364779308245843 ) ) ;
#8070=CARTESIAN_POINT ( 'NONE',  ( 205.1300674467857164, 275.3512963525735131, -12.60245643603069610 ) ) ;
#8071=B_SPLINE_CURVE_WITH_KNOTS ( 'NONE', 3,
 ( #51600, #28289, #35894, #96748 ),
 .UNSPECIFIED., .F., .F.,
 ( 4, 4 ),
 ( 0.009085677135906682078, 0.01422205901525189567 ),
 .UNSPECIFIED. ) ;
#8073=CARTESIAN_POINT ( 'NONE',  ( 138.9560545341254851, 251.0333772461660260, 9.188101187500095079 ) ) ;
#8075=CARTESIAN_POINT ( 'NONE',  ( 166.5418805794664934, 264.7512503615053561, 17.71810435351582669 ) ) ;
#8076=CARTESIAN_POINT ( 'NONE',  ( 181.3477783452750316, 260.0325310163331096, 9.501399873363059356 ) ) ;
#8077=CARTESIAN_POINT ( 'NONE',  ( 81.12205585946965414, 208.4548013555409796, -4.594050593750042211 ) ) ;
#8079=CARTESIAN_POINT ( 'NONE',  ( 191.5451565139252068, 298.8810523045859213, 7.782291334092181323 ) ) ;
#8081=ORIENTED_EDGE ( 'NONE', *, *, #91677, .F. ) ;
#8085=CARTESIAN_POINT ( 'NONE',  ( 197.9292284917571862, 286.8924113709215362, 16.93415600513534969 ) ) ;
#8086=CARTESIAN_POINT ( 'NONE',  ( 147.2999496562918296, 275.5159985734018164, -0.1418322875769767455 ) ) ;
#8089=CARTESIAN_POINT ( 'NONE',  ( 86.64296780859545777, 211.6423013555409796, -4.594050593750043987 ) ) ;
#8090=ORIENTED_EDGE ( 'NONE', *, *, #96617, .T. ) ;
#8094=CARTESIAN_POINT ( 'NONE',  ( 200.3809179181201614, 283.5770646289640240, -17.08954332461089365 ) ) ;
#8095=ORIENTED_EDGE ( 'NONE', *, *, #39768, .T. ) ;
#8097=CARTESIAN_POINT ( 'NONE',  ( 184.1785766904203001, 275.2410092694960895, 16.37069233236986676 ) ) ;
#8098=CARTESIAN_POINT ( 'NONE',  ( 164.6869624841032191, 245.4008089637804346, 1.435659848726088317 ) ) ;
#8100=CARTESIAN_POINT ( 'NONE',  ( 162.5148320529283126, 285.2034568178174254, 0.5437328601018158736 ) ) ;
#8103=ORIENTED_EDGE ( 'NONE', *, *, #42003, .T. ) ;
#8105=CARTESIAN_POINT ( 'NONE',  ( 186.0258092806693355, 259.0446144625114471, 6.352418251517233827 ) ) ;
#8107=CARTESIAN_POINT ( 'NONE',  ( 152.8721808860877616, 265.8646109718731623, -17.65676496037632504 ) ) ;
#8111=ORIENTED_EDGE ( 'NONE', *, *, #81856, .F. ) ;
#8112=CARTESIAN_POINT ( 'NONE',  ( 195.7809538458540999, 265.2618777367464418, 5.140530321345854858 ) ) ;
#8113=CYLINDRICAL_SURFACE ( 'NONE', #74186, 17.82106496071139645 ) ;
#8115=CARTESIAN_POINT ( 'NONE',  ( 170.2203850864397339, 251.3096531866638657, 6.994710684270507350 ) ) ;
#8119=VERTEX_POINT ( 'NONE', #9775 ) ;
#8120=CARTESIAN_POINT ( 'NONE',  ( 182.6549766561670651, 262.8541459689510020, 13.52474329316464896 ) ) ;
#8122=CARTESIAN_POINT ( 'NONE',  ( 205.2121761402296443, 275.2090799237855094, -14.05269615702442465 ) ) ;
#8125=CARTESIAN_POINT ( 'NONE',  ( 59.71366722694061480, 216.8297689869269220, -2.679491924311252493 ) ) ;
#8127=CARTESIAN_POINT ( 'NONE',  ( 162.6991225460172927, 284.8212170328912975, -3.897741803361528756 ) ) ;
#8129=CARTESIAN_POINT ( 'NONE',  ( 191.3281377348044714, 262.2149640667300332, 2.921411013909792853 ) ) ;
#8130=CARTESIAN_POINT ( 'NONE',  ( -17.68663747114990770, 172.8464784336661353, 1.353441290958777327E-15 ) ) ;
#8131=FACE_OUTER_BOUND ( 'NONE', #15741, .T. ) ;
#8134=CARTESIAN_POINT ( 'NONE',  ( 175.0396866787711474, 255.0033583533873980, 9.305020555032612606 ) ) ;
#8136=CARTESIAN_POINT ( 'NONE',  ( 160.5893190321802138, 270.9897182155185078, 16.60663562724527864 ) ) ;
#8137=CARTESIAN_POINT ( 'NONE',  ( 23.01690360248371903, 184.0958772461660544, -9.188101187500095079 ) ) ;
#8140=CARTESIAN_POINT ( 'NONE',  ( 172.1705709408975054, 271.8423139197483920, -16.44096766034999035 ) ) ;
#8143=CARTESIAN_POINT ( 'NONE',  ( 187.7916437398309313, 259.1520801313256470, -0.7955774063839984311 ) ) ;
#8144=AXIS2_PLACEMENT_3D ( 'NONE', #3520, #96240, #26800 ) ;
#8145=CARTESIAN_POINT ( 'NONE',  ( 78.97477422587097351, 209.7365022471902023, 10.00000000000009592 ) ) ;
#8146=CARTESIAN_POINT ( 'NONE',  ( 164.4888076835817401, 246.1997653861143647, 1.812879387509452656 ) ) ;
#8147=CARTESIAN_POINT ( 'NONE',  ( 206.7596416265183734, 271.4678399409689291, 6.202658291405857227 ) ) ;
#8148=CARTESIAN_POINT ( 'NONE',  ( 25.61497981383703149, 185.5958772461660544, -9.188101187500095079 ) ) ;
#8149=CARTESIAN_POINT ( 'NONE',  ( 120.4921787521148246, 228.8262482093457777, 3.021315404115420679E-15 ) ) ;
#8152=CARTESIAN_POINT ( 'NONE',  ( 151.1699610800269511, 268.8129421616204695, -14.28929860221299286 ) ) ;
#8155=CARTESIAN_POINT ( 'NONE',  ( 163.1227589771032456, 280.8252380815225138, -10.04696615151233630 ) ) ;
#8156=CARTESIAN_POINT ( 'NONE',  ( 163.7939847032603780, 282.2082574975837019, 10.05568170618017554 ) ) ;
#8159=CARTESIAN_POINT ( 'NONE',  ( 148.3190727836317535, 273.7508255376806119, 8.080277324579027365 ) ) ;
#8161=EDGE_CURVE ( 'NONE', #87772, #65984, #36864, .T. ) ;
#8162=CARTESIAN_POINT ( 'NONE',  ( 189.0689802957956260, 269.8288687927027354, -15.50864081522695415 ) ) ;
#8164=CARTESIAN_POINT ( 'NONE',  ( 185.3610915123994118, 291.1297846198819457, 13.42384461072851387 ) ) ;
#8176=VERTEX_POINT ( 'NONE', #92884 ) ;
#8177=CARTESIAN_POINT ( 'NONE',  ( 189.5516473586634731, 274.6233775832965875, -15.96870692800988678 ) ) ;
#8180=CARTESIAN_POINT ( 'NONE',  ( 201.1060504099706350, 282.3210983108598384, -18.18000168485860257 ) ) ;
#8185=CARTESIAN_POINT ( 'NONE',  ( 148.3837145175834280, 273.6388627701866767, 8.841971351370922605 ) ) ;
#8187=VERTEX_POINT ( 'NONE', #55821 ) ;
#8188=CARTESIAN_POINT ( 'NONE',  ( 157.0935036675524827, 258.5530654392286465, 17.32636058289560665 ) ) ;
#8189=CARTESIAN_POINT ( 'NONE',  ( 160.9230069893865789, 266.6111081704525532, 16.55276295507343320 ) ) ;
#8192=CARTESIAN_POINT ( 'NONE',  ( 149.1856130393175306, 272.2499337880290682, 11.44243872309708188 ) ) ;
#8196=CARTESIAN_POINT ( 'NONE',  ( 190.7851751463332164, 300.1973786460605425, 8.237717828100052486 ) ) ;
#8197=CARTESIAN_POINT ( 'NONE',  ( 167.7294354343802354, 268.7536494340877766, 17.80279610524468126 ) ) ;
#8198=CARTESIAN_POINT ( 'NONE',  ( -17.42236680055705023, 149.2012482093457777, 0.000000000000000000 ) ) ;
#8203=CARTESIAN_POINT ( 'NONE',  ( 180.7942833579522812, 266.7097690628117448, -16.23795806611159520 ) ) ;
#8204=CARTESIAN_POINT ( 'NONE',  ( 148.3190727836317535, 273.7508255376806119, 8.080277324579027365 ) ) ;
#8206=CARTESIAN_POINT ( 'NONE',  ( 190.7222376050763444, 300.3063896652212179, 3.365789908110941475 ) ) ;
#8207=CARTESIAN_POINT ( 'NONE',  ( 171.3649617487770911, 251.0102673366500596, 7.372720983288576946 ) ) ;
#8209=CARTESIAN_POINT ( 'NONE',  ( 193.2100161762185735, 295.9974307820218087, -12.46499585622781758 ) ) ;
#8210=DIRECTION ( 'NONE',  ( 0.4999999999999998890, -0.8660254037844385966, 0.000000000000000000 ) ) ;
#8216=CARTESIAN_POINT ( 'NONE',  ( 111.8384605302426991, 241.5024278399160664, -9.188101187500093303 ) ) ;
#8218=CARTESIAN_POINT ( 'NONE',  ( 147.3047606266276546, 275.5076657283461827, -0.02269072295920609994 ) ) ;
#8221=ADVANCED_FACE ( 'NONE', ( #77677 ), #51703, .F. ) ;
#8223=CARTESIAN_POINT ( 'NONE',  ( 155.5322964227545413, 261.2571557083629159, -18.35853982030605280 ) ) ;
#8224=CARTESIAN_POINT ( 'NONE',  ( 164.2712161151136172, 246.1209027979328710, 7.276091357954241445 ) ) ;
#8226=CARTESIAN_POINT ( 'NONE',  ( 169.2964062698280543, 285.1489873681304630, -7.912550111543783515 ) ) ;
#8229=B_SPLINE_CURVE_WITH_KNOTS ( 'NONE', 3,
 ( #8918, #63118, #25111, #47899 ),
 .UNSPECIFIED., .F., .F.,
 ( 4, 4 ),
 ( 0.04273337087810722551, 0.04887066958154943214 ),
 .UNSPECIFIED. ) ;
#8233=CARTESIAN_POINT ( 'NONE',  ( 128.5905526607566856, 254.2369531367911293, -4.594050593750048428 ) ) ;
#8234=CARTESIAN_POINT ( 'NONE',  ( 198.5511052797322975, 286.7463930869835167, -17.24711022262289006 ) ) ;
#8236=CYLINDRICAL_SURFACE ( 'NONE', #62725, 17.82106496071139645 ) ;
#8237=CARTESIAN_POINT ( 'NONE',  ( 157.4656258344471098, 257.9085309395441641, 18.30485740784190796 ) ) ;
#8238=CARTESIAN_POINT ( 'NONE',  ( 167.5421813246326792, 287.5986610761024167, 3.969292590682533373 ) ) ;
#8239=CARTESIAN_POINT ( 'NONE',  ( 55.76366273096530080, 196.8768266524160140, 9.188101187500098632 ) ) ;
#8243=ADVANCED_FACE ( 'NONE', ( #97632 ), #22620, .F. ) ;
#8244=CARTESIAN_POINT ( 'NONE',  ( 191.4420812244453600, 260.8157448279923187, -1.331758356259544085 ) ) ;
#8247=CARTESIAN_POINT ( 'NONE',  ( 15.77842244150312645, 191.4637435831425307, 2.679491924311251605 ) ) ;
#8248=CARTESIAN_POINT ( 'NONE',  ( 190.4240181651484818, 300.8229208869809668, -4.214281362166949485 ) ) ;
#8250=CARTESIAN_POINT ( 'NONE',  ( 202.9547455376043672, 279.1190644220934018, -15.19669173352461478 ) ) ;
#8251=CARTESIAN_POINT ( 'NONE',  ( 181.5435273739199715, 262.6800588168453032, 12.44797431397677379 ) ) ;
#8252=CARTESIAN_POINT ( 'NONE',  ( 117.3505249275209792, 231.8927522451417929, -10.00000000000009059 ) ) ;
#8253=CARTESIAN_POINT ( 'NONE',  ( 194.5617139857802442, 293.2599130566108556, -14.58798304743176821 ) ) ;
#8255=B_SPLINE_CURVE_WITH_KNOTS ( 'NONE', 3,
 ( #96730, #12603, #58178, #89636 ),
 .UNSPECIFIED., .F., .F.,
 ( 4, 4 ),
 ( 0.000000000000000000, 0.002752262309457068155 ),
 .UNSPECIFIED. ) ;
#8256=CARTESIAN_POINT ( 'NONE',  ( 189.8147415777049218, 301.8782188922952514, -0.5019643756309712934 ) ) ;
#8258=CARTESIAN_POINT ( 'NONE',  ( 23.88258191050314494, 196.8464784336661637, 1.353441290958777327E-15 ) ) ;
#8262=B_SPLINE_CURVE_WITH_KNOTS ( 'NONE', 3,
 ( #63642, #33241, #78362, #95093, #78865, #10452, #87527, #47926, #17034, #24638, #9451, #41325, #1354, #18058, #16538, #88012, #33766, #63139, #1855, #41835, #47434, #25658, #62623, #40323, #39810, #56537, #10963, #80393, #56016, #70742, #87012, #17541, #64654, #48954, #32239, #48448, #32737, #24145, #95604, #94084, #72269, #93578, #9959, #86506, #40818, #2363, #55030, #86012, #3851, #82398, #66635, #97087, #27656, #96591 ),
 .UNSPECIFIED., .F., .F.,
 ( 4, 2, 2, 2, 2, 2, 2, 2, 2, 2, 2, 2, 2, 2, 2, 2, 2, 2, 2, 2, 2, 2, 2, 2, 2, 2, 4 ),
 ( 0.0006996174624294505600, 0.0009087055706953546834, 0.001117793678961258915, 0.001222337733094224855, 0.001326881787227190794, 0.001431425841360156950, 0.001535969895493122890, 0.001745058003759054552, 0.001954146112024986864, 0.002372322328556768223, 0.003208674761620287138, 0.004045027194683806053, 0.004881379627747325402, 0.005299555844279047780, 0.005508643952544909836, 0.005613188006677764103, 0.005665460033744189501, 0.005717732060810614900, 0.005770004087877040298, 0.005822276114943466564, 0.005926820169076324300, 0.006135908277342071865, 0.006554084493873547045, 0.006763172602139241700, 0.006972260710404936355, 0.007181348818670631011, 0.007390436926936325666 ),
 .UNSPECIFIED. ) ;
#8264=CARTESIAN_POINT ( 'NONE',  ( 177.4980249182310104, 288.1765118805776069, 10.70887779921548422 ) ) ;
#8265=CARTESIAN_POINT ( 'NONE',  ( 62.31280629920263436, 206.7833772461660828, -9.188101187500095079 ) ) ;
#8266=CARTESIAN_POINT ( 'NONE',  ( 200.1385401540174769, 283.9968752310148830, 17.30012534137638625 ) ) ;
#8271=CARTESIAN_POINT ( 'NONE',  ( 30.33301404664494427, 194.9865022471903160, -10.00000000000009415 ) ) ;
#8273=CARTESIAN_POINT ( 'NONE',  ( -16.90171517502901466, 170.2369531367911293, -4.594050593750048428 ) ) ;
#8275=CARTESIAN_POINT ( 'NONE',  ( 167.3985425305344563, 262.3805089322066237, -16.46154190842169740 ) ) ;
#8276=CARTESIAN_POINT ( 'NONE',  ( 186.6027929891679662, 261.0133341855545268, 6.348929212563308333 ) ) ;
#8277=CARTESIAN_POINT ( 'NONE',  ( 205.8452707775803390, 274.1125278458945900, 11.42742867493066328 ) ) ;
#8280=ORIENTED_EDGE ( 'NONE', *, *, #31399, .T. ) ;
#8281=CARTESIAN_POINT ( 'NONE',  ( -22.42236680055709641, 157.8615022471902591, 0.000000000000000000 ) ) ;
#8283=LINE ( 'NONE', #15868, #38586 ) ;
#8285=VERTEX_POINT ( 'NONE', #99116 ) ;
#8286=CARTESIAN_POINT ( 'NONE',  ( 159.8869478387880747, 253.7146782065408672, 15.67510143967828995 ) ) ;
#8287=EDGE_CURVE ( 'NONE', #15150, #11106, #69133, .T. ) ;
#8290=EDGE_CURVE ( 'NONE', #47161, #11048, #87902, .T. ) ;
#8291=CARTESIAN_POINT ( 'NONE',  ( 153.3100492430090753, 265.1062007306585997, 16.32434963471121492 ) ) ;
#8292=CARTESIAN_POINT ( 'NONE',  ( 207.6628070930962906, 270.9644626028195376, 7.378217122120054761 ) ) ;
#8293=CARTESIAN_POINT ( 'NONE',  ( 149.6775655717086124, 272.1443760297916583, 11.34356142435849968 ) ) ;
#8294=CARTESIAN_POINT ( 'NONE',  ( 162.6757594134126350, 248.8843148665554281, -10.86406770146305867 ) ) ;
#8296=CARTESIAN_POINT ( 'NONE',  ( 200.7484899876179441, 282.9404111291507888, -16.88964748465601673 ) ) ;
#8297=ORIENTED_EDGE ( 'NONE', *, *, #78443, .T. ) ;
#8301=ORIENTED_EDGE ( 'NONE', *, *, #52583, .F. ) ;
#8302=LINE ( 'NONE', #85340, #7862 ) ;
#8304=VERTEX_POINT ( 'NONE', #77298 ) ;
#8305=ADVANCED_FACE ( 'NONE', ( #29698 ), #82946, .T. ) ;
#8307=CARTESIAN_POINT ( 'NONE',  ( 180.2836023094594395, 259.4510097613480752, -11.78144428920749753 ) ) ;
#8308=CARTESIAN_POINT ( 'NONE',  ( 149.2923684163597784, 272.0650280510108701, -12.99082738998495756 ) ) ;
#8311=CARTESIAN_POINT ( 'NONE',  ( 203.6735071151937575, 277.8741328511802635, 15.93813992116388434 ) ) ;
#8312=CARTESIAN_POINT ( 'NONE',  ( 151.3284628043366524, 268.5384091220288383, 14.49047510809488237 ) ) ;
#8315=EDGE_CURVE ( 'NONE', #82473, #7026, #12805, .T. ) ;
#8317=EDGE_CURVE ( 'NONE', #26527, #41212, #18910, .T. ) ;
#8318=EDGE_LOOP ( 'NONE', ( #92089, #92490, #7204, #44804, #47810, #34508, #32729 ) ) ;
#8321=LINE ( 'NONE', #84359, #65467 ) ;
#8323=CARTESIAN_POINT ( 'NONE',  ( 164.3053959849042087, 246.0617015268593661, -7.251939739328854273 ) ) ;
#8325=CARTESIAN_POINT ( 'NONE',  ( 167.8360140743272666, 281.0956243233280816, 11.63507309386356248 ) ) ;
#8326=CARTESIAN_POINT ( 'NONE',  ( 147.7112127936102866, 274.8036699242858276, -9.124700685424272706 ) ) ;
#8328=CARTESIAN_POINT ( 'NONE',  ( 158.9097751959179448, 255.4071908717584449, -17.55082260428511631 ) ) ;
#8331=CARTESIAN_POINT ( 'NONE',  ( 163.8187377589169955, 282.1776765746977844, 8.479121753608614753 ) ) ;
#8332=DIRECTION ( 'NONE',  ( -0.8660254037844387076, -0.4999999999999998890, -0.000000000000000000 ) ) ;
#8333=CARTESIAN_POINT ( 'NONE',  ( 159.5764336135613632, 254.2525046211064819, 15.32981087583629076 ) ) ;
#8335=CARTESIAN_POINT ( 'NONE',  ( 190.4882032423914211, 300.7117490721083755, 5.365042449410100112 ) ) ;
#8336=EDGE_CURVE ( 'NONE', #82018, #90758, #77814, .T. ) ;
#8337=FACE_OUTER_BOUND ( 'NONE', #45670, .T. ) ;
#8338=CARTESIAN_POINT ( 'NONE',  ( 159.9788992190088948, 253.5554137441726255, -15.81862932303382330 ) ) ;
#8344=CARTESIAN_POINT ( 'NONE',  ( 194.0719046999502666, 294.5045960684578858, -14.15255333265519333 ) ) ;
#8345=EDGE_CURVE ( 'NONE', #66029, #36928, #44159, .T. ) ;
#8348=CARTESIAN_POINT ( 'NONE',  ( 7.365298646897277202, 168.3927522451418213, 10.00000000000009592 ) ) ;
#8349=CARTESIAN_POINT ( 'NONE',  ( 84.34250105585179824, 213.3768266524160140, 9.188101187500096856 ) ) ;
#8351=ADVANCED_FACE ( 'NONE', ( #78808 ), #84139, .F. ) ;
#8353=CARTESIAN_POINT ( 'NONE',  ( 167.0511520614714129, 278.3166273224070437, -13.37090358088792286 ) ) ;
#8354=CARTESIAN_POINT ( 'NONE',  ( 170.8054577101068219, 287.4915981561377976, 8.526299399445241178 ) ) ;
#8355=CARTESIAN_POINT ( 'NONE',  ( 9.864316330390064280, 170.3768266524160140, -9.188101187500091527 ) ) ;
#8358=CARTESIAN_POINT ( 'NONE',  ( 200.1444820856229967, 283.9865835035790269, 17.93386694781497326 ) ) ;
#8359=ORIENTED_EDGE ( 'NONE', *, *, #40222, .F. ) ;
#8361=ORIENTED_EDGE ( 'NONE', *, *, #38134, .F. ) ;
#8364=CARTESIAN_POINT ( 'NONE',  ( 198.7984568860927084, 266.5006840448155572, -2.860727480615956608 ) ) ;
#8367=CARTESIAN_POINT ( 'NONE',  ( 144.6270795744234476, 268.7413018095040798, -2.761272660171008000E-15 ) ) ;
#8368=CARTESIAN_POINT ( 'NONE',  ( 113.8346084569740242, 224.9824982072974251, 3.021315404115420679E-15 ) ) ;
#8370=CARTESIAN_POINT ( 'NONE',  ( 30.97368554763575688, 182.5643266524159856, -9.188101187500093303 ) ) ;
#8371=CARTESIAN_POINT ( 'NONE',  ( 128.5097966488581562, 238.8768266524159856, 9.188101187500098632 ) ) ;
#8372=CARTESIAN_POINT ( 'NONE',  ( 196.9839693152069344, 276.0740101548715302, 15.26896795715265220 ) ) ;
#8374=CARTESIAN_POINT ( 'NONE',  ( 206.8217325168575371, 270.0045844243117017, 3.350393751014514532 ) ) ;
#8375=CARTESIAN_POINT ( 'NONE',  ( 181.9483594117699568, 259.9271416659100851, -11.10351924915216948 ) ) ;
#8378=CARTESIAN_POINT ( 'NONE',  ( 155.3017250444513024, 261.6565170503553190, 18.58368563027307374 ) ) ;
#8379=CARTESIAN_POINT ( 'NONE',  ( 161.8882824960653579, 250.2482648971885340, -13.83574485983625557 ) ) ;
#8381=CARTESIAN_POINT ( 'NONE',  ( 194.2154056360670040, 294.2560451561701029, -15.66696967429384557 ) ) ;
#8382=CARTESIAN_POINT ( 'NONE',  ( 191.8200757322313166, 264.7651863584280250, 7.775292329195298890 ) ) ;
#8384=CARTESIAN_POINT ( 'NONE',  ( 18.71383987920370728, 191.6115022471903160, -5.000000000000047962 ) ) ;
#8385=CARTESIAN_POINT ( 'NONE',  ( 146.6138605399200117, 276.7043397814778132, -0.5394499176159462950 ) ) ;
#8386=CARTESIAN_POINT ( 'NONE',  ( 148.2267527339363369, 273.9107285543102535, 7.913369084260907016 ) ) ;
#8391=CARTESIAN_POINT ( 'NONE',  ( 110.6480226958041158, 228.5643266524160708, 9.188101187500095079 ) ) ;
#8393=CARTESIAN_POINT ( 'NONE',  ( 190.9501423151522772, 299.9116471280854626, 8.746938802470586083 ) ) ;
#8395=CARTESIAN_POINT ( 'NONE',  ( 144.5581563630821051, 244.2677522451417929, -5.000000000000041744 ) ) ;
#8397=CARTESIAN_POINT ( 'NONE',  ( 190.8990369860722183, 300.0001641545892994, -8.015708032567667729 ) ) ;
#8399=CARTESIAN_POINT ( 'NONE',  ( 196.4808189786114951, 290.3322341467384717, -17.84817245450773271 ) ) ;
#8400=CARTESIAN_POINT ( 'NONE',  ( 192.5076277540105423, 297.2140032159341558, -13.10094381206144298 ) ) ;
#8403=CARTESIAN_POINT ( 'NONE',  ( 192.8451718961534311, 267.2100971994023553, 11.16589986606910756 ) ) ;
#8404=CARTESIAN_POINT ( 'NONE',  ( 177.5337925685473408, 280.1858537220425092, 16.79564202278857721 ) ) ;
#8405=CARTESIAN_POINT ( 'NONE',  ( 196.8542736181493922, 268.1164828960293676, 9.403776070750170746 ) ) ;
#8407=B_SPLINE_SURFACE_WITH_KNOTS ( 'NONE', 3, 1, ( 
 ( #32735, #1853 ),
 ( #96589, #64652 ),
 ( #17538, #26646 ),
 ( #49941, #72266 ),
 ( #26149, #3848 ),
 ( #41322, #19572 ),
 ( #9447, #27153 ),
 ( #40816, #19067 ),
 ( #33762, #57027 ),
 ( #49437, #87010 ),
 ( #71259, #2872 ),
 ( #18558, #79391 ),
 ( #80390, #63639 ),
 ( #48445, #25132 ),
 ( #9957, #56014 ),
 ( #64141, #71763 ),
 ( #87524, #2359 ),
 ( #56535, #34732 ),
 ( #10960, #33237 ),
 ( #41832, #72778 ),
 ( #95091, #18056 ),
 ( #25655, #34244 ),
 ( #65140, #88505 ),
 ( #65632, #11472 ),
 ( #80901, #50432 ),
 ( #42326, #73254 ),
 ( #58038, #44317 ),
 ( #75747, #74269 ),
 ( #11955, #82877 ),
 ( #12453, #43323 ),
 ( #91459, #90487 ),
 ( #36222, #6330 ),
 ( #82394, #60503 ),
 ( #81387, #99047 ) ),
 .UNSPECIFIED., .T., .F., .F.,
 ( 4, 2, 2, 2, 2, 2, 2, 2, 2, 2, 2, 2, 2, 2, 2, 2, 4 ),
 ( 2, 2 ),
 ( 0.000000000000000000, 0.06250000000000000000, 0.1250000000000000000, 0.1875000000000000000, 0.2500000000000000000, 0.3125000000000000000, 0.3750000000000000000, 0.4375000000000000000, 0.5000000000000000000, 0.5625000000000000000, 0.6250000000000000000, 0.6875000000000000000, 0.7500000000000000000, 0.8125000000000000000, 0.8750000000000000000, 0.9375000000000000000, 1.000000000000000000 ),
 ( 0.000000000000000000, 1.000000000000000000 ),
 .UNSPECIFIED. ) ;
#8408=CARTESIAN_POINT ( 'NONE',  ( 190.6688270659779221, 284.0946164064107506, -17.60360843008351495 ) ) ;
#8409=CARTESIAN_POINT ( 'NONE',  ( 179.9379124811931945, 262.8721604542064370, -12.83149901144461147 ) ) ;
#8411=CARTESIAN_POINT ( 'NONE',  ( 175.7824178399792174, 285.8628427244275372, -13.39878279634721103 ) ) ;
#8416=CARTESIAN_POINT ( 'NONE',  ( 165.7186082895867685, 248.5901142549738836, 7.040988221872656716 ) ) ;
#8418=CARTESIAN_POINT ( 'NONE',  ( 204.4329329219251861, 276.5587687693421799, 13.28840463846547948 ) ) ;
#8422=CARTESIAN_POINT ( 'NONE',  ( 158.8391802440265508, 255.5294649151923636, 17.60341940305819364 ) ) ;
#8423=CARTESIAN_POINT ( 'NONE',  ( 192.8238735239056325, 296.6662494747970982, -11.98739424064265791 ) ) ;
#8424=CARTESIAN_POINT ( 'NONE',  ( 160.8697417715285951, 254.0124291816641176, 15.72951850990217437 ) ) ;
#8428=VERTEX_POINT ( 'NONE', #27606 ) ;
#8432=CARTESIAN_POINT ( 'NONE',  ( 163.4927498574098763, 249.4692459082536686, 11.48939803020791750 ) ) ;
#8433=EDGE_CURVE ( 'NONE', #23987, #52618, #46688, .T. ) ;
#8437=CARTESIAN_POINT ( 'NONE',  ( 170.2642345923708547, 269.6161715210895409, 17.76022440076183884 ) ) ;
#8440=CARTESIAN_POINT ( 'NONE',  ( 189.5059428776464756, 300.4130739301078279, -3.423561384717671796 ) ) ;
#8441=CARTESIAN_POINT ( 'NONE',  ( 164.9133935349224203, 245.0086188793504505, -2.355115420316610919 ) ) ;
#8442=CARTESIAN_POINT ( 'NONE',  ( 147.6498877563539338, 274.9098880045899591, -7.398802595780497704 ) ) ;
#8447=CARTESIAN_POINT ( 'NONE',  ( 178.2153940782017401, 255.1407320482941827, 5.786499683232065649 ) ) ;
#8448=CARTESIAN_POINT ( 'NONE',  ( 123.3944002380500677, 251.2369531367911293, -4.594050593750048428 ) ) ;
#8449=CARTESIAN_POINT ( 'NONE',  ( 186.6324081443715386, 262.7608654827037640, -9.067671514656064247 ) ) ;
#8451=CARTESIAN_POINT ( 'NONE',  ( 177.3599088863647353, 288.7283238914923800, -9.631439042632086611 ) ) ;
#8453=CARTESIAN_POINT ( 'NONE',  ( 202.4565886109826067, 275.5626669239693456, 13.30823948595258344 ) ) ;
#8454=CARTESIAN_POINT ( 'NONE',  ( 178.2432059713528645, 254.4564803675171163, 1.335616806069444884 ) ) ;
#8455=CARTESIAN_POINT ( 'NONE',  ( 173.6388580828917441, 290.5488920705779492, -4.957402522865826278 ) ) ;
#8456=CARTESIAN_POINT ( 'NONE',  ( 157.7365441389748923, 257.4392866714015895, 18.13124212464487073 ) ) ;
#8457=DIRECTION ( 'NONE',  ( 0.4999999999999992784, -0.8660254037844390407, 0.000000000000000000 ) ) ;
#8458=CARTESIAN_POINT ( 'NONE',  ( 152.6692142062575499, 266.2161595735824449, -16.77985299603479419 ) ) ;
#8459=CARTESIAN_POINT ( 'NONE',  ( 173.4606779374792325, 267.5814416807811540, -17.58000433512257032 ) ) ;
#8464=CARTESIAN_POINT ( 'NONE',  ( 200.5914588262792222, 282.7033700937254821, -16.73555027083989444 ) ) ;
#8466=CARTESIAN_POINT ( 'NONE',  ( 191.2366886875849161, 273.4737008325631109, 16.52053026652336243 ) ) ;
#8467=ORIENTED_EDGE ( 'NONE', *, *, #91733, .T. ) ;
#8468=CARTESIAN_POINT ( 'NONE',  ( 191.7469437388539859, 267.7966411536362443, -12.31490334707406831 ) ) ;
#8470=CARTESIAN_POINT ( 'NONE',  ( 190.8075292873213300, 283.8500300119202961, -16.71192585804572417 ) ) ;
#8471=CARTESIAN_POINT ( 'NONE',  ( 173.8469137325424185, 256.4471593116459189, -12.44389045026504270 ) ) ;
#8472=CARTESIAN_POINT ( 'NONE',  ( 182.3700640764176342, 263.2847133751610045, -13.94439451147478337 ) ) ;
#8474=CARTESIAN_POINT ( 'NONE',  ( 164.4287473828328245, 284.2046671292196720, -6.974946200865640655 ) ) ;
#8475=CARTESIAN_POINT ( 'NONE',  ( 154.9387540737944278, 277.5755234473050450, -8.926225623114506291 ) ) ;
#8479=CARTESIAN_POINT ( 'NONE',  ( 205.2147764766343414, 272.0456487616545473, -9.529409070406817506 ) ) ;
#8480=CARTESIAN_POINT ( 'NONE',  ( 188.6301707762981152, 265.0060877223691591, -12.46499516475016733 ) ) ;
#8484=CARTESIAN_POINT ( 'NONE',  ( 25.04665064082949755, 195.2677522451419350, -5.000000000000047962 ) ) ;
#8485=CARTESIAN_POINT ( 'NONE',  ( 184.5690160051166515, 296.9465964437451930, -4.422075520720778030 ) ) ;
#8486=FACE_OUTER_BOUND ( 'NONE', #25343, .T. ) ;
#8487=CARTESIAN_POINT ( 'NONE',  ( 32.84087927488948822, 189.7677522451418497, 10.00000000000009592 ) ) ;
#8488=CARTESIAN_POINT ( 'NONE',  ( 194.1153812227096864, 294.4292925221022870, 15.54001482840963710 ) ) ;
#8490=CARTESIAN_POINT ( 'NONE',  ( -16.14394294671762253, 170.6744531367911293, 4.594050593750047540 ) ) ;
#8491=CARTESIAN_POINT ( 'NONE',  ( 92.13672968991174628, 217.8768266524159856, 9.188101187500098632 ) ) ;
#8492=CARTESIAN_POINT ( 'NONE',  ( 31.70422093597033353, 189.1115022471902591, 10.00000000000009592 ) ) ;
#8493=CARTESIAN_POINT ( 'NONE',  ( 193.2053309019613891, 296.0055459150826778, -12.79465285318189061 ) ) ;
#8499=DIRECTION ( 'NONE',  ( 0.4999999999999998890, -0.8660254037844385966, 0.000000000000000000 ) ) ;
#8502=CARTESIAN_POINT ( 'NONE',  ( 161.2489332459614957, 251.3556502821494121, 13.48038699008507990 ) ) ;
#8503=CARTESIAN_POINT ( 'NONE',  ( 167.5395076046425800, 250.9340159416122447, -8.858151787760693452 ) ) ;
#8504=CARTESIAN_POINT ( 'NONE',  ( 161.5266078408477597, 251.3399204103630211, 13.01505764280997468 ) ) ;
#8505=CARTESIAN_POINT ( 'NONE',  ( 195.6986305151803549, 291.6870243064952888, 16.84182339398051909 ) ) ;
#8508=CARTESIAN_POINT ( 'NONE',  ( 161.3145230519951951, 251.2420454056404822, -14.44869077440025151 ) ) ;
#8509=CARTESIAN_POINT ( 'NONE',  ( 36.16983797034238535, 185.5643266524159856, -9.188101187500093303 ) ) ;
#8511=CARTESIAN_POINT ( 'NONE',  ( 75.14098114064213974, 208.0643266524159571, -9.188101187500093303 ) ) ;
#8512=CARTESIAN_POINT ( 'NONE',  ( 164.5641499066685469, 246.8022252770303169, -5.664862832761055955 ) ) ;
#8514=CARTESIAN_POINT ( 'NONE',  ( 167.2234229972659421, 259.6915297064097672, 16.30524142717095515 ) ) ;
#8515=CARTESIAN_POINT ( 'NONE',  ( 143.5566409438477820, 259.8149278399160949, 9.188101187500093303 ) ) ;
#8518=CARTESIAN_POINT ( 'NONE',  ( 14.20097916528452942, 190.5530062829863311, -4.648177544792955347E-16 ) ) ;
#8520=CARTESIAN_POINT ( 'NONE',  ( 150.6386650955079176, 269.7331738006648720, -15.06054658539322766 ) ) ;
#8523=CARTESIAN_POINT ( 'NONE',  ( 65.10058588945754821, 199.2048013555409796, 4.594050593750051981 ) ) ;
#8525=CARTESIAN_POINT ( 'NONE',  ( 202.8549823380854491, 279.2918593523859272, -16.39745931995414807 ) ) ;
#8526=CARTESIAN_POINT ( 'NONE',  ( 198.0858447170796524, 287.5522480202560018, 18.44384186289807559 ) ) ;
#8528=CARTESIAN_POINT ( 'NONE',  ( 153.3566685561987413, 276.8094205549507478, 7.774810562162696392 ) ) ;
#8530=CARTESIAN_POINT ( 'NONE',  ( 108.3474691708931630, 233.3615022471902591, -10.00000000000009592 ) ) ;
#8532=CARTESIAN_POINT ( 'NONE',  ( 206.9258336080761183, 272.2409381227055292, 6.776000910836894597 ) ) ;
#8533=ORIENTED_EDGE ( 'NONE', *, *, #96544, .T. ) ;
#8535=CARTESIAN_POINT ( 'NONE',  ( 184.7142690891777477, 271.2188788038347411, 16.19071692680373431 ) ) ;
#8536=ORIENTED_EDGE ( 'NONE', *, *, #63108, .F. ) ;
#8537=CARTESIAN_POINT ( 'NONE',  ( 159.6288139302610887, 254.1617792512662675, -15.32287760493869477 ) ) ;
#8538=CARTESIAN_POINT ( 'NONE',  ( 187.2565225563074023, 276.7898775566360996, -17.55325849615163492 ) ) ;
#8539=DIRECTION ( 'NONE',  ( 0.4999999999999992784, -0.8660254037844390407, 0.000000000000000000 ) ) ;
#8540=VERTEX_POINT ( 'NONE', #88336 ) ;
#8541=CARTESIAN_POINT ( 'NONE',  ( 175.2877164847554923, 252.7615608265838034, -0.2531314936308718955 ) ) ;
#8543=DIRECTION ( 'NONE',  ( 0.8660254037844395958, 0.4999999999999985567, 0.000000000000000000 ) ) ;
#8544=CARTESIAN_POINT ( 'NONE',  ( 194.9636675848471441, 292.9600174435121289, -15.57898232594655319 ) ) ;
#8545=DIRECTION ( 'NONE',  ( -0.4999999999999998890, 0.8660254037844385966, 0.000000000000000000 ) ) ;
#8554=ORIENTED_EDGE ( 'NONE', *, *, #83804, .F. ) ;
#8557=CARTESIAN_POINT ( 'NONE',  ( 194.5579492401075186, 286.5235815387566163, 17.58388259748475235 ) ) ;
#8558=ADVANCED_FACE ( 'NONE', ( #64981 ), #50263, .T. ) ;
#8559=ORIENTED_EDGE ( 'NONE', *, *, #6093, .F. ) ;
#8560=CARTESIAN_POINT ( 'NONE',  ( 174.6714692322213409, 286.2187378199596424, 10.51693356748920039 ) ) ;
#8561=CARTESIAN_POINT ( 'NONE',  ( 162.7259096899686313, 284.7569079919674095, -2.578525105315500721 ) ) ;
#8563=CARTESIAN_POINT ( 'NONE',  ( 163.3409975114459485, 247.7320886816312111, -10.96358124877083640 ) ) ;
#8564=CARTESIAN_POINT ( 'NONE',  ( 194.5051734451974426, 293.7541525883582381, 14.61790433731063921 ) ) ;
#8565=CARTESIAN_POINT ( 'NONE',  ( 185.4106159949853634, 292.5018125113814449, -10.86630696919762684 ) ) ;
#8566=CARTESIAN_POINT ( 'NONE',  ( 205.2414727015710412, 275.1583367910551488, -12.71338796362297963 ) ) ;
#8567=B_SPLINE_CURVE_WITH_KNOTS ( 'NONE', 3,
 ( #23163, #46457, #79425, #71295 ),
 .UNSPECIFIED., .F., .F.,
 ( 4, 4 ),
 ( 0.01134742446246735960, 0.01727584594350520253 ),
 .UNSPECIFIED. ) ;
#8568=CARTESIAN_POINT ( 'NONE',  ( 139.3076170325891212, 260.4244531367911577, -4.594050593750046652 ) ) ;
#8569=CARTESIAN_POINT ( 'NONE',  ( 206.3616846321097853, 270.5654860604214491, 2.445568098436429416 ) ) ;
#8570=AXIS2_PLACEMENT_3D ( 'NONE', #10162, #33454, #99504 ) ;
#8571=CARTESIAN_POINT ( 'NONE',  ( 195.3767056438044847, 291.5845065600011026, -15.69873944039788860 ) ) ;
#8572=CARTESIAN_POINT ( 'NONE',  ( 84.42325706775034178, 228.7369531367911293, -4.594050593750048428 ) ) ;
#8574=CARTESIAN_POINT ( 'NONE',  ( 191.4044787581200069, 299.1247133251352466, 7.435199718141230818 ) ) ;
#8576=ORIENTED_EDGE ( 'NONE', *, *, #29047, .F. ) ;
#8577=CARTESIAN_POINT ( 'NONE',  ( 195.5022618529877150, 292.0271448064274296, -15.80620227310758352 ) ) ;
#8582=CARTESIAN_POINT ( 'NONE',  ( 146.5310397537613483, 276.8477895910274356, -0.2793038414862049068 ) ) ;
#8585=DIRECTION ( 'NONE',  ( 0.4999999999999998890, -0.8660254037844385966, 0.000000000000000000 ) ) ;
#8586=CARTESIAN_POINT ( 'NONE',  ( 84.39645409570583467, 219.5333772461660544, 9.188101187500095079 ) ) ;
#8590=CARTESIAN_POINT ( 'NONE',  ( 161.4108037507797917, 251.0752823435572623, -14.11420789677157650 ) ) ;
#8594=CARTESIAN_POINT ( 'NONE',  ( 185.7838608033968910, 272.9513126759449051, -17.26505740043860726 ) ) ;
#8595=CARTESIAN_POINT ( 'NONE',  ( 207.4096351507161557, 270.9099127066079973, -1.362988047887532694 ) ) ;
#8598=CARTESIAN_POINT ( 'NONE',  ( 192.2355776333048425, 296.5101708762551311, 11.25704082661979477 ) ) ;
#8599=CARTESIAN_POINT ( 'NONE',  ( 185.7481537963866458, 259.5269681845950345, 5.863452686169032368 ) ) ;
#8600=CARTESIAN_POINT ( 'NONE',  ( 200.5039526449628795, 267.3497397166782434, 6.370409075474873006 ) ) ;
#8601=CARTESIAN_POINT ( 'NONE',  ( 200.7484899876179441, 282.9404111291507888, -16.88964748465601673 ) ) ;
#8605=CARTESIAN_POINT ( 'NONE',  ( 196.2017069210582747, 264.5352342889651709, 5.385840044374106128 ) ) ;
#8606=DIRECTION ( 'NONE',  ( 0.4999999999999998890, -0.8660254037844385966, 0.000000000000000000 ) ) ;
#8607=CARTESIAN_POINT ( 'NONE',  ( 29.67553675853319461, 176.3932355074535963, -2.679491924311248496 ) ) ;
#8608=CARTESIAN_POINT ( 'NONE',  ( 187.9832561701559541, 266.1096952060750596, -13.00726351221733346 ) ) ;
#8609=FACE_OUTER_BOUND ( 'NONE', #67362, .T. ) ;
#8610=CARTESIAN_POINT ( 'NONE',  ( 152.8019897319685185, 271.1875699278143088, 14.22014587818035380 ) ) ;
#8611=ORIENTED_EDGE ( 'NONE', *, *, #75542, .F. ) ;
#8612=DIRECTION ( 'NONE',  ( -0.8660254037844387076, -0.4999999999999998890, -0.000000000000000000 ) ) ;
#8613=CARTESIAN_POINT ( 'NONE',  ( 162.9796882977680639, 248.3578945969637743, 9.683801903336119565 ) ) ;
#8616=CARTESIAN_POINT ( 'NONE',  ( 178.5603549463671698, 264.9494309603151692, -15.99590783900550761 ) ) ;
#8621=CARTESIAN_POINT ( 'NONE',  ( 163.3828304853718407, 283.7865500842125925, -3.144285925872225107 ) ) ;
#8623=CARTESIAN_POINT ( 'NONE',  ( 188.7356621499138214, 259.9383745115107445, 3.760742190882747860 ) ) ;
#8624=CARTESIAN_POINT ( 'NONE',  ( 161.8807657183444064, 250.2612843381103573, -13.52770735624900311 ) ) ;
#8625=CARTESIAN_POINT ( 'NONE',  ( 0.9872088458345583684, 177.5024278399160949, 9.188101187500095079 ) ) ;
#8629=CARTESIAN_POINT ( 'NONE',  ( 160.2015549049794174, 253.9709619308573849, -15.20936558711751552 ) ) ;
#8631=DIRECTION ( 'NONE',  ( -0.8660254037844387076, -0.4999999999999998890, -0.000000000000000000 ) ) ;
#8632=CARTESIAN_POINT ( 'NONE',  ( 21.44705901024191519, 189.3149278399161233, 9.188101187500093303 ) ) ;
#8636=CARTESIAN_POINT ( 'NONE',  ( 173.4196987977404092, 273.2181934944644013, -16.51998383881567989 ) ) ;
#8637=CARTESIAN_POINT ( 'NONE',  ( 142.4134467818605572, 241.4824982072973967, 3.021315404115420679E-15 ) ) ;
#8639=CARTESIAN_POINT ( 'NONE',  ( 187.8983670083758000, 296.6038788229786292, -7.730668491481425875 ) ) ;
#8641=CARTESIAN_POINT ( 'NONE',  ( 65.47921168356340615, 218.6115022471903160, -5.000000000000047962 ) ) ;
#8642=CARTESIAN_POINT ( 'NONE',  ( 164.4633416896444658, 246.1841640495187846, 1.498163193773305091 ) ) ;
#8643=CARTESIAN_POINT ( 'NONE',  ( 203.4246719454474146, 270.0952167377922706, 6.029947592111899013 ) ) ;
#8644=CARTESIAN_POINT ( 'NONE',  ( 31.83936385565518279, 195.3149278399160664, 9.188101187500093303 ) ) ;
#8646=CARTESIAN_POINT ( 'NONE',  ( 135.9646106164503010, 237.7592609112380160, 2.679491924311254714 ) ) ;
#8647=CARTESIAN_POINT ( 'NONE',  ( 203.4080297268528170, 270.2650173722573186, -6.439894855938525176 ) ) ;
#8651=CARTESIAN_POINT ( 'NONE',  ( 161.0699900735471601, 279.2409086475570916, -9.794691631822578515 ) ) ;
#8654=CARTESIAN_POINT ( 'NONE',  ( 202.7041331321765938, 279.5531378413010657, 17.14708438049711248 ) ) ;
#8655=FACE_OUTER_BOUND ( 'NONE', #97014, .T. ) ;
#8656=CARTESIAN_POINT ( 'NONE',  ( 185.6236042504581008, 267.5736580584572266, -14.81396297063468026 ) ) ;
#8659=CARTESIAN_POINT ( 'NONE',  ( 196.8309065691697128, 264.2445955198643901, -3.407952846926960877 ) ) ;
#8663=CARTESIAN_POINT ( 'NONE',  ( 21.14953632379956616, 183.0177522451418497, -10.00000000000009592 ) ) ;
#8665=ADVANCED_FACE ( 'NONE', ( #66463 ), #75176, .F. ) ;
#8666=B_SPLINE_CURVE_WITH_KNOTS ( 'NONE', 3,
 ( #97704, #82027, #12092, #50573, #83019, #42954, #35377, #97221, #5485, #35875, #41982, #43469 ),
 .UNSPECIFIED., .F., .F.,
 ( 4, 2, 2, 2, 2, 4 ),
 ( 0.0009047221135296957921, 0.001170349639185115859, 0.001435977164840535926, 0.001967232216151415091, 0.002498487267462294256, 0.003029742318773173421 ),
 .UNSPECIFIED. ) ;
#8667=CARTESIAN_POINT ( 'NONE',  ( 191.0816511748900268, 299.6838671013740623, 7.311127128005925790 ) ) ;
#8668=CARTESIAN_POINT ( 'NONE',  ( 180.3265683508092820, 256.4805248161748636, -7.849693535446355064 ) ) ;
#8672=CARTESIAN_POINT ( 'NONE',  ( 189.3318025282030135, 274.0192145183515322, -15.65849137438579319 ) ) ;
#8675=CARTESIAN_POINT ( 'NONE',  ( 150.6655900823359389, 269.6865383554857090, 15.31288044136207205 ) ) ;
#8679=CARTESIAN_POINT ( 'NONE',  ( 190.2476911738421848, 301.1283281946692796, -1.360079143321618611 ) ) ;
#8680=EDGE_CURVE ( 'NONE', #2343, #53789, #71805, .T. ) ;
#8681=CARTESIAN_POINT ( 'NONE',  ( 180.3688922265450287, 287.0481539434517231, -13.70161974464981469 ) ) ;
#8684=CARTESIAN_POINT ( 'NONE',  ( 157.2333142128019858, 258.3109064714224132, 16.87956768598436597 ) ) ;
#8685=CARTESIAN_POINT ( 'NONE',  ( 159.5569985709834384, 265.8568429881750603, 16.74439774012073556 ) ) ;
#8688=CARTESIAN_POINT ( 'NONE',  ( 157.5331533759313913, 259.5764018409500409, 17.61237877605050173 ) ) ;
#8690=CARTESIAN_POINT ( 'NONE',  ( 52.46142023538962462, 213.3464784336661637, 1.353441290958777525E-15 ) ) ;
#8693=CARTESIAN_POINT ( 'NONE',  ( 159.9040744856012850, 255.4269131533854420, 16.38690128260775936 ) ) ;
#8695=CARTESIAN_POINT ( 'NONE',  ( 173.5145074140515362, 271.4604948858709008, 16.42671096914147810 ) ) ;
#8697=ORIENTED_EDGE ( 'NONE', *, *, #17582, .F. ) ;
#8700=CARTESIAN_POINT ( 'NONE',  ( 190.6218339396177441, 300.4802939150614520, -4.178005820806754755 ) ) ;
#8701=CARTESIAN_POINT ( 'NONE',  ( 190.5154909595809727, 300.6644853595138329, -0.04129855346138300298 ) ) ;
#8703=CARTESIAN_POINT ( 'NONE',  ( 174.6738009877982449, 260.4501079225292415, -14.90946296650636604 ) ) ;
#8704=CARTESIAN_POINT ( 'NONE',  ( 134.2560625007776025, 254.9865022471902876, -10.00000000000009592 ) ) ;
#8705=CARTESIAN_POINT ( 'NONE',  ( 161.8926315922002743, 250.2407320417157166, -13.77020595223768495 ) ) ;
#8706=CARTESIAN_POINT ( 'NONE',  ( 147.3379027498079381, 275.4502618871274535, -3.695260257281167249 ) ) ;
#8707=AXIS2_PLACEMENT_3D ( 'NONE', #35331, #66241, #36824 ) ;
#8708=CARTESIAN_POINT ( 'NONE',  ( 163.2951241624277827, 257.7631431858913515, 15.56583983124304638 ) ) ;
#8710=CARTESIAN_POINT ( 'NONE',  ( 164.2813349609167517, 246.1033764428878214, 1.949810150281061638 ) ) ;
#8714=CARTESIAN_POINT ( 'NONE',  ( 110.6480226958041158, 228.5643266524160708, 9.188101187500095079 ) ) ;
#8716=CARTESIAN_POINT ( 'NONE',  ( 191.5521510896938935, 298.8689373439769952, -9.847378829740700112 ) ) ;
#8719=CARTESIAN_POINT ( 'NONE',  ( 203.3041373168503299, 278.5139001086923827, -16.61929732091214973 ) ) ;
#8720=CARTESIAN_POINT ( 'NONE',  ( 183.2981546842155751, 284.6900415564330160, -14.97990253935919469 ) ) ;
#8722=CARTESIAN_POINT ( 'NONE',  ( 166.5497620933320775, 284.9599651698292178, -8.643830016708903941 ) ) ;
#8725=CARTESIAN_POINT ( 'NONE',  ( 182.2911844765873184, 260.6002554270507403, 9.501293399576107745 ) ) ;
#8727=CARTESIAN_POINT ( 'NONE',  ( 122.7720312530212396, 247.8149278399160949, 9.188101187500093303 ) ) ;
#8728=CARTESIAN_POINT ( 'NONE',  ( 198.8194531333411419, 286.2816009704309863, -17.01510935557533344 ) ) ;
#8729=CARTESIAN_POINT ( 'NONE',  ( 186.0371838319158542, 296.8243199225140643, 4.660811700844511130 ) ) ;
#8730=CARTESIAN_POINT ( 'NONE',  ( 187.3796900879174245, 281.3202307012271604, -17.28651300096462151 ) ) ;
#8732=CARTESIAN_POINT ( 'NONE',  ( 43.96371950863733247, 202.3149278399160949, -9.188101187500095079 ) ) ;
#8738=CARTESIAN_POINT ( 'NONE',  ( 47.97596991287763757, 210.0530062829863027, 1.101618078115930403E-13 ) ) ;
#8739=CARTESIAN_POINT ( 'NONE',  ( 175.0982648744423216, 261.2275428049201196, 15.10619652427497428 ) ) ;
#8741=EDGE_CURVE ( 'NONE', #55876, #74996, #43366, .T. ) ;
#8742=CARTESIAN_POINT ( 'NONE',  ( 154.8545429534089237, 262.4310591522755089, -17.81746354318405778 ) ) ;
#8743=CARTESIAN_POINT ( 'NONE',  ( 181.3882225691092742, 262.6214322978779592, 12.41810020290828120 ) ) ;
#8744=CARTESIAN_POINT ( 'NONE',  ( 119.9486011388743236, 233.3927522451417929, -10.00000000000009059 ) ) ;
#8745=CARTESIAN_POINT ( 'NONE',  ( 194.1125532102549300, 292.6514872621661993, -15.55923223616878204 ) ) ;
#8748=CARTESIAN_POINT ( 'NONE',  ( 162.7644741734472120, 248.7306563947940958, 9.865755277559742353 ) ) ;
#8750=CARTESIAN_POINT ( 'NONE',  ( 33.19304919271588972, 177.7202760586659736, -5.415160957724236172E-17 ) ) ;
#8753=CARTESIAN_POINT ( 'NONE',  ( 39.95181620016202118, 182.3262482093457209, 3.021315404115420679E-15 ) ) ;
#8755=CARTESIAN_POINT ( 'NONE',  ( 198.1679321590325458, 277.6257778925182720, -16.56331389466651061 ) ) ;
#8756=CARTESIAN_POINT ( 'NONE',  ( 65.42534541587671981, 199.3923013555409796, 4.594050593750050204 ) ) ;
#8758=CARTESIAN_POINT ( 'NONE',  ( 184.7849722178042668, 257.5454927209563607, 1.385182159486959774 ) ) ;
#8759=CARTESIAN_POINT ( 'NONE',  ( 157.8429099974857195, 257.2550556002704525, -17.85752049034686095 ) ) ;
#8764=CARTESIAN_POINT ( 'NONE',  ( 163.7828826429516766, 268.2613608475996898, 16.53282274799222407 ) ) ;
#8765=CARTESIAN_POINT ( 'NONE',  ( 16.54877636974260824, 190.3615022471903160, 5.000000000000046185 ) ) ;
#8767=CARTESIAN_POINT ( 'NONE',  ( 164.4817765375028102, 245.7562014482918755, -6.334578229142199035 ) ) ;
#8768=CARTESIAN_POINT ( 'NONE',  ( -9.729855525997876953, 171.3149278399160664, 9.188101187500093303 ) ) ;
#8770=CARTESIAN_POINT ( 'NONE',  ( 166.1729740367198644, 261.7477518458006216, -16.21765485240585747 ) ) ;
#8771=CARTESIAN_POINT ( 'NONE',  ( 169.8916322304794733, 263.4028382525763732, 15.84815012191193695 ) ) ;
#8772=CARTESIAN_POINT ( 'NONE',  ( 185.7044324113292646, 259.6182011128160525, 7.428341809090757586 ) ) ;
#8773=CARTESIAN_POINT ( 'NONE',  ( 194.5253693406981483, 291.7191722712467481, 16.18900132190417551 ) ) ;
#8774=CARTESIAN_POINT ( 'NONE',  ( 186.2106335195739462, 257.9955712153812328, -2.495042034395281938 ) ) ;
#8777=CARTESIAN_POINT ( 'NONE',  ( 150.2345823034905550, 271.5449826357299230, -12.44854083486978347 ) ) ;
#8778=CARTESIAN_POINT ( 'NONE',  ( 177.9669014565158704, 286.2669617536872124, 13.02687325745571378 ) ) ;
#8781=CYLINDRICAL_SURFACE ( 'NONE', #66756, 17.82106496071139645 ) ;
#8784=CARTESIAN_POINT ( 'NONE',  ( 152.6845319923753834, 266.1896283897672220, 17.20844521882669653 ) ) ;
#8786=B_SPLINE_CURVE_WITH_KNOTS ( 'NONE', 3,
 ( #85864, #84832, #62467, #53870 ),
 .UNSPECIFIED., .F., .F.,
 ( 4, 4 ),
 ( 0.004989422848796198559, 0.009972366782226169124 ),
 .UNSPECIFIED. ) ;
#8787=CARTESIAN_POINT ( 'NONE',  ( 136.0806360202347491, 237.8262482093457493, 3.021315404115420679E-15 ) ) ;
#8788=CARTESIAN_POINT ( 'NONE',  ( 163.4222916751007801, 247.5912830598222172, -10.52132777929285012 ) ) ;
#8790=VERTEX_POINT ( 'NONE', #61045 ) ;
#8792=CARTESIAN_POINT ( 'NONE',  ( 155.8093079659346074, 277.0108043004451588, -10.30466594370042621 ) ) ;
#8796=CARTESIAN_POINT ( 'NONE',  ( 155.5450984722979229, 262.5874973419817024, -17.41340391108767705 ) ) ;
#8797=VERTEX_POINT ( 'NONE', #28175 ) ;
#8798=CARTESIAN_POINT ( 'NONE',  ( 191.0604813119340690, 299.7205343796033503, -9.270812881586136811 ) ) ;
#8800=CARTESIAN_POINT ( 'NONE',  ( -22.42236680055709641, 157.8615022471902591, 0.000000000000000000 ) ) ;
#8803=VERTEX_POINT ( 'NONE', #36762 ) ;
#8804=CARTESIAN_POINT ( 'NONE',  ( 155.6413935076475639, 261.0681940143705901, 18.42569256965892421 ) ) ;
#8805=CARTESIAN_POINT ( 'NONE',  ( 191.4044787581200069, 299.1247133251352466, 7.435199718141230818 ) ) ;
#8811=ORIENTED_EDGE ( 'NONE', *, *, #60241, .T. ) ;
#8812=CARTESIAN_POINT ( 'NONE',  ( 160.5893190321802138, 270.9897182155185078, 16.60663562724527864 ) ) ;
#8814=CARTESIAN_POINT ( 'NONE',  ( 164.4817765375028102, 245.7562014482918755, -6.334578229142199035 ) ) ;
#8816=FACE_OUTER_BOUND ( 'NONE', #63321, .T. ) ;
#8817=CARTESIAN_POINT ( 'NONE',  ( 148.4042165687623083, 273.6033521758856750, -8.709765892313745539 ) ) ;
#8818=B_SPLINE_CURVE_WITH_KNOTS ( 'NONE', 3,
 ( #37812, #91077, #76824, #46409 ),
 .UNSPECIFIED., .F., .F.,
 ( 4, 4 ),
 ( 0.01052722645609634883, 0.01597497186318108664 ),
 .UNSPECIFIED. ) ;
#8820=CARTESIAN_POINT ( 'NONE',  ( 159.1177508122425195, 255.0469665375489399, -17.04660126523272012 ) ) ;
#8821=CARTESIAN_POINT ( 'NONE',  ( 166.6156759393427080, 247.0710755757112054, 1.913997305269410587 ) ) ;
#8823=CARTESIAN_POINT ( 'NONE',  ( 193.6780271845242964, 277.9462545196296333, -17.36184529900156548 ) ) ;
#8824=CARTESIAN_POINT ( 'NONE',  ( 164.9103019330012216, 245.0139736909548560, 2.841678961959298810 ) ) ;
#8825=CARTESIAN_POINT ( 'NONE',  ( 206.9919585703311213, 271.2130891193729099, 4.989103036379466616 ) ) ;
#8827=CARTESIAN_POINT ( 'NONE',  ( 147.4517449145323269, 275.2530814737808669, -3.583987543978726986 ) ) ;
#8828=CARTESIAN_POINT ( 'NONE',  ( 155.5798705649511930, 269.2207634517940278, 16.19704775669435648 ) ) ;
#8829=CARTESIAN_POINT ( 'NONE',  ( 206.3454060440500086, 273.2462681537123785, -9.268083217908118954 ) ) ;
#8833=CARTESIAN_POINT ( 'NONE',  ( 161.7101619467568980, 250.5567787384628389, 13.05644392949610655 ) ) ;
#8834=CARTESIAN_POINT ( 'NONE',  ( 104.8833675557553704, 241.3615022471903160, 5.000000000000046185 ) ) ;
#8836=CARTESIAN_POINT ( 'NONE',  ( 155.1935823099396430, 261.8438257609990956, -17.10498131462595595 ) ) ;
#8837=CYLINDRICAL_SURFACE ( 'NONE', #96566, 10.00000000000010658 ) ;
#8838=CARTESIAN_POINT ( 'NONE',  ( 177.4096984176076148, 293.8085471629082122, -0.6315254070814751985 ) ) ;
#8839=CARTESIAN_POINT ( 'NONE',  ( 17.75760349231054391, 174.3927522451418213, 10.00000000000009592 ) ) ;
#8840=CARTESIAN_POINT ( 'NONE',  ( 85.88519558028406209, 211.2048013555409796, 4.594050593750051981 ) ) ;
#8844=CARTESIAN_POINT ( 'NONE',  ( 167.0053736619712765, 278.0716144694669083, -13.57399711851867785 ) ) ;
#8845=CARTESIAN_POINT ( 'NONE',  ( 10.02652254571713719, 176.5958772461660544, -9.188101187500095079 ) ) ;
#8848=CARTESIAN_POINT ( 'NONE',  ( 200.6097954076514895, 283.1806371883870383, 16.82611162221071766 ) ) ;
#8853=CARTESIAN_POINT ( 'NONE',  ( 197.5308359676227212, 265.1308937032743529, -2.955964573451065558 ) ) ;
#8857=CARTESIAN_POINT ( 'NONE',  ( 42.09652578138363310, 185.1115022471902023, -5.000000000000041744 ) ) ;
#8860=CARTESIAN_POINT ( 'NONE',  ( 26.48065812185646806, 198.3464784336661637, 1.353441290958777525E-15 ) ) ;
#8861=CARTESIAN_POINT ( 'NONE',  ( 196.4397788971523653, 275.7035216443041463, 15.37058611766792993 ) ) ;
#8864=CARTESIAN_POINT ( 'NONE',  ( 150.0678585083896905, 271.7085566807550663, -11.68900650907589522 ) ) ;
#8865=CARTESIAN_POINT ( 'NONE',  ( 182.6207078668202257, 260.7553341194429208, -10.79722308874143266 ) ) ;
#8867=FACE_OUTER_BOUND ( 'NONE', #57270, .T. ) ;
#8869=CARTESIAN_POINT ( 'NONE',  ( 194.3799873100184641, 293.9709813348915191, 15.33105633561973669 ) ) ;
#8870=CARTESIAN_POINT ( 'NONE',  ( 186.7967035978091133, 279.0542505165097396, -17.82519856243605005 ) ) ;
#8872=CARTESIAN_POINT ( 'NONE',  ( 194.6782745185928434, 293.4543327343926080, -14.56555309295305634 ) ) ;
#8873=EDGE_CURVE ( 'NONE', #48040, #28763, #75049, .T. ) ;
#8874=CARTESIAN_POINT ( 'NONE',  ( 204.3371846825755824, 276.7246095846310823, 14.72513001683937262 ) ) ;
#8877=CARTESIAN_POINT ( 'NONE',  ( 147.7157269441172218, 274.7958511862549926, 8.036290321896261801 ) ) ;
#8882=CARTESIAN_POINT ( 'NONE',  ( 139.5243837071329267, 251.3615022471902307, -10.00000000000009592 ) ) ;
#8883=CARTESIAN_POINT ( 'NONE',  ( 104.4229444624559733, 243.3464784336661353, 1.353441290958777327E-15 ) ) ;
#8887=CARTESIAN_POINT ( 'NONE',  ( 188.6826127332440421, 272.6057162039079458, 16.71479996418005243 ) ) ;
#8888=CARTESIAN_POINT ( 'NONE',  ( 192.1943038168404314, 277.1473907896511264, 17.36549850453357635 ) ) ;
#8889=CARTESIAN_POINT ( 'NONE',  ( 150.9989172662526471, 269.1091987373977190, -14.13682882617413306 ) ) ;
#8890=CARTESIAN_POINT ( 'NONE',  ( 192.4717705703029651, 263.5766868200552722, -4.344887308562926265 ) ) ;
#8891=CARTESIAN_POINT ( 'NONE',  ( 149.9258927270312824, 271.7122074278049695, -11.62661048439495382 ) ) ;
#8892=CARTESIAN_POINT ( 'NONE',  ( 115.5463053363034476, 227.5177522451418213, 5.000000000000051514 ) ) ;
#8895=VERTEX_POINT ( 'NONE', #55931 ) ;
#8897=DIRECTION ( 'NONE',  ( 0.5000000000000048850, -0.8660254037844358210, 0.000000000000000000 ) ) ;
#8898=CARTESIAN_POINT ( 'NONE',  ( 199.9473046934823230, 270.1330773050400467, 9.225012586806066395 ) ) ;
#8899=EDGE_CURVE ( 'NONE', #43165, #59283, #61412, .T. ) ;
#8900=EDGE_LOOP ( 'NONE', ( #11588, #42042, #57015 ) ) ;
#8904=CARTESIAN_POINT ( 'NONE',  ( 181.7171926400567656, 295.8235151057616008, -3.827279785929341038 ) ) ;
#8905=CARTESIAN_POINT ( 'NONE',  ( 168.7096392155106344, 280.2107777274362093, -14.47775774749160682 ) ) ;
#8906=EDGE_CURVE ( 'NONE', #90508, #24776, #39301, .T. ) ;
#8907=VERTEX_POINT ( 'NONE', #55433 ) ;
#8912=CARTESIAN_POINT ( 'NONE',  ( 171.3171204526115616, 271.4791138034659070, -17.75561031716327420 ) ) ;
#8913=FACE_OUTER_BOUND ( 'NONE', #3938, .T. ) ;
#8914=AXIS2_PLACEMENT_3D ( 'NONE', #13755, #45148, #12789 ) ;
#8917=EDGE_CURVE ( 'NONE', #441, #5671, #86582, .T. ) ;
#8918=CARTESIAN_POINT ( 'NONE',  ( 168.4809247738020019, 252.9187805847961670, 12.05003015331094041 ) ) ;
#8919=CARTESIAN_POINT ( 'NONE',  ( 61.85273030166814578, 216.5177522451419065, 5.000000000000046185 ) ) ;
#8922=FACE_OUTER_BOUND ( 'NONE', #46045, .T. ) ;
#8924=CARTESIAN_POINT ( 'NONE',  ( 155.2922060645262263, 261.6730044072216401, -16.98884022075611355 ) ) ;
#8926=ORIENTED_EDGE ( 'NONE', *, *, #90160, .T. ) ;
#8927=EDGE_CURVE ( 'NONE', #85762, #46298, #33659, .T. ) ;
#8928=EDGE_LOOP ( 'NONE', ( #2060, #63248, #100266, #19855 ) ) ;
#8937=CARTESIAN_POINT ( 'NONE',  ( 206.0013442967545245, 273.8422005809691768, -10.96701481760672792 ) ) ;
#8938=CARTESIAN_POINT ( 'NONE',  ( 147.8220999374534586, 274.6116077572435188, -7.200782152036906858 ) ) ;
#8941=CARTESIAN_POINT ( 'NONE',  ( 171.5081661771196195, 250.9258183615457085, -5.630105313893144725 ) ) ;
#8942=CARTESIAN_POINT ( 'NONE',  ( 24.36335893204212155, 173.3262482093457777, 3.021315404115420679E-15 ) ) ;
#8943=CARTESIAN_POINT ( 'NONE',  ( 163.1953264782998758, 283.8895661455310915, -7.125257539458086598 ) ) ;
#8944=CARTESIAN_POINT ( 'NONE',  ( 131.1078728602114722, 240.3768266524160424, 9.188101187500098632 ) ) ;
#8945=CARTESIAN_POINT ( 'NONE',  ( 186.2596960937134156, 262.5193429868782005, -9.036614942780335724 ) ) ;
#8951=CARTESIAN_POINT ( 'NONE',  ( 201.2017102119751826, 274.7757513898055777, 13.37679397288412453 ) ) ;
#8952=CARTESIAN_POINT ( 'NONE',  ( 180.0144465046176663, 255.7853420670775506, 1.312520848803033324 ) ) ;
#8954=CARTESIAN_POINT ( 'NONE',  ( 146.8211202654633496, 276.3453554064738569, 4.006087063231699830 ) ) ;
#8956=CARTESIAN_POINT ( 'NONE',  ( 163.7584496161371419, 249.5830917119055243, 11.44878023424904256 ) ) ;
#8957=CARTESIAN_POINT ( 'NONE',  ( 173.6149320458357295, 287.7500054338993891, -9.932635149992773194 ) ) ;
#8961=CARTESIAN_POINT ( 'NONE',  ( 147.8819534105757043, 274.5079385007862811, -9.338341377131436971 ) ) ;
#8962=CARTESIAN_POINT ( 'NONE',  ( 152.6809499003229860, 273.9044486092186048, 12.24870461040242553 ) ) ;
#8963=ORIENTED_EDGE ( 'NONE', *, *, #3828, .F. ) ;
#8964=CARTESIAN_POINT ( 'NONE',  ( 188.7303249615299592, 266.5716613699773347, -11.84797561876724181 ) ) ;
#8965=CARTESIAN_POINT ( 'NONE',  ( 160.2698612238776263, 279.1124238657968135, 10.65817527884720306 ) ) ;
#8966=CARTESIAN_POINT ( 'NONE',  ( 152.1679110164900237, 267.0844421682562029, -17.00361552756096728 ) ) ;
#8969=CARTESIAN_POINT ( 'NONE',  ( 153.0404527213268864, 270.0709234468621389, 14.04439096357963379 ) ) ;
#8970=CARTESIAN_POINT ( 'NONE',  ( 151.5490211047388414, 275.0384667395342149, -8.636128745347312119 ) ) ;
#8971=CARTESIAN_POINT ( 'NONE',  ( 201.1060504099706350, 282.3210983108598384, -18.18000168485860257 ) ) ;
#8973=CARTESIAN_POINT ( 'NONE',  ( 190.2287563641723978, 301.1611242470490311, -4.521471513871881953 ) ) ;
#8974=CARTESIAN_POINT ( 'NONE',  ( 164.5084652402306347, 247.3538846981742267, -7.514466451347210807 ) ) ;
#8975=CARTESIAN_POINT ( 'NONE',  ( 189.9462279001383536, 274.3542461691521339, -15.66465755634487422 ) ) ;
#8981=CARTESIAN_POINT ( 'NONE',  ( 155.4812142336614329, 261.3456326552338282, 18.45193178807985745 ) ) ;
#8983=CARTESIAN_POINT ( 'NONE',  ( -7.997457622663985966, 160.0643266524160140, -9.188101187500093303 ) ) ;
#8984=CARTESIAN_POINT ( 'NONE',  ( 95.76303752037657091, 226.0958772461660260, -9.188101187500095079 ) ) ;
#8986=CARTESIAN_POINT ( 'NONE',  ( 192.5143468344189728, 297.2023654272867361, -12.06830393602581530 ) ) ;
#8989=CARTESIAN_POINT ( 'NONE',  ( 202.8549823380854491, 279.2918593523859272, -16.39745931995414807 ) ) ;
#8990=CYLINDRICAL_SURFACE ( 'NONE', #65243, 10.00000000000010658 ) ;
#8995=CARTESIAN_POINT ( 'NONE',  ( 161.8938357633344651, 250.2386463561303458, 14.09469623995626719 ) ) ;
#8996=EDGE_CURVE ( 'NONE', #5449, #7185, #96377, .T. ) ;
#8997=CARTESIAN_POINT ( 'NONE',  ( 166.1003953386458249, 249.2057617637232738, -9.336859914837196683 ) ) ;
#8998=CARTESIAN_POINT ( 'NONE',  ( 204.8391661702352735, 275.8551521435456380, -13.37474513291600431 ) ) ;
#8999=CARTESIAN_POINT ( 'NONE',  ( 157.1606030646430554, 258.4368458743103361, 17.96998724893680688 ) ) ;
#9000=B_SPLINE_CURVE_WITH_KNOTS ( 'NONE', 3,
 ( #74437, #81065, #73423, #19729 ),
 .UNSPECIFIED., .F., .F.,
 ( 4, 4 ),
 ( 0.03993246080742687137, 0.04837343171532907521 ),
 .UNSPECIFIED. ) ;
#9001=CARTESIAN_POINT ( 'NONE',  ( 169.4078252042709778, 250.4262823970964007, 8.341134405704034194 ) ) ;
#9003=CARTESIAN_POINT ( 'NONE',  ( 32.78649236710315762, 198.9244531367911293, -4.594050593750046652 ) ) ;
#9004=CARTESIAN_POINT ( 'NONE',  ( 59.20026718252854891, 214.1744531367911293, 4.594050593750047540 ) ) ;
#9005=CARTESIAN_POINT ( 'NONE',  ( 65.93257831369518840, 197.3262482093457777, 3.021315404115420679E-15 ) ) ;
#9006=B_SPLINE_CURVE_WITH_KNOTS ( 'NONE', 3,
 ( #30977, #84235, #45666, #76590, #7175, #30485, #38062, #13316, #44177, #22877, #84724, #46159, #77080, #7684, #38574, #94, #8685, #62874, #39554, #63882, #8189, #2603, #85226, #56270, #25382, #70478, #40566, #87267, #79631, #584, #31469, #40062, #79129, #55259, #46678, #93831, #1092, #61864, #93317, #62360, #54255, #71004, #24386, #86241, #78094, #23871 ),
 .UNSPECIFIED., .F., .F.,
 ( 4, 2, 2, 2, 2, 2, 2, 2, 2, 2, 2, 2, 2, 2, 2, 2, 2, 2, 2, 2, 2, 2, 4 ),
 ( 0.0008836965591771303846, 0.001081134423596614253, 0.001179853355806375053, 0.001278572288016136069, 0.001476010152435624492, 0.001673448016855112915, 0.002068323745694089326, 0.002463199474533066605, 0.003252950932210945702, 0.004042702389888824799, 0.004832453847566703896, 0.005227329576405679440, 0.005424767440825208412, 0.005523486373034932999, 0.005572845839139830421, 0.005622205305244727842, 0.005671564771349624397, 0.005720924237454521818, 0.005819643169664226456, 0.006017081034083765836, 0.006411956762922983374, 0.006806832491762201780, 0.007201708220601420185 ),
 .UNSPECIFIED. ) ;
#9008=CARTESIAN_POINT ( 'NONE',  ( 98.74902094561561228, 234.4865022471903160, 10.00000000000009415 ) ) ;
#9011=CARTESIAN_POINT ( 'NONE',  ( 196.5129603538013612, 268.9685797610468398, -10.52983625242027976 ) ) ;
#9014=CARTESIAN_POINT ( 'NONE',  ( 150.9115585710837877, 269.2605084359132093, -15.80434701481532578 ) ) ;
#9015=CARTESIAN_POINT ( 'NONE',  ( 196.2421909983451940, 290.7455499326673021, -17.31908925000307065 ) ) ;
#9017=CARTESIAN_POINT ( 'NONE',  ( 66.23672358827711548, 218.2369531367911293, -4.594050593750048428 ) ) ;
#9019=CARTESIAN_POINT ( 'NONE',  ( 155.0453531195792038, 262.1005662498678817, -18.46987289964740953 ) ) ;
#9020=CARTESIAN_POINT ( 'NONE',  ( 198.6755293322981117, 286.5308843062557571, 17.86676876308990103 ) ) ;
#9022=CARTESIAN_POINT ( 'NONE',  ( 153.9009929122451013, 264.0826562711307020, 18.02690668714909705 ) ) ;
#9026=CARTESIAN_POINT ( 'NONE',  ( 113.4714528099511455, 222.9865022471901455, 1.119607411625061291E-15 ) ) ;
#9027=CARTESIAN_POINT ( 'NONE',  ( 161.6256441450323678, 250.7031678651938762, 14.48526717260977037 ) ) ;
#9029=CARTESIAN_POINT ( 'NONE',  ( 206.9878665138179770, 272.1334939782196329, 6.566295309274049252 ) ) ;
#9030=ORIENTED_EDGE ( 'NONE', *, *, #9370, .F. ) ;
#9032=CARTESIAN_POINT ( 'NONE',  ( 188.0748052926907405, 273.3533922738282058, 15.64113677151411608 ) ) ;
#9034=CARTESIAN_POINT ( 'NONE',  ( 206.8659638600981623, 272.3446355680395641, -10.26115277030573125 ) ) ;
#9035=CARTESIAN_POINT ( 'NONE',  ( 194.0754204476036762, 293.3896858871647169, 14.78846558403258094 ) ) ;
#9042=EDGE_CURVE ( 'NONE', #44048, #47944, #16362, .T. ) ;
#9043=CARTESIAN_POINT ( 'NONE',  ( 167.4088369852190681, 247.5279131301515179, 3.600464852340231836 ) ) ;
#9044=CARTESIAN_POINT ( 'NONE',  ( 148.6594212568597868, 273.7599597785030596, 8.554715638618541007 ) ) ;
#9052=EDGE_CURVE ( 'NONE', #56021, #57780, #34489, .T. ) ;
#9053=EDGE_LOOP ( 'NONE', ( #21732, #49167 ) ) ;
#9054=CARTESIAN_POINT ( 'NONE',  ( 166.9369206129118197, 276.4285397603561591, 15.88976881163156563 ) ) ;
#9055=CARTESIAN_POINT ( 'NONE',  ( -0.5967702463563150372, 158.9155109091896350, 2.679491924311254714 ) ) ;
#9057=CARTESIAN_POINT ( 'NONE',  ( 170.8439975286642607, 284.8586297143663728, 11.08717077125447936 ) ) ;
#9058=( BOUNDED_CURVE ( )  B_SPLINE_CURVE ( 1, ( #72214, #32686 ),
 .UNSPECIFIED., .F., .F. ) 
 B_SPLINE_CURVE_WITH_KNOTS ( ( 2, 2 ),
 ( 0.000000000000000000, 0.001312499995903266495 ),
 .UNSPECIFIED. ) 
 CURVE ( )  GEOMETRIC_REPRESENTATION_ITEM ( )  RATIONAL_B_SPLINE_CURVE ( ( 0.9368410486966849415, 0.9368410486966849415 ) ) 
 REPRESENTATION_ITEM ( '' )  );
#9059=CARTESIAN_POINT ( 'NONE',  ( 163.2652593887152364, 283.8092165855917983, -2.903001196033301312 ) ) ;
#9062=CARTESIAN_POINT ( 'NONE',  ( 194.3799873100184641, 293.9709813348915191, 15.33105633561973669 ) ) ;
#9063=CARTESIAN_POINT ( 'NONE',  ( 185.6579485543611270, 292.7763231470134428, -10.71670576288961207 ) ) ;
#9064=CARTESIAN_POINT ( 'NONE',  ( 157.4893260420801653, 257.8674809757739013, -18.30842125257398223 ) ) ;
#9065=CARTESIAN_POINT ( 'NONE',  ( 164.7389676833716976, 245.3107333163898716, 5.284562706098457241 ) ) ;
#9066=CARTESIAN_POINT ( 'NONE',  ( 203.4636416406178512, 268.6914787556956981, 2.471263131328804707 ) ) ;
#9068=CARTESIAN_POINT ( 'NONE',  ( 93.16496130902324069, 224.5958772461660260, -9.188101187500095079 ) ) ;
#9069=B_SPLINE_CURVE_WITH_KNOTS ( 'NONE', 3,
 ( #23829, #32446, #2053, #70438 ),
 .UNSPECIFIED., .F., .F.,
 ( 4, 4 ),
 ( 0.01705236508060226780, 0.02596178682224619186 ),
 .UNSPECIFIED. ) ;
#9071=CARTESIAN_POINT ( 'NONE',  ( 150.8757650385446993, 269.3225046528533539, 14.31332712971473953 ) ) ;
#9075=CARTESIAN_POINT ( 'NONE',  ( 157.0759360137626572, 258.5834935081620642, -16.84194680719508597 ) ) ;
#9082=CARTESIAN_POINT ( 'NONE',  ( 207.8040920112677270, 270.7197499462034784, 3.100718407159808176 ) ) ;
#9083=CARTESIAN_POINT ( 'NONE',  ( 82.14994038281616895, 227.4244531367911293, -4.594050593750046652 ) ) ;
#9086=CARTESIAN_POINT ( 'NONE',  ( 161.8723090575478807, 250.2759317042724376, -14.13132104777860221 ) ) ;
#9087=ORIENTED_EDGE ( 'NONE', *, *, #4586, .T. ) ;
#9090=VECTOR ( 'NONE', #73908, 1000.000000000000000 ) ;
#9092=CARTESIAN_POINT ( 'NONE',  ( 183.2572639141025093, 259.6883485553630635, -10.14808137897176898 ) ) ;
#9094=EDGE_LOOP ( 'NONE', ( #70749, #65524, #19674, #15290 ) ) ;
#9098=CARTESIAN_POINT ( 'NONE',  ( 147.8132215089878798, 275.1406199707106452, -4.592798751325347872 ) ) ;
#9099=CARTESIAN_POINT ( 'NONE',  ( 175.5358861210679322, 284.6783754363922867, 14.06838304944039564 ) ) ;
#9101=FACE_OUTER_BOUND ( 'NONE', #30344, .T. ) ;
#9103=ORIENTED_EDGE ( 'NONE', *, *, #37140, .T. ) ;
#9105=CARTESIAN_POINT ( 'NONE',  ( 200.9111546617170916, 282.6586676490145464, 17.66063511622358106 ) ) ;
#9107=CARTESIAN_POINT ( 'NONE',  ( 171.4520973777158304, 251.1120003641540848, 7.352569034034808659 ) ) ;
#9108=CARTESIAN_POINT ( 'NONE',  ( 198.5250552234815018, 266.2012769527108276, 1.136986010074936937 ) ) ;
#9109=CARTESIAN_POINT ( 'NONE',  ( 156.9036059482025678, 272.7077526247311425, 14.56380410095424871 ) ) ;
#9111=EDGE_CURVE ( 'NONE', #483, #84750, #35752, .T. ) ;
#9112=CARTESIAN_POINT ( 'NONE',  ( 202.8499463704053198, 279.3005819042728604, 17.04674939340617001 ) ) ;
#9114=CARTESIAN_POINT ( 'NONE',  ( 207.6209998424140792, 271.0368748851258260, 6.610167240481342965 ) ) ;
#9119=CARTESIAN_POINT ( 'NONE',  ( 172.1288327371077003, 274.9361716132315792, 16.40855730066342133 ) ) ;
#9120=CARTESIAN_POINT ( 'NONE',  ( 166.5660939988957239, 286.4811537094821006, -3.256692973398967794 ) ) ;
#9125=CARTESIAN_POINT ( 'NONE',  ( 161.6755750489535046, 250.6166850027345276, -13.01404233079112061 ) ) ;
#9126=EDGE_CURVE ( 'NONE', #90599, #80986, #72009, .T. ) ;
#9127=CARTESIAN_POINT ( 'NONE',  ( 5.669592554750444435, 164.8923013555410080, 4.594050593750050204 ) ) ;
#9130=CARTESIAN_POINT ( 'NONE',  ( 160.4993420583414263, 253.2460122621210132, -14.64862292197809879 ) ) ;
#9131=FACE_BOUND ( 'NONE', #61972, .T. ) ;
#9133=CARTESIAN_POINT ( 'NONE',  ( 25.07406103223677007, 173.0327760586659736, 1.948934522072302763E-15 ) ) ;
#9134=CARTESIAN_POINT ( 'NONE',  ( 181.7815785431583038, 276.1505370498239813, -17.81783396216490445 ) ) ;
#9137=CARTESIAN_POINT ( 'NONE',  ( 146.6647111637776106, 276.6162639173599587, -0.6373001129109082674 ) ) ;
#9139=CARTESIAN_POINT ( 'NONE',  ( 167.8099530253072089, 271.3928698661641761, -17.53051755021046532 ) ) ;
#9140=CARTESIAN_POINT ( 'NONE',  ( 189.4796331244937164, 297.8479079567700296, -7.877982910326568167 ) ) ;
#9141=CARTESIAN_POINT ( 'NONE',  ( 189.2845499996045930, 259.5340837477176024, -0.8149847707460528001 ) ) ;
#9142=CARTESIAN_POINT ( 'NONE',  ( 58.11799575139567509, 214.3615022471903160, 5.000000000000046185 ) ) ;
#9145=EDGE_CURVE ( 'NONE', #86118, #1456, #9663, .T. ) ;
#9146=CARTESIAN_POINT ( 'NONE',  ( 172.0630936339023265, 254.4764114392720273, 11.54978638049990103 ) ) ;
#9147=CARTESIAN_POINT ( 'NONE',  ( 30.27021345494340565, 176.0327760586659736, 1.948934522072303157E-15 ) ) ;
#9149=CARTESIAN_POINT ( 'NONE',  ( 203.3700558458376122, 269.3551942510547406, -5.938188790449932419 ) ) ;
#9150=CARTESIAN_POINT ( 'NONE',  ( 151.2964716097791325, 268.5938194963972592, -15.66250187539618111 ) ) ;
#9151=CARTESIAN_POINT ( 'NONE',  ( 198.2505066714982149, 285.2670451491296149, 0.000000000000000000 ) ) ;
#9153=CARTESIAN_POINT ( 'NONE',  ( 168.0910689791846266, 281.7684205924134062, -11.46037133588631818 ) ) ;
#9154=CARTESIAN_POINT ( 'NONE',  ( 163.0740133991062351, 281.1655447304752897, -10.28074664187252196 ) ) ;
#9155=DIRECTION ( 'NONE',  ( -0.8660254037844387076, -0.4999999999999998890, -0.000000000000000000 ) ) ;
#9157=CARTESIAN_POINT ( 'NONE',  ( 202.4017613376760494, 280.0768611521521620, 15.73960524502980540 ) ) ;
#9158=CARTESIAN_POINT ( 'NONE',  ( 196.7130436017243653, 289.9300093007386749, -16.33278734947153765 ) ) ;
#9159=CARTESIAN_POINT ( 'NONE',  ( 186.5747885479362935, 268.5526011410998990, -14.20271085587731541 ) ) ;
#9167=ORIENTED_EDGE ( 'NONE', *, *, #2150, .F. ) ;
#9168=CARTESIAN_POINT ( 'NONE',  ( 23.81978131880161698, 177.8927522451418213, -10.00000000000009237 ) ) ;
#9170=CARTESIAN_POINT ( 'NONE',  ( 190.8604783348975502, 300.0669496974951471, 7.597731640149610222 ) ) ;
#9171=CARTESIAN_POINT ( 'NONE',  ( 168.7096392155106344, 280.2107777274362093, -14.47775774749160682 ) ) ;
#9177=ORIENTED_EDGE ( 'NONE', *, *, #72191, .T. ) ;
#9182=CARTESIAN_POINT ( 'NONE',  ( 147.6947327179224487, 274.8322142526899370, 9.090449717876689206 ) ) ;
#9184=CARTESIAN_POINT ( 'NONE',  ( 183.6532122277409655, 289.8064359948238007, -13.38300012774528369 ) ) ;
#9190=CARTESIAN_POINT ( 'NONE',  ( 198.2489255580726422, 287.2697837179150042, 18.53597557040773225 ) ) ;
#9192=CARTESIAN_POINT ( 'NONE',  ( 50.97302584657637681, 209.4244531367911577, -4.594050593750046652 ) ) ;
#9195=CARTESIAN_POINT ( 'NONE',  ( 197.9679655381963244, 287.7564207472362341, 17.61949439995294497 ) ) ;
#9196=CARTESIAN_POINT ( 'NONE',  ( 205.0859877718122561, 268.9368413191317586, -3.038556538008958974 ) ) ;
#9202=CARTESIAN_POINT ( 'NONE',  ( 190.3625087333586521, 300.9294583479858147, -4.271886578030237303 ) ) ;
#9205=CARTESIAN_POINT ( 'NONE',  ( 175.4707219612219831, 261.2647045857924581, -14.43885454850885708 ) ) ;
#9206=CARTESIAN_POINT ( 'NONE',  ( 139.5965524907817041, 244.7365022471901739, -10.00000000000009237 ) ) ;
#9207=CARTESIAN_POINT ( 'NONE',  ( 161.6755750489535046, 250.6166850027345276, -13.01404233079112061 ) ) ;
#9208=CARTESIAN_POINT ( 'NONE',  ( 147.1125781744767949, 275.8405354997948962, -5.216646253929903665 ) ) ;
#9209=CARTESIAN_POINT ( 'NONE',  ( 190.8187029736043883, 300.1393067457597681, 3.941064102378585954 ) ) ;
#9210=CARTESIAN_POINT ( 'NONE',  ( 177.6686998861319466, 269.6967534512956490, 16.10014392654021265 ) ) ;
#9211=CARTESIAN_POINT ( 'NONE',  ( 205.8030308266901898, 274.1856895869457844, 10.55961490432110317 ) ) ;
#9213=CARTESIAN_POINT ( 'NONE',  ( 154.8376827341003548, 264.3318404447347802, -17.39305756353265409 ) ) ;
#9215=CARTESIAN_POINT ( 'NONE',  ( 107.0210206738092609, 244.8464784336661353, 1.353441290958777327E-15 ) ) ;
#9216=EDGE_LOOP ( 'NONE', ( #93305, #455, #67911, #18178 ) ) ;
#9217=CARTESIAN_POINT ( 'NONE',  ( 190.1358581116424489, 301.3220287403654538, -4.546659160351699036 ) ) ;
#9220=CARTESIAN_POINT ( 'NONE',  ( 163.7707306762541748, 246.9877690064858484, 7.021959502997312086 ) ) ;
#9221=CARTESIAN_POINT ( 'NONE',  ( -22.42236680055709641, 157.8615022471902591, 0.000000000000000000 ) ) ;
#9222=CARTESIAN_POINT ( 'NONE',  ( 175.0461098480248552, 253.1596597119220462, 5.026615068813665488 ) ) ;
#9223=ORIENTED_EDGE ( 'NONE', *, *, #87220, .T. ) ;
#9224=CARTESIAN_POINT ( 'NONE',  ( 132.5758265486178971, 258.8967562850347122, -4.648177544792955347E-16 ) ) ;
#9225=CARTESIAN_POINT ( 'NONE',  ( 154.5661245500915015, 273.4098658877936714, -13.25401299587792536 ) ) ;
#9226=CARTESIAN_POINT ( 'NONE',  ( 185.7214976327387319, 261.5265365697691777, 10.13965854201554073 ) ) ;
#9227=CARTESIAN_POINT ( 'NONE',  ( 206.6395994010593427, 272.7367103121227387, -10.00948282007047219 ) ) ;
#9228=CARTESIAN_POINT ( 'NONE',  ( 138.2797325092426490, 241.4548013555409796, -4.594050593750042211 ) ) ;
#9229=CARTESIAN_POINT ( 'NONE',  ( 189.7369823924603338, 294.6074541219386447, -12.51098987926648753 ) ) ;
#9230=DIRECTION ( 'NONE',  ( -0.8660254037844387076, -0.4999999999999998890, -0.000000000000000000 ) ) ;
#9231=CARTESIAN_POINT ( 'NONE',  ( 187.8039889606625934, 281.5091355175276249, -16.87056948680890756 ) ) ;
#9233=CARTESIAN_POINT ( 'NONE',  ( 42.85403768609726427, 204.7369531367911293, -4.594050593750048428 ) ) ;
#9240=EDGE_CURVE ( 'NONE', #5477, #28117, #47743, .T. ) ;
#9244=CARTESIAN_POINT ( 'NONE',  ( 179.4875127409551112, 292.1681930985448048, -6.151068379627264271 ) ) ;
#9245=CARTESIAN_POINT ( 'NONE',  ( 203.5080190724872011, 278.1607665491929993, -15.47044080916498743 ) ) ;
#9246=EDGE_CURVE ( 'NONE', #84862, #76229, #50278, .T. ) ;
#9247=CARTESIAN_POINT ( 'NONE',  ( 178.3290183710584529, 261.2520505181978479, 12.40287639665870145 ) ) ;
#9249=CARTESIAN_POINT ( 'NONE',  ( 111.2161783173811500, 245.0177522451419065, 5.000000000000046185 ) ) ;
#9252=CARTESIAN_POINT ( 'NONE',  ( 194.6369916712518204, 292.8781080588906889, -14.94731529897440048 ) ) ;
#9253=EDGE_LOOP ( 'NONE', ( #12333, #88653, #19354, #58497 ) ) ;
#9255=CARTESIAN_POINT ( 'NONE',  ( 190.1158090214649405, 301.3567547831981983, -1.340987185199551845 ) ) ;
#9257=CARTESIAN_POINT ( 'NONE',  ( 20.22912401222880519, 191.6744531367911293, 4.594050593750047540 ) ) ;
#9264=CARTESIAN_POINT ( 'NONE',  ( 54.99669585504133096, 215.8927522451419634, 2.944929066748280225E-16 ) ) ;
#9265=CARTESIAN_POINT ( 'NONE',  ( 174.3371462983394338, 288.7746536429086746, 7.657097062861912384 ) ) ;
#9266=CARTESIAN_POINT ( 'NONE',  ( 163.1696954135087481, 256.1584459594707255, -15.01642121154493736 ) ) ;
#9267=CARTESIAN_POINT ( 'NONE',  ( 205.1300674467857164, 275.3512963525735131, -12.60245643603069610 ) ) ;
#9268=CARTESIAN_POINT ( 'NONE',  ( 162.2378990465211928, 251.8756868931907320, -13.00729240934857955 ) ) ;
#9270=CARTESIAN_POINT ( 'NONE',  ( 22.53878541258498558, 190.4865022471903444, -10.00000000000009415 ) ) ;
#9271=CARTESIAN_POINT ( 'NONE',  ( 41.08847453908118297, 182.9824982072973967, 3.021315404115420679E-15 ) ) ;
#9272=CARTESIAN_POINT ( 'NONE',  ( 156.6812872898450735, 261.2670451491295012, 0.000000000000000000 ) ) ;
#9273=CARTESIAN_POINT ( 'NONE',  ( 0.5816933075168655431, 161.9548013555410080, -4.594050593750042211 ) ) ;
#9275=CARTESIAN_POINT ( 'NONE',  ( 167.7414737014567834, 262.5146601742941925, -16.66767127326160036 ) ) ;
#9277=CARTESIAN_POINT ( 'NONE',  ( 186.1263547150109900, 286.8862237501084564, -16.18252752151998308 ) ) ;
#9278=CARTESIAN_POINT ( 'NONE',  ( 164.4494343874829099, 245.8122196953522121, 2.922779519406129456 ) ) ;
#9279=CARTESIAN_POINT ( 'NONE',  ( 183.1778755954215683, 257.7828824734294813, -2.226899175085497617 ) ) ;
#9281=ORIENTED_EDGE ( 'NONE', *, *, #26945, .T. ) ;
#9283=CARTESIAN_POINT ( 'NONE',  ( 178.2609860250628913, 285.7659328021885585, 12.86945330790232411 ) ) ;
#9284=CARTESIAN_POINT ( 'NONE',  ( 155.1343413150030415, 278.7935486042013622, -5.217350409981026615 ) ) ;
#9288=CARTESIAN_POINT ( 'NONE',  ( 206.7923762329701276, 272.4720930770340033, -9.496103119940368487 ) ) ;
#9289=CARTESIAN_POINT ( 'NONE',  ( -22.42236680055709641, 157.8615022471902591, 0.000000000000000000 ) ) ;
#9293=CARTESIAN_POINT ( 'NONE',  ( 193.7261517370125432, 295.1034577671335342, 14.97744313279139661 ) ) ;
#9295=ORIENTED_EDGE ( 'NONE', *, *, #41699, .T. ) ;
#9297=CARTESIAN_POINT ( 'NONE',  ( 192.1396999271463812, 297.8512729055811974, 12.32430960859512403 ) ) ;
#9300=CARTESIAN_POINT ( 'NONE',  ( 201.9093327396327595, 266.8014760598600219, -0.4683226809548139413 ) ) ;
#9302=CARTESIAN_POINT ( 'NONE',  ( 146.6834825911944620, 276.5837508513432681, 0.6716460511724984261 ) ) ;
#9304=AXIS2_PLACEMENT_3D ( 'NONE', #45465, #13592, #60157 ) ;
#9305=EDGE_CURVE ( 'NONE', #59249, #93085, #9000, .T. ) ;
#9307=ORIENTED_EDGE ( 'NONE', *, *, #41896, .T. ) ;
#9308=CARTESIAN_POINT ( 'NONE',  ( 200.1782072557437857, 283.9281697954355650, 18.05177561285849208 ) ) ;
#9311=CARTESIAN_POINT ( 'NONE',  ( 150.6487462746963502, 269.7157126861102370, 15.18501655901553704 ) ) ;
#9313=EDGE_LOOP ( 'NONE', ( #33858, #44053, #54989, #957 ) ) ;
#9314=CARTESIAN_POINT ( 'NONE',  ( 150.4988332210255351, 277.8983191490532363, -3.431260130123086505 ) ) ;
#9315=ORIENTED_EDGE ( 'NONE', *, *, #67086, .F. ) ;
#9316=ORIENTED_EDGE ( 'NONE', *, *, #98609, .F. ) ;
#9319=CARTESIAN_POINT ( 'NONE',  ( 181.5558742819051474, 255.2544784655372894, -2.503599602330015994 ) ) ;
#9325=CARTESIAN_POINT ( 'NONE',  ( 147.7785919239399846, 274.6869658471848652, -7.924750738206837397 ) ) ;
#9331=CARTESIAN_POINT ( 'NONE',  ( 164.3939401533646958, 245.9083385283718712, 2.844462461176849200 ) ) ;
#9332=CARTESIAN_POINT ( 'NONE',  ( 191.5682800193031312, 298.2129472994870412, -9.046807561926330621 ) ) ;
#9333=CARTESIAN_POINT ( 'NONE',  ( 159.3767386493506137, 254.5983864451355032, 15.47015898230477760 ) ) ;
#9336=CARTESIAN_POINT ( 'NONE',  ( 146.8562391379555834, 276.2845277350126025, -4.054588560171046296 ) ) ;
#9337=CARTESIAN_POINT ( 'NONE',  ( 64.47116044126103418, 196.4824982072973683, 3.021315404115420679E-15 ) ) ;
#9338=CARTESIAN_POINT ( 'NONE',  ( 159.8732321751776624, 253.7384344327741132, -15.51998349828054202 ) ) ;
#9339=CARTESIAN_POINT ( 'NONE',  ( 162.8751945631634612, 272.8900720096677333, -16.40198242748087054 ) ) ;
#9340=CARTESIAN_POINT ( 'NONE',  ( 161.2313178023453588, 251.3861611254901618, 13.12937145726518473 ) ) ;
#9341=CARTESIAN_POINT ( 'NONE',  ( 191.0846563742120736, 261.4476523433388593, -0.01535826789041113555 ) ) ;
#9343=CARTESIAN_POINT ( 'NONE',  ( 189.1639574110850504, 261.6477222806883560, 8.036472575680770447 ) ) ;
#9345=CARTESIAN_POINT ( 'NONE',  ( 129.4027117968543621, 255.5177522451419350, 5.000000000000046185 ) ) ;
#9346=CARTESIAN_POINT ( 'NONE',  ( -2.070769811622737766, 159.6115022471902023, -5.000000000000041744 ) ) ;
#9347=CARTESIAN_POINT ( 'NONE',  ( 17.25242200676959570, 180.7677522451418497, 10.00000000000009592 ) ) ;
#9348=CARTESIAN_POINT ( 'NONE',  ( 87.96880888631662287, 221.5958772461660544, -9.188101187500095079 ) ) ;
#9351=CARTESIAN_POINT ( 'NONE',  ( 163.0959165854295065, 248.1565812974573930, 11.58894702640622754 ) ) ;
#9352=CARTESIAN_POINT ( 'NONE',  ( 10.54098545103790840, 167.7048013555410080, 4.594050593750051981 ) ) ;
#9354=CARTESIAN_POINT ( 'NONE',  ( 200.3765029811139584, 283.5847115241710981, 16.85207472104531590 ) ) ;
#9357=FACE_BOUND ( 'NONE', #18930, .T. ) ;
#9358=EDGE_CURVE ( 'NONE', #87622, #32549, #78910, .T. ) ;
#9359=( BOUNDED_CURVE ( )  B_SPLINE_CURVE ( 2, ( #42435, #4450, #49066, #96696, #35350, #41955, #66259, #72890, #34357 ),
 .UNSPECIFIED., .F., .T. ) 
 B_SPLINE_CURVE_WITH_KNOTS ( ( 3, 2, 2, 2, 3 ),
 ( 0.8588709677419354982, 0.8602150537634408733, 0.8629032258064516236, 0.8655913978494623739, 0.8669354838709677491 ),
 .UNSPECIFIED. ) 
 CURVE ( )  GEOMETRIC_REPRESENTATION_ITEM ( )  RATIONAL_B_SPLINE_CURVE ( ( 0.9330127018922194093, 0.9330127018922194093, 1.000000000000000000, 0.8660254037844387076, 1.000000000000000000, 0.8660254037844387076, 1.000000000000000000, 0.9330127018922194093, 0.9330127018922194093 ) ) 
 REPRESENTATION_ITEM ( '' )  );
#9362=CARTESIAN_POINT ( 'NONE',  ( 33.73290511340745468, 201.8297689869269504, -2.679491924311252493 ) ) ;
#9363=CARTESIAN_POINT ( 'NONE',  ( 159.0361281840726804, 267.0969579672368468, 17.40288047604528998 ) ) ;
#9365=CARTESIAN_POINT ( 'NONE',  ( 34.24843087963692767, 181.3923013555409796, 4.594050593750050204 ) ) ;
#9367=CARTESIAN_POINT ( 'NONE',  ( 200.0313018224816801, 276.5939864008022369, 15.71640468486303099 ) ) ;
#9369=CARTESIAN_POINT ( 'NONE',  ( 153.5154549565421291, 274.0811790276123361, -11.99900565267187424 ) ) ;
#9370=EDGE_CURVE ( 'NONE', #19800, #24285, #73081, .T. ) ;
#9371=CARTESIAN_POINT ( 'NONE',  ( 175.2906584782881794, 281.1313530038279964, -15.08317350289036618 ) ) ;
#9373=CARTESIAN_POINT ( 'NONE',  ( -7.997457622663985966, 160.0643266524160140, -9.188101187500093303 ) ) ;
#9374=CARTESIAN_POINT ( 'NONE',  ( 157.8849654228661166, 257.1822134667773980, 17.43614750057631468 ) ) ;
#9376=CARTESIAN_POINT ( 'NONE',  ( 193.9495889092963807, 294.7164532324382549, 15.46986001312306058 ) ) ;
#9377=CARTESIAN_POINT ( 'NONE',  ( 161.7412967960748915, 250.5028515975580774, -14.36228887024421041 ) ) ;
#9378=CARTESIAN_POINT ( 'NONE',  ( 186.3912171902924229, 282.9454464878770068, 16.19148905196400179 ) ) ;
#9379=CARTESIAN_POINT ( 'NONE',  ( 194.1972774922283236, 294.2874440223457100, -15.09915398317898649 ) ) ;
#9380=CARTESIAN_POINT ( 'NONE',  ( 192.5650826088840404, 265.1375965416604004, 7.693037692392531213 ) ) ;
#9381=CARTESIAN_POINT ( 'NONE',  ( 171.6563989851293286, 279.7469309265732704, 14.09156877542037378 ) ) ;
#9382=CARTESIAN_POINT ( 'NONE',  ( 147.2405539530007559, 275.6188749492528132, 0.4306668706573002492 ) ) ;
#9383=CARTESIAN_POINT ( 'NONE',  ( 148.4049257185216106, 273.6021238924720365, 8.639190357831699529 ) ) ;
#9386=CARTESIAN_POINT ( 'NONE',  ( 208.2939409893161553, 269.8713066281881083, 2.523744790997269227 ) ) ;
#9389=CARTESIAN_POINT ( 'NONE',  ( 107.4275774994220001, 223.6423013555409796, -4.594050593750043987 ) ) ;
#9391=CARTESIAN_POINT ( 'NONE',  ( 190.8860811105559208, 300.0226043892405414, 8.636347304323541252 ) ) ;
#9392=CARTESIAN_POINT ( 'NONE',  ( -22.42236680055709641, 157.8615022471902591, 0.000000000000000000 ) ) ;
#9394=CARTESIAN_POINT ( 'NONE',  ( 157.1837449796689725, 258.3967629017010381, 16.97243084443542216 ) ) ;
#9395=CARTESIAN_POINT ( 'NONE',  ( 162.1966646769166402, 251.8715883092360741, -14.10328369067750920 ) ) ;
#9396=CARTESIAN_POINT ( 'NONE',  ( 148.5272680744187141, 275.3902207161408455, -7.185975151065171929 ) ) ;
#9397=CARTESIAN_POINT ( 'NONE',  ( 193.5005633302724277, 262.8551920378705518, -5.236817587991198231 ) ) ;
#9398=CARTESIAN_POINT ( 'NONE',  ( 149.4456112649506281, 271.7996036513546869, -12.95648166494593667 ) ) ;
#9400=CARTESIAN_POINT ( 'NONE',  ( 175.8870957750795583, 292.5986786893511749, -1.137309599147465544 ) ) ;
#9404=CARTESIAN_POINT ( 'NONE',  ( 191.1334924437351219, 271.5868773173968975, -15.78614548220010150 ) ) ;
#9409=CARTESIAN_POINT ( 'NONE',  ( 180.2260403442535051, 295.0423342771414923, -3.480517403894910711 ) ) ;
#9410=CARTESIAN_POINT ( 'NONE',  ( 152.7531861616124615, 266.0707158804971186, 17.45453282433162556 ) ) ;
#9412=ORIENTED_EDGE ( 'NONE', *, *, #19558, .T. ) ;
#9413=B_SPLINE_CURVE_WITH_KNOTS ( 'NONE', 3,
 ( #26087, #41258, #10891, #56962 ),
 .UNSPECIFIED., .F., .F.,
 ( 4, 4 ),
 ( 0.02929424324998682050, 0.03843412274503782422 ),
 .UNSPECIFIED. ) ;
#9414=CARTESIAN_POINT ( 'NONE',  ( 202.6051175132338926, 273.9538057854381350, -13.19822448684500849 ) ) ;
#9417=EDGE_LOOP ( 'NONE', ( #17550, #95200, #90866, #25561 ) ) ;
#9420=CARTESIAN_POINT ( 'NONE',  ( 13.01250597095616612, 184.9865022471903160, 10.00000000000009415 ) ) ;
#9421=ORIENTED_EDGE ( 'NONE', *, *, #3648, .T. ) ;
#9423=DIRECTION ( 'NONE',  ( -0.8660254037844387076, -0.4999999999999998890, -0.000000000000000000 ) ) ;
#9424=CARTESIAN_POINT ( 'NONE',  ( 164.2059258710715994, 246.2339888178522926, 7.329631442356459914 ) ) ;
#9429=CARTESIAN_POINT ( 'NONE',  ( 155.6535436963908694, 261.0471492701456668, -17.87366571046205976 ) ) ;
#9431=EDGE_CURVE ( 'NONE', #24288, #80596, #84055, .T. ) ;
#9433=CARTESIAN_POINT ( 'NONE',  ( 178.7753799676760593, 260.4554649793954582, 12.02876886862545902 ) ) ;
#9436=EDGE_LOOP ( 'NONE', ( #87482, #85290 ) ) ;
#9437=CARTESIAN_POINT ( 'NONE',  ( 173.2337249902883798, 270.7486416191997023, 17.82094672905207133 ) ) ;
#9439=ORIENTED_EDGE ( 'NONE', *, *, #8873, .F. ) ;
#9440=CARTESIAN_POINT ( 'NONE',  ( 185.9161404575009158, 282.4097951900486123, -17.21525070205280628 ) ) ;
#9443=CARTESIAN_POINT ( 'NONE',  ( 170.8805640699686990, 257.7213711969266114, 14.63406020945912367 ) ) ;
#9444=CARTESIAN_POINT ( 'NONE',  ( 196.2953682204578456, 263.5854184417236752, 0.8810977108677261471 ) ) ;
#9445=AXIS2_PLACEMENT_3D ( 'NONE', #2121, #72023, #40085 ) ;
#9446=B_SPLINE_CURVE_WITH_KNOTS ( 'NONE', 3,
 ( #45027, #90695, #59209, #68327 ),
 .UNSPECIFIED., .F., .F.,
 ( 4, 4 ),
 ( 0.01331880355540019864, 0.01957602511303062343 ),
 .UNSPECIFIED. ) ;
#9447=CARTESIAN_POINT ( 'NONE',  ( 201.4066285247549786, 281.8004817444100354, -17.79749223817309201 ) ) ;
#9450=CIRCLE ( 'NONE', #85564, 17.82106496071138935 ) ;
#9451=CARTESIAN_POINT ( 'NONE',  ( 153.9322886533809083, 279.5979162416960548, 2.179338631777613333 ) ) ;
#9452=CARTESIAN_POINT ( 'NONE',  ( 131.5951856977227123, 234.5327760586659451, 1.948934522072303157E-15 ) ) ;
#9453=CARTESIAN_POINT ( 'NONE',  ( 186.1868697629463725, 262.4753163803031271, -9.036959360852598877 ) ) ;
#9454=B_SPLINE_CURVE_WITH_KNOTS ( 'NONE', 3,
 ( #92109, #29264, #22656, #60134, #21661, #52542, #83493, #44940, #75884, #6462, #29755, #60627, #47436, #15033, #78869, #77351, #86014, #45925, #16541, #40325, #15525, #70745, #46426, #24640, #46946, #9453, #8945, #55520, #7958, #39813, #94583, #77863, #8449, #86508, #47929, #69240, #1356, #17037, #38832, #39320, #7440, #31235, #30756, #100170, #71265, #32241, #16044, #38332, #62625, #84489 ),
 .UNSPECIFIED., .F., .F.,
 ( 4, 2, 2, 2, 2, 2, 2, 2, 2, 2, 2, 2, 2, 2, 2, 2, 2, 2, 2, 2, 2, 2, 2, 2, 4 ),
 ( 0.0002765172614649375328, 0.001291974074908197687, 0.001799702481629788598, 0.002053566684990593919, 0.002180498786671015987, 0.002307430888351438489, 0.002434362990031860557, 0.002561295091712283058, 0.002815159295073127628, 0.003322887701794880085, 0.004338344515238447448, 0.005353801328682013944, 0.005861529735403797625, 0.006115393938764732834, 0.006369258142125667176, 0.006432724192965878426, 0.006496190243806089677, 0.006559656294646300928, 0.006623122345486511311, 0.006876986548847315549, 0.007384714955568918819, 0.007638579158929679688, 0.007892443362290439690, 0.008146307565651199692, 0.008400171769011959694 ),
 .UNSPECIFIED. ) ;
#9456=AXIS2_PLACEMENT_3D ( 'NONE', #41110, #78649, #94370 ) ;
#9457=ORIENTED_EDGE ( 'NONE', *, *, #90113, .T. ) ;
#9461=CARTESIAN_POINT ( 'NONE',  ( 200.1427641401880066, 273.7077546088841586, 13.87784847088884810 ) ) ;
#9463=CARTESIAN_POINT ( 'NONE',  ( 165.3413037017489273, 246.0692819571209213, -2.848003664914541044 ) ) ;
#9467=CARTESIAN_POINT ( 'NONE',  ( 174.3231258461450466, 287.3639690219702061, -9.459891945542938885 ) ) ;
#9468=EDGE_CURVE ( 'NONE', #8907, #68859, #6146, .T. ) ;
#9473=CARTESIAN_POINT ( 'NONE',  ( 194.4032909867620447, 293.9306181827685123, -16.05392006271526384 ) ) ;
#9474=CARTESIAN_POINT ( 'NONE',  ( 8.159155267032986103, 175.5177522451418781, -10.00000000000009592 ) ) ;
#9477=CARTESIAN_POINT ( 'NONE',  ( 190.4221740917990928, 282.9812683428133369, -16.56494496364181401 ) ) ;
#9478=CARTESIAN_POINT ( 'NONE',  ( 191.9719415786559864, 298.1418388885606419, -10.91218611428179663 ) ) ;
#9479=CARTESIAN_POINT ( 'NONE',  ( 190.0274641710971082, 301.5097725526222803, 3.738976720635653450 ) ) ;
#9480=CARTESIAN_POINT ( 'NONE',  ( 163.0171530587457767, 248.2930037274571191, 9.677214176418313940 ) ) ;
#9481=CARTESIAN_POINT ( 'NONE',  ( 162.6609004217042127, 282.2048157055750153, -6.605852966852150843 ) ) ;
#9482=CARTESIAN_POINT ( 'NONE',  ( 154.9430233944070494, 277.5162282063104158, -8.894456736302846167 ) ) ;
#9483=CARTESIAN_POINT ( 'NONE',  ( 199.9620668144054036, 267.3927500580807077, 6.252404634128969185 ) ) ;
#9486=B_SPLINE_SURFACE_WITH_KNOTS ( 'NONE', 3, 1, ( 
 ( #41780, #1801 ),
 ( #2309, #56974 ),
 ( #64090, #40269 ),
 ( #87473, #71718 ),
 ( #2817, #25079 ),
 ( #33190, #17489 ),
 ( #48899, #87960 ),
 ( #56485, #18504 ),
 ( #78806, #79835 ),
 ( #32685, #9394 ),
 ( #10904, #86954 ),
 ( #18007, #48395 ),
 ( #72213, #80335 ),
 ( #47382, #78306 ),
 ( #63586, #39756 ),
 ( #33708, #9908 ),
 ( #64599, #49390 ),
 ( #72726, #3317 ),
 ( #1299, #63085 ),
 ( #34197, #65087 ),
 ( #94031, #24582 ),
 ( #27101, #67073 ),
 ( #28576, #67573 ),
 ( #36170, #50382 ),
 ( #11420, #89443 ),
 ( #26599, #13398 ),
 ( #19999, #58470 ),
 ( #21008, #5777 ),
 ( #42763, #44270 ),
 ( #58951, #81334 ),
 ( #35179, #89923 ),
 ( #57985, #96531 ),
 ( #20501, #3801 ),
 ( #97996, #12402 ) ),
 .UNSPECIFIED., .T., .F., .F.,
 ( 4, 2, 2, 2, 2, 2, 2, 2, 2, 2, 2, 2, 2, 2, 2, 2, 4 ),
 ( 2, 2 ),
 ( 0.000000000000000000, 0.06250000000000000000, 0.1250000000000000000, 0.1875000000000000000, 0.2500000000000000000, 0.3125000000000000000, 0.3750000000000000000, 0.4375000000000000000, 0.5000000000000000000, 0.5625000000000000000, 0.6250000000000000000, 0.6875000000000000000, 0.7500000000000000000, 0.8125000000000000000, 0.8750000000000000000, 0.9375000000000000000, 1.000000000000000000 ),
 ( 0.000000000000000000, 1.000000000000000000 ),
 .UNSPECIFIED. ) ;
#9488=CARTESIAN_POINT ( 'NONE',  ( 164.1364336533802373, 247.9930260721589832, -8.912795639077232934 ) ) ;
#9489=CARTESIAN_POINT ( 'NONE',  ( 190.0387662407789549, 274.4106552748930312, -15.66928402959891997 ) ) ;
#9492=B_SPLINE_CURVE_WITH_KNOTS ( 'NONE', 3,
 ( #83602, #37936, #90214, #99279 ),
 .UNSPECIFIED., .F., .F.,
 ( 4, 4 ),
 ( 0.01043980270801778479, 0.01580741937697933627 ),
 .UNSPECIFIED. ) ;
#9493=CARTESIAN_POINT ( 'NONE',  ( 186.8081210542937356, 297.5510969845519753, -4.266410382973029769 ) ) ;
#9494=CARTESIAN_POINT ( 'NONE',  ( 192.6470966816805230, 296.9724359471326807, 11.11268290051284424 ) ) ;
#9497=CARTESIAN_POINT ( 'NONE',  ( 194.0672051292551430, 294.5127359636757660, 15.53337744471869364 ) ) ;
#9499=CARTESIAN_POINT ( 'NONE',  ( 2.016134656476094023, 159.7202760586659451, -5.415160957724236172E-17 ) ) ;
#9500=CARTESIAN_POINT ( 'NONE',  ( 86.39896429407481548, 226.8149278399160664, 9.188101187500093303 ) ) ;
#9502=CARTESIAN_POINT ( 'NONE',  ( 192.4335622838504207, 297.3422883733380786, -12.83044365323471325 ) ) ;
#9503=CARTESIAN_POINT ( 'NONE',  ( 147.7258779941464297, 275.3197464395427119, 3.871639344198308574 ) ) ;
#9505=CARTESIAN_POINT ( 'NONE',  ( 203.2369479875374623, 278.6302754407888074, -16.66242713208754367 ) ) ;
#9512=CARTESIAN_POINT ( 'NONE',  ( 163.4139553296302267, 247.6057220337265505, -10.31482883765270842 ) ) ;
#9514=CARTESIAN_POINT ( 'NONE',  ( 178.0260107266225020, 289.8946666044191716, 9.616295053996276820 ) ) ;
#9517=B_SPLINE_CURVE_WITH_KNOTS ( 'NONE', 3,
 ( #49937, #96587, #57024, #65629, #65137, #66135, #11469, #27151, #3846, #96085, #35234, #4854, #20053, #12452 ),
 .UNSPECIFIED., .F., .F.,
 ( 4, 2, 2, 2, 2, 2, 4 ),
 ( 0.001120812635800888610, 0.001358725036700777480, 0.001596637437600666133, 0.001834549838500555002, 0.002072462239400443655, 0.002548287041200175858, 0.003024111842999908061 ),
 .UNSPECIFIED. ) ;
#9520=CARTESIAN_POINT ( 'NONE',  ( -12.69762320744227502, 170.1427522451419350, -10.00000000000009592 ) ) ;
#9521=CARTESIAN_POINT ( 'NONE',  ( 34.76219959342768107, 197.0024278399161233, 9.188101187500095079 ) ) ;
#9524=CARTESIAN_POINT ( 'NONE',  ( 59.87693630317638593, 211.5024278399160949, -9.188101187500093303 ) ) ;
#9532=CARTESIAN_POINT ( 'NONE',  ( 196.8111907360481609, 268.4516160315483830, -10.82598805925545626 ) ) ;
#9534=CARTESIAN_POINT ( 'NONE',  ( 41.08847453908118297, 182.9824982072973967, 3.021315404115420679E-15 ) ) ;
#9536=ORIENTED_EDGE ( 'NONE', *, *, #67306, .F. ) ;
#9538=CARTESIAN_POINT ( 'NONE',  ( 58.09093245575348874, 204.3458772461660544, 9.188101187500095079 ) ) ;
#9542=CARTESIAN_POINT ( 'NONE',  ( 198.5612432604688991, 286.7288335892616260, 18.30793681285053509 ) ) ;
#9544=CARTESIAN_POINT ( 'NONE',  ( 153.8017027926681521, 264.2546318029277472, 18.09987928383549516 ) ) ;
#9548=CARTESIAN_POINT ( 'NONE',  ( 130.4311169673963775, 236.1115022471901739, -5.000000000000041744 ) ) ;
#9549=CARTESIAN_POINT ( 'NONE',  ( 165.0156970625405108, 244.8314239717225007, -1.890480716182876719 ) ) ;
#9552=CARTESIAN_POINT ( 'NONE',  ( 188.2373216092262282, 273.3416365267268588, 15.62028696804763683 ) ) ;
#9554=CARTESIAN_POINT ( 'NONE',  ( 206.2809287719926488, 273.3579460648492159, -10.70911012174624588 ) ) ;
#9558=CARTESIAN_POINT ( 'NONE',  ( 177.0689902789707730, 252.6641302495915511, -0.2682384293953795629 ) ) ;
#9559=EDGE_LOOP ( 'NONE', ( #67347, #82118, #10949, #76829 ) ) ;
#9561=CARTESIAN_POINT ( 'NONE',  ( 170.5571078448917888, 250.3859201599777293, 3.400624622539324182 ) ) ;
#9562=CARTESIAN_POINT ( 'NONE',  ( 148.7859755799365189, 273.9149749650962349, 8.803960254582356981 ) ) ;
#9564=ADVANCED_FACE ( 'NONE', ( #85423 ), #68706, .F. ) ;
#9569=EDGE_LOOP ( 'NONE', ( #81376, #43308, #66224, #44522 ) ) ;
#9571=CARTESIAN_POINT ( 'NONE',  ( 159.5895502557670795, 254.2297859303815244, -16.92708575547316485 ) ) ;
#9574=CARTESIAN_POINT ( 'NONE',  ( 185.4975199963478474, 297.4654133624536598, 1.032910119675109817 ) ) ;
#9575=CARTESIAN_POINT ( 'NONE',  ( 194.8708600166808651, 293.1207648669033006, -14.79199694356877970 ) ) ;
#9577=CARTESIAN_POINT ( 'NONE',  ( 193.9966098916996771, 294.6350105018939871, 13.97117019253516013 ) ) ;
#9578=CARTESIAN_POINT ( 'NONE',  ( 185.4470681627111901, 292.4290838876615908, -11.21142039403692259 ) ) ;
#9579=CARTESIAN_POINT ( 'NONE',  ( 157.8239779013331372, 257.2878469527003062, -17.92251383114021479 ) ) ;
#9581=ADVANCED_FACE ( 'NONE', ( #52105 ), #7497, .T. ) ;
#9583=CARTESIAN_POINT ( 'NONE',  ( 179.3546098028610061, 287.2282261399536196, -13.91071825436259601 ) ) ;
#9584=CARTESIAN_POINT ( 'NONE',  ( 92.13672968991174628, 217.8768266524159856, 9.188101187500098632 ) ) ;
#9586=CARTESIAN_POINT ( 'NONE',  ( 190.8094645593471341, 300.1553081486349015, 8.399847186519689757 ) ) ;
#9590=CARTESIAN_POINT ( 'NONE',  ( 156.6856598554248023, 259.2594716433859503, -17.52902947127937949 ) ) ;
#9592=CARTESIAN_POINT ( 'NONE',  ( 189.0689802957956260, 269.8288687927027354, -15.50864081522695415 ) ) ;
#9594=EDGE_CURVE ( 'NONE', #35100, #44921, #94800, .T. ) ;
#9595=CARTESIAN_POINT ( 'NONE',  ( 191.7187529716733820, 298.5803744197520473, -8.487597704798396592 ) ) ;
#9596=DIRECTION ( 'NONE',  ( 0.5000000000000048850, -0.8660254037844358210, 0.000000000000000000 ) ) ;
#9598=CARTESIAN_POINT ( 'NONE',  ( 162.6419541827858950, 248.9428672435623184, 10.30167521348375459 ) ) ;
#9600=CARTESIAN_POINT ( 'NONE',  ( 89.86341300497758766, 216.5643266524160140, 9.188101187500095079 ) ) ;
#9601=VERTEX_POINT ( 'NONE', #28819 ) ;
#9603=CARTESIAN_POINT ( 'NONE',  ( 123.3405339703633672, 232.0177522451417929, 5.000000000000051514 ) ) ;
#9604=CARTESIAN_POINT ( 'NONE',  ( 163.3473224498206093, 247.7211335670114352, -10.00320358166632850 ) ) ;
#9608=CARTESIAN_POINT ( 'NONE',  ( -22.42236680055709641, 157.8615022471902591, 0.000000000000000000 ) ) ;
#9609=CARTESIAN_POINT ( 'NONE',  ( 165.1340499804484523, 285.1150614822342391, 0.5054430236558116185 ) ) ;
#9610=CARTESIAN_POINT ( 'NONE',  ( 101.3470971569689141, 235.9865022471903160, 10.00000000000009415 ) ) ;
#9612=AXIS2_PLACEMENT_3D ( 'NONE', #95245, #25814, #12098 ) ;
#9615=CARTESIAN_POINT ( 'NONE',  ( 160.6168281341388422, 275.7216313598870556, 14.06045084403267609 ) ) ;
#9617=CARTESIAN_POINT ( 'NONE',  ( 206.8659638600981623, 272.3446355680395641, -10.26115277030573125 ) ) ;
#9619=CARTESIAN_POINT ( 'NONE',  ( 176.8429236348229381, 284.5432036437209717, 13.07041713469269162 ) ) ;
#9620=CARTESIAN_POINT ( 'NONE',  ( 106.8860512984590088, 232.5177522451418781, -10.00000000000009592 ) ) ;
#9621=CARTESIAN_POINT ( 'NONE',  ( 195.4522889637296146, 279.6111606360764767, -17.26969813293585787 ) ) ;
#9623=CARTESIAN_POINT ( 'NONE',  ( 8.774901663922227257, 164.3262482093457777, 3.021315404115420679E-15 ) ) ;
#9625=EDGE_CURVE ( 'NONE', #14882, #41928, #6398, .T. ) ;
#9626=CARTESIAN_POINT ( 'NONE',  ( 161.1611771195837548, 251.5076483517112536, 14.17749514252127163 ) ) ;
#9628=CARTESIAN_POINT ( 'NONE',  ( 188.1686623141184782, 265.7851399264815768, -13.17430125897227455 ) ) ;
#9632=ORIENTED_EDGE ( 'NONE', *, *, #59835, .F. ) ;
#9634=CIRCLE ( 'NONE', #50045, 17.82106496071138224 ) ;
#9640=CARTESIAN_POINT ( 'NONE',  ( 99.25420243115659957, 218.1115022471901739, -5.000000000000041744 ) ) ;
#9641=CARTESIAN_POINT ( 'NONE',  ( 168.8294252543820448, 272.9399934659655287, 15.96329185404338524 ) ) ;
#9642=CARTESIAN_POINT ( 'NONE',  ( 180.5963630788930061, 273.1050420172064719, 16.83617887608246022 ) ) ;
#9644=CARTESIAN_POINT ( 'NONE',  ( 188.2974456734137902, 260.8608515763677360, 2.891147047799000447 ) ) ;
#9645=CARTESIAN_POINT ( 'NONE',  ( 195.4288765293300401, 265.1666311804774523, -7.729559632884401843 ) ) ;
#9646=CARTESIAN_POINT ( 'NONE',  ( -2.639098984630277922, 169.2833772461660828, -9.188101187500095079 ) ) ;
#9648=VERTEX_POINT ( 'NONE', #47008 ) ;
#9649=CARTESIAN_POINT ( 'NONE',  ( 161.2566224172725242, 253.0718664474237869, -14.99040694173076993 ) ) ;
#9653=CARTESIAN_POINT ( 'NONE',  ( 24.04513522159523475, 190.8149278399161233, 9.188101187500093303 ) ) ;
#9656=CARTESIAN_POINT ( 'NONE',  ( 178.5176923076055573, 291.6601484728420814, 5.967418820694346593 ) ) ;
#9657=CARTESIAN_POINT ( 'NONE',  ( 196.3455846056825465, 290.5664669515812761, 16.75698796588176265 ) ) ;
#9658=CARTESIAN_POINT ( 'NONE',  ( 133.4825598088814047, 236.3262482093457493, 3.021315404115420679E-15 ) ) ;
#9659=CARTESIAN_POINT ( 'NONE',  ( 168.3557124657904467, 273.6222795104500278, 17.14480014634877136 ) ) ;
#9660=CARTESIAN_POINT ( 'NONE',  ( 187.2709071308663056, 296.1806672229488413, -7.704019758776238902 ) ) ;
#9662=CARTESIAN_POINT ( 'NONE',  ( 65.47921168356343458, 208.6115022471902307, 10.00000000000009592 ) ) ;
#9663=( BOUNDED_CURVE ( )  B_SPLINE_CURVE ( 2, ( #96251, #42980, #72941, #74925, #57196, #73918, #4011, #5507, #34894 ),
 .UNSPECIFIED., .F., .T. ) 
 B_SPLINE_CURVE_WITH_KNOTS ( ( 3, 2, 2, 2, 3 ),
 ( 0.5362903225806451291, 0.5376344086021505042, 0.5403225806451612545, 0.5430107526881720048, 0.5443548387096773800 ),
 .UNSPECIFIED. ) 
 CURVE ( )  GEOMETRIC_REPRESENTATION_ITEM ( )  RATIONAL_B_SPLINE_CURVE ( ( 0.9330127018922194093, 0.9330127018922194093, 1.000000000000000000, 0.8660254037844387076, 1.000000000000000000, 0.8660254037844387076, 1.000000000000000000, 0.9330127018922194093, 0.9330127018922194093 ) ) 
 REPRESENTATION_ITEM ( '' )  );
#9664=CARTESIAN_POINT ( 'NONE',  ( 165.2807093860638474, 245.9288570166273473, 0.7599370718198323882 ) ) ;
#9665=CARTESIAN_POINT ( 'NONE',  ( 189.6738045434663320, 300.1223289962524063, 4.832295392723879424 ) ) ;
#9667=CARTESIAN_POINT ( 'NONE',  ( 33.92367135321775606, 181.2048013555409796, 4.594050593750051981 ) ) ;
#9669=EDGE_CURVE ( 'NONE', #18151, #99635, #53663, .T. ) ;
#9670=CARTESIAN_POINT ( 'NONE',  ( 66.70608100559137199, 215.9865022471902876, -10.00000000000009592 ) ) ;
#9671=CARTESIAN_POINT ( 'NONE',  ( 205.7230952882032966, 269.3306732399635735, -3.168671107954665445 ) ) ;
#9673=ORIENTED_EDGE ( 'NONE', *, *, #38121, .T. ) ;
#9675=CARTESIAN_POINT ( 'NONE',  ( 168.0327857633167241, 281.9162007134196415, -10.99116794043863976 ) ) ;
#9677=CARTESIAN_POINT ( 'NONE',  ( 205.6976855946065825, 269.4214810134713503, -1.331547403361390325 ) ) ;
#9679=CARTESIAN_POINT ( 'NONE',  ( 163.0309151244508712, 248.2691671304387739, 11.27270415168660200 ) ) ;
#9680=CARTESIAN_POINT ( 'NONE',  ( 149.6564118588553924, 271.4344863124460971, -11.76165597393390172 ) ) ;
#9681=CARTESIAN_POINT ( 'NONE',  ( 188.6600893746942802, 269.8527292173970409, -14.07731609263537997 ) ) ;
#9682=ORIENTED_EDGE ( 'NONE', *, *, #87329, .F. ) ;
#9691=CARTESIAN_POINT ( 'NONE',  ( 190.6661865267473104, 300.4034729807058852, 4.523489664447863490 ) ) ;
#9692=VERTEX_POINT ( 'NONE', #10518 ) ;
#9694=ORIENTED_EDGE ( 'NONE', *, *, #52208, .T. ) ;
#9695=FACE_OUTER_BOUND ( 'NONE', #11570, .T. ) ;
#9702=CARTESIAN_POINT ( 'NONE',  ( 168.5910505471324257, 286.4687829538495976, 8.106709794022206594 ) ) ;
#9703=CARTESIAN_POINT ( 'NONE',  ( 102.2314250767153538, 220.6423013555409796, -4.594050593750043987 ) ) ;
#9705=CARTESIAN_POINT ( 'NONE',  ( 196.2379679265050925, 290.7528645076583871, -16.93678934971137906 ) ) ;
#9708=ORIENTED_EDGE ( 'NONE', *, *, #66888, .T. ) ;
#9709=CARTESIAN_POINT ( 'NONE',  ( 164.2647213391612979, 246.1321520798662164, -5.830872732487307530 ) ) ;
#9712=CARTESIAN_POINT ( 'NONE',  ( 198.0006249058153003, 287.6998530631771587, 18.31850453277666801 ) ) ;
#9714=CARTESIAN_POINT ( 'NONE',  ( 56.95444766116892055, 197.5643266524159856, -9.188101187500093303 ) ) ;
#9718=CARTESIAN_POINT ( 'NONE',  ( 190.8001679306945277, 300.1714103817999444, 7.815449226872675403 ) ) ;
#9719=CARTESIAN_POINT ( 'NONE',  ( 150.2452556859942376, 270.4145788861182496, 14.49525683977126533 ) ) ;
#9720=CARTESIAN_POINT ( 'NONE',  ( 175.1864013481757354, 272.4254438080928935, 16.55480563948633943 ) ) ;
#9721=ADVANCED_FACE ( 'NONE', ( #88573 ), #27218, .T. ) ;
#9727=ORIENTED_EDGE ( 'NONE', *, *, #7528, .T. ) ;
#9728=CARTESIAN_POINT ( 'NONE',  ( 175.4002342268021835, 261.2927254388914662, -14.34716763164142783 ) ) ;
#9730=B_SPLINE_CURVE_WITH_KNOTS ( 'NONE', 3,
 ( #7014, #82581, #53605, #68312 ),
 .UNSPECIFIED., .F., .F.,
 ( 4, 4 ),
 ( 0.002571105401923278258, 0.005038221485946379335 ),
 .UNSPECIFIED. ) ;
#9731=CARTESIAN_POINT ( 'NONE',  ( 146.5088695963383429, 276.8861894300958966, 0.09882562957467418141 ) ) ;
#9732=CARTESIAN_POINT ( 'NONE',  ( 146.7944005049231180, 276.3916353892955726, -4.243051111306586520 ) ) ;
#9733=CARTESIAN_POINT ( 'NONE',  ( 190.7222376050763444, 300.3063896652212179, 3.365789908110941475 ) ) ;
#9734=CARTESIAN_POINT ( 'NONE',  ( 178.5543832690894703, 270.1946074348090292, 16.14052137089361949 ) ) ;
#9737=CARTESIAN_POINT ( 'NONE',  ( 154.4594390210350809, 264.0928981614183044, -16.94021933189004514 ) ) ;
#9739=CARTESIAN_POINT ( 'NONE',  ( 111.1617914095948692, 244.1744531367911293, 4.594050593750047540 ) ) ;
#9741=CARTESIAN_POINT ( 'NONE',  ( 146.7373254022577100, 276.4904923669593586, -0.7242168585908188572 ) ) ;
#9743=CARTESIAN_POINT ( 'NONE',  ( 203.3740894404336927, 278.3927394765486838, -15.19753795879846869 ) ) ;
#9746=CARTESIAN_POINT ( 'NONE',  ( 175.6023453674955022, 252.6114453084666991, 5.260320833529300799 ) ) ;
#9750=CARTESIAN_POINT ( 'NONE',  ( 158.4848075976798327, 275.1236941057235299, -12.43667617850595875 ) ) ;
#9751=CARTESIAN_POINT ( 'NONE',  ( 185.8714895211756755, 261.7232839879937956, 10.07181324648456311 ) ) ;
#9752=FACE_OUTER_BOUND ( 'NONE', #12412, .T. ) ;
#9753=CARTESIAN_POINT ( 'NONE',  ( 198.5201458116119397, 286.8000164587433005, -18.30276554821096013 ) ) ;
#9754=CARTESIAN_POINT ( 'NONE',  ( 185.5176298084847417, 297.3635137698159383, 4.083851266084445264 ) ) ;
#9756=CARTESIAN_POINT ( 'NONE',  ( 60.33744616864313315, 196.4548013555410080, -4.594050593750042211 ) ) ;
#9760=CARTESIAN_POINT ( 'NONE',  ( 171.8127856075278430, 259.9554699241354569, 15.47650383583072653 ) ) ;
#9763=FACE_OUTER_BOUND ( 'NONE', #60638, .T. ) ;
#9764=CARTESIAN_POINT ( 'NONE',  ( 157.2286243502475429, 270.8137009750436732, -14.73200381606329223 ) ) ;
#9765=CARTESIAN_POINT ( 'NONE',  ( 126.8768043691498377, 237.3927522451418213, 10.00000000000009592 ) ) ;
#9766=B_SPLINE_SURFACE_WITH_KNOTS ( 'NONE', 3, 1, ( 
 ( #94632, #2927 ),
 ( #12381, #9512 ),
 ( #79939, #40376 ),
 ( #26203, #72322 ),
 ( #71817, #48505 ),
 ( #20480, #10498 ),
 ( #57082, #79443 ),
 ( #32788, #18103 ),
 ( #56071, #82319 ),
 ( #5269, #10008 ),
 ( #74691, #40871 ),
 ( #43247, #64194 ),
 ( #28551, #47980 ),
 ( #49005, #78925 ),
 ( #41382, #33817 ),
 ( #64704, #4781 ),
 ( #66564, #97491 ),
 ( #28056, #58931 ),
 ( #51353, #12890 ),
 ( #43747, #36148 ),
 ( #67052, #97975 ),
 ( #75669, #29074 ),
 ( #68051, #22939 ),
 ( #68545, #6757 ),
 ( #38640, #98973 ),
 ( #90911, #91388 ),
 ( #22450, #21950 ),
 ( #82808, #99471 ),
 ( #99970, #92392 ),
 ( #29558, #152 ),
 ( #53828, #98483 ),
 ( #61438, #83292 ),
 ( #84788, #60431 ),
 ( #37151, #61928 ) ),
 .UNSPECIFIED., .T., .F., .F.,
 ( 4, 2, 2, 2, 2, 2, 2, 2, 2, 2, 2, 2, 2, 2, 2, 2, 4 ),
 ( 2, 2 ),
 ( 0.000000000000000000, 0.06250000000000000000, 0.1250000000000000000, 0.1875000000000000000, 0.2500000000000000000, 0.3125000000000000000, 0.3750000000000000000, 0.4375000000000000000, 0.5000000000000000000, 0.5625000000000000000, 0.6250000000000000000, 0.6875000000000000000, 0.7500000000000000000, 0.8125000000000000000, 0.8750000000000000000, 0.9375000000000000000, 1.000000000000000000 ),
 ( 0.000000000000000000, 1.000000000000000000 ),
 .UNSPECIFIED. ) ;
#9769=CARTESIAN_POINT ( 'NONE',  ( 163.4004183463084416, 247.6291687766210146, 10.19167732382099345 ) ) ;
#9771=CARTESIAN_POINT ( 'NONE',  ( 49.16021902710897251, 193.0643266524159856, -9.188101187500093303 ) ) ;
#9775=CARTESIAN_POINT ( 'NONE',  ( 177.1262862392189845, 269.6057104283654553, 17.56656865388298172 ) ) ;
#9778=CARTESIAN_POINT ( 'NONE',  ( 58.31645990288169656, 211.1427522451419065, 10.00000000000009237 ) ) ;
#9779=CARTESIAN_POINT ( 'NONE',  ( 171.6130448281033125, 286.7680181827872730, 7.456980690989077232 ) ) ;
#9780=CARTESIAN_POINT ( 'NONE',  ( 183.3475561009241233, 257.5467204516681363, 1.327541498361791694 ) ) ;
#9781=CARTESIAN_POINT ( 'NONE',  ( 204.9658583905037688, 275.6357147811169170, -12.57240504404813564 ) ) ;
#9782=CARTESIAN_POINT ( 'NONE',  ( -27.42236680055714260, 166.5217562850347406, 1.224646799147364892E-15 ) ) ;
#9784=ADVANCED_FACE ( 'NONE', ( #35799 ), #36291, .T. ) ;
#9785=CARTESIAN_POINT ( 'NONE',  ( 161.8086887434684797, 267.2572688397011689, 16.48344843794798820 ) ) ;
#9786=CARTESIAN_POINT ( 'NONE',  ( 24.41517378745133371, 178.2365022471902307, 10.00000000000009592 ) ) ;
#9787=CARTESIAN_POINT ( 'NONE',  ( 198.2505066714982149, 285.2670451491296149, 0.000000000000000000 ) ) ;
#9789=CARTESIAN_POINT ( 'NONE',  ( -13.19395714113563045, 169.3149278399160949, -9.188101187500095079 ) ) ;
#9791=CARTESIAN_POINT ( 'NONE',  ( 170.2708277436370565, 263.6177537115055429, 15.82973544656882403 ) ) ;
#9793=CARTESIAN_POINT ( 'NONE',  ( 33.17822050123679389, 178.4155109091895781, 2.679491924311254714 ) ) ;
#9795=CARTESIAN_POINT ( 'NONE',  ( 206.3505875407052486, 273.2372935382459787, 11.62318091048137880 ) ) ;
#9796=CARTESIAN_POINT ( 'NONE',  ( 183.1752028583183574, 257.7612102956644549, -2.166713690560386762 ) ) ;
#9800=CARTESIAN_POINT ( 'NONE',  ( 150.1530336415601710, 271.4893706449333877, -12.31841913146343082 ) ) ;
#9803=CARTESIAN_POINT ( 'NONE',  ( 168.3660592861385226, 287.3002883228049313, 0.5084154714863498015 ) ) ;
#9805=CARTESIAN_POINT ( 'NONE',  ( 207.2299632185859650, 271.7141701852165738, 8.357384014234831682 ) ) ;
#9807=CARTESIAN_POINT ( 'NONE',  ( 159.2536436069973718, 254.8115933126508992, -15.76697951715411250 ) ) ;
#9808=CARTESIAN_POINT ( 'NONE',  ( 63.45052750612631343, 195.8932355074535678, -2.679491924311248496 ) ) ;
#9811=CARTESIAN_POINT ( 'NONE',  ( 207.5338226493333025, 271.1878702128032614, 6.432541580693135863 ) ) ;
#9812=CARTESIAN_POINT ( 'NONE',  ( 104.0173421519710217, 220.8615022471902023, 5.000000000000051514 ) ) ;
#9816=EDGE_LOOP ( 'NONE', ( #49184, #3581, #17309, #59304 ) ) ;
#9821=CARTESIAN_POINT ( 'NONE',  ( 188.9790587790324992, 297.2113717040124925, 7.911450463245256692 ) ) ;
#9822=ORIENTED_EDGE ( 'NONE', *, *, #94621, .T. ) ;
#9827=CARTESIAN_POINT ( 'NONE',  ( 175.0917972779528213, 268.1668903562270430, 16.25173907998583900 ) ) ;
#9829=CARTESIAN_POINT ( 'NONE',  ( 151.4361976351029000, 268.3518069213970421, 15.15218985681980612 ) ) ;
#9830=CARTESIAN_POINT ( 'NONE',  ( 149.0959704726320751, 273.8919761871559331, -8.765438422576197652 ) ) ;
#9831=ORIENTED_EDGE ( 'NONE', *, *, #57284, .F. ) ;
#9832=CARTESIAN_POINT ( 'NONE',  ( 173.4125187911463684, 257.0454188278081915, -11.72670941500022757 ) ) ;
#9833=CARTESIAN_POINT ( 'NONE',  ( 202.9685995779611858, 279.0950685203052899, 16.84977534244423580 ) ) ;
#9835=EDGE_CURVE ( 'NONE', #43311, #42198, #51341, .T. ) ;
#9836=ORIENTED_EDGE ( 'NONE', *, *, #78555, .T. ) ;
#9838=VERTEX_POINT ( 'NONE', #75819 ) ;
#9840=CARTESIAN_POINT ( 'NONE',  ( 161.1595886466168679, 271.1349891283304601, 16.19772519489564999 ) ) ;
#9841=ORIENTED_EDGE ( 'NONE', *, *, #23026, .T. ) ;
#9848=B_SPLINE_CURVE_WITH_KNOTS ( 'NONE', 3,
 ( #75280, #83395, #67658, #12992, #66661, #74301, #81907, #37250, #42840, #89524, #51460, #5864, #36253, #59538, #52450, #28163, #36749, #97116, #19601, #5370, #98588, #4883, #27181, #35765, #89051, #29171, #67156, #59033, #90004, #58068, #75780, #13478, #20085, #98077, #91005, #44349, #81411, #60039, #73778, #28655, #20579, #43851, #21567, #90517, #82426, #68149, #74792, #50461, #11984, #44843 ),
 .UNSPECIFIED., .F., .F.,
 ( 4, 2, 2, 2, 2, 2, 2, 2, 2, 2, 2, 2, 2, 2, 2, 2, 2, 2, 2, 2, 2, 2, 2, 2, 4 ),
 ( 0.0005508003809566546210, 0.0009892564418127341736, 0.001208484472240721041, 0.001318098487454664276, 0.001427712502668604042, 0.001537326517882543807, 0.001646940533096483356, 0.001866168563524404521, 0.002304624624380174208, 0.003181536746091786876, 0.004058448867803400410, 0.004935360989515013945, 0.005373817050370783416, 0.005593045080798705014, 0.005702659096012628950, 0.005757466103619628649, 0.005812273111226628347, 0.005867080118833628913, 0.005921887126440628611, 0.006031501141654588109, 0.006250729172082574760, 0.006689185232938636531, 0.007127641293794699170, 0.007346869324222742199, 0.007566097354650785228 ),
 .UNSPECIFIED. ) ;
#9849=CARTESIAN_POINT ( 'NONE',  ( 174.6745456591689845, 289.9937384206305637, 6.288497583336834396 ) ) ;
#9850=CARTESIAN_POINT ( 'NONE',  ( 154.2853090730916676, 265.4170011543745886, 17.16471700533586642 ) ) ;
#9852=CARTESIAN_POINT ( 'NONE',  ( 169.6445766797212116, 289.2987616194045017, 1.143403053474568054 ) ) ;
#9854=CARTESIAN_POINT ( 'NONE',  ( 191.3122624219907664, 298.1811694523752863, -9.332778507267013524 ) ) ;
#9855=CARTESIAN_POINT ( 'NONE',  ( 198.0006249058153003, 287.6998530631771587, 18.31850453277666801 ) ) ;
#9856=ORIENTED_EDGE ( 'NONE', *, *, #72713, .T. ) ;
#9857=ORIENTED_EDGE ( 'NONE', *, *, #47408, .T. ) ;
#9858=CARTESIAN_POINT ( 'NONE',  ( 147.4604237891675780, 275.2380492219603525, -3.488979611022138716 ) ) ;
#9859=CARTESIAN_POINT ( 'NONE',  ( 168.3813732014777145, 257.2211975074816905, -14.37470435435323424 ) ) ;
#9860=CARTESIAN_POINT ( 'NONE',  ( 159.2186641046529303, 254.8721795879351646, -15.96198087403305443 ) ) ;
#9862=CARTESIAN_POINT ( 'NONE',  ( 200.7079229450794173, 283.0106753079404029, 16.90512463913211505 ) ) ;
#9864=VERTEX_POINT ( 'NONE', #30189 ) ;
#9865=DIRECTION ( 'NONE',  ( 0.4999999999999998890, -0.8660254037844385966, 0.000000000000000000 ) ) ;
#9868=FACE_OUTER_BOUND ( 'NONE', #5921, .T. ) ;
#9870=CARTESIAN_POINT ( 'NONE',  ( 10.82940026203495520, 190.3927522451419634, 2.944929066748280225E-16 ) ) ;
#9871=CARTESIAN_POINT ( 'NONE',  ( 80.33678646758374953, 223.3149278399160664, -9.188101187500095079 ) ) ;
#9874=CARTESIAN_POINT ( 'NONE',  ( 208.0148989748639394, 270.3546215746652592, 3.138818306258006618 ) ) ;
#9875=CARTESIAN_POINT ( 'NONE',  ( 0.6624493194153854292, 177.3149278399160664, 9.188101187500093303 ) ) ;
#9876=FACE_OUTER_BOUND ( 'NONE', #63988, .T. ) ;
#9877=CARTESIAN_POINT ( 'NONE',  ( 178.7600897929267774, 254.1784503161647706, 4.743017227330367014 ) ) ;
#9881=CARTESIAN_POINT ( 'NONE',  ( 200.9077156035369001, 267.7919832835530656, -3.066172851167955127 ) ) ;
#9887=CARTESIAN_POINT ( 'NONE',  ( 30.62142885764206568, 197.6744531367911293, 4.594050593750047540 ) ) ;
#9888=CARTESIAN_POINT ( 'NONE',  ( 92.14326550588401687, 235.5530062829863027, -4.648177544792955347E-16 ) ) ;
#9891=CARTESIAN_POINT ( 'NONE',  ( 168.1589593212097498, 275.9390298053305628, -16.40258036402506647 ) ) ;
#9893=CARTESIAN_POINT ( 'NONE',  ( -12.86919761471646773, 169.5024278399161233, -9.188101187500093303 ) ) ;
#9896=CARTESIAN_POINT ( 'NONE',  ( 147.9133274879049793, 274.4535970048112290, -9.359166267164972908 ) ) ;
#9898=CARTESIAN_POINT ( 'NONE',  ( 204.5831314780710954, 276.2986172388744421, 13.28075685133257089 ) ) ;
#9899=CARTESIAN_POINT ( 'NONE',  ( 191.7741832257749195, 298.4843664033717801, -8.615487418695501276 ) ) ;
#9900=CARTESIAN_POINT ( 'NONE',  ( 190.5444288681022442, 300.6143634316900943, -1.000014190476072873 ) ) ;
#9901=EDGE_LOOP ( 'NONE', ( #30638, #98275, #41587, #40548 ) ) ;
#9902=CARTESIAN_POINT ( 'NONE',  ( 163.9910908123517288, 246.6060940548019289, -7.333295033952830444 ) ) ;
#9903=CARTESIAN_POINT ( 'NONE',  ( 135.1739027599712131, 260.3967562850347122, -4.648177544792955347E-16 ) ) ;
#9904=CARTESIAN_POINT ( 'NONE',  ( 118.4422513298640638, 233.0643266524159856, 9.188101187500095079 ) ) ;
#9908=CARTESIAN_POINT ( 'NONE',  ( 157.6335212189247557, 257.6177276032722716, 16.76495363836117036 ) ) ;
#9910=CARTESIAN_POINT ( 'NONE',  ( 191.2176660212971626, 299.4482824768133469, -7.870254471783424854 ) ) ;
#9912=CARTESIAN_POINT ( 'NONE',  ( 196.2878005184348353, 290.6665519265632724, -16.69183432842427806 ) ) ;
#9914=CARTESIAN_POINT ( 'NONE',  ( 173.3685877188761424, 289.8321177535186735, -1.072859328093765052 ) ) ;
#9917=CARTESIAN_POINT ( 'NONE',  ( 188.9872881452310196, 265.7805097164244330, 11.31253184319408156 ) ) ;
#9919=CARTESIAN_POINT ( 'NONE',  ( 168.8883095508243457, 271.9124168116484270, -17.04002696021108676 ) ) ;
#9921=CARTESIAN_POINT ( 'NONE',  ( 185.2570508126727873, 282.0811717828997303, -17.42469797758589678 ) ) ;
#9925=CARTESIAN_POINT ( 'NONE',  ( 192.6773196027083372, 296.9200883123592689, 11.15745042875121484 ) ) ;
#9927=FACE_OUTER_BOUND ( 'NONE', #34276, .T. ) ;
#9929=CARTESIAN_POINT ( 'NONE',  ( 173.7927290169602372, 272.7279150489933386, -16.36119466774314191 ) ) ;
#9930=ORIENTED_EDGE ( 'NONE', *, *, #23524, .T. ) ;
#9931=CARTESIAN_POINT ( 'NONE',  ( 163.7939465169801281, 279.4726423028532167, 12.28070329374801517 ) ) ;
#9936=CARTESIAN_POINT ( 'NONE',  ( 188.1760652356224739, 292.9042221405367741, 12.45412430059673170 ) ) ;
#9939=CARTESIAN_POINT ( 'NONE',  ( 202.8874463667715133, 279.2356300052831557, -15.29930322226033468 ) ) ;
#9942=EDGE_CURVE ( 'NONE', #59130, #95735, #36804, .T. ) ;
#9943=CARTESIAN_POINT ( 'NONE',  ( 175.0547837195394152, 258.6252918682578752, 12.74266989511996151 ) ) ;
#9944=ORIENTED_EDGE ( 'NONE', *, *, #80337, .F. ) ;
#9948=CYLINDRICAL_SURFACE ( 'NONE', #29810, 10.00000000000010658 ) ;
#9951=ORIENTED_EDGE ( 'NONE', *, *, #34755, .F. ) ;
#9952=CARTESIAN_POINT ( 'NONE',  ( 185.9234121912444948, 282.2675293692463470, -16.62240104205559632 ) ) ;
#9955=CARTESIAN_POINT ( 'NONE',  ( 196.0802517080272764, 284.4438967393610938, -17.76628030232408761 ) ) ;
#9956=CARTESIAN_POINT ( 'NONE',  ( 146.9422184197532317, 276.1356072505412840, -5.063317562214876943 ) ) ;
#9957=CARTESIAN_POINT ( 'NONE',  ( 201.1679199471075492, 282.2139371290980989, -16.62385308864941535 ) ) ;
#9959=CARTESIAN_POINT ( 'NONE',  ( 157.9535068807132348, 281.0419050908307099, 2.461037685683107323 ) ) ;
#9961=CARTESIAN_POINT ( 'NONE',  ( 125.9117204375048544, 237.3768266524159856, 9.188101187500098632 ) ) ;
#9965=ORIENTED_EDGE ( 'NONE', *, *, #66203, .F. ) ;
#9966=CARTESIAN_POINT ( 'NONE',  ( 203.5888783976779735, 276.1984687194538424, 13.33151786231322156 ) ) ;
#9967=CARTESIAN_POINT ( 'NONE',  ( 172.5942616442810333, 282.2509914604344203, 14.60726632573390305 ) ) ;
#9968=CARTESIAN_POINT ( 'NONE',  ( 173.1155682512793419, 289.1052356982697233, -4.667333446098393068 ) ) ;
#9969=CARTESIAN_POINT ( 'NONE',  ( 146.7466845547833429, 276.4742818392692243, 3.855766036253278184 ) ) ;
#9973=( BOUNDED_CURVE ( )  B_SPLINE_CURVE ( 2, ( #34232, #49425, #17018, #79876, #71751, #71247, #65620, #10948, #41818 ),
 .UNSPECIFIED., .F., .T. ) 
 B_SPLINE_CURVE_WITH_KNOTS ( ( 3, 2, 2, 2, 3 ),
 ( 0.6975806451612903691, 0.6989247311827957443, 0.7016129032258064946, 0.7043010752688172449, 0.7056451612903226200 ),
 .UNSPECIFIED. ) 
 CURVE ( )  GEOMETRIC_REPRESENTATION_ITEM ( )  RATIONAL_B_SPLINE_CURVE ( ( 0.9330127018922194093, 0.9330127018922194093, 1.000000000000000000, 0.8660254037844387076, 1.000000000000000000, 0.8660254037844387076, 1.000000000000000000, 0.9330127018922194093, 0.9330127018922194093 ) ) 
 REPRESENTATION_ITEM ( '' )  );
#9974=CARTESIAN_POINT ( 'NONE',  ( 9.911560002841389050, 164.9824982072973967, 3.021315404115420679E-15 ) ) ;
#9976=CARTESIAN_POINT ( 'NONE',  ( 177.1886485508865974, 256.0379014559142092, -7.297321842872941389 ) ) ;
#9979=CARTESIAN_POINT ( 'NONE',  ( 196.3249884498792994, 275.2518087180711177, 16.06659936265807431 ) ) ;
#9982=CARTESIAN_POINT ( 'NONE',  ( 157.6514191749160716, 276.9937859392390465, 10.24612596229098038 ) ) ;
#9983=CARTESIAN_POINT ( 'NONE',  ( 151.8090328414793930, 267.7060374011022077, -15.68750330915316660 ) ) ;
#9984=CARTESIAN_POINT ( 'NONE',  ( 149.1856130393175306, 272.2499337880290682, 11.44243872309708188 ) ) ;
#9985=CARTESIAN_POINT ( 'NONE',  ( 163.3543347837650686, 247.7089878483399730, 10.92686688779373405 ) ) ;
#9986=CARTESIAN_POINT ( 'NONE',  ( 153.3527095124072162, 270.2041312749430517, 14.05198471302335328 ) ) ;
#9987=CARTESIAN_POINT ( 'NONE',  ( 151.6065062536777646, 275.0711347837637959, -8.632019726508788793 ) ) ;
#9988=CARTESIAN_POINT ( 'NONE',  ( 199.9757505641556747, 267.6639986697646805, 6.164811578842619433 ) ) ;
#9989=ORIENTED_EDGE ( 'NONE', *, *, #46060, .T. ) ;
#9990=CARTESIAN_POINT ( 'NONE',  ( 164.4821770989429695, 280.3560663856659971, -11.24245345476798086 ) ) ;
#9993=CARTESIAN_POINT ( 'NONE',  ( 76.50299338235490154, 221.6427522451419065, 10.00000000000009415 ) ) ;
#9997=CARTESIAN_POINT ( 'NONE',  ( -4.099453989059914427, 156.8932355074535963, -2.679491924311252493 ) ) ;
#9999=CARTESIAN_POINT ( 'NONE',  ( -5.778093977583854013, 155.2202760586659451, -5.415160957724236172E-17 ) ) ;
#10000=CARTESIAN_POINT ( 'NONE',  ( 91.86592320334659689, 223.8458772461660544, 9.188101187500095079 ) ) ;
#10002=CARTESIAN_POINT ( 'NONE',  ( 147.7395812515338491, 275.4447818272566337, 3.760927250875937489 ) ) ;
#10003=DIRECTION ( 'NONE',  ( -0.8660254037844387076, -0.4999999999999998890, -0.000000000000000000 ) ) ;
#10005=CYLINDRICAL_SURFACE ( 'NONE', #94275, 10.00000000000010658 ) ;
#10006=CARTESIAN_POINT ( 'NONE',  ( 164.2057239597426985, 284.2837641608711579, 5.838786750481579801 ) ) ;
#10008=CARTESIAN_POINT ( 'NONE',  ( 162.9111474110223412, 248.4766108952035211, -9.702990628959184960 ) ) ;
#10009=CARTESIAN_POINT ( 'NONE',  ( 161.8690507138996395, 250.2815753210195737, 12.79467889464216945 ) ) ;
#10010=CARTESIAN_POINT ( 'NONE',  ( 166.1309782654906257, 249.2029336093187339, -9.347746458946922132 ) ) ;
#10012=DIRECTION ( 'NONE',  ( -0.8660254037844387076, -0.4999999999999998890, -0.000000000000000000 ) ) ;
#10015=CARTESIAN_POINT ( 'NONE',  ( 33.21950506899538880, 199.1744531367911293, 4.594050593750047540 ) ) ;
#10018=CARTESIAN_POINT ( 'NONE',  ( 60.74296170696083408, 212.0024278399160949, 9.188101187500095079 ) ) ;
#10019=CARTESIAN_POINT ( 'NONE',  ( 161.2488013048736377, 251.3558788108169040, -13.10044423494716170 ) ) ;
#10021=CARTESIAN_POINT ( 'NONE',  ( 165.5574043327790150, 259.0627220984302426, 15.59678351321189638 ) ) ;
#10022=CARTESIAN_POINT ( 'NONE',  ( 198.7246006328481087, 286.0324930241461630, -17.02257870953173224 ) ) ;
#10023=CARTESIAN_POINT ( 'NONE',  ( 151.7165138354984038, 267.8662850201268952, 16.09268003789171431 ) ) ;
#10024=CARTESIAN_POINT ( 'NONE',  ( 173.9772233185703669, 268.6891927935771491, -16.30485447805711274 ) ) ;
#10027=CARTESIAN_POINT ( 'NONE',  ( 149.0598351764325002, 272.4677874370131576, -11.59078276432863674 ) ) ;
#10030=CARTESIAN_POINT ( 'NONE',  ( 79.63366147065640632, 204.5327760586659451, 1.948934522072302763E-15 ) ) ;
#10032=CARTESIAN_POINT ( 'NONE',  ( 169.6880240292687176, 288.1769740498922374, -1.088266952603743842 ) ) ;
#10033=CARTESIAN_POINT ( 'NONE',  ( 187.1412927779018673, 261.9835105880691231, -10.20549468610707322 ) ) ;
#10034=CARTESIAN_POINT ( 'NONE',  ( 153.6752087927504533, 264.4737258376377440, 16.52473746413441091 ) ) ;
#10035=ORIENTED_EDGE ( 'NONE', *, *, #72159, .F. ) ;
#10038=CARTESIAN_POINT ( 'NONE',  ( 118.8119427999550624, 252.7365022471903444, 2.944929066748280225E-16 ) ) ;
#10039=CARTESIAN_POINT ( 'NONE',  ( 161.8948331661419218, 250.2369188037922356, 13.64419044796309777 ) ) ;
#10041=ORIENTED_EDGE ( 'NONE', *, *, #22958, .F. ) ;
#10042=CARTESIAN_POINT ( 'NONE',  ( 187.7720937987822083, 273.1901695715338292, 15.64266941918570097 ) ) ;
#10044=CARTESIAN_POINT ( 'NONE',  ( 163.0309151244508712, 248.2691671304387739, 11.27270415168660200 ) ) ;
#10047=VERTEX_POINT ( 'NONE', #5408 ) ;
#10048=CARTESIAN_POINT ( 'NONE',  ( 177.2167214159767070, 253.2638437126931592, -0.2615130296398746612 ) ) ;
#10049=ORIENTED_EDGE ( 'NONE', *, *, #20714, .T. ) ;
#10051=CARTESIAN_POINT ( 'NONE',  ( 167.5688045394477967, 247.4305784569795605, 3.634624977922704669 ) ) ;
#10058=CARTESIAN_POINT ( 'NONE',  ( 163.1218343930725894, 256.2508100442478849, -16.13596270478102923 ) ) ;
#10059=DIRECTION ( 'NONE',  ( 0.4999999999999992784, -0.8660254037844390407, 0.000000000000000000 ) ) ;
#10060=ORIENTED_EDGE ( 'NONE', *, *, #52016, .F. ) ;
#10062=CARTESIAN_POINT ( 'NONE',  ( 183.1143161927901133, 295.7630023993714872, 0.8723711145391563893 ) ) ;
#10063=CARTESIAN_POINT ( 'NONE',  ( 163.0627400685409327, 284.1756707159956932, -2.513755478446318747 ) ) ;
#10066=CARTESIAN_POINT ( 'NONE',  ( 194.4165969972361552, 293.9075714965812267, 14.23342188338008718 ) ) ;
#10069=CARTESIAN_POINT ( 'NONE',  ( 164.7591420166619400, 245.2757903461224203, 4.883783760312801370 ) ) ;
#10070=ADVANCED_FACE ( 'NONE', ( #38778 ), #288, .T. ) ;
#10073=CARTESIAN_POINT ( 'NONE',  ( 85.20852645963621796, 213.8768266524159856, -9.188101187500091527 ) ) ;
#10075=CARTESIAN_POINT ( 'NONE',  ( 191.0170959869219303, 299.7956799668270946, 7.353346939903929069 ) ) ;
#10079=CARTESIAN_POINT ( 'NONE',  ( 167.6704087901883895, 266.8335129934314978, -16.83350944486469913 ) ) ;
#10080=ORIENTED_EDGE ( 'NONE', *, *, #55972, .F. ) ;
#10083=CARTESIAN_POINT ( 'NONE',  ( -13.03140383004354241, 163.2833772461660544, -9.188101187500095079 ) ) ;
#10084=B_SPLINE_SURFACE_WITH_KNOTS ( 'NONE', 3, 1, ( 
 ( #84621, #91219 ),
 ( #6088, #14687 ),
 ( #69381, #99798 ),
 ( #14194, #45569 ),
 ( #68379, #83630 ),
 ( #45079, #23771 ),
 ( #38968, #4213 ),
 ( #29883, #30885 ),
 ( #76498, #30384 ),
 ( #77501, #98815 ),
 ( #85119, #60757 ),
 ( #36981, #7076 ),
 ( #46061, #61269 ),
 ( #92239, #67893 ),
 ( #29394, #22788 ),
 ( #15164, #92718 ),
 ( #8094, #61771 ),
 ( #23267, #54158 ),
 ( #69874, #487 ),
 ( #31374, #62258 ),
 ( #54662, #63780 ),
 ( #94223, #79015 ),
 ( #39958, #986 ),
 ( #33381, #40955 ),
 ( #41464, #63280 ),
 ( #47573, #8590 ),
 ( #24775, #26290 ),
 ( #1990, #79531 ),
 ( #64285, #85637 ),
 ( #16185, #62768 ),
 ( #78502, #71401 ),
 ( #93726, #9086 ),
 ( #47078, #80022 ),
 ( #87159, #24287 ) ),
 .UNSPECIFIED., .T., .F., .F.,
 ( 4, 2, 2, 2, 2, 2, 2, 2, 2, 2, 2, 2, 2, 2, 2, 2, 4 ),
 ( 2, 2 ),
 ( 0.000000000000000000, 0.06250000000000000000, 0.1250000000000000000, 0.1875000000000000000, 0.2500000000000000000, 0.3125000000000000000, 0.3750000000000000000, 0.4375000000000000000, 0.5000000000000000000, 0.5625000000000000000, 0.6250000000000000000, 0.6875000000000000000, 0.7500000000000000000, 0.8125000000000000000, 0.8750000000000000000, 0.9375000000000000000, 1.000000000000000000 ),
 ( 0.000000000000000000, 1.000000000000000000 ),
 .UNSPECIFIED. ) ;
#10087=CARTESIAN_POINT ( 'NONE',  ( 208.0148989748639394, 270.3546215746652592, 3.138818306258006618 ) ) ;
#10088=CARTESIAN_POINT ( 'NONE',  ( 90.72943840876202160, 217.0643266524159571, -9.188101187500093303 ) ) ;
#10096=CARTESIAN_POINT ( 'NONE',  ( -4.903394573382245269, 154.6427522451417644, 1.119607411625061291E-15 ) ) ;
#10099=CARTESIAN_POINT ( 'NONE',  ( 156.9652392049574132, 258.7752260052484985, 18.40175728539550448 ) ) ;
#10100=CARTESIAN_POINT ( 'NONE',  ( 160.0124400273076333, 275.3606515527212650, 12.84424831609223716 ) ) ;
#10102=CARTESIAN_POINT ( 'NONE',  ( 189.0767002963758330, 269.5454149288324857, 14.97099974568435066 ) ) ;
#10103=CARTESIAN_POINT ( 'NONE',  ( 175.4995246435592833, 283.9138537061506327, 13.23358799048017076 ) ) ;
#10105=CARTESIAN_POINT ( 'NONE',  ( 163.8070446421170629, 255.0663642890118581, -15.42060242571707818 ) ) ;
#10106=ORIENTED_EDGE ( 'NONE', *, *, #51770, .F. ) ;
#10107=CARTESIAN_POINT ( 'NONE',  ( 200.4116241316243645, 283.5238799070667142, 18.37703770054986663 ) ) ;
#10109=CARTESIAN_POINT ( 'NONE',  ( 168.2952158864145531, 250.3176572863741285, 6.948728081753761110 ) ) ;
#10111=CARTESIAN_POINT ( 'NONE',  ( 178.7002874096667426, 291.6869041091368899, -6.125093610568141500 ) ) ;
#10112=CARTESIAN_POINT ( 'NONE',  ( 202.7367043553907990, 279.4967228278296716, -16.72422094393309777 ) ) ;
#10116=CARTESIAN_POINT ( 'NONE',  ( 206.9258336080761183, 272.2409381227055292, 6.776000910836894597 ) ) ;
#10117=CARTESIAN_POINT ( 'NONE',  ( 181.9374065758725862, 264.0954804722510971, 13.73142499530935723 ) ) ;
#10121=CARTESIAN_POINT ( 'NONE',  ( 152.8522706834672533, 265.8990964544007056, 17.63080661522264947 ) ) ;
#10122=CARTESIAN_POINT ( 'NONE',  ( 171.8837275538034532, 274.9715841211527163, 17.02018998718227749 ) ) ;
#10125=CARTESIAN_POINT ( 'NONE',  ( 188.4962938548358409, 260.9679252005893773, 2.869700643444213828 ) ) ;
#10127=CARTESIAN_POINT ( 'NONE',  ( 3.856091543753019213, 173.0333772461660828, 9.188101187500095079 ) ) ;
#10129=ORIENTED_EDGE ( 'NONE', *, *, #58254, .T. ) ;
#10131=CARTESIAN_POINT ( 'NONE',  ( 178.8388798781788296, 256.8338936803557431, 8.575590808577006285 ) ) ;
#10132=B_SPLINE_CURVE_WITH_KNOTS ( 'NONE', 3,
 ( #56395, #71120, #87390, #63999 ),
 .UNSPECIFIED., .F., .F.,
 ( 4, 4 ),
 ( 0.009125246467023215291, 0.01512799987379969541 ),
 .UNSPECIFIED. ) ;
#10135=CARTESIAN_POINT ( 'NONE',  ( 26.15589859543730000, 198.1589784336661353, -6.496448406907676862E-16 ) ) ;
#10138=CARTESIAN_POINT ( 'NONE',  ( 161.1238074876215478, 251.5723744529297505, 13.42537408252843179 ) ) ;
#10141=CARTESIAN_POINT ( 'NONE',  ( 181.5900847557695670, 293.9353123765011446, 6.270096989977908208 ) ) ;
#10142=CARTESIAN_POINT ( 'NONE',  ( 173.2748909899069076, 273.4713738435106620, -17.11406341994456781 ) ) ;
#10143=CARTESIAN_POINT ( 'NONE',  ( 149.7132193248854435, 271.3360928950326638, 12.70265921103533380 ) ) ;
#10146=CARTESIAN_POINT ( 'NONE',  ( 190.0660857974371822, 298.8038670201426044, -8.153583364850311099 ) ) ;
#10151=CARTESIAN_POINT ( 'NONE',  ( 77.09838585100465025, 221.9865022471902876, -10.00000000000009415 ) ) ;
#10153=CARTESIAN_POINT ( 'NONE',  ( 203.3655854462036530, 270.0990294040706772, 6.133038700129080922 ) ) ;
#10154=CARTESIAN_POINT ( 'NONE',  ( 43.28705038798948124, 204.9869531367911293, 4.594050593750046652 ) ) ;
#10155=CARTESIAN_POINT ( 'NONE',  ( 159.4574711498080433, 254.4585536525209477, 16.86100557095418395 ) ) ;
#10156=ORIENTED_EDGE ( 'NONE', *, *, #36707, .T. ) ;
#10158=CARTESIAN_POINT ( 'NONE',  ( 190.1752790837055045, 301.2537496138681945, -5.177773110520776711 ) ) ;
#10162=CARTESIAN_POINT ( 'NONE',  ( 156.6812872898450735, 261.2670451491295012, 0.000000000000000000 ) ) ;
#10163=CARTESIAN_POINT ( 'NONE',  ( 159.5180972751518595, 279.0588588540967976, -11.03979334413982016 ) ) ;
#10164=CARTESIAN_POINT ( 'NONE',  ( 203.1858896750085535, 273.4118621242805602, 12.47033584857523003 ) ) ;
#10166=CARTESIAN_POINT ( 'NONE',  ( 203.0507839702407580, 278.9527209772879814, 16.21318481136342626 ) ) ;
#10168=CARTESIAN_POINT ( 'NONE',  ( 171.4451181911705930, 255.5540518477252760, 12.38484697617079178 ) ) ;
#10172=CARTESIAN_POINT ( 'NONE',  ( 171.6833113595534712, 252.4132807094040061, 8.718741680673185002 ) ) ;
#10182=ADVANCED_FACE ( 'NONE', ( #32684 ), #24581, .T. ) ;
#10183=CARTESIAN_POINT ( 'NONE',  ( 189.4877677241300944, 274.7371391580670092, -16.41815265926193845 ) ) ;
#10185=ORIENTED_EDGE ( 'NONE', *, *, #68824, .F. ) ;
#10186=CARTESIAN_POINT ( 'NONE',  ( 152.8721808860877616, 265.8646109718731623, -17.65676496037632504 ) ) ;
#10190=CARTESIAN_POINT ( 'NONE',  ( 205.2660270307054304, 275.1158074454486382, -13.97598661256119179 ) ) ;
#10192=CARTESIAN_POINT ( 'NONE',  ( 110.3772162092389948, 234.5333772461660828, 9.188101187500095079 ) ) ;
#10193=EDGE_CURVE ( 'NONE', #91972, #8803, #5798, .T. ) ;
#10194=CARTESIAN_POINT ( 'NONE',  ( 181.0943051178491885, 287.1835064078692312, -13.38063930454047323 ) ) ;
#10196=CARTESIAN_POINT ( 'NONE',  ( 164.4698008747318738, 245.7769439046653019, -6.272955660526681854 ) ) ;
#10197=EDGE_LOOP ( 'NONE', ( #29543, #15514, #73978, #5112 ) ) ;
#10200=CARTESIAN_POINT ( 'NONE',  ( 157.3467993828755880, 258.5604024866626673, 16.83275751048395108 ) ) ;
#10202=EDGE_CURVE ( 'NONE', #32950, #66029, #9634, .T. ) ;
#10203=CARTESIAN_POINT ( 'NONE',  ( 60.74296170696083408, 212.0024278399160949, 9.188101187500095079 ) ) ;
#10205=CARTESIAN_POINT ( 'NONE',  ( 191.3375250863502970, 299.2406804863936145, 8.828791580707859410 ) ) ;
#10207=CARTESIAN_POINT ( 'NONE',  ( 173.8797520427797849, 271.6693953237884784, 16.43749877907051982 ) ) ;
#10208=ORIENTED_EDGE ( 'NONE', *, *, #66550, .T. ) ;
#10210=CARTESIAN_POINT ( 'NONE',  ( 177.9856817937294124, 288.6971931234167528, 10.88127348114070259 ) ) ;
#10213=CARTESIAN_POINT ( 'NONE',  ( 175.4379314651181119, 261.1390654822758393, -14.58016465811829576 ) ) ;
#10214=CARTESIAN_POINT ( 'NONE',  ( 174.2802897980567138, 277.2551486598794099, -15.61713791557879993 ) ) ;
#10215=CARTESIAN_POINT ( 'NONE',  ( 161.4143265314674522, 251.0691807084224365, -12.94469757303959234 ) ) ;
#10216=CARTESIAN_POINT ( 'NONE',  ( 206.9349434189263661, 269.8064106017384916, 1.784245431258210113 ) ) ;
#10217=CARTESIAN_POINT ( 'NONE',  ( 149.6676065383367416, 271.4150965588098074, 11.80358707172367261 ) ) ;
#10218=CARTESIAN_POINT ( 'NONE',  ( 177.2917107194376740, 269.5050067700457816, 16.10103962328780369 ) ) ;
#10219=CARTESIAN_POINT ( 'NONE',  ( 206.3505875407052486, 273.2372935382459787, 11.62318091048137880 ) ) ;
#10221=CARTESIAN_POINT ( 'NONE',  ( 167.8085051679049116, 256.1148727468539619, 13.55799742952848419 ) ) ;
#10223=CARTESIAN_POINT ( 'NONE',  ( 120.4179585561885659, 231.1423013555409796, -4.594050593750043987 ) ) ;
#10225=CARTESIAN_POINT ( 'NONE',  ( 191.8453338867844877, 298.3611298435110371, -9.039024722281077118 ) ) ;
#10227=FACE_OUTER_BOUND ( 'NONE', #36232, .T. ) ;
#10230=CARTESIAN_POINT ( 'NONE',  ( 174.7959030193343608, 252.7028669189593870, 5.110487748453643064 ) ) ;
#10233=CARTESIAN_POINT ( 'NONE',  ( 155.4293395016508725, 273.5175306886564499, -12.86640682340763320 ) ) ;
#10235=CARTESIAN_POINT ( 'NONE',  ( 185.9187572292423170, 261.7931673995647657, 10.04575878863954941 ) ) ;
#10237=CARTESIAN_POINT ( 'NONE',  ( 133.7867050834633460, 257.2369531367911009, -4.594050593750048428 ) ) ;
#10238=CARTESIAN_POINT ( 'NONE',  ( 189.7697392812929138, 294.5961115088648512, -12.48438950990594698 ) ) ;
#10239=VECTOR ( 'NONE', #45877, 1000.000000000000000 ) ;
#10242=CARTESIAN_POINT ( 'NONE',  ( 62.15025298811053034, 212.8149278399160949, -9.188101187500095079 ) ) ;
#10243=CARTESIAN_POINT ( 'NONE',  ( 207.6477529416552557, 270.9905371579805546, 7.447146952410988341 ) ) ;
#10244=CARTESIAN_POINT ( 'NONE',  ( 193.6967711697749905, 268.4383357953667542, 12.84685063220190671 ) ) ;
#10246=CARTESIAN_POINT ( 'NONE',  ( 173.4606779374792325, 267.5814416807811540, -17.58000433512257032 ) ) ;
#10247=CARTESIAN_POINT ( 'NONE',  ( 155.3426119516925610, 279.6488991376975264, -1.568138233356304534 ) ) ;
#10249=CARTESIAN_POINT ( 'NONE',  ( 203.3205561747472814, 278.4854618126124706, -15.14439614831292147 ) ) ;
#10250=CARTESIAN_POINT ( 'NONE',  ( 193.0673971409008232, 289.3950934321782142, 16.62649702710665522 ) ) ;
#10252=CARTESIAN_POINT ( 'NONE',  ( 125.1447535615809414, 236.3927522451417929, -10.00000000000009059 ) ) ;
#10255=EDGE_CURVE ( 'NONE', #76205, #76868, #56176, .T. ) ;
#10256=CARTESIAN_POINT ( 'NONE',  ( 65.02584505343169496, 219.8967562850346837, -4.648177544792955347E-16 ) ) ;
#10257=CARTESIAN_POINT ( 'NONE',  ( -18.01139699756907930, 172.6589784336661353, -6.496448406907676862E-16 ) ) ;
#10258=CARTESIAN_POINT ( 'NONE',  ( 38.41565749170202082, 202.1744531367911293, 4.594050593750047540 ) ) ;
#10262=CARTESIAN_POINT ( 'NONE',  ( 147.4368675721658519, 275.2788497866417288, 5.050119523016719292 ) ) ;
#10264=CARTESIAN_POINT ( 'NONE',  ( 171.6654525870716554, 267.7842514992769907, 17.73500564707179095 ) ) ;
#10265=CARTESIAN_POINT ( 'NONE',  ( 59.25465409031482977, 215.0177522451419065, 5.000000000000046185 ) ) ;
#10266=DIRECTION ( 'NONE',  ( -0.8660254037844387076, -0.4999999999999998890, -0.000000000000000000 ) ) ;
#10267=CARTESIAN_POINT ( 'NONE',  ( 180.8260447606230912, 256.2909217566163989, 1.374377561445572438 ) ) ;
#10269=CARTESIAN_POINT ( 'NONE',  ( 157.6668627405778409, 257.5599783937680058, -16.78811156090270629 ) ) ;
#10270=CARTESIAN_POINT ( 'NONE',  ( 162.1264656378374696, 252.0740353423958595, -13.51783732343398903 ) ) ;
#10272=CARTESIAN_POINT ( 'NONE',  ( 44.69460199273694911, 186.6115022471902023, -5.000000000000041744 ) ) ;
#10273=CARTESIAN_POINT ( 'NONE',  ( 149.2944063396847412, 250.8768266524159856, 9.188101187500098632 ) ) ;
#10274=CARTESIAN_POINT ( 'NONE',  ( 162.6774150396764469, 248.8814472377480911, 10.88033986792731689 ) ) ;
#10275=CARTESIAN_POINT ( 'NONE',  ( 3.531332017333847606, 172.8458772461660828, 9.188101187500095079 ) ) ;
#10278=CARTESIAN_POINT ( 'NONE',  ( 170.3916841401598958, 263.6555044952191906, 15.81889653756881131 ) ) ;
#10279=CARTESIAN_POINT ( 'NONE',  ( 192.7259387352017939, 296.8358775046606297, 11.24705370801146209 ) ) ;
#10281=CARTESIAN_POINT ( 'NONE',  ( 165.0087721269838710, 244.8434183119457543, 2.604344609212914108 ) ) ;
#10282=CARTESIAN_POINT ( 'NONE',  ( 186.8350843013657823, 259.3184771713918053, -2.377127750769511660 ) ) ;
#10284=CARTESIAN_POINT ( 'NONE',  ( 149.2223635749290622, 272.1862799931444670, -12.97307652490353647 ) ) ;
#10287=CARTESIAN_POINT ( 'NONE',  ( 165.7255960892794349, 285.4442248579660486, 0.4815049898957938779 ) ) ;
#10289=CARTESIAN_POINT ( 'NONE',  ( -13.76211276271272865, 162.8615022471902307, 0.000000000000000000 ) ) ;
#10291=CARTESIAN_POINT ( 'NONE',  ( 153.3433014850764096, 275.0156552373531440, 10.59304337032270915 ) ) ;
#10292=CARTESIAN_POINT ( 'NONE',  ( 206.8775514429320026, 272.3245652858344670, -9.838455694836268250 ) ) ;
#10294=CARTESIAN_POINT ( 'NONE',  ( 153.1745822862813498, 265.3408363824576668, 16.18092354043443493 ) ) ;
#10295=CARTESIAN_POINT ( 'NONE',  ( 164.6649740431187183, 245.4388940607451843, -1.430729255012818557 ) ) ;
#10298=CARTESIAN_POINT ( 'NONE',  ( 194.3562588153086779, 294.0120802933159325, 14.11474987148825200 ) ) ;
#10301=ADVANCED_FACE ( 'NONE', ( #11906 ), #18503, .T. ) ;
#10305=ORIENTED_EDGE ( 'NONE', *, *, #57742, .F. ) ;
#10315=ORIENTED_EDGE ( 'NONE', *, *, #97417, .T. ) ;
#10316=CARTESIAN_POINT ( 'NONE',  ( 161.5875797534026219, 250.7690973254556468, 12.95526170413129030 ) ) ;
#10317=CARTESIAN_POINT ( 'NONE',  ( 168.9356066370792462, 275.9063550870135373, -15.42059771712085059 ) ) ;
#10321=ORIENTED_EDGE ( 'NONE', *, *, #79862, .F. ) ;
#10323=CARTESIAN_POINT ( 'NONE',  ( 170.7128543530930926, 255.6187006993503985, -11.59851742352739912 ) ) ;
#10325=ORIENTED_EDGE ( 'NONE', *, *, #34755, .T. ) ;
#10329=CYLINDRICAL_SURFACE ( 'NONE', #50854, 10.00000000000010658 ) ;
#10330=ORIENTED_EDGE ( 'NONE', *, *, #13954, .F. ) ;
#10331=CARTESIAN_POINT ( 'NONE',  ( 159.2431593014864575, 259.5309889387258409, 16.68740487222246216 ) ) ;
#10332=CARTESIAN_POINT ( 'NONE',  ( 168.7305174143800741, 272.8130231889026049, 15.98073601715322845 ) ) ;
#10333=CARTESIAN_POINT ( 'NONE',  ( 147.6685936899311287, 274.8774883772312592, 5.860645049887598823 ) ) ;
#10334=CARTESIAN_POINT ( 'NONE',  ( 177.4997901991728781, 288.9581381731804299, -9.329869128273438506 ) ) ;
#10336=CARTESIAN_POINT ( 'NONE',  ( 192.7787710433387360, 295.2766471658688943, 13.34619424850646752 ) ) ;
#10340=CARTESIAN_POINT ( 'NONE',  ( 183.6498318386265396, 256.3252116762061519, 1.424693195823348635 ) ) ;
#10342=CARTESIAN_POINT ( 'NONE',  ( 164.4573439719129340, 245.7985198932525748, 1.541132361166968501 ) ) ;
#10343=CARTESIAN_POINT ( 'NONE',  ( 164.7762319088960794, 245.2461897844768828, 2.994040459560653122 ) ) ;
#10347=CYLINDRICAL_SURFACE ( 'NONE', #51380, 17.82106496071139645 ) ;
#10348=CARTESIAN_POINT ( 'NONE',  ( 171.5826572751710160, 259.5044536903516246, -13.90678447660475925 ) ) ;
#10349=FACE_OUTER_BOUND ( 'NONE', #24863, .T. ) ;
#10351=EDGE_CURVE ( 'NONE', #75738, #63237, #50381, .T. ) ;
#10352=CARTESIAN_POINT ( 'NONE',  ( 161.4726291907278721, 250.9681975403669867, 14.52346149734912117 ) ) ;
#10353=CARTESIAN_POINT ( 'NONE',  ( 191.1149281592727789, 262.1737860021522692, -0.7454788891368452353 ) ) ;
#10355=CARTESIAN_POINT ( 'NONE',  ( 179.9804556880129383, 273.2999562016793789, -17.78099266527076949 ) ) ;
#10357=CARTESIAN_POINT ( 'NONE',  ( 51.59680478827888805, 189.0494855054051868, -2.679491924311248496 ) ) ;
#10360=CARTESIAN_POINT ( 'NONE',  ( 18.47929132879751890, 188.1427522451419350, -10.00000000000009415 ) ) ;
#10361=CARTESIAN_POINT ( 'NONE',  ( 93.32716752435031538, 230.8149278399160949, -9.188101187500095079 ) ) ;
#10364=CARTESIAN_POINT ( 'NONE',  ( 162.6076392040105816, 249.0023025302617725, 11.70000256607044165 ) ) ;
#10365=CARTESIAN_POINT ( 'NONE',  ( 23.96437920969670898, 175.4548013555409796, -4.594050593750042211 ) ) ;
#10366=CARTESIAN_POINT ( 'NONE',  ( -5.122212653107841795, 179.3967562850347406, 2.649461200531984646E-14 ) ) ;
#10368=VERTEX_POINT ( 'NONE', #49888 ) ;
#10369=CARTESIAN_POINT ( 'NONE',  ( 200.9615411070818425, 267.7048942554176847, -3.403220809365973931 ) ) ;
#10372=CARTESIAN_POINT ( 'NONE',  ( 194.0465404961993556, 264.4183967981790602, -4.354813327397827116 ) ) ;
#10374=CARTESIAN_POINT ( 'NONE',  ( 161.2977680094314223, 251.2710659906439616, -13.03191437619249982 ) ) ;
#10375=CARTESIAN_POINT ( 'NONE',  ( 182.6041507127388002, 284.2934025591197269, 14.95852815553201864 ) ) ;
#10377=CARTESIAN_POINT ( 'NONE',  ( 25.42527643493543366, 194.6744531367911293, 4.594050593750047540 ) ) ;
#10378=CARTESIAN_POINT ( 'NONE',  ( 77.44118756978804186, 225.5177522451419350, 5.000000000000046185 ) ) ;
#10379=ORIENTED_EDGE ( 'NONE', *, *, #88321, .T. ) ;
#10381=VECTOR ( 'NONE', #76819, 1000.000000000000000 ) ;
#10383=CARTESIAN_POINT ( 'NONE',  ( 178.7980240951186488, 259.0421912297024392, -10.14286040655596288 ) ) ;
#10384=CARTESIAN_POINT ( 'NONE',  ( -10.94779052401099051, 173.6744531367911293, 4.594050593750047540 ) ) ;
#10386=CARTESIAN_POINT ( 'NONE',  ( 198.9225589249066957, 286.1030165008847916, -17.03502353404871883 ) ) ;
#10387=DIRECTION ( 'NONE',  ( 0.4999999999999992784, -0.8660254037844390407, 0.000000000000000000 ) ) ;
#10388=CARTESIAN_POINT ( 'NONE',  ( 147.5851099763508216, 275.0220864107570264, -4.372720440640867956 ) ) ;
#10389=CARTESIAN_POINT ( 'NONE',  ( -11.77978294824862893, 175.5530062829863311, 1.347971487989956912E-14 ) ) ;
#10390=CARTESIAN_POINT ( 'NONE',  ( 163.9149533033796047, 246.7379680887036670, 7.273005089308705706 ) ) ;
#10391=EDGE_CURVE ( 'NONE', #49538, #76828, #41647, .T. ) ;
#10392=CARTESIAN_POINT ( 'NONE',  ( 191.7187529716733820, 298.5803744197520473, -8.487597704798396592 ) ) ;
#10393=CARTESIAN_POINT ( 'NONE',  ( 206.9408877595175511, 272.2148635675444552, 6.707071080545934372 ) ) ;
#10395=CARTESIAN_POINT ( 'NONE',  ( 151.2701135660092007, 248.9548013555409796, -4.594050593750042211 ) ) ;
#10396=CARTESIAN_POINT ( 'NONE',  ( 7.752142999874299001, 186.8297689869269220, -2.679491924311252493 ) ) ;
#10397=CARTESIAN_POINT ( 'NONE',  ( 111.5140480995885497, 229.0643266524159856, -9.188101187500093303 ) ) ;
#10400=DIRECTION ( 'NONE',  ( -0.8660254037844387076, -0.4999999999999998890, -0.000000000000000000 ) ) ;
#10401=CARTESIAN_POINT ( 'NONE',  ( 180.3268137483904354, 258.1330830615356149, 10.30874540274224849 ) ) ;
#10402=CARTESIAN_POINT ( 'NONE',  ( 162.1596889173749787, 251.8569052447999184, -14.10774048472399222 ) ) ;
#10403=CARTESIAN_POINT ( 'NONE',  ( 191.3193808042797741, 299.2721073048064682, -6.832536527061075837 ) ) ;
#10405=CARTESIAN_POINT ( 'NONE',  ( 191.6416599777803071, 263.0665572907887508, -4.349148431717937413 ) ) ;
#10406=CARTESIAN_POINT ( 'NONE',  ( 196.2630260332681189, 290.7094625936034049, -17.43112004684450866 ) ) ;
#10407=CARTESIAN_POINT ( 'NONE',  ( 190.5500884410106153, 299.9961840195823015, 4.185962364582526796 ) ) ;
#10408=CARTESIAN_POINT ( 'NONE',  ( 173.2992799364793655, 289.7901017517768878, -1.077829072056774473 ) ) ;
#10410=ORIENTED_EDGE ( 'NONE', *, *, #10623, .T. ) ;
#10412=CARTESIAN_POINT ( 'NONE',  ( 176.4230820045180224, 279.0088413606695781, 15.48324227125391239 ) ) ;
#10413=CARTESIAN_POINT ( 'NONE',  ( 196.8708119716154954, 268.3476497963631573, -11.07389558091716708 ) ) ;
#10418=CARTESIAN_POINT ( 'NONE',  ( 148.5240811353718016, 275.0344138590257330, 7.425379614582615417 ) ) ;
#10420=CARTESIAN_POINT ( 'NONE',  ( 191.2272277623841035, 280.2561453075193754, 17.73953484063011388 ) ) ;
#10422=CARTESIAN_POINT ( 'NONE',  ( 173.8066869025494441, 272.5896278189234181, -16.38874741603444107 ) ) ;
#10425=CARTESIAN_POINT ( 'NONE',  ( 194.9819925439454664, 292.9282776833073285, -15.33279721168237586 ) ) ;
#10426=DIRECTION ( 'NONE',  ( 0.4999999999999998890, -0.8660254037844385966, 0.000000000000000000 ) ) ;
#10439=B_SPLINE_CURVE_WITH_KNOTS ( 'NONE', 3,
 ( #12330, #6709, #37587, #43194, #66513, #82763, #97439, #44192, #67501, #86258, #31487, #23890, #77622, #69989 ),
 .UNSPECIFIED., .F., .F.,
 ( 4, 2, 2, 2, 2, 2, 4 ),
 ( 0.0009839635007110013321, 0.001239636163184778313, 0.001495308825658555512, 0.001750981488132332493, 0.002006654150606109691, 0.002517999475553669292, 0.003029344800501229326 ),
 .UNSPECIFIED. ) ;
#10446=CARTESIAN_POINT ( 'NONE',  ( 189.9165526381299571, 301.7018769628665495, 2.876435567632701584 ) ) ;
#10448=CARTESIAN_POINT ( 'NONE',  ( 192.4743214706506365, 297.2716913909250707, -12.17804856100553046 ) ) ;
#10452=CARTESIAN_POINT ( 'NONE',  ( 153.8556153531656321, 279.8124448561599706, 2.207844972829135166 ) ) ;
#10453=CARTESIAN_POINT ( 'NONE',  ( 130.5662598870812019, 252.3149278399160664, 9.188101187500093303 ) ) ;
#10456=EDGE_CURVE ( 'NONE', #55671, #93478, #90434, .T. ) ;
#10457=ORIENTED_EDGE ( 'NONE', *, *, #81456, .T. ) ;
#10460=CARTESIAN_POINT ( 'NONE',  ( 203.5517807763935991, 276.4131063546051337, 14.32831804246049678 ) ) ;
#10461=CYLINDRICAL_SURFACE ( 'NONE', #5936, 17.82106496071139645 ) ;
#10463=CARTESIAN_POINT ( 'NONE',  ( 146.6727924462101669, 276.6022667255962801, 3.481050673020940511 ) ) ;
#10464=CARTESIAN_POINT ( 'NONE',  ( 153.4235286554718130, 276.8959503085853839, 7.157280695494672607 ) ) ;
#10465=CARTESIAN_POINT ( 'NONE',  ( 163.4927498574098763, 249.4692459082536686, 11.48939803020791750 ) ) ;
#10467=CARTESIAN_POINT ( 'NONE',  ( 171.1570684511148102, 280.6390554436904949, 13.86101101377389533 ) ) ;
#10469=CARTESIAN_POINT ( 'NONE',  ( 177.3728554691246018, 255.8828027512285530, -8.252538712637369045 ) ) ;
#10470=EDGE_LOOP ( 'NONE', ( #42659, #6542, #89818, #48063 ) ) ;
#10472=CARTESIAN_POINT ( 'NONE',  ( 10.82940026203503336, 170.3927522451417929, -10.00000000000009237 ) ) ;
#10475=CARTESIAN_POINT ( 'NONE',  ( 204.6703448838256918, 269.2340485566120947, -2.958164987615520936 ) ) ;
#10476=CARTESIAN_POINT ( 'NONE',  ( 191.4657099001964866, 299.0186578760529983, -10.61565110258011480 ) ) ;
#10477=CARTESIAN_POINT ( 'NONE',  ( 149.0761751337341821, 272.4394858007734683, 11.56094486755886130 ) ) ;
#10478=CARTESIAN_POINT ( 'NONE',  ( 163.2442700311756596, 247.8996255919473697, 11.14021925110252020 ) ) ;
#10480=CARTESIAN_POINT ( 'NONE',  ( 152.5863647195084809, 275.6253943308787484, -8.621472240177467938 ) ) ;
#10482=VERTEX_POINT ( 'NONE', #21481 ) ;
#10484=CARTESIAN_POINT ( 'NONE',  ( 193.2812998533557618, 275.8456789399431273, -16.80650560145133809 ) ) ;
#10489=CARTESIAN_POINT ( 'NONE',  ( -0.2032289886040369309, 164.5643266524160140, -9.188101187500093303 ) ) ;
#10490=CARTESIAN_POINT ( 'NONE',  ( 100.4182711614829486, 216.5327760586659451, 1.948934522072303157E-15 ) ) ;
#10491=CARTESIAN_POINT ( 'NONE',  ( 155.6048174803203210, 261.1315455520403361, -17.38645169541727498 ) ) ;
#10492=CARTESIAN_POINT ( 'NONE',  ( 146.9129474150286683, 276.1863061179126930, -5.016087650759920358 ) ) ;
#10494=CARTESIAN_POINT ( 'NONE',  ( -4.163664537435148638, 161.7365022471902307, 10.00000000000009948 ) ) ;
#10496=CARTESIAN_POINT ( 'NONE',  ( 164.2093793230265817, 284.1672360007073053, 5.801580848943813429 ) ) ;
#10497=CARTESIAN_POINT ( 'NONE',  ( 190.3965342815112933, 300.3990912182416650, -0.9262266978771579451 ) ) ;
#10498=CARTESIAN_POINT ( 'NONE',  ( 163.2742264920156572, 247.8477394797576778, -9.850275379362519956 ) ) ;
#10499=CARTESIAN_POINT ( 'NONE',  ( 207.4561410457603472, 271.3224186970049914, 4.887894857253799685 ) ) ;
#10501=DIRECTION ( 'NONE',  ( -0.8660254037844387076, -0.4999999999999998890, -0.000000000000000000 ) ) ;
#10506=B_SPLINE_CURVE_WITH_KNOTS ( 'NONE', 3,
 ( #24159, #32253, #55044, #8459 ),
 .UNSPECIFIED., .F., .F.,
 ( 4, 4 ),
 ( 0.009739077263292133385, 0.01805476430672628765 ),
 .UNSPECIFIED. ) ;
#10507=CARTESIAN_POINT ( 'NONE',  ( 90.56794795857862823, 211.5494855054051584, -2.679491924311248496 ) ) ;
#10510=CARTESIAN_POINT ( 'NONE',  ( 46.72434903108273119, 197.7833772461660828, -9.188101187500095079 ) ) ;
#10514=CARTESIAN_POINT ( 'NONE',  ( 69.94482871793547929, 205.0643266524159856, -9.188101187500093303 ) ) ;
#10515=CARTESIAN_POINT ( 'NONE',  ( 161.3145230519951951, 251.2420454056404822, -14.44869077440025151 ) ) ;
#10518=CARTESIAN_POINT ( 'NONE',  ( 163.4927498574098763, 249.4692459082536686, 11.48939803020791750 ) ) ;
#10520=CARTESIAN_POINT ( 'NONE',  ( 200.3107031111897243, 283.6986802420111644, 17.10973405491822419 ) ) ;
#10521=B_SPLINE_CURVE_WITH_KNOTS ( 'NONE', 3,
 ( #47818, #78756, #9343, #71162 ),
 .UNSPECIFIED., .F., .F.,
 ( 4, 4 ),
 ( 0.01197369137472301809, 0.01810739594695707014 ),
 .UNSPECIFIED. ) ;
#10522=CARTESIAN_POINT ( 'NONE',  ( 17.25242200676959570, 180.7677522451418497, 10.00000000000009592 ) ) ;
#10526=EDGE_LOOP ( 'NONE', ( #58229, #26025, #78330, #8554, #64602, #47909, #72766, #96977, #46188, #29430, #77336, #33155, #68915, #98031, #36335, #71659, #4846, #10951, #25302, #331, #43335, #98823, #18782, #85278, #65640, #89263, #25789, #37698, #80257, #88003, #29709, #72495, #46012, #20778, #28661, #4245, #89965, #63132, #14454, #18543, #73176, #39298, #42103, #7819, #65321, #68510, #52177, #20182, #94043, #28992, #65122, #52930, #77214, #34539, #37417, #45231, #70251, #56767, #31169, #85243, #2568, #22810, #70988, #85626, #96809, #50453, #4067, #97171, #79464, #32579, #86350, #70097, #30886, #35828, #84878, #95698, #38571, #79751, #82722, #98922, #26054, #25379, #71016, #51682, #34708, #17123, #62956, #22878, #68832, #51917, #74507, #75390, #11829, #31358, #74717, #56895, #10599, #54487, #23782, #6943, #50632, #15782, #72133, #11454, #96963, #31096, #37705, #41934, #16970, #24500, #10669, #17502, #31097, #39063, #93455, #53618, #76453, #67998, #38699, #98654, #42754, #27240, #1991, #5438, #14373, #5047, #52281 ) ) ;
#10528=CARTESIAN_POINT ( 'NONE',  ( 70.81050702595493362, 217.8149278399160949, 9.188101187500093303 ) ) ;
#10529=CARTESIAN_POINT ( 'NONE',  ( 89.29491028763546012, 232.3615022471903160, 5.000000000000046185 ) ) ;
#10530=CARTESIAN_POINT ( 'NONE',  ( 159.4889735931715222, 254.4039898200529706, 16.88104032092801887 ) ) ;
#10532=CARTESIAN_POINT ( 'NONE',  ( 201.7913750587587458, 281.1340811994797946, 17.83190890278124741 ) ) ;
#10535=CARTESIAN_POINT ( 'NONE',  ( 193.5431251303248530, 288.4874559808632171, 16.06641325508723384 ) ) ;
#10536=CARTESIAN_POINT ( 'NONE',  ( 12.50963621419470329, 166.4824982072973967, 3.021315404115420679E-15 ) ) ;
#10537=CARTESIAN_POINT ( 'NONE',  ( 127.4000280541508516, 234.3615022471901739, 5.000000000000051514 ) ) ;
#10538=( BOUNDED_CURVE ( )  B_SPLINE_CURVE ( 2, ( #69431, #22334, #28950, #6646, #44616, #60313, #92283, #45128, #98361 ),
 .UNSPECIFIED., .F., .T. ) 
 B_SPLINE_CURVE_WITH_KNOTS ( ( 3, 2, 2, 2, 3 ),
 ( 0.4959677419354838745, 0.4973118279569892497, 0.5000000000000000000, 0.5026881720430107503, 0.5040322580645161255 ),
 .UNSPECIFIED. ) 
 CURVE ( )  GEOMETRIC_REPRESENTATION_ITEM ( )  RATIONAL_B_SPLINE_CURVE ( ( 0.9330127018922194093, 0.9330127018922194093, 1.000000000000000000, 0.8660254037844387076, 1.000000000000000000, 0.8660254037844387076, 1.000000000000000000, 0.9330127018922194093, 0.9330127018922194093 ) ) 
 REPRESENTATION_ITEM ( '' )  );
#10539=CARTESIAN_POINT ( 'NONE',  ( 20.08504676852914628, 175.7365022471902307, -10.00000000000009237 ) ) ;
#10541=ORIENTED_EDGE ( 'NONE', *, *, #69760, .T. ) ;
#10542=CARTESIAN_POINT ( 'NONE',  ( 184.9257308103695436, 271.4024368688196205, 16.03004893721198343 ) ) ;
#10544=CARTESIAN_POINT ( 'NONE',  ( 202.2603678735342214, 280.3217618159037556, 16.49712126737133744 ) ) ;
#10546=CARTESIAN_POINT ( 'NONE',  ( 150.0694502760089222, 271.4680435213315945, -12.17790201236558545 ) ) ;
#10549=ORIENTED_EDGE ( 'NONE', *, *, #25802, .T. ) ;
#10551=CARTESIAN_POINT ( 'NONE',  ( 170.7055562504701527, 250.3708107612802110, 3.163906886382704009 ) ) ;
#10559=CARTESIAN_POINT ( 'NONE',  ( 167.3614853001860752, 276.6147906615189527, 15.78902546434338561 ) ) ;
#10563=CARTESIAN_POINT ( 'NONE',  ( 186.2060483959004102, 298.7711416952031414, 1.080402104957500331 ) ) ;
#10564=B_SPLINE_CURVE_WITH_KNOTS ( 'NONE', 3,
 ( #58999, #60008, #43818, #27146 ),
 .UNSPECIFIED., .F., .F.,
 ( 4, 4 ),
 ( 0.04343396320418384943, 0.04853114605566435924 ),
 .UNSPECIFIED. ) ;
#10565=CARTESIAN_POINT ( 'NONE',  ( 204.6780326111993986, 276.1342436545999703, 14.85609018352459287 ) ) ;
#10566=CARTESIAN_POINT ( 'NONE',  ( 148.0637215040603394, 274.1931069276759558, -7.795633835291665648 ) ) ;
#10568=CARTESIAN_POINT ( 'NONE',  ( 155.5888570658010508, 261.1591898008976500, 17.34682632352454945 ) ) ;
#10569=CARTESIAN_POINT ( 'NONE',  ( 154.8332767207531901, 280.7459370637686220, -0.9958211956073632631 ) ) ;
#10571=CARTESIAN_POINT ( 'NONE',  ( 207.4143746336561094, 271.3947602448195084, -4.799001228152785181 ) ) ;
#10572=CARTESIAN_POINT ( 'NONE',  ( 169.0547802094920371, 266.9661960260407909, 17.74255763397777130 ) ) ;
#10574=CARTESIAN_POINT ( 'NONE',  ( 84.34250105585179824, 213.3768266524160140, 9.188101187500098632 ) ) ;
#10577=CARTESIAN_POINT ( 'NONE',  ( 163.6377088202057166, 277.2438325465888056, -14.42846884688455589 ) ) ;
#10578=EDGE_CURVE ( 'NONE', #40485, #47191, #60958, .T. ) ;
#10580=CARTESIAN_POINT ( 'NONE',  ( 167.9757358556196039, 266.9719029692253116, -17.65027412328727152 ) ) ;
#10582=CARTESIAN_POINT ( 'NONE',  ( 201.3053657339852691, 274.7141922394133076, -14.27644254562359372 ) ) ;
#10584=CARTESIAN_POINT ( 'NONE',  ( 146.7434471017767521, 276.4798892723637209, 0.7354350123930684102 ) ) ;
#10586=CARTESIAN_POINT ( 'NONE',  ( 206.8317058779879574, 272.4039721336197317, -10.41591514895975834 ) ) ;
#10587=CARTESIAN_POINT ( 'NONE',  ( 208.1303038335461224, 270.1547344959873840, 3.060743731163897863 ) ) ;
#10588=CARTESIAN_POINT ( 'NONE',  ( 96.08779704679574252, 226.2833772461660260, -9.188101187500095079 ) ) ;
#10595=CARTESIAN_POINT ( 'NONE',  ( 164.9656603750091506, 286.4677819567733650, 1.164111042001980678 ) ) ;
#10597=CARTESIAN_POINT ( 'NONE',  ( -3.965200385949115169, 158.5177522451418213, 5.000000000000051514 ) ) ;
#10599=ORIENTED_EDGE ( 'NONE', *, *, #13600, .F. ) ;
#10601=B_SPLINE_CURVE_WITH_KNOTS ( 'NONE', 3,
 ( #36839, #97674, #6933, #90089, #28747, #37822, #59627, #99654, #52047, #44926, #82985, #13561, #75366, #30240, #5946, #67748, #98672, #60121, #91084, #72127, #79261, #9832, #2732, #10820, #61622, #33620, #48824, #64516, #86873, #56403, #2229, #17406, #10323, #65016, #40693, #48316, #41697, #16901, #49807, #69229, #87879, #7429, #47790, #38322, #95473, #57398, #72642, #33109, #94949, #18426, #87397, #94446, #3239, #26026 ),
 .UNSPECIFIED., .F., .F.,
 ( 4, 2, 2, 2, 2, 2, 2, 2, 2, 2, 2, 2, 2, 2, 2, 2, 2, 2, 2, 2, 2, 2, 2, 2, 2, 2, 4 ),
 ( 0.001822495010402024659, 0.002272902490822721697, 0.002498106231033042461, 0.002723309971243363659, 0.002835911841348543773, 0.002948513711453724321, 0.003061115581558904435, 0.003173717451664084983, 0.003398921191874445646, 0.003624124932084806308, 0.004074532412505526766, 0.004524939892926247223, 0.005425754853767611810, 0.006326569814608976397, 0.006776977295029658691, 0.007227384775450340984, 0.007339986645555551456, 0.007396287580608187917, 0.007452588515660822643, 0.007565190385766093831, 0.007677792255871365018, 0.007902995996081869229, 0.008128199736292375174, 0.008353403476502881120, 0.008578607216713385331, 0.008803810956923891276, 0.009029014697134397222 ),
 .UNSPECIFIED. ) ;
#10603=CARTESIAN_POINT ( 'NONE',  ( 159.7132918459648181, 254.0154592091499239, -16.90058287995827158 ) ) ;
#10604=CARTESIAN_POINT ( 'NONE',  ( 191.0627567933567548, 271.2378347160873204, 14.18540690319008135 ) ) ;
#10605=CARTESIAN_POINT ( 'NONE',  ( 174.6143879786744151, 283.7077023516287682, 13.57591769828411543 ) ) ;
#10607=CARTESIAN_POINT ( 'NONE',  ( 139.0246627140281248, 262.6199935810940360, 2.679491924311251605 ) ) ;
#10609=CARTESIAN_POINT ( 'NONE',  ( 3.125382611083852957, 172.6115022471902591, 10.00000000000009592 ) ) ;
#10610=CARTESIAN_POINT ( 'NONE',  ( 200.4775477985258760, 283.4096967665721536, 16.80647240730505487 ) ) ;
#10612=CARTESIAN_POINT ( 'NONE',  ( 167.6039016024858768, 249.9644671705272287, 7.137948275192514735 ) ) ;
#10614=CARTESIAN_POINT ( 'NONE',  ( 178.7802048856326849, 291.7431450991714428, -6.108826784319776770 ) ) ;
#10615=CARTESIAN_POINT ( 'NONE',  ( 163.2175214641260652, 247.9459554691067638, -11.09782983415651181 ) ) ;
#10620=CARTESIAN_POINT ( 'NONE',  ( 180.6242511116918763, 266.9822466815605253, -14.84429364384706496 ) ) ;
#10621=CARTESIAN_POINT ( 'NONE',  ( 185.4835256528986633, 266.2441379785080358, 13.04562320151002908 ) ) ;
#10623=EDGE_CURVE ( 'NONE', #81988, #23533, #93541, .T. ) ;
#10625=CARTESIAN_POINT ( 'NONE',  ( 152.7531861616124615, 266.0707158804971186, 17.45453282433162556 ) ) ;
#10630=CARTESIAN_POINT ( 'NONE',  ( 156.6084421796713002, 261.3932165810376205, -17.82046942966612590 ) ) ;
#10631=CARTESIAN_POINT ( 'NONE',  ( 207.1007598919583472, 271.9379569114424271, -6.086525981869248092 ) ) ;
#10632=CARTESIAN_POINT ( 'NONE',  ( 11.29875767934929520, 168.1423013555409796, -4.594050593750043987 ) ) ;
#10635=EDGE_CURVE ( 'NONE', #2437, #48869, #23325, .T. ) ;
#10637=B_SPLINE_CURVE_WITH_KNOTS ( 'NONE', 3,
 ( #57123, #96182, #19168, #18656, #39913, #40915 ),
 .UNSPECIFIED., .F., .F.,
 ( 4, 2, 4 ),
 ( 0.01970985617426966596, 0.02425325239201692878, 0.02879664860976419161 ),
 .UNSPECIFIED. ) ;
#10640=CARTESIAN_POINT ( 'NONE',  ( 35.84507844392322085, 185.3768266524159856, -9.188101187500093303 ) ) ;
#10641=CARTESIAN_POINT ( 'NONE',  ( 161.5504728662519369, 250.8333683393111926, 12.94300825113363373 ) ) ;
#10644=CARTESIAN_POINT ( 'NONE',  ( 200.0629734989200301, 267.3250638936581822, -6.802650431247307061 ) ) ;
#10645=CARTESIAN_POINT ( 'NONE',  ( 176.7349755076185716, 291.6822743229055277, 2.566495134243914400 ) ) ;
#10646=AXIS2_PLACEMENT_3D ( 'NONE', #77050, #99382, #85725 ) ;
#10647=CARTESIAN_POINT ( 'NONE',  ( 149.0581491015862241, 272.4707078043124966, 11.78139744831781321 ) ) ;
#10648=CARTESIAN_POINT ( 'NONE',  ( 180.2906925969918177, 272.3403866223749787, 17.68789668772514290 ) ) ;
#10651=CARTESIAN_POINT ( 'NONE',  ( 81.50068165357551209, 227.8615022471903160, 5.000000000000046185 ) ) ;
#10652=CARTESIAN_POINT ( 'NONE',  ( 8.754547735682661980, 185.8615022471903160, 5.000000000000046185 ) ) ;
#10654=CARTESIAN_POINT ( 'NONE',  ( 54.70828104404427705, 193.2048013555409796, 4.594050593750051981 ) ) ;
#10655=CARTESIAN_POINT ( 'NONE',  ( 198.1230806404959139, 287.4877535090322453, 17.00698319228197164 ) ) ;
#10658=CARTESIAN_POINT ( 'NONE',  ( 190.9586609929293104, 299.8968923453624598, -4.970176667899034229 ) ) ;
#10661=CARTESIAN_POINT ( 'NONE',  ( 170.4597437522810424, 286.1127027945369719, 7.473822327501647322 ) ) ;
#10662=CARTESIAN_POINT ( 'NONE',  ( 164.7243055739305078, 245.3361288348881999, -1.445094907380085170 ) ) ;
#10663=CARTESIAN_POINT ( 'NONE',  ( 193.3082004299502046, 295.8273706660551738, 13.84301442133521043 ) ) ;
#10666=CARTESIAN_POINT ( 'NONE',  ( 202.6070187115982719, 279.7213449518906145, 15.56322169823762280 ) ) ;
#10667=CARTESIAN_POINT ( 'NONE',  ( 149.0164813726494799, 272.5428784278667536, -11.67305721329070423 ) ) ;
#10668=CARTESIAN_POINT ( 'NONE',  ( 173.4136195317119018, 256.7516932182500113, 11.26842845872458376 ) ) ;
#10669=ORIENTED_EDGE ( 'NONE', *, *, #55561, .F. ) ;
#10675=CARTESIAN_POINT ( 'NONE',  ( 190.8443993347725325, 300.0947993426467519, 8.522468760355437212 ) ) ;
#10676=CARTESIAN_POINT ( 'NONE',  ( 177.5792917427869497, 255.5367556796404074, -6.834657972258073144 ) ) ;
#10679=CARTESIAN_POINT ( 'NONE',  ( 207.2167723318516153, 271.7370174712370954, -6.606038862010207957 ) ) ;
#10680=CYLINDRICAL_SURFACE ( 'NONE', #16790, 17.82106496071139645 ) ;
#10681=CARTESIAN_POINT ( 'NONE',  ( 196.9098758191317700, 289.5890858996224324, -16.54412079817003800 ) ) ;
#10683=CARTESIAN_POINT ( 'NONE',  ( 200.8147387322574957, 282.8256649374973790, -18.02438097732020239 ) ) ;
#10687=CARTESIAN_POINT ( 'NONE',  ( 205.4029933437358295, 274.8785748323546159, -13.50815392427034922 ) ) ;
#10688=CARTESIAN_POINT ( 'NONE',  ( 117.9006383567337792, 245.0024278399160949, 9.188101187500095079 ) ) ;
#10689=CARTESIAN_POINT ( 'NONE',  ( 196.4170778717353585, 290.4426369823788718, -17.78762421190030452 ) ) ;
#10690=CARTESIAN_POINT ( 'NONE',  ( 183.7819271391472853, 288.5527987327671440, -13.16916153635029829 ) ) ;
#10694=CARTESIAN_POINT ( 'NONE',  ( 207.5408646414791178, 271.1756731246201753, 3.050859480894625886 ) ) ;
#10695=VERTEX_POINT ( 'NONE', #69062 ) ;
#10697=CARTESIAN_POINT ( 'NONE',  ( 198.2114954873088948, 287.3346145022089786, 18.52864136173620935 ) ) ;
#10700=CARTESIAN_POINT ( 'NONE',  ( 62.15060008387555968, 200.5643266524159856, -9.188101187500093303 ) ) ;
#10702=CARTESIAN_POINT ( 'NONE',  ( 190.9907605556751093, 299.8412942717858414, 8.799173206188184437 ) ) ;
#10703=CARTESIAN_POINT ( 'NONE',  ( 198.6859012307616581, 286.5129196511462624, 18.23225590904412030 ) ) ;
#10705=CARTESIAN_POINT ( 'NONE',  ( 172.6048621181717806, 271.8561855147940491, 17.03490788493881425 ) ) ;
#10706=ORIENTED_EDGE ( 'NONE', *, *, #91364, .T. ) ;
#10708=CARTESIAN_POINT ( 'NONE',  ( 199.1041333440138317, 265.1832257255362038, 0.2027868546939186056 ) ) ;
#10711=CARTESIAN_POINT ( 'NONE',  ( 173.1855788362566955, 260.3541085725848916, -13.89348164722228240 ) ) ;
#10712=CARTESIAN_POINT ( 'NONE',  ( 174.2579852878230895, 277.3140177265087800, -15.60830308234947061 ) ) ;
#10713=EDGE_CURVE ( 'NONE', #41328, #59881, #29766, .T. ) ;
#10714=CARTESIAN_POINT ( 'NONE',  ( 161.7938256150359848, 259.1648011204742375, -16.40003089747464671 ) ) ;
#10715=CARTESIAN_POINT ( 'NONE',  ( 206.8889038998294723, 269.8868643644167378, 1.765609235721585568 ) ) ;
#10716=CARTESIAN_POINT ( 'NONE',  ( 190.0550686570564949, 301.4619601804237732, 4.203010638620038542 ) ) ;
#10717=CARTESIAN_POINT ( 'NONE',  ( 177.1677292396067287, 269.5601071575461560, 16.13534633437323507 ) ) ;
#10718=CARTESIAN_POINT ( 'NONE',  ( 186.3805605339445606, 261.9022306725897238, 10.64329021816346454 ) ) ;
#10720=CARTESIAN_POINT ( 'NONE',  ( 194.9471474500919896, 290.9886311562445371, 16.55118206508679890 ) ) ;
#10721=CARTESIAN_POINT ( 'NONE',  ( 208.1876422586379647, 270.0554214305024630, 3.377638779759113863 ) ) ;
#10722=CARTESIAN_POINT ( 'NONE',  ( 124.6666353716822186, 242.7833772461660544, -9.188101187500095079 ) ) ;
#10727=CARTESIAN_POINT ( 'NONE',  ( 155.1601726304954809, 261.9016930232608615, -18.56587418422714464 ) ) ;
#10731=CARTESIAN_POINT ( 'NONE',  ( -10.31836507581447471, 176.3967562850347406, -4.648177544792955347E-16 ) ) ;
#10732=CARTESIAN_POINT ( 'NONE',  ( 177.7461146735995214, 255.2454472211425127, 4.878792714415012277 ) ) ;
#10735=CARTESIAN_POINT ( 'NONE',  ( 158.5161628873921131, 275.0455875265674308, -12.48876142424470714 ) ) ;
#10736=CARTESIAN_POINT ( 'NONE',  ( 147.6238900292995879, 275.3621543041489872, 3.125955112918928691 ) ) ;
#10737=CARTESIAN_POINT ( 'NONE',  ( 182.5145075214082340, 260.7231217271532273, 9.500621738068392830 ) ) ;
#10738=CARTESIAN_POINT ( 'NONE',  ( 140.4447960187037552, 242.7048013555409796, 4.594050593750051981 ) ) ;
#10741=CARTESIAN_POINT ( 'NONE',  ( 68.13167480270307408, 200.9548013555409796, -4.594050593750042211 ) ) ;
#10742=CARTESIAN_POINT ( 'NONE',  ( 157.8239779013331372, 257.2878469527003062, -17.92251383114021479 ) ) ;
#10743=CARTESIAN_POINT ( 'NONE',  ( 170.6659753671055171, 250.4757724785690698, 3.524607026314700242 ) ) ;
#10746=CARTESIAN_POINT ( 'NONE',  ( 190.8072577185990610, 300.1591305089344814, 3.698484652594827171 ) ) ;
#10747=CARTESIAN_POINT ( 'NONE',  ( 155.2672715809540591, 279.9936962574083736, -0.9937612457601998628 ) ) ;
#10748=CARTESIAN_POINT ( 'NONE',  ( 168.9333898618331489, 285.8808315938983924, -9.126212950214783959 ) ) ;
#10749=CARTESIAN_POINT ( 'NONE',  ( 197.8809552785519656, 287.9071269377202498, 17.61728046362068412 ) ) ;
#10751=ADVANCED_FACE ( 'NONE', ( #42643 ), #53341, .F. ) ;
#10752=CARTESIAN_POINT ( 'NONE',  ( 113.8142545287344802, 246.5177522451419065, 5.000000000000046185 ) ) ;
#10756=CARTESIAN_POINT ( 'NONE',  ( 159.9924463476198753, 283.3850188831759169, -3.371971149216307140 ) ) ;
#10757=CARTESIAN_POINT ( 'NONE',  ( -5.561934722402757991, 167.5958772461660544, -9.188101187500095079 ) ) ;
#10759=CARTESIAN_POINT ( 'NONE',  ( 41.69040282370318096, 201.0024278399160664, -9.188101187500093303 ) ) ;
#10760=CARTESIAN_POINT ( 'NONE',  ( 25.28119919123577475, 178.7365022471902023, -10.00000000000009237 ) ) ;
#10766=CARTESIAN_POINT ( 'NONE',  ( 190.7403173041394950, 300.2750747078583800, -4.254144485856557800 ) ) ;
#10768=EDGE_CURVE ( 'NONE', #22014, #68457, #58167, .T. ) ;
#10770=CARTESIAN_POINT ( 'NONE',  ( 62.64658692180396571, 193.6427522451417644, 1.119607411625061291E-15 ) ) ;
#10771=CARTESIAN_POINT ( 'NONE',  ( 180.8099474207024286, 256.2767700812191265, 1.456173454511005660 ) ) ;
#10772=CARTESIAN_POINT ( 'NONE',  ( 157.1269483542914998, 258.4951375425532092, -17.15328932028234377 ) ) ;
#10773=CARTESIAN_POINT ( 'NONE',  ( 80.61430232155159104, 228.8967562850347122, -4.648177544792955347E-16 ) ) ;
#10775=CARTESIAN_POINT ( 'NONE',  ( 47.29267820409027934, 188.1115022471902023, -5.000000000000041744 ) ) ;
#10777=CARTESIAN_POINT ( 'NONE',  ( 163.1332433029523372, 248.0919295262283981, 11.24052392390482957 ) ) ;
#10778=CARTESIAN_POINT ( 'NONE',  ( 4.289451341410244645, 161.0327760586659451, 1.948934522072303157E-15 ) ) ;
#10781=CARTESIAN_POINT ( 'NONE',  ( 192.1859061758433143, 297.7712413352111298, 11.15082371775444336 ) ) ;
#10783=CARTESIAN_POINT ( 'NONE',  ( 77.09838585100463604, 221.9865022471902876, -10.00000000000009592 ) ) ;
#10784=CARTESIAN_POINT ( 'NONE',  ( 183.1758135086024595, 257.7755843168840784, -2.206437414030474109 ) ) ;
#10786=CARTESIAN_POINT ( 'NONE',  ( 176.4797194055593934, 260.2797452624257630, -13.51627001118733773 ) ) ;
#10789=CARTESIAN_POINT ( 'NONE',  ( 154.4302508464143102, 278.3454869111918697, -5.206030047134956540 ) ) ;
#10796=B_SPLINE_CURVE_WITH_KNOTS ( 'NONE', 3,
 ( #75775, #51456, #36250, #90001 ),
 .UNSPECIFIED., .F., .F.,
 ( 4, 4 ),
 ( 0.02733452390982080843, 0.03654861343160081127 ),
 .UNSPECIFIED. ) ;
#10798=ORIENTED_EDGE ( 'NONE', *, *, #29598, .T. ) ;
#10799=CARTESIAN_POINT ( 'NONE',  ( 152.8522706834672533, 265.8990964544007056, 17.63080661522264947 ) ) ;
#10800=CARTESIAN_POINT ( 'NONE',  ( 207.2824254892180704, 271.6233028670009162, 6.274396967990798046 ) ) ;
#10802=CARTESIAN_POINT ( 'NONE',  ( 116.8713438767135813, 249.8297689869268936, -2.679491924311252493 ) ) ;
#10809=CARTESIAN_POINT ( 'NONE',  ( 169.8880101891228378, 248.5302279630965927, 2.598380334187264218 ) ) ;
#10810=ORIENTED_EDGE ( 'NONE', *, *, #81375, .F. ) ;
#10816=CARTESIAN_POINT ( 'NONE',  ( 161.8016137473484548, 250.3983795733946636, 14.25000412375400316 ) ) ;
#10817=CARTESIAN_POINT ( 'NONE',  ( 166.2792040466741526, 273.7071925000096826, -16.00520433647330520 ) ) ;
#10819=ORIENTED_EDGE ( 'NONE', *, *, #85203, .F. ) ;
#10820=CARTESIAN_POINT ( 'NONE',  ( 172.8704676289727047, 256.8043734995969771, -11.66604796816862866 ) ) ;
#10823=EDGE_LOOP ( 'NONE', ( #18399, #13420, #28629, #54661 ) ) ;
#10824=CARTESIAN_POINT ( 'NONE',  ( 157.0122940985184528, 266.1029671896999389, -16.89663335517050768 ) ) ;
#10825=ORIENTED_EDGE ( 'NONE', *, *, #17598, .F. ) ;
#10828=CARTESIAN_POINT ( 'NONE',  ( 147.9411595194912934, 274.4053905120259742, 6.673340298825284123 ) ) ;
#10829=CARTESIAN_POINT ( 'NONE',  ( 180.5607909224531227, 291.5613472329837350, -9.815939981736717002 ) ) ;
#10830=CARTESIAN_POINT ( 'NONE',  ( 190.4083125682826392, 267.3722578230377280, -13.56112132691750105 ) ) ;
#10834=CARTESIAN_POINT ( 'NONE',  ( 197.1145765276632460, 289.2345338721006556, -16.80523350695997564 ) ) ;
#10838=VECTOR ( 'NONE', #68363, 1000.000000000000000 ) ;
#10839=CARTESIAN_POINT ( 'NONE',  ( 164.2572333502590709, 246.1451216570909253, 2.155809084027023204 ) ) ;
#10840=CARTESIAN_POINT ( 'NONE',  ( 196.4808189786114951, 290.3322341467384717, -17.84817245450773271 ) ) ;
#10841=DIRECTION ( 'NONE',  ( 0.4999999999999998890, -0.8660254037844385966, 0.000000000000000000 ) ) ;
#10846=CARTESIAN_POINT ( 'NONE',  ( 190.3269285683297198, 300.9910850015572805, 5.981691054164898880 ) ) ;
#10847=CARTESIAN_POINT ( 'NONE',  ( 171.5510444326116613, 259.6073805218057942, -14.00194690452766189 ) ) ;
#10848=CARTESIAN_POINT ( 'NONE',  ( 164.0005577228977529, 247.4545569590189587, 7.324775775061132421 ) ) ;
#10852=CARTESIAN_POINT ( 'NONE',  ( 199.4035972599234867, 285.2698336642472441, -18.06228912948296284 ) ) ;
#10853=CARTESIAN_POINT ( 'NONE',  ( 148.6048294702719375, 273.2558804378169839, -10.20107683747840888 ) ) ;
#10858=CARTESIAN_POINT ( 'NONE',  ( 43.23318412030271674, 205.7677522451419350, -5.000000000000047962 ) ) ;
#10861=CARTESIAN_POINT ( 'NONE',  ( 23.81978131880161342, 177.8927522451418213, -10.00000000000009059 ) ) ;
#10862=CARTESIAN_POINT ( 'NONE',  ( 104.0717290597573026, 221.7048013555409796, 4.594050593750051981 ) ) ;
#10863=CARTESIAN_POINT ( 'NONE',  ( 180.7931344147162349, 294.0809750825963533, -2.761424145458095225 ) ) ;
#10865=CARTESIAN_POINT ( 'NONE',  ( 207.5603179267596374, 271.1419790461399089, 2.162348062361596490 ) ) ;
#10866=CARTESIAN_POINT ( 'NONE',  ( 22.50244069716294959, 192.9869531367911293, 4.594050593750046652 ) ) ;
#10867=CARTESIAN_POINT ( 'NONE',  ( 200.6129772034685175, 283.1751261563724142, 18.36811917402039640 ) ) ;
#10869=AXIS2_PLACEMENT_3D ( 'NONE', #92828, #40073, #85240 ) ;
#10871=CARTESIAN_POINT ( 'NONE',  ( 185.9634666876222866, 260.4317438331094081, -5.811366535968028657 ) ) ;
#10872=CARTESIAN_POINT ( 'NONE',  ( 180.4448332398771129, 260.5583812017072205, 12.70931349753900008 ) ) ;
#10873=CARTESIAN_POINT ( 'NONE',  ( 194.3204549332184001, 264.5487851543980469, -4.361261795965002186 ) ) ;
#10874=CARTESIAN_POINT ( 'NONE',  ( 183.0847682432378463, 284.5747524302673241, 14.98238360739832764 ) ) ;
#10875=CARTESIAN_POINT ( 'NONE',  ( 168.0462690533684338, 251.4142709888886884, 10.74789308012043954 ) ) ;
#10877=CARTESIAN_POINT ( 'NONE',  ( 48.78150646083578579, 186.7202760586659736, -5.415160957724236172E-17 ) ) ;
#10878=CARTESIAN_POINT ( 'NONE',  ( 84.80240350195582266, 219.7677522451418497, 10.00000000000009592 ) ) ;
#10879=B_SPLINE_CURVE_WITH_KNOTS ( 'NONE', 3,
 ( #22100, #52996, #61084, #5416 ),
 .UNSPECIFIED., .F., .F.,
 ( 4, 4 ),
 ( 0.02303826909059158295, 0.03226139655626733549 ),
 .UNSPECIFIED. ) ;
#10884=CARTESIAN_POINT ( 'NONE',  ( 158.2696483452693030, 282.4806668385787134, -1.679042238831097489 ) ) ;
#10885=CARTESIAN_POINT ( 'NONE',  ( 6.724974241671477060, 168.5643266524160424, 9.188101187500095079 ) ) ;
#10888=CARTESIAN_POINT ( 'NONE',  ( 151.4428545556028780, 268.3402767968688067, -15.03309903163500749 ) ) ;
#10889=CARTESIAN_POINT ( 'NONE',  ( -22.42236680055709641, 157.8615022471902591, 0.000000000000000000 ) ) ;
#10890=CARTESIAN_POINT ( 'NONE',  ( 193.0065576635309412, 296.3498312632291913, -11.90044991639595295 ) ) ;
#10891=CARTESIAN_POINT ( 'NONE',  ( 169.3986711591969367, 265.8083199790463027, 17.66272553310151494 ) ) ;
#10892=CARTESIAN_POINT ( 'NONE',  ( 204.1793240545508752, 276.9980322128846524, 14.17550310845996187 ) ) ;
#10893=CARTESIAN_POINT ( 'NONE',  ( 191.0862225170008628, 299.6759493045793192, -9.402218231374108726 ) ) ;
#10894=CARTESIAN_POINT ( 'NONE',  ( 206.9258336080761183, 272.2409381227055292, 6.776000910836894597 ) ) ;
#10896=CARTESIAN_POINT ( 'NONE',  ( 0.5273063997305368344, 171.1115022471902591, 10.00000000000009592 ) ) ;
#10899=CARTESIAN_POINT ( 'NONE',  ( 124.1257165900819359, 230.2202760586659736, -5.415160957724236172E-17 ) ) ;
#10901=B_SPLINE_CURVE_WITH_KNOTS ( 'NONE', 3,
 ( #44256, #51880, #59444, #14856 ),
 .UNSPECIFIED., .F., .F.,
 ( 4, 4 ),
 ( 0.04471951162845413247, 0.04887066958154934887 ),
 .UNSPECIFIED. ) ;
#10903=CARTESIAN_POINT ( 'NONE',  ( 151.1920263787787349, 270.5503660113284923, 14.04656984271712439 ) ) ;
#10904=CARTESIAN_POINT ( 'NONE',  ( 195.7617614321055157, 291.5776783508526364, 16.33009124109666033 ) ) ;
#10906=CARTESIAN_POINT ( 'NONE',  ( 190.7283810415139271, 300.2957489211784718, -7.863702551849829803 ) ) ;
#10908=CARTESIAN_POINT ( 'NONE',  ( 189.9271880503060572, 261.0444523307733675, -4.592131172855204113 ) ) ;
#10909=CARTESIAN_POINT ( 'NONE',  ( 196.7130436017243653, 289.9300093007386749, -16.33278734947153765 ) ) ;
#10911=CARTESIAN_POINT ( 'NONE',  ( 190.2911366393398680, 300.0106470811841177, 4.501196058731199656 ) ) ;
#10912=CARTESIAN_POINT ( 'NONE',  ( 176.3606141446090874, 292.2811541075674313, -1.103747915900352705 ) ) ;
#10915=CARTESIAN_POINT ( 'NONE',  ( 189.0809633534686043, 265.6194490791910994, 11.75540354764823547 ) ) ;
#10916=CYLINDRICAL_SURFACE ( 'NONE', #99310, 17.82106496071139645 ) ;
#10918=CARTESIAN_POINT ( 'NONE',  ( 168.6645287092987360, 271.8237458140437752, -17.23257543817958037 ) ) ;
#10920=B_SPLINE_SURFACE_WITH_KNOTS ( 'NONE', 3, 1, ( 
 ( #48697, #10196 ),
 ( #77604, #1606 ),
 ( #32490, #63383 ),
 ( #24878, #55752 ),
 ( #17279, #41061 ),
 ( #48183, #9709 ),
 ( #71998, #15772 ),
 ( #81618, #3123 ),
 ( #95839, #42560 ),
 ( #64893, #72514 ),
 ( #11210, #18299 ),
 ( #49677, #96827 ),
 ( #88246, #4580 ),
 ( #4077, #74506 ),
 ( #10694, #27390 ),
 ( #82129, #96322 ),
 ( #20289, #12191 ),
 ( #73009, #58273 ),
 ( #33491, #89248 ),
 ( #58758, #43050 ),
 ( #19799, #65379 ),
 ( #26393, #51166 ),
 ( #50666, #73494 ),
 ( #34008, #3601 ),
 ( #73995, #18795 ),
 ( #49196, #57271 ),
 ( #56777, #35475 ),
 ( #19317, #66379 ),
 ( #80633, #80131 ),
 ( #97309, #34968 ),
 ( #87760, #50180 ),
 ( #27876, #42077 ),
 ( #88744, #34480 ),
 ( #26891, #89728 ) ),
 .UNSPECIFIED., .T., .F., .F.,
 ( 4, 2, 2, 2, 2, 2, 2, 2, 2, 2, 2, 2, 2, 2, 2, 2, 4 ),
 ( 2, 2 ),
 ( 0.000000000000000000, 0.06250000000000000000, 0.1250000000000000000, 0.1875000000000000000, 0.2500000000000000000, 0.3125000000000000000, 0.3750000000000000000, 0.4375000000000000000, 0.5000000000000000000, 0.5625000000000000000, 0.6250000000000000000, 0.6875000000000000000, 0.7500000000000000000, 0.8125000000000000000, 0.8750000000000000000, 0.9375000000000000000, 1.000000000000000000 ),
 ( 0.000000000000000000, 1.000000000000000000 ),
 .UNSPECIFIED. ) ;
#10921=CARTESIAN_POINT ( 'NONE',  ( 196.3917908427449106, 270.9162700290431758, 12.02664507717766895 ) ) ;
#10922=CARTESIAN_POINT ( 'NONE',  ( 156.7442704525034571, 261.1579551113846378, 17.82061976529222846 ) ) ;
#10923=CARTESIAN_POINT ( 'NONE',  ( 177.9342434413450746, 262.3724634088865173, 14.97940413522559311 ) ) ;
#10924=CARTESIAN_POINT ( 'NONE',  ( 148.2612186747170711, 275.6732389230651847, 6.000192647976810179 ) ) ;
#10927=CARTESIAN_POINT ( 'NONE',  ( 190.8747839792335412, 280.8223637028987127, 16.64593989182785805 ) ) ;
#10929=CARTESIAN_POINT ( 'NONE',  ( 195.0281415497474882, 290.0432247540097705, -16.40372058219452356 ) ) ;
#10930=ORIENTED_EDGE ( 'NONE', *, *, #86734, .F. ) ;
#10933=CARTESIAN_POINT ( 'NONE',  ( 194.6310785344323904, 293.5360785768717165, -14.54510914272505495 ) ) ;
#10934=CARTESIAN_POINT ( 'NONE',  ( 165.1399196574946018, 246.6162641258139843, 5.603258891903981187 ) ) ;
#10935=ORIENTED_EDGE ( 'NONE', *, *, #45369, .T. ) ;
#10937=CARTESIAN_POINT ( 'NONE',  ( -17.42236680055705023, 149.2012482093457777, 0.000000000000000000 ) ) ;
#10941=B_SPLINE_CURVE_WITH_KNOTS ( 'NONE', 3,
 ( #84965, #15509, #61115, #22637, #62105, #16523, #31219, #23607, #46928, #94070, #328, #45421, #15016, #55503 ),
 .UNSPECIFIED., .F., .F.,
 ( 4, 2, 2, 2, 2, 2, 4 ),
 ( 0.0009227269066335377912, 0.001449417115908541165, 0.001712762220546040250, 0.001976107325183539334, 0.002239452429821038419, 0.002502797534458537504, 0.003029487743733528735 ),
 .UNSPECIFIED. ) ;
#10944=CARTESIAN_POINT ( 'NONE',  ( 155.4661767250933622, 261.3716783840932294, -17.10192542004562810 ) ) ;
#10947=B_SPLINE_CURVE_WITH_KNOTS ( 'NONE', 3,
 ( #67965, #29463, #21860, #52744 ),
 .UNSPECIFIED., .F., .F.,
 ( 4, 4 ),
 ( 0.03703073727535406701, 0.04566479234050394020 ),
 .UNSPECIFIED. ) ;
#10948=CARTESIAN_POINT ( 'NONE',  ( 105.9243544191296422, 220.4155109091896065, 2.679491924311254714 ) ) ;
#10949=ORIENTED_EDGE ( 'NONE', *, *, #95172, .F. ) ;
#10950=PLANE ( 'NONE',  #80582 ) ;
#10951=ORIENTED_EDGE ( 'NONE', *, *, #60800, .F. ) ;
#10952=CARTESIAN_POINT ( 'NONE',  ( 173.3453504041607971, 270.5580986211186314, 17.57651758220006855 ) ) ;
#10953=CARTESIAN_POINT ( 'NONE',  ( 203.3205561747472814, 278.4854618126124706, -15.14439614831292147 ) ) ;
#10954=ORIENTED_EDGE ( 'NONE', *, *, #161, .T. ) ;
#10957=CARTESIAN_POINT ( 'NONE',  ( 161.6049555880495063, 255.0146571223070282, -15.06743769531358623 ) ) ;
#10958=CARTESIAN_POINT ( 'NONE',  ( 161.9909766791130608, 277.5219621271734241, -13.08164419582714721 ) ) ;
#10959=CARTESIAN_POINT ( 'NONE',  ( 146.9129474150286683, 276.1863061179126930, -5.016087650759920358 ) ) ;
#10960=CARTESIAN_POINT ( 'NONE',  ( 200.9445292274600092, 282.6008612054670266, -16.62830946367346741 ) ) ;
#10962=EDGE_CURVE ( 'NONE', #6447, #42087, #89299, .T. ) ;
#10963=CARTESIAN_POINT ( 'NONE',  ( 157.4545252365239776, 280.7287273452560612, 2.083561193472878603 ) ) ;
#10964=CARTESIAN_POINT ( 'NONE',  ( 132.2983106946500982, 253.3149278399160949, -9.188101187500095079 ) ) ;
#10970=VERTEX_POINT ( 'NONE', #10536 ) ;
#10972=CARTESIAN_POINT ( 'NONE',  ( 162.7561251957091031, 248.7451172484279027, 11.07313294959361194 ) ) ;
#10973=CARTESIAN_POINT ( 'NONE',  ( 120.7221038307704788, 252.0530062829862743, -4.648177544792955347E-16 ) ) ;
#10975=CARTESIAN_POINT ( 'NONE',  ( 152.7626916759926985, 277.8440032964028887, 6.837158938718278733 ) ) ;
#10977=CARTESIAN_POINT ( 'NONE',  ( 153.1627746953036535, 265.3612877299463548, -17.72069958822647351 ) ) ;
#10979=CARTESIAN_POINT ( 'NONE',  ( 170.9811431790156462, 280.9458665424763240, 14.82329785628973440 ) ) ;
#10984=CARTESIAN_POINT ( 'NONE',  ( 184.7187487274096327, 272.8151481436858035, -17.12587133286889696 ) ) ;
#10986=ORIENTED_EDGE ( 'NONE', *, *, #62898, .T. ) ;
#10988=B_SPLINE_CURVE_WITH_KNOTS ( 'NONE', 3,
 ( #56662, #77979, #71886, #93707 ),
 .UNSPECIFIED., .F., .F.,
 ( 4, 4 ),
 ( 0.03198279863331025819, 0.04097217294255945524 ),
 .UNSPECIFIED. ) ;
#10990=CARTESIAN_POINT ( 'NONE',  ( 156.7543839089325957, 276.7182480148175046, 10.07123213494488212 ) ) ;
#10991=CARTESIAN_POINT ( 'NONE',  ( 152.1196796635681494, 267.1679813220347910, -17.00838471677149144 ) ) ;
#10994=CARTESIAN_POINT ( 'NONE',  ( 202.9689790241539242, 279.0944113002206564, 15.85114608332523289 ) ) ;
#10998=ORIENTED_EDGE ( 'NONE', *, *, #46067, .F. ) ;
#11000=CARTESIAN_POINT ( 'NONE',  ( 2.096977440541873516, 182.0177522451419350, 5.000000000000046185 ) ) ;
#11004=VECTOR ( 'NONE', #21742, 1000.000000000000000 ) ;
#11006=DIRECTION ( 'NONE',  ( -0.8660254037844387076, -0.4999999999999998890, -0.000000000000000000 ) ) ;
#11007=EDGE_CURVE ( 'NONE', #75397, #49368, #11371, .T. ) ;
#11008=CARTESIAN_POINT ( 'NONE',  ( 162.8789161433191452, 248.5324370884573568, 9.731756914259689140 ) ) ;
#11009=CARTESIAN_POINT ( 'NONE',  ( 6.724974241671478836, 168.5643266524160140, 9.188101187500095079 ) ) ;
#11010=CARTESIAN_POINT ( 'NONE',  ( 102.2582280487598609, 229.8458772461660544, 9.188101187500095079 ) ) ;
#11012=CARTESIAN_POINT ( 'NONE',  ( 180.0322305761642383, 254.9176317891389090, -2.436366251733914190 ) ) ;
#11016=CARTESIAN_POINT ( 'NONE',  ( 172.5994563415556513, 290.7548730510699784, 2.767649011580872731 ) ) ;
#11017=CARTESIAN_POINT ( 'NONE',  ( 164.2149278243714150, 284.2439244671650727, 5.824652686812012981 ) ) ;
#11019=CARTESIAN_POINT ( 'NONE',  ( 178.1946494622069395, 290.5425167686889267, 9.940919530699707352 ) ) ;
#11020=EDGE_CURVE ( 'NONE', #98801, #63065, #24597, .T. ) ;
#11021=CARTESIAN_POINT ( 'NONE',  ( 205.5756302247097267, 274.5795589832478640, -13.28165401105990640 ) ) ;
#11024=CARTESIAN_POINT ( 'NONE',  ( 176.0325359971707542, 265.4089874483971130, -16.36978886597187355 ) ) ;
#11025=CARTESIAN_POINT ( 'NONE',  ( 79.20030167299918844, 216.5333772461660544, 9.188101187500095079 ) ) ;
#11026=CARTESIAN_POINT ( 'NONE',  ( 207.1770866921659717, 271.8057550155037347, -5.569195235244989384 ) ) ;
#11028=CARTESIAN_POINT ( 'NONE',  ( 163.4176914027354997, 257.9558872812714299, 15.60721039003836808 ) ) ;
#11031=CARTESIAN_POINT ( 'NONE',  ( 176.3672203485075727, 269.8998402218351202, -17.39506173205459305 ) ) ;
#11037=CARTESIAN_POINT ( 'NONE',  ( 67.72511797709034909, 222.1589784336661637, -6.496448406907676862E-16 ) ) ;
#11039=CARTESIAN_POINT ( 'NONE',  ( 169.4352824855270399, 288.1566314908686763, -1.095578661510785423 ) ) ;
#11040=CARTESIAN_POINT ( 'NONE',  ( 192.5076277540105423, 297.2140032159341558, -13.10094381206144298 ) ) ;
#11041=CARTESIAN_POINT ( 'NONE',  ( 200.1233510698300222, 282.0231834965481994, 17.42297826929840809 ) ) ;
#11043=CARTESIAN_POINT ( 'NONE',  ( 190.0370014622527322, 286.8089957100377205, 16.96978714573610247 ) ) ;
#11045=CARTESIAN_POINT ( 'NONE',  ( 128.3382222415839919, 238.2365022471902307, 10.00000000000009592 ) ) ;
#11046=CARTESIAN_POINT ( 'NONE',  ( 157.1850763439666139, 258.3944569110938687, -16.98181238659443437 ) ) ;
#11048=VERTEX_POINT ( 'NONE', #34326 ) ;
#11050=CARTESIAN_POINT ( 'NONE',  ( 169.5996950482089574, 248.5186537671148699, -1.940243715008109993 ) ) ;
#11051=VERTEX_POINT ( 'NONE', #96166 ) ;
#11052=CARTESIAN_POINT ( 'NONE',  ( 163.0683798854284703, 248.2042762609320903, 11.26611642476872710 ) ) ;
#11054=EDGE_CURVE ( 'NONE', #87622, #37700, #66227, .T. ) ;
#11058=ORIENTED_EDGE ( 'NONE', *, *, #46785, .F. ) ;
#11060=CARTESIAN_POINT ( 'NONE',  ( 171.2741013746033332, 249.3936815359432728, 2.927055546763141169 ) ) ;
#11061=CARTESIAN_POINT ( 'NONE',  ( 194.1631857443810816, 280.7988080397683461, -17.36965744553461377 ) ) ;
#11062=CARTESIAN_POINT ( 'NONE',  ( 206.7927593038066618, 270.4714295788825780, 5.070506503021109168 ) ) ;
#11065=CARTESIAN_POINT ( 'NONE',  ( 101.5149374161625815, 240.9637435831424739, 2.679491924311251605 ) ) ;
#11070=DIRECTION ( 'NONE',  ( -0.8660254037844387076, -0.4999999999999998890, -0.000000000000000000 ) ) ;
#11071=ORIENTED_EDGE ( 'NONE', *, *, #38649, .T. ) ;
#11072=ORIENTED_EDGE ( 'NONE', *, *, #42172, .T. ) ;
#11075=CARTESIAN_POINT ( 'NONE',  ( 204.2799274532736433, 276.8237820148827950, 13.55359442435934803 ) ) ;
#11076=CARTESIAN_POINT ( 'NONE',  ( 148.3874010092782498, 273.6324775792697892, -8.328854486678444857 ) ) ;
#11079=CARTESIAN_POINT ( 'NONE',  ( 147.5263885827495471, 275.7695129196879975, 0.5021707157977391978 ) ) ;
#11081=CARTESIAN_POINT ( 'NONE',  ( 208.1506335189424988, 270.1195224479792500, -4.283595630760618889 ) ) ;
#11082=CARTESIAN_POINT ( 'NONE',  ( 165.9965283720889033, 265.7099112032472021, 16.66492205199346444 ) ) ;
#11083=AXIS2_PLACEMENT_3D ( 'NONE', #9221, #71039, #62914 ) ;
#11085=CARTESIAN_POINT ( 'NONE',  ( 91.59511671678144751, 229.8149278399160664, 9.188101187500093303 ) ) ;
#11086=ORIENTED_EDGE ( 'NONE', *, *, #45199, .T. ) ;
#11088=CARTESIAN_POINT ( 'NONE',  ( 164.1573742157265201, 276.8569001291454015, -13.59881056395027521 ) ) ;
#11091=VERTEX_POINT ( 'NONE', #88590 ) ;
#11093=CARTESIAN_POINT ( 'NONE',  ( 179.9534164099970042, 293.6013641453405967, -2.637859770436314921 ) ) ;
#11095=CARTESIAN_POINT ( 'NONE',  ( 159.6288139302610887, 254.1617792512662675, -15.32287760493869477 ) ) ;
#11097=CARTESIAN_POINT ( 'NONE',  ( 207.2158346629843493, 271.3235102996118826, -3.977316185394199177 ) ) ;
#11098=CARTESIAN_POINT ( 'NONE',  ( 92.54224522822943300, 233.4244531367911009, -4.594050593750046652 ) ) ;
#11099=EDGE_LOOP ( 'NONE', ( #60262, #82910, #446, #66097, #39169, #34849, #52077, #60581, #17316, #67597, #82421, #61851, #9223, #22280, #88432, #71999, #81239, #32873, #2258, #51299, #94115 ) ) ;
#11102=ORIENTED_EDGE ( 'NONE', *, *, #87841, .T. ) ;
#11104=CARTESIAN_POINT ( 'NONE',  ( 207.5886452961740076, 271.0929146030698007, -1.661373005306138184 ) ) ;
#11106=VERTEX_POINT ( 'NONE', #20136 ) ;
#11109=CARTESIAN_POINT ( 'NONE',  ( 95.19470834736904408, 235.7677522451419065, -5.000000000000047962 ) ) ;
#11112=CARTESIAN_POINT ( 'NONE',  ( 131.1886288721100300, 255.7369531367911293, -4.594050593750048428 ) ) ;
#11114=CARTESIAN_POINT ( 'NONE',  ( -6.130263895410211994, 157.2677522451417929, -5.000000000000041744 ) ) ;
#11116=EDGE_LOOP ( 'NONE', ( #24283, #72862, #51165, #6672, #98904, #71218, #82952, #53057, #53051, #11072, #53929, #70254, #84830, #842, #34249, #72255, #12174, #63011, #22868, #52043, #63053 ) ) ;
#11117=CARTESIAN_POINT ( 'NONE',  ( 156.7786475906069938, 259.0984121615696836, 17.12081851550279055 ) ) ;
#11118=CARTESIAN_POINT ( 'NONE',  ( 160.7433166061900920, 275.5038296165459997, 13.74271022849526780 ) ) ;
#11119=CARTESIAN_POINT ( 'NONE',  ( 159.9770824720811220, 253.5585604421560788, -16.42166711341322483 ) ) ;
#11120=CARTESIAN_POINT ( 'NONE',  ( 191.9985291012005462, 271.7866236224816703, 14.17061973602814007 ) ) ;
#11122=CARTESIAN_POINT ( 'NONE',  ( 187.4676533354318906, 272.4601757945604845, -16.88503403312462936 ) ) ;
#11125=CARTESIAN_POINT ( 'NONE',  ( 161.8662906133268393, 250.2863559554455719, 14.03735902266321744 ) ) ;
#11127=FACE_OUTER_BOUND ( 'NONE', #15410, .T. ) ;
#11130=FACE_OUTER_BOUND ( 'NONE', #95496, .T. ) ;
#11134=CARTESIAN_POINT ( 'NONE',  ( 165.0437781805843258, 244.7827860485373606, -2.050141714668513693 ) ) ;
#11135=CARTESIAN_POINT ( 'NONE',  ( 183.3360699033760568, 264.4351057451253837, 14.27812921404662383 ) ) ;
#11145=( BOUNDED_CURVE ( )  B_SPLINE_CURVE ( 2, ( #49700, #32514, #18322, #87783, #95859, #86264, #25925, #3143, #24900 ),
 .UNSPECIFIED., .F., .T. ) 
 B_SPLINE_CURVE_WITH_KNOTS ( ( 3, 2, 2, 2, 3 ),
 ( 0.3104838709677419373, 0.3118279569892473124, 0.3145161290322580627, 0.3172043010752688130, 0.3185483870967741882 ),
 .UNSPECIFIED. ) 
 CURVE ( )  GEOMETRIC_REPRESENTATION_ITEM ( )  RATIONAL_B_SPLINE_CURVE ( ( 0.9330127018922194093, 0.9330127018922194093, 1.000000000000000000, 0.8660254037844387076, 1.000000000000000000, 0.8660254037844387076, 1.000000000000000000, 0.9330127018922194093, 0.9330127018922194093 ) ) 
 REPRESENTATION_ITEM ( '' )  );
#11146=CARTESIAN_POINT ( 'NONE',  ( 18.14551070619625150, 181.2833772461660544, -9.188101187500095079 ) ) ;
#11148=ORIENTED_EDGE ( 'NONE', *, *, #20412, .F. ) ;
#11151=CARTESIAN_POINT ( 'NONE',  ( 207.9622466093905189, 270.4458181468041289, 3.586592550214158681 ) ) ;
#11153=CARTESIAN_POINT ( 'NONE',  ( 31.35205101814392847, 201.1589784336661353, -6.496448406907676862E-16 ) ) ;
#11156=CARTESIAN_POINT ( 'NONE',  ( 200.8432122835317841, 282.7763473000181307, 17.15137370990203891 ) ) ;
#11157=CARTESIAN_POINT ( 'NONE',  ( 190.1693911629507738, 301.2639477917662703, -5.112716700269980485 ) ) ;
#11159=CARTESIAN_POINT ( 'NONE',  ( 178.2476854491459903, 292.1019644849587849, 5.583694897891509967 ) ) ;
#11160=CARTESIAN_POINT ( 'NONE',  ( 191.1687199697037443, 299.5330595250031820, -8.491751560014430211 ) ) ;
#11161=CARTESIAN_POINT ( 'NONE',  ( 157.7255603307123408, 268.5163524934444013, 16.86592485641857309 ) ) ;
#11162=B_SPLINE_SURFACE_WITH_KNOTS ( 'NONE', 3, 1, ( 
 ( #8399, #45389 ),
 ( #53486, #46892 ),
 ( #14983, #24585 ),
 ( #73211, #9398 ),
 ( #55471, #26105 ),
 ( #64604, #72731 ),
 ( #72218, #2822 ),
 ( #71214, #47873 ),
 ( #87478, #26603 ),
 ( #71722, #55964 ),
 ( #94035, #3321 ),
 ( #57478, #95559 ),
 ( #32689, #56979 ),
 ( #42277, #87965 ),
 ( #63089, #1805 ),
 ( #18509, #88461 ),
 ( #78811, #19021 ),
 ( #94531, #56491 ),
 ( #10909, #96044 ),
 ( #63590, #2314 ),
 ( #40272, #18012 ),
 ( #25083, #49895 ),
 ( #49395, #80853 ),
 ( #80342, #86958 ),
 ( #9912, #33194 ),
 ( #41785, #40770 ),
 ( #17494, #48905 ),
 ( #48399, #34202 ),
 ( #10406, #79345 ),
 ( #11425, #32187 ),
 ( #65092, #64095 ),
 ( #95040, #25604 ),
 ( #79840, #86457 ),
 ( #41276, #16982 ) ),
 .UNSPECIFIED., .T., .F., .F.,
 ( 4, 2, 2, 2, 2, 2, 2, 2, 2, 2, 2, 2, 2, 2, 2, 2, 4 ),
 ( 2, 2 ),
 ( 0.000000000000000000, 0.06250000000000000000, 0.1250000000000000000, 0.1875000000000000000, 0.2500000000000000000, 0.3125000000000000000, 0.3750000000000000000, 0.4375000000000000000, 0.5000000000000000000, 0.5625000000000000000, 0.6250000000000000000, 0.6875000000000000000, 0.7500000000000000000, 0.8125000000000000000, 0.8750000000000000000, 0.9375000000000000000, 1.000000000000000000 ),
 ( 0.000000000000000000, 1.000000000000000000 ),
 .UNSPECIFIED. ) ;
#11163=CARTESIAN_POINT ( 'NONE',  ( 166.0171423212046022, 257.5822672037136272, -15.03208011136822009 ) ) ;
#11165=CARTESIAN_POINT ( 'NONE',  ( 82.29453827371126806, 224.9865022471902876, -10.00000000000009415 ) ) ;
#11166=CARTESIAN_POINT ( 'NONE',  ( 19.05118110555104849, 170.2592609112379876, 2.679491924311254714 ) ) ;
#11167=CARTESIAN_POINT ( 'NONE',  ( 161.5827144264378887, 267.7246213421781249, -17.17800402044808195 ) ) ;
#11168=CARTESIAN_POINT ( 'NONE',  ( 45.10055139898691579, 196.8458772461660544, 9.188101187500095079 ) ) ;
#11169=EDGE_CURVE ( 'NONE', #49174, #86134, #22085, .T. ) ;
#11172=CARTESIAN_POINT ( 'NONE',  ( 150.8168331730346949, 269.4245776381016526, -15.71017957295074652 ) ) ;
#11173=B_SPLINE_CURVE_WITH_KNOTS ( 'NONE', 3,
 ( #20113, #18615, #80449, #3426, #19627, #34301, #96143, #57586, #50002, #79448, #50485, #42868, #73802, #44379, #66688, #67690, #98619, #13993, #91032, #51488, #76307, #13019, #12511, #28690, #82457, #68178, #83427, #4910, #14494, #75811, #28188, #90546, #21116, #59570, #92037, #51994 ),
 .UNSPECIFIED., .F., .F.,
 ( 4, 2, 2, 2, 2, 2, 2, 2, 2, 2, 2, 2, 2, 2, 2, 2, 2, 4 ),
 ( 0.003351528275103934310, 0.003542274814850215284, 0.003637648084723309801, 0.003733021354596404318, 0.003923767894342636287, 0.004114514434088867821, 0.004496007513581369922, 0.004877500593073871155, 0.005640486752058733975, 0.006403472911043596796, 0.007929445229013240906, 0.008120191768759348408, 0.008167878403695857936, 0.008215565038632367464, 0.008310938308505362235, 0.008692431387997369072, 0.009073924467489377643, 0.009455417546981384480 ),
 .UNSPECIFIED. ) ;
#11176=CARTESIAN_POINT ( 'NONE',  ( 167.3544567060031056, 285.1758971363884712, 7.850027993811327320 ) ) ;
#11177=CARTESIAN_POINT ( 'NONE',  ( 207.3502731283117555, 271.5057873089173768, 6.280625384230454245 ) ) ;
#11182=CARTESIAN_POINT ( 'NONE',  ( 172.8753696232004415, 256.4781477760785720, 11.23930794150890478 ) ) ;
#11183=ORIENTED_EDGE ( 'NONE', *, *, #65141, .T. ) ;
#11185=CARTESIAN_POINT ( 'NONE',  ( 171.8846141982767222, 252.9912589899345221, 8.488787739703381519 ) ) ;
#11186=LINE ( 'NONE', #50159, #65098 ) ;
#11189=CARTESIAN_POINT ( 'NONE',  ( -22.42236680055709641, 157.8615022471902591, 0.000000000000000000 ) ) ;
#11194=CARTESIAN_POINT ( 'NONE',  ( 207.1211793645798878, 271.9025893473983047, -6.294110402770905388 ) ) ;
#11195=CARTESIAN_POINT ( 'NONE',  ( 150.9847884352320762, 269.5419465100882803, -13.76858632224513279 ) ) ;
#11196=CARTESIAN_POINT ( 'NONE',  ( 188.2520712372829621, 265.6420100395978920, -13.17850047611677766 ) ) ;
#11197=ORIENTED_EDGE ( 'NONE', *, *, #64448, .T. ) ;
#11200=FACE_OUTER_BOUND ( 'NONE', #439, .T. ) ;
#11203=CARTESIAN_POINT ( 'NONE',  ( 157.0978663001774862, 258.5455091378672137, -17.31223197570816552 ) ) ;
#11204=CARTESIAN_POINT ( 'NONE',  ( 119.9849458542963561, 230.8923013555409796, 4.594050593750050204 ) ) ;
#11208=DIRECTION ( 'NONE',  ( -0.8660254037844387076, -0.4999999999999998890, -0.000000000000000000 ) ) ;
#11210=CARTESIAN_POINT ( 'NONE',  ( 207.7655736232174206, 270.7864657513322300, 3.530742899761726949 ) ) ;
#11215=CARTESIAN_POINT ( 'NONE',  ( 72.70511114461589841, 212.7833772461660544, -9.188101187500095079 ) ) ;
#11217=CARTESIAN_POINT ( 'NONE',  ( 150.8757650385446993, 269.3225046528533539, 14.31332712971473953 ) ) ;
#11219=CARTESIAN_POINT ( 'NONE',  ( 174.2807072416181597, 277.7764784826417213, 15.50750675594299643 ) ) ;
#11220=EDGE_LOOP ( 'NONE', ( #42178, #82154, #19072, #44529 ) ) ;
#11223=CARTESIAN_POINT ( 'NONE',  ( 147.6220714307702622, 274.9580672937808572, 8.392894244419288441 ) ) ;
#11225=CARTESIAN_POINT ( 'NONE',  ( 195.5106104057018968, 292.0126846889568810, 15.81382758565595736 ) ) ;
#11226=CARTESIAN_POINT ( 'NONE',  ( 173.8661040448295694, 278.0172980323289380, -16.69473935971507572 ) ) ;
#11227=CARTESIAN_POINT ( 'NONE',  ( 160.7200862735817850, 258.4377271483461413, -16.74603599744149918 ) ) ;
#11229=CARTESIAN_POINT ( 'NONE',  ( 206.4737064409647189, 270.6076388844679173, 2.372787432230063942 ) ) ;
#11230=CARTESIAN_POINT ( 'NONE',  ( 149.4491471355718772, 271.7934793437897270, 11.43912701239353780 ) ) ;
#11231=B_SPLINE_CURVE_WITH_KNOTS ( 'NONE', 3,
 ( #5105, #39335, #91222, #29397, #21789, #67896, #89746, #28904, #36987, #59781, #82151, #28387, #363, #31250, #35984, #66889 ),
 .UNSPECIFIED., .F., .F.,
 ( 4, 2, 2, 2, 2, 2, 2, 4 ),
 ( 0.000000000000000000, 0.0003786681000626568642, 0.0007573362001253137283, 0.001136004300187970538, 0.001514672400250627457, 0.001893340500313284158, 0.002272008600375941077, 0.003029344800501280934 ),
 .UNSPECIFIED. ) ;
#11232=CARTESIAN_POINT ( 'NONE',  ( 179.4402317224691501, 270.6826544746222112, 16.24075135540241988 ) ) ;
#11233=VECTOR ( 'NONE', #57472, 1000.000000000000000 ) ;
#11234=CARTESIAN_POINT ( 'NONE',  ( 206.0627831668701901, 273.7357853363691902, 10.14454147593459687 ) ) ;
#11236=CARTESIAN_POINT ( 'NONE',  ( 166.6284335572192958, 255.9663351304055539, 13.75844111390426683 ) ) ;
#11237=ORIENTED_EDGE ( 'NONE', *, *, #9305, .F. ) ;
#11238=CARTESIAN_POINT ( 'NONE',  ( 208.3057440179679531, 269.8508631828800617, 2.969924427282375046 ) ) ;
#11239=CARTESIAN_POINT ( 'NONE',  ( 127.7791744883563183, 235.3923013555409796, 4.594050593750050204 ) ) ;
#11244=CARTESIAN_POINT ( 'NONE',  ( 164.4936379324916516, 245.7356569095223051, 6.719479797016231437 ) ) ;
#11247=ORIENTED_EDGE ( 'NONE', *, *, #16841, .T. ) ;
#11249=CARTESIAN_POINT ( 'NONE',  ( 157.9297271802291220, 276.0988248505941556, -12.89341868665208679 ) ) ;
#11251=CARTESIAN_POINT ( 'NONE',  ( 207.0571114767778624, 269.8739652884199245, 1.758464922131628860 ) ) ;
#11252=CARTESIAN_POINT ( 'NONE',  ( 206.4839639422192192, 273.0062788342933118, -11.22308919026441210 ) ) ;
#11253=CARTESIAN_POINT ( 'NONE',  ( 148.2390246527636748, 247.2048013555409511, 4.594050593750051981 ) ) ;
#11255=CARTESIAN_POINT ( 'NONE',  ( 29.55951135474875358, 176.3262482093457777, 3.021315404115420679E-15 ) ) ;
#11257=CARTESIAN_POINT ( 'NONE',  ( 65.53359859134977228, 199.4548013555410080, -4.594050593750042211 ) ) ;
#11258=CARTESIAN_POINT ( 'NONE',  ( 157.6668627405778409, 257.5599783937680058, -16.78811156090270629 ) ) ;
#11259=CARTESIAN_POINT ( 'NONE',  ( 172.5875758667829984, 251.5272254664457989, 3.418950794502710000 ) ) ;
#11261=CARTESIAN_POINT ( 'NONE',  ( 149.0323968763055689, 272.5153119669064949, 11.64231532207353403 ) ) ;
#11262=CARTESIAN_POINT ( 'NONE',  ( 154.9461157776194966, 279.4417561161487242, -1.582898759582469284 ) ) ;
#11263=CARTESIAN_POINT ( 'NONE',  ( 170.6705325584632931, 285.9596063569311468, -7.984020550193259069 ) ) ;
#11265=CARTESIAN_POINT ( 'NONE',  ( 149.0242096487241383, 274.5281563735073860, 9.114748174487145249 ) ) ;
#11266=CARTESIAN_POINT ( 'NONE',  ( 135.3927208396967785, 255.6427522451419065, -10.00000000000009415 ) ) ;
#11271=CARTESIAN_POINT ( 'NONE',  ( 148.1672759425158290, 274.0137453789218398, 7.847779094015780110 ) ) ;
#11272=CARTESIAN_POINT ( 'NONE',  ( -9.188242552867590618, 159.3768266524160140, 9.188101187500096856 ) ) ;
#11274=CARTESIAN_POINT ( 'NONE',  ( 40.49996498926459765, 188.0643266524160140, 9.188101187500095079 ) ) ;
#11276=CARTESIAN_POINT ( 'NONE',  ( 179.3158450784500246, 274.1411853107688898, -17.71003609510279730 ) ) ;
#11279=CARTESIAN_POINT ( 'NONE',  ( 205.0716081116550527, 275.4525508911965517, -12.57761053684872188 ) ) ;
#11280=CARTESIAN_POINT ( 'NONE',  ( 192.6160155272557688, 292.3720383156061757, -14.34532783140716106 ) ) ;
#11281=CARTESIAN_POINT ( 'NONE',  ( 190.2287563641723978, 301.1611242470490311, -4.521471513871881953 ) ) ;
#11283=CARTESIAN_POINT ( 'NONE',  ( 168.9800899256908053, 257.3656399283672727, 13.71095777019204576 ) ) ;
#11284=CARTESIAN_POINT ( 'NONE',  ( 52.25428207639063061, 207.6427522451419350, -10.00000000000009415 ) ) ;
#11287=CARTESIAN_POINT ( 'NONE',  ( 162.1789081252419464, 251.9841321976889503, -13.95467832899616845 ) ) ;
#11288=EDGE_CURVE ( 'NONE', #14234, #2713, #77731, .T. ) ;
#11290=CARTESIAN_POINT ( 'NONE',  ( 32.13723363786251497, 199.3615022471903160, 5.000000000000046185 ) ) ;
#11291=DIRECTION ( 'NONE',  ( 0.4999999999999998890, -0.8660254037844387076, 0.000000000000000000 ) ) ;
#11292=CARTESIAN_POINT ( 'NONE',  ( 203.0507839702407580, 278.9527209772879814, 16.21318481136342626 ) ) ;
#11293=CARTESIAN_POINT ( 'NONE',  ( -3.911334118262431936, 177.7369531367911293, -4.594050593750048428 ) ) ;
#11295=CARTESIAN_POINT ( 'NONE',  ( 164.8761197389183906, 246.7675571797174428, 5.899305509596029395 ) ) ;
#11297=CARTESIAN_POINT ( 'NONE',  ( 192.8132846206021611, 296.6845899933152850, 11.53748932578252351 ) ) ;
#11299=B_SPLINE_CURVE_WITH_KNOTS ( 'NONE', 3,
 ( #23719, #63739, #63236, #9558, #32334, #94178, #94674, #55119, #39910, #24729, #78456, #10048, #40421, #55613, #86596, #71354, #93168, #1946, #25231, #87109, #17647, #62720, #8541, #25755, #71859, #86105, #64235, #38924, #54613, #85597, #48545, #79485, #2456, #16632, #95185, #31818, #77455, #85072, #15619, #440, #46518, #31329, #16137, #47035, #77952, #39413, #70328, #93677, #24242, #18653, #80485, #50521 ),
 .UNSPECIFIED., .F., .F.,
 ( 4, 2, 2, 2, 2, 2, 2, 2, 2, 2, 2, 2, 2, 2, 2, 2, 2, 2, 2, 2, 2, 2, 2, 2, 2, 4 ),
 ( 0.001762225997650664847, 0.002214759945835987828, 0.002667293894021311243, 0.002780427381067715822, 0.002893560868114120836, 0.003006694355160525849, 0.003119827842206930428, 0.003346094816299740454, 0.003572361790392550480, 0.004024895738578136706, 0.004477429686763722064, 0.005382497583134956097, 0.006287565479506190130, 0.006740099427691806713, 0.007192633375877425031, 0.007305766862923767160, 0.007362333606446948633, 0.007418900349970128372, 0.007532033837016489583, 0.007645167324062849060, 0.007871434298155587095, 0.008097701272248325130, 0.008323968246341063165, 0.008550235220433801200, 0.008776502194526539236, 0.009002769168619277271 ),
 .UNSPECIFIED. ) ;
#11301=CARTESIAN_POINT ( 'NONE',  ( 179.3456124633583499, 277.5962114444210442, 17.35945876020667100 ) ) ;
#11304=CARTESIAN_POINT ( 'NONE',  ( 179.5567261186911594, 262.6765698908865829, -12.85373963981448497 ) ) ;
#11307=CARTESIAN_POINT ( 'NONE',  ( 125.9386101817166974, 233.5177522451417929, 5.000000000000051514 ) ) ;
#11310=CARTESIAN_POINT ( 'NONE',  ( 158.9661858079439298, 259.3592988854380224, 16.70105242487986530 ) ) ;
#11312=CARTESIAN_POINT ( 'NONE',  ( 111.0177141658951854, 228.2365022471901739, -10.00000000000009237 ) ) ;
#11315=ORIENTED_EDGE ( 'NONE', *, *, #75108, .T. ) ;
#11317=CARTESIAN_POINT ( 'NONE',  ( 207.4285356523023154, 271.3702326410368642, 7.833982582429932506 ) ) ;
#11322=CARTESIAN_POINT ( 'NONE',  ( 159.6251152260277308, 278.4128260634272465, -9.785471751044605426 ) ) ;
#11330=CARTESIAN_POINT ( 'NONE',  ( 85.25577013208754806, 208.4824982072973967, 3.021315404115420679E-15 ) ) ;
#11331=CARTESIAN_POINT ( 'NONE',  ( 149.6564118588553924, 271.4344863124460971, -11.76165597393390172 ) ) ;
#11332=CARTESIAN_POINT ( 'NONE',  ( 43.80257615421894712, 184.5494855054052152, -2.679491924311248496 ) ) ;
#11334=CARTESIAN_POINT ( 'NONE',  ( 161.8662906133268393, 250.2863559554455719, 14.03735902266321744 ) ) ;
#11335=CARTESIAN_POINT ( 'NONE',  ( 166.0972222936661638, 274.0867323433699880, -15.20829511115417887 ) ) ;
#11338=EDGE_CURVE ( 'NONE', #48833, #89111, #90574, .T. ) ;
#11340=CARTESIAN_POINT ( 'NONE',  ( 174.6263263390559928, 276.7176742049951486, -16.26821278762835732 ) ) ;
#11341=CARTESIAN_POINT ( 'NONE',  ( 163.4260108471723640, 247.5848412648317662, 10.45113099391573108 ) ) ;
#11343=CARTESIAN_POINT ( 'NONE',  ( 159.4451596000803306, 268.2047196561628084, -16.33042910166371442 ) ) ;
#11347=CARTESIAN_POINT ( 'NONE',  ( 168.8123838728505177, 272.7757763755409997, 16.00497778368365331 ) ) ;
#11348=CARTESIAN_POINT ( 'NONE',  ( 147.1674053649995528, 275.7455720201731424, 6.878590988502374159 ) ) ;
#11349=CARTESIAN_POINT ( 'NONE',  ( 177.3345340752408674, 288.7672428955659711, -10.08588367977367461 ) ) ;
#11351=CARTESIAN_POINT ( 'NONE',  ( 193.5315086250829211, 294.9135581674226501, 13.30815287220877607 ) ) ;
#11354=EDGE_CURVE ( 'NONE', #71188, #54504, #41461, .T. ) ;
#11355=CARTESIAN_POINT ( 'NONE',  ( 197.0726333729855639, 289.3071815470320303, -18.06554324141507095 ) ) ;
#11357=CARTESIAN_POINT ( 'NONE',  ( 100.3908607700757472, 218.7677522451417644, -5.000000000000041744 ) ) ;
#11359=CARTESIAN_POINT ( 'NONE',  ( 164.3022921857394749, 246.0670774647090582, 1.862798784958315856 ) ) ;
#11361=CARTESIAN_POINT ( 'NONE',  ( 206.4943150373521803, 272.9883502116088039, 11.34100825923693101 ) ) ;
#11362=CARTESIAN_POINT ( 'NONE',  ( 198.6562788533279615, 286.5642271139020636, 17.47134757795404525 ) ) ;
#11366=CARTESIAN_POINT ( 'NONE',  ( 190.3324536135930600, 300.9815153424474374, 5.885744744784173754 ) ) ;
#11367=CARTESIAN_POINT ( 'NONE',  ( 171.5022402205397611, 259.7078029901424543, -14.90461411186678475 ) ) ;
#11370=CARTESIAN_POINT ( 'NONE',  ( 119.8042635715768540, 246.6427522451419065, -10.00000000000009592 ) ) ;
#11371=B_SPLINE_CURVE_WITH_KNOTS ( 'NONE', 3,
 ( #81960, #74353, #89574, #12037 ),
 .UNSPECIFIED., .F., .F.,
 ( 4, 4 ),
 ( 0.01060329708585674990, 0.01613402798502076851 ),
 .UNSPECIFIED. ) ;
#11372=CARTESIAN_POINT ( 'NONE',  ( 160.5669369365265027, 252.5369025406650678, -14.88991766242778247 ) ) ;
#11373=CARTESIAN_POINT ( 'NONE',  ( 148.6789780052693004, 273.1274514078948528, -9.289896596434795484 ) ) ;
#11376=LINE ( 'NONE', #80287, #25139 ) ;
#11378=DIRECTION ( 'NONE',  ( 0.4999999999999998890, -0.8660254037844385966, 0.000000000000000000 ) ) ;
#11380=CARTESIAN_POINT ( 'NONE',  ( 41.14028939449039513, 187.8927522451418213, 10.00000000000009592 ) ) ;
#11381=CARTESIAN_POINT ( 'NONE',  ( 99.93095832397169431, 222.3768266524160140, 9.188101187500096856 ) ) ;
#11383=CARTESIAN_POINT ( 'NONE',  ( 183.6498318386265396, 256.3252116762061519, 1.424693195823348635 ) ) ;
#11384=CARTESIAN_POINT ( 'NONE',  ( 161.3981413584396876, 253.0972142504356270, -15.11937522241654719 ) ) ;
#11385=CARTESIAN_POINT ( 'NONE',  ( 19.90436448580963713, 191.4869531367911293, 4.594050593750046652 ) ) ;
#11387=EDGE_LOOP ( 'NONE', ( #83839, #16448, #80694, #92794 ) ) ;
#11389=CARTESIAN_POINT ( 'NONE',  ( 185.5167381441177099, 260.1903814095311986, -5.802878996917316456 ) ) ;
#11391=CARTESIAN_POINT ( 'NONE',  ( 193.2033031094106263, 263.3857463355129198, -3.783757748560594880 ) ) ;
#11392=CARTESIAN_POINT ( 'NONE',  ( 207.2167723318516153, 271.7370174712370954, -6.606038862010207957 ) ) ;
#11393=CARTESIAN_POINT ( 'NONE',  ( 181.8935795008488867, 285.0832480758294309, 15.32078685669571882 ) ) ;
#11394=CARTESIAN_POINT ( 'NONE',  ( 168.1183126599903517, 251.5151909822113225, 10.70881076761038031 ) ) ;
#11395=CARTESIAN_POINT ( 'NONE',  ( 51.37958267218910180, 188.2202760586659451, -5.415160957724236172E-17 ) ) ;
#11396=CARTESIAN_POINT ( 'NONE',  ( 80.97745796857449818, 230.8927522451419350, 2.944929066748280225E-16 ) ) ;
#11398=CARTESIAN_POINT ( 'NONE',  ( 178.7556533234623544, 259.1617598374694467, -10.24969492202171750 ) ) ;
#11399=EDGE_CURVE ( 'NONE', #52618, #31479, #39112, .T. ) ;
#11400=CARTESIAN_POINT ( 'NONE',  ( -1.069254392388470976, 164.0643266524160140, 9.188101187500095079 ) ) ;
#11402=CARTESIAN_POINT ( 'NONE',  ( 151.0013883899287066, 269.1049186256390726, -14.25461351222133466 ) ) ;
#11404=CARTESIAN_POINT ( 'NONE',  ( 147.5749551500760788, 275.0396750858066639, -4.254929048021584670 ) ) ;
#11406=CARTESIAN_POINT ( 'NONE',  ( 179.4583960273904211, 270.4090523040318885, 17.47970616590194837 ) ) ;
#11407=CARTESIAN_POINT ( 'NONE',  ( 204.9004517216375518, 275.7490024547470853, 14.55104398969427670 ) ) ;
#11408=CARTESIAN_POINT ( 'NONE',  ( 73.27344031762339682, 213.1115022471902591, 10.00000000000009592 ) ) ;
#11411=CARTESIAN_POINT ( 'NONE',  ( 207.6471633721571379, 270.9915583223058206, 2.196965492132801678 ) ) ;
#11412=CARTESIAN_POINT ( 'NONE',  ( 0.02212491418958350761, 177.4865022471903160, 10.00000000000009237 ) ) ;
#11414=CARTESIAN_POINT ( 'NONE',  ( 116.8724067376222706, 238.2833772461660544, -9.188101187500095079 ) ) ;
#11418=AXIS2_PLACEMENT_3D ( 'NONE', #53449, #53935, #15953 ) ;
#11420=CARTESIAN_POINT ( 'NONE',  ( 196.4994169513186364, 290.3000215130921902, 16.82935102260526961 ) ) ;
#11421=CYLINDRICAL_SURFACE ( 'NONE', #61886, 17.82106496071139645 ) ;
#11422=CARTESIAN_POINT ( 'NONE',  ( 190.7283684373172434, 300.2957707522874102, -6.596676114545077851 ) ) ;
#11424=CARTESIAN_POINT ( 'NONE',  ( 151.3284628043366524, 268.5384091220288383, 14.49047510809488237 ) ) ;
#11425=CARTESIAN_POINT ( 'NONE',  ( 196.3174919959537306, 290.6151247789487684, -17.61248417473235151 ) ) ;
#11426=CARTESIAN_POINT ( 'NONE',  ( 190.4273386993099280, 300.1655951281246075, 3.362114210485594779 ) ) ;
#11427=CARTESIAN_POINT ( 'NONE',  ( 173.0801454197684279, 289.8428614808497059, -1.592028862751424301 ) ) ;
#11430=CARTESIAN_POINT ( 'NONE',  ( 189.0071503145738632, 265.7560967367359694, 11.07595847811888135 ) ) ;
#11431=CARTESIAN_POINT ( 'NONE',  ( 165.4151454494500513, 269.5741751986499253, -16.33037408709135008 ) ) ;
#11432=EDGE_CURVE ( 'NONE', #36629, #21068, #382, .T. ) ;
#11433=EDGE_CURVE ( 'NONE', #55151, #19809, #18518, .T. ) ;
#11439=CARTESIAN_POINT ( 'NONE',  ( 148.0764158854584593, 274.5517338476317946, 6.287425945023585427 ) ) ;
#11440=CARTESIAN_POINT ( 'NONE',  ( 194.3471816728315673, 282.8997524079796904, 17.29725935490247579 ) ) ;
#11442=CARTESIAN_POINT ( 'NONE',  ( 174.5819976565091736, 273.2228988371514333, -16.37309483920122943 ) ) ;
#11443=ORIENTED_EDGE ( 'NONE', *, *, #54849, .F. ) ;
#11445=CARTESIAN_POINT ( 'NONE',  ( 147.8819534105757043, 274.5079385007862811, -9.338341377131436971 ) ) ;
#11449=CARTESIAN_POINT ( 'NONE',  ( 184.9969017503452164, 291.7732855071091649, 12.02731214230744428 ) ) ;
#11450=VERTEX_POINT ( 'NONE', #85459 ) ;
#11453=CARTESIAN_POINT ( 'NONE',  ( 185.0543182570741294, 259.9533911388629690, -5.863674189508556900 ) ) ;
#11454=ORIENTED_EDGE ( 'NONE', *, *, #45369, .F. ) ;
#11457=VERTEX_POINT ( 'NONE', #1819 ) ;
#11458=CARTESIAN_POINT ( 'NONE',  ( 175.8048057498829735, 259.3838861800913946, 12.42913708267750472 ) ) ;
#11460=FACE_BOUND ( 'NONE', #36476, .T. ) ;
#11461=ORIENTED_EDGE ( 'NONE', *, *, #60254, .T. ) ;
#11463=CARTESIAN_POINT ( 'NONE',  ( 203.4682009197399566, 278.2297336128146412, -15.36039508894693206 ) ) ;
#11466=CARTESIAN_POINT ( 'NONE',  ( 182.9784873362611961, 280.4349440833490235, -16.11357538915770604 ) ) ;
#11467=( BOUNDED_CURVE ( )  B_SPLINE_CURVE ( 2, ( #94288, #40028, #93794, #70968, #56237, #87230, #69936, #17764, #1570 ),
 .UNSPECIFIED., .F., .T. ) 
 B_SPLINE_CURVE_WITH_KNOTS ( ( 3, 2, 2, 2, 3 ),
 ( 0.6008064516129032473, 0.6021505376344086224, 0.6048387096774193727, 0.6075268817204301230, 0.6088709677419354982 ),
 .UNSPECIFIED. ) 
 CURVE ( )  GEOMETRIC_REPRESENTATION_ITEM ( )  RATIONAL_B_SPLINE_CURVE ( ( 0.9330127018922194093, 0.9330127018922194093, 1.000000000000000000, 0.8660254037844387076, 1.000000000000000000, 0.8660254037844387076, 1.000000000000000000, 0.9330127018922194093, 0.9330127018922194093 ) ) 
 REPRESENTATION_ITEM ( '' )  );
#11469=CARTESIAN_POINT ( 'NONE',  ( 151.5020479237435609, 268.6693028843759521, 14.46568410587973652 ) ) ;
#11470=CARTESIAN_POINT ( 'NONE',  ( 160.7509603171012031, 276.3162894764463431, -12.59630221962144958 ) ) ;
#11471=CARTESIAN_POINT ( 'NONE',  ( 193.0065576635309412, 296.3498312632291913, -11.90044991639595295 ) ) ;
#11472=CARTESIAN_POINT ( 'NONE',  ( 152.6621968174709991, 266.2283140474973493, -17.02835521334403168 ) ) ;
#11476=CARTESIAN_POINT ( 'NONE',  ( 144.5855667544892924, 242.0327760586659451, 1.948934522072303157E-15 ) ) ;
#11482=EDGE_LOOP ( 'NONE', ( #47390, #93843, #95824, #39453, #50357 ) ) ;
#11484=DIRECTION ( 'NONE',  ( 0.4999999999999992784, -0.8660254037844390407, 0.000000000000000000 ) ) ;
#11485=CARTESIAN_POINT ( 'NONE',  ( 128.9696990949622659, 235.2677522451417929, -5.000000000000041744 ) ) ;
#11486=CARTESIAN_POINT ( 'NONE',  ( 157.3343857493933058, 280.1478128481105045, -6.988461411397997480 ) ) ;
#11487=CARTESIAN_POINT ( 'NONE',  ( 34.98558885611105751, 202.5530062829863027, -4.648177544792955347E-16 ) ) ;
#11488=CARTESIAN_POINT ( 'NONE',  ( 176.2024152284932370, 253.2971236404176238, 6.345151448921726001 ) ) ;
#11491=ORIENTED_EDGE ( 'NONE', *, *, #50591, .F. ) ;
#11492=CARTESIAN_POINT ( 'NONE',  ( 184.3893518601747417, 272.5925419477008518, -17.24544351097261696 ) ) ;
#11494=ORIENTED_EDGE ( 'NONE', *, *, #31829, .F. ) ;
#11495=CARTESIAN_POINT ( 'NONE',  ( 162.1283350843791311, 276.5786735129873932, 12.83412388560665285 ) ) ;
#11497=CARTESIAN_POINT ( 'NONE',  ( 156.6021870925794133, 276.9767950607789544, 9.957507455165190535 ) ) ;
#11499=CARTESIAN_POINT ( 'NONE',  ( 149.6700657135140489, 271.4108371424580355, 12.58635654151485284 ) ) ;
#11500=CARTESIAN_POINT ( 'NONE',  ( 162.9796882977680639, 248.3578945969637743, 9.683801903336119565 ) ) ;
#11501=CARTESIAN_POINT ( 'NONE',  ( 171.7948998666937541, 269.4667684067869686, 17.81952346552377620 ) ) ;
#11503=CARTESIAN_POINT ( 'NONE',  ( 67.06923665261433598, 197.9824982072973967, 3.021315404115420679E-15 ) ) ;
#11504=ORIENTED_EDGE ( 'NONE', *, *, #52956, .F. ) ;
#11508=CARTESIAN_POINT ( 'NONE',  ( 192.7944000592152634, 296.7172990131160759, 11.44860011299869740 ) ) ;
#11510=CARTESIAN_POINT ( 'NONE',  ( 110.3297989853572005, 246.0530062829863311, -4.648177544792955347E-16 ) ) ;
#11511=CARTESIAN_POINT ( 'NONE',  ( 7.238742955462222461, 184.1744531367911293, 4.594050593750047540 ) ) ;
#11512=CARTESIAN_POINT ( 'NONE',  ( 104.8563042601131770, 231.3458772461660544, 9.188101187500095079 ) ) ;
#11513=CARTESIAN_POINT ( 'NONE',  ( 154.8545429534089237, 262.4310591522755089, -17.81746354318405778 ) ) ;
#11515=CARTESIAN_POINT ( 'NONE',  ( 186.7639553457436534, 295.8781545368645425, -7.658116578984559553 ) ) ;
#11516=CARTESIAN_POINT ( 'NONE',  ( -2.503782513514959174, 159.3615022471902023, 5.000000000000051514 ) ) ;
#11517=LINE ( 'NONE', #81434, #36087 ) ;
#11518=CARTESIAN_POINT ( 'NONE',  ( 163.4597682148788920, 284.3339965611676803, 5.988904932330388675 ) ) ;
#11519=CARTESIAN_POINT ( 'NONE',  ( 194.4826705584825390, 293.7931287314651740, -16.11258321617245315 ) ) ;
#11520=CARTESIAN_POINT ( 'NONE',  ( 181.8379482810746879, 291.5118755679804963, 9.487367419015216186 ) ) ;
#11521=CARTESIAN_POINT ( 'NONE',  ( 164.7432774000302800, 245.3032686681709720, -5.267720626764685221 ) ) ;
#11524=CARTESIAN_POINT ( 'NONE',  ( 172.9438399295877957, 262.8668947608421718, -16.49499919880818766 ) ) ;
#11525=CARTESIAN_POINT ( 'NONE',  ( 86.99453030705913648, 221.0333772461660544, 9.188101187500095079 ) ) ;
#11526=CARTESIAN_POINT ( 'NONE',  ( 207.8996209429610360, 270.5542889829179103, -5.987818313449536411 ) ) ;
#11530=CARTESIAN_POINT ( 'NONE',  ( 195.6986305151803549, 291.6870243064952888, 16.84182339398051909 ) ) ;
#11531=CARTESIAN_POINT ( 'NONE',  ( 151.0388915836658725, 269.0399611886400635, -14.24896787280406585 ) ) ;
#11532=CARTESIAN_POINT ( 'NONE',  ( 173.1967572896427043, 268.2116334800467143, -16.29158950216322665 ) ) ;
#11534=CARTESIAN_POINT ( 'NONE',  ( 128.5163324648304410, 256.5530062829863027, -4.648177544792955347E-16 ) ) ;
#11535=CARTESIAN_POINT ( 'NONE',  ( 129.0599100780709421, 251.9865022471902876, -10.00000000000009592 ) ) ;
#11538=CARTESIAN_POINT ( 'NONE',  ( 75.14063404487711750, 220.3149278399160664, -9.188101187500095079 ) ) ;
#11539=CARTESIAN_POINT ( 'NONE',  ( 173.0274122914222517, 289.6322751625752403, -1.044431133429226000 ) ) ;
#11541=CARTESIAN_POINT ( 'NONE',  ( 191.3058253459265075, 288.7823831380905517, -16.22814272653723933 ) ) ;
#11543=EDGE_CURVE ( 'NONE', #23912, #41184, #48452, .T. ) ;
#11545=CARTESIAN_POINT ( 'NONE',  ( 193.7119801207757064, 288.2734703750227823, 16.20783580877855456 ) ) ;
#11547=CARTESIAN_POINT ( 'NONE',  ( 126.6061714340151241, 237.2365022471902023, -10.00000000000009059 ) ) ;
#11551=CARTESIAN_POINT ( 'NONE',  ( 165.5623119752849846, 246.9337586618608498, -1.855523153196440234 ) ) ;
#11552=ORIENTED_EDGE ( 'NONE', *, *, #35650, .T. ) ;
#11553=CARTESIAN_POINT ( 'NONE',  ( 202.2773826701151165, 280.2922913237452462, 16.62862787739668846 ) ) ;
#11559=CARTESIAN_POINT ( 'NONE',  ( 188.9581516566892674, 290.6722666539587863, 14.45932873867149482 ) ) ;
#11561=CARTESIAN_POINT ( 'NONE',  ( 143.8814004702669536, 260.0024278399161517, 9.188101187500095079 ) ) ;
#11563=CARTESIAN_POINT ( 'NONE',  ( 201.6662765003921152, 274.8599008263099677, -14.23589684381435738 ) ) ;
#11565=CYLINDRICAL_SURFACE ( 'NONE', #60723, 17.82106496071139645 ) ;
#11566=CARTESIAN_POINT ( 'NONE',  ( 168.1726423428391399, 255.4859975196775963, 14.21197738914692366 ) ) ;
#11567=CARTESIAN_POINT ( 'NONE',  ( 45.92147131476482969, 203.9865022471903160, -10.00000000000009592 ) ) ;
#11570=EDGE_LOOP ( 'NONE', ( #15358, #60350, #81884, #54239 ) ) ;
#11571=CARTESIAN_POINT ( 'NONE',  ( 184.2559797716583603, 296.4936185974571572, 1.018868464677917363 ) ) ;
#11573=CARTESIAN_POINT ( 'NONE',  ( 204.4781092559247782, 276.4805210635553863, 13.30606382016679490 ) ) ;
#11574=CARTESIAN_POINT ( 'NONE',  ( 194.6310785344323904, 293.5360785768717165, -14.54510914272505495 ) ) ;
#11576=CARTESIAN_POINT ( 'NONE',  ( 201.3394753198586500, 274.7605675011590733, -14.24554608861767946 ) ) ;
#11577=CARTESIAN_POINT ( 'NONE',  ( 147.6453533338496129, 276.1788777465205840, 0.8289047639747788576 ) ) ;
#11578=CARTESIAN_POINT ( 'NONE',  ( 157.7593757092099906, 257.3997412317380054, -18.08445832352326121 ) ) ;
#11579=CARTESIAN_POINT ( 'NONE',  ( -27.42236680055714260, 166.5217562850347406, 1.224646799147364892E-15 ) ) ;
#11580=CARTESIAN_POINT ( 'NONE',  ( 168.2018854272548083, 266.5653299185787546, 16.61820373829572617 ) ) ;
#11581=CARTESIAN_POINT ( 'NONE',  ( 179.6412324868688302, 256.3037255040319451, 4.896461366237743640 ) ) ;
#11583=CARTESIAN_POINT ( 'NONE',  ( 103.5572661544365332, 230.5958772461660260, -9.188101187500095079 ) ) ;
#11584=ORIENTED_EDGE ( 'NONE', *, *, #12887, .T. ) ;
#11586=CARTESIAN_POINT ( 'NONE',  ( 163.3044915899828879, 276.5565773319555660, -13.83122682706599704 ) ) ;
#11588=ORIENTED_EDGE ( 'NONE', *, *, #4795, .T. ) ;
#11591=CARTESIAN_POINT ( 'NONE',  ( 176.8027066500977469, 292.5242457368331657, -2.743196636303242730 ) ) ;
#11593=CARTESIAN_POINT ( 'NONE',  ( 206.6298919378964740, 272.7535241315335384, -9.267551915974392429 ) ) ;
#11594=CARTESIAN_POINT ( 'NONE',  ( 208.2995279947827783, 269.8616296508574237, 2.738519832864397152 ) ) ;
#11595=CARTESIAN_POINT ( 'NONE',  ( 95.14032143958276322, 234.9244531367911009, -4.594050593750046652 ) ) ;
#11597=B_SPLINE_CURVE_WITH_KNOTS ( 'NONE', 3,
 ( #72277, #55039, #55527, #87021, #86020, #2373, #17552, #54523, #85504, #70243, #33251, #64152, #95103, #848, #16546, #62127, #48459, #32746, #78371, #56547, #8454, #31241, #16051, #87534, #18066, #8952, #48962, #41337, #93075, #39819, #46952, #79401, #1862, #17044, #39326, #32248, #70751, #47442, #1364, #47935, #63148, #40333, #71272, #73265, #97099, #12975, #49955, #57539 ),
 .UNSPECIFIED., .F., .F.,
 ( 4, 2, 2, 2, 2, 2, 2, 2, 2, 2, 2, 2, 2, 2, 2, 2, 2, 2, 2, 2, 2, 2, 2, 4 ),
 ( 0.0002509531133599470203, 0.0007282208505926920017, 0.001205488587825436983, 0.001444122456441809419, 0.001563439390749959967, 0.001682756325058110732, 0.001802073259366261280, 0.001921390193674411828, 0.002160024062290898106, 0.002637291799524055409, 0.003114559536757212713, 0.004069095011223527319, 0.005023630485689842794, 0.005500898222923000097, 0.005739532091539544488, 0.005978165960156088012, 0.006037824427310304123, 0.006097482894464520235, 0.006216799828772952459, 0.006455433697389797824, 0.006932701434623462534, 0.007409969171857128112, 0.007648603040473891945, 0.007887236909090657513 ),
 .UNSPECIFIED. ) ;
#11602=CARTESIAN_POINT ( 'NONE',  ( 194.6936158627724751, 266.3821769738702869, -7.823464608937872988 ) ) ;
#11603=DIRECTION ( 'NONE',  ( -0.8660254037844387076, -0.4999999999999998890, -0.000000000000000000 ) ) ;
#11605=CARTESIAN_POINT ( 'NONE',  ( 134.5719744753492364, 242.3768266524159856, -9.188101187500091527 ) ) ;
#11607=CARTESIAN_POINT ( 'NONE',  ( -16.52256874082355864, 171.2677522451419350, -5.000000000000047962 ) ) ;
#11609=ORIENTED_EDGE ( 'NONE', *, *, #90867, .T. ) ;
#11610=CARTESIAN_POINT ( 'NONE',  ( 204.3531539698473978, 276.6969499677158524, 13.47943239092699841 ) ) ;
#11611=CARTESIAN_POINT ( 'NONE',  ( 160.7477323183478006, 275.4922477318379492, 13.14247883376535420 ) ) ;
#11613=CARTESIAN_POINT ( 'NONE',  ( 189.3527614026753270, 269.6247310899153149, 15.08597367144959733 ) ) ;
#11614=CARTESIAN_POINT ( 'NONE',  ( 178.5210264805825204, 285.2939240913069625, 14.13561587336957359 ) ) ;
#11616=CARTESIAN_POINT ( 'NONE',  ( 188.3784916956350344, 286.3721210266486992, -16.81851773412965301 ) ) ;
#11617=CARTESIAN_POINT ( 'NONE',  ( 123.8637576553643100, 248.9865022471902876, -10.00000000000009592 ) ) ;
#11618=CARTESIAN_POINT ( 'NONE',  ( 161.6256441450323678, 250.7031678651938762, 14.48526717260977037 ) ) ;
#11620=CARTESIAN_POINT ( 'NONE',  ( 206.8659638600981623, 272.3446355680395641, -10.26115277030573125 ) ) ;
#11622=CARTESIAN_POINT ( 'NONE',  ( 163.2256942281324541, 247.9317998266098471, -9.780520296312531059 ) ) ;
#11627=CARTESIAN_POINT ( 'NONE',  ( 182.5610248314471846, 264.1229073254193622, 14.12000187221130609 ) ) ;
#11630=CYLINDRICAL_SURFACE ( 'NONE', #87130, 10.00000000000010658 ) ;
#11632=CARTESIAN_POINT ( 'NONE',  ( 157.6156715759294116, 270.9999693453487453, -14.72877181860486751 ) ) ;
#11635=CARTESIAN_POINT ( 'NONE',  ( 161.0974665087481981, 251.6179983666593216, -13.69252715295363210 ) ) ;
#11636=B_SPLINE_CURVE_WITH_KNOTS ( 'NONE', 3,
 ( #40660, #3207, #71597, #2193 ),
 .UNSPECIFIED., .F., .F.,
 ( 4, 4 ),
 ( 0.008328144461416385133, 0.01467133638754275146 ),
 .UNSPECIFIED. ) ;
#11637=CARTESIAN_POINT ( 'NONE',  ( 11.37951369124782453, 183.5024278399160949, 9.188101187500095079 ) ) ;
#11638=CARTESIAN_POINT ( 'NONE',  ( 41.52713374746741692, 206.3297689869269220, -2.679491924311252493 ) ) ;
#11642=CARTESIAN_POINT ( 'NONE',  ( 163.8947349411736525, 246.7729873192901664, -5.868803394723933309 ) ) ;
#11644=CARTESIAN_POINT ( 'NONE',  ( 36.00728465925030974, 191.5958772461660544, -9.188101187500095079 ) ) ;
#11646=CARTESIAN_POINT ( 'NONE',  ( 190.8907028847385448, 300.0145992415348815, -5.421341690443150618 ) ) ;
#11648=CARTESIAN_POINT ( 'NONE',  ( 199.5283806629861942, 267.5346968016396545, -6.617246389697492681 ) ) ;
#11649=CARTESIAN_POINT ( 'NONE',  ( 178.8515547497951559, 293.8219541337840042, 2.692371752549619135 ) ) ;
#11650=CARTESIAN_POINT ( 'NONE',  ( 179.1981449177366130, 278.3664918542738747, -16.54318165528815143 ) ) ;
#11652=CARTESIAN_POINT ( 'NONE',  ( 166.9996108681188218, 257.9679880018421159, -15.33282310006317495 ) ) ;
#11656=CARTESIAN_POINT ( 'NONE',  ( 75.36633504343573975, 220.9865022471902876, 10.00000000000009237 ) ) ;
#11660=CARTESIAN_POINT ( 'NONE',  ( 35.05980905203730913, 200.2369531367911293, -4.594050593750048428 ) ) ;
#11662=CARTESIAN_POINT ( 'NONE',  ( 162.6118520434669392, 263.2546530415788766, 17.62269466845149068 ) ) ;
#11663=CARTESIAN_POINT ( 'NONE',  ( 150.6386650955079176, 269.7331738006648720, -15.06054658539322766 ) ) ;
#11666=B_SPLINE_CURVE_WITH_KNOTS ( 'NONE', 3,
 ( #15616, #92669, #939, #9035, #84576, #37912, #68822, #70840, #46514, #77452, #77949, #8048, #93674, #24238, #47525, #78453 ),
 .UNSPECIFIED., .F., .F.,
 ( 4, 2, 2, 2, 2, 2, 2, 4 ),
 ( 8.537055041414144432E-15, 0.0005636500808654369178, 0.0008454751212938848128, 0.001127300161722332708, 0.001409125202150780711, 0.001690950242579228715, 0.001972775283007676718, 0.002254600323436124504 ),
 .UNSPECIFIED. ) ;
#11667=CARTESIAN_POINT ( 'NONE',  ( 171.2998820311650263, 286.5525287771079661, 7.511819249465659709 ) ) ;
#11668=CARTESIAN_POINT ( 'NONE',  ( 207.1601050488701503, 271.8351680844880889, 6.320235450527015075 ) ) ;
#11669=CARTESIAN_POINT ( 'NONE',  ( 159.7654401674316205, 278.6271376734871978, -10.85853086775617449 ) ) ;
#11671=CARTESIAN_POINT ( 'NONE',  ( 189.0745626194224087, 265.5475558152633653, 10.70054544839699773 ) ) ;
#11672=CARTESIAN_POINT ( 'NONE',  ( 154.0986224399686648, 280.1916420498395155, 2.233781007141098396 ) ) ;
#11673=CARTESIAN_POINT ( 'NONE',  ( 171.3843415847181291, 255.6973737389273253, 11.29858615387269083 ) ) ;
#11680=VERTEX_POINT ( 'NONE', #91428 ) ;
#11682=CARTESIAN_POINT ( 'NONE',  ( 191.5694459269389824, 298.8389818071599962, 7.944420692511652504 ) ) ;
#11686=EDGE_CURVE ( 'NONE', #92439, #41192, #40701, .T. ) ;
#11687=CARTESIAN_POINT ( 'NONE',  ( 161.0974665087481981, 251.6179983666593216, -13.69252715295363210 ) ) ;
#11688=CARTESIAN_POINT ( 'NONE',  ( 150.9356804500963278, 270.2479074161392987, -13.67838782973983669 ) ) ;
#11690=CARTESIAN_POINT ( 'NONE',  ( 179.4404154152157105, 291.3709498135804097, -10.08759257512885199 ) ) ;
#11693=CARTESIAN_POINT ( 'NONE',  ( 159.2876523829509665, 254.7526883847961017, 15.64395448151312351 ) ) ;
#11696=CARTESIAN_POINT ( 'NONE',  ( 157.1539462478114615, 258.4483758192793061, -17.96006278656275867 ) ) ;
#11697=CARTESIAN_POINT ( 'NONE',  ( 115.9249311304092771, 246.9244531367911293, -4.594050593750046652 ) ) ;
#11699=CARTESIAN_POINT ( 'NONE',  ( 184.1192235817496794, 260.9197926262456235, 11.00856571192608513 ) ) ;
#11700=CARTESIAN_POINT ( 'NONE',  ( 201.4510510982464666, 281.3426432124285839, 16.26095448192928927 ) ) ;
#11703=CARTESIAN_POINT ( 'NONE',  ( 159.9014600375868440, 253.6895423408921886, 15.57825579621527368 ) ) ;
#11704=CARTESIAN_POINT ( 'NONE',  ( 194.6547327110108370, 291.6682678161738522, -16.14356736919946300 ) ) ;
#11705=CARTESIAN_POINT ( 'NONE',  ( 72.19064823929512897, 221.6744531367911293, 4.594050593750047540 ) ) ;
#11706=CARTESIAN_POINT ( 'NONE',  ( 169.3571508527084291, 283.0956279022483955, 12.63651818596384935 ) ) ;
#11707=CARTESIAN_POINT ( 'NONE',  ( 191.4941427383744781, 298.9694107557253346, 8.584406880462095657 ) ) ;
#11708=CARTESIAN_POINT ( 'NONE',  ( 150.6881537519499830, 269.6474569333088311, 15.31267828461696467 ) ) ;
#11709=CARTESIAN_POINT ( 'NONE',  ( 172.1891475301837033, 276.7325189785484554, 15.90371275011163910 ) ) ;
#11710=ORIENTED_EDGE ( 'NONE', *, *, #5964, .T. ) ;
#11715=CARTESIAN_POINT ( 'NONE',  ( 148.2459810799481943, 273.8774240820723662, 8.845211566752345433 ) ) ;
#11717=CARTESIAN_POINT ( 'NONE',  ( 161.1750406344237661, 251.4836360396366501, -14.21198410781773802 ) ) ;
#11718=CARTESIAN_POINT ( 'NONE',  ( 78.46959274033007148, 206.1115022471901739, -5.000000000000041744 ) ) ;
#11719=CARTESIAN_POINT ( 'NONE',  ( 61.75705882612326292, 194.9155109091896634, 2.679491924311254714 ) ) ;
#11720=ADVANCED_FACE ( 'NONE', ( #44286 ), #37962, .F. ) ;
#11721=CARTESIAN_POINT ( 'NONE',  ( 164.3022921857394749, 246.0670774647090582, 1.862798784958315856 ) ) ;
#11722=CARTESIAN_POINT ( 'NONE',  ( 151.7991800818630850, 269.5918300736246920, -14.34690986903463283 ) ) ;
#11723=CARTESIAN_POINT ( 'NONE',  ( 134.6192181478005523, 236.9824982072973967, 3.021315404115420679E-15 ) ) ;
#11724=CARTESIAN_POINT ( 'NONE',  ( 167.6123132579195953, 256.4410626529074761, 13.64026455462122911 ) ) ;
#11725=CARTESIAN_POINT ( 'NONE',  ( 207.5195222358739784, 271.2126392554839640, 2.810970398613041432 ) ) ;
#11726=CARTESIAN_POINT ( 'NONE',  ( 121.9063529450018137, 235.0643266524159856, -9.188101187500093303 ) ) ;
#11729=DIRECTION ( 'NONE',  ( -0.8660254037844359321, -0.5000000000000051070, -0.000000000000000000 ) ) ;
#11730=CARTESIAN_POINT ( 'NONE',  ( 161.6402223331288610, 284.6042864318112038, 1.832567169484626168 ) ) ;
#11731=CARTESIAN_POINT ( 'NONE',  ( 164.0777181605478745, 246.4560510864015441, 5.763760713451748785 ) ) ;
#11733=ORIENTED_EDGE ( 'NONE', *, *, #13718, .T. ) ;
#11735=( BOUNDED_CURVE ( )  B_SPLINE_CURVE ( 2, ( #31620, #1248, #9345, #56437, #93480, #54413, #32640, #46317, #40725 ),
 .UNSPECIFIED., .F., .T. ) 
 B_SPLINE_CURVE_WITH_KNOTS ( ( 3, 2, 2, 2, 3 ),
 ( 0.9072580645161290036, 0.9086021505376343788, 0.9112903225806451291, 0.9139784946236558794, 0.9153225806451612545 ),
 .UNSPECIFIED. ) 
 CURVE ( )  GEOMETRIC_REPRESENTATION_ITEM ( )  RATIONAL_B_SPLINE_CURVE ( ( 0.9330127018922194093, 0.9330127018922194093, 1.000000000000000000, 0.8660254037844387076, 1.000000000000000000, 0.8660254037844387076, 1.000000000000000000, 0.9330127018922194093, 0.9330127018922194093 ) ) 
 REPRESENTATION_ITEM ( '' )  );
#11736=CARTESIAN_POINT ( 'NONE',  ( 167.4300203585630413, 249.0882148589028304, -5.481496684248728712 ) ) ;
#11737=CARTESIAN_POINT ( 'NONE',  ( 164.6027939175806125, 245.5465931973980105, -2.481135897876769913 ) ) ;
#11740=B_SPLINE_CURVE_WITH_KNOTS ( 'NONE', 3,
 ( #76039, #52198, #91243, #6617, #99326, #45591, #29905, #91742, #22306, #76519, #22808, #7101, #30404, #53686, #84643, #46084, #55675, #32403, #46587, #70916, #55185, #23291, #17194, #93750, #69894, #16702, #70398, #2522, #31888, #86168, #47594, #25298, #86662, #48097, #78018, #24794, #506, #16204, #32895, #31395, #63300, #38989, #54680, #79038, #8608, #92737, #78522, #9628, #63802, #15692 ),
 .UNSPECIFIED., .F., .F.,
 ( 4, 2, 2, 2, 2, 2, 2, 2, 2, 2, 2, 2, 2, 2, 2, 2, 2, 2, 2, 2, 2, 2, 2, 2, 4 ),
 ( 0.0005200597963811503860, 0.001534264867450421416, 0.002041367402985044301, 0.002168143036868656979, 0.002294918670752269223, 0.002421694304635881468, 0.002548469938519494146, 0.002802021206286847439, 0.003055572474054200297, 0.003562675009589019639, 0.004576880080658723808, 0.005591085151728427544, 0.006098187687263286784, 0.006351738955030682143, 0.006605290222798075768, 0.006668678039739819874, 0.006732065856681563980, 0.006795453673623308086, 0.006858841490565051324, 0.007112392758331753662, 0.007619495293865116703, 0.007873046561631806897, 0.008126597829398497091, 0.008380149097165187286, 0.008633700364931875745 ),
 .UNSPECIFIED. ) ;
#11744=CARTESIAN_POINT ( 'NONE',  ( 157.3029956111992362, 258.1902147490555421, -18.22269824972649843 ) ) ;
#11745=CARTESIAN_POINT ( 'NONE',  ( 174.1921478203586560, 252.1247383714452894, 3.477943671650291169 ) ) ;
#11748=CARTESIAN_POINT ( 'NONE',  ( 190.0607312434325138, 301.4521522931182176, 3.538147641957853473 ) ) ;
#11749=CARTESIAN_POINT ( 'NONE',  ( 154.4702041996320361, 279.2069854860779401, -1.587565366136612699 ) ) ;
#11750=CARTESIAN_POINT ( 'NONE',  ( 169.3965326574621315, 285.1119705909437130, -8.078821750416475211 ) ) ;
#11751=CARTESIAN_POINT ( 'NONE',  ( 198.2819808855875863, 287.2125302111982705, 18.53535247371401695 ) ) ;
#11752=CARTESIAN_POINT ( 'NONE',  ( 157.4281126377775593, 271.2014885723156112, -14.63201430359713662 ) ) ;
#11753=CARTESIAN_POINT ( 'NONE',  ( 125.1447535615808988, 256.3927522451419918, 2.944929066748280225E-16 ) ) ;
#11754=B_SPLINE_CURVE_WITH_KNOTS ( 'NONE', 3,
 ( #79341, #34682, #65584, #96040 ),
 .UNSPECIFIED., .F., .F.,
 ( 4, 4 ),
 ( 0.0004588294438088373985, 0.008388525337162593826 ),
 .UNSPECIFIED. ) ;
#11758=CARTESIAN_POINT ( 'NONE',  ( 196.3720681610792553, 290.5205960880691691, 16.18360420724715354 ) ) ;
#11759=CARTESIAN_POINT ( 'NONE',  ( 148.3837145175834280, 273.6388627701866767, 8.841971351370922605 ) ) ;
#11760=CARTESIAN_POINT ( 'NONE',  ( -0.5279885150232012103, 164.3768266524160140, -9.188101187500093303 ) ) ;
#11762=CARTESIAN_POINT ( 'NONE',  ( 47.23881193640350062, 188.8923013555410080, 4.594050593750050204 ) ) ;
#11763=CARTESIAN_POINT ( 'NONE',  ( 177.2703692633946844, 258.2913615668659304, -10.36463420540507308 ) ) ;
#11765=DIRECTION ( 'NONE',  ( -0.8660254037844387076, -0.4999999999999998890, -0.000000000000000000 ) ) ;
#11766=CARTESIAN_POINT ( 'NONE',  ( 157.1458804504438831, 258.4623461901232417, -17.08829597948888335 ) ) ;
#11767=CARTESIAN_POINT ( 'NONE',  ( 189.2157573186698016, 290.5516144355429446, -14.57334616014404460 ) ) ;
#11768=CARTESIAN_POINT ( 'NONE',  ( 146.8201187048455267, 276.3470901603510015, 4.112223577763169047 ) ) ;
#11770=CARTESIAN_POINT ( 'NONE',  ( 169.7431851515004837, 257.7669204232371385, 13.75914435124215274 ) ) ;
#11771=CARTESIAN_POINT ( 'NONE',  ( 79.17323837735700920, 206.5177522451417929, 5.000000000000051514 ) ) ;
#11773=CARTESIAN_POINT ( 'NONE',  ( 157.1539462478114615, 258.4483758192793061, -17.96006278656275867 ) ) ;
#11774=CARTESIAN_POINT ( 'NONE',  ( 91.91334042722833431, 212.3262482093457777, 3.021315404115420679E-15 ) ) ;
#11776=EDGE_CURVE ( 'NONE', #82130, #37468, #37438, .T. ) ;
#11777=CARTESIAN_POINT ( 'NONE',  ( 43.32339510341159894, 182.4865022471901455, 1.119607411625061291E-15 ) ) ;
#11779=CARTESIAN_POINT ( 'NONE',  ( 168.6156890688689884, 286.4116463664167895, -8.226575548882113509 ) ) ;
#11781=CARTESIAN_POINT ( 'NONE',  ( 3.882894515797516988, 182.2369531367911009, -4.594050593750048428 ) ) ;
#11782=CARTESIAN_POINT ( 'NONE',  ( 167.8073358443718064, 286.0487684481980182, 4.087165526909992685 ) ) ;
#11783=B_SPLINE_CURVE_WITH_KNOTS ( 'NONE', 3,
 ( #29684, #13989, #44866, #91514, #53465, #45851, #99100, #53954, #92510, #23056, #273, #22080, #92032, #99592, #37277, #30175, #68173, #54445, #85422, #61062, #22578, #84415, #52977, #56470, #78790, #63570, #25067, #71196, #33691, #2296, #41256, #63071, #55944, #48886, #25584, #1283, #70668, #94014, #95021, #64585, #87946, #95537, #9378, #56959, #62550, #47364, #16468, #94513, #72198, #79327, #40256, #18490, #24566, #766 ),
 .UNSPECIFIED., .F., .F.,
 ( 4, 2, 2, 2, 2, 2, 2, 2, 2, 2, 2, 2, 2, 2, 2, 2, 2, 2, 2, 2, 2, 2, 2, 2, 2, 2, 4 ),
 ( 0.0006528422629810665513, 0.0008645749101140807850, 0.001076307557247095127, 0.001182173880813599479, 0.001288040204380103615, 0.001393906527946607750, 0.001499772851513112102, 0.001711505498646120373, 0.001923238145779129077, 0.002346703440045146052, 0.003193634028577111480, 0.004040564617109077342, 0.004887495205641041902, 0.005310960499907025484, 0.005522693147040058474, 0.005628559470606574536, 0.005681492632389832133, 0.005734425794173090597, 0.005787358955956349062, 0.005840292117739606659, 0.005946158441306171293, 0.006157891088439202548, 0.006369623735572234671, 0.006581356382705265927, 0.007004821676971320632, 0.007216554324104351888, 0.007428286971237384011 ),
 .UNSPECIFIED. ) ;
#11785=ADVANCED_FACE ( 'NONE', ( #95940 ), #79363, .F. ) ;
#11786=CARTESIAN_POINT ( 'NONE',  ( 153.4477557824949940, 264.8676860077344486, 17.16010094972647693 ) ) ;
#11788=CARTESIAN_POINT ( 'NONE',  ( 83.66574516303668929, 209.1115022471902023, -5.000000000000041744 ) ) ;
#11789=CARTESIAN_POINT ( 'NONE',  ( 179.3259839114000158, 277.6273404258797086, 17.12033975729926638 ) ) ;
#11790=CARTESIAN_POINT ( 'NONE',  ( 154.9455285025717615, 262.2734675583710100, 18.28470720339922551 ) ) ;
#11791=B_SPLINE_CURVE_WITH_KNOTS ( 'NONE', 3,
 ( #53418, #69619, #14915, #38713, #45804, #61999, #76728, #85895, #84367, #38200 ),
 .UNSPECIFIED., .F., .F.,
 ( 4, 3, 3, 4 ),
 ( 0.0005899778860174007163, 0.001498044977030944455, 0.004494154408253303763, 0.005834865480722558825 ),
 .UNSPECIFIED. ) ;
#11793=B_SPLINE_CURVE_WITH_KNOTS ( 'NONE', 3,
 ( #97040, #74718, #28085, #42768 ),
 .UNSPECIFIED., .F., .F.,
 ( 4, 4 ),
 ( 0.008066038982947665303, 0.01417919469606437194 ),
 .UNSPECIFIED. ) ;
#11794=CARTESIAN_POINT ( 'NONE',  ( 179.4170627276716345, 262.5904822696095380, -12.85500290294408288 ) ) ;
#11798=CARTESIAN_POINT ( 'NONE',  ( 159.1349094508772737, 259.4340307094828404, 16.68893039409465828 ) ) ;
#11799=CARTESIAN_POINT ( 'NONE',  ( 154.8989000222956349, 262.3542304552891551, 17.41779271305265908 ) ) ;
#11800=ORIENTED_EDGE ( 'NONE', *, *, #39155, .F. ) ;
#11801=CARTESIAN_POINT ( 'NONE',  ( 154.9380580364485525, 275.5880567444434064, 10.35765824813548619 ) ) ;
#11802=CARTESIAN_POINT ( 'NONE',  ( 159.9770824720811220, 253.5585604421560788, -16.42166711341322483 ) ) ;
#11804=CARTESIAN_POINT ( 'NONE',  ( 192.2185419806677942, 297.7147144631093170, 12.45868041609393728 ) ) ;
#11805=CARTESIAN_POINT ( 'NONE',  ( 207.3062152119541679, 271.5820978585240368, 7.879821064966149535 ) ) ;
#11806=CARTESIAN_POINT ( 'NONE',  ( 181.4791476608088487, 255.0645862387702039, -1.457838961102627895 ) ) ;
#11808=ORIENTED_EDGE ( 'NONE', *, *, #45491, .F. ) ;
#11810=CARTESIAN_POINT ( 'NONE',  ( 159.6784519327069063, 278.7635212910759606, -9.544083088951406779 ) ) ;
#11811=CARTESIAN_POINT ( 'NONE',  ( 204.5133713884061706, 276.4194452585140311, 14.87364779308245843 ) ) ;
#11812=CARTESIAN_POINT ( 'NONE',  ( 152.6945189806187955, 266.1723304187151484, 16.62409282110771613 ) ) ;
#11813=VERTEX_POINT ( 'NONE', #77586 ) ;
#11815=CARTESIAN_POINT ( 'NONE',  ( 175.8349158976987212, 262.9913934397512207, 14.38086816053275108 ) ) ;
#11818=CARTESIAN_POINT ( 'NONE',  ( 76.43878283397967266, 226.4860189848784842, -2.679491924311252493 ) ) ;
#11822=CARTESIAN_POINT ( 'NONE',  ( 161.8289209813647176, 250.3510820566641257, 13.28523796267037937 ) ) ;
#11823=FACE_OUTER_BOUND ( 'NONE', #47046, .T. ) ;
#11824=FACE_OUTER_BOUND ( 'NONE', #16930, .T. ) ;
#11825=ORIENTED_EDGE ( 'NONE', *, *, #95333, .F. ) ;
#11826=CARTESIAN_POINT ( 'NONE',  ( 174.4652129899553472, 277.2261295425576577, -15.64854957247286471 ) ) ;
#11827=CARTESIAN_POINT ( 'NONE',  ( 201.5074933251657399, 279.6257787853921286, 16.58790246189369100 ) ) ;
#11829=ORIENTED_EDGE ( 'NONE', *, *, #91560, .F. ) ;
#11830=CARTESIAN_POINT ( 'NONE',  ( 156.8551930071947140, 266.3782999250777266, -16.34332614469098743 ) ) ;
#11838=CARTESIAN_POINT ( 'NONE',  ( 177.8017954917369252, 291.1815355444027205, 6.079021535780970709 ) ) ;
#11839=CARTESIAN_POINT ( 'NONE',  ( 191.1192699377806719, 299.6187094927299199, -9.526914969203620132 ) ) ;
#11846=CARTESIAN_POINT ( 'NONE',  ( 206.3106310032756596, 273.3065002911688453, 10.17860425536756175 ) ) ;
#11847=CARTESIAN_POINT ( 'NONE',  ( 198.5558597050348908, 286.7381581807989051, 17.16554469393394200 ) ) ;
#11848=EDGE_LOOP ( 'NONE', ( #26565, #14154, #682, #65055 ) ) ;
#11849=CARTESIAN_POINT ( 'NONE',  ( 187.5205457192285223, 277.0860194500085640, 16.99091369793140061 ) ) ;
#11851=CARTESIAN_POINT ( 'NONE',  ( 198.7408816115379864, 285.9624092822338071, -17.04496721243561197 ) ) ;
#11852=CARTESIAN_POINT ( 'NONE',  ( 177.9661674680945112, 277.1853473926717015, -17.54411374166730297 ) ) ;
#11853=EDGE_CURVE ( 'NONE', #92061, #14896, #73751, .T. ) ;
#11854=CARTESIAN_POINT ( 'NONE',  ( 160.5165517222688436, 252.6241722917100390, -14.79882802290810595 ) ) ;
#11855=CARTESIAN_POINT ( 'NONE',  ( 148.7168577282835713, 273.0618418030571206, -9.544069619348908518 ) ) ;
#11857=CARTESIAN_POINT ( 'NONE',  ( 167.2812095546786679, 252.8454341180955680, -12.28570835557802177 ) ) ;
#11859=CARTESIAN_POINT ( 'NONE',  ( 124.2065593741477301, 252.5177522451419350, 5.000000000000046185 ) ) ;
#11860=CARTESIAN_POINT ( 'NONE',  ( 164.2672861321391053, 246.1277097281173667, -2.417001679502223777 ) ) ;
#11862=CARTESIAN_POINT ( 'NONE',  ( 30.24280306353613312, 198.2677522451419350, -5.000000000000047962 ) ) ;
#11863=CARTESIAN_POINT ( 'NONE',  ( 110.3232631693849441, 228.3768266524160140, 9.188101187500096856 ) ) ;
#11864=CARTESIAN_POINT ( 'NONE',  ( 183.5927363050826955, 297.0638526922078313, -2.830836570955955978 ) ) ;
#11865=CARTESIAN_POINT ( 'NONE',  ( 167.3110030245129281, 283.1034262774602439, -11.14282353764315303 ) ) ;
#11867=CARTESIAN_POINT ( 'NONE',  ( 162.7894281526998839, 248.6874348348773651, 10.21811719309735622 ) ) ;
#11868=CARTESIAN_POINT ( 'NONE',  ( 25.07406103223676652, 173.0327760586659451, 1.948934522072303157E-15 ) ) ;
#11871=B_SPLINE_CURVE_WITH_KNOTS ( 'NONE', 3,
 ( #97313, #73498, #67373, #74510 ),
 .UNSPECIFIED., .F., .F.,
 ( 4, 4 ),
 ( 0.005351796179668294809, 0.01338782376300005385 ),
 .UNSPECIFIED. ) ;
#11874=CARTESIAN_POINT ( 'NONE',  ( 185.3920610038572647, 259.4640903649777783, -5.312017440010943226 ) ) ;
#11876=CARTESIAN_POINT ( 'NONE',  ( 190.6954410837624607, 300.3528026016029457, -5.728531842148099962 ) ) ;
#11877=CARTESIAN_POINT ( 'NONE',  ( 193.0090100919386202, 263.8705414732962709, -4.314308890231003168 ) ) ;
#11878=CARTESIAN_POINT ( 'NONE',  ( 161.0974665087481981, 251.6179983666593216, -13.69252715295363210 ) ) ;
#11879=CARTESIAN_POINT ( 'NONE',  ( 185.8273812090706940, 286.4779426780396534, 15.58107062954017330 ) ) ;
#11881=CARTESIAN_POINT ( 'NONE',  ( 39.95835201613431309, 200.0024278399160949, 9.188101187500095079 ) ) ;
#11882=CARTESIAN_POINT ( 'NONE',  ( 106.8138825148103450, 219.1427522451417644, 1.119607411625061291E-15 ) ) ;
#11885=CARTESIAN_POINT ( 'NONE',  ( 179.1927739452798676, 258.3510491419078221, -10.08736568086201579 ) ) ;
#11887=CARTESIAN_POINT ( 'NONE',  ( -4.696256414383327638, 180.3464784336661637, 1.353441290958777327E-15 ) ) ;
#11889=CARTESIAN_POINT ( 'NONE',  ( 198.4344074287054696, 286.9485196940960918, -17.83642855442570152 ) ) ;
#11890=DIRECTION ( 'NONE',  ( -0.8660254037844387076, -0.4999999999999998890, -0.000000000000000000 ) ) ;
#11891=CARTESIAN_POINT ( 'NONE',  ( 192.5284579606305613, 297.1779242397361713, -13.15228012403107272 ) ) ;
#11893=CARTESIAN_POINT ( 'NONE',  ( 193.2494886543572363, 263.9923760144491780, 7.744585581713212541 ) ) ;
#11894=CARTESIAN_POINT ( 'NONE',  ( 203.7436594101163507, 276.0772935449583656, 13.22569794353039363 ) ) ;
#11896=CARTESIAN_POINT ( 'NONE',  ( 207.5686001603237116, 271.1276337968068333, 7.659944433763431704 ) ) ;
#11898=CARTESIAN_POINT ( 'NONE',  ( 0.5273063997305784678, 161.1115022471902023, -5.000000000000041744 ) ) ;
#11901=CARTESIAN_POINT ( 'NONE',  ( 120.4987145680870952, 246.5024278399160949, 9.188101187500095079 ) ) ;
#11905=EDGE_CURVE ( 'NONE', #53889, #22875, #43592, .T. ) ;
#11906=FACE_OUTER_BOUND ( 'NONE', #9216, .T. ) ;
#11907=AXIS2_PLACEMENT_3D ( 'NONE', #72242, #95582, #27132 ) ;
#11910=CARTESIAN_POINT ( 'NONE',  ( 190.6083555345403795, 300.5036391974608136, -6.894354067666211172 ) ) ;
#11911=EDGE_LOOP ( 'NONE', ( #88743, #69038, #82164, #90521, #89357 ) ) ;
#11913=CARTESIAN_POINT ( 'NONE',  ( 163.3351346677209506, 247.7422434248393586, 8.151360907120263732 ) ) ;
#11914=CARTESIAN_POINT ( 'NONE',  ( 195.4436462626574667, 265.1414692012189676, -7.795071168451356058 ) ) ;
#11915=CARTESIAN_POINT ( 'NONE',  ( 173.0073966428915071, 268.1627966282908915, -16.30112163756558630 ) ) ;
#11918=CARTESIAN_POINT ( 'NONE',  ( -27.42236680055714260, 166.5217562850347406, 1.224646799147364892E-15 ) ) ;
#11919=CARTESIAN_POINT ( 'NONE',  ( 167.3709722853970163, 270.8926238990931665, -16.36061349221664329 ) ) ;
#11922=CARTESIAN_POINT ( 'NONE',  ( 185.8931680259638028, 296.6947360474555921, 4.853906208423047985 ) ) ;
#11924=CYLINDRICAL_SURFACE ( 'NONE', #71082, 17.82106496071139645 ) ;
#11926=CARTESIAN_POINT ( 'NONE',  ( 194.5078867822585664, 282.9899840733189080, 17.68867816471975019 ) ) ;
#11928=CARTESIAN_POINT ( 'NONE',  ( 173.9683356937793519, 272.2847035684981734, -17.69864048336468088 ) ) ;
#11931=CARTESIAN_POINT ( 'NONE',  ( 194.3541845315608612, 294.0156730581561533, -14.67567721756631016 ) ) ;
#11933=ORIENTED_EDGE ( 'NONE', *, *, #28143, .T. ) ;
#11939=CARTESIAN_POINT ( 'NONE',  ( 86.99453030705913648, 221.0333772461660544, 9.188101187500095079 ) ) ;
#11941=CARTESIAN_POINT ( 'NONE',  ( 184.6889223697928912, 259.7167601846132925, -5.813120004385227801 ) ) ;
#11947=VERTEX_POINT ( 'NONE', #88726 ) ;
#11949=CARTESIAN_POINT ( 'NONE',  ( 155.4810912439522212, 261.3458456796594760, -18.44218279064527266 ) ) ;
#11951=CARTESIAN_POINT ( 'NONE',  ( 187.1789365411204926, 291.3781964708418286, -14.15416893886036220 ) ) ;
#11953=CARTESIAN_POINT ( 'NONE',  ( 189.9197469165544874, 301.6963443103418854, 2.546707301993238026 ) ) ;
#11954=CARTESIAN_POINT ( 'NONE',  ( 159.7566137705401843, 275.6830047768774534, -12.53866916850027025 ) ) ;
#11955=CARTESIAN_POINT ( 'NONE',  ( 200.8147387322574957, 282.8256649374973790, -18.02438097732020239 ) ) ;
#11956=CARTESIAN_POINT ( 'NONE',  ( 165.5093369583051128, 275.0219039653110258, -16.16693748275729803 ) ) ;
#11957=CARTESIAN_POINT ( 'NONE',  ( 141.5001777056247931, 246.3768266524160140, 9.188101187500098632 ) ) ;
#11960=VERTEX_POINT ( 'NONE', #17780 ) ;
#11965=CARTESIAN_POINT ( 'NONE',  ( 156.6812872898450735, 261.2670451491295012, 0.000000000000000000 ) ) ;
#11968=CARTESIAN_POINT ( 'NONE',  ( 156.7598395624803231, 279.4774680247458605, 7.438909857426141414 ) ) ;
#11969=CARTESIAN_POINT ( 'NONE',  ( 165.5287065161056717, 246.9177196700316870, -2.014791919525022568 ) ) ;
#11970=CARTESIAN_POINT ( 'NONE',  ( 172.4473134597787976, 280.4758190227907448, 13.90356073592574049 ) ) ;
#11971=CARTESIAN_POINT ( 'NONE',  ( 168.1310046488833905, 252.8833719797225967, 11.91735455981645764 ) ) ;
#11973=EDGE_LOOP ( 'NONE', ( #9965, #79740, #16505, #32960, #95386 ) ) ;
#11974=CARTESIAN_POINT ( 'NONE',  ( 185.0366554279405022, 273.1381174272470957, -16.61285403035061137 ) ) ;
#11977=B_SPLINE_CURVE_WITH_KNOTS ( 'NONE', 3,
 ( #84577, #15115, #78454, #62214 ),
 .UNSPECIFIED., .F., .F.,
 ( 4, 4 ),
 ( 0.02596114015397115241, 0.03520195514588816271 ),
 .UNSPECIFIED. ) ;
#11981=CARTESIAN_POINT ( 'NONE',  ( 200.9434809886455469, 267.7932726406668849, -2.812590155380607637 ) ) ;
#11983=CARTESIAN_POINT ( 'NONE',  ( 198.4097421844162170, 265.0824675037606539, -3.039349057205883664 ) ) ;
#11984=CARTESIAN_POINT ( 'NONE',  ( 164.6405626616606526, 274.4174134527740989, 16.14945534314108144 ) ) ;
#11985=CARTESIAN_POINT ( 'NONE',  ( 161.3190595899150139, 281.5918341196443748, -7.463758623216700805 ) ) ;
#11987=CARTESIAN_POINT ( 'NONE',  ( 203.8395512996133334, 269.2639942102448458, 5.522558735337302238 ) ) ;
#11988=EDGE_LOOP ( 'NONE', ( #69968, #41676, #63994, #75461 ) ) ;
#11991=CARTESIAN_POINT ( 'NONE',  ( 189.8329410786966491, 274.2658440874778876, -15.65430098090321565 ) ) ;
#11994=CARTESIAN_POINT ( 'NONE',  ( 172.4827362167600029, 289.4993777119672700, 2.605925812672743813 ) ) ;
#11998=CARTESIAN_POINT ( 'NONE',  ( 4.640666744108908226, 182.6744531367911577, 4.594050593750047540 ) ) ;
#11999=CARTESIAN_POINT ( 'NONE',  ( 110.3232631693849726, 228.3768266524160140, 9.188101187500098632 ) ) ;
#12001=CARTESIAN_POINT ( 'NONE',  ( 181.5558742819051474, 255.2544784655372894, -2.503599602330015994 ) ) ;
#12002=CARTESIAN_POINT ( 'NONE',  ( 197.9901163037401943, 272.1418500761980681, -13.83221381771805625 ) ) ;
#12003=DIRECTION ( 'NONE',  ( 0.4999999999999992784, -0.8660254037844390407, 0.000000000000000000 ) ) ;
#12005=CARTESIAN_POINT ( 'NONE',  ( 164.0383833005010956, 283.8578478928177447, 5.735541721561834727 ) ) ;
#12006=CARTESIAN_POINT ( 'NONE',  ( 194.5252985417586729, 293.7192948986070178, -14.54632727629426370 ) ) ;
#12009=B_SPLINE_CURVE_WITH_KNOTS ( 'NONE', 3,
 ( #27004, #41683, #20407, #89356, #19909, #51276, #50288, #57889, #96440, #73605, #34592, #35087, #97415, #3228, #27983, #65005, #72627, #50781, #65991, #34113, #81241, #82243, #59361, #96944, #74622, #81731, #11815, #26509, #12818, #19432, #58862, #88867, #42672, #89831, #5195, #90338, #43680, #95948, #27510, #80756, #80242, #57387, #36077, #42185, #12308, #73121, #43168, #74110, #66978, #88361 ),
 .UNSPECIFIED., .F., .F.,
 ( 4, 2, 2, 2, 2, 2, 2, 2, 2, 2, 2, 2, 2, 2, 2, 2, 2, 2, 2, 2, 2, 2, 2, 2, 4 ),
 ( 0.0007549782464651950487, 0.001244381850067043365, 0.001733785453668891356, 0.001978487255469815569, 0.002223189057270739781, 0.002345539958171201887, 0.002467890859071663993, 0.002590241759972126100, 0.002712592660872587772, 0.002957294462673536704, 0.003201996264474486070, 0.003691399868076324087, 0.004670207075280077315, 0.005649014282483829676, 0.006138417886085665090, 0.006627821489687500504, 0.006750172390587940927, 0.006811347841038178919, 0.006872523291488416043, 0.006994874192388890292, 0.007117225093289364542, 0.007361926895090339061, 0.007606628696891313580, 0.008096032300493266956, 0.008585435904095221199 ),
 .UNSPECIFIED. ) ;
#12010=CARTESIAN_POINT ( 'NONE',  ( 195.4436462626574667, 265.1414692012189676, -7.795071168451356058 ) ) ;
#12013=CARTESIAN_POINT ( 'NONE',  ( 172.9541071254618316, 262.8455706559834653, -15.93875919266165120 ) ) ;
#12014=CARTESIAN_POINT ( 'NONE',  ( 78.92949518643405327, 222.5024278399160949, 9.188101187500095079 ) ) ;
#12019=CARTESIAN_POINT ( 'NONE',  ( 157.2333142128019858, 258.3109064714224132, 16.87956768598436597 ) ) ;
#12020=CARTESIAN_POINT ( 'NONE',  ( 199.7779437056017571, 284.6214466006996417, 18.28733359541573478 ) ) ;
#12021=CARTESIAN_POINT ( 'NONE',  ( 150.9363692955544991, 269.2175350005573478, -14.27857383982596140 ) ) ;
#12022=CARTESIAN_POINT ( 'NONE',  ( 165.7433911102912987, 286.0540145108149090, -5.579755643435937884 ) ) ;
#12024=CARTESIAN_POINT ( 'NONE',  ( 147.5381343315788172, 275.1034506142203782, -4.056595942992749393 ) ) ;
#12025=CARTESIAN_POINT ( 'NONE',  ( 156.7442704525034571, 261.1579551113846378, 17.82061976529222846 ) ) ;
#12026=ORIENTED_EDGE ( 'NONE', *, *, #77163, .F. ) ;
#12030=CARTESIAN_POINT ( 'NONE',  ( 189.2189693547002776, 286.5034521383401511, -15.94273063411117874 ) ) ;
#12032=VERTEX_POINT ( 'NONE', #86064 ) ;
#12033=( BOUNDED_CURVE ( )  B_SPLINE_CURVE ( 2, ( #4260, #3781, #48881, #66068, #3297, #2800, #27587, #19979, #50855 ),
 .UNSPECIFIED., .F., .T. ) 
 B_SPLINE_CURVE_WITH_KNOTS ( ( 3, 2, 2, 2, 3 ),
 ( 0.06854838709677418818, 0.06989247311827956333, 0.07258064516129032751, 0.07526881720430107781, 0.07661290322580645296 ),
 .UNSPECIFIED. ) 
 CURVE ( )  GEOMETRIC_REPRESENTATION_ITEM ( )  RATIONAL_B_SPLINE_CURVE ( ( 0.9330127018922194093, 0.9330127018922194093, 1.000000000000000000, 0.8660254037844387076, 1.000000000000000000, 0.8660254037844387076, 1.000000000000000000, 0.9330127018922194093, 0.9330127018922194093 ) ) 
 REPRESENTATION_ITEM ( '' )  );
#12035=CIRCLE ( 'NONE', #92963, 17.82106496071138224 ) ;
#12037=CARTESIAN_POINT ( 'NONE',  ( 188.0361769804965206, 281.7550819701144746, -17.70093714309158983 ) ) ;
#12038=CARTESIAN_POINT ( 'NONE',  ( 136.9263074957796675, 249.8615022471902591, -10.00000000000009592 ) ) ;
#12039=CARTESIAN_POINT ( 'NONE',  ( 157.2777284163744582, 258.2339788142568864, -16.82360006463426316 ) ) ;
#12042=CARTESIAN_POINT ( 'NONE',  ( 165.8692079773426826, 246.3314739835906835, -1.162168092255636775 ) ) ;
#12044=CARTESIAN_POINT ( 'NONE',  ( 202.4943568615953779, 279.9164810001701085, 17.09064351659286984 ) ) ;
#12046=ORIENTED_EDGE ( 'NONE', *, *, #89482, .F. ) ;
#12054=CARTESIAN_POINT ( 'NONE',  ( 95.64807497750081211, 214.4824982072973683, 3.021315404115420679E-15 ) ) ;
#12057=CARTESIAN_POINT ( 'NONE',  ( 164.2758297317967902, 275.0605672077817871, 14.75495795951908740 ) ) ;
#12062=CARTESIAN_POINT ( 'NONE',  ( 164.2413944571582078, 246.1725554246774834, 7.304616466633322425 ) ) ;
#12063=CARTESIAN_POINT ( 'NONE',  ( 165.8703699689788493, 274.3934474687724219, -15.11696372367774721 ) ) ;
#12067=CARTESIAN_POINT ( 'NONE',  ( 164.9009427471078766, 270.4319544559331234, -17.40525121274953335 ) ) ;
#12068=CARTESIAN_POINT ( 'NONE',  ( 207.3954518193029912, 271.4275355207012694, -4.733997076022094852 ) ) ;
#12069=CARTESIAN_POINT ( 'NONE',  ( 163.8835510476618254, 277.4261113242017132, -14.47671527678674330 ) ) ;
#12070=CARTESIAN_POINT ( 'NONE',  ( 182.0294364313458857, 256.9024481669246143, 5.105451491673651532 ) ) ;
#12071=CARTESIAN_POINT ( 'NONE',  ( 95.92524373570365981, 232.3149278399160949, -9.188101187500095079 ) ) ;
#12072=ORIENTED_EDGE ( 'NONE', *, *, #11853, .F. ) ;
#12073=CARTESIAN_POINT ( 'NONE',  ( 190.8860811105559208, 300.0226043892405414, 8.636347304323541252 ) ) ;
#12074=CARTESIAN_POINT ( 'NONE',  ( 166.6051582734733358, 278.7391106529776721, -13.20946712174476545 ) ) ;
#12076=ORIENTED_EDGE ( 'NONE', *, *, #57162, .F. ) ;
#12077=EDGE_LOOP ( 'NONE', ( #86720, #97898, #21982, #83721, #76467 ) ) ;
#12079=CARTESIAN_POINT ( 'NONE',  ( 180.3528982427918663, 293.8293478312841671, -2.635769195210191818 ) ) ;
#12080=CARTESIAN_POINT ( 'NONE',  ( 164.2537261577595586, 249.8683019904829621, 10.06821014759007404 ) ) ;
#12082=CARTESIAN_POINT ( 'NONE',  ( 163.0311878320900121, 248.2686947869521532, 10.33250033289960435 ) ) ;
#12085=CARTESIAN_POINT ( 'NONE',  ( 162.9383752892161397, 248.4294508267893491, -11.25953730674605957 ) ) ;
#12086=ORIENTED_EDGE ( 'NONE', *, *, #77743, .T. ) ;
#12087=ADVANCED_FACE ( 'NONE', ( #38884 ), #46477, .T. ) ;
#12088=CARTESIAN_POINT ( 'NONE',  ( 194.9900005546388968, 265.9144807066997487, -8.896229505766779511 ) ) ;
#12089=CARTESIAN_POINT ( 'NONE',  ( 153.2524140410926918, 266.3468094423246271, 16.28161397018561374 ) ) ;
#12091=CARTESIAN_POINT ( 'NONE',  ( 129.5380282679697075, 245.5958772461660544, -9.188101187500095079 ) ) ;
#12092=CARTESIAN_POINT ( 'NONE',  ( 199.9329555241513106, 283.7849761008080804, 16.97275319715699737 ) ) ;
#12097=CARTESIAN_POINT ( 'NONE',  ( 177.2212890013350659, 257.5021112054951686, 11.61326389234794298 ) ) ;
#12098=DIRECTION ( 'NONE',  ( 0.4999999999999992784, -0.8660254037844390407, 0.000000000000000000 ) ) ;
#12099=CARTESIAN_POINT ( 'NONE',  ( 189.5156151668331290, 270.2242446231968529, 14.35960433212074250 ) ) ;
#12103=EDGE_CURVE ( 'NONE', #99288, #13470, #99604, .T. ) ;
#12106=CARTESIAN_POINT ( 'NONE',  ( 142.6123662252853421, 259.5780487066560340, -7.305945665944390655 ) ) ;
#12108=CARTESIAN_POINT ( 'NONE',  ( 206.7424236707713305, 272.1642866507044118, 6.817570650586102232 ) ) ;
#12109=CARTESIAN_POINT ( 'NONE',  ( 159.9894443651313338, 253.5371490153152081, -16.36035038356864391 ) ) ;
#12111=CARTESIAN_POINT ( 'NONE',  ( 207.6067494229581314, 271.0615573356529353, -1.924113146155245868 ) ) ;
#12115=CARTESIAN_POINT ( 'NONE',  ( 181.9913877802205775, 264.0113901683749305, 13.86632907263398096 ) ) ;
#12116=CARTESIAN_POINT ( 'NONE',  ( 181.2370176562050688, 263.3306497680472944, -14.40870033085988666 ) ) ;
#12119=CARTESIAN_POINT ( 'NONE',  ( 157.6058986277583642, 270.9393266711600177, -14.76023724535021664 ) ) ;
#12121=CARTESIAN_POINT ( 'NONE',  ( 207.1285138014047504, 271.8898857301724661, -5.752177443817618752 ) ) ;
#12123=CARTESIAN_POINT ( 'NONE',  ( 21.69106252476256458, 174.1423013555409796, -4.594050593750043987 ) ) ;
#12126=EDGE_CURVE ( 'NONE', #77337, #87147, #62972, .T. ) ;
#12129=FACE_OUTER_BOUND ( 'NONE', #97585, .T. ) ;
#12131=CARTESIAN_POINT ( 'NONE',  ( 45.85867072306329817, 185.0327760586659451, 1.948934522072302763E-15 ) ) ;
#12133=CARTESIAN_POINT ( 'NONE',  ( 200.7897860911934913, 282.8688841796032420, 18.17522996445731920 ) ) ;
#12134=CARTESIAN_POINT ( 'NONE',  ( 174.0050912145983659, 289.3368536554620505, 7.990428673744625065 ) ) ;
#12135=CARTESIAN_POINT ( 'NONE',  ( 190.2510882691990730, 301.1224442529128851, -5.480893437181090455 ) ) ;
#12137=CARTESIAN_POINT ( 'NONE',  ( 203.0446730937520954, 269.9112416612543939, -7.271914997583759366 ) ) ;
#12138=CARTESIAN_POINT ( 'NONE',  ( 191.0724301404414689, 299.6998384015373063, -9.342134220577969828 ) ) ;
#12142=CARTESIAN_POINT ( 'NONE',  ( 113.3812418268422846, 236.2677522451418497, 10.00000000000009592 ) ) ;
#12146=CARTESIAN_POINT ( 'NONE',  ( 83.66574516303668929, 209.1115022471902023, -5.000000000000041744 ) ) ;
#12147=CARTESIAN_POINT ( 'NONE',  ( 7.868168403658736487, 186.8967562850346837, -4.648177544792955347E-16 ) ) ;
#12150=CARTESIAN_POINT ( 'NONE',  ( 50.56751030825869009, 193.8768266524160140, 9.188101187500098632 ) ) ;
#12153=CARTESIAN_POINT ( 'NONE',  ( 146.9376205018946848, 276.1435710778808925, 5.066564108429441937 ) ) ;
#12156=CARTESIAN_POINT ( 'NONE',  ( 167.3572442387605577, 285.1339219078583938, 7.830934403729975735 ) ) ;
#12157=CARTESIAN_POINT ( 'NONE',  ( 164.8670003495851404, 245.0889742334797177, -1.557028074864921674 ) ) ;
#12161=CARTESIAN_POINT ( 'NONE',  ( 176.7491000883603078, 284.2402667147796933, -14.85471036738550055 ) ) ;
#12166=CARTESIAN_POINT ( 'NONE',  ( 174.9106947789025241, 255.1781923355507899, 8.157823743021118901 ) ) ;
#12169=CARTESIAN_POINT ( 'NONE',  ( 182.4004271739244700, 284.1903799708203451, 16.39187655311515002 ) ) ;
#12171=CARTESIAN_POINT ( 'NONE',  ( 165.5845016731641124, 245.8462254865437160, 0.7221155814038995313 ) ) ;
#12172=AXIS2_PLACEMENT_3D ( 'NONE', #74261, #35731, #28125 ) ;
#12173=EDGE_LOOP ( 'NONE', ( #47654, #53343, #69862, #80647 ) ) ;
#12174=ORIENTED_EDGE ( 'NONE', *, *, #90000, .T. ) ;
#12175=CARTESIAN_POINT ( 'NONE',  ( 207.8844858873204657, 270.5805036682629066, -6.251308616122969397 ) ) ;
#12177=CARTESIAN_POINT ( 'NONE',  ( 198.2505066714982149, 285.2670451491296149, 0.000000000000000000 ) ) ;
#12183=EDGE_CURVE ( 'NONE', #71188, #86782, #56861, .T. ) ;
#12184=CARTESIAN_POINT ( 'NONE',  ( 157.7593757092099906, 257.3997412317380054, -18.08445832352326121 ) ) ;
#12186=CARTESIAN_POINT ( 'NONE',  ( 126.7237928014352804, 231.7202760586659736, -5.415160957724236172E-17 ) ) ;
#12187=CARTESIAN_POINT ( 'NONE',  ( 164.2413944571582078, 246.1725554246774834, 7.304616466633322425 ) ) ;
#12188=CYLINDRICAL_SURFACE ( 'NONE', #67366, 17.82106496071139645 ) ;
#12190=B_SPLINE_CURVE_WITH_KNOTS ( 'NONE', 3,
 ( #97186, #29248, #43926, #20162 ),
 .UNSPECIFIED., .F., .F.,
 ( 4, 4 ),
 ( 0.01237858375601574683, 0.02090696561293280478 ),
 .UNSPECIFIED. ) ;
#12191=CARTESIAN_POINT ( 'NONE',  ( 163.7183543885751078, 247.0784873978576854, -6.786164904910574336 ) ) ;
#12196=CARTESIAN_POINT ( 'NONE',  ( 76.60222546164588664, 215.0333772461660544, 9.188101187500095079 ) ) ;
#12199=CARTESIAN_POINT ( 'NONE',  ( 120.3761533483303907, 228.7592609112379591, 2.679491924311254714 ) ) ;
#12200=CARTESIAN_POINT ( 'NONE',  ( 150.9982109096994520, 269.1104221828363734, 14.90714565999273766 ) ) ;
#12201=CARTESIAN_POINT ( 'NONE',  ( 175.6099198705963431, 278.4306179087495252, 15.49799073493723967 ) ) ;
#12202=VERTEX_POINT ( 'NONE', #57581 ) ;
#12206=ORIENTED_EDGE ( 'NONE', *, *, #18483, .T. ) ;
#12207=CARTESIAN_POINT ( 'NONE',  ( 143.0969038086192597, 260.4263049900483225, -7.951529393128359935 ) ) ;
#12208=DIRECTION ( 'NONE',  ( -0.4999999999999987788, 0.8660254037844392627, 0.000000000000000000 ) ) ;
#12214=CARTESIAN_POINT ( 'NONE',  ( 151.6960368807307873, 276.4293682816003752, 8.579070964960488155 ) ) ;
#12215=VECTOR ( 'NONE', #64162, 1000.000000000000000 ) ;
#12216=CARTESIAN_POINT ( 'NONE',  ( 152.3784850679831493, 270.1081530411233302, -14.58078914583996344 ) ) ;
#12218=ORIENTED_EDGE ( 'NONE', *, *, #77788, .T. ) ;
#12219=CARTESIAN_POINT ( 'NONE',  ( 207.5408646414791178, 271.1756731246201753, 3.050859480894625886 ) ) ;
#12220=CARTESIAN_POINT ( 'NONE',  ( 127.2647115830355347, 244.2833772461660544, -9.188101187500095079 ) ) ;
#12221=EDGE_LOOP ( 'NONE', ( #85211, #60745, #73215, #46154 ) ) ;
#12222=CARTESIAN_POINT ( 'NONE',  ( 191.0724301404414689, 299.6998384015373063, -9.342134220577969828 ) ) ;
#12224=CARTESIAN_POINT ( 'NONE',  ( 155.3250150347760723, 261.6161776038049425, -18.57420904020362684 ) ) ;
#12225=ADVANCED_FACE ( 'NONE', ( #42374 ), #3898, .T. ) ;
#12226=CARTESIAN_POINT ( 'NONE',  ( 204.8762144138505903, 275.7909827032724479, 14.60855957933206817 ) ) ;
#12227=EDGE_CURVE ( 'NONE', #71064, #42571, #1256, .T. ) ;
#12230=VERTEX_POINT ( 'NONE', #97138 ) ;
#12232=CARTESIAN_POINT ( 'NONE',  ( 157.5458375898066663, 275.8685363031948441, 12.98959349559163634 ) ) ;
#12234=CARTESIAN_POINT ( 'NONE',  ( 31.46967238556409896, 195.6427522451419350, -10.00000000000009592 ) ) ;
#12235=CARTESIAN_POINT ( 'NONE',  ( 137.8731756836298814, 262.6589784336661637, -6.496448406907676862E-16 ) ) ;
#12236=B_SPLINE_CURVE_WITH_KNOTS ( 'NONE', 3,
 ( #15748, #22858, #68455, #53742 ),
 .UNSPECIFIED., .F., .F.,
 ( 4, 4 ),
 ( 0.03872932741557565117, 0.04724607957928941143 ),
 .UNSPECIFIED. ) ;
#12237=CARTESIAN_POINT ( 'NONE',  ( 146.8516045228164160, 276.2925551239072774, 3.995954059407343273 ) ) ;
#12240=B_SPLINE_CURVE_WITH_KNOTS ( 'NONE', 3,
 ( #35701, #66600, #58001, #58968, #89940, #5307, #82357, #42779, #67590, #20016, #75214, #89461, #36184, #21503, #4817, #74729, #19536, #67089, #50893, #21022, #28590, #81842, #83332, #12418, #43285, #97527, #12925, #59472, #98013, #58486, #51904, #50398, #74230, #35197, #90948, #11922, #81352, #73713, #28097, #82845, #13416, #20516, #27118, #42289, #51393, #4295, #88983, #43784 ),
 .UNSPECIFIED., .F., .F.,
 ( 4, 2, 2, 2, 2, 2, 2, 2, 2, 2, 2, 2, 2, 2, 2, 2, 2, 2, 2, 2, 2, 2, 2, 4 ),
 ( 0.002594831937057109125, 0.003014445506990537805, 0.003224252291957272962, 0.003329155684440719687, 0.003434059076924166412, 0.003538962469407613137, 0.003643865861891059862, 0.003853672646858035278, 0.004273286216791986544, 0.005112513356659858718, 0.005951740496527732627, 0.006790967636395604801, 0.007210581206329462825, 0.007630194776263320849, 0.007735098168746732880, 0.007787549864988394660, 0.007840001561230058175, 0.007944904953713385204, 0.008049808346196712233, 0.008469421916130011677, 0.008679228701096703899, 0.008889035486063394387, 0.009098842271030084874, 0.009308649055996777097 ),
 .UNSPECIFIED. ) ;
#12241=CARTESIAN_POINT ( 'NONE',  ( 171.8245779312147477, 251.1353067130050363, 3.410672705103630076 ) ) ;
#12243=CARTESIAN_POINT ( 'NONE',  ( 190.7805732161387766, 300.2053494229706985, 4.237982805666590025 ) ) ;
#12245=CARTESIAN_POINT ( 'NONE',  ( 169.3462360422239499, 285.1681312824781571, -8.761088339260869162 ) ) ;
#12248=CARTESIAN_POINT ( 'NONE',  ( 157.4719395156559472, 271.1205387963237854, -14.65500712271581385 ) ) ;
#12250=CARTESIAN_POINT ( 'NONE',  ( 136.7639277290221855, 239.7677522451417929, -5.000000000000041744 ) ) ;
#12253=CARTESIAN_POINT ( 'NONE',  ( 157.8763546842245376, 257.1971277035954699, 17.68444922773363004 ) ) ;
#12254=CARTESIAN_POINT ( 'NONE',  ( 150.8247211172754589, 269.4109153179094278, -14.37608026040300402 ) ) ;
#12255=CARTESIAN_POINT ( 'NONE',  ( -0.3657822996961275219, 170.5958772461660544, -9.188101187500095079 ) ) ;
#12256=CARTESIAN_POINT ( 'NONE',  ( 63.88265089144443465, 201.5643266524160424, 9.188101187500095079 ) ) ;
#12260=CARTESIAN_POINT ( 'NONE',  ( 205.2660270307054304, 275.1158074454486382, -13.97598661256119179 ) ) ;
#12261=CARTESIAN_POINT ( 'NONE',  ( 191.5311128828054734, 291.7127007975493598, -14.32894664656410910 ) ) ;
#12262=CARTESIAN_POINT ( 'NONE',  ( 146.8881680668833951, 276.2292252078784145, 4.973452195244782104 ) ) ;
#12264=CARTESIAN_POINT ( 'NONE',  ( 170.8805640699686990, 257.7213711969266114, 14.63406020945912367 ) ) ;
#12265=CARTESIAN_POINT ( 'NONE',  ( 75.63696797857055287, 201.1427522451417644, 1.119607411625061291E-15 ) ) ;
#12267=CARTESIAN_POINT ( 'NONE',  ( 178.7496050114017123, 254.0362436929630121, -4.160075916196277035 ) ) ;
#12269=CARTESIAN_POINT ( 'NONE',  ( 151.0254882145115971, 269.0631765050081299, 14.78274390654921078 ) ) ;
#12270=CARTESIAN_POINT ( 'NONE',  ( 42.09652578138359047, 195.1115022471902591, 10.00000000000009592 ) ) ;
#12271=CARTESIAN_POINT ( 'NONE',  ( 181.7891714221429709, 291.6511982500477984, 9.251581008942281414 ) ) ;
#12273=CARTESIAN_POINT ( 'NONE',  ( 1.284818304444202530, 180.7369531367911293, -4.594050593750048428 ) ) ;
#12274=CARTESIAN_POINT ( 'NONE',  ( 167.7976356284401334, 287.1346734032483710, 5.039741953860431778 ) ) ;
#12275=CARTESIAN_POINT ( 'NONE',  ( 153.1973045377566507, 265.3014802884401320, 17.70608187426261892 ) ) ;
#12278=CARTESIAN_POINT ( 'NONE',  ( 207.1122325394003951, 271.9180857031755636, 7.794245785756032774 ) ) ;
#12279=CARTESIAN_POINT ( 'NONE',  ( 193.7275870247597425, 295.1009717758319084, 14.48058678254265885 ) ) ;
#12281=CARTESIAN_POINT ( 'NONE',  ( 176.6809650034762740, 260.2657671503346251, -13.65821825376172782 ) ) ;
#12290=ORIENTED_EDGE ( 'NONE', *, *, #25559, .F. ) ;
#12294=CARTESIAN_POINT ( 'NONE',  ( 190.0534303668326288, 269.9073674132432643, 15.26070177760127322 ) ) ;
#12296=CARTESIAN_POINT ( 'NONE',  ( 153.1973045377566507, 265.3014802884401320, 17.70608187426261892 ) ) ;
#12301=VERTEX_POINT ( 'NONE', #83419 ) ;
#12303=CARTESIAN_POINT ( 'NONE',  ( 164.8271680874279923, 246.4386526519062102, -4.335244565372774694 ) ) ;
#12305=CARTESIAN_POINT ( 'NONE',  ( 153.1314981037513121, 265.4154603756023789, 17.73969815997475408 ) ) ;
#12308=CARTESIAN_POINT ( 'NONE',  ( 174.3163775853039965, 262.5928350672832607, 14.99201191324070948 ) ) ;
#12309=ORIENTED_EDGE ( 'NONE', *, *, #85833, .F. ) ;
#12311=CARTESIAN_POINT ( 'NONE',  ( 76.55480823776410659, 226.5530062829863027, -4.648177544792955347E-16 ) ) ;
#12314=CARTESIAN_POINT ( 'NONE',  ( 167.5922211047578401, 275.0307474144973980, -15.21854255687822999 ) ) ;
#12317=CARTESIAN_POINT ( 'NONE',  ( 177.5270958125545064, 279.1683514342866488, -16.05247689478367690 ) ) ;
#12318=CARTESIAN_POINT ( 'NONE',  ( 168.9651915494897878, 261.4198009647504932, -16.16106606682127023 ) ) ;
#12324=ORIENTED_EDGE ( 'NONE', *, *, #57378, .T. ) ;
#12325=( BOUNDED_CURVE ( )  B_SPLINE_CURVE ( 2, ( #18460, #65536, #64548, #50828, #12352, #35635, #28031, #17963, #48860 ),
 .UNSPECIFIED., .F., .T. ) 
 B_SPLINE_CURVE_WITH_KNOTS ( ( 3, 2, 2, 2, 3 ),
 ( 0.4314516129032258118, 0.4327956989247311870, 0.4354838709677419373, 0.4381720430107526876, 0.4395161290322580627 ),
 .UNSPECIFIED. ) 
 CURVE ( )  GEOMETRIC_REPRESENTATION_ITEM ( )  RATIONAL_B_SPLINE_CURVE ( ( 0.9330127018922194093, 0.9330127018922194093, 1.000000000000000000, 0.8660254037844387076, 1.000000000000000000, 0.8660254037844387076, 1.000000000000000000, 0.9330127018922194093, 0.9330127018922194093 ) ) 
 REPRESENTATION_ITEM ( '' )  );
#12330=CARTESIAN_POINT ( 'NONE',  ( 157.5215017335775940, 258.4853116787141971, -16.92298772477023761 ) ) ;
#12331=CARTESIAN_POINT ( 'NONE',  ( 178.1054448038686076, 292.3333982356375600, 7.160286041890884690 ) ) ;
#12332=CARTESIAN_POINT ( 'NONE',  ( 158.5163285992952922, 256.0886603671742705, -16.16665996632518798 ) ) ;
#12333=ORIENTED_EDGE ( 'NONE', *, *, #93576, .F. ) ;
#12335=CARTESIAN_POINT ( 'NONE',  ( 164.9356397357043704, 244.9700873293209042, 2.799217332519396972 ) ) ;
#12336=CARTESIAN_POINT ( 'NONE',  ( 196.5475899070771675, 290.2165835061676944, -17.89382743182097002 ) ) ;
#12337=CARTESIAN_POINT ( 'NONE',  ( 164.8616299252405213, 245.0982760813026857, 1.544363874765093625 ) ) ;
#12338=CARTESIAN_POINT ( 'NONE',  ( 198.4706398937704819, 286.8857632237200619, 17.04020736381253798 ) ) ;
#12339=ORIENTED_EDGE ( 'NONE', *, *, #3999, .F. ) ;
#12341=CARTESIAN_POINT ( 'NONE',  ( 146.6710848822482660, 276.6052243131355226, -3.256337828262574785 ) ) ;
#12344=CARTESIAN_POINT ( 'NONE',  ( 118.1240276194171770, 250.5530062829863311, -4.648177544792955347E-16 ) ) ;
#12346=CARTESIAN_POINT ( 'NONE',  ( 159.8797902884228392, 253.7270754474314458, -15.26054831571763160 ) ) ;
#12347=EDGE_CURVE ( 'NONE', #90262, #5319, #83469, .T. ) ;
#12348=CARTESIAN_POINT ( 'NONE',  ( 189.9902393611022546, 301.5742478148356440, 0.007239494267619051016 ) ) ;
#12349=ORIENTED_EDGE ( 'NONE', *, *, #29235, .T. ) ;
#12350=CARTESIAN_POINT ( 'NONE',  ( 170.5099130517262722, 255.7343107893726994, -11.93865830361121816 ) ) ;
#12352=CARTESIAN_POINT ( 'NONE',  ( 56.38594494382682853, 203.3615022471902307, -10.00000000000009592 ) ) ;
#12353=ADVANCED_FACE ( 'NONE', ( #74321 ), #37763, .T. ) ;
#12354=DIRECTION ( 'NONE',  ( -0.8660254037844387076, -0.4999999999999998890, -0.000000000000000000 ) ) ;
#12356=CARTESIAN_POINT ( 'NONE',  ( 20.28351092001508960, 192.5177522451419350, 5.000000000000046185 ) ) ;
#12357=CARTESIAN_POINT ( 'NONE',  ( 108.2124997955428967, 221.0327760586659451, 1.948934522072302763E-15 ) ) ;
#12358=CARTESIAN_POINT ( 'NONE',  ( 162.1227137712282342, 251.8422180177273901, -14.11218862277787345 ) ) ;
#12359=CARTESIAN_POINT ( 'NONE',  ( 162.6150040737615257, 249.4375296638992268, -10.77107874254045505 ) ) ;
#12360=CARTESIAN_POINT ( 'NONE',  ( 96.20275958967147290, 237.8967562850346837, -4.648177544792955347E-16 ) ) ;
#12361=CARTESIAN_POINT ( 'NONE',  ( 171.3649617487770911, 251.0102673366500596, 7.372720983288576946 ) ) ;
#12362=CARTESIAN_POINT ( 'NONE',  ( 28.21305602519035460, 187.0958772461660544, -9.188101187500095079 ) ) ;
#12364=DIRECTION ( 'NONE',  ( -0.8660254037844387076, -0.4999999999999998890, -0.000000000000000000 ) ) ;
#12367=ORIENTED_EDGE ( 'NONE', *, *, #45328, .T. ) ;
#12368=CARTESIAN_POINT ( 'NONE',  ( 142.9371257517045137, 259.7655487066560340, -7.305945665944389766 ) ) ;
#12371=AXIS2_PLACEMENT_3D ( 'NONE', #30121, #45800, #15913 ) ;
#12373=CARTESIAN_POINT ( 'NONE',  ( -22.42236680055709641, 157.8615022471902591, 0.000000000000000000 ) ) ;
#12374=CARTESIAN_POINT ( 'NONE',  ( 176.1793590593251224, 285.1801416094290289, -12.37630502171867697 ) ) ;
#12376=CARTESIAN_POINT ( 'NONE',  ( 55.46605327235566563, 193.6423013555410080, -4.594050593750043987 ) ) ;
#12377=CARTESIAN_POINT ( 'NONE',  ( 89.49337443912149581, 229.1427522451419065, 10.00000000000009237 ) ) ;
#12379=CARTESIAN_POINT ( 'NONE',  ( 196.5569465129259186, 267.2703004868020003, -7.811843761257617480 ) ) ;
#12380=CYLINDRICAL_SURFACE ( 'NONE', #84138, 10.00000000000010658 ) ;
#12381=CARTESIAN_POINT ( 'NONE',  ( 208.3829315663354862, 269.7171704273955015, -1.768817828503133072 ) ) ;
#12383=CARTESIAN_POINT ( 'NONE',  ( -9.405095999578703569, 171.5024278399160949, 9.188101187500095079 ) ) ;
#12384=CARTESIAN_POINT ( 'NONE',  ( 198.8194531333411419, 286.2816009704309863, -17.01510935557533344 ) ) ;
#12385=VECTOR ( 'NONE', #55762, 1000.000000000000000 ) ;
#12386=DIRECTION ( 'NONE',  ( 0.4999999999999998890, -0.8660254037844385966, 0.000000000000000000 ) ) ;
#12387=CARTESIAN_POINT ( 'NONE',  ( 192.9633865298379476, 296.4246058602058156, -11.85717392250713864 ) ) ;
#12389=CARTESIAN_POINT ( 'NONE',  ( 49.48463145776311478, 205.5024278399160949, -9.188101187500093303 ) ) ;
#12390=CARTESIAN_POINT ( 'NONE',  ( 164.0854748117396582, 246.4426161724408928, -5.757837433625331514 ) ) ;
#12395=CARTESIAN_POINT ( 'NONE',  ( 5.723458822437168081, 174.1115022471902591, 10.00000000000009592 ) ) ;
#12397=CARTESIAN_POINT ( 'NONE',  ( 115.9249311304092771, 246.9244531367911293, -4.594050593750046652 ) ) ;
#12399=CARTESIAN_POINT ( 'NONE',  ( 171.3751619920873281, 280.2398791927632828, 15.33202389549764888 ) ) ;
#12400=CARTESIAN_POINT ( 'NONE',  ( 45.39824762976388683, 187.0177522451417929, 5.000000000000051514 ) ) ;
#12402=CARTESIAN_POINT ( 'NONE',  ( 157.2744851780909414, 258.2395962677452985, 18.17792129701959070 ) ) ;
#12403=CARTESIAN_POINT ( 'NONE',  ( 187.4983404922351156, 288.8742233168966891, 14.46822738816536358 ) ) ;
#12406=CARTESIAN_POINT ( 'NONE',  ( 191.5766842709549280, 298.8264446275616137, 8.039910086100929831 ) ) ;
#12407=CARTESIAN_POINT ( 'NONE',  ( 163.4933893861717706, 247.4681382119453588, 7.531590497957860286 ) ) ;
#12408=EDGE_CURVE ( 'NONE', #99455, #88304, #37472, .T. ) ;
#12410=CARTESIAN_POINT ( 'NONE',  ( 172.9301907270271954, 268.1031614781803114, -16.30088698181723927 ) ) ;
#12412=EDGE_LOOP ( 'NONE', ( #93334, #99067, #49693, #28617 ) ) ;
#12414=CARTESIAN_POINT ( 'NONE',  ( 170.6697357073235253, 284.5009364175209043, -11.68571669126542822 ) ) ;
#12417=CARTESIAN_POINT ( 'NONE',  ( 196.2233686317883326, 270.8944000944912887, 13.08481226931415442 ) ) ;
#12418=CARTESIAN_POINT ( 'NONE',  ( 185.1111192456979211, 296.2605552703855096, 4.659568135049322990 ) ) ;
#12420=CARTESIAN_POINT ( 'NONE',  ( 148.4964438259718520, 274.1392353305065512, -7.906637339856966484 ) ) ;
#12423=ORIENTED_EDGE ( 'NONE', *, *, #9942, .F. ) ;
#12425=ADVANCED_FACE ( 'NONE', ( #21589 ), #48592, .F. ) ;
#12426=CARTESIAN_POINT ( 'NONE',  ( 147.6264044922760377, 274.9505622111005323, -8.841872555777701592 ) ) ;
#12427=CARTESIAN_POINT ( 'NONE',  ( 156.1012082241142309, 261.7660268653759772, -17.00573470575184487 ) ) ;
#12430=CARTESIAN_POINT ( 'NONE',  ( 185.4183139185963967, 291.0678344243584093, 12.11208453829537213 ) ) ;
#12431=CARTESIAN_POINT ( 'NONE',  ( 204.7610021263893429, 275.9905362388115577, 13.36619428527026976 ) ) ;
#12432=CARTESIAN_POINT ( 'NONE',  ( 20.30386484825465132, 170.9824982072973967, 3.021315404115420679E-15 ) ) ;
#12433=VECTOR ( 'NONE', #79439, 1000.000000000000000 ) ;
#12435=ORIENTED_EDGE ( 'NONE', *, *, #58313, .F. ) ;
#12436=CARTESIAN_POINT ( 'NONE',  ( 85.53328598605538957, 214.0643266524159856, -9.188101187500093303 ) ) ;
#12437=CARTESIAN_POINT ( 'NONE',  ( 155.1411698516235163, 261.9346068017520679, 17.17606690776768374 ) ) ;
#12440=ORIENTED_EDGE ( 'NONE', *, *, #94458, .T. ) ;
#12441=ORIENTED_EDGE ( 'NONE', *, *, #90113, .F. ) ;
#12442=CARTESIAN_POINT ( 'NONE',  ( 207.1906716859447499, 270.1669981132436078, 1.693978511116863261 ) ) ;
#12448=CARTESIAN_POINT ( 'NONE',  ( 202.8535267948003593, 279.2943804273081696, -15.36804658072946062 ) ) ;
#12450=CARTESIAN_POINT ( 'NONE',  ( 182.7578341729287104, 280.0865842805126249, -16.17247614028536873 ) ) ;
#12452=CARTESIAN_POINT ( 'NONE',  ( 152.1671311979278016, 269.0857928536317445, 15.36489295260887822 ) ) ;
#12453=CARTESIAN_POINT ( 'NONE',  ( 200.9061540366740246, 282.6673289856585143, -18.13083321883407351 ) ) ;
#12456=CARTESIAN_POINT ( 'NONE',  ( 138.9828575061699496, 260.2369531367911009, -4.594050593750048428 ) ) ;
#12457=CARTESIAN_POINT ( 'NONE',  ( 156.8640796903996488, 258.9504394241315595, -18.30920512684366841 ) ) ;
#12459=FACE_OUTER_BOUND ( 'NONE', #11848, .T. ) ;
#12462=CARTESIAN_POINT ( 'NONE',  ( 160.5893190321802138, 270.9897182155185078, 16.60663562724527864 ) ) ;
#12463=CARTESIAN_POINT ( 'NONE',  ( 200.1100745001128303, 270.2489798220258308, 9.265985437337555197 ) ) ;
#12469=CARTESIAN_POINT ( 'NONE',  ( 160.0293279782301568, 280.7546693694226860, -6.628616199906209872 ) ) ;
#12475=CARTESIAN_POINT ( 'NONE',  ( 194.6016098382413873, 292.7469416705026788, 15.11077049397369976 ) ) ;
#12476=EDGE_LOOP ( 'NONE', ( #12997, #60780, #7426 ) ) ;
#12477=CARTESIAN_POINT ( 'NONE',  ( 184.6983412747724742, 272.9958233129013934, -16.41604421047053464 ) ) ;
#12480=CARTESIAN_POINT ( 'NONE',  ( 160.0377410834880720, 276.7385967903648520, 13.05697007622473294 ) ) ;
#12482=B_SPLINE_CURVE_WITH_KNOTS ( 'NONE', 3,
 ( #50178, #11699, #50664, #26391 ),
 .UNSPECIFIED., .F., .F.,
 ( 4, 4 ),
 ( 0.01264251196720198728, 0.01893505409154686361 ),
 .UNSPECIFIED. ) ;
#12483=CARTESIAN_POINT ( 'NONE',  ( 156.7047097395129924, 276.7985503127216020, 10.01792283833032648 ) ) ;
#12484=CARTESIAN_POINT ( 'NONE',  ( 204.2264919259983174, 276.9163350630529976, -14.79221891897802799 ) ) ;
#12489=CARTESIAN_POINT ( 'NONE',  ( 203.4034827258358007, 270.0124503379752241, 5.894888531434947510 ) ) ;
#12495=CARTESIAN_POINT ( 'NONE',  ( 175.3447835617839985, 290.8124204970986284, 2.566043682277154847 ) ) ;
#12496=CARTESIAN_POINT ( 'NONE',  ( 192.4454213697443095, 297.3217478340386606, 12.58566886711101596 ) ) ;
#12499=CARTESIAN_POINT ( 'NONE',  ( 8.700681467995980967, 166.6423013555410080, -4.594050593750043987 ) ) ;
#12500=CARTESIAN_POINT ( 'NONE',  ( 100.0117143358702236, 237.7369531367911009, -4.594050593750048428 ) ) ;
#12502=CARTESIAN_POINT ( 'NONE',  ( 179.9032037953561201, 255.0686240464731895, -2.409017592585954937 ) ) ;
#12506=DIRECTION ( 'NONE',  ( -0.8660254037844387076, -0.4999999999999998890, -0.000000000000000000 ) ) ;
#12507=CARTESIAN_POINT ( 'NONE',  ( 147.7112127936102866, 274.8036699242858276, -9.124700685424272706 ) ) ;
#12509=CARTESIAN_POINT ( 'NONE',  ( 196.5044318023951178, 266.6999416850621287, 8.135797318270522993 ) ) ;
#12511=CARTESIAN_POINT ( 'NONE',  ( 162.3863246888976732, 251.8997027923403493, -12.94925132143062463 ) ) ;
#12513=CARTESIAN_POINT ( 'NONE',  ( 172.7048577836360721, 263.2835701223090155, -15.44053096649166079 ) ) ;
#12514=CARTESIAN_POINT ( 'NONE',  ( 73.24602992621615272, 225.3464784336661353, 1.353441290958777327E-15 ) ) ;
#12516=CARTESIAN_POINT ( 'NONE',  ( 151.4025156491502742, 268.4101458323662541, 14.71049357081981235 ) ) ;
#12518=CARTESIAN_POINT ( 'NONE',  ( 157.8849654228661166, 257.1822134667773980, 17.43614750057631468 ) ) ;
#12520=CARTESIAN_POINT ( 'NONE',  ( 148.9874996956617395, 272.5930761648982070, 12.54755420039906078 ) ) ;
#12521=CARTESIAN_POINT ( 'NONE',  ( 198.9590707264871412, 286.0397762054715827, -17.05306195936250191 ) ) ;
#12525=CARTESIAN_POINT ( 'NONE',  ( 192.8301672656986341, 296.6553483942417415, -13.40355799340913556 ) ) ;
#12530=CARTESIAN_POINT ( 'NONE',  ( 146.9129474150286683, 276.1863061179126930, -5.016087650759920358 ) ) ;
#12531=CARTESIAN_POINT ( 'NONE',  ( 188.1389331190833047, 286.0020158130019468, -16.24451441855859102 ) ) ;
#12534=CARTESIAN_POINT ( 'NONE',  ( 155.2602186481262265, 267.5823991184574879, 15.87441468340182382 ) ) ;
#12536=CARTESIAN_POINT ( 'NONE',  ( 144.7927049134883077, 247.7365022471901739, -10.00000000000009059 ) ) ;
#12537=CARTESIAN_POINT ( 'NONE',  ( 17.41480177352709191, 180.8615022471902591, -10.00000000000009592 ) ) ;
#12541=CARTESIAN_POINT ( 'NONE',  ( 191.1126307253469747, 299.2020206802192206, -6.759625617318037349 ) ) ;
#12542=CARTESIAN_POINT ( 'NONE',  ( 169.5007657120409874, 248.2156828994837099, -1.963647642838588503 ) ) ;
#12544=CARTESIAN_POINT ( 'NONE',  ( 196.9385840439278752, 265.2769846543552035, -4.547345364390803724 ) ) ;
#12547=ORIENTED_EDGE ( 'NONE', *, *, #33282, .F. ) ;
#12551=CARTESIAN_POINT ( 'NONE',  ( 158.3546312691470348, 256.3687283584388865, 16.55374228798595126 ) ) ;
#12553=CARTESIAN_POINT ( 'NONE',  ( 204.1541407990405332, 272.6956988606675623, 11.22829397770025395 ) ) ;
#12554=CARTESIAN_POINT ( 'NONE',  ( 153.2906404175950854, 265.1398178023911782, -17.60231834963988007 ) ) ;
#12558=CARTESIAN_POINT ( 'NONE',  ( 164.6179597924970039, 274.5158082661938579, 14.71820543651746327 ) ) ;
#12560=CARTESIAN_POINT ( 'NONE',  ( 189.6662795060866529, 300.6105458049610775, 0.3572493495538390240 ) ) ;
#12563=CARTESIAN_POINT ( 'NONE',  ( 182.8792571200491750, 296.1546806419740960, 0.3348460080343949041 ) ) ;
#12565=CARTESIAN_POINT ( 'NONE',  ( 165.9605670965306672, 274.2117924623952376, -15.14287719899917661 ) ) ;
#12567=CARTESIAN_POINT ( 'NONE',  ( 19.16720650933548953, 170.3262482093457777, 3.021315404115420679E-15 ) ) ;
#12568=CARTESIAN_POINT ( 'NONE',  ( 156.5981606942930853, 279.2183417136616868, -8.654364236849055203 ) ) ;
#12570=CARTESIAN_POINT ( 'NONE',  ( 167.3807934234146160, 286.2060637682922675, -4.770210317880093420 ) ) ;
#12573=CARTESIAN_POINT ( 'NONE',  ( 98.87557663705065636, 218.7048013555409796, 4.594050593750051981 ) ) ;
#12574=ORIENTED_EDGE ( 'NONE', *, *, #41613, .T. ) ;
#12576=CARTESIAN_POINT ( 'NONE',  ( 188.4688990864094080, 295.3997683978527675, -11.43812978727723717 ) ) ;
#12577=CARTESIAN_POINT ( 'NONE',  ( 110.2137735815727808, 245.9860189848785126, -2.679491924311252493 ) ) ;
#12585=CARTESIAN_POINT ( 'NONE',  ( 176.7716622781765921, 292.6737166345459968, -2.766366243292323279 ) ) ;
#12586=B_SPLINE_SURFACE_WITH_KNOTS ( 'NONE', 3, 1, ( 
 ( #91713, #60749 ),
 ( #22274, #7070 ),
 ( #15662, #46053 ),
 ( #29877, #76969 ),
 ( #53178, #23260 ),
 ( #22782, #68863 ),
 ( #99788, #30378 ),
 ( #7569, #38459 ),
 ( #38959, #100292 ),
 ( #30876, #92710 ),
 ( #46557, #52665 ),
 ( #85111, #8086 ),
 ( #69865, #31367 ),
 ( #62251, #93205 ),
 ( #52168, #13687 ),
 ( #91213, #75495 ),
 ( #6080, #67885 ),
 ( #29388, #83619 ),
 ( #21775, #79523 ),
 ( #9595, #2490 ),
 ( #62759, #39447 ),
 ( #17682, #16175 ),
 ( #93717, #64784 ),
 ( #56154, #10584 ),
 ( #78493, #1490 ),
 ( #70368, #79008 ),
 ( #23760, #47071 ),
 ( #87653, #32373 ),
 ( #18184, #41457 ),
 ( #72399, #48582 ),
 ( #17167, #8582 ),
 ( #3007, #86632 ),
 ( #33372, #87150 ),
 ( #24768, #978 ) ),
 .UNSPECIFIED., .T., .F., .F.,
 ( 4, 2, 2, 2, 2, 2, 2, 2, 2, 2, 2, 2, 2, 2, 2, 2, 4 ),
 ( 2, 2 ),
 ( 0.000000000000000000, 0.06250000000000000000, 0.1250000000000000000, 0.1875000000000000000, 0.2500000000000000000, 0.3125000000000000000, 0.3750000000000000000, 0.4375000000000000000, 0.5000000000000000000, 0.5625000000000000000, 0.6250000000000000000, 0.6875000000000000000, 0.7500000000000000000, 0.8125000000000000000, 0.8750000000000000000, 0.9375000000000000000, 1.000000000000000000 ),
 ( 0.000000000000000000, 1.000000000000000000 ),
 .UNSPECIFIED. ) ;
#12587=CARTESIAN_POINT ( 'NONE',  ( 196.4677102463732012, 290.3549391369982686, 16.45225250689336249 ) ) ;
#12589=CARTESIAN_POINT ( 'NONE',  ( 208.2161171980831682, 270.0061013886409569, 2.944709006235987747 ) ) ;
#12590=B_SPLINE_CURVE_WITH_KNOTS ( 'NONE', 3,
 ( #32149, #99575, #22563, #92017 ),
 .UNSPECIFIED., .F., .F.,
 ( 4, 4 ),
 ( 0.000000000000000000, 0.004985884173467201863 ),
 .UNSPECIFIED. ) ;
#12593=AXIS2_PLACEMENT_3D ( 'NONE', #15827, #68535, #52833 ) ;
#12595=CARTESIAN_POINT ( 'NONE',  ( 207.6050568035884680, 271.0644890383991310, -1.456818755242089702 ) ) ;
#12598=CARTESIAN_POINT ( 'NONE',  ( 191.3831180832644066, 263.8491544962765829, -8.012675887993349733 ) ) ;
#12601=CARTESIAN_POINT ( 'NONE',  ( 134.7341806906763395, 248.5958772461660544, -9.188101187500095079 ) ) ;
#12602=FACE_OUTER_BOUND ( 'NONE', #13312, .T. ) ;
#12603=CARTESIAN_POINT ( 'NONE',  ( 155.5777206977276990, 264.9826732634378459, -17.41861857130547975 ) ) ;
#12604=VERTEX_POINT ( 'NONE', #16724 ) ;
#12606=FACE_OUTER_BOUND ( 'NONE', #98322, .T. ) ;
#12609=CARTESIAN_POINT ( 'NONE',  ( 159.5895502557670795, 254.2297859303815244, -16.92708575547316485 ) ) ;
#12610=ADVANCED_FACE ( 'NONE', ( #78543, #9131 ), #18237, .F. ) ;
#12611=CARTESIAN_POINT ( 'NONE',  ( 172.3471576652249269, 251.0617913708788649, -0.2555901567849299671 ) ) ;
#12612=CARTESIAN_POINT ( 'NONE',  ( 34.73530984921583098, 200.8615022471903160, 5.000000000000046185 ) ) ;
#12614=CARTESIAN_POINT ( 'NONE',  ( 199.0981677397162457, 281.8773224221018268, -16.59884707263596226 ) ) ;
#12618=CARTESIAN_POINT ( 'NONE',  ( 206.7147678843052461, 272.1735785942267967, 6.914908267696407762 ) ) ;
#12619=CARTESIAN_POINT ( 'NONE',  ( 167.5937759011995638, 249.9759899836699901, 7.306980044439311150 ) ) ;
#12622=FACE_OUTER_BOUND ( 'NONE', #10470, .T. ) ;
#12628=( BOUNDED_CURVE ( )  B_SPLINE_CURVE ( 2, ( #35062, #4165, #52254, #89336, #44147, #19408, #11307, #73101, #27489 ),
 .UNSPECIFIED., .F., .T. ) 
 B_SPLINE_CURVE_WITH_KNOTS ( ( 3, 2, 2, 2, 3 ),
 ( 0.8266129032258064946, 0.8279569892473118697, 0.8306451612903226200, 0.8333333333333333703, 0.8346774193548387455 ),
 .UNSPECIFIED. ) 
 CURVE ( )  GEOMETRIC_REPRESENTATION_ITEM ( )  RATIONAL_B_SPLINE_CURVE ( ( 0.9330127018922194093, 0.9330127018922194093, 1.000000000000000000, 0.8660254037844387076, 1.000000000000000000, 0.8660254037844387076, 1.000000000000000000, 0.9330127018922194093, 0.9330127018922194093 ) ) 
 REPRESENTATION_ITEM ( '' )  );
#12631=CARTESIAN_POINT ( 'NONE',  ( 14.59995888762994554, 188.4244531367911293, -4.594050593750046652 ) ) ;
#12632=B_SPLINE_CURVE_WITH_KNOTS ( 'NONE', 3,
 ( #87814, #64945, #42126, #73058, #26451, #57326, #34055, #81183, #18352, #95890, #56828, #64442, #88298, #50718, #18854, #96373, #34532, #49735, #66430, #80688, #26939, #49245, #11263, #41624, #50228, #3652, #65432, #41119, #57824, #88802, #27447, #19850, #4127, #89296, #58321, #19369, #11750, #80182, #72052, #35021, #42613, #73544, #12245, #65923, #72566, #96880, #89770, #43104, #10748, #81671 ),
 .UNSPECIFIED., .F., .F.,
 ( 4, 2, 2, 2, 2, 2, 2, 2, 2, 2, 2, 2, 2, 2, 2, 2, 2, 2, 2, 2, 2, 2, 2, 2, 4 ),
 ( 0.0001458946000596443712, 0.001144903916429049467, 0.001644408574613814844, 0.001894160903706147443, 0.002019037068252331306, 0.002143913232798515169, 0.002268789397344698599, 0.002393665561890882029, 0.002643417890983249322, 0.003142922549168039419, 0.004141931865537725431, 0.005140941181907411443, 0.005640445840092211081, 0.005890198169184619574, 0.006139950498277027199, 0.006202388580550207385, 0.006264826662823387571, 0.006327264745096566889, 0.006389702827369747942, 0.006639455156462413174, 0.006889207485555077538, 0.007138959814647742770, 0.007388712143740408869, 0.007638464472833074101, 0.008137969131018543342 ),
 .UNSPECIFIED. ) ;
#12633=CARTESIAN_POINT ( 'NONE',  ( 42.09652578138355494, 205.1115022471903160, -5.000000000000047962 ) ) ;
#12639=CARTESIAN_POINT ( 'NONE',  ( 60.33744616864313315, 196.4548013555410080, -4.594050593750042211 ) ) ;
#12641=EDGE_CURVE ( 'NONE', #82130, #76711, #40002, .T. ) ;
#12642=CARTESIAN_POINT ( 'NONE',  ( 161.6707029936031574, 250.6251236501384483, 14.45053103226186231 ) ) ;
#12643=CARTESIAN_POINT ( 'NONE',  ( 170.9744194226895786, 287.2191983458180857, 7.031205856223269102 ) ) ;
#12644=CARTESIAN_POINT ( 'NONE',  ( 146.8881680668833951, 276.2292252078784145, 4.973452195244782104 ) ) ;
#12647=CARTESIAN_POINT ( 'NONE',  ( 178.8525359564782775, 293.5924254160544820, 2.661079731265041382 ) ) ;
#12649=CARTESIAN_POINT ( 'NONE',  ( 176.1198908959743221, 274.8737079364501597, 17.13331764512671285 ) ) ;
#12650=CARTESIAN_POINT ( 'NONE',  ( 165.9091197491159164, 246.2627970730538323, -2.747640711776688338 ) ) ;
#12652=CARTESIAN_POINT ( 'NONE',  ( 91.36976281398784749, 216.8927522451417929, -10.00000000000009237 ) ) ;
#12656=CARTESIAN_POINT ( 'NONE',  ( 98.82118972926437550, 217.8615022471902023, 5.000000000000051514 ) ) ;
#12658=CARTESIAN_POINT ( 'NONE',  ( 161.7100178915388824, 267.7548849422799435, -16.97131824026628877 ) ) ;
#12659=VERTEX_POINT ( 'NONE', #31416 ) ;
#12660=CARTESIAN_POINT ( 'NONE',  ( 52.62397354648171444, 207.3149278399161233, 9.188101187500093303 ) ) ;
#12662=CARTESIAN_POINT ( 'NONE',  ( 52.94219725692860834, 189.8262482093458061, 3.021315404115420679E-15 ) ) ;
#12663=CARTESIAN_POINT ( 'NONE',  ( 147.5177358149801421, 275.1387818813681179, 4.867883209065928085 ) ) ;
#12668=CARTESIAN_POINT ( 'NONE',  ( 164.3274319858398087, 246.0235340536434592, -1.770631424362269168 ) ) ;
#12671=CARTESIAN_POINT ( 'NONE',  ( 188.8667127848526661, 265.4704850057313479, 10.73802221655500233 ) ) ;
#12672=CARTESIAN_POINT ( 'NONE',  ( 148.9322735291567597, 272.6887306911919495, -12.40988026045598858 ) ) ;
#12673=CARTESIAN_POINT ( 'NONE',  ( 157.0808507922293131, 258.5749808621497436, 16.84357500595720580 ) ) ;
#12677=CARTESIAN_POINT ( 'NONE',  ( 175.3131846714599362, 254.5210658486609532, 7.854781054984586675 ) ) ;
#12681=CARTESIAN_POINT ( 'NONE',  ( 182.3022624411334220, 284.0886791389093560, 14.96227919629477832 ) ) ;
#12684=CARTESIAN_POINT ( 'NONE',  ( 159.3995226465659982, 254.5589234043588078, -16.81133486613867234 ) ) ;
#12688=CARTESIAN_POINT ( 'NONE',  ( 161.1492466472929266, 251.5283125358769212, -13.33353587056634915 ) ) ;
#12689=CARTESIAN_POINT ( 'NONE',  ( 54.85235828774394662, 209.1427522451419350, -10.00000000000009592 ) ) ;
#12693=DIRECTION ( 'NONE',  ( 0.4999999999999998890, -0.8660254037844385966, 0.000000000000000000 ) ) ;
#12696=CARTESIAN_POINT ( 'NONE',  ( 118.9560200436548314, 248.6744531367911293, 4.594050593750047540 ) ) ;
#12697=CARTESIAN_POINT ( 'NONE',  ( 150.6571681785161445, 269.7011255207979730, 15.24894850018880454 ) ) ;
#12699=ORIENTED_EDGE ( 'NONE', *, *, #90708, .T. ) ;
#12700=CARTESIAN_POINT ( 'NONE',  ( 201.2142882557298265, 280.3114506667780574, 16.76591128755623572 ) ) ;
#12701=ORIENTED_EDGE ( 'NONE', *, *, #41723, .F. ) ;
#12706=CARTESIAN_POINT ( 'NONE',  ( 73.21957404993666785, 203.8923013555409796, 4.594050593750050204 ) ) ;
#12707=CARTESIAN_POINT ( 'NONE',  ( 175.4967466201937611, 291.2628096033125189, 6.560984766252938805 ) ) ;
#12708=CARTESIAN_POINT ( 'NONE',  ( 194.6050500505458842, 285.5465367126718093, -17.70104686455487553 ) ) ;
#12709=CARTESIAN_POINT ( 'NONE',  ( 150.5355989389948093, 269.9116896202863245, 15.28294032643914768 ) ) ;
#12710=CARTESIAN_POINT ( 'NONE',  ( 172.6757217805928235, 277.3386798770395103, 16.69748815113853979 ) ) ;
#12717=ORIENTED_EDGE ( 'NONE', *, *, #29961, .T. ) ;
#12719=CARTESIAN_POINT ( 'NONE',  ( 163.9665353451645160, 260.5250585567103485, -16.17572278673254615 ) ) ;
#12725=CARTESIAN_POINT ( 'NONE',  ( 206.1932826529868805, 273.5097535960530877, 11.72208607728249241 ) ) ;
#12726=CYLINDRICAL_SURFACE ( 'NONE', #42803, 17.82106496071139645 ) ;
#12728=CARTESIAN_POINT ( 'NONE',  ( 164.4817765375028102, 245.7562014482918755, -6.334578229142199035 ) ) ;
#12730=EDGE_CURVE ( 'NONE', #36195, #99407, #47168, .T. ) ;
#12731=CARTESIAN_POINT ( 'NONE',  ( 125.6948669907937415, 249.5024278399160949, 9.188101187500095079 ) ) ;
#12738=CARTESIAN_POINT ( 'NONE',  ( 190.2204363742943656, 300.4646209966566062, -1.328626404316530739E-11 ) ) ;
#12742=CARTESIAN_POINT ( 'NONE',  ( 184.7266634662323952, 277.2745127826178759, -16.72297256227146534 ) ) ;
#12744=CARTESIAN_POINT ( 'NONE',  ( 206.0013442967545245, 273.8422005809691768, -10.96701481760672792 ) ) ;
#12746=B_SPLINE_CURVE_WITH_KNOTS ( 'NONE', 3,
 ( #97761, #28331, #82091, #83578, #21736, #97275, #14139, #27842, #98257, #83077, #6544, #90183 ),
 .UNSPECIFIED., .F., .F.,
 ( 4, 2, 2, 2, 2, 4 ),
 ( 0.001227138907740844311, 0.001452414644335943937, 0.001677690380931043564, 0.002128241854121296159, 0.002578793327311548322, 0.003029344800501800918 ),
 .UNSPECIFIED. ) ;
#12747=CARTESIAN_POINT ( 'NONE',  ( 190.7569505155522904, 300.2462651405980978, -5.670926626284815697 ) ) ;
#12750=CARTESIAN_POINT ( 'NONE',  ( 157.1965120183049578, 258.3746497421212780, -18.06591467563559306 ) ) ;
#12751=CARTESIAN_POINT ( 'NONE',  ( 195.9623275608007589, 270.6700471875816447, 12.00925747662462406 ) ) ;
#12753=CARTESIAN_POINT ( 'NONE',  ( 177.4877928417686803, 293.5951873982637608, -2.837372163671336267 ) ) ;
#12754=CARTESIAN_POINT ( 'NONE',  ( 71.81202244518919997, 222.2677522451419065, -5.000000000000047962 ) ) ;
#12756=CARTESIAN_POINT ( 'NONE',  ( 162.2482745412403631, 281.2414901047574745, 10.34674202811327248 ) ) ;
#12758=CARTESIAN_POINT ( 'NONE',  ( 139.8671854259164036, 244.8927522451418497, 10.00000000000009592 ) ) ;
#12759=CARTESIAN_POINT ( 'NONE',  ( 172.2535748400142097, 283.6734274018703559, -12.51371615245540880 ) ) ;
#12761=CARTESIAN_POINT ( 'NONE',  ( 157.6673516573649181, 257.5591315650518141, 16.79781451397666103 ) ) ;
#12762=CARTESIAN_POINT ( 'NONE',  ( 198.8157103782086210, 286.2880836124806478, -18.60729372713428020 ) ) ;
#12763=CARTESIAN_POINT ( 'NONE',  ( 5.344833028331274605, 164.7048013555410080, 4.594050593750051981 ) ) ;
#12764=CARTESIAN_POINT ( 'NONE',  ( 50.35065686154756293, 206.0024278399160949, 9.188101187500095079 ) ) ;
#12768=CARTESIAN_POINT ( 'NONE',  ( 157.1539462478114615, 258.4483758192793061, -17.96006278656275867 ) ) ;
#12769=CARTESIAN_POINT ( 'NONE',  ( 192.6020092295239010, 292.3528725471387020, -14.35004337652128470 ) ) ;
#12770=CARTESIAN_POINT ( 'NONE',  ( 147.7395812515338491, 275.4447818272566337, 3.760927250875937489 ) ) ;
#12771=CARTESIAN_POINT ( 'NONE',  ( 167.5542314069692793, 256.6061373407214319, 13.74842419216645695 ) ) ;
#12772=CARTESIAN_POINT ( 'NONE',  ( 64.01779381112923772, 217.7677522451419065, -5.000000000000047962 ) ) ;
#12773=CARTESIAN_POINT ( 'NONE',  ( 181.4027557144102900, 255.2212836150004023, 2.052969345246689503 ) ) ;
#12774=CARTESIAN_POINT ( 'NONE',  ( 150.4255120825602887, 270.1023656488765710, 15.17857413906334507 ) ) ;
#12775=CARTESIAN_POINT ( 'NONE',  ( 179.2832723880610786, 294.0843149181845320, 1.044996869123359318 ) ) ;
#12776=CARTESIAN_POINT ( 'NONE',  ( 58.19016453504443831, 197.7365022471902307, 10.00000000000009592 ) ) ;
#12777=CARTESIAN_POINT ( 'NONE',  ( 184.1284384789660749, 293.1887098790314212, 9.479892220414697590 ) ) ;
#12778=CARTESIAN_POINT ( 'NONE',  ( 163.4260108471723640, 247.5848412648317662, 10.45113099391573108 ) ) ;
#12779=CIRCLE ( 'NONE', #82393, 10.00000000000011369 ) ;
#12780=CARTESIAN_POINT ( 'NONE',  ( 18.36166996137734841, 193.6589784336661637, -6.496448406907675876E-16 ) ) ;
#12781=CARTESIAN_POINT ( 'NONE',  ( 167.9915683551312782, 286.1490694072173824, 4.089171754536926606 ) ) ;
#12782=CARTESIAN_POINT ( 'NONE',  ( 153.1314981037513121, 265.4154603756023789, 17.73969815997475408 ) ) ;
#12784=CARTESIAN_POINT ( 'NONE',  ( 139.3620039403754731, 251.2677522451418497, 10.00000000000009592 ) ) ;
#12787=CARTESIAN_POINT ( 'NONE',  ( 183.0432481310025992, 278.8237664249871273, 16.78443556766483624 ) ) ;
#12788=CARTESIAN_POINT ( 'NONE',  ( 175.0686550866780635, 279.4321407445321483, 16.32612376929353815 ) ) ;
#12789=DIRECTION ( 'NONE',  ( 0.4999999999999992784, -0.8660254037844390407, 0.000000000000000000 ) ) ;
#12790=CARTESIAN_POINT ( 'NONE',  ( 177.7668908026954284, 261.5253217029109010, -12.97050892711601300 ) ) ;
#12795=CARTESIAN_POINT ( 'NONE',  ( 175.8027662909930484, 284.8719843250962072, 14.11304877541382119 ) ) ;
#12796=CARTESIAN_POINT ( 'NONE',  ( 153.2146083375174328, 277.7743879745896720, -5.000743142145255504 ) ) ;
#12797=ORIENTED_EDGE ( 'NONE', *, *, #61148, .T. ) ;
#12798=CARTESIAN_POINT ( 'NONE',  ( 181.9257749470477563, 289.8349502344528901, 12.95467248944978422 ) ) ;
#12800=CARTESIAN_POINT ( 'NONE',  ( 159.9647205790309101, 253.5799718689968927, -16.48298384325780219 ) ) ;
#12803=CARTESIAN_POINT ( 'NONE',  ( 152.7043854946215049, 268.1552411151685078, 15.94764448997051964 ) ) ;
#12805=B_SPLINE_CURVE_WITH_KNOTS ( 'NONE', 3,
 ( #84436, #68186, #7905, #45387 ),
 .UNSPECIFIED., .F., .F.,
 ( 4, 4 ),
 ( 0.03473529416486713373, 0.04353459421610011981 ),
 .UNSPECIFIED. ) ;
#12806=CARTESIAN_POINT ( 'NONE',  ( 200.0411626275569574, 270.6720010161316736, -11.59284015024147152 ) ) ;
#12808=CARTESIAN_POINT ( 'NONE',  ( 155.4661767250933622, 261.3716783840932294, -17.10192542004562810 ) ) ;
#12810=VECTOR ( 'NONE', #41667, 1000.000000000000000 ) ;
#12811=ORIENTED_EDGE ( 'NONE', *, *, #35527, .F. ) ;
#12812=CARTESIAN_POINT ( 'NONE',  ( 159.3076723029256812, 279.4120732660696262, -9.573196759042872372 ) ) ;
#12813=CARTESIAN_POINT ( 'NONE',  ( 164.3961040135806968, 245.9045906125373904, 7.095190383188031191 ) ) ;
#12814=CARTESIAN_POINT ( 'NONE',  ( 192.6773196027083372, 296.9200883123592689, 11.15745042875121484 ) ) ;
#12818=CARTESIAN_POINT ( 'NONE',  ( 175.2632563419276721, 262.6760348153215432, 14.36099408182738912 ) ) ;
#12824=CARTESIAN_POINT ( 'NONE',  ( 205.7867067512454184, 274.2139637150027056, 10.62737868262404106 ) ) ;
#12828=CARTESIAN_POINT ( 'NONE',  ( 177.7722849220445482, 279.4784791579494936, -16.51336255298548394 ) ) ;
#12832=ORIENTED_EDGE ( 'NONE', *, *, #85999, .T. ) ;
#12833=CARTESIAN_POINT ( 'NONE',  ( 157.5260732920700661, 268.8916645685611115, 15.61200622228795254 ) ) ;
#12836=CARTESIAN_POINT ( 'NONE',  ( 156.5505791614179145, 266.8975169099628602, -16.19599294687877489 ) ) ;
#12837=CARTESIAN_POINT ( 'NONE',  ( 198.2505066714982149, 285.2670451491296149, 0.000000000000000000 ) ) ;
#12838=CARTESIAN_POINT ( 'NONE',  ( 190.1693911629507738, 301.2639477917662703, -5.112716700269980485 ) ) ;
#12840=CARTESIAN_POINT ( 'NONE',  ( 190.0445576990143195, 301.4801656937889902, 4.140328216824785912 ) ) ;
#12841=CARTESIAN_POINT ( 'NONE',  ( 192.7259387352017939, 296.8358775046606297, 11.24705370801146209 ) ) ;
#12842=CARTESIAN_POINT ( 'NONE',  ( 39.06543686813810012, 183.3615022471902023, 5.000000000000051514 ) ) ;
#12843=CARTESIAN_POINT ( 'NONE',  ( 159.0312449811773376, 255.1967990321049058, -16.31084382475164674 ) ) ;
#12844=EDGE_LOOP ( 'NONE', ( #81144, #19702, #63111, #85220 ) ) ;
#12845=EDGE_CURVE ( 'NONE', #62907, #83615, #53205, .T. ) ;
#12847=CARTESIAN_POINT ( 'NONE',  ( 206.4229368915142686, 273.1119807867502800, 10.31819530520674810 ) ) ;
#12848=CARTESIAN_POINT ( 'NONE',  ( 149.6191398986701415, 271.4990432411842676, -11.66821883946526839 ) ) ;
#12849=CARTESIAN_POINT ( 'NONE',  ( 164.3493441216711517, 245.9855811210807417, 1.722120810491653664 ) ) ;
#12850=CARTESIAN_POINT ( 'NONE',  ( 168.7107245727987390, 286.5688979659043980, 4.076349780630120101 ) ) ;
#12854=ADVANCED_FACE ( 'NONE', ( #12129 ), #95781, .T. ) ;
#12857=CARTESIAN_POINT ( 'NONE',  ( 160.0264454347010883, 253.4730612828859364, -14.80461457038359541 ) ) ;
#12858=CARTESIAN_POINT ( 'NONE',  ( 148.1504907822988457, 274.0428181292306249, -10.36053812211976144 ) ) ;
#12860=CARTESIAN_POINT ( 'NONE',  ( 170.6724042201842622, 255.4561172912020481, -12.81820913873951717 ) ) ;
#12862=CARTESIAN_POINT ( 'NONE',  ( 200.8147387322574957, 282.8256649374973790, -18.02438097732020239 ) ) ;
#12863=CARTESIAN_POINT ( 'NONE',  ( 164.5867587387928950, 245.5743669417666126, -3.022048486790635202 ) ) ;
#12864=CARTESIAN_POINT ( 'NONE',  ( 27.64472685218281711, 196.7677522451419350, -5.000000000000047962 ) ) ;
#12865=CARTESIAN_POINT ( 'NONE',  ( 125.2893514524760548, 233.9548013555409796, -4.594050593750042211 ) ) ;
#12866=CARTESIAN_POINT ( 'NONE',  ( 180.9267084132501964, 294.1738383600696238, -2.651135849888626606 ) ) ;
#12868=CARTESIAN_POINT ( 'NONE',  ( 162.6810519034260665, 249.2653427326025906, -10.49599293899969688 ) ) ;
#12869=CARTESIAN_POINT ( 'NONE',  ( 157.2333142128019858, 258.3109064714224132, 16.87956768598436597 ) ) ;
#12870=CARTESIAN_POINT ( 'NONE',  ( 207.5987293781265919, 271.0754484607800237, 1.965225377555418484 ) ) ;
#12871=CARTESIAN_POINT ( 'NONE',  ( 42.77328167419873495, 189.3768266524160140, 9.188101187500098632 ) ) ;
#12875=ORIENTED_EDGE ( 'NONE', *, *, #42459, .T. ) ;
#12878=CARTESIAN_POINT ( 'NONE',  ( 30.69616969366791537, 176.9824982072973967, 3.021315404115420679E-15 ) ) ;
#12879=CARTESIAN_POINT ( 'NONE',  ( 146.9709166616330549, 276.0859004375172390, 3.755270622130282732 ) ) ;
#12881=EDGE_CURVE ( 'NONE', #94756, #72513, #64164, .T. ) ;
#12882=CARTESIAN_POINT ( 'NONE',  ( 207.7666684749232786, 270.7845694125510931, -6.630926507062123498 ) ) ;
#12883=CARTESIAN_POINT ( 'NONE',  ( 168.0703335804080609, 251.8096463010647312, 10.49794630816577445 ) ) ;
#12884=CARTESIAN_POINT ( 'NONE',  ( 88.69951781898578247, 222.0177522451418781, -10.00000000000009592 ) ) ;
#12885=B_SPLINE_SURFACE_WITH_KNOTS ( 'NONE', 3, 1, ( 
 ( #43531, #3786 ),
 ( #11891, #58456 ),
 ( #42749, #26086 ),
 ( #56960, #4786 ),
 ( #81811, #87461 ),
 ( #80320, #80836 ),
 ( #87947, #72712 ),
 ( #17993, #34668 ),
 ( #88954, #41257 ),
 ( #49376, #41766 ),
 ( #48887, #89429 ),
 ( #27592, #10388 ),
 ( #88440, #11404 ),
 ( #19983, #72199 ),
 ( #34181, #2805 ),
 ( #65570, #33692 ),
 ( #64586, #96517 ),
 ( #73683, #50860 ),
 ( #4267, #18491 ),
 ( #10890, #95538 ),
 ( #12387, #3302 ),
 ( #19000, #65075 ),
 ( #96024, #26587 ),
 ( #43252, #74197 ),
 ( #57460, #27086 ),
 ( #35165, #66075 ),
 ( #49875, #42258 ),
 ( #73192, #57969 ),
 ( #19509, #50366 ),
 ( #81320, #97022 ),
 ( #59944, #28557 ),
 ( #37156, #13380 ),
 ( #30051, #14364 ),
 ( #84301, #14849 ) ),
 .UNSPECIFIED., .T., .F., .F.,
 ( 4, 2, 2, 2, 2, 2, 2, 2, 2, 2, 2, 2, 2, 2, 2, 2, 4 ),
 ( 2, 2 ),
 ( 0.000000000000000000, 0.06250000000000000000, 0.1250000000000000000, 0.1875000000000000000, 0.2500000000000000000, 0.3125000000000000000, 0.3750000000000000000, 0.4375000000000000000, 0.5000000000000000000, 0.5625000000000000000, 0.6250000000000000000, 0.6875000000000000000, 0.7500000000000000000, 0.8125000000000000000, 0.8750000000000000000, 0.9375000000000000000, 1.000000000000000000 ),
 ( 0.000000000000000000, 1.000000000000000000 ),
 .UNSPECIFIED. ) ;
#12887=EDGE_CURVE ( 'NONE', #63662, #58917, #67928, .T. ) ;
#12888=CARTESIAN_POINT ( 'NONE',  ( 195.2652153521346463, 266.6463243828191025, -7.753748465262478184 ) ) ;
#12889=CARTESIAN_POINT ( 'NONE',  ( 155.5460960050927213, 279.7549409233841402, -1.594755899433322854 ) ) ;
#12890=CARTESIAN_POINT ( 'NONE',  ( 162.6425574510925003, 248.9418223522047526, -10.70838742014210077 ) ) ;
#12891=CARTESIAN_POINT ( 'NONE',  ( 11.37951369124782453, 183.5024278399160949, 9.188101187500095079 ) ) ;
#12894=FACE_OUTER_BOUND ( 'NONE', #80263, .T. ) ;
#12897=CARTESIAN_POINT ( 'NONE',  ( 57.63111678181675757, 194.8923013555409796, 4.594050593750050204 ) ) ;
#12899=CARTESIAN_POINT ( 'NONE',  ( 164.3010377730689981, 246.0692501711882869, 7.247566249275159578 ) ) ;
#12901=CARTESIAN_POINT ( 'NONE',  ( 207.6508796976096107, 270.9851214578045528, 6.713685698622268383 ) ) ;
#12903=CARTESIAN_POINT ( 'NONE',  ( 2.692369909191673294, 162.3615022471902023, 5.000000000000051514 ) ) ;
#12905=CARTESIAN_POINT ( 'NONE',  ( 145.9657079678295020, 245.8923013555409511, 4.594050593750050204 ) ) ;
#12907=CARTESIAN_POINT ( 'NONE',  ( 206.7843909389352177, 272.4859240120160280, -7.614953610527129158 ) ) ;
#12911=CARTESIAN_POINT ( 'NONE',  ( 189.4521523383693875, 289.8044986729786388, 14.56744347494121961 ) ) ;
#12912=CARTESIAN_POINT ( 'NONE',  ( 190.5730759679604773, 300.5647451992460333, -7.149221719703987787 ) ) ;
#12914=CARTESIAN_POINT ( 'NONE',  ( 191.4941427383744781, 298.9694107557253346, 8.584406880462095657 ) ) ;
#12915=CARTESIAN_POINT ( 'NONE',  ( 208.2813134324037492, 269.8931781983357041, -0.4511785827856357178 ) ) ;
#12916=CARTESIAN_POINT ( 'NONE',  ( 151.3881894390805485, 268.8414657422088681, -14.32066872820409742 ) ) ;
#12918=CARTESIAN_POINT ( 'NONE',  ( 197.2082756938223440, 273.4841093250385597, -13.85768748786135340 ) ) ;
#12919=ORIENTED_EDGE ( 'NONE', *, *, #34421, .T. ) ;
#12921=CARTESIAN_POINT ( 'NONE',  ( 169.2808828497843763, 282.7368009450043473, -10.94465088845561773 ) ) ;
#12922=EDGE_CURVE ( 'NONE', #14901, #59762, #44752, .T. ) ;
#12925=CARTESIAN_POINT ( 'NONE',  ( 185.5894612333727309, 296.5431996284972911, 4.661688250043606985 ) ) ;
#12926=EDGE_CURVE ( 'NONE', #17056, #8797, #31482, .T. ) ;
#12928=CARTESIAN_POINT ( 'NONE',  ( 150.4933457285363261, 277.6093123845979562, -0.0001770771435699358459 ) ) ;
#12932=CARTESIAN_POINT ( 'NONE',  ( 192.0604745424677446, 287.4852189256589554, -16.59597026331354286 ) ) ;
#12933=EDGE_LOOP ( 'NONE', ( #3732, #59001, #80770, #93215 ) ) ;
#12937=CARTESIAN_POINT ( 'NONE',  ( 159.7314908411816248, 264.1435442130865567, -17.48313506953057939 ) ) ;
#12938=ORIENTED_EDGE ( 'NONE', *, *, #78890, .F. ) ;
#12940=CARTESIAN_POINT ( 'NONE',  ( 147.1731211915891322, 275.7356719181125868, 0.5879280619134324981 ) ) ;
#12941=CARTESIAN_POINT ( 'NONE',  ( 185.7591078734260464, 291.2087897148937827, 12.17200245411944692 ) ) ;
#12942=CARTESIAN_POINT ( 'NONE',  ( 204.1953342137782954, 276.9703018036655067, 13.84727111424505885 ) ) ;
#12945=CARTESIAN_POINT ( 'NONE',  ( 81.04025856027610075, 229.8464784336661637, 1.353441290958777525E-15 ) ) ;
#12946=CARTESIAN_POINT ( 'NONE',  ( 203.2362765626855889, 278.6314383827457846, 14.95873044600159929 ) ) ;
#12947=CARTESIAN_POINT ( 'NONE',  ( 181.2982806733463974, 271.4113319947247760, -17.41859542398102434 ) ) ;
#12948=CARTESIAN_POINT ( 'NONE',  ( 181.8697498269454513, 257.4598785196697008, -6.014196373383785321 ) ) ;
#12949=ORIENTED_EDGE ( 'NONE', *, *, #86723, .F. ) ;
#12950=ORIENTED_EDGE ( 'NONE', *, *, #46025, .T. ) ;
#12951=CARTESIAN_POINT ( 'NONE',  ( 196.1252721995043942, 284.4712197134549001, -17.81715240067734030 ) ) ;
#12957=CARTESIAN_POINT ( 'NONE',  ( 154.8786460229866577, 262.3893114111486398, -18.06164891362396929 ) ) ;
#12960=ADVANCED_FACE ( 'NONE', ( #51618 ), #82573, .T. ) ;
#12961=CARTESIAN_POINT ( 'NONE',  ( 148.7588072053147243, 273.7711778218048835, -8.803803025135483296 ) ) ;
#12965=CARTESIAN_POINT ( 'NONE',  ( 156.8158635136204850, 259.0339522920597233, -18.23857867748462880 ) ) ;
#12966=ORIENTED_EDGE ( 'NONE', *, *, #67208, .F. ) ;
#12972=CARTESIAN_POINT ( 'NONE',  ( 200.1387068151675237, 270.2636360650371330, 9.266071134921585184 ) ) ;
#12973=ORIENTED_EDGE ( 'NONE', *, *, #98728, .F. ) ;
#12975=CARTESIAN_POINT ( 'NONE',  ( 181.4433080673849474, 255.1351033649908402, 0.7872376121522187686 ) ) ;
#12976=CARTESIAN_POINT ( 'NONE',  ( 188.9516232634142909, 259.5449388965931234, 2.625812016075142807 ) ) ;
#12977=CARTESIAN_POINT ( 'NONE',  ( 160.8219329449452744, 281.1493571213889027, -6.602944771620161468 ) ) ;
#12978=CARTESIAN_POINT ( 'NONE',  ( 164.6573736076317402, 246.3298132620209060, -1.876867566021173328 ) ) ;
#12979=CARTESIAN_POINT ( 'NONE',  ( 157.6552178212553486, 258.0004517741330687, 16.70547076031876088 ) ) ;
#12980=B_SPLINE_CURVE_WITH_KNOTS ( 'NONE', 3,
 ( #53368, #14865, #60960, #23453 ),
 .UNSPECIFIED., .F., .F.,
 ( 4, 4 ),
 ( 0.0002127203767480665916, 0.005436920270846633783 ),
 .UNSPECIFIED. ) ;
#12981=CARTESIAN_POINT ( 'NONE',  ( 169.5829390051931966, 248.1378239353514914, -0.09087230163007473105 ) ) ;
#12984=CARTESIAN_POINT ( 'NONE',  ( 181.7205532481384012, 270.6930945944329778, -16.08030108815028214 ) ) ;
#12986=ORIENTED_EDGE ( 'NONE', *, *, #32416, .F. ) ;
#12987=CARTESIAN_POINT ( 'NONE',  ( 160.7513685639857783, 275.7766557047398805, 12.80917292314146572 ) ) ;
#12989=CARTESIAN_POINT ( 'NONE',  ( 204.1357312349132087, 277.0735371913424387, -14.51687998123883716 ) ) ;
#12992=CARTESIAN_POINT ( 'NONE',  ( 160.9438941661644549, 272.8970580874148482, 15.77033046387437842 ) ) ;
#12993=CARTESIAN_POINT ( 'NONE',  ( -18.01139699756907930, 172.6589784336661637, -6.496448406907675876E-16 ) ) ;
#12995=CARTESIAN_POINT ( 'NONE',  ( 165.0735250206753619, 246.7312630101393722, 5.989302113854410692 ) ) ;
#12997=ORIENTED_EDGE ( 'NONE', *, *, #7738, .F. ) ;
#12999=CARTESIAN_POINT ( 'NONE',  ( 189.7410647174195901, 285.7743870009521743, -17.19896820403054605 ) ) ;
#13001=CARTESIAN_POINT ( 'NONE',  ( 171.7934946240355600, 289.9441787457215582, 2.720480149874153764 ) ) ;
#13002=CARTESIAN_POINT ( 'NONE',  ( 153.3616370783189211, 265.0168479788495688, 17.48287904751960653 ) ) ;
#13004=CARTESIAN_POINT ( 'NONE',  ( 189.6666044902458168, 284.7049877867155487, 17.41007887138588117 ) ) ;
#13005=CARTESIAN_POINT ( 'NONE',  ( 17.60459192459599365, 168.7202760586660020, -5.415160957724236172E-17 ) ) ;
#13006=CARTESIAN_POINT ( 'NONE',  ( 99.93095832397169431, 222.3768266524160140, 9.188101187500098632 ) ) ;
#13007=CARTESIAN_POINT ( 'NONE',  ( 48.42933654300943402, 188.7677522451417929, -5.000000000000041744 ) ) ;
#13008=CARTESIAN_POINT ( 'NONE',  ( 186.7650389526093022, 295.9085115873210157, -7.616436736632654636 ) ) ;
#13011=CARTESIAN_POINT ( 'NONE',  ( 177.9870452976290380, 283.3051803591353064, -14.47979671836508508 ) ) ;
#13012=CARTESIAN_POINT ( 'NONE',  ( 190.7734523378904896, 299.7926839710546574, -4.885404362283661150 ) ) ;
#13014=CARTESIAN_POINT ( 'NONE',  ( 181.1312229881957592, 273.4383946350568522, 16.62563511410547079 ) ) ;
#13015=CARTESIAN_POINT ( 'NONE',  ( 148.1974503712686158, 273.9614817352322120, -7.884397846570731616 ) ) ;
#13017=CARTESIAN_POINT ( 'NONE',  ( 196.2299774253775411, 266.0274705162634632, 8.373944587636422909 ) ) ;
#13018=CARTESIAN_POINT ( 'NONE',  ( 53.86003751612224733, 195.2365022471902023, -10.00000000000009237 ) ) ;
#13019=CARTESIAN_POINT ( 'NONE',  ( 162.4413493851164958, 251.9320596174019045, -12.94637656145141591 ) ) ;
#13022=CARTESIAN_POINT ( 'NONE',  ( 172.9387157878505263, 262.8721711101524079, -15.86194836379059225 ) ) ;
#13023=CARTESIAN_POINT ( 'NONE',  ( 81.44681538588882574, 208.6423013555409796, -4.594050593750043987 ) ) ;
#13025=CARTESIAN_POINT ( 'NONE',  ( 190.8604783348975502, 300.0669496974951471, 7.597731640149610222 ) ) ;
#13027=CARTESIAN_POINT ( 'NONE',  ( 196.1241105319816143, 290.9500712997905794, 15.97146679939154268 ) ) ;
#13029=CARTESIAN_POINT ( 'NONE',  ( 149.4009768994915248, 271.8769126400935079, 11.50055073237692049 ) ) ;
#13030=CARTESIAN_POINT ( 'NONE',  ( 199.0756812798354645, 285.8378008023734083, -18.45377816087746936 ) ) ;
#13033=CARTESIAN_POINT ( 'NONE',  ( 146.9370072200009645, 276.1446333132804511, -3.799807221059707363 ) ) ;
#13038=CARTESIAN_POINT ( 'NONE',  ( 192.5076277540105423, 297.2140032159341558, -13.10094381206144298 ) ) ;
#13043=CARTESIAN_POINT ( 'NONE',  ( 198.4334039703542771, 286.9502577349437615, 18.47706603442866680 ) ) ;
#13045=ADVANCED_FACE ( 'NONE', ( #85065 ), #21369, .T. ) ;
#13047=CARTESIAN_POINT ( 'NONE',  ( 138.2253456014562403, 260.6115022471903444, -5.000000000000047962 ) ) ;
#13049=ORIENTED_EDGE ( 'NONE', *, *, #27670, .T. ) ;
#13050=CARTESIAN_POINT ( 'NONE',  ( 91.29759403033908427, 223.5177522451418781, -10.00000000000009592 ) ) ;
#13052=CARTESIAN_POINT ( 'NONE',  ( -22.42236680055709641, 157.8615022471902591, 0.000000000000000000 ) ) ;
#13054=EDGE_CURVE ( 'NONE', #22165, #99984, #72511, .T. ) ;
#13055=ORIENTED_EDGE ( 'NONE', *, *, #48308, .T. ) ;
#13056=CYLINDRICAL_SURFACE ( 'NONE', #17627, 10.00000000000010658 ) ;
#13057=ORIENTED_EDGE ( 'NONE', *, *, #52830, .F. ) ;
#13059=CARTESIAN_POINT ( 'NONE',  ( 205.9504341145390924, 273.9303796031887259, 10.73680394385792525 ) ) ;
#13060=CARTESIAN_POINT ( 'NONE',  ( 157.5065816067722722, 258.4198049196606917, -16.86844230480359741 ) ) ;
#13062=CARTESIAN_POINT ( 'NONE',  ( 201.4066285247549786, 281.8004817444100354, -17.79749223817309201 ) ) ;
#13063=CARTESIAN_POINT ( 'NONE',  ( -22.42236680055709641, 157.8615022471902591, 0.000000000000000000 ) ) ;
#13066=CARTESIAN_POINT ( 'NONE',  ( 164.4948408606173302, 274.6928532213739800, 14.67008970210409657 ) ) ;
#13067=EDGE_LOOP ( 'NONE', ( #40475, #39675, #71504, #96208, #62221, #13206, #66218 ) ) ;
#13069=CARTESIAN_POINT ( 'NONE',  ( 182.3632850533476812, 274.9408504765579551, 17.79507043724071735 ) ) ;
#13071=CARTESIAN_POINT ( 'NONE',  ( 194.1972774922283236, 294.2874440223457100, -15.09915398317898649 ) ) ;
#13076=CARTESIAN_POINT ( 'NONE',  ( 170.9887030610543661, 287.7172861656689520, -4.592964840281122285 ) ) ;
#13078=CARTESIAN_POINT ( 'NONE',  ( 181.8344274857143432, 257.0251970467633669, 5.042215935203653743 ) ) ;
#13079=CARTESIAN_POINT ( 'NONE',  ( 105.6144235841895664, 219.5327760586659451, 1.948934522072303157E-15 ) ) ;
#13082=CARTESIAN_POINT ( 'NONE',  ( 165.0450258753809294, 270.9524041312169516, 16.77974215795885016 ) ) ;
#13083=CARTESIAN_POINT ( 'NONE',  ( 179.5846872273510826, 291.4261084640538115, -10.07075702116988758 ) ) ;
#13084=ORIENTED_EDGE ( 'NONE', *, *, #36055, .F. ) ;
#13086=CARTESIAN_POINT ( 'NONE',  ( 185.4241002709785846, 298.2501943955377328, -2.445652077582521233 ) ) ;
#13088=CARTESIAN_POINT ( 'NONE',  ( 164.7199312521631214, 249.0629007997009126, 10.02713358784743747 ) ) ;
#13095=CARTESIAN_POINT ( 'NONE',  ( 207.6875671281972870, 270.9215769640275653, -2.211577121115235300 ) ) ;
#13096=ORIENTED_EDGE ( 'NONE', *, *, #60680, .F. ) ;
#13097=CARTESIAN_POINT ( 'NONE',  ( 191.9465615534260792, 264.5235098129936091, -7.852620813520595711 ) ) ;
#13098=CARTESIAN_POINT ( 'NONE',  ( 24.36335893204212155, 173.3262482093457777, 3.021315404115420679E-15 ) ) ;
#13101=CARTESIAN_POINT ( 'NONE',  ( 144.5855667544892924, 242.0327760586659451, 1.948934522072303157E-15 ) ) ;
#13105=CARTESIAN_POINT ( 'NONE',  ( 147.5498377207569263, 275.0831797495432056, 4.097967709737811326 ) ) ;
#13106=DIRECTION ( 'NONE',  ( -0.8660254037844387076, -0.4999999999999998890, -0.000000000000000000 ) ) ;
#13107=CARTESIAN_POINT ( 'NONE',  ( 190.1998581979997311, 263.5875986082893405, -9.717754213320489498 ) ) ;
#13108=CARTESIAN_POINT ( 'NONE',  ( 173.2404090740162133, 251.6421966675173678, -0.2950645122926903730 ) ) ;
#13109=CARTESIAN_POINT ( 'NONE',  ( 178.3382078955913528, 285.3547819717112475, 13.04039342192868745 ) ) ;
#13111=EDGE_CURVE ( 'NONE', #59762, #72864, #99157, .T. ) ;
#13112=CARTESIAN_POINT ( 'NONE',  ( 199.0831254908205210, 281.9212699178648904, -16.61011480125563011 ) ) ;
#13116=CARTESIAN_POINT ( 'NONE',  ( 52.13666070897046012, 213.1589784336661637, -6.496448406907675876E-16 ) ) ;
#13117=CARTESIAN_POINT ( 'NONE',  ( 206.1062572280473546, 273.6604860535989587, -9.773577984388410300 ) ) ;
#13119=CARTESIAN_POINT ( 'NONE',  ( 162.6396274730868186, 248.9468972229755082, -10.26162218571527518 ) ) ;
#13120=EDGE_CURVE ( 'NONE', #7544, #63230, #13391, .T. ) ;
#13125=CARTESIAN_POINT ( 'NONE',  ( 172.9897703034535539, 283.7959595487852766, 13.73707729917544285 ) ) ;
#13130=CARTESIAN_POINT ( 'NONE',  ( 19.71535529843806245, 176.0643266524160424, 9.188101187500095079 ) ) ;
#13131=CARTESIAN_POINT ( 'NONE',  ( 45.99364009841357159, 197.3615022471902591, -10.00000000000009592 ) ) ;
#13132=ORIENTED_EDGE ( 'NONE', *, *, #7938, .T. ) ;
#13133=CARTESIAN_POINT ( 'NONE',  ( 196.4994169513186364, 290.3000215130921902, 16.82935102260526961 ) ) ;
#13134=CARTESIAN_POINT ( 'NONE',  ( 202.1030944152313111, 278.9078238741668656, 15.49021988960157792 ) ) ;
#13136=CARTESIAN_POINT ( 'NONE',  ( 163.8455942243524248, 246.8581015375447691, -7.178103170949780676 ) ) ;
#13138=CARTESIAN_POINT ( 'NONE',  ( 44.34243207491051209, 208.6589784336661921, -6.496448406907676862E-16 ) ) ;
#13139=CARTESIAN_POINT ( 'NONE',  ( 161.7101619467568980, 250.5567787384628389, 13.05644392949610655 ) ) ;
#13140=CARTESIAN_POINT ( 'NONE',  ( 171.0964841634227298, 287.0058847005474263, 7.064598226519137825 ) ) ;
#13141=CARTESIAN_POINT ( 'NONE',  ( 147.5848197185516142, 275.0225891520124151, 4.420251097676741736 ) ) ;
#13143=CARTESIAN_POINT ( 'NONE',  ( 203.2428933715266623, 269.5665350485680278, -7.504532614354034514 ) ) ;
#13145=CARTESIAN_POINT ( 'NONE',  ( 177.5660330061924128, 275.6111645067952622, 16.43781890528649114 ) ) ;
#13149=CARTESIAN_POINT ( 'NONE',  ( 163.6657122372590720, 255.3124181700179918, -14.98584762205334542 ) ) ;
#13151=CARTESIAN_POINT ( 'NONE',  ( 204.6823371430232896, 272.9704135290961062, -9.754921121218281144 ) ) ;
#13153=CARTESIAN_POINT ( 'NONE',  ( 106.6154183633243377, 222.3615022471902023, 5.000000000000051514 ) ) ;
#13154=CARTESIAN_POINT ( 'NONE',  ( 200.5438717407500917, 283.2948203288816558, 18.39667691545567152 ) ) ;
#13157=CARTESIAN_POINT ( 'NONE',  ( 59.38997056143013964, 205.0958772461660828, -9.188101187500095079 ) ) ;
#13160=DIRECTION ( 'NONE',  ( -0.8660254037844387076, -0.4999999999999998890, -0.000000000000000000 ) ) ;
#13169=CARTESIAN_POINT ( 'NONE',  ( 185.9748738598958369, 262.9711142029209441, 11.36824966179820251 ) ) ;
#13170=CARTESIAN_POINT ( 'NONE',  ( 148.9831146496684084, 272.6006712873522133, -12.63706091291043343 ) ) ;
#13171=CARTESIAN_POINT ( 'NONE',  ( 157.2470923712064348, 258.2870420010311250, 16.90933983342926439 ) ) ;
#13177=EDGE_LOOP ( 'NONE', ( #40247, #63883, #63594, #53875, #2482 ) ) ;
#13178=CARTESIAN_POINT ( 'NONE',  ( 182.3585487608926883, 284.1109264421751277, 14.96762621272966243 ) ) ;
#13179=CARTESIAN_POINT ( 'NONE',  ( 151.4384131719918685, 268.3479694989391078, 14.98299707687648841 ) ) ;
#13182=EDGE_LOOP ( 'NONE', ( #62104, #14432, #9856, #38700 ) ) ;
#13183=CARTESIAN_POINT ( 'NONE',  ( 159.5335386611425861, 282.9547953765525108, -3.344663661812444566 ) ) ;
#13185=CARTESIAN_POINT ( 'NONE',  ( 149.1939152435731728, 272.2355539484436235, -11.44223522189843933 ) ) ;
#13187=CARTESIAN_POINT ( 'NONE',  ( 159.2111180226792726, 254.8852497853115722, 16.01057445397460910 ) ) ;
#13189=CARTESIAN_POINT ( 'NONE',  ( 161.0784938446909393, 262.9894285514246235, -17.68042406554819834 ) ) ;
#13190=CARTESIAN_POINT ( 'NONE',  ( 126.3172359758225554, 252.9244531367911293, -4.594050593750046652 ) ) ;
#13191=CARTESIAN_POINT ( 'NONE',  ( 123.0902549634681407, 230.3262482093458061, 3.021315404115420679E-15 ) ) ;
#13192=VERTEX_POINT ( 'NONE', #3287 ) ;
#13193=CARTESIAN_POINT ( 'NONE',  ( 171.2823453295078195, 264.2191545540018183, 15.82956524986185798 ) ) ;
#13194=CARTESIAN_POINT ( 'NONE',  ( 66.61587002248256795, 219.2677522451419065, -5.000000000000047962 ) ) ;
#13195=VERTEX_POINT ( 'NONE', #33158 ) ;
#13196=CARTESIAN_POINT ( 'NONE',  ( 149.1653648461108617, 275.5304674000249179, 7.618651205328232479 ) ) ;
#13197=ORIENTED_EDGE ( 'NONE', *, *, #34417, .T. ) ;
#13201=CARTESIAN_POINT ( 'NONE',  ( 64.39641960523518094, 217.1744531367911293, 4.594050593750047540 ) ) ;
#13204=CARTESIAN_POINT ( 'NONE',  ( 193.9401685343300699, 294.7327698005063326, 14.01047396938887069 ) ) ;
#13205=CARTESIAN_POINT ( 'NONE',  ( 175.7203579514784053, 278.2834176361697587, 16.78628766804663996 ) ) ;
#13206=ORIENTED_EDGE ( 'NONE', *, *, #73082, .F. ) ;
#13209=B_SPLINE_CURVE_WITH_KNOTS ( 'NONE', 3,
 ( #81832, #88462, #41277, #42278 ),
 .UNSPECIFIED., .F., .F.,
 ( 4, 4 ),
 ( 0.008185576491779684646, 0.01406236705198208627 ),
 .UNSPECIFIED. ) ;
#13210=CARTESIAN_POINT ( 'NONE',  ( 201.3715986869907510, 281.8611552031986776, -17.89433714524984964 ) ) ;
#13211=CARTESIAN_POINT ( 'NONE',  ( 155.6328838216860220, 261.0829332228125850, -17.51014940606912518 ) ) ;
#13213=CARTESIAN_POINT ( 'NONE',  ( -15.29569941879559281, 168.6427522451419350, -10.00000000000009592 ) ) ;
#13215=CARTESIAN_POINT ( 'NONE',  ( 174.0844628251548727, 253.6050010518140994, -7.541462950351128569 ) ) ;
#13217=CARTESIAN_POINT ( 'NONE',  ( 164.4494343874829099, 245.8122196953522121, 2.922779519406129456 ) ) ;
#13219=CARTESIAN_POINT ( 'NONE',  ( 149.2923684163597784, 272.0650280510108701, -12.99082738998495756 ) ) ;
#13220=CARTESIAN_POINT ( 'NONE',  ( 154.8782533782051871, 264.3899914918594050, -17.45241046926759765 ) ) ;
#13222=CARTESIAN_POINT ( 'NONE',  ( 207.8060684685902686, 270.7163266217015689, 2.015725026008670540 ) ) ;
#13223=CARTESIAN_POINT ( 'NONE',  ( 128.9153121871758572, 254.4244531367911293, -4.594050593750046652 ) ) ;
#13224=VERTEX_POINT ( 'NONE', #17979 ) ;
#13225=CARTESIAN_POINT ( 'NONE',  ( -7.836314268245596182, 177.8297689869269220, -2.679491924311252493 ) ) ;
#13226=CARTESIAN_POINT ( 'NONE',  ( 182.2900984803647475, 257.5098244155703355, 6.713694854764257869 ) ) ;
#13231=CARTESIAN_POINT ( 'NONE',  ( -22.42236680055709641, 157.8615022471902591, 0.000000000000000000 ) ) ;
#13233=CARTESIAN_POINT ( 'NONE',  ( 183.4480379275034920, 257.0748008084844400, -5.332061893044733658 ) ) ;
#13234=ORIENTED_EDGE ( 'NONE', *, *, #54762, .T. ) ;
#13236=CARTESIAN_POINT ( 'NONE',  ( 182.1086373701226933, 275.6374269030367827, -16.43891936414332733 ) ) ;
#13237=CARTESIAN_POINT ( 'NONE',  ( 158.6496056213609904, 257.8578177934796258, 17.38082990300775776 ) ) ;
#13239=CARTESIAN_POINT ( 'NONE',  ( 202.1505501530674849, 267.6816150296156138, 0.8512892188848613095 ) ) ;
#13241=CARTESIAN_POINT ( 'NONE',  ( 146.8000281410530192, 276.3818880375922049, 4.652863924796177386 ) ) ;
#13242=CARTESIAN_POINT ( 'NONE',  ( 185.7490732957863031, 282.1293503020006028, 16.17923647030573875 ) ) ;
#13243=CARTESIAN_POINT ( 'NONE',  ( 204.9463377925012253, 275.6695254486514841, -14.15865086131798378 ) ) ;
#13244=CARTESIAN_POINT ( 'NONE',  ( 196.1276372599845388, 270.7547217853674510, 12.00612363897915991 ) ) ;
#13248=CARTESIAN_POINT ( 'NONE',  ( 190.0445576990143195, 301.4801656937889902, 4.140328216824785912 ) ) ;
#13249=CARTESIAN_POINT ( 'NONE',  ( 80.17564311316536418, 205.5494855054051584, -2.679491924311248496 ) ) ;
#13251=CARTESIAN_POINT ( 'NONE',  ( 198.4334039703542771, 286.9502577349437615, 18.47706603442866680 ) ) ;
#13252=CARTESIAN_POINT ( 'NONE',  ( 207.4071614940804125, 271.4072537690463491, 6.386333739406530263 ) ) ;
#13253=CARTESIAN_POINT ( 'NONE',  ( 144.5581563630821051, 244.2677522451417929, -5.000000000000041744 ) ) ;
#13254=CARTESIAN_POINT ( 'NONE',  ( 176.0042927459173541, 285.4150976940742339, -11.97940611282195711 ) ) ;
#13257=CARTESIAN_POINT ( 'NONE',  ( 198.5201458116119397, 286.8000164587433005, -18.30276554821096013 ) ) ;
#13258=CARTESIAN_POINT ( 'NONE',  ( 9.079046938504149011, 185.2369531367911293, -4.594050593750048428 ) ) ;
#13259=CARTESIAN_POINT ( 'NONE',  ( 178.8948291856917194, 273.8999092347531246, -17.56902132216663404 ) ) ;
#13262=CARTESIAN_POINT ( 'NONE',  ( 157.8159121039657293, 257.3018173235443555, -17.05074702406642118 ) ) ;
#13265=ADVANCED_FACE ( 'NONE', ( #96500 ), #63939, .F. ) ;
#13266=CARTESIAN_POINT ( 'NONE',  ( 169.4877538909896657, 257.6357214041063344, 13.73911095073034971 ) ) ;
#13267=CARTESIAN_POINT ( 'NONE',  ( 7.313483791488072150, 163.4824982072973683, 3.021315404115420679E-15 ) ) ;
#13268=CARTESIAN_POINT ( 'NONE',  ( 150.9982109096994520, 269.1104221828363734, 14.90714565999273766 ) ) ;
#13270=CARTESIAN_POINT ( 'NONE',  ( 179.1768322581812072, 294.1168262153754540, 1.049777515246110626 ) ) ;
#13271=CARTESIAN_POINT ( 'NONE',  ( 57.25197034761130510, 193.8615022471901739, 5.000000000000051514 ) ) ;
#13273=CARTESIAN_POINT ( 'NONE',  ( 190.5969391768923913, 300.5234129089444650, -0.7564693504096553500 ) ) ;
#13274=CARTESIAN_POINT ( 'NONE',  ( 24.31594170816038059, 184.8458772461660544, 9.188101187500095079 ) ) ;
#13275=CARTESIAN_POINT ( 'NONE',  ( 165.1207195983944018, 284.8810180499550597, 4.168337116055295333 ) ) ;
#13279=CARTESIAN_POINT ( 'NONE',  ( 164.3524132573224392, 245.9802652221976587, -2.749586949851067441 ) ) ;
#13280=EDGE_CURVE ( 'NONE', #66266, #99455, #31377, .T. ) ;
#13281=CARTESIAN_POINT ( 'NONE',  ( 189.0748872544347421, 267.9482830477340940, 14.04708774900528923 ) ) ;
#13282=CARTESIAN_POINT ( 'NONE',  ( 178.6026051973306323, 254.4708812555809345, 5.813106864979912913 ) ) ;
#13283=CARTESIAN_POINT ( 'NONE',  ( 164.1573396782106329, 281.5441427519270974, 8.957208755700603930 ) ) ;
#13286=CARTESIAN_POINT ( 'NONE',  ( 165.1857505493459826, 286.1010072127883177, -0.2758970588906190513 ) ) ;
#13288=CARTESIAN_POINT ( 'NONE',  ( 159.5035715461357597, 258.8388755763825202, 16.93030532244410935 ) ) ;
#13290=CARTESIAN_POINT ( 'NONE',  ( 155.6559071247401960, 261.0430556921643870, 17.79853447468815375 ) ) ;
#13292=CARTESIAN_POINT ( 'NONE',  ( 181.6354493118350035, 289.5265713693888756, 12.82447052786679542 ) ) ;
#13293=CARTESIAN_POINT ( 'NONE',  ( 176.0788078253698075, 257.6164099357736177, 12.34344903931495629 ) ) ;
#13297=B_SPLINE_CURVE_WITH_KNOTS ( 'NONE', 3,
 ( #36944, #22244, #67857, #44533 ),
 .UNSPECIFIED., .F., .F.,
 ( 4, 4 ),
 ( 0.004102704876220263433, 0.008715148612197043745 ),
 .UNSPECIFIED. ) ;
#13298=VERTEX_POINT ( 'NONE', #72050 ) ;
#13299=CARTESIAN_POINT ( 'NONE',  ( 196.6089555368279775, 289.7213370384957329, -16.36024457473861204 ) ) ;
#13300=CARTESIAN_POINT ( 'NONE',  ( 148.5203124366314285, 276.0708632542248893, -5.652538179724669654 ) ) ;
#13301=CARTESIAN_POINT ( 'NONE',  ( 179.0755312288822267, 253.6311214754194907, -0.8622901554475785879 ) ) ;
#13302=CARTESIAN_POINT ( 'NONE',  ( 155.0304386007204016, 262.1263989543018056, -17.12961552904782181 ) ) ;
#13304=VERTEX_POINT ( 'NONE', #10246 ) ;
#13306=CARTESIAN_POINT ( 'NONE',  ( 164.4761815919938215, 245.7658921781788592, 6.833796894895563412 ) ) ;
#13307=CARTESIAN_POINT ( 'NONE',  ( 192.1859061758433143, 297.7712413352111298, 11.15082371775444336 ) ) ;
#13309=CARTESIAN_POINT ( 'NONE',  ( 150.8167050463783312, 269.4247995599803289, 14.38040671671637938 ) ) ;
#13312=EDGE_LOOP ( 'NONE', ( #61220, #65838, #19420, #27984 ) ) ;
#13313=DIRECTION ( 'NONE',  ( -0.8660254037844387076, -0.4999999999999998890, -0.000000000000000000 ) ) ;
#13315=CARTESIAN_POINT ( 'NONE',  ( 164.7762319088960794, 245.2461897844768828, 2.994040459560653122 ) ) ;
#13316=CARTESIAN_POINT ( 'NONE',  ( 158.1790816997512081, 265.1500479989031192, 17.24717362645544583 ) ) ;
#13318=CARTESIAN_POINT ( 'NONE',  ( 174.4214100286941687, 277.0989115522935435, -15.68430753576282477 ) ) ;
#13319=CARTESIAN_POINT ( 'NONE',  ( 172.3722536416338755, 263.7283137945269686, -15.47002134700890608 ) ) ;
#13320=ORIENTED_EDGE ( 'NONE', *, *, #43309, .T. ) ;
#13322=CARTESIAN_POINT ( 'NONE',  ( 193.0761489135300906, 296.2292956824684893, -11.99675185248219655 ) ) ;
#13326=CARTESIAN_POINT ( 'NONE',  ( 147.0670278774466908, 275.9194309285509235, 3.666898409139099257 ) ) ;
#13327=CARTESIAN_POINT ( 'NONE',  ( 188.8233448568038000, 298.7241042047116935, -4.267409509285561953 ) ) ;
#13328=CARTESIAN_POINT ( 'NONE',  ( 148.9266665119372703, 272.6984423298952152, 12.06339424062075061 ) ) ;
#13329=DIRECTION ( 'NONE',  ( 0.4999999999999998890, -0.8660254037844385966, 0.000000000000000000 ) ) ;
#13330=CARTESIAN_POINT ( 'NONE',  ( 146.5103748552642458, 276.8835822451575268, -0.1083234189483069515 ) ) ;
#13331=CARTESIAN_POINT ( 'NONE',  ( 147.2784190576484491, 275.5532906641692534, 0.2793038414862047958 ) ) ;
#13334=CARTESIAN_POINT ( 'NONE',  ( 165.0020474182383339, 244.8550658491588479, 1.825383354618924425 ) ) ;
#13338=CARTESIAN_POINT ( 'NONE',  ( 171.3900039105615747, 288.6384802392489064, 4.197201579658607962 ) ) ;
#13341=FACE_OUTER_BOUND ( 'NONE', #20079, .T. ) ;
#13343=CARTESIAN_POINT ( 'NONE',  ( 144.9899443387551798, 254.5170451491295296, 0.000000000000000000 ) ) ;
#13345=CARTESIAN_POINT ( 'NONE',  ( 47.86207023800641025, 186.8932355074536247, -2.679491924311248496 ) ) ;
#13346=LINE ( 'NONE', #45701, #43373 ) ;
#13347=ORIENTED_EDGE ( 'NONE', *, *, #50076, .T. ) ;
#13348=CARTESIAN_POINT ( 'NONE',  ( 170.5469799148650623, 255.6610463425538740, -11.75595153296455386 ) ) ;
#13349=CARTESIAN_POINT ( 'NONE',  ( 205.4925884257800988, 274.0740247280971857, 10.80283695292349222 ) ) ;
#13350=CARTESIAN_POINT ( 'NONE',  ( 164.9779129355220562, 244.8968679994381148, -1.771286574179712803 ) ) ;
#13351=CARTESIAN_POINT ( 'NONE',  ( 33.27389197678166965, 200.0177522451419350, 5.000000000000046185 ) ) ;
#13352=CARTESIAN_POINT ( 'NONE',  ( 118.1982478153434357, 248.2369531367911293, -4.594050593750048428 ) ) ;
#13353=EDGE_CURVE ( 'NONE', #7177, #41184, #82335, .T. ) ;
#13354=CARTESIAN_POINT ( 'NONE',  ( 151.1230807375396807, 268.8941412966845519, -14.26613110909109849 ) ) ;
#13356=CARTESIAN_POINT ( 'NONE',  ( 164.8364259028313938, 281.3006012430400915, -11.81268714249731744 ) ) ;
#13358=CARTESIAN_POINT ( 'NONE',  ( 175.4442551608554197, 253.5494353995385097, -3.969463160058352980 ) ) ;
#13359=CARTESIAN_POINT ( 'NONE',  ( 40.17520546284541894, 187.8768266524160140, 9.188101187500098632 ) ) ;
#13360=CARTESIAN_POINT ( 'NONE',  ( 160.4237162281696953, 273.2376347127639633, -15.66572034412998882 ) ) ;
#13361=EDGE_LOOP ( 'NONE', ( #88641, #12699, #30043, #83456 ) ) ;
#13362=CARTESIAN_POINT ( 'NONE',  ( -1.271452699050922508, 181.6199935810941497, 2.679491924311264039 ) ) ;
#13363=CARTESIAN_POINT ( 'NONE',  ( 181.8730065081939529, 266.9336132126444454, 16.02317259067967115 ) ) ;
#13366=EDGE_CURVE ( 'NONE', #4112, #36600, #41175, .T. ) ;
#13372=CARTESIAN_POINT ( 'NONE',  ( 96.42157766939708097, 213.1427522451417644, 1.119607411625061291E-15 ) ) ;
#13374=CARTESIAN_POINT ( 'NONE',  ( 194.8081329026015283, 266.2519905409982357, -7.562986739740034992 ) ) ;
#13375=CARTESIAN_POINT ( 'NONE',  ( 162.7561251957091031, 248.7451172484279027, 11.07313294959361194 ) ) ;
#13376=CARTESIAN_POINT ( 'NONE',  ( 153.9103552012488478, 264.4948476654334968, 16.51460358841814013 ) ) ;
#13377=CARTESIAN_POINT ( 'NONE',  ( 10.86574497745707646, 167.8923013555410080, 4.594050593750050204 ) ) ;
#13379=CARTESIAN_POINT ( 'NONE',  ( 195.8285188278500470, 273.2427770020486832, 15.26130794574777383 ) ) ;
#13380=CARTESIAN_POINT ( 'NONE',  ( 146.9129474150286683, 276.1863061179126930, -5.016087650759920358 ) ) ;
#13382=CARTESIAN_POINT ( 'NONE',  ( 51.92050145378936321, 200.7833772461660828, -9.188101187500095079 ) ) ;
#13383=CARTESIAN_POINT ( 'NONE',  ( 208.3135187673106543, 269.8373969220020285, 2.829653198597726682 ) ) ;
#13384=CARTESIAN_POINT ( 'NONE',  ( 203.9008254367631423, 275.8039027522635251, 13.14957672819812906 ) ) ;
#13388=ADVANCED_FACE ( 'NONE', ( #19367 ), #17000, .F. ) ;
#13390=CARTESIAN_POINT ( 'NONE',  ( 23.47697960001819695, 174.3615022471901739, 5.000000000000051514 ) ) ;
#13391=B_SPLINE_CURVE_WITH_KNOTS ( 'NONE', 3,
 ( #12542, #34332, #96671, #35824, #65715, #11050, #89104, #27736, #3453, #3931, #81966, #50032, #19654, #50516, #18646, #89581, #27239, #57616, #80985, #43415, #74361, #58605, #58123, #72863, #26732, #4425, #57114, #19158, #11551, #65228, #66719, #4945, #33859, #95693, #42410, #64743, #81468, #12042, #96171, #41927 ),
 .UNSPECIFIED., .F., .F.,
 ( 4, 2, 2, 2, 2, 2, 2, 2, 2, 2, 2, 2, 2, 2, 2, 2, 2, 2, 2, 4 ),
 ( 0.003288512847727886965, 0.003481580978879881844, 0.003578115044455918315, 0.003674649110031955219, 0.003771183175607992124, 0.003867717241184029028, 0.004060785372336020438, 0.004446921634640086524, 0.004833057896944153477, 0.005605330421552257025, 0.006377602946160361441, 0.007922147995376568538, 0.008018682060952613683, 0.008115216126528658827, 0.008163483159316682267, 0.008211750192104705706, 0.008308284257680728299, 0.008694420519984849896, 0.009080556782288969758, 0.009466693044593091355 ),
 .UNSPECIFIED. ) ;
#13393=CARTESIAN_POINT ( 'NONE',  ( 141.2833242589136375, 258.5024278399160380, 9.188101187500095079 ) ) ;
#13395=CARTESIAN_POINT ( 'NONE',  ( 207.5810977459049127, 271.1059873436086036, -7.529053122148023469 ) ) ;
#13398=CARTESIAN_POINT ( 'NONE',  ( 157.7861133721078772, 257.3534302411229646, 18.03837896619386783 ) ) ;
#13399=CARTESIAN_POINT ( 'NONE',  ( 189.2359190933219679, 289.8534420722585310, 14.44421633591829845 ) ) ;
#13403=CARTESIAN_POINT ( 'NONE',  ( 190.7851866479434761, 300.1973587246873194, 7.931162401707728016 ) ) ;
#13404=CARTESIAN_POINT ( 'NONE',  ( 163.5920121195164256, 247.2973186270110091, 8.917636558496976562 ) ) ;
#13405=CARTESIAN_POINT ( 'NONE',  ( 175.5746833524315775, 278.5347786252573314, 16.94864957847115505 ) ) ;
#13406=CARTESIAN_POINT ( 'NONE',  ( 172.8373704755632332, 268.6438884681230661, -16.58280638298598575 ) ) ;
#13407=CARTESIAN_POINT ( 'NONE',  ( 193.8727374453239349, 270.7503200800575769, -13.89828984444790017 ) ) ;
#13408=ORIENTED_EDGE ( 'NONE', *, *, #1703, .F. ) ;
#13410=VECTOR ( 'NONE', #42774, 1000.000000000000000 ) ;
#13413=B_SPLINE_SURFACE_WITH_KNOTS ( 'NONE', 3, 1, ( 
 ( #1565, #86703 ),
 ( #23332, #54220 ),
 ( #47633, #30446 ),
 ( #40024, #85186 ),
 ( #69442, #9150 ),
 ( #32450, #92294 ),
 ( #62835, #78565 ),
 ( #53728, #62325 ),
 ( #84687, #15733 ),
 ( #46638, #23834 ),
 ( #77563, #93791 ),
 ( #94284, #39519 ),
 ( #1053, #77038 ),
 ( #15228, #8152 ),
 ( #46122, #93279 ),
 ( #39026, #7644 ),
 ( #24352, #69932 ),
 ( #551, #54728 ),
 ( #85709, #16245 ),
 ( #47136, #38535 ),
 ( #60, #96792 ),
 ( #26356, #18758 ),
 ( #71962, #58233 ),
 ( #80091, #56234 ),
 ( #57232, #11663 ),
 ( #49637, #42039 ),
 ( #95803, #40531 ),
 ( #50630, #26852 ),
 ( #42525, #11172 ),
 ( #87227, #49156 ),
 ( #88707, #64346 ),
 ( #65827, #41534 ),
 ( #79594, #32939 ),
 ( #19277, #27352 ) ),
 .UNSPECIFIED., .T., .F., .F.,
 ( 4, 2, 2, 2, 2, 2, 2, 2, 2, 2, 2, 2, 2, 2, 2, 2, 4 ),
 ( 2, 2 ),
 ( 0.000000000000000000, 0.06250000000000000000, 0.1250000000000000000, 0.1875000000000000000, 0.2500000000000000000, 0.3125000000000000000, 0.3750000000000000000, 0.4375000000000000000, 0.5000000000000000000, 0.5625000000000000000, 0.6250000000000000000, 0.6875000000000000000, 0.7500000000000000000, 0.8125000000000000000, 0.8750000000000000000, 0.9375000000000000000, 1.000000000000000000 ),
 ( 0.000000000000000000, 1.000000000000000000 ),
 .UNSPECIFIED. ) ;
#13414=CARTESIAN_POINT ( 'NONE',  ( 200.8510819094290696, 281.8070453751917057, -16.75700185107683282 ) ) ;
#13415=CARTESIAN_POINT ( 'NONE',  ( 196.1722677117792557, 270.9862039110303158, 12.91586066753414919 ) ) ;
#13416=CARTESIAN_POINT ( 'NONE',  ( 185.7938733065929853, 296.8758775647544894, 5.418709528595011982 ) ) ;
#13417=CARTESIAN_POINT ( 'NONE',  ( 137.8880043751089772, 261.9637435831424455, 2.679491924311251605 ) ) ;
#13418=CARTESIAN_POINT ( 'NONE',  ( 175.1271263694729328, 272.4273639404348728, 17.81557788710851042 ) ) ;
#13420=ORIENTED_EDGE ( 'NONE', *, *, #98027, .T. ) ;
#13426=CARTESIAN_POINT ( 'NONE',  ( 159.6494826941923861, 264.1119501240779073, -17.72553829314773566 ) ) ;
#13427=B_SPLINE_CURVE_WITH_KNOTS ( 'NONE', 3,
 ( #4751, #66040, #60404, #74663 ),
 .UNSPECIFIED., .F., .F.,
 ( 4, 4 ),
 ( 0.01047501919852616287, 0.01579130575507147610 ),
 .UNSPECIFIED. ) ;
#13429=CARTESIAN_POINT ( 'NONE',  ( 147.1447476476323004, 275.7848163378367872, 0.6373001129109078233 ) ) ;
#13430=CARTESIAN_POINT ( 'NONE',  ( 185.6176320207485446, 291.1239150995572231, 12.16464820431206206 ) ) ;
#13431=B_SPLINE_CURVE_WITH_KNOTS ( 'NONE', 3,
 ( #24669, #47467, #93098, #55552, #22686, #53565, #30783, #45952, #872, #16072, #86536, #17066, #46974, #78900, #8479, #61664 ),
 .UNSPECIFIED., .F., .F.,
 ( 4, 2, 2, 2, 2, 2, 2, 4 ),
 ( -9.576356418732827919E-06, 3.142278651979172423E-05, 7.242192945831627806E-05, 0.0001544202153353389177, 0.0003184167870893806732, 0.0006464099305974667321, 0.0009744030741055529537, 0.001302396217613638850 ),
 .UNSPECIFIED. ) ;
#13432=CARTESIAN_POINT ( 'NONE',  ( 204.2556901454867955, 276.8657622634082713, 13.61111001399713949 ) ) ;
#13433=CARTESIAN_POINT ( 'NONE',  ( 159.3655983545995127, 283.2591999228209829, -2.078818975303923899 ) ) ;
#13434=CARTESIAN_POINT ( 'NONE',  ( 49.32136238152735785, 210.8297689869269220, -2.679491924311252493 ) ) ;
#13436=CARTESIAN_POINT ( 'NONE',  ( 92.46148921633090367, 218.0643266524160140, 9.188101187500095079 ) ) ;
#13437=CARTESIAN_POINT ( 'NONE',  ( 155.2317605920271717, 261.7776990366773475, 17.06683146360218828 ) ) ;
#13443=CARTESIAN_POINT ( 'NONE',  ( 207.3790894204113613, 271.0808592135389858, 2.321707834868911302 ) ) ;
#13444=ORIENTED_EDGE ( 'NONE', *, *, #54776, .T. ) ;
#13449=VERTEX_POINT ( 'NONE', #29919 ) ;
#13450=CARTESIAN_POINT ( 'NONE',  ( 165.5428789467008244, 248.7867348279617659, -9.239987926238155680 ) ) ;
#13451=CARTESIAN_POINT ( 'NONE',  ( 174.4380169027350291, 291.1401200322444538, -5.384106100014290242 ) ) ;
#13453=CARTESIAN_POINT ( 'NONE',  ( 10.46624461501205872, 188.3967562850346837, -4.648177544792955347E-16 ) ) ;
#13455=CARTESIAN_POINT ( 'NONE',  ( 164.7447033178649747, 265.0565378767570905, -16.62346194256757315 ) ) ;
#13456=ORIENTED_EDGE ( 'NONE', *, *, #48506, .F. ) ;
#13461=CARTESIAN_POINT ( 'NONE',  ( 200.0161915203198362, 270.0763376282534409, 10.26060645788218295 ) ) ;
#13463=DIRECTION ( 'NONE',  ( -0.8660254037844387076, -0.4999999999999998890, -0.000000000000000000 ) ) ;
#13464=CARTESIAN_POINT ( 'NONE',  ( 187.3586742363142150, 260.2951279848165882, 2.860953161626957009 ) ) ;
#13465=CARTESIAN_POINT ( 'NONE',  ( 150.9020882617336383, 276.5917379820504038, -5.284388463461365149 ) ) ;
#13467=DIRECTION ( 'NONE',  ( -0.8660254037844387076, -0.4999999999999998890, -0.000000000000000000 ) ) ;
#13468=CARTESIAN_POINT ( 'NONE',  ( 147.1270795744234476, 264.4111747905818675, -1.822351119449947324E-15 ) ) ;
#13469=CARTESIAN_POINT ( 'NONE',  ( 195.1831177385782894, 292.1517303617533230, 15.29763345156017174 ) ) ;
#13470=VERTEX_POINT ( 'NONE', #36514 ) ;
#13473=CARTESIAN_POINT ( 'NONE',  ( 160.3055490814878681, 276.2749098051363603, 12.65412181104003508 ) ) ;
#13475=CARTESIAN_POINT ( 'NONE',  ( 171.3124858205567023, 279.6758709237702760, -14.80999945890478742 ) ) ;
#13476=CARTESIAN_POINT ( 'NONE',  ( 203.9713276076765283, 277.3582926266647632, -14.32166128205299138 ) ) ;
#13478=CARTESIAN_POINT ( 'NONE',  ( 164.5892160260162882, 274.3781231134265681, 14.76927392745111334 ) ) ;
#13479=CARTESIAN_POINT ( 'NONE',  ( -5.561934722402757991, 167.5958772461660544, -9.188101187500095079 ) ) ;
#13481=CARTESIAN_POINT ( 'NONE',  ( 28.09809348231459936, 175.4824982072973967, 3.021315404115420679E-15 ) ) ;
#13484=CARTESIAN_POINT ( 'NONE',  ( 156.6812872898450735, 261.2670451491295012, 0.000000000000000000 ) ) ;
#13489=CARTESIAN_POINT ( 'NONE',  ( 174.0250796533206312, 290.1103312770194407, 2.568368125944323843 ) ) ;
#13493=CARTESIAN_POINT ( 'NONE',  ( 171.1295603993285965, 249.6517061031812545, 4.344809613321301889 ) ) ;
#13494=CARTESIAN_POINT ( 'NONE',  ( 10.51348828746337816, 183.0024278399160949, -9.188101187500093303 ) ) ;
#13496=CARTESIAN_POINT ( 'NONE',  ( 114.9778026189612632, 243.3149278399160664, 9.188101187500093303 ) ) ;
#13500=AXIS2_PLACEMENT_3D ( 'NONE', #40536, #22486, #53378 ) ;
#13501=CARTESIAN_POINT ( 'NONE',  ( 181.1156277128715431, 292.7914473640799997, 9.490545386343454126 ) ) ;
#13502=CARTESIAN_POINT ( 'NONE',  ( 190.0977106519948450, 299.8480667433163944, -5.515936301684110532 ) ) ;
#13503=CARTESIAN_POINT ( 'NONE',  ( 154.8596847415876994, 262.4221533139083817, 17.65401077761399762 ) ) ;
#13504=LINE ( 'NONE', #98613, #93405 ) ;
#13505=CARTESIAN_POINT ( 'NONE',  ( 147.6095889327917803, 274.9796876144846465, -8.460961150142429332 ) ) ;
#13507=CARTESIAN_POINT ( 'NONE',  ( 187.7344944884639801, 299.0281582812487500, -0.5885417617450732219 ) ) ;
#13508=CARTESIAN_POINT ( 'NONE',  ( 78.46959274032997200, 226.1115022471903160, -5.000000000000047962 ) ) ;
#13509=CARTESIAN_POINT ( 'NONE',  ( 183.8229730883442130, 268.4974150671761777, -15.08127568743503311 ) ) ;
#13514=CARTESIAN_POINT ( 'NONE',  ( 93.48972083544241229, 224.7833772461660260, -9.188101187500095079 ) ) ;
#13516=CARTESIAN_POINT ( 'NONE',  ( 172.9380501958987111, 251.0613099074927561, -5.462789090222858412 ) ) ;
#13517=CARTESIAN_POINT ( 'NONE',  ( 196.4390255720217908, 290.4046224503736653, 16.34739044515864848 ) ) ;
#13518=CARTESIAN_POINT ( 'NONE',  ( 200.4229826824105203, 283.5042063200048119, 17.40835197696380376 ) ) ;
#13519=CARTESIAN_POINT ( 'NONE',  ( 149.1848515893298952, 272.2512526580950407, 13.00839212001256229 ) ) ;
#13520=CARTESIAN_POINT ( 'NONE',  ( 151.1699610800269511, 268.8129421616204695, -14.28929860221299286 ) ) ;
#13523=CARTESIAN_POINT ( 'NONE',  ( 192.9633865298379476, 296.4246058602058156, -11.85717392250713864 ) ) ;
#13528=CARTESIAN_POINT ( 'NONE',  ( 197.1972787308770023, 267.5603457548782558, 9.837912184082732381 ) ) ;
#13529=CARTESIAN_POINT ( 'NONE',  ( 191.6361107213085120, 287.8645130632154974, -15.84396015365595289 ) ) ;
#13532=CARTESIAN_POINT ( 'NONE',  ( 198.6012358295098750, 286.6595644277572887, 18.21911298807435386 ) ) ;
#13534=CARTESIAN_POINT ( 'NONE',  ( 170.7170432258869255, 252.9330647848325668, -8.768963007360460082 ) ) ;
#13536=CARTESIAN_POINT ( 'NONE',  ( 135.1220879045620507, 255.4865022471903444, 10.00000000000009237 ) ) ;
#13537=CARTESIAN_POINT ( 'NONE',  ( 157.0887340267001946, 258.5613266995183039, -17.61824281915036394 ) ) ;
#13541=CARTESIAN_POINT ( 'NONE',  ( 196.8307300463833087, 264.7821886061209966, -4.649540328500814113 ) ) ;
#13542=DIRECTION ( 'NONE',  ( 0.4999999999999998890, -0.8660254037844385966, 0.000000000000000000 ) ) ;
#13543=ORIENTED_EDGE ( 'NONE', *, *, #32562, .T. ) ;
#13544=CARTESIAN_POINT ( 'NONE',  ( 185.2870392614587445, 292.5660204067580139, -10.68714641920701602 ) ) ;
#13546=CYLINDRICAL_SURFACE ( 'NONE', #81433, 17.82106496071139645 ) ;
#13548=CARTESIAN_POINT ( 'NONE',  ( 158.4014687745750223, 256.2876034193376427, 17.30374031384843292 ) ) ;
#13550=CARTESIAN_POINT ( 'NONE',  ( 152.8328714238065515, 265.9326969577624027, -16.29536156676786263 ) ) ;
#13561=CARTESIAN_POINT ( 'NONE',  ( 174.5182925596964196, 257.2711356623013899, -12.07587375265958229 ) ) ;
#13562=CARTESIAN_POINT ( 'NONE',  ( 163.8998849419727435, 272.9681336415193869, -15.35406178914973907 ) ) ;
#13563=CARTESIAN_POINT ( 'NONE',  ( -22.42236680055709641, 157.8615022471902591, 0.000000000000000000 ) ) ;
#13564=CARTESIAN_POINT ( 'NONE',  ( 197.8534124529632834, 273.4752411235029967, -13.40023471225654106 ) ) ;
#13567=CARTESIAN_POINT ( 'NONE',  ( 190.5154909595809727, 300.6644853595138329, -0.04129855346138300298 ) ) ;
#13568=CARTESIAN_POINT ( 'NONE',  ( 167.3389692517741878, 286.2055908521544438, -4.776237697990188380 ) ) ;
#13572=CARTESIAN_POINT ( 'NONE',  ( 107.8059429699301575, 242.2369531367911009, -4.594050593750048428 ) ) ;
#13574=CARTESIAN_POINT ( 'NONE',  ( 191.6404332549959690, 275.2293478342741651, 16.16297667511041425 ) ) ;
#13575=EDGE_LOOP ( 'NONE', ( #67097, #45065, #10208, #73381 ) ) ;
#13578=CARTESIAN_POINT ( 'NONE',  ( 157.8360072705708603, 257.2670114739976839, 17.12122855844125269 ) ) ;
#13581=ORIENTED_EDGE ( 'NONE', *, *, #62001, .F. ) ;
#13583=CARTESIAN_POINT ( 'NONE',  ( 201.3911183001464451, 266.9640362439821502, -3.754059931952923534 ) ) ;
#13584=ORIENTED_EDGE ( 'NONE', *, *, #26286, .F. ) ;
#13585=CARTESIAN_POINT ( 'NONE',  ( 192.4760896514942203, 263.8193595997221337, -8.316349228157742246 ) ) ;
#13587=FACE_OUTER_BOUND ( 'NONE', #15754, .T. ) ;
#13588=CARTESIAN_POINT ( 'NONE',  ( 198.2391837281077756, 286.3575794386269422, 17.25947343406376078 ) ) ;
#13590=CARTESIAN_POINT ( 'NONE',  ( 202.7282074973916792, 277.5114398175890642, -15.40750263959311184 ) ) ;
#13591=ORIENTED_EDGE ( 'NONE', *, *, #49408, .F. ) ;
#13592=DIRECTION ( 'NONE',  ( 0.8660254037844395958, 0.4999999999999985567, 0.000000000000000000 ) ) ;
#13593=CARTESIAN_POINT ( 'NONE',  ( 179.8432160940321296, 258.5759063625694694, 11.15262217193699001 ) ) ;
#13595=CARTESIAN_POINT ( 'NONE',  ( 173.7083855031236510, 250.9142590195035325, -1.051028738215985303 ) ) ;
#13596=CARTESIAN_POINT ( 'NONE',  ( 122.6368883333364295, 231.6115022471901739, -5.000000000000041744 ) ) ;
#13600=EDGE_CURVE ( 'NONE', #87229, #49470, #20020, .T. ) ;
#13601=CARTESIAN_POINT ( 'NONE',  ( -17.42236680055705023, 149.2012482093457777, 0.000000000000000000 ) ) ;
#13605=CARTESIAN_POINT ( 'NONE',  ( 80.01237403692960015, 210.8768266524159856, -9.188101187500091527 ) ) ;
#13606=CARTESIAN_POINT ( 'NONE',  ( 159.8946522441011382, 253.7013337850969492, -16.68230890105693121 ) ) ;
#13608=CARTESIAN_POINT ( 'NONE',  ( 162.6425574510925003, 248.9418223522047526, -10.70838742014210077 ) ) ;
#13609=EDGE_CURVE ( 'NONE', #2782, #29718, #21806, .T. ) ;
#13611=CARTESIAN_POINT ( 'NONE',  ( 207.6129110656513035, 271.0508850574501025, -5.265106572941297358 ) ) ;
#13621=CARTESIAN_POINT ( 'NONE',  ( 30.10766014385131939, 182.0643266524160424, 9.188101187500095079 ) ) ;
#13624=CARTESIAN_POINT ( 'NONE',  ( 199.7368853651836105, 277.6985558088923653, 15.20939665263245111 ) ) ;
#13625=CARTESIAN_POINT ( 'NONE',  ( 194.3442947553755005, 294.0328026529847421, -15.97648891113594871 ) ) ;
#13627=CARTESIAN_POINT ( 'NONE',  ( 58.84905177982987823, 192.5327760586659451, 1.948934522072302763E-15 ) ) ;
#13629=CARTESIAN_POINT ( 'NONE',  ( 198.9590707264871412, 286.0397762054715827, -17.05306195936250191 ) ) ;
#13632=CARTESIAN_POINT ( 'NONE',  ( 201.1507709783248004, 268.9741687161805999, -6.437191260250949121 ) ) ;
#13634=CARTESIAN_POINT ( 'NONE',  ( 179.9883836461400506, 276.4655832705219041, 17.64582730720814752 ) ) ;
#13638=CARTESIAN_POINT ( 'NONE',  ( 163.4836020540464006, 255.6328358810647785, -14.84222631813321236 ) ) ;
#13640=CARTESIAN_POINT ( 'NONE',  ( 86.69683407628214411, 230.8615022471903160, 5.000000000000046185 ) ) ;
#13641=CARTESIAN_POINT ( 'NONE',  ( 200.1385401540174769, 283.9968752310148830, 17.30012534137638625 ) ) ;
#13642=CARTESIAN_POINT ( 'NONE',  ( 165.0023938551389051, 269.5197546249395941, -16.29883053466163645 ) ) ;
#13644=CARTESIAN_POINT ( 'NONE',  ( 50.64826632015721231, 209.2369531367911293, -4.594050593750048428 ) ) ;
#13645=ORIENTED_EDGE ( 'NONE', *, *, #82293, .F. ) ;
#13647=CARTESIAN_POINT ( 'NONE',  ( 147.4368675721658519, 275.2788497866417288, 5.050119523016719292 ) ) ;
#13650=EDGE_CURVE ( 'NONE', #4734, #52681, #44539, .T. ) ;
#13651=CARTESIAN_POINT ( 'NONE',  ( -22.42236680055709641, 157.8615022471902591, 0.000000000000000000 ) ) ;
#13654=CARTESIAN_POINT ( 'NONE',  ( 176.1831251786226176, 274.1662096868063259, -16.54240975180354312 ) ) ;
#13656=EDGE_CURVE ( 'NONE', #20045, #29993, #18233, .T. ) ;
#13657=CARTESIAN_POINT ( 'NONE',  ( 204.7705395286511703, 275.9740169735222821, 14.67688412961845579 ) ) ;
#13664=CARTESIAN_POINT ( 'NONE',  ( 182.6072171861806623, 283.8313970932354664, 15.32190259022742929 ) ) ;
#13665=CARTESIAN_POINT ( 'NONE',  ( 206.6298919378964740, 272.7535241315335384, -9.267551915974392429 ) ) ;
#13667=CARTESIAN_POINT ( 'NONE',  ( 165.5951377484445288, 285.5575308855258641, -6.564525145918313598 ) ) ;
#13669=FACE_OUTER_BOUND ( 'NONE', #57048, .T. ) ;
#13671=CARTESIAN_POINT ( 'NONE',  ( 160.0105735053945182, 253.5005522708592594, 16.10371386499367929 ) ) ;
#13675=CARTESIAN_POINT ( 'NONE',  ( 121.1210835531159091, 249.9244531367911293, -4.594050593750046652 ) ) ;
#13676=CARTESIAN_POINT ( 'NONE',  ( 204.8523313866422484, 275.8323493198358847, 14.65426965484541100 ) ) ;
#13678=CARTESIAN_POINT ( 'NONE',  ( 170.1416266488643316, 264.1956996214873357, 16.71664234929178505 ) ) ;
#13681=CARTESIAN_POINT ( 'NONE',  ( 160.2165948300100808, 253.5243271026905632, 14.75162392979510528 ) ) ;
#13683=ORIENTED_EDGE ( 'NONE', *, *, #23169, .T. ) ;
#13686=CARTESIAN_POINT ( 'NONE',  ( 2.117331368781439682, 160.4824982072973683, 3.021315404115420679E-15 ) ) ;
#13687=CARTESIAN_POINT ( 'NONE',  ( 147.2784190576484491, 275.5532906641692534, 0.2793038414862047958 ) ) ;
#13689=CARTESIAN_POINT ( 'NONE',  ( 194.2669918475045279, 294.1666952169902629, 14.00965265288584050 ) ) ;
#13693=AXIS2_PLACEMENT_3D ( 'NONE', #30130, #22535, #53422 ) ;
#13697=EDGE_LOOP ( 'NONE', ( #37024, #42691, #35607, #46963 ) ) ;
#13700=CARTESIAN_POINT ( 'NONE',  ( 174.2182000476488781, 253.7820565303687772, -7.498782541138584889 ) ) ;
#13702=CARTESIAN_POINT ( 'NONE',  ( 206.4768661561222984, 273.0185725604343361, 11.39716120335626925 ) ) ;
#13704=CARTESIAN_POINT ( 'NONE',  ( 144.9103262809084924, 242.2202760586659167, -5.415160957724236172E-17 ) ) ;
#13705=ORIENTED_EDGE ( 'NONE', *, *, #21120, .T. ) ;
#13709=CARTESIAN_POINT ( 'NONE',  ( 150.1593742671934137, 278.0125080970104250, -1.457479655811878994 ) ) ;
#13711=ORIENTED_EDGE ( 'NONE', *, *, #46180, .F. ) ;
#13713=CARTESIAN_POINT ( 'NONE',  ( 185.2639226435235287, 277.5828175794305253, -16.89321975366465622 ) ) ;
#13714=CARTESIAN_POINT ( 'NONE',  ( 167.5773306199838260, 249.1887448877641020, -5.496113628205799628 ) ) ;
#13717=CARTESIAN_POINT ( 'NONE',  ( 195.6138585057339014, 264.3086811827035376, 0.8332931476443066199 ) ) ;
#13718=EDGE_CURVE ( 'NONE', #59645, #38166, #67629, .T. ) ;
#13720=CARTESIAN_POINT ( 'NONE',  ( 182.9739835170253741, 280.6533030732829275, 16.67168179050610277 ) ) ;
#13721=CARTESIAN_POINT ( 'NONE',  ( 195.8334532154173075, 270.5958172793855852, 12.00696150519691585 ) ) ;
#13725=CYLINDRICAL_SURFACE ( 'NONE', #3019, 17.82106496071139645 ) ;
#13726=CARTESIAN_POINT ( 'NONE',  ( 198.1230806404959139, 287.4877535090322453, 17.00698319228197164 ) ) ;
#13727=CARTESIAN_POINT ( 'NONE',  ( 161.8938357633344651, 250.2386463561303458, 14.09469623995626719 ) ) ;
#13728=CARTESIAN_POINT ( 'NONE',  ( -4.722712290662820500, 158.8923013555410080, 4.594050593750050204 ) ) ;
#13729=CARTESIAN_POINT ( 'NONE',  ( 172.1838089403669585, 283.7306525937339075, -12.60449918999284513 ) ) ;
#13732=CARTESIAN_POINT ( 'NONE',  ( 198.7136873185829984, 286.4647927352960437, -18.57144721070432070 ) ) ;
#13733=CARTESIAN_POINT ( 'NONE',  ( -1.313257906909115480, 179.2369531367911293, -4.594050593750048428 ) ) ;
#13736=CARTESIAN_POINT ( 'NONE',  ( 205.2121761402296443, 275.2090799237855094, -14.05269615702442465 ) ) ;
#13740=CARTESIAN_POINT ( 'NONE',  ( 70.44081555586384980, 218.1427522451419065, -10.00000000000009415 ) ) ;
#13741=CARTESIAN_POINT ( 'NONE',  ( 176.1981167356123308, 253.9691465762882672, -3.865530600323666466 ) ) ;
#13742=CARTESIAN_POINT ( 'NONE',  ( 198.2555168952299027, 287.2583671870688704, 16.98288975666356748 ) ) ;
#13744=CARTESIAN_POINT ( 'NONE',  ( 64.25234236153551137, 201.2365022471902023, -10.00000000000009059 ) ) ;
#13746=CARTESIAN_POINT ( 'NONE',  ( 148.2980785574368952, 273.7871886041155562, 9.134436720559454770 ) ) ;
#13747=CARTESIAN_POINT ( 'NONE',  ( 15.73713787374454043, 170.7048013555409796, 4.594050593750051981 ) ) ;
#13748=CARTESIAN_POINT ( 'NONE',  ( 168.2754412017935977, 286.2846751750494150, 4.214248324995869766 ) ) ;
#13751=CARTESIAN_POINT ( 'NONE',  ( 165.5845016731641124, 245.8462254865437160, 0.7221155814038995313 ) ) ;
#13753=FACE_OUTER_BOUND ( 'NONE', #94286, .T. ) ;
#13754=CARTESIAN_POINT ( 'NONE',  ( 185.7319119612792520, 266.7507276504825313, 13.19901251433546641 ) ) ;
#13755=CARTESIAN_POINT ( 'NONE',  ( -22.42236680055709641, 157.8615022471902591, 0.000000000000000000 ) ) ;
#13756=CARTESIAN_POINT ( 'NONE',  ( 160.8891438268352374, 281.0495864612497599, 9.578199528566821996 ) ) ;
#13759=CARTESIAN_POINT ( 'NONE',  ( 189.8123550829396891, 301.8823524224806647, -0.5679054518196169354 ) ) ;
#13760=DIRECTION ( 'NONE',  ( -0.8660254037844387076, -0.4999999999999998890, -0.000000000000000000 ) ) ;
#13763=CARTESIAN_POINT ( 'NONE',  ( 154.9344967692067598, 262.2925750810547356, 17.30210568643136781 ) ) ;
#13765=CARTESIAN_POINT ( 'NONE',  ( 185.3399667980721972, 290.9400795177430155, 12.16828865084649536 ) ) ;
#13766=CARTESIAN_POINT ( 'NONE',  ( 187.4166251561426293, 263.4339899954952102, 11.64397722261905166 ) ) ;
#13768=ADVANCED_FACE ( 'NONE', ( #49256 ), #23557, .T. ) ;
#13770=CARTESIAN_POINT ( 'NONE',  ( 195.4590938341275717, 290.3887709481238062, -16.68818639969873985 ) ) ;
#13773=CARTESIAN_POINT ( 'NONE',  ( 202.9490938173916561, 279.1288534886517709, -16.56031645010252973 ) ) ;
#13775=( BOUNDED_CURVE ( )  B_SPLINE_CURVE ( 2, ( #73222, #34696, #65598, #83835, #99011, #45769, #68584, #15365, #92915 ),
 .UNSPECIFIED., .F., .T. ) 
 B_SPLINE_CURVE_WITH_KNOTS ( ( 3, 2, 2, 2, 3 ),
 ( 0.2943548387096774355, 0.2956989247311828106, 0.2983870967741935609, 0.3010752688172043112, 0.3024193548387096864 ),
 .UNSPECIFIED. ) 
 CURVE ( )  GEOMETRIC_REPRESENTATION_ITEM ( )  RATIONAL_B_SPLINE_CURVE ( ( 0.9330127018922194093, 0.9330127018922194093, 1.000000000000000000, 0.8660254037844387076, 1.000000000000000000, 0.8660254037844387076, 1.000000000000000000, 0.9330127018922194093, 0.9330127018922194093 ) ) 
 REPRESENTATION_ITEM ( '' )  );
#13776=ORIENTED_EDGE ( 'NONE', *, *, #20226, .T. ) ;
#13777=CARTESIAN_POINT ( 'NONE',  ( 186.5702472824191318, 272.0476927240400755, -16.61350243714774066 ) ) ;
#13778=CARTESIAN_POINT ( 'NONE',  ( 204.6427704787179493, 276.1953194596412118, 13.28850621060895953 ) ) ;
#13780=CARTESIAN_POINT ( 'NONE',  ( 151.2455280670316711, 268.6820563007532314, 14.35914944935941229 ) ) ;
#13784=VERTEX_POINT ( 'NONE', #84914 ) ;
#13787=B_SPLINE_CURVE_WITH_KNOTS ( 'NONE', 3,
 ( #8693, #39562, #101, #31476, #23376, #76597, #85233, #38068, #47675, #16288, #15779, #69977, #7182, #24884, #93841, #38581, #47182, #40069 ),
 .UNSPECIFIED., .F., .F.,
 ( 4, 2, 2, 2, 2, 2, 2, 2, 4 ),
 ( 0.0001829895512004093639, 0.0005381298376754407690, 0.0008932701241504720658, 0.001248410410625503363, 0.001603550697100531407, 0.001958690983575559017, 0.002313831270050587061, 0.002668971556525614672, 0.003024111843000642282 ),
 .UNSPECIFIED. ) ;
#13789=CARTESIAN_POINT ( 'NONE',  ( 164.2813349609167517, 246.1033764428878214, 1.949810150281061638 ) ) ;
#13790=CARTESIAN_POINT ( 'NONE',  ( 150.8555837531579868, 276.0290483310748755, -8.437460036063264113 ) ) ;
#13792=CARTESIAN_POINT ( 'NONE',  ( 149.3833831332874240, 271.9073859370555510, 11.40518020539810173 ) ) ;
#13793=CARTESIAN_POINT ( 'NONE',  ( 172.2573413188522977, 264.0388785342783535, -16.66050399420761607 ) ) ;
#13795=CARTESIAN_POINT ( 'NONE',  ( 161.1881684952116416, 277.3746372515906273, -13.39559945919683948 ) ) ;
#13796=EDGE_CURVE ( 'NONE', #13906, #74614, #45898, .T. ) ;
#13801=VERTEX_POINT ( 'NONE', #61566 ) ;
#13803=CARTESIAN_POINT ( 'NONE',  ( 190.1858949294064871, 301.2353624297489887, -5.249932979468886707 ) ) ;
#13804=CARTESIAN_POINT ( 'NONE',  ( 188.3515280933679890, 299.0335169455429423, -5.233410187156488647 ) ) ;
#13806=CARTESIAN_POINT ( 'NONE',  ( 153.1973045377566507, 265.3014802884401320, 17.70608187426261892 ) ) ;
#13807=CARTESIAN_POINT ( 'NONE',  ( 191.2490492842387368, 299.3939250708912141, 9.771632328273542001 ) ) ;
#13808=CARTESIAN_POINT ( 'NONE',  ( 146.9456733906991417, 276.1296230653242105, -0.7988785540157754550 ) ) ;
#13809=ORIENTED_EDGE ( 'NONE', *, *, #39078, .F. ) ;
#13811=CARTESIAN_POINT ( 'NONE',  ( 149.3141802193904368, 272.0272488999566463, -11.40332369054239336 ) ) ;
#13813=CARTESIAN_POINT ( 'NONE',  ( 189.5821670815687412, 300.5718190871559159, 1.753508275674212413 ) ) ;
#13815=CARTESIAN_POINT ( 'NONE',  ( 102.8537940617441819, 224.0643266524160140, 9.188101187500095079 ) ) ;
#13817=CARTESIAN_POINT ( 'NONE',  ( 149.5844699681647683, 271.5590933223148227, -11.62982666799845788 ) ) ;
#13818=EDGE_CURVE ( 'NONE', #88596, #30831, #51670, .T. ) ;
#13821=CARTESIAN_POINT ( 'NONE',  ( 149.0332838374355617, 273.1880737991430124, 9.708030931401681940 ) ) ;
#13827=CARTESIAN_POINT ( 'NONE',  ( 168.1460105092157846, 253.8898197004758117, -11.82587461664797779 ) ) ;
#13830=CARTESIAN_POINT ( 'NONE',  ( 155.3692710881836661, 261.9322098443626601, 16.97327933481185624 ) ) ;
#13831=CARTESIAN_POINT ( 'NONE',  ( 43.66619682219493370, 206.0177522451419350, 5.000000000000046185 ) ) ;
#13832=CARTESIAN_POINT ( 'NONE',  ( 120.0931990297694085, 230.9548013555409796, -4.594050593750042211 ) ) ;
#13835=ADVANCED_FACE ( 'NONE', ( #95903 ), #78292, .T. ) ;
#13836=CARTESIAN_POINT ( 'NONE',  ( 165.5298684834693574, 269.3554679133272884, -17.63324793928101997 ) ) ;
#13837=CARTESIAN_POINT ( 'NONE',  ( 157.0957870390718369, 258.5491105237443321, 17.69218919045495397 ) ) ;
#13838=CARTESIAN_POINT ( 'NONE',  ( 172.2297690901025646, 250.8531890094506878, -4.040578270607043443 ) ) ;
#13839=CARTESIAN_POINT ( 'NONE',  ( 39.55283647781661216, 184.4548013555409796, -4.594050593750042211 ) ) ;
#13843=EDGE_CURVE ( 'NONE', #8304, #130, #90655, .T. ) ;
#13846=CARTESIAN_POINT ( 'NONE',  ( 19.39713158799116499, 193.5530062829863311, -4.648177544792955347E-16 ) ) ;
#13847=CARTESIAN_POINT ( 'NONE',  ( 190.9380839614473473, 299.9325328093580652, -5.232187664503159752 ) ) ;
#13849=CARTESIAN_POINT ( 'NONE',  ( 164.4288763552480646, 253.6070193120362148, -14.40234560624782389 ) ) ;
#13850=CARTESIAN_POINT ( 'NONE',  ( 178.0315741628076012, 287.5935043698759728, -13.06113257055532451 ) ) ;
#13852=CARTESIAN_POINT ( 'NONE',  ( 111.2883471010299274, 228.3927522451418213, 10.00000000000009592 ) ) ;
#13854=CARTESIAN_POINT ( 'NONE',  ( 195.0751939884018782, 266.5450544056012063, -7.747489274975008833 ) ) ;
#13855=CARTESIAN_POINT ( 'NONE',  ( 155.1510707464528025, 280.2034007906984812, -2.423017525748603962 ) ) ;
#13856=CARTESIAN_POINT ( 'NONE',  ( 154.0926933875380485, 264.1656124941568464, 16.59860039027621426 ) ) ;
#13858=CARTESIAN_POINT ( 'NONE',  ( 12.40843950188935629, 165.7202760586659736, -5.415160957724236172E-17 ) ) ;
#13860=CARTESIAN_POINT ( 'NONE',  ( 192.3455884257783453, 272.0184315964207258, 14.19712417015736605 ) ) ;
#13863=CARTESIAN_POINT ( 'NONE',  ( 197.6572998268543699, 277.0061036579921279, -15.32695017695141892 ) ) ;
#13864=CARTESIAN_POINT ( 'NONE',  ( 45.15450443884093090, 203.0024278399160949, 9.188101187500095079 ) ) ;
#13865=CARTESIAN_POINT ( 'NONE',  ( 208.0287371622045782, 270.3306531311065442, 3.558879245883286746 ) ) ;
#13871=CARTESIAN_POINT ( 'NONE',  ( 13.08467475460494001, 168.3615022471902023, 5.000000000000051514 ) ) ;
#13872=CARTESIAN_POINT ( 'NONE',  ( 163.8947349411736525, 246.7729873192901664, -5.868803394723933309 ) ) ;
#13873=CARTESIAN_POINT ( 'NONE',  ( 141.5541307454787727, 252.5333772461660260, 9.188101187500095079 ) ) ;
#13875=CARTESIAN_POINT ( 'NONE',  ( 164.3112480427713251, 246.0515654653044351, 1.977753308040909319 ) ) ;
#13877=CARTESIAN_POINT ( 'NONE',  ( 66.11068853694165171, 215.6427522451419065, 10.00000000000009415 ) ) ;
#13882=CARTESIAN_POINT ( 'NONE',  ( 190.8623743139412454, 300.0636657654615647, 8.577953960666059530 ) ) ;
#13883=CARTESIAN_POINT ( 'NONE',  ( 164.0776496603550925, 246.4561697322156419, 8.566708626497000267 ) ) ;
#13884=CARTESIAN_POINT ( 'NONE',  ( 151.3542526322075901, 269.2885850756041464, -14.28695254860580199 ) ) ;
#13886=CARTESIAN_POINT ( 'NONE',  ( 194.0943399085664396, 271.0983644945322339, -13.64356464264049507 ) ) ;
#13889=EDGE_CURVE ( 'NONE', #705, #37697, #36144, .T. ) ;
#13894=CYLINDRICAL_SURFACE ( 'NONE', #66760, 10.00000000000010658 ) ;
#13895=CARTESIAN_POINT ( 'NONE',  ( 20.97457486420976380, 194.4637435831424739, 2.679491924311251605 ) ) ;
#13896=CARTESIAN_POINT ( 'NONE',  ( 89.42916389074625272, 233.9860189848785694, -2.679491924311252493 ) ) ;
#13897=CARTESIAN_POINT ( 'NONE',  ( 149.0710170770012724, 245.3262482093457777, 3.021315404115420679E-15 ) ) ;
#13898=CARTESIAN_POINT ( 'NONE',  ( 201.1060504099706350, 282.3210983108598384, -18.18000168485860257 ) ) ;
#13901=CARTESIAN_POINT ( 'NONE',  ( 192.0527661830250565, 287.4924844977863359, -16.47094169987085266 ) ) ;
#13902=VERTEX_POINT ( 'NONE', #63826 ) ;
#13903=CARTESIAN_POINT ( 'NONE',  ( 190.8072577185990610, 300.1591305089344814, 3.698484652594827171 ) ) ;
#13905=CARTESIAN_POINT ( 'NONE',  ( 189.2141853381722001, 297.1461156523275235, 8.137912133790496938 ) ) ;
#13906=VERTEX_POINT ( 'NONE', #6285 ) ;
#13910=CARTESIAN_POINT ( 'NONE',  ( 176.6943099527350682, 256.7931168052207340, -11.17617521364210731 ) ) ;
#13912=CARTESIAN_POINT ( 'NONE',  ( 204.7986527064648214, 275.9253235211867263, 14.74587861556245905 ) ) ;
#13914=CARTESIAN_POINT ( 'NONE',  ( 56.45811372747556334, 196.7365022471902023, -10.00000000000009237 ) ) ;
#13915=ORIENTED_EDGE ( 'NONE', *, *, #81117, .T. ) ;
#13916=CARTESIAN_POINT ( 'NONE',  ( 98.14495447654879001, 215.2202760586659167, -5.415160957724236172E-17 ) ) ;
#13917=CARTESIAN_POINT ( 'NONE',  ( 155.0965287368403835, 262.0119274806629051, 17.25554003307136597 ) ) ;
#13919=CARTESIAN_POINT ( 'NONE',  ( 177.8829175822941693, 268.9868278392930847, -16.69667492248571250 ) ) ;
#13921=ORIENTED_EDGE ( 'NONE', *, *, #67570, .T. ) ;
#13924=ORIENTED_EDGE ( 'NONE', *, *, #76177, .F. ) ;
#13926=ORIENTED_EDGE ( 'NONE', *, *, #41427, .T. ) ;
#13928=ORIENTED_EDGE ( 'NONE', *, *, #96808, .T. ) ;
#13930=EDGE_LOOP ( 'NONE', ( #85636, #48558, #61291, #64500 ) ) ;
#13934=CARTESIAN_POINT ( 'NONE',  ( 165.0963524469224808, 264.4083487871739067, -17.41401503043321952 ) ) ;
#13940=CARTESIAN_POINT ( 'NONE',  ( 164.0935187385000802, 281.7221265701088555, 8.691696607283486031 ) ) ;
#13941=CARTESIAN_POINT ( 'NONE',  ( 183.5953950971229744, 289.9057545191589043, -13.74357891376704544 ) ) ;
#13944=CARTESIAN_POINT ( 'NONE',  ( 163.3706531435203146, 247.6807236201477735, 10.06957846017757241 ) ) ;
#13945=CARTESIAN_POINT ( 'NONE',  ( 188.2597630871935905, 260.7361237437183377, 2.610217646800272906 ) ) ;
#13946=CARTESIAN_POINT ( 'NONE',  ( 160.2954372498352598, 280.8823328917059712, -6.618626993187716856 ) ) ;
#13950=CARTESIAN_POINT ( 'NONE',  ( 161.1990332043106946, 251.4420796895884394, 14.26998817770995487 ) ) ;
#13951=CARTESIAN_POINT ( 'NONE',  ( 159.2007417150840922, 281.7182816310744329, 2.076871834512827864 ) ) ;
#13953=CARTESIAN_POINT ( 'NONE',  ( 194.5735419582797192, 293.6357348500615103, -15.26985155323035137 ) ) ;
#13954=EDGE_CURVE ( 'NONE', #31220, #57520, #51057, .T. ) ;
#13956=CARTESIAN_POINT ( 'NONE',  ( 160.5931239613893524, 275.7977860495605000, 12.74539326669525252 ) ) ;
#13957=CARTESIAN_POINT ( 'NONE',  ( -3.099174982164758951, 179.0177522451419350, 5.000000000000046185 ) ) ;
#13959=CARTESIAN_POINT ( 'NONE',  ( 192.7698958495311388, 267.0084935405105853, -11.19755117076729256 ) ) ;
#13960=EDGE_CURVE ( 'NONE', #79412, #51044, #74931, .T. ) ;
#13961=CARTESIAN_POINT ( 'NONE',  ( 171.5105039590924321, 279.6811076753780867, -14.64826990109219551 ) ) ;
#13962=CARTESIAN_POINT ( 'NONE',  ( 163.4609802778453513, 247.5242724341946712, -7.586713275286927072 ) ) ;
#13963=CARTESIAN_POINT ( 'NONE',  ( 169.6860864027741798, 284.9274174890383620, -11.04576083116783103 ) ) ;
#13965=CARTESIAN_POINT ( 'NONE',  ( -10.21716836350912949, 177.1589784336661637, -6.496448406907675876E-16 ) ) ;
#13967=CARTESIAN_POINT ( 'NONE',  ( 27.98206807853016542, 175.4155109091896065, 2.679491924311254714 ) ) ;
#13974=CARTESIAN_POINT ( 'NONE',  ( 171.6461529521897944, 289.6503080272315174, 2.692092882840170454 ) ) ;
#13976=CARTESIAN_POINT ( 'NONE',  ( -22.42236680055709641, 157.8615022471902591, 0.000000000000000000 ) ) ;
#13977=CARTESIAN_POINT ( 'NONE',  ( 202.0120093381390802, 280.7519314177017691, -17.07120787497099101 ) ) ;
#13979=CARTESIAN_POINT ( 'NONE',  ( 150.1232578106812241, 276.5731483457047943, 3.538916378592138923 ) ) ;
#13980=CARTESIAN_POINT ( 'NONE',  ( 9.836819166815537585, 185.6744531367911293, 4.594050593750047540 ) ) ;
#13981=CARTESIAN_POINT ( 'NONE',  ( 119.3079296378835181, 245.8149278399160949, -9.188101187500095079 ) ) ;
#13983=CARTESIAN_POINT ( 'NONE',  ( 183.2725204446199143, 257.5467570156531565, -3.032576513086016057 ) ) ;
#13985=CARTESIAN_POINT ( 'NONE',  ( 178.4067385319158632, 283.6684656904566282, -14.65910435069753781 ) ) ;
#13988=CARTESIAN_POINT ( 'NONE',  ( 161.8150574665248200, 250.3750943687383881, -13.25074899737357903 ) ) ;
#13989=CARTESIAN_POINT ( 'NONE',  ( 189.7272758596897972, 284.7347432595483383, 17.38904331496314271 ) ) ;
#13991=CARTESIAN_POINT ( 'NONE',  ( 186.8003541658358984, 299.2222177555264011, -0.6103433986344138917 ) ) ;
#13992=FACE_OUTER_BOUND ( 'NONE', #57411, .T. ) ;
#13993=CARTESIAN_POINT ( 'NONE',  ( 164.2659629401757968, 252.9733372042652491, -12.96157098613237046 ) ) ;
#13995=CARTESIAN_POINT ( 'NONE',  ( 181.7546150825112932, 268.0742755205600361, 15.00729537999377072 ) ) ;
#13997=CARTESIAN_POINT ( 'NONE',  ( 97.11602866590727956, 233.0024278399160664, 9.188101187500095079 ) ) ;
#13999=CARTESIAN_POINT ( 'NONE',  ( 190.7851751463332164, 300.1973786460605425, 8.237717828100052486 ) ) ;
#14000=CARTESIAN_POINT ( 'NONE',  ( 158.9391986220684885, 259.2430622464574981, -17.23821710380677530 ) ) ;
#14003=CARTESIAN_POINT ( 'NONE',  ( 203.2640693213759846, 272.1719133495528240, -9.742646638232304923 ) ) ;
#14004=CARTESIAN_POINT ( 'NONE',  ( 198.5954523381739989, 286.6695817285962562, -18.45134152028667174 ) ) ;
#14006=AXIS2_PLACEMENT_3D ( 'NONE', #23254, #91703, #100285 ) ;
#14008=CARTESIAN_POINT ( 'NONE',  ( 192.6170194583582429, 297.0245312260774995, -11.90166228306590490 ) ) ;
#14009=CARTESIAN_POINT ( 'NONE',  ( 203.3286960320409094, 267.8359400968079171, 2.569349860321338941 ) ) ;
#14013=VECTOR ( 'NONE', #81523, 1000.000000000000000 ) ;
#14014=CARTESIAN_POINT ( 'NONE',  ( 192.4212750754384160, 297.3635704425909125, -12.73704185013552248 ) ) ;
#14015=CARTESIAN_POINT ( 'NONE',  ( 196.7130436017243653, 289.9300093007386749, -16.33278734947153765 ) ) ;
#14016=AXIS2_PLACEMENT_3D ( 'NONE', #44816, #75752, #6336 ) ;
#14020=CARTESIAN_POINT ( 'NONE',  ( 172.9891656436891196, 253.8445998218816726, -8.983167006877987859 ) ) ;
#14021=CARTESIAN_POINT ( 'NONE',  ( 142.0502911348376358, 239.4865022471901455, 1.119607411625061291E-15 ) ) ;
#14027=CARTESIAN_POINT ( 'NONE',  ( 181.4130213927826389, 290.9717498374031379, -11.17998538662018326 ) ) ;
#14031=CARTESIAN_POINT ( 'NONE',  ( 158.7260964210017562, 256.4256569865397637, 16.36035822569746756 ) ) ;
#14032=CARTESIAN_POINT ( 'NONE',  ( 190.7223573502357681, 278.9099053379666771, -16.52215294300326320 ) ) ;
#14033=CARTESIAN_POINT ( 'NONE',  ( 153.7548618668677705, 264.3357626662872235, -16.52670224644400676 ) ) ;
#14034=CARTESIAN_POINT ( 'NONE',  ( 200.6680263064462792, 283.0797783131037022, -17.21821073473145347 ) ) ;
#14038=CARTESIAN_POINT ( 'NONE',  ( 148.6829486123639015, 276.4333369876038091, 4.903683765799150329 ) ) ;
#14040=ADVANCED_FACE ( 'NONE', ( #2036 ), #72057, .F. ) ;
#14046=CARTESIAN_POINT ( 'NONE',  ( 198.0693404800861970, 286.9154998458281511, 16.94403134481562390 ) ) ;
#14048=CARTESIAN_POINT ( 'NONE',  ( 204.8762144138505903, 275.7909827032724479, 14.60855957933206817 ) ) ;
#14049=CARTESIAN_POINT ( 'NONE',  ( 194.1852025340051284, 294.3083584634874796, -15.46421316575964688 ) ) ;
#14050=CARTESIAN_POINT ( 'NONE',  ( 164.5696622524448287, 245.6039789247527096, -0.9250471598561700315 ) ) ;
#14053=CARTESIAN_POINT ( 'NONE',  ( 147.6140518775699491, 274.9719575673779559, 8.457032797753797126 ) ) ;
#14054=CARTESIAN_POINT ( 'NONE',  ( 170.1618648994021896, 287.2524135899183193, -4.625886296424732258 ) ) ;
#14056=CARTESIAN_POINT ( 'NONE',  ( 184.3726654517722068, 285.2721521148185957, -15.05498701587415411 ) ) ;
#14057=CARTESIAN_POINT ( 'NONE',  ( 107.1835739849013578, 238.8149278399160664, 9.188101187500093303 ) ) ;
#14059=CARTESIAN_POINT ( 'NONE',  ( 148.0905168928549074, 274.5273101863830334, -6.357871172357103973 ) ) ;
#14061=CARTESIAN_POINT ( 'NONE',  ( 191.9783149651901510, 275.2774038663249598, 16.54544651655929144 ) ) ;
#14062=ORIENTED_EDGE ( 'NONE', *, *, #38471, .T. ) ;
#14063=CARTESIAN_POINT ( 'NONE',  ( 163.8579349293242444, 248.3789907627131583, -9.588306200948446545 ) ) ;
#14065=CARTESIAN_POINT ( 'NONE',  ( 196.0034224882197975, 291.1591091234520263, 17.53794140922627776 ) ) ;
#14066=CARTESIAN_POINT ( 'NONE',  ( 206.7893622945242385, 272.4773133715531230, -10.52881283832460291 ) ) ;
#14069=CARTESIAN_POINT ( 'NONE',  ( 148.5256826847395359, 273.3929666916147312, 8.949121270729929023 ) ) ;
#14073=ORIENTED_EDGE ( 'NONE', *, *, #87329, .T. ) ;
#14076=CARTESIAN_POINT ( 'NONE',  ( 157.4345159935474783, 262.7946473092207498, 17.12007574691928369 ) ) ;
#14078=DIRECTION ( 'NONE',  ( 0.4999999999999992784, -0.8660254037844390407, 0.000000000000000000 ) ) ;
#14079=CARTESIAN_POINT ( 'NONE',  ( -22.42236680055709641, 157.8615022471902591, 0.000000000000000000 ) ) ;
#14081=CARTESIAN_POINT ( 'NONE',  ( 162.6991225460172927, 284.8212170328912975, -3.897741803361528756 ) ) ;
#14084=CARTESIAN_POINT ( 'NONE',  ( 190.1752790837055045, 301.2537496138681945, -5.177773110520776711 ) ) ;
#14085=CARTESIAN_POINT ( 'NONE',  ( 63.33450210234187239, 195.8262482093458061, 3.021315404115420679E-15 ) ) ;
#14087=EDGE_CURVE ( 'NONE', #39984, #18565, #33629, .T. ) ;
#14088=CARTESIAN_POINT ( 'NONE',  ( 170.1900998099124251, 249.2102026740786300, -0.2624473253846250076 ) ) ;
#14089=CARTESIAN_POINT ( 'NONE',  ( 189.0595448167310906, 269.8736603083619912, -13.99715981437423906 ) ) ;
#14092=CARTESIAN_POINT ( 'NONE',  ( 50.45802072044652675, 211.4860189848785410, -2.679491924311252493 ) ) ;
#14093=AXIS2_PLACEMENT_3D ( 'NONE', #32272, #31756, #23659 ) ;
#14097=CARTESIAN_POINT ( 'NONE',  ( 72.92127039979699532, 225.1589784336661637, -6.496448406907675876E-16 ) ) ;
#14098=CARTESIAN_POINT ( 'NONE',  ( 206.2809287719926488, 273.3579460648492159, -10.70911012174624588 ) ) ;
#14100=CARTESIAN_POINT ( 'NONE',  ( 163.4218292706009095, 247.5920839679097014, -10.44611490715852042 ) ) ;
#14101=B_SPLINE_CURVE_WITH_KNOTS ( 'NONE', 3,
 ( #33922, #40486, #32400, #72430, #18711, #71416, #71917, #70912, #86659, #39977, #48611, #63799, #32892, #56181, #94733, #80042 ),
 .UNSPECIFIED., .F., .F.,
 ( 4, 2, 2, 2, 2, 2, 2, 4 ),
 ( 7.775354953989597285E-17, 0.0003787177898469638068, 0.0007574355796938498763, 0.001136153369540736108, 0.001514871159387622124, 0.001893588949234508139, 0.002272306739081394154, 0.003029742318775003988 ),
 .UNSPECIFIED. ) ;
#14103=CARTESIAN_POINT ( 'NONE',  ( 207.1285138014047504, 271.8898857301724661, -5.752177443817618752 ) ) ;
#14104=CARTESIAN_POINT ( 'NONE',  ( 154.6982851380984130, 273.6571292083216349, -13.42362762759460892 ) ) ;
#14113=CARTESIAN_POINT ( 'NONE',  ( 25.42527643493543366, 194.6744531367911293, 4.594050593750047540 ) ) ;
#14116=CARTESIAN_POINT ( 'NONE',  ( 196.3720681610792553, 290.5205960880691691, 16.18360420724715354 ) ) ;
#14120=CARTESIAN_POINT ( 'NONE',  ( 49.15987193134397160, 205.3149278399160949, -9.188101187500095079 ) ) ;
#14122=CARTESIAN_POINT ( 'NONE',  ( 171.4108310039837875, 286.6584375100259763, 7.439453781534334453 ) ) ;
#14123=CARTESIAN_POINT ( 'NONE',  ( 197.0313051377892748, 289.3787641501790517, -17.15509075150697882 ) ) ;
#14126=CARTESIAN_POINT ( 'NONE',  ( 182.0814719340378645, 255.7199348603173519, -3.369638453849108206 ) ) ;
#14127=CARTESIAN_POINT ( 'NONE',  ( 175.8186258879950685, 291.0967586842824630, 2.548988351986237522 ) ) ;
#14128=CARTESIAN_POINT ( 'NONE',  ( 176.1090663942078436, 274.8498405251406780, 17.00816766817632342 ) ) ;
#14132=CARTESIAN_POINT ( 'NONE',  ( 96.15094473426229627, 232.9865022471902876, 10.00000000000009237 ) ) ;
#14133=CARTESIAN_POINT ( 'NONE',  ( 200.2631011806900005, 283.7811292041749311, 18.23377125296567058 ) ) ;
#14134=CARTESIAN_POINT ( 'NONE',  ( 165.2613035890315132, 269.7019032284875379, -16.28361342814668689 ) ) ;
#14136=CARTESIAN_POINT ( 'NONE',  ( 68.13167480270307408, 200.9548013555409796, -4.594050593750042211 ) ) ;
#14138=CARTESIAN_POINT ( 'NONE',  ( 166.0424944338363105, 265.3088416721781755, 16.55799481498140224 ) ) ;
#14139=CARTESIAN_POINT ( 'NONE',  ( 161.9111943820872170, 250.8713438377554326, 12.61905948367559027 ) ) ;
#14142=CARTESIAN_POINT ( 'NONE',  ( 174.0424481033923314, 287.4814580433055653, 10.99910921803667208 ) ) ;
#14144=CARTESIAN_POINT ( 'NONE',  ( 178.6782777294722848, 260.6412425082613709, 13.57969907341511551 ) ) ;
#14148=CARTESIAN_POINT ( 'NONE',  ( 157.4729130248890954, 257.8959091554543761, 17.83439074639795052 ) ) ;
#14150=AXIS2_PLACEMENT_3D ( 'NONE', #66125, #43310, #89484 ) ;
#14152=CARTESIAN_POINT ( 'NONE',  ( 175.3483744890668277, 254.4581768569554185, 7.871548991938851714 ) ) ;
#14153=CARTESIAN_POINT ( 'NONE',  ( 170.3198432486256024, 250.1987702182942996, -6.980229573997380754 ) ) ;
#14154=ORIENTED_EDGE ( 'NONE', *, *, #3400, .F. ) ;
#14155=CARTESIAN_POINT ( 'NONE',  ( 183.8570876466514790, 294.7988146780254510, 8.885945338395226045 ) ) ;
#14156=ADVANCED_FACE ( 'NONE', ( #84559 ), #33210, .F. ) ;
#14157=CARTESIAN_POINT ( 'NONE',  ( 206.3454060440500086, 273.2462681537123785, -9.268083217908118954 ) ) ;
#14160=EDGE_LOOP ( 'NONE', ( #30952, #7186, #92331, #79641 ) ) ;
#14161=AXIS2_PLACEMENT_3D ( 'NONE', #36632, #97481, #74177 ) ;
#14163=CARTESIAN_POINT ( 'NONE',  ( -22.42236680055709641, 157.8615022471902591, 0.000000000000000000 ) ) ;
#14165=CARTESIAN_POINT ( 'NONE',  ( 204.8189571845487080, 275.8901551335242175, 13.43702398685204358 ) ) ;
#14166=EDGE_CURVE ( 'NONE', #39829, #41328, #79957, .T. ) ;
#14167=CARTESIAN_POINT ( 'NONE',  ( 198.6755293322981117, 286.5308843062557571, 17.86676876308990103 ) ) ;
#14169=DIRECTION ( 'NONE',  ( 0.4999999999999992784, -0.8660254037844390407, 0.000000000000000000 ) ) ;
#14171=CARTESIAN_POINT ( 'NONE',  ( 134.5180214354952284, 236.2202760586659736, -5.415160957724236172E-17 ) ) ;
#14172=CARTESIAN_POINT ( 'NONE',  ( 159.8882960419693120, 255.1631675222682532, -16.13735980308360496 ) ) ;
#14173=CARTESIAN_POINT ( 'NONE',  ( 180.0191955535601949, 258.0046308849226762, 10.27888219584907858 ) ) ;
#14174=CARTESIAN_POINT ( 'NONE',  ( 64.07166007881600933, 216.9869531367911293, 4.594050593750046652 ) ) ;
#14175=VERTEX_POINT ( 'NONE', #12025 ) ;
#14176=CARTESIAN_POINT ( 'NONE',  ( 170.2148871637432705, 264.0733095026099022, 16.11244079653449646 ) ) ;
#14177=CARTESIAN_POINT ( 'NONE',  ( 165.5046005952566475, 282.3973782299070763, -11.17475345190591973 ) ) ;
#14178=ORIENTED_EDGE ( 'NONE', *, *, #41565, .F. ) ;
#14181=ORIENTED_EDGE ( 'NONE', *, *, #34705, .T. ) ;
#14186=CARTESIAN_POINT ( 'NONE',  ( 194.2232752567778675, 284.7421936660649067, 17.38045846422785345 ) ) ;
#14189=CARTESIAN_POINT ( 'NONE',  ( 155.0929244053699847, 262.0181703658971628, 18.51426604808664678 ) ) ;
#14194=CARTESIAN_POINT ( 'NONE',  ( 201.1075649649426111, 282.3184750246975909, -17.62722514768381998 ) ) ;
#14196=CARTESIAN_POINT ( 'NONE',  ( 163.8938939028770392, 260.7256311026002891, -16.27231015239807732 ) ) ;
#14197=CARTESIAN_POINT ( 'NONE',  ( 174.5211454378950009, 254.1122819737915393, -7.432909296658919196 ) ) ;
#14198=CARTESIAN_POINT ( 'NONE',  ( 191.0504085702373800, 299.7379808799933016, 6.468263574011999140 ) ) ;
#14199=CARTESIAN_POINT ( 'NONE',  ( 164.7462163020046262, 245.2981783406326599, 1.451255823150352064 ) ) ;
#14200=CARTESIAN_POINT ( 'NONE',  ( 36.44700672854521883, 203.3967562850347122, 1.101618078115930403E-13 ) ) ;
#14202=CARTESIAN_POINT ( 'NONE',  ( 137.6570164284488271, 250.2833772461660544, -9.188101187500095079 ) ) ;
#14204=CARTESIAN_POINT ( 'NONE',  ( 185.1790142135946837, 260.5378326486920741, -9.806357480331048038 ) ) ;
#14205=CARTESIAN_POINT ( 'NONE',  ( 182.2071301927472575, 257.5162533253280230, 6.694102600255701141 ) ) ;
#14210=CARTESIAN_POINT ( 'NONE',  ( 199.6670208576438768, 266.3510233136422016, 4.737243403722396273 ) ) ;
#14215=CARTESIAN_POINT ( 'NONE',  ( 198.2014190056785310, 266.0765624434006327, 0.8202294858332698224 ) ) ;
#14221=EDGE_CURVE ( 'NONE', #42087, #98884, #54908, .T. ) ;
#14223=CARTESIAN_POINT ( 'NONE',  ( 207.6628070930962906, 270.9644626028195376, 7.378217122120054761 ) ) ;
#14224=CARTESIAN_POINT ( 'NONE',  ( 167.2515702596184042, 262.0622343731731689, -17.21809106051008342 ) ) ;
#14225=B_SPLINE_SURFACE_WITH_KNOTS ( 'NONE', 3, 1, ( 
 ( #14554, #59629 ),
 ( #45429, #92100 ),
 ( #5948, #98171 ),
 ( #21651, #67750 ),
 ( #30747, #30242 ),
 ( #22645, #15023 ),
 ( #98674, #38324 ),
 ( #45914, #52534 ),
 ( #7431, #100161 ),
 ( #83484, #43933 ),
 ( #74872, #14050 ),
 ( #44928, #31712 ),
 ( #24139, #25128 ),
 ( #17027, #94078 ),
 ( #84971, #56010 ),
 ( #46418, #55024 ),
 ( #63133, #16531 ),
 ( #15516, #1346 ),
 ( #87006, #38823 ),
 ( #8937, #46936 ),
 ( #62113, #79387 ),
 ( #24631, #95087 ),
 ( #62617, #86005 ),
 ( #70735, #2354 ),
 ( #16035, #94572 ),
 ( #39803, #32232 ),
 ( #47428, #33233 ),
 ( #70227, #8441 ),
 ( #93570, #64137 ),
 ( #55511, #78355 ),
 ( #86499, #47920 ),
 ( #31227, #63635 ),
 ( #17533, #78859 ),
 ( #7950, #25650 ) ),
 .UNSPECIFIED., .T., .F., .F.,
 ( 4, 2, 2, 2, 2, 2, 2, 2, 2, 2, 2, 2, 2, 2, 2, 2, 4 ),
 ( 2, 2 ),
 ( 0.000000000000000000, 0.06250000000000000000, 0.1250000000000000000, 0.1875000000000000000, 0.2500000000000000000, 0.3125000000000000000, 0.3750000000000000000, 0.4375000000000000000, 0.5000000000000000000, 0.5625000000000000000, 0.6250000000000000000, 0.6875000000000000000, 0.7500000000000000000, 0.8125000000000000000, 0.8750000000000000000, 0.9375000000000000000, 1.000000000000000000 ),
 ( 0.000000000000000000, 1.000000000000000000 ),
 .UNSPECIFIED. ) ;
#14228=CARTESIAN_POINT ( 'NONE',  ( 204.9751544352041890, 274.4268820053481477, 11.86595640911393268 ) ) ;
#14230=CARTESIAN_POINT ( 'NONE',  ( 159.7608930362198407, 253.9330115291272421, 15.38895778945778581 ) ) ;
#14232=CARTESIAN_POINT ( 'NONE',  ( 139.7950166422676261, 261.5177522451418781, 5.000000000000046185 ) ) ;
#14233=CARTESIAN_POINT ( 'NONE',  ( 182.5998193346738390, 278.6774981096693864, 17.57078003122366283 ) ) ;
#14234=VERTEX_POINT ( 'NONE', #3916 ) ;
#14236=CARTESIAN_POINT ( 'NONE',  ( 178.0923676029798344, 255.8199948319143573, 8.866499536866403020 ) ) ;
#14238=CARTESIAN_POINT ( 'NONE',  ( 150.7850480413316632, 269.4796311011364764, -14.43114374163211089 ) ) ;
#14239=CARTESIAN_POINT ( 'NONE',  ( 3.882894515797516988, 182.2369531367911009, -4.594050593750048428 ) ) ;
#14242=CARTESIAN_POINT ( 'NONE',  ( 157.7593757092099906, 257.3997412317380054, -18.08445832352326121 ) ) ;
#14244=CARTESIAN_POINT ( 'NONE',  ( 122.1835217032046330, 252.8967562850346553, -4.648177544792955347E-16 ) ) ;
#14247=CARTESIAN_POINT ( 'NONE',  ( 151.0438343122359584, 269.0314001316289705, 14.41873139571475626 ) ) ;
#14248=CARTESIAN_POINT ( 'NONE',  ( 43.46773267070889091, 209.2365022471903444, 2.944929066748280225E-16 ) ) ;
#14251=CARTESIAN_POINT ( 'NONE',  ( 190.5154909595809727, 300.6644853595138329, -0.04129855346138300298 ) ) ;
#14252=CARTESIAN_POINT ( 'NONE',  ( 5.371288904610766579, 186.1589784336661637, -6.496448406907675876E-16 ) ) ;
#14254=CARTESIAN_POINT ( 'NONE',  ( 192.7693357657653053, 296.7607116428271183, 12.22606306887835714 ) ) ;
#14256=CARTESIAN_POINT ( 'NONE',  ( 142.4652616372697480, 246.3927522451418497, 10.00000000000009948 ) ) ;
#14257=CARTESIAN_POINT ( 'NONE',  ( 207.3502731283117555, 271.5057873089173768, 6.280625384230454245 ) ) ;
#14258=CARTESIAN_POINT ( 'NONE',  ( 189.1359039112073503, 268.2262726479567618, 13.76342687570769030 ) ) ;
#14259=CARTESIAN_POINT ( 'NONE',  ( 164.1724755390579276, 281.5534210847879422, 9.615559972177582182 ) ) ;
#14263=CARTESIAN_POINT ( 'NONE',  ( 193.9204722154232741, 294.7668848255750049, 15.43855698596013859 ) ) ;
#14265=CARTESIAN_POINT ( 'NONE',  ( 181.5930883117324868, 289.4714290587421033, 12.79629105351733109 ) ) ;
#14273=CARTESIAN_POINT ( 'NONE',  ( 155.0453531195792038, 262.1005662498678817, -18.46987289964740953 ) ) ;
#14274=ORIENTED_EDGE ( 'NONE', *, *, #92811, .F. ) ;
#14276=CARTESIAN_POINT ( 'NONE',  ( 202.4683350698883544, 279.2420349807568414, 15.54043181306517774 ) ) ;
#14277=CARTESIAN_POINT ( 'NONE',  ( 151.8574524980327567, 274.5526676221680873, 11.13270052181353975 ) ) ;
#14278=ORIENTED_EDGE ( 'NONE', *, *, #73528, .T. ) ;
#14279=CARTESIAN_POINT ( 'NONE',  ( 201.2139346379346705, 282.1342373466909521, -16.65315141107179286 ) ) ;
#14283=CARTESIAN_POINT ( 'NONE',  ( 45.37789370152431445, 208.5530062829863027, -4.648177544792955347E-16 ) ) ;
#14289=CARTESIAN_POINT ( 'NONE',  ( 149.4171629335945681, 271.8488776066536730, -11.42564036194071520 ) ) ;
#14292=CARTESIAN_POINT ( 'NONE',  ( 164.9356397357043704, 244.9700873293209042, 2.799217332519396972 ) ) ;
#14294=CARTESIAN_POINT ( 'NONE',  ( 53.17212233558426959, 213.0530062829863311, -4.648177544792955347E-16 ) ) ;
#14295=VERTEX_POINT ( 'NONE', #97156 ) ;
#14296=CARTESIAN_POINT ( 'NONE',  ( 149.6877696051026305, 271.3801731027346591, 11.89134584187677390 ) ) ;
#14305=CARTESIAN_POINT ( 'NONE',  ( 156.0580231375089681, 266.2288738017929290, -16.26249046113716545 ) ) ;
#14307=CARTESIAN_POINT ( 'NONE',  ( 148.3519871123208986, 273.6938162480936398, 8.180046468253793890 ) ) ;
#14308=CARTESIAN_POINT ( 'NONE',  ( 190.6893905452545823, 300.3632824417117604, 3.294993852933539191 ) ) ;
#14309=CARTESIAN_POINT ( 'NONE',  ( 152.8522706834672533, 265.8990964544007056, 17.63080661522264947 ) ) ;
#14310=CARTESIAN_POINT ( 'NONE',  ( 191.1855251068263328, 299.5039521736787265, 8.464810282331489688 ) ) ;
#14311=CARTESIAN_POINT ( 'NONE',  ( 191.3610003135137276, 299.2000202002271294, -9.855749861282104618 ) ) ;
#14313=CARTESIAN_POINT ( 'NONE',  ( 163.5175435169129798, 257.7444940288048087, 15.51854699187649089 ) ) ;
#14315=CARTESIAN_POINT ( 'NONE',  ( 96.22311351791105949, 216.3615022471902023, 5.000000000000051514 ) ) ;
#14317=CARTESIAN_POINT ( 'NONE',  ( 170.3267854104257992, 288.9614774289731827, 4.405198534815358613 ) ) ;
#14318=CARTESIAN_POINT ( 'NONE',  ( 178.2382707639212356, 285.7843550335422833, 14.43266090959460435 ) ) ;
#14319=CARTESIAN_POINT ( 'NONE',  ( 98.84807947347611901, 234.0024278399160664, -9.188101187500093303 ) ) ;
#14320=ORIENTED_EDGE ( 'NONE', *, *, #66712, .F. ) ;
#14321=CARTESIAN_POINT ( 'NONE',  ( 190.0509677963674164, 301.4690630794920594, -3.786306570772668412 ) ) ;
#14325=CARTESIAN_POINT ( 'NONE',  ( 191.6458595453738099, 297.4183736063205288, -10.67255559255732855 ) ) ;
#14326=CARTESIAN_POINT ( 'NONE',  ( 190.3911359119452413, 288.4005044049387720, 16.54395277729882707 ) ) ;
#14329=CARTESIAN_POINT ( 'NONE',  ( 167.8408648507877956, 253.6332239154487240, -11.89335889730976348 ) ) ;
#14330=CARTESIAN_POINT ( 'NONE',  ( 159.2122473525774069, 254.8832937285494609, -16.22689353966294590 ) ) ;
#14333=CARTESIAN_POINT ( 'NONE',  ( 49.65620586503739986, 186.1427522451417644, 1.119607411625061291E-15 ) ) ;
#14334=CARTESIAN_POINT ( 'NONE',  ( 116.0067284296028589, 225.5327760586659451, 1.948934522072302763E-15 ) ) ;
#14337=CARTESIAN_POINT ( 'NONE',  ( 157.0848929289108469, 258.5679796760466047, 17.57466231005294688 ) ) ;
#14338=CARTESIAN_POINT ( 'NONE',  ( 172.2319936421038449, 250.7099816150368383, -4.070406209060837277 ) ) ;
#14339=CARTESIAN_POINT ( 'NONE',  ( 34.43744006700849525, 196.8149278399160664, 9.188101187500093303 ) ) ;
#14341=EDGE_CURVE ( 'NONE', #43956, #4734, #43953, .T. ) ;
#14344=CARTESIAN_POINT ( 'NONE',  ( 201.5036534377215958, 270.3153034880852488, -10.25451236307256409 ) ) ;
#14345=CARTESIAN_POINT ( 'NONE',  ( 181.8197068046096661, 267.0272984663218949, 15.22864918630029329 ) ) ;
#14347=CARTESIAN_POINT ( 'NONE',  ( 147.0538900202505488, 275.9421863647172017, 5.192507380313251986 ) ) ;
#14351=CARTESIAN_POINT ( 'NONE',  ( 164.1573714183803361, 250.0513545240398230, 10.30907450286302840 ) ) ;
#14352=CARTESIAN_POINT ( 'NONE',  ( 109.4841275098123248, 234.0177522451418781, -10.00000000000009592 ) ) ;
#14358=CARTESIAN_POINT ( 'NONE',  ( 155.0438369506338177, 280.3867491788369080, -2.458805040944644915 ) ) ;
#14359=CARTESIAN_POINT ( 'NONE',  ( 153.9680911965096470, 265.0746596462684579, 16.74034374412752513 ) ) ;
#14360=CARTESIAN_POINT ( 'NONE',  ( 13.11156449881669595, 184.5024278399160949, -9.188101187500093303 ) ) ;
#14361=AXIS2_PLACEMENT_3D ( 'NONE', #38804, #53993, #78332 ) ;
#14363=CARTESIAN_POINT ( 'NONE',  ( 196.1978789692381895, 273.6107559518669632, 15.03886906253136146 ) ) ;
#14364=CARTESIAN_POINT ( 'NONE',  ( 146.9422184197532317, 276.1356072505412840, -5.063317562214876943 ) ) ;
#14365=B_SPLINE_CURVE_WITH_KNOTS ( 'NONE', 3,
 ( #97590, #74790, #50954, #81905 ),
 .UNSPECIFIED., .F., .F.,
 ( 4, 4 ),
 ( 0.002278044366665053690, 0.01021365927721262952 ),
 .UNSPECIFIED. ) ;
#14367=CARTESIAN_POINT ( 'NONE',  ( 174.1634402936988977, 287.2696604785184036, 10.41966287398365232 ) ) ;
#14368=CARTESIAN_POINT ( 'NONE',  ( 70.62149783858335184, 202.3923013555409796, 4.594050593750050204 ) ) ;
#14369=CARTESIAN_POINT ( 'NONE',  ( 207.8302079587528794, 270.6745157982714431, 3.572475529330238153 ) ) ;
#14373=ORIENTED_EDGE ( 'NONE', *, *, #74681, .F. ) ;
#14375=( BOUNDED_CURVE ( )  B_SPLINE_CURVE ( 2, ( #59272, #19344, #43594, #27420, #90250, #36492, #3628, #34506, #65407 ),
 .UNSPECIFIED., .F., .T. ) 
 B_SPLINE_CURVE_WITH_KNOTS ( ( 3, 2, 2, 2, 3 ),
 ( 0.1088709677419354843, 0.1102150537634408595, 0.1129032258064516098, 0.1155913978494623601, 0.1169354838709677491 ),
 .UNSPECIFIED. ) 
 CURVE ( )  GEOMETRIC_REPRESENTATION_ITEM ( )  RATIONAL_B_SPLINE_CURVE ( ( 0.9330127018922194093, 0.9330127018922194093, 1.000000000000000000, 0.8660254037844387076, 1.000000000000000000, 0.8660254037844387076, 1.000000000000000000, 0.9330127018922189652, 0.9330127018922192983 ) ) 
 REPRESENTATION_ITEM ( '' )  );
#14376=CARTESIAN_POINT ( 'NONE',  ( 165.3951733978771017, 269.2638120270026434, 16.94313702576530289 ) ) ;
#14377=CARTESIAN_POINT ( 'NONE',  ( 7.094665711762471183, 188.2365022471903444, 2.944929066748280225E-16 ) ) ;
#14378=CARTESIAN_POINT ( 'NONE',  ( 164.4578252119609090, 245.7976863610386999, -6.211333091911165560 ) ) ;
#14379=CARTESIAN_POINT ( 'NONE',  ( 136.3579783227721691, 249.5333772461660544, 9.188101187500095079 ) ) ;
#14381=CARTESIAN_POINT ( 'NONE',  ( 164.6787707939755023, 245.4149973872815167, 0.8898042037103690571 ) ) ;
#14383=CARTESIAN_POINT ( 'NONE',  ( 198.6417698102810903, 282.3377161438529015, -17.61035883595712548 ) ) ;
#14385=CARTESIAN_POINT ( 'NONE',  ( 185.0625584367380156, 277.4576075603951608, -17.68842772276633823 ) ) ;
#14388=CARTESIAN_POINT ( 'NONE',  ( 156.9440562780969231, 274.4750137900673508, 13.77464823823377316 ) ) ;
#14389=CARTESIAN_POINT ( 'NONE',  ( -22.42236680055709641, 157.8615022471902591, 0.000000000000000000 ) ) ;
#14390=CARTESIAN_POINT ( 'NONE',  ( 189.2060028741113626, 262.3212090535250809, -9.063150766256741875 ) ) ;
#14391=CARTESIAN_POINT ( 'NONE',  ( 172.8981760910776586, 268.5351074533131168, -17.67640058404859360 ) ) ;
#14396=CARTESIAN_POINT ( 'NONE',  ( 171.0863495110653218, 284.1046068702937646, -11.19458109666653023 ) ) ;
#14398=EDGE_CURVE ( 'NONE', #38805, #35, #50678, .T. ) ;
#14399=CARTESIAN_POINT ( 'NONE',  ( 200.8877589446975094, 282.0066036887982364, -16.66018347811495204 ) ) ;
#14400=CARTESIAN_POINT ( 'NONE',  ( 192.0603001030472683, 293.3461588932823929, -14.68827779892621344 ) ) ;
#14401=CARTESIAN_POINT ( 'NONE',  ( 183.8037341582430884, 275.4624792557407318, 17.77592483611231700 ) ) ;
#14402=CARTESIAN_POINT ( 'NONE',  ( 163.2256942281324541, 247.9317998266098471, -9.780520296312531059 ) ) ;
#14404=ORIENTED_EDGE ( 'NONE', *, *, #49575, .F. ) ;
#14409=CARTESIAN_POINT ( 'NONE',  ( 190.7222376050763444, 300.3063896652212179, 3.365789908110941475 ) ) ;
#14413=CARTESIAN_POINT ( 'NONE',  ( 146.6647111637776106, 276.6162639173599587, -0.6373001129109082674 ) ) ;
#14416=CARTESIAN_POINT ( 'NONE',  ( 204.4781092559247782, 276.4805210635553863, 13.30606382016679490 ) ) ;
#14419=EDGE_LOOP ( 'NONE', ( #83204, #29267, #74619, #23546 ) ) ;
#14420=CARTESIAN_POINT ( 'NONE',  ( 96.62871582839601103, 238.8464784336661637, 1.353441290958777525E-15 ) ) ;
#14421=CARTESIAN_POINT ( 'NONE',  ( 203.0654848288144478, 278.9272583433232171, 16.42392292156888445 ) ) ;
#14422=CARTESIAN_POINT ( 'NONE',  ( 169.2345181364990765, 254.6337805363678228, -13.16056876093153427 ) ) ;
#14423=CARTESIAN_POINT ( 'NONE',  ( 178.2910397215446494, 269.1225465846854945, -17.06547196193329796 ) ) ;
#14425=VERTEX_POINT ( 'NONE', #99121 ) ;
#14426=ADVANCED_FACE ( 'NONE', ( #90049 ), #37786, .T. ) ;
#14430=ORIENTED_EDGE ( 'NONE', *, *, #45700, .F. ) ;
#14431=CARTESIAN_POINT ( 'NONE',  ( 159.1311797733062861, 257.0237068946943282, -17.13424826516079946 ) ) ;
#14432=ORIENTED_EDGE ( 'NONE', *, *, #1944, .T. ) ;
#14433=CARTESIAN_POINT ( 'NONE',  ( 164.2090401137261892, 246.2285947913476889, -5.787448100099915393 ) ) ;
#14435=CARTESIAN_POINT ( 'NONE',  ( 170.1297270883495969, 282.5512338199900455, 11.77438199859611956 ) ) ;
#14441=CARTESIAN_POINT ( 'NONE',  ( 201.5505397922970587, 279.0059902033771664, -15.80381168536360370 ) ) ;
#14444=CARTESIAN_POINT ( 'NONE',  ( 179.1458458498692039, 281.5336445223243800, 16.66751556302194359 ) ) ;
#14446=CARTESIAN_POINT ( 'NONE',  ( 202.7599932440484451, 279.4563852894229967, 15.58249343055423353 ) ) ;
#14447=CARTESIAN_POINT ( 'NONE',  ( 188.6122357780320442, 260.1364690911672142, 2.208924378594173010 ) ) ;
#14448=CARTESIAN_POINT ( 'NONE',  ( 161.3400561738205852, 281.5235411820722220, -6.446175152765177607 ) ) ;
#14451=CARTESIAN_POINT ( 'NONE',  ( 171.2679739083015988, 255.5491317200628885, 11.22258467113546310 ) ) ;
#14452=CARTESIAN_POINT ( 'NONE',  ( 157.3860572040868533, 282.0393593213248664, 1.488781532780958372 ) ) ;
#14454=ORIENTED_EDGE ( 'NONE', *, *, #21336, .F. ) ;
#14455=CARTESIAN_POINT ( 'NONE',  ( 181.8559704853444430, 270.4563004562098740, -16.38363252787888413 ) ) ;
#14458=CARTESIAN_POINT ( 'NONE',  ( 1.158783253108745637, 178.1427522451419065, 10.00000000000009237 ) ) ;
#14460=CARTESIAN_POINT ( 'NONE',  ( 201.5189872289815867, 266.7509884862435570, -2.318412474989284267 ) ) ;
#14461=CARTESIAN_POINT ( 'NONE',  ( 204.0543048838297864, 277.2145717684933857, -15.78942579435808824 ) ) ;
#14464=CARTESIAN_POINT ( 'NONE',  ( -6.590166341514275494, 160.8768266524160140, 9.188101187500098632 ) ) ;
#14465=CARTESIAN_POINT ( 'NONE',  ( 3.829028248110833754, 163.0177522451418213, 5.000000000000051514 ) ) ;
#14466=EDGE_CURVE ( 'NONE', #21, #89234, #10879, .T. ) ;
#14467=CARTESIAN_POINT ( 'NONE',  ( 25.55183212637049195, 178.8927522451418497, 10.00000000000009948 ) ) ;
#14469=ORIENTED_EDGE ( 'NONE', *, *, #26762, .T. ) ;
#14475=CARTESIAN_POINT ( 'NONE',  ( 162.8063655212930314, 248.6580984519274296, -10.21361106748447334 ) ) ;
#14477=CARTESIAN_POINT ( 'NONE',  ( 169.1417317201558319, 248.6322817555173401, 4.786625344359500822 ) ) ;
#14478=CARTESIAN_POINT ( 'NONE',  ( 27.99689677000926125, 174.7202760586659736, -5.415160957724236172E-17 ) ) ;
#14479=CARTESIAN_POINT ( 'NONE',  ( 115.6001716039901055, 246.7369531367911009, -4.594050593750048428 ) ) ;
#14480=CARTESIAN_POINT ( 'NONE',  ( 181.9266546068691639, 294.6628528558310336, -6.525654968116115562 ) ) ;
#14482=ADVANCED_FACE ( 'NONE', ( #76797 ), #82951, .T. ) ;
#14486=CARTESIAN_POINT ( 'NONE',  ( 67.98707691180798918, 203.3927522451417929, -10.00000000000009237 ) ) ;
#14487=CARTESIAN_POINT ( 'NONE',  ( 193.9204722154232741, 294.7668848255750049, 15.43855698596013859 ) ) ;
#14488=CARTESIAN_POINT ( 'NONE',  ( 184.0057710604646388, 275.0402031074996216, 16.36095971177830322 ) ) ;
#14489=CARTESIAN_POINT ( 'NONE',  ( 147.8505793332463725, 274.5622799967613332, -9.317516487097901035 ) ) ;
#14491=CARTESIAN_POINT ( 'NONE',  ( 167.7509841405270095, 278.2029002482612441, 14.51312790891695137 ) ) ;
#14492=CARTESIAN_POINT ( 'NONE',  ( -1.503503506619806140, 181.4860189848785694, -2.679491924311240503 ) ) ;
#14493=CARTESIAN_POINT ( 'NONE',  ( 191.1747001918821525, 299.5227014763493116, -9.654804683100723040 ) ) ;
#14494=CARTESIAN_POINT ( 'NONE',  ( 162.3216239674494261, 251.7437731844563871, -12.88187769518047610 ) ) ;
#14497=CARTESIAN_POINT ( 'NONE',  ( 185.0442626281781031, 269.6655662514531855, 15.59706165446737813 ) ) ;
#14498=CARTESIAN_POINT ( 'NONE',  ( 87.77910550741502504, 230.6744531367911293, 4.594050593750047540 ) ) ;
#14499=CARTESIAN_POINT ( 'NONE',  ( 207.8575108622103755, 270.6272257822888037, -6.381720258959569847 ) ) ;
#14501=CARTESIAN_POINT ( 'NONE',  ( 174.4781466557367651, 251.8266234104975467, -5.118404912015881436 ) ) ;
#14504=CARTESIAN_POINT ( 'NONE',  ( 193.4618118942367175, 290.7196881563408510, -16.34060166011831328 ) ) ;
#14505=CARTESIAN_POINT ( 'NONE',  ( 188.9122134955663910, 290.7695941481946988, -15.11888497690123678 ) ) ;
#14506=CARTESIAN_POINT ( 'NONE',  ( 146.4729408656479563, 243.8262482093457493, 3.021315404115420679E-15 ) ) ;
#14509=CARTESIAN_POINT ( 'NONE',  ( 6.427104459464150210, 164.5177522451418213, 5.000000000000051514 ) ) ;
#14513=CARTESIAN_POINT ( 'NONE',  ( 178.9682364468813773, 280.6870550632783647, 15.99938731543359971 ) ) ;
#14514=CARTESIAN_POINT ( 'NONE',  ( 146.7943851877206214, 276.3916619194686746, -4.608908220452185844 ) ) ;
#14517=ORIENTED_EDGE ( 'NONE', *, *, #43673, .T. ) ;
#14518=B_SPLINE_CURVE_WITH_KNOTS ( 'NONE', 3,
 ( #23842, #93288, #47145, #39527, #70452, #1062, #93800, #24361, #55232, #2577, #80605, #19287, #49166, #95813, #4051, #80102, #35449, #50154, #57738, #81106, #10668, #11182, #89223, #26367, #58729, #56752, #27361, #57242, #96802, #50640, #88217, #18272, #11673, #42535, #27851, #34455, #42049, #43024, #73468, #34941, #65837, #72983, #79605, #49647, #58244, #10168, #71972, #88717, #19771, #81593 ),
 .UNSPECIFIED., .F., .F.,
 ( 4, 2, 2, 2, 2, 2, 2, 2, 2, 2, 2, 2, 2, 2, 2, 2, 2, 2, 2, 2, 2, 2, 2, 2, 4 ),
 ( 0.001702369874200513212, 0.002155302416493423082, 0.002608234958786333386, 0.002834701229932852073, 0.002947934365506177552, 0.003061167501079503465, 0.003287633772226124067, 0.003514100043372744668, 0.003967032585666028371, 0.004419965127959312942, 0.005325830212545880349, 0.006231695297132447756, 0.006684627839425727122, 0.007137560381719008223, 0.007250793517292348014, 0.007307410085079029186, 0.007364026652865710357, 0.007477259788438970350, 0.007590492924012230344, 0.007816959195158743393, 0.008043425466305256441, 0.008269891737451771224, 0.008496358008598284273, 0.008722824279744799056, 0.008949290550891312104 ),
 .UNSPECIFIED. ) ;
#14521=CARTESIAN_POINT ( 'NONE',  ( 180.1973166148897576, 262.1945337904856501, -12.69576189704895519 ) ) ;
#14522=CARTESIAN_POINT ( 'NONE',  ( 173.2643044339734786, 253.6696019359482364, -9.161360666162188693 ) ) ;
#14524=CARTESIAN_POINT ( 'NONE',  ( 173.4036004108148177, 284.0055530444776650, -13.75802448165205405 ) ) ;
#14528=B_SPLINE_SURFACE_WITH_KNOTS ( 'NONE', 3, 1, ( 
 ( #47921, #63134 ),
 ( #94079, #2355 ),
 ( #39311, #64138 ),
 ( #23616, #54509 ),
 ( #70736, #1850 ),
 ( #24632, #86006 ),
 ( #31713, #47429 ),
 ( #16036, #1347 ),
 ( #17534, #8442 ),
 ( #62114, #55512 ),
 ( #46937, #8938 ),
 ( #71256, #87521 ),
 ( #70228, #62618 ),
 ( #48442, #32233 ),
 ( #40317, #93571 ),
 ( #2869, #32732 ),
 ( #93061, #79883 ),
 ( #39804, #48948 ),
 ( #40813, #95088 ),
 ( #63636, #86500 ),
 ( #24140, #94573 ),
 ( #41319, #33234 ),
 ( #17028, #77854 ),
 ( #25129, #55025 ),
 ( #56011, #87007 ),
 ( #79388, #71760 ),
 ( #25651, #56532 ),
 ( #10446, #18053 ),
 ( #16532, #78356 ),
 ( #11953, #80898 ),
 ( #58521, #89494 ),
 ( #3367, #49434 ),
 ( #19064, #81875 ),
 ( #34730, #50925 ) ),
 .UNSPECIFIED., .T., .F., .F.,
 ( 4, 2, 2, 2, 2, 2, 2, 2, 2, 2, 2, 2, 2, 2, 2, 2, 4 ),
 ( 2, 2 ),
 ( 0.000000000000000000, 0.06250000000000000000, 0.1250000000000000000, 0.1875000000000000000, 0.2500000000000000000, 0.3125000000000000000, 0.3750000000000000000, 0.4375000000000000000, 0.5000000000000000000, 0.5625000000000000000, 0.6250000000000000000, 0.6875000000000000000, 0.7500000000000000000, 0.8125000000000000000, 0.8750000000000000000, 0.9375000000000000000, 1.000000000000000000 ),
 ( 0.000000000000000000, 1.000000000000000000 ),
 .UNSPECIFIED. ) ;
#14529=ORIENTED_EDGE ( 'NONE', *, *, #17227, .T. ) ;
#14531=CARTESIAN_POINT ( 'NONE',  ( 184.7674300623272359, 293.5985477127894683, -10.64018628136773970 ) ) ;
#14532=VERTEX_POINT ( 'NONE', #32692 ) ;
#14535=CARTESIAN_POINT ( 'NONE',  ( 159.3056354669941470, 256.7215407695565546, 17.03060606420897471 ) ) ;
#14536=CARTESIAN_POINT ( 'NONE',  ( 190.4965153239555775, 278.7350028254225549, -16.50919675735249115 ) ) ;
#14537=CARTESIAN_POINT ( 'NONE',  ( 192.5136100383170401, 297.2036415955699340, -12.98767194394231872 ) ) ;
#14538=CARTESIAN_POINT ( 'NONE',  ( 188.8544700204132880, 297.4231428397746413, 9.261439979758030461 ) ) ;
#14553=CARTESIAN_POINT ( 'NONE',  ( 164.4219970653926453, 246.2565599513234815, 2.253343996881020050 ) ) ;
#14554=CARTESIAN_POINT ( 'NONE',  ( 206.7044739906782809, 272.6243442267827959, -10.28926534613781030 ) ) ;
#14556=CARTESIAN_POINT ( 'NONE',  ( 200.0313018224816801, 276.5939864008022369, 15.71640468486303099 ) ) ;
#14557=CARTESIAN_POINT ( 'NONE',  ( 189.9457600613112902, 301.6512882219586800, 0.04117870562599101891 ) ) ;
#14558=CARTESIAN_POINT ( 'NONE',  ( 170.9803632111054128, 287.8799287371469973, -4.334810812907764266 ) ) ;
#14560=CARTESIAN_POINT ( 'NONE',  ( 183.6912085166904944, 284.8534958222698492, -15.01658379341915683 ) ) ;
#14561=CARTESIAN_POINT ( 'NONE',  ( 114.8970466070627907, 227.9548013555409796, -4.594050593750042211 ) ) ;
#14563=CARTESIAN_POINT ( 'NONE',  ( 148.2066559145867757, 274.5764911490276177, -6.721604152511306829 ) ) ;
#14565=CARTESIAN_POINT ( 'NONE',  ( 188.4921780175364177, 291.9130024176957932, -14.30062038179651474 ) ) ;
#14571=CARTESIAN_POINT ( 'NONE',  ( 146.6682761148193777, 276.6100892410288452, 3.415557024771299410 ) ) ;
#14572=CARTESIAN_POINT ( 'NONE',  ( 159.2102594322688844, 254.8867369075254885, -16.13039487917589199 ) ) ;
#14575=CARTESIAN_POINT ( 'NONE',  ( 147.9582107679231626, 274.3758568834094262, 9.970076002444663743 ) ) ;
#14576=ORIENTED_EDGE ( 'NONE', *, *, #29555, .F. ) ;
#14577=CARTESIAN_POINT ( 'NONE',  ( 46.28462696178780789, 185.9824982072973967, 3.021315404115420679E-15 ) ) ;
#14580=CARTESIAN_POINT ( 'NONE',  ( 191.7730772792068308, 298.4862819590180720, -10.97593358402262886 ) ) ;
#14583=CARTESIAN_POINT ( 'NONE',  ( 184.3598761222536382, 288.8827646574232517, -13.18844735319207118 ) ) ;
#14585=CARTESIAN_POINT ( 'NONE',  ( 200.9450245801223787, 276.0628505547339273, -15.19655820136303070 ) ) ;
#14586=ORIENTED_EDGE ( 'NONE', *, *, #16992, .T. ) ;
#14587=CARTESIAN_POINT ( 'NONE',  ( 204.6861706212249885, 276.1201482077632363, 14.69005155300678922 ) ) ;
#14590=CARTESIAN_POINT ( 'NONE',  ( 173.3159035555527225, 251.5876627122220555, -0.6300199127931779275 ) ) ;
#14591=CARTESIAN_POINT ( 'NONE',  ( 190.8844566442973303, 271.0387251322553084, -14.20173667283605567 ) ) ;
#14596=CARTESIAN_POINT ( 'NONE',  ( 191.3748554418409356, 282.8820735151286954, -16.91564750171852438 ) ) ;
#14598=CARTESIAN_POINT ( 'NONE',  ( 71.43287601098374751, 221.2369531367911293, -4.594050593750048428 ) ) ;
#14599=CARTESIAN_POINT ( 'NONE',  ( -13.51183432020139819, 142.4280072687214442, 0.000000000000000000 ) ) ;
#14600=CARTESIAN_POINT ( 'NONE',  ( 147.4824818982269790, 275.1998434563504929, -4.972419998968698351 ) ) ;
#14602=EDGE_CURVE ( 'NONE', #92597, #15171, #7910, .T. ) ;
#14604=CARTESIAN_POINT ( 'NONE',  ( 207.1158949475991164, 271.9117422260973740, -5.823035679195911918 ) ) ;
#14606=CARTESIAN_POINT ( 'NONE',  ( 106.9582200821077578, 225.8927522451417929, -10.00000000000009237 ) ) ;
#14611=CARTESIAN_POINT ( 'NONE',  ( 204.9365032683681704, 275.6865593441178817, -12.41571226031502206 ) ) ;
#14615=CARTESIAN_POINT ( 'NONE',  ( 46.88655524640979166, 204.0024278399160949, -9.188101187500093303 ) ) ;
#14616=CARTESIAN_POINT ( 'NONE',  ( 157.7861133721078772, 257.3534302411229646, 18.03837896619386783 ) ) ;
#14617=CARTESIAN_POINT ( 'NONE',  ( 199.2515784447019200, 277.9484561788881933, 15.93523832605907664 ) ) ;
#14619=CARTESIAN_POINT ( 'NONE',  ( -16.28802019041737026, 174.7365022471903444, 2.944929066748280225E-16 ) ) ;
#14620=CARTESIAN_POINT ( 'NONE',  ( 49.51212862133765213, 190.2048013555409796, 4.594050593750051981 ) ) ;
#14622=CARTESIAN_POINT ( 'NONE',  ( 151.3681950933278983, 268.4695907787949523, -15.50699599486383917 ) ) ;
#14625=CARTESIAN_POINT ( 'NONE',  ( 168.9579038699606315, 279.3139280689009070, 15.08363371378442608 ) ) ;
#14628=CARTESIAN_POINT ( 'NONE',  ( 178.8898168495310586, 276.3570583279081916, 16.31703817734112150 ) ) ;
#14630=CARTESIAN_POINT ( 'NONE',  ( 153.3530509526309515, 276.8034356616051355, 7.280424537284008402 ) ) ;
#14631=CARTESIAN_POINT ( 'NONE',  ( 151.3998834813064036, 275.6155462708605342, 9.529510778888534261 ) ) ;
#14632=CARTESIAN_POINT ( 'NONE',  ( 90.95479231155565003, 229.9865022471903160, 10.00000000000009237 ) ) ;
#14633=CARTESIAN_POINT ( 'NONE',  ( 200.6097954076514895, 283.1806371883870383, 16.82611162221071766 ) ) ;
#14635=CARTESIAN_POINT ( 'NONE',  ( 194.2178510179977025, 285.2388007311112119, -17.07337800795351512 ) ) ;
#14639=CARTESIAN_POINT ( 'NONE',  ( 163.5580161323163111, 263.8619878914579431, 16.86834041886016777 ) ) ;
#14640=CARTESIAN_POINT ( 'NONE',  ( 187.6409835355971438, 276.9958261499423315, -17.68842699041714184 ) ) ;
#14641=FACE_OUTER_BOUND ( 'NONE', #61987, .T. ) ;
#14645=EDGE_CURVE ( 'NONE', #85510, #97286, #67547, .T. ) ;
#14646=CARTESIAN_POINT ( 'NONE',  ( 194.2223991963907963, 294.2439319543634610, -14.97294938100067441 ) ) ;
#14648=DIRECTION ( 'NONE',  ( -0.8660254037844387076, -0.4999999999999998890, -0.000000000000000000 ) ) ;
#14649=CARTESIAN_POINT ( 'NONE',  ( 204.8176812644112204, 275.8923650920285695, 14.65594551021579051 ) ) ;
#14653=FACE_OUTER_BOUND ( 'NONE', #34252, .T. ) ;
#14654=EDGE_CURVE ( 'NONE', #28879, #90346, #5299, .T. ) ;
#14655=ORIENTED_EDGE ( 'NONE', *, *, #28143, .F. ) ;
#14656=CARTESIAN_POINT ( 'NONE',  ( 109.1931406464380530, 245.3967562850346837, -4.648177544792955347E-16 ) ) ;
#14657=CARTESIAN_POINT ( 'NONE',  ( 206.8791291248445532, 272.3218326606039454, -10.16823074922856840 ) ) ;
#14661=CARTESIAN_POINT ( 'NONE',  ( 174.6137555705638249, 286.1945818789523628, 10.50642072453899090 ) ) ;
#14662=CARTESIAN_POINT ( 'NONE',  ( 159.6624207053301063, 282.2709084101314829, -3.217951961837643982 ) ) ;
#14664=CARTESIAN_POINT ( 'NONE',  ( 208.0006710756887287, 270.3792650189220126, -0.8737665032493013850 ) ) ;
#14665=CARTESIAN_POINT ( 'NONE',  ( 164.4864504671816690, 245.7481059646165704, 6.337356894698421783 ) ) ;
#14666=CARTESIAN_POINT ( 'NONE',  ( 159.5204760365350012, 254.3494259875849082, 16.90107507090185379 ) ) ;
#14667=CARTESIAN_POINT ( 'NONE',  ( 164.5425133943092817, 265.0501716792783213, -16.62885785886519230 ) ) ;
#14668=CARTESIAN_POINT ( 'NONE',  ( 138.6044920356617922, 241.6423013555409796, -4.594050593750043987 ) ) ;
#14669=CARTESIAN_POINT ( 'NONE',  ( 159.5747039080428351, 254.6547520131815929, -15.43565639722316796 ) ) ;
#14670=CARTESIAN_POINT ( 'NONE',  ( 195.7711535398184708, 291.1477395053983628, -15.80671369234383938 ) ) ;
#14671=CARTESIAN_POINT ( 'NONE',  ( 71.83943283659645829, 200.0327760586659451, 1.948934522072303157E-15 ) ) ;
#14672=VERTEX_POINT ( 'NONE', #99501 ) ;
#14673=CARTESIAN_POINT ( 'NONE',  ( 178.9714194486930694, 253.6239517424200187, 1.422777586239305059 ) ) ;
#14674=FACE_OUTER_BOUND ( 'NONE', #64447, .T. ) ;
#14676=CARTESIAN_POINT ( 'NONE',  ( 160.3870543052771325, 253.9566894099726824, 15.32724566468392169 ) ) ;
#14680=CARTESIAN_POINT ( 'NONE',  ( 190.5360041683329655, 260.2350817476381621, -0.09936466574572885846 ) ) ;
#14682=( BOUNDED_CURVE ( )  B_SPLINE_CURVE ( 2, ( #70060, #677, #39647, #78694, #86332, #89806, #57863, #35565, #26980 ),
 .UNSPECIFIED., .F., .T. ) 
 B_SPLINE_CURVE_WITH_KNOTS ( ( 3, 2, 2, 2, 3 ),
 ( 0.9556451612903226200, 0.9569892473118279952, 0.9596774193548387455, 0.9623655913978494958, 0.9637096774193548709 ),
 .UNSPECIFIED. ) 
 CURVE ( )  GEOMETRIC_REPRESENTATION_ITEM ( )  RATIONAL_B_SPLINE_CURVE ( ( 0.9330127018922194093, 0.9330127018922194093, 1.000000000000000000, 0.8660254037844387076, 1.000000000000000000, 0.8660254037844387076, 1.000000000000000000, 0.9330127018922194093, 0.9330127018922194093 ) ) 
 REPRESENTATION_ITEM ( '' )  );
#14684=CARTESIAN_POINT ( 'NONE',  ( 194.3562588153086779, 294.0120802933159325, 14.11474987148825200 ) ) ;
#14687=CARTESIAN_POINT ( 'NONE',  ( 161.9495997252073209, 250.1420603409351031, -13.99339207224158166 ) ) ;
#14692=CARTESIAN_POINT ( 'NONE',  ( 195.4492297588524821, 279.3069192732683064, 16.32671115009019758 ) ) ;
#14693=CARTESIAN_POINT ( 'NONE',  ( 162.5087209356614437, 261.3603897694041507, 16.94627484035424203 ) ) ;
#14694=CARTESIAN_POINT ( 'NONE',  ( 141.5541307454787727, 252.5333772461660260, 9.188101187500095079 ) ) ;
#14697=CARTESIAN_POINT ( 'NONE',  ( 182.0267153670255880, 257.6526772771978813, 6.606610945396032442 ) ) ;
#14698=CARTESIAN_POINT ( 'NONE',  ( 155.5207183646172950, 261.6826666266933898, -16.99780945766855922 ) ) ;
#14699=CARTESIAN_POINT ( 'NONE',  ( 153.3544108199959908, 265.0293642254135307, -17.49105661178601423 ) ) ;
#14703=CARTESIAN_POINT ( 'NONE',  ( 195.7085553319017492, 265.4126769123801637, 4.537051660298946132 ) ) ;
#14704=CARTESIAN_POINT ( 'NONE',  ( 147.9367384712558362, 275.7520979690174840, -3.798240563252472946 ) ) ;
#14705=CARTESIAN_POINT ( 'NONE',  ( 196.4666053756248800, 263.7899124407235263, 2.070580867331794028 ) ) ;
#14710=CARTESIAN_POINT ( 'NONE',  ( 190.1696443193688708, 301.2635093119881162, -4.804312979389741223 ) ) ;
#14711=CARTESIAN_POINT ( 'NONE',  ( 186.7554075434758545, 282.3000898601083577, 17.53539547572453827 ) ) ;
#14712=CARTESIAN_POINT ( 'NONE',  ( 164.6649740431187183, 245.4388940607451843, -1.430729255012818557 ) ) ;
#14713=CARTESIAN_POINT ( 'NONE',  ( 154.9683083969241011, 262.2340116239618055, 18.33261662430134109 ) ) ;
#14715=EDGE_CURVE ( 'NONE', #59283, #93478, #72409, .T. ) ;
#14721=EDGE_CURVE ( 'NONE', #28370, #70463, #82185, .T. ) ;
#14723=CARTESIAN_POINT ( 'NONE',  ( 143.1869494737567265, 260.1427522451419350, -10.00000000000009415 ) ) ;
#14724=CARTESIAN_POINT ( 'NONE',  ( 74.41009865654250177, 223.7677522451419350, -5.000000000000047962 ) ) ;
#14726=B_SPLINE_CURVE_WITH_KNOTS ( 'NONE', 3,
 ( #7234, #61922, #92384, #84781 ),
 .UNSPECIFIED., .F., .F.,
 ( 4, 4 ),
 ( 0.002373312334363397030, 0.007735900001989939878 ),
 .UNSPECIFIED. ) ;
#14729=CARTESIAN_POINT ( 'NONE',  ( 202.5873807299470002, 274.2480181431063215, -12.90768986605086788 ) ) ;
#14730=CARTESIAN_POINT ( 'NONE',  ( 184.7894305693181138, 292.1317680087225881, 12.52679022050396895 ) ) ;
#14731=CARTESIAN_POINT ( 'NONE',  ( 4.315907217689738395, 182.4869531367911293, 4.594050593750046652 ) ) ;
#14734=CARTESIAN_POINT ( 'NONE',  ( 170.1044942758423133, 270.7333397699701436, -17.30097750721906991 ) ) ;
#14735=CARTESIAN_POINT ( 'NONE',  ( 132.5961804768574837, 237.3615022471901739, 5.000000000000051514 ) ) ;
#14736=B_SPLINE_CURVE_WITH_KNOTS ( 'NONE', 3,
 ( #47884, #78826, #86972, #27619 ),
 .UNSPECIFIED., .F., .F.,
 ( 4, 4 ),
 ( 0.02417385730324417628, 0.03341671179551596732 ),
 .UNSPECIFIED. ) ;
#14737=CARTESIAN_POINT ( 'NONE',  ( 179.4558704258684827, 255.0642153075463625, -4.031494673986889765 ) ) ;
#14738=CARTESIAN_POINT ( 'NONE',  ( 191.2664131384496784, 261.1238491898760685, -1.547456513327413630 ) ) ;
#14739=CARTESIAN_POINT ( 'NONE',  ( 182.6994280064950829, 295.4856873408559750, 1.017319240502663202 ) ) ;
#14740=CARTESIAN_POINT ( 'NONE',  ( 55.51991954004235907, 212.8615022471903160, 5.000000000000046185 ) ) ;
#14741=CARTESIAN_POINT ( 'NONE',  ( 170.8843335314017509, 274.4719442773359219, 17.28596511953734449 ) ) ;
#14743=CARTESIAN_POINT ( 'NONE',  ( 190.5726849661229210, 300.5654224342945326, -0.2192718484028965964 ) ) ;
#14744=CARTESIAN_POINT ( 'NONE',  ( 25.07406103223676652, 173.0327760586659451, 1.948934522072303157E-15 ) ) ;
#14749=CARTESIAN_POINT ( 'NONE',  ( 164.9836323268835940, 244.8869617230113249, -2.696511969808454534 ) ) ;
#14751=CARTESIAN_POINT ( 'NONE',  ( 202.1313593282997090, 279.2250639425520831, -15.94178289068968368 ) ) ;
#14752=CARTESIAN_POINT ( 'NONE',  ( 180.0662822340164269, 262.4007578510376675, -14.24330825748563534 ) ) ;
#14754=CARTESIAN_POINT ( 'NONE',  ( 190.5969391768923913, 300.5234129089444650, -0.7564693504096553500 ) ) ;
#14756=CARTESIAN_POINT ( 'NONE',  ( 155.4812142336614329, 261.3456326552338282, 18.45193178807985745 ) ) ;
#14758=CARTESIAN_POINT ( 'NONE',  ( 153.6392919293977002, 266.5359356698173769, -16.75038546547492402 ) ) ;
#14764=CARTESIAN_POINT ( 'NONE',  ( 196.4104189369360256, 289.1535926469882725, -16.93751511765341533 ) ) ;
#14766=B_SPLINE_CURVE_WITH_KNOTS ( 'NONE', 3,
 ( #17554, #33252, #56549, #8455, #71775, #25668, #54524, #55528, #23632, #70752, #16547, #46953, #1365, #86514, #56028, #77870, #1863, #17045, #39329, #78878, #31729, #93587, #9968, #18067, #71273, #32747, #87022, #63651, #48460, #24155, #64153, #79402, #2374, #31243, #48963, #38839, #69745, #356, #62130, #93076, #85505, #50447, #49956, #19080, #51443, #80914, #3860, #65645, #74285, #4353, #66154, #26658 ),
 .UNSPECIFIED., .F., .F.,
 ( 4, 2, 2, 2, 2, 2, 2, 2, 2, 2, 2, 2, 2, 2, 2, 2, 2, 2, 2, 2, 2, 2, 2, 2, 2, 4 ),
 ( 9.707348704973383356E-05, 0.001109464165947084092, 0.001362561835671441965, 0.001615659505395799838, 0.001742208340257978124, 0.001868757175120156844, 0.001995306009982335347, 0.002121854844844514500, 0.002374952514568721886, 0.002628050184292929706, 0.003134245523741467209, 0.004146636202638430760, 0.005159026881535394744, 0.005665222220983831200, 0.005918319890708004759, 0.006044868725570091104, 0.006171417560432177450, 0.006234691977863176388, 0.006297966395294174458, 0.006424515230156154118, 0.006677612899880115173, 0.006930710569604075361, 0.007183808239328036416, 0.007436905909051997471, 0.007690003578775958526, 0.008196198918223731450 ),
 .UNSPECIFIED. ) ;
#14768=CARTESIAN_POINT ( 'NONE',  ( 154.8579861482817535, 262.4250953638155011, -17.69813260923097786 ) ) ;
#14769=ORIENTED_EDGE ( 'NONE', *, *, #34866, .F. ) ;
#14773=VERTEX_POINT ( 'NONE', #63090 ) ;
#14774=CARTESIAN_POINT ( 'NONE',  ( 201.1679199471075492, 282.2139371290980989, -16.62385308864941535 ) ) ;
#14776=CARTESIAN_POINT ( 'NONE',  ( 198.8028075628465103, 265.8836465705114165, -5.166853741832800218 ) ) ;
#14778=ORIENTED_EDGE ( 'NONE', *, *, #25590, .F. ) ;
#14779=CARTESIAN_POINT ( 'NONE',  ( 190.6084209867335915, 300.5035258309363826, -0.5505750481748228342 ) ) ;
#14780=B_SPLINE_CURVE_WITH_KNOTS ( 'NONE', 3,
 ( #77268, #93504, #30677, #38756, #69659, #7361, #14954, #78784, #9369, #92993, #85936, #31644, #23547, #40248, #16461, #62544, #54438, #71189, #85414, #78279, #69160, #15962, #77787, #8864, #39730, #1784, #61053, #92026, #22572, #100090, #45844, #92504, #88945, #80829 ),
 .UNSPECIFIED., .F., .F.,
 ( 4, 2, 2, 2, 2, 2, 2, 2, 2, 2, 2, 2, 2, 2, 2, 2, 4 ),
 ( 0.003474253451082755413, 0.003638662506878291483, 0.003720867034776073612, 0.003803071562673856175, 0.003967480618469285993, 0.004131889674264716678, 0.004460707785855577180, 0.004789525897446437683, 0.005447162120628222873, 0.006104798343810008930, 0.007420070790173648699, 0.008077707013355505880, 0.008159911541253200840, 0.008201013805202004084, 0.008242116069150809063, 0.008406525124946115715, 0.008735343236536794939 ),
 .UNSPECIFIED. ) ;
#14783=CARTESIAN_POINT ( 'NONE',  ( 206.2520115784021471, 273.4080321133600933, 11.69992874350409018 ) ) ;
#14786=CARTESIAN_POINT ( 'NONE',  ( 149.6071296322179194, 271.5198456328920997, 12.75640156477042453 ) ) ;
#14787=CARTESIAN_POINT ( 'NONE',  ( 172.7371573690596449, 271.6299009131761864, 17.79590902495428040 ) ) ;
#14788=ORIENTED_EDGE ( 'NONE', *, *, #69711, .T. ) ;
#14792=ORIENTED_EDGE ( 'NONE', *, *, #35208, .T. ) ;
#14796=CARTESIAN_POINT ( 'NONE',  ( 146.8201187048455267, 276.3470901603510015, 4.112223577763169047 ) ) ;
#14797=CARTESIAN_POINT ( 'NONE',  ( 147.8503508990560533, 274.5626756563852950, 7.845851077393495743 ) ) ;
#14798=CARTESIAN_POINT ( 'NONE',  ( 190.7805732161387766, 300.2053494229706985, 4.237982805666590025 ) ) ;
#14799=CARTESIAN_POINT ( 'NONE',  ( 170.6146439245076181, 275.3170351586339848, -16.42974606418417594 ) ) ;
#14800=CARTESIAN_POINT ( 'NONE',  ( 147.0565364609189487, 275.9376025950204507, -0.7434588459654102310 ) ) ;
#14801=CARTESIAN_POINT ( 'NONE',  ( 191.4082244002820516, 299.1182256826033949, -8.271837126846561361 ) ) ;
#14804=CARTESIAN_POINT ( 'NONE',  ( 196.8435556370661459, 289.7039558245273838, -16.43899056939217118 ) ) ;
#14808=ORIENTED_EDGE ( 'NONE', *, *, #64009, .T. ) ;
#14809=CARTESIAN_POINT ( 'NONE',  ( 190.8303853669842738, 300.1190722468715535, -3.872629674854036086 ) ) ;
#14811=CARTESIAN_POINT ( 'NONE',  ( 202.9971867686660687, 278.5713445860434376, 14.97348638629241790 ) ) ;
#14813=CARTESIAN_POINT ( 'NONE',  ( 179.7037933464966670, 282.7974177266479501, -15.46501558881825744 ) ) ;
#14814=CARTESIAN_POINT ( 'NONE',  ( 189.9718059322956094, 301.6061754500863117, -1.293200095882213185 ) ) ;
#14815=CARTESIAN_POINT ( 'NONE',  ( 169.2550101512937033, 285.1084512606926751, -7.936393743500282483 ) ) ;
#14816=ORIENTED_EDGE ( 'NONE', *, *, #83508, .T. ) ;
#14817=CARTESIAN_POINT ( 'NONE',  ( 207.9743173328493526, 270.4249110404894054, -2.481515874287090639 ) ) ;
#14818=CARTESIAN_POINT ( 'NONE',  ( 206.8317058779879574, 272.4039721336197317, -10.41591514895975834 ) ) ;
#14820=CARTESIAN_POINT ( 'NONE',  ( 42.00631479827475800, 208.3927522451419918, 2.944929066748280225E-16 ) ) ;
#14821=CARTESIAN_POINT ( 'NONE',  ( 119.1457234225564008, 239.5958772461660544, -9.188101187500095079 ) ) ;
#14822=CARTESIAN_POINT ( 'NONE',  ( 175.9678885359534206, 274.3885454833871336, 17.74267894519478261 ) ) ;
#14824=CARTESIAN_POINT ( 'NONE',  ( 196.4677102463732012, 290.3549391369982686, 16.45225250689336249 ) ) ;
#14825=CARTESIAN_POINT ( 'NONE',  ( 175.3928363776315678, 253.5036201821030488, -3.893038171866270325 ) ) ;
#14826=CARTESIAN_POINT ( 'NONE',  ( 43.26059451170998216, 183.5327760586659451, 1.948934522072303157E-15 ) ) ;
#14829=CARTESIAN_POINT ( 'NONE',  ( 191.3888075987175341, 298.7058057693718069, 7.964122443251637762 ) ) ;
#14830=CARTESIAN_POINT ( 'NONE',  ( 181.4151141111755123, 267.7021082867859718, 14.95001734426726259 ) ) ;
#14831=B_SPLINE_SURFACE_WITH_KNOTS ( 'NONE', 3, 1, ( 
 ( #54040, #8961 ),
 ( #86030, #40837 ),
 ( #9473, #71783 ),
 ( #47451, #17562 ),
 ( #54533, #84995 ),
 ( #62139, #70252 ),
 ( #71281, #23146 ),
 ( #87030, #38850 ),
 ( #39337, #78380 ),
 ( #859, #46440 ),
 ( #77371, #31739 ),
 ( #48469, #32755 ),
 ( #30770, #32257 ),
 ( #77881, #62640 ),
 ( #39830, #24655 ),
 ( #40342, #61652 ),
 ( #92600, #7975 ),
 ( #85515, #70761 ),
 ( #15541, #93597 ),
 ( #94104, #365 ),
 ( #16060, #63158 ),
 ( #1374, #79410 ),
 ( #17054, #55538 ),
 ( #86522, #47945 ),
 ( #25153, #56037 ),
 ( #31252, #78886 ),
 ( #1872, #63659 ),
 ( #94600, #96610 ),
 ( #41855, #89518 ),
 ( #88030, #57550 ),
 ( #65159, #49967 ),
 ( #72290, #2893 ),
 ( #33262, #64674 ),
 ( #2382, #26665 ) ),
 .UNSPECIFIED., .T., .F., .F.,
 ( 4, 2, 2, 2, 2, 2, 2, 2, 2, 2, 2, 2, 2, 2, 2, 2, 4 ),
 ( 2, 2 ),
 ( 0.000000000000000000, 0.06250000000000000000, 0.1250000000000000000, 0.1875000000000000000, 0.2500000000000000000, 0.3125000000000000000, 0.3750000000000000000, 0.4375000000000000000, 0.5000000000000000000, 0.5625000000000000000, 0.6250000000000000000, 0.6875000000000000000, 0.7500000000000000000, 0.8125000000000000000, 0.8750000000000000000, 0.9375000000000000000, 1.000000000000000000 ),
 ( 0.000000000000000000, 1.000000000000000000 ),
 .UNSPECIFIED. ) ;
#14832=EDGE_CURVE ( 'NONE', #69383, #69588, #16153, .T. ) ;
#14834=CARTESIAN_POINT ( 'NONE',  ( 190.5541309856500050, 300.5975588711562523, -4.167177996129430184 ) ) ;
#14835=CARTESIAN_POINT ( 'NONE',  ( 97.79278455872236009, 237.2677522451419065, -5.000000000000047962 ) ) ;
#14839=CARTESIAN_POINT ( 'NONE',  ( 110.2779841299479955, 241.1427522451419065, 10.00000000000009237 ) ) ;
#14840=EDGE_CURVE ( 'NONE', #63534, #99839, #43503, .T. ) ;
#14844=CARTESIAN_POINT ( 'NONE',  ( 156.2475800219573046, 280.1524317834912381, -1.584389128937929492 ) ) ;
#14846=CARTESIAN_POINT ( 'NONE',  ( 17.60459192459599365, 168.7202760586659736, -5.415160957724236172E-17 ) ) ;
#14849=CARTESIAN_POINT ( 'NONE',  ( 146.9700173529739970, 276.0874580858064746, -5.099093031535578469 ) ) ;
#14851=CARTESIAN_POINT ( 'NONE',  ( 206.9349434189263661, 269.8064106017384916, 1.784245431258210113 ) ) ;
#14852=CARTESIAN_POINT ( 'NONE',  ( 74.27495573685767738, 207.5643266524160424, 9.188101187500095079 ) ) ;
#14853=CARTESIAN_POINT ( 'NONE',  ( 161.3227470381586102, 251.2278010437646856, 14.45097375514160731 ) ) ;
#14856=CARTESIAN_POINT ( 'NONE',  ( 147.8527080755910958, 276.5585929068648170, -2.411454450074328903 ) ) ;
#14857=VERTEX_POINT ( 'NONE', #25605 ) ;
#14858=CARTESIAN_POINT ( 'NONE',  ( 7.022496928113825199, 174.8615022471902591, -10.00000000000009592 ) ) ;
#14859=CARTESIAN_POINT ( 'NONE',  ( 208.0692320075777957, 270.2605140014760536, 2.043861372130216569 ) ) ;
#14860=CARTESIAN_POINT ( 'NONE',  ( 129.3483248890680954, 254.6744531367911577, 4.594050593750047540 ) ) ;
#14862=CARTESIAN_POINT ( 'NONE',  ( 165.1934173706906392, 261.2005776251094744, -16.15582037233899726 ) ) ;
#14863=CARTESIAN_POINT ( 'NONE',  ( 185.3203834979958344, 260.3518937614031188, 6.392263009190532586 ) ) ;
#14865=CARTESIAN_POINT ( 'NONE',  ( 205.4659066454071876, 268.9227294828852450, 1.478439533706684017 ) ) ;
#14870=CARTESIAN_POINT ( 'NONE',  ( 164.1097555145034903, 246.4005607616103077, 8.441031814699046620 ) ) ;
#14872=CARTESIAN_POINT ( 'NONE',  ( 172.8211258227677263, 268.6731136379477221, -17.49577356889009749 ) ) ;
#14873=CARTESIAN_POINT ( 'NONE',  ( 193.9563577622949708, 270.9517976046026888, -13.72115171226643682 ) ) ;
#14874=ORIENTED_EDGE ( 'NONE', *, *, #80771, .F. ) ;
#14875=CARTESIAN_POINT ( 'NONE',  ( 207.0113543900018840, 272.0928117833072406, 7.993282520509792377 ) ) ;
#14876=CARTESIAN_POINT ( 'NONE',  ( 168.0320555621825633, 281.9299508771385945, -10.97411773085330822 ) ) ;
#14877=CARTESIAN_POINT ( 'NONE',  ( -22.42236680055709641, 157.8615022471902591, 0.000000000000000000 ) ) ;
#14879=CARTESIAN_POINT ( 'NONE',  ( 91.22542524669037789, 230.1427522451419065, -10.00000000000009592 ) ) ;
#14881=CARTESIAN_POINT ( 'NONE',  ( 201.2139346379346705, 282.1342373466909521, -16.65315141107179286 ) ) ;
#14882=VERTEX_POINT ( 'NONE', #2824 ) ;
#14884=CARTESIAN_POINT ( 'NONE',  ( 164.7647380297938184, 248.9862001899016946, 10.10785415616959071 ) ) ;
#14886=CARTESIAN_POINT ( 'NONE',  ( 190.3572031550745294, 300.9386478791372497, 3.093832330100951378 ) ) ;
#14888=CARTESIAN_POINT ( 'NONE',  ( 189.0406113324428077, 297.1088540668469591, 8.037437795754774683 ) ) ;
#14889=ORIENTED_EDGE ( 'NONE', *, *, #99932, .F. ) ;
#14891=CARTESIAN_POINT ( 'NONE',  ( 164.4111102060550991, 279.1452848850144619, 13.51928863813949633 ) ) ;
#14892=EDGE_CURVE ( 'NONE', #25891, #73044, #13209, .T. ) ;
#14893=CARTESIAN_POINT ( 'NONE',  ( 149.3801359649374092, 271.9130101976182914, -11.41245530317637424 ) ) ;
#14896=VERTEX_POINT ( 'NONE', #89449 ) ;
#14897=CARTESIAN_POINT ( 'NONE',  ( 105.1810637865323628, 231.5333772461660828, 9.188101187500095079 ) ) ;
#14898=CARTESIAN_POINT ( 'NONE',  ( 203.4303926360161086, 278.2952194811716709, 16.49722835243206021 ) ) ;
#14899=CARTESIAN_POINT ( 'NONE',  ( 181.3308514678389258, 271.2102151123074805, -15.98608675868754680 ) ) ;
#14900=CARTESIAN_POINT ( 'NONE',  ( 131.1144086761837571, 258.0530062829863027, -4.648177544792955347E-16 ) ) ;
#14901=VERTEX_POINT ( 'NONE', #73704 ) ;
#14909=FACE_OUTER_BOUND ( 'NONE', #53553, .T. ) ;
#14910=CARTESIAN_POINT ( 'NONE',  ( 165.4414073703629526, 271.0891460371367998, 16.46202333746585111 ) ) ;
#14911=CARTESIAN_POINT ( 'NONE',  ( 170.8853045030261342, 283.1981579494924972, 11.95786326274130396 ) ) ;
#14912=EDGE_CURVE ( 'NONE', #82888, #38166, #18052, .T. ) ;
#14915=CARTESIAN_POINT ( 'NONE',  ( 204.2521851317371215, 272.5184155020062349, -10.97406441561872548 ) ) ;
#14917=CARTESIAN_POINT ( 'NONE',  ( 198.8683739244561082, 276.4215138120039796, -15.93986209720707414 ) ) ;
#14920=ORIENTED_EDGE ( 'NONE', *, *, #22452, .F. ) ;
#14921=CARTESIAN_POINT ( 'NONE',  ( 162.8789161433191452, 248.5324370884573568, 9.731756914259689140 ) ) ;
#14925=CARTESIAN_POINT ( 'NONE',  ( 170.4549130973286140, 255.0430615571639521, 11.26541777191281568 ) ) ;
#14926=CARTESIAN_POINT ( 'NONE',  ( 194.8368544504894828, 263.2804105082292381, -0.7921045588880984978 ) ) ;
#14927=ORIENTED_EDGE ( 'NONE', *, *, #59618, .T. ) ;
#14928=CARTESIAN_POINT ( 'NONE',  ( 182.9621872738214279, 272.0904772814410535, -16.05491882940554760 ) ) ;
#14931=CARTESIAN_POINT ( 'NONE',  ( 5.488910272031021442, 160.6427522451417644, 1.119607411625061291E-15 ) ) ;
#14932=CARTESIAN_POINT ( 'NONE',  ( 196.0902246659342154, 269.6848923550738846, -11.36688942032260385 ) ) ;
#14933=CARTESIAN_POINT ( 'NONE',  ( 174.5432515410337544, 282.4104588529930311, -15.15290805577315680 ) ) ;
#14937=CARTESIAN_POINT ( 'NONE',  ( -6.509410329615746171, 176.2369531367911293, -4.594050593750048428 ) ) ;
#14939=CARTESIAN_POINT ( 'NONE',  ( 197.3327212804159103, 267.5970440452412049, 9.861675131224707513 ) ) ;
#14946=CARTESIAN_POINT ( 'NONE',  ( 163.1438579415164156, 248.0735444329312713, -11.47272517958888116 ) ) ;
#14949=CARTESIAN_POINT ( 'NONE',  ( 153.6013573859479209, 279.1680573449844474, 3.826191094887242183 ) ) ;
#14950=CARTESIAN_POINT ( 'NONE',  ( 13.49027706508988089, 190.8464784336661637, 1.353441290958777525E-15 ) ) ;
#14951=CARTESIAN_POINT ( 'NONE',  ( 114.8970466070627907, 227.9548013555409796, -4.594050593750042211 ) ) ;
#14952=CARTESIAN_POINT ( 'NONE',  ( 182.0607763290098262, 294.6140211400301610, -6.481743162254417712 ) ) ;
#14953=CARTESIAN_POINT ( 'NONE',  ( 196.3249884498792994, 275.2518087180711177, 16.06659936265807431 ) ) ;
#14954=CARTESIAN_POINT ( 'NONE',  ( 153.5230417281645714, 274.1903830991208793, -12.08502709614621651 ) ) ;
#14956=B_SPLINE_CURVE_WITH_KNOTS ( 'NONE', 3,
 ( #69274, #84032, #61169, #76404, #61668, #92618, #22185, #15558, #68276, #75403, #77391, #7470, #75912, #38364, #53569, #45469, #6979, #37371, #30279, #52569, #67787, #99695, #14591, #84521, #15067, #45956, #76873, #5986, #83525, #23166, #36882, #98713, #30788, #99198, #29299, #54058, #60161, #85014, #21690, #14089, #44974, #29784, #6492, #60656, #91612, #53079, #36697, #66117, #36201, #66614 ),
 .UNSPECIFIED., .F., .F.,
 ( 4, 2, 2, 2, 2, 2, 2, 2, 2, 2, 2, 2, 2, 2, 2, 2, 2, 2, 2, 2, 2, 2, 2, 2, 4 ),
 ( 0.0003739468527002533975, 0.0008345414556833621964, 0.001064838757174917192, 0.001295136058666471971, 0.001410284709412328724, 0.001525433360158185044, 0.001640582010904041797, 0.001755730661649898116, 0.001986027963141681445, 0.002216325264633465207, 0.003137514470600615869, 0.004058703676567767399, 0.004979892882534918928, 0.005440487485518494259, 0.005670784787010286696, 0.005785933437756182914, 0.005843507763129083751, 0.005901082088501983722, 0.005958656413874884560, 0.006016230739247785397, 0.006131379389993588808, 0.006361676691485088075, 0.006822271294468086611, 0.007282865897451086881, 0.007743460500434085417 ),
 .UNSPECIFIED. ) ;
#14957=B_SPLINE_CURVE_WITH_KNOTS ( 'NONE', 3,
 ( #68743, #23624, #54518, #99666, #85496, #30252, #92110, #53540, #16045, #46947, #61635, #85385, #53430, #38727, #46836, #92965, #84379, #31122, #76740, #37724, #100060, #44833, #76266, #15931, #13951, #91992, #69631, #7333, #90994, #5853, #54410, #23022, #92475, #75766, #30645, #77238, #61532, #53915, #60524, #36737, #6839, #52438, #91477, #22544, #240, #62013, #14452, #83386 ),
 .UNSPECIFIED., .F., .F.,
 ( 4, 2, 2, 2, 2, 2, 2, 2, 2, 2, 2, 2, 2, 2, 2, 2, 2, 2, 2, 2, 2, 2, 2, 4 ),
 ( 0.001525744563423052889, 0.001989215674126778178, 0.002452686784830503466, 0.002684422340182411430, 0.002800290117858385795, 0.002916157895534359727, 0.003032025673210333658, 0.003147893450886307155, 0.003379629006238109735, 0.003843100116941790354, 0.004306571227645470540, 0.005233513449052831779, 0.006160455670460193017, 0.006623926781163830269, 0.007087397891867466652, 0.007203265669543395047, 0.007261199558381358811, 0.007319133447219321707, 0.007550869002571125588, 0.007782604557922930336, 0.008014340113274735083, 0.008246075668626538097, 0.008477811223978342844, 0.008941282334681908972 ),
 .UNSPECIFIED. ) ;
#14958=CARTESIAN_POINT ( 'NONE',  ( 125.6883311748214425, 231.8262482093457493, 3.021315404115420679E-15 ) ) ;
#14959=CARTESIAN_POINT ( 'NONE',  ( 190.7350272470297341, 299.8690974414012089, -4.572277333844146696 ) ) ;
#14962=CARTESIAN_POINT ( 'NONE',  ( 184.3272200602622775, 274.5360433806101241, 16.60951854980709541 ) ) ;
#14966=CARTESIAN_POINT ( 'NONE',  ( 164.9407228494403057, 249.8614573468021547, -10.59005222520834621 ) ) ;
#14970=DIRECTION ( 'NONE',  ( 0.8660254037844387076, 0.4999999999999998890, 0.000000000000000000 ) ) ;
#14971=ORIENTED_EDGE ( 'NONE', *, *, #87627, .F. ) ;
#14972=CARTESIAN_POINT ( 'NONE',  ( 159.1344352748853055, 279.7114264697810313, -10.00621538743078354 ) ) ;
#14974=CARTESIAN_POINT ( 'NONE',  ( 99.20033616346982797, 218.8923013555410080, 4.594050593750050204 ) ) ;
#14980=CARTESIAN_POINT ( 'NONE',  ( 113.7185830531895903, 224.9155109091896634, 2.679491924311254714 ) ) ;
#14981=CARTESIAN_POINT ( 'NONE',  ( 196.7270510492836877, 289.9057476898814230, 17.95127088795220160 ) ) ;
#14982=CARTESIAN_POINT ( 'NONE',  ( 190.9513712376748060, 261.2677970607517182, -4.679362068315001899 ) ) ;
#14983=CARTESIAN_POINT ( 'NONE',  ( 196.5475899070771675, 290.2165835061676944, -17.89382743182097002 ) ) ;
#14985=CARTESIAN_POINT ( 'NONE',  ( 192.4867975473904949, 297.2500821921321972, -13.04960750009181325 ) ) ;
#14989=CARTESIAN_POINT ( 'NONE',  ( 179.0715434446022130, 280.8390982330867587, 16.22398002533389771 ) ) ;
#14990=CARTESIAN_POINT ( 'NONE',  ( 197.1680355107441471, 268.3962010867043659, 9.346870724141478348 ) ) ;
#14991=CARTESIAN_POINT ( 'NONE',  ( 196.4242782546697015, 290.4301655533025155, -16.42402868779123537 ) ) ;
#14993=CARTESIAN_POINT ( 'NONE',  ( 159.6419305724666344, 254.1390605605417079, 16.92015248457581933 ) ) ;
#14994=CARTESIAN_POINT ( 'NONE',  ( 182.8336677718184546, 264.3499445543482693, -13.07731979293364866 ) ) ;
#14995=CARTESIAN_POINT ( 'NONE',  ( 169.3689075499657122, 251.9910147621546344, -8.596408333947868741 ) ) ;
#15001=EDGE_LOOP ( 'NONE', ( #41421, #29984, #28274, #83222 ) ) ;
#15002=FACE_OUTER_BOUND ( 'NONE', #74541, .T. ) ;
#15004=VERTEX_POINT ( 'NONE', #80343 ) ;
#15005=CARTESIAN_POINT ( 'NONE',  ( 206.8217325168575371, 270.0045844243117017, 3.350393751014514532 ) ) ;
#15007=CARTESIAN_POINT ( 'NONE',  ( 193.7694484332697016, 280.6102121743993507, -17.05218128339958383 ) ) ;
#15008=CARTESIAN_POINT ( 'NONE',  ( 153.8558716659707954, 264.1608085621786586, -16.57261382954067130 ) ) ;
#15009=CARTESIAN_POINT ( 'NONE',  ( 200.7694952279801157, 282.9040289856181403, -17.94628235092568502 ) ) ;
#15016=CARTESIAN_POINT ( 'NONE',  ( 195.0619961850419486, 291.0373835071860640, 16.42391134123714380 ) ) ;
#15019=CARTESIAN_POINT ( 'NONE',  ( 198.0204369024629045, 286.8851334562542092, 16.94118585317415082 ) ) ;
#15022=CARTESIAN_POINT ( 'NONE',  ( 165.6600941239869087, 274.7658140146604637, -15.24034129512801528 ) ) ;
#15023=CARTESIAN_POINT ( 'NONE',  ( 164.9825360643182535, 244.8888605054729624, -1.157747536866345461 ) ) ;
#15024=CARTESIAN_POINT ( 'NONE',  ( 197.4084121877038172, 273.1799603734787638, -13.34748769055383200 ) ) ;
#15027=CARTESIAN_POINT ( 'NONE',  ( 171.3928239984006723, 250.3015599828365509, -5.796133048607560845 ) ) ;
#15028=EDGE_CURVE ( 'NONE', #76220, #61239, #86804, .T. ) ;
#15030=CARTESIAN_POINT ( 'NONE',  ( 183.4471554107105931, 284.5186797981741620, -15.10776214044594745 ) ) ;
#15031=CARTESIAN_POINT ( 'NONE',  ( 114.1117772151768577, 242.8149278399161233, -9.188101187500095079 ) ) ;
#15033=CARTESIAN_POINT ( 'NONE',  ( 183.4504012090349931, 260.3740723431718607, -9.329707687019228146 ) ) ;
#15035=CARTESIAN_POINT ( 'NONE',  ( 188.3932030005877323, 273.5611838242375597, 15.65614328840583092 ) ) ;
#15037=AXIS2_PLACEMENT_3D ( 'NONE', #48522, #2945, #34310 ) ;
#15038=VERTEX_POINT ( 'NONE', #27108 ) ;
#15039=CARTESIAN_POINT ( 'NONE',  ( 162.8643913348946342, 249.0653215557598799, -10.24700337220267166 ) ) ;
#15040=CARTESIAN_POINT ( 'NONE',  ( 121.7448624948184204, 229.5494855054051584, -2.679491924311248496 ) ) ;
#15042=CARTESIAN_POINT ( 'NONE',  ( 147.4451090059320109, 275.2645752046312850, 3.125785074907880823 ) ) ;
#15043=CARTESIAN_POINT ( 'NONE',  ( 206.0946696452135427, 273.6805563358039421, -10.19627505985792837 ) ) ;
#15045=EDGE_CURVE ( 'NONE', #49678, #16991, #32381, .T. ) ;
#15047=CARTESIAN_POINT ( 'NONE',  ( 195.1394560277449841, 292.6555429290298207, 16.72738487262295948 ) ) ;
#15051=ORIENTED_EDGE ( 'NONE', *, *, #60788, .F. ) ;
#15052=CARTESIAN_POINT ( 'NONE',  ( 191.7251117466753101, 267.4289849328922628, -12.63340514153103200 ) ) ;
#15053=AXIS2_PLACEMENT_3D ( 'NONE', #56101, #23209, #17113 ) ;
#15054=CARTESIAN_POINT ( 'NONE',  ( 152.0354063984034951, 267.3139468990199816, -16.99296076417658341 ) ) ;
#15055=CARTESIAN_POINT ( 'NONE',  ( 158.4595209236517519, 263.4143799451769041, 17.55458220974047379 ) ) ;
#15056=CARTESIAN_POINT ( 'NONE',  ( 168.5910505471324257, 286.4687829538495976, 8.106709794022206594 ) ) ;
#15057=CARTESIAN_POINT ( 'NONE',  ( 184.3873580908706913, 288.5454924782333705, -13.82082247699642430 ) ) ;
#15058=CARTESIAN_POINT ( 'NONE',  ( 157.1870951989065190, 280.8757593961267389, 6.041051901132188817 ) ) ;
#15059=CARTESIAN_POINT ( 'NONE',  ( 153.4542976351440302, 264.8563551865710224, -17.11782692037292009 ) ) ;
#15061=CARTESIAN_POINT ( 'NONE',  ( 190.4240181651484818, 300.8229208869809668, -4.214281362166949485 ) ) ;
#15066=CYLINDRICAL_SURFACE ( 'NONE', #14093, 10.00000000000010658 ) ;
#15067=CARTESIAN_POINT ( 'NONE',  ( 190.0718168876597076, 270.6242987759774223, -14.12311039011201785 ) ) ;
#15070=CARTESIAN_POINT ( 'NONE',  ( 35.94413697178374889, 184.8927522451418213, 10.00000000000009948 ) ) ;
#15072=CARTESIAN_POINT ( 'NONE',  ( 191.3337820289262936, 282.9518992253598526, -16.81566807114812789 ) ) ;
#15074=CARTESIAN_POINT ( 'NONE',  ( 75.49289073487081225, 205.2048013555409796, 4.594050593750051981 ) ) ;
#15076=CARTESIAN_POINT ( 'NONE',  ( 193.0761489135300906, 296.2292956824684893, -11.99675185248219655 ) ) ;
#15077=CARTESIAN_POINT ( 'NONE',  ( 208.3699316049496133, 269.7396870210121733, -1.898463622294385811 ) ) ;
#15080=CARTESIAN_POINT ( 'NONE',  ( 161.6127771116929921, 250.7254542206800352, -12.96229604595372464 ) ) ;
#15081=CARTESIAN_POINT ( 'NONE',  ( -22.42236680055709641, 157.8615022471902591, 0.000000000000000000 ) ) ;
#15084=EDGE_CURVE ( 'NONE', #86525, #99556, #19130, .T. ) ;
#15086=CARTESIAN_POINT ( 'NONE',  ( 164.5204976463763558, 245.6891345203973174, -4.279147110458541903 ) ) ;
#15087=CARTESIAN_POINT ( 'NONE',  ( 196.3341081413628899, 290.5863447708742342, 16.12390540996472410 ) ) ;
#15089=CARTESIAN_POINT ( 'NONE',  ( 25.77753312492912841, 179.5643266524160140, -9.188101187500093303 ) ) ;
#15090=CARTESIAN_POINT ( 'NONE',  ( 47.26526781268299260, 210.3464784336661637, 1.353441290958777327E-15 ) ) ;
#15091=CARTESIAN_POINT ( 'NONE',  ( 157.7529601300917363, 257.4108533407307959, 16.91445305439664892 ) ) ;
#15093=CARTESIAN_POINT ( 'NONE',  ( 165.0642700556339264, 248.7133924234977371, -9.523431784498571417 ) ) ;
#15094=CARTESIAN_POINT ( 'NONE',  ( -8.493791556357338735, 159.2365022471901739, -10.00000000000009059 ) ) ;
#15095=DIRECTION ( 'NONE',  ( 0.4999999999999998890, -0.8660254037844385966, 0.000000000000000000 ) ) ;
#15097=CARTESIAN_POINT ( 'NONE',  ( -4.331504796628791176, 156.7592609112379876, 2.679491924311251605 ) ) ;
#15098=CARTESIAN_POINT ( 'NONE',  ( -17.22621437785049636, 170.8615022471903160, 5.000000000000046185 ) ) ;
#15100=CARTESIAN_POINT ( 'NONE',  ( 55.22204975783502334, 208.8149278399160664, 9.188101187500093303 ) ) ;
#15101=CARTESIAN_POINT ( 'NONE',  ( 175.5847330776380204, 258.8848994771980188, -13.61208222109076615 ) ) ;
#15103=CARTESIAN_POINT ( 'NONE',  ( 159.9014600375868440, 253.6895423408921886, 15.57825579621527368 ) ) ;
#15105=CARTESIAN_POINT ( 'NONE',  ( 201.5827075904949766, 281.4955038563991252, 16.28834193516912165 ) ) ;
#15107=CARTESIAN_POINT ( 'NONE',  ( 116.1416978049531110, 237.8615022471902307, -10.00000000000009592 ) ) ;
#15108=CARTESIAN_POINT ( 'NONE',  ( 200.5810378487751393, 283.2304467414622877, 18.38516374632547112 ) ) ;
#15109=CARTESIAN_POINT ( 'NONE',  ( 165.1536807772045279, 269.6115192885357033, -16.29157638650531226 ) ) ;
#15112=ORIENTED_EDGE ( 'NONE', *, *, #549, .F. ) ;
#15113=CARTESIAN_POINT ( 'NONE',  ( 206.6703863510205679, 272.6833857505801006, -10.72500664779635393 ) ) ;
#15114=CARTESIAN_POINT ( 'NONE',  ( 188.9750831269214757, 277.9074358098590096, -16.52746066141228809 ) ) ;
#15115=CARTESIAN_POINT ( 'NONE',  ( 170.3489334754653441, 276.6636095645281443, 16.60343083925547347 ) ) ;
#15116=VERTEX_POINT ( 'NONE', #58957 ) ;
#15117=AXIS2_PLACEMENT_3D ( 'NONE', #59830, #48, #44124 ) ;
#15118=ORIENTED_EDGE ( 'NONE', *, *, #30523, .F. ) ;
#15120=CARTESIAN_POINT ( 'NONE',  ( 194.2154056360670040, 294.2560451561701029, -15.66696967429384557 ) ) ;
#15121=CARTESIAN_POINT ( 'NONE',  ( 177.1487090986248063, 274.7577274326447991, -16.88435297823402337 ) ) ;
#15128=CARTESIAN_POINT ( 'NONE',  ( 141.1607630391569330, 240.7592609112380160, 2.679491924311254714 ) ) ;
#15134=CARTESIAN_POINT ( 'NONE',  ( 162.6262389125959373, 248.9700868899859074, -10.50380342094597808 ) ) ;
#15135=CARTESIAN_POINT ( 'NONE',  ( 163.7064929935861244, 247.0990319366274548, 6.401263337036986023 ) ) ;
#15136=CARTESIAN_POINT ( 'NONE',  ( 188.6905595153717741, 295.3522105695485607, -11.31054681824411290 ) ) ;
#15137=CARTESIAN_POINT ( 'NONE',  ( 161.7922706396030605, 263.4318561585560587, -17.02534324577779401 ) ) ;
#15138=CARTESIAN_POINT ( 'NONE',  ( 142.3122500695552048, 240.7202760586659736, -5.415160957724236172E-17 ) ) ;
#15140=CARTESIAN_POINT ( 'NONE',  ( 176.7284915028678824, 269.1415778121231597, 16.10409147245672301 ) ) ;
#15141=CARTESIAN_POINT ( 'NONE',  ( 195.8006847607455825, 290.9998369522246549, -15.91509253693118531 ) ) ;
#15142=CARTESIAN_POINT ( 'NONE',  ( 64.74832919946385346, 214.3149278399160949, -9.188101187500095079 ) ) ;
#15143=B_SPLINE_CURVE_WITH_KNOTS ( 'NONE', 3,
 ( #46986, #78912, #63684, #64184 ),
 .UNSPECIFIED., .F., .F.,
 ( 4, 4 ),
 ( 0.000000000000000000, 0.003498996904287751328 ),
 .UNSPECIFIED. ) ;
#15144=ORIENTED_EDGE ( 'NONE', *, *, #60920, .F. ) ;
#15146=DIRECTION ( 'NONE',  ( -0.8660254037844387076, -0.4999999999999998890, -0.000000000000000000 ) ) ;
#15147=CARTESIAN_POINT ( 'NONE',  ( 205.1956247482881110, 271.9973608250444954, 9.678236287800089599 ) ) ;
#15149=CARTESIAN_POINT ( 'NONE',  ( 168.0439751434946629, 261.0016734627291726, -16.81520615430363108 ) ) ;
#15150=VERTEX_POINT ( 'NONE', #67579 ) ;
#15154=CARTESIAN_POINT ( 'NONE',  ( 197.5324136461498767, 286.6052654224091611, 16.91853012670608791 ) ) ;
#15158=CARTESIAN_POINT ( 'NONE',  ( 193.7261517370125432, 295.1034577671335342, 14.97744313279139661 ) ) ;
#15160=EDGE_CURVE ( 'NONE', #81343, #94798, #79621, .T. ) ;
#15161=CARTESIAN_POINT ( 'NONE',  ( 74.35571174875622091, 222.9244531367911293, -4.594050593750046652 ) ) ;
#15164=CARTESIAN_POINT ( 'NONE',  ( 200.4026220252542032, 283.5394720126751622, -17.02811402915289918 ) ) ;
#15168=CARTESIAN_POINT ( 'NONE',  ( 165.2054706378175126, 285.1533889500111627, 0.5060398096789098243 ) ) ;
#15171=VERTEX_POINT ( 'NONE', #82836 ) ;
#15173=CARTESIAN_POINT ( 'NONE',  ( 156.6685347489093090, 274.1288574488814902, 13.57745094969755328 ) ) ;
#15174=CARTESIAN_POINT ( 'NONE',  ( 178.0315741628076012, 287.5935043698759728, -13.06113257055532451 ) ) ;
#15175=CARTESIAN_POINT ( 'NONE',  ( 153.4361244163197000, 264.8878321249116539, -17.23169627811277493 ) ) ;
#15180=CARTESIAN_POINT ( 'NONE',  ( 196.2350291401047571, 264.4780031501763347, 5.359379669934941859 ) ) ;
#15181=EDGE_CURVE ( 'NONE', #72513, #2782, #74761, .T. ) ;
#15182=CARTESIAN_POINT ( 'NONE',  ( 82.20432729060250665, 218.2677522451418497, 10.00000000000009592 ) ) ;
#15183=CARTESIAN_POINT ( 'NONE',  ( 191.2190380946134951, 260.9445496458436651, 3.106810577783889915 ) ) ;
#15186=CARTESIAN_POINT ( 'NONE',  ( 198.9686279331660899, 265.4156631160248025, 0.08760027866574053579 ) ) ;
#15189=CARTESIAN_POINT ( 'NONE',  ( 190.3625087333586521, 300.9294583479858147, -4.271886578030237303 ) ) ;
#15190=EDGE_CURVE ( 'NONE', #73044, #3083, #88070, .T. ) ;
#15196=EDGE_CURVE ( 'NONE', #6903, #23257, #78298, .T. ) ;
#15199=CARTESIAN_POINT ( 'NONE',  ( 26.41785753015494009, 179.3927522451418213, -10.00000000000009237 ) ) ;
#15200=CARTESIAN_POINT ( 'NONE',  ( 163.7895146392965842, 284.0257305568636070, -3.118330620146652077 ) ) ;
#15202=CARTESIAN_POINT ( 'NONE',  ( 159.2876523829509665, 254.7526883847961017, 15.64395448151312351 ) ) ;
#15203=CARTESIAN_POINT ( 'NONE',  ( -7.320788502016136512, 157.3923013555410080, 4.594050593750050204 ) ) ;
#15204=CARTESIAN_POINT ( 'NONE',  ( 189.0622672619279001, 295.6589450522362199, -11.52442905864715250 ) ) ;
#15207=CARTESIAN_POINT ( 'NONE',  ( 178.8238403317331233, 256.6237485836615519, 8.676301928053684165 ) ) ;
#15210=CARTESIAN_POINT ( 'NONE',  ( 9.512059640396367755, 185.4869531367911293, 4.594050593750046652 ) ) ;
#15211=CARTESIAN_POINT ( 'NONE',  ( 176.1988396708435687, 265.5930599550684406, -16.16477898283384107 ) ) ;
#15212=CARTESIAN_POINT ( 'NONE',  ( 179.8452673937777320, 274.4601373947340335, -16.56085817225330103 ) ) ;
#15214=CARTESIAN_POINT ( 'NONE',  ( 187.1412927779018673, 261.9835105880691231, -10.20549468610707322 ) ) ;
#15215=CARTESIAN_POINT ( 'NONE',  ( 173.2317256228830047, 272.4512950130714444, -16.36800549663501769 ) ) ;
#15217=CARTESIAN_POINT ( 'NONE',  ( 175.6012255355377931, 253.3303057574685226, -3.452269288186304408 ) ) ;
#15219=CARTESIAN_POINT ( 'NONE',  ( 183.0280766574859399, 295.8866060358298569, 1.576309391735440046 ) ) ;
#15220=CARTESIAN_POINT ( 'NONE',  ( 73.27344031762339682, 213.1115022471902591, 10.00000000000009592 ) ) ;
#15222=CARTESIAN_POINT ( 'NONE',  ( 189.8171280724701546, 301.8740853621098950, -0.4360232994423257624 ) ) ;
#15223=CARTESIAN_POINT ( 'NONE',  ( 28.72751893051112049, 178.2048013555409796, 4.594050593750051981 ) ) ;
#15227=CARTESIAN_POINT ( 'NONE',  ( 205.5636066921878466, 271.2094078441786564, -6.548282385051860999 ) ) ;
#15228=CARTESIAN_POINT ( 'NONE',  ( 199.0773057068961123, 285.8349872121713702, -17.17316764978006560 ) ) ;
#15229=CARTESIAN_POINT ( 'NONE',  ( 165.0156970625405108, 244.8314239717225007, -1.890480716182876719 ) ) ;
#15230=CARTESIAN_POINT ( 'NONE',  ( 187.4731087846878381, 267.6488792197166617, 13.31701845521303618 ) ) ;
#15231=CARTESIAN_POINT ( 'NONE',  ( 202.8814167162130673, 278.7900253483502411, -15.09576271200930719 ) ) ;
#15232=CARTESIAN_POINT ( 'NONE',  ( 163.7573486046460971, 281.3881871899058638, 8.856914258957445441 ) ) ;
#15235=CARTESIAN_POINT ( 'NONE',  ( 190.0515794655415789, 301.4680036374047063, -1.296825456579539626 ) ) ;
#15236=CARTESIAN_POINT ( 'NONE',  ( 194.5051734451974426, 293.7541525883582381, 14.61790433731063921 ) ) ;
#15237=ORIENTED_EDGE ( 'NONE', *, *, #12227, .T. ) ;
#15238=CARTESIAN_POINT ( 'NONE',  ( 166.5497620933320775, 284.9599651698292178, -8.643830016708903941 ) ) ;
#15243=( BOUNDED_CURVE ( )  B_SPLINE_CURVE ( 2, ( #14506, #23080, #7907, #77816, #15993, #69688, #22598, #76794, #293 ),
 .UNSPECIFIED., .F., .T. ) 
 B_SPLINE_CURVE_WITH_KNOTS ( ( 3, 2, 2, 2, 3 ),
 ( 0.9637096774193548709, 0.9650537634408602461, 0.9677419354838709964, 0.9704301075268817467, 0.9717741935483871218 ),
 .UNSPECIFIED. ) 
 CURVE ( )  GEOMETRIC_REPRESENTATION_ITEM ( )  RATIONAL_B_SPLINE_CURVE ( ( 0.9330127018922194093, 0.9330127018922194093, 1.000000000000000000, 0.8660254037844387076, 1.000000000000000000, 0.8660254037844387076, 1.000000000000000000, 0.9330127018922194093, 0.9330127018922194093 ) ) 
 REPRESENTATION_ITEM ( '' )  );
#15247=CARTESIAN_POINT ( 'NONE',  ( 180.8079597460555306, 256.9122500747120057, -7.784400698518015638 ) ) ;
#15249=ORIENTED_EDGE ( 'NONE', *, *, #63976, .F. ) ;
#15253=CARTESIAN_POINT ( 'NONE',  ( 191.5694344253287511, 298.8390017285333897, 8.250976118904059575 ) ) ;
#15258=CARTESIAN_POINT ( 'NONE',  ( 190.5674408456512765, 300.5745055173924811, -0.9151048603553563199 ) ) ;
#15261=CARTESIAN_POINT ( 'NONE',  ( 196.6288634187112052, 290.0758136547079289, -16.31544900032282186 ) ) ;
#15263=CARTESIAN_POINT ( 'NONE',  ( 157.3412122618683497, 258.1240215684019290, 16.75554199904894048 ) ) ;
#15266=CARTESIAN_POINT ( 'NONE',  ( 149.7162292714551199, 271.3308795146458010, 12.12826134257344357 ) ) ;
#15275=EDGE_CURVE ( 'NONE', #99556, #19691, #39706, .T. ) ;
#15279=CARTESIAN_POINT ( 'NONE',  ( 177.8194257969418288, 292.8449071177858514, 6.006967295066290013 ) ) ;
#15280=CARTESIAN_POINT ( 'NONE',  ( 190.1730848958311810, 301.2575500587478814, 0.2415986433272204748 ) ) ;
#15281=CARTESIAN_POINT ( 'NONE',  ( 148.9719199701866899, 272.6200610409887872, 12.59512981512031438 ) ) ;
#15282=CARTESIAN_POINT ( 'NONE',  ( 171.2772883960535921, 275.5355528887071728, -15.97953745914274393 ) ) ;
#15283=CARTESIAN_POINT ( 'NONE',  ( 146.9919008828670712, 276.0495547001825116, -0.7851837772504084434 ) ) ;
#15284=CARTESIAN_POINT ( 'NONE',  ( 191.8329718516215223, 298.3825415164982928, -8.871589506312979267 ) ) ;
#15285=CARTESIAN_POINT ( 'NONE',  ( 163.4342283790118699, 257.8248486636775851, 15.55239418657778039 ) ) ;
#15287=CARTESIAN_POINT ( 'NONE',  ( -22.42236680055709641, 157.8615022471902591, 0.000000000000000000 ) ) ;
#15290=ORIENTED_EDGE ( 'NONE', *, *, #82176, .T. ) ;
#15291=CARTESIAN_POINT ( 'NONE',  ( 190.7169416771396584, 300.3155624814804128, -4.593597193813289792 ) ) ;
#15295=CARTESIAN_POINT ( 'NONE',  ( 191.9984247749195561, 297.6035878492737083, -10.02952061679425455 ) ) ;
#15297=CARTESIAN_POINT ( 'NONE',  ( 168.6359126097832473, 286.3801639820744640, -8.064224562910773386 ) ) ;
#15298=ORIENTED_EDGE ( 'NONE', *, *, #76052, .T. ) ;
#15299=CARTESIAN_POINT ( 'NONE',  ( 207.8136982414359579, 270.7031114674828700, -0.9536989003868096004 ) ) ;
#15302=CARTESIAN_POINT ( 'NONE',  ( 51.02741275436270030, 200.2677522451418781, 10.00000000000009592 ) ) ;
#15303=CARTESIAN_POINT ( 'NONE',  ( 125.9924764494033980, 252.7369531367911293, -4.594050593750048428 ) ) ;
#15304=CARTESIAN_POINT ( 'NONE',  ( 199.1526122334580862, 285.7045524820243259, -17.32174362185583050 ) ) ;
#15306=CARTESIAN_POINT ( 'NONE',  ( 196.2255671652529259, 290.7743432561995860, 16.01325193769018185 ) ) ;
#15307=CARTESIAN_POINT ( 'NONE',  ( 175.3637715581867553, 253.4841092191606435, -3.886637052182763785 ) ) ;
#15308=CARTESIAN_POINT ( 'NONE',  ( 46.94050828626382099, 210.1589784336661637, -6.496448406907675876E-16 ) ) ;
#15309=CARTESIAN_POINT ( 'NONE',  ( 178.8042996781391594, 291.7804106544875253, -6.068280820113288065 ) ) ;
#15319=FACE_OUTER_BOUND ( 'NONE', #16277, .T. ) ;
#15321=CARTESIAN_POINT ( 'NONE',  ( 116.4844995237365453, 231.3927522451418497, 10.00000000000009592 ) ) ;
#15325=B_SPLINE_CURVE_WITH_KNOTS ( 'NONE', 3,
 ( #65534, #27051, #57933, #88915, #19476, #81283, #11857, #96986, #42714, #27558, #17439, #45217, #37119, #89874, #99442, #44214, #14329, #13827, #60403, #82287, #44706, #19950, #36118, #83768, #97949, #90383, #4750, #68025, #51843, #20959, #58904, #81776, #67022, #6731, #21433, #13348, #28029, #82782, #12350, #67522, #89399, #28522, #35633, #43215, #91359, #21923, #12860, #52320, #98452, #59405 ),
 .UNSPECIFIED., .F., .F.,
 ( 4, 2, 2, 2, 2, 2, 2, 2, 2, 2, 2, 2, 2, 2, 2, 2, 2, 2, 2, 2, 2, 2, 2, 2, 4 ),
 ( 0.0007932220939086581961, 0.0009974390316302987787, 0.001099547500491155662, 0.001201655969352012545, 0.001303764438212869428, 0.001405872907073726311, 0.001610089844795440078, 0.002018523720238867610, 0.002426957595682295143, 0.003243825346569043956, 0.004060693097455792336, 0.004877560848342540716, 0.005285994723785950034, 0.005490211661507618697, 0.005592320130368408360, 0.005643374364798802757, 0.005694428599229196288, 0.005796537068089966868, 0.005898645536950736581, 0.006102862474672225701, 0.006511296350115173583, 0.006715513287836669641, 0.006919730225558166567, 0.007123947163279662625, 0.007328164101001158684 ),
 .UNSPECIFIED. ) ;
#15326=CARTESIAN_POINT ( 'NONE',  ( 163.2437751800324293, 247.9004826992694461, 9.806027032984305336 ) ) ;
#15327=CARTESIAN_POINT ( 'NONE',  ( 154.1805642697389658, 264.0898361600615090, 16.66230817378441387 ) ) ;
#15328=B_SPLINE_CURVE_WITH_KNOTS ( 'NONE', 3,
 ( #54993, #100127, #40281, #30713 ),
 .UNSPECIFIED., .F., .F.,
 ( 4, 4 ),
 ( 0.008674612601377954327, 0.01501830814127132901 ),
 .UNSPECIFIED. ) ;
#15330=CARTESIAN_POINT ( 'NONE',  ( 22.82720022358212120, 193.1744531367911293, 4.594050593750047540 ) ) ;
#15332=CARTESIAN_POINT ( 'NONE',  ( 192.1647585107599525, 272.2333635845343451, 15.21426396329954045 ) ) ;
#15333=CARTESIAN_POINT ( 'NONE',  ( 146.8358616138309571, 276.3198226421291679, 4.054088818585255716 ) ) ;
#15335=CARTESIAN_POINT ( 'NONE',  ( 175.9267864427629036, 287.0167237252017571, 10.52631150458905651 ) ) ;
#15336=CARTESIAN_POINT ( 'NONE',  ( 61.36533069198963375, 215.4244531367911293, -4.594050593750046652 ) ) ;
#15337=CARTESIAN_POINT ( 'NONE',  ( 161.1027382213887336, 251.6088674925233022, 13.55451100897754557 ) ) ;
#15342=CARTESIAN_POINT ( 'NONE',  ( 26.07505581137152006, 175.8615022471901739, 5.000000000000051514 ) ) ;
#15343=CARTESIAN_POINT ( 'NONE',  ( 164.2647213391612979, 246.1321520798662164, -5.830872732487307530 ) ) ;
#15344=CARTESIAN_POINT ( 'NONE',  ( 149.6191658661038559, 251.0643266524160140, 9.188101187500095079 ) ) ;
#15346=CARTESIAN_POINT ( 'NONE',  ( 164.1633302916340824, 260.5967636326182628, -16.15833842069452686 ) ) ;
#15347=CARTESIAN_POINT ( 'NONE',  ( 189.1076172387113843, 261.3318216691852172, 6.756518968376207468 ) ) ;
#15348=CARTESIAN_POINT ( 'NONE',  ( 205.7668501412109663, 274.2483563724483133, 11.09689540819876896 ) ) ;
#15352=VERTEX_POINT ( 'NONE', #48509 ) ;
#15354=CARTESIAN_POINT ( 'NONE',  ( 0.000000000000000000, 0.000000000000000000, 0.000000000000000000 ) ) ;
#15355=CARTESIAN_POINT ( 'NONE',  ( 181.8264173286149799, 287.9594419360853976, 13.67222989781667586 ) ) ;
#15358=ORIENTED_EDGE ( 'NONE', *, *, #55587, .F. ) ;
#15359=CARTESIAN_POINT ( 'NONE',  ( 159.8751497196749654, 253.7351131482786855, 15.29343696838486544 ) ) ;
#15361=CARTESIAN_POINT ( 'NONE',  ( 167.7953476065451639, 282.2792976936870559, -12.21232899106869851 ) ) ;
#15362=CARTESIAN_POINT ( 'NONE',  ( 204.7764732025852084, 275.9637395487929439, -14.02287343454361412 ) ) ;
#15365=CARTESIAN_POINT ( 'NONE',  ( 40.97244913529674193, 182.9155109091896065, 2.679491924311254714 ) ) ;
#15366=CARTESIAN_POINT ( 'NONE',  ( 207.6050568035884680, 271.0644890383991310, -1.456818755242089702 ) ) ;
#15367=CARTESIAN_POINT ( 'NONE',  ( 152.6873874250818517, 266.1846826352417565, -16.66598363829485763 ) ) ;
#15368=ORIENTED_EDGE ( 'NONE', *, *, #1703, .T. ) ;
#15369=CARTESIAN_POINT ( 'NONE',  ( 190.8064681396529068, 281.0104612406800015, 16.65631368068653728 ) ) ;
#15372=CARTESIAN_POINT ( 'NONE',  ( 190.8153366230912411, 300.1451374358846920, 3.771947273125533684 ) ) ;
#15374=CARTESIAN_POINT ( 'NONE',  ( 189.1789294126936340, 297.1237049920401887, 8.136854452066948795 ) ) ;
#15382=CARTESIAN_POINT ( 'NONE',  ( 103.3411068992554220, 218.2202760586659167, -5.415160957724236172E-17 ) ) ;
#15383=CARTESIAN_POINT ( 'NONE',  ( 192.6946760137320780, 261.4813915186712165, 3.932628284434791966E-12 ) ) ;
#15384=CARTESIAN_POINT ( 'NONE',  ( 150.7254409736883645, 269.5828735707850683, 14.54962197351449049 ) ) ;
#15385=CARTESIAN_POINT ( 'NONE',  ( 142.4134467818605572, 241.4824982072973967, 3.021315404115420679E-15 ) ) ;
#15386=ORIENTED_EDGE ( 'NONE', *, *, #1993, .T. ) ;
#15387=B_SPLINE_CURVE_WITH_KNOTS ( 'NONE', 3,
 ( #34826, #66731, #81977, #81481, #65726, #11563, #65238 ),
 .UNSPECIFIED., .F., .F.,
 ( 4, 3, 4 ),
 ( 0.000000000000000000, 0.001498044977021306765, 0.002672006358302393171 ),
 .UNSPECIFIED. ) ;
#15388=ORIENTED_EDGE ( 'NONE', *, *, #79719, .T. ) ;
#15389=EDGE_CURVE ( 'NONE', #44921, #87111, #42065, .T. ) ;
#15397=CARTESIAN_POINT ( 'NONE',  ( 164.2647213391612979, 246.1321520798662164, -5.830872732487307530 ) ) ;
#15399=EDGE_CURVE ( 'NONE', #49104, #29135, #5828, .T. ) ;
#15400=B_SPLINE_CURVE_WITH_KNOTS ( 'NONE', 3,
 ( #14953, #76765, #7360, #38244, #69159, #100089, #92502, #23048, #53945, #84903, #47842, #32662, #46863, #71691, #70146, #93502, #78782, #33165, #8861, #39236, #8372, #70659, #758, #63562, #77785, #94006, #31642, #40246, #86933, #23545, #54436, #85412, #71187, #62542, #55438, #64069, #85934, #1273, #86427, #32157, #16459, #16952, #95013, #24061, #1782, #9367 ),
 .UNSPECIFIED., .F., .F.,
 ( 4, 2, 2, 2, 2, 2, 2, 2, 2, 2, 2, 2, 2, 2, 2, 2, 2, 2, 2, 2, 2, 2, 4 ),
 ( 0.002967356509382767290, 0.003167624148080007852, 0.003367891786777247980, 0.003468025606125868261, 0.003568159425474488541, 0.003668293244823108822, 0.003768427064171732573, 0.003968694702869130994, 0.004168962341566530283, 0.004569497618961164062, 0.005370568173750500142, 0.006171638728539835354, 0.006972709283329171434, 0.007773779838118506647, 0.007873913657467229710, 0.007974047476815952773, 0.007999080931653133539, 0.008024114386490314305, 0.008074181296164674101, 0.008174315115513393695, 0.008574850392908331051, 0.008975385670303270141, 0.009375920947698207497 ),
 .UNSPECIFIED. ) ;
#15401=CARTESIAN_POINT ( 'NONE',  ( 167.7775688379433348, 281.0729446972871415, 11.62645973616006501 ) ) ;
#15402=EDGE_CURVE ( 'NONE', #24115, #90465, #50470, .T. ) ;
#15403=CARTESIAN_POINT ( 'NONE',  ( 148.0637215040603394, 274.1931069276759558, -7.795633835291665648 ) ) ;
#15407=LINE ( 'NONE', #46302, #38070 ) ;
#15409=CARTESIAN_POINT ( 'NONE',  ( 9.891206074601820220, 186.5177522451419065, 5.000000000000046185 ) ) ;
#15410=EDGE_LOOP ( 'NONE', ( #43278, #46679, #23857, #44056 ) ) ;
#15411=B_SPLINE_CURVE_WITH_KNOTS ( 'NONE', 3,
 ( #34011, #8688, #86748, #25385, #49200, #94821, #55756, #1095, #95353, #94326, #72001, #63386, #71007, #10200, #80134, #64896 ),
 .UNSPECIFIED., .F., .F.,
 ( 4, 2, 2, 2, 2, 2, 2, 4 ),
 ( 1.387778780781445676E-17, 0.0004582705960242376567, 0.0006874058940363459141, 0.0009165411920484541715, 0.001145676490060562212, 0.001374811788072670578, 0.001603947086084778727, 0.001833082384096887093 ),
 .UNSPECIFIED. ) ;
#15412=CARTESIAN_POINT ( 'NONE',  ( 163.3854574543125580, 247.6550818016845597, 10.82482370245618775 ) ) ;
#15416=CARTESIAN_POINT ( 'NONE',  ( 200.2631011806900005, 283.7811292041749311, 18.23377125296567058 ) ) ;
#15417=CARTESIAN_POINT ( 'NONE',  ( 194.5211191180186745, 263.4685241113479606, -0.7776144546925115586 ) ) ;
#15419=CARTESIAN_POINT ( 'NONE',  ( 155.1975950535502591, 261.8368754851878180, -18.50127729957631928 ) ) ;
#15422=CARTESIAN_POINT ( 'NONE',  ( 2.963002844326352747, 172.5177522451418781, -10.00000000000009592 ) ) ;
#15423=CARTESIAN_POINT ( 'NONE',  ( 84.07169456928664886, 219.3458772461660544, 9.188101187500095079 ) ) ;
#15425=CARTESIAN_POINT ( 'NONE',  ( 173.3452888887486552, 252.5859834778788695, -8.152990710749371317 ) ) ;
#15426=CARTESIAN_POINT ( 'NONE',  ( 169.9924644626855468, 280.7086247968809403, -14.18413335164717992 ) ) ;
#15428=CARTESIAN_POINT ( 'NONE',  ( 8.456677953475336906, 181.8149278399161233, 9.188101187500093303 ) ) ;
#15429=CARTESIAN_POINT ( 'NONE',  ( 110.9455453822464790, 234.8615022471902591, -10.00000000000009592 ) ) ;
#15431=CARTESIAN_POINT ( 'NONE',  ( 185.4344586771987338, 295.2833515559589728, 8.292135446962131340 ) ) ;
#15435=DIRECTION ( 'NONE',  ( 0.4999999999999998890, -0.8660254037844385966, 0.000000000000000000 ) ) ;
#15437=CARTESIAN_POINT ( 'NONE',  ( 205.2391015854675516, 275.1624436846170738, -14.01434138479280911 ) ) ;
#15440=CARTESIAN_POINT ( 'NONE',  ( 150.3289749894144336, 276.6211844997497451, 3.694860788824919418 ) ) ;
#15441=CARTESIAN_POINT ( 'NONE',  ( 19.44454881187291662, 182.0333772461660544, 9.188101187500095079 ) ) ;
#15442=CARTESIAN_POINT ( 'NONE',  ( 118.1174918034448922, 232.8768266524160140, 9.188101187500098632 ) ) ;
#15444=CARTESIAN_POINT ( 'NONE',  ( 183.0115390112375167, 257.7047719680322757, -2.320578905925934965 ) ) ;
#15446=CARTESIAN_POINT ( 'NONE',  ( 175.2976095297026973, 281.1217093493183938, -14.67621037160238373 ) ) ;
#15448=CARTESIAN_POINT ( 'NONE',  ( -10.27112140336314994, 171.0024278399161233, -9.188101187500093303 ) ) ;
#15449=CARTESIAN_POINT ( 'NONE',  ( 157.3412122618683497, 258.1240215684019290, 16.75554199904894048 ) ) ;
#15450=CARTESIAN_POINT ( 'NONE',  ( 194.2764122224708103, 294.1503786489221284, 15.46903869661980835 ) ) ;
#15451=CARTESIAN_POINT ( 'NONE',  ( 161.1492466472929266, 251.5283125358769212, -13.33353587056634915 ) ) ;
#15454=CARTESIAN_POINT ( 'NONE',  ( 147.6054094044680198, 274.9869267698931594, -8.596541856229405809 ) ) ;
#15455=CARTESIAN_POINT ( 'NONE',  ( 190.4966860832860220, 262.7064732693366409, 8.377472714625252337 ) ) ;
#15456=CARTESIAN_POINT ( 'NONE',  ( 171.6100400556340162, 279.8152386110159000, 13.99908611435833983 ) ) ;
#15457=CARTESIAN_POINT ( 'NONE',  ( 185.4867332780130766, 297.4061142773095412, 5.671143563000668131 ) ) ;
#15459=CARTESIAN_POINT ( 'NONE',  ( 190.5969391768923913, 300.5234129089444650, -0.7564693504096553500 ) ) ;
#15460=CARTESIAN_POINT ( 'NONE',  ( 180.7719503181222080, 266.8161623102827775, -14.72789016211928370 ) ) ;
#15464=CARTESIAN_POINT ( 'NONE',  ( 207.5230514910949182, 271.2065264061283756, 2.678931747975364708 ) ) ;
#15465=CARTESIAN_POINT ( 'NONE',  ( 184.9512090389555397, 269.4173353161797877, 15.97780096459446320 ) ) ;
#15467=CARTESIAN_POINT ( 'NONE',  ( 97.03527265400872182, 217.6423013555409796, -4.594050593750043987 ) ) ;
#15469=CARTESIAN_POINT ( 'NONE',  ( 151.2057546125658973, 268.7509459446807227, 15.78031848731319187 ) ) ;
#15472=CARTESIAN_POINT ( 'NONE',  ( 194.7690439115086178, 278.9149514252409290, 16.30030903610881055 ) ) ;
#15473=CARTESIAN_POINT ( 'NONE',  ( 202.2429319221604374, 271.5051878758352473, -9.789492590983266851 ) ) ;
#15474=CARTESIAN_POINT ( 'NONE',  ( 151.0426280674448378, 269.0334894088936153, -15.84467774422408581 ) ) ;
#15476=CARTESIAN_POINT ( 'NONE',  ( 57.25197034761130510, 193.8615022471901739, 5.000000000000051514 ) ) ;
#15480=CARTESIAN_POINT ( 'NONE',  ( 163.6671909760687527, 256.2992013055660436, -14.91259676482536456 ) ) ;
#15482=CARTESIAN_POINT ( 'NONE',  ( 198.2505066714982149, 285.2670451491296149, 0.000000000000000000 ) ) ;
#15483=CARTESIAN_POINT ( 'NONE',  ( 160.8891438268352374, 281.0495864612497599, 9.578199528566821996 ) ) ;
#15485=ORIENTED_EDGE ( 'NONE', *, *, #44110, .T. ) ;
#15486=CARTESIAN_POINT ( 'NONE',  ( 152.8239686330211953, 275.0022943016427348, 10.78622480446937537 ) ) ;
#15487=DIRECTION ( 'NONE',  ( 0.4999999999999998335, -0.8660254037844388186, 0.000000000000000000 ) ) ;
#15488=CARTESIAN_POINT ( 'NONE',  ( 179.9008876211633492, 262.7362030500133301, -12.76817184108253223 ) ) ;
#15489=CARTESIAN_POINT ( 'NONE',  ( 169.3738444220689416, 252.1525573315904296, -8.754927670012239815 ) ) ;
#15490=CARTESIAN_POINT ( 'NONE',  ( 192.3606619183491091, 297.4685555102766443, 10.99569063633359889 ) ) ;
#15492=B_SPLINE_CURVE_WITH_KNOTS ( 'NONE', 3,
 ( #95147, #19124, #49999, #73310 ),
 .UNSPECIFIED., .F., .F.,
 ( 4, 4 ),
 ( 0.02338672457796607887, 0.03261727987500769727 ),
 .UNSPECIFIED. ) ;
#15493=CARTESIAN_POINT ( 'NONE',  ( 187.5741477178530374, 278.9861021591872259, 17.66168452547810475 ) ) ;
#15496=CARTESIAN_POINT ( 'NONE',  ( 178.2005841394030199, 289.7860138253658420, 11.11017618330963508 ) ) ;
#15498=ORIENTED_EDGE ( 'NONE', *, *, #63187, .F. ) ;
#15502=CARTESIAN_POINT ( 'NONE',  ( 153.3124474400112831, 265.1020469316042636, -17.30303149702894316 ) ) ;
#15508=ORIENTED_EDGE ( 'NONE', *, *, #45457, .F. ) ;
#15509=CARTESIAN_POINT ( 'NONE',  ( 196.1763519989319775, 290.2392196892972720, 16.27711669441661613 ) ) ;
#15513=CARTESIAN_POINT ( 'NONE',  ( 169.3676301360849550, 269.0840628972123341, 17.25023024943055461 ) ) ;
#15514=ORIENTED_EDGE ( 'NONE', *, *, #81979, .T. ) ;
#15515=CARTESIAN_POINT ( 'NONE',  ( 190.2731979903009858, 300.2022605500126815, -3.404760317914321988 ) ) ;
#15516=CARTESIAN_POINT ( 'NONE',  ( 205.9447606851647947, 273.9402062711180861, -10.75123264850128102 ) ) ;
#15517=CARTESIAN_POINT ( 'NONE',  ( 197.5123600491583034, 273.2865668918312281, -13.38184978029139671 ) ) ;
#15520=CARTESIAN_POINT ( 'NONE',  ( 171.6426604480640776, 250.7983711109617673, -5.691410925449850389 ) ) ;
#15522=DIRECTION ( 'NONE',  ( 0.4999999999999992784, -0.8660254037844390407, 0.000000000000000000 ) ) ;
#15523=CARTESIAN_POINT ( 'NONE',  ( 183.6291305219023968, 284.8155054853089609, -15.01443082426404985 ) ) ;
#15524=CARTESIAN_POINT ( 'NONE',  ( 120.7155680147981940, 234.3768266524159856, 9.188101187500098632 ) ) ;
#15525=CARTESIAN_POINT ( 'NONE',  ( 184.5558809902196344, 261.3976952126757851, -9.110542280346439981 ) ) ;
#15527=CARTESIAN_POINT ( 'NONE',  ( 177.3582130212591608, 288.8584996472486068, -9.346563926071064898 ) ) ;
#15533=CARTESIAN_POINT ( 'NONE',  ( 192.1032606970431971, 297.9143875035085784, 11.39438513385636043 ) ) ;
#15536=CARTESIAN_POINT ( 'NONE',  ( 177.1467926689314538, 288.7641837594472349, -9.305349299006246966 ) ) ;
#15541=CARTESIAN_POINT ( 'NONE',  ( 194.7576540903134799, 293.3168432830895540, -14.62421624641040196 ) ) ;
#15545=CARTESIAN_POINT ( 'NONE',  ( 158.2756371360163143, 277.3693515115958235, 10.25742348846014984 ) ) ;
#15547=CARTESIAN_POINT ( 'NONE',  ( 190.0667283601964357, 259.9641452334862493, -5.090329199819447104E-14 ) ) ;
#15548=CARTESIAN_POINT ( 'NONE',  ( 163.0683798854284703, 248.2042762609320903, 11.26611642476872710 ) ) ;
#15551=CARTESIAN_POINT ( 'NONE',  ( 152.8328714238065515, 265.9326969577624027, -16.29536156676786263 ) ) ;
#15553=CARTESIAN_POINT ( 'NONE',  ( 190.1813752874636805, 301.2431906792259042, -4.710625539811892359 ) ) ;
#15554=CARTESIAN_POINT ( 'NONE',  ( 170.6178593158246315, 266.5408558992322696, -17.65857870869936974 ) ) ;
#15555=CARTESIAN_POINT ( 'NONE',  ( 186.7785090572402282, 262.7977421546021333, -9.006081414252482986 ) ) ;
#15556=CARTESIAN_POINT ( 'NONE',  ( 182.7953794973296056, 276.1600416569049230, -16.45808333016647040 ) ) ;
#15558=CARTESIAN_POINT ( 'NONE',  ( 192.7870477231578548, 271.6154284180436775, -14.94562697032598741 ) ) ;
#15559=CARTESIAN_POINT ( 'NONE',  ( 164.0781508658037637, 275.4055464209769752, 15.63836535835214114 ) ) ;
#15561=CARTESIAN_POINT ( 'NONE',  ( 27.30738562583555762, 198.1199935810940929, 2.679491924311251605 ) ) ;
#15565=CARTESIAN_POINT ( 'NONE',  ( 68.21243081460160340, 216.3149278399160664, 9.188101187500093303 ) ) ;
#15567=CARTESIAN_POINT ( 'NONE',  ( 192.5076277540105423, 297.2140032159341558, -13.10094381206144298 ) ) ;
#15568=CARTESIAN_POINT ( 'NONE',  ( 50.32376711733572705, 209.8615022471902876, 5.000000000000046185 ) ) ;
#15569=CARTESIAN_POINT ( 'NONE',  ( 154.8786460229866577, 262.3893114111486398, -18.06164891362396929 ) ) ;
#15570=VECTOR ( 'NONE', #66865, 1000.000000000000000 ) ;
#15572=CARTESIAN_POINT ( 'NONE',  ( 207.2707369601997982, 271.6435479931266173, -5.381413637561199614 ) ) ;
#15578=CARTESIAN_POINT ( 'NONE',  ( 169.5608527833963421, 251.6396950762901952, -9.960993533446050208 ) ) ;
#15579=CARTESIAN_POINT ( 'NONE',  ( 164.7508860646548783, 245.2900900744633930, -5.203382148009804808 ) ) ;
#15580=CARTESIAN_POINT ( 'NONE',  ( 157.0935036675524827, 258.5530654392286465, 17.32636058289560665 ) ) ;
#15583=EDGE_CURVE ( 'NONE', #11680, #75397, #15492, .T. ) ;
#15584=CARTESIAN_POINT ( 'NONE',  ( 161.8408514536557163, 250.3304178724980318, -14.12919723462510646 ) ) ;
#15585=CARTESIAN_POINT ( 'NONE',  ( 35.38456857845647363, 200.4244531367911293, -4.594050593750046652 ) ) ;
#15587=CARTESIAN_POINT ( 'NONE',  ( 49.32242524243604720, 199.2833772461660828, -9.188101187500095079 ) ) ;
#15591=CARTESIAN_POINT ( 'NONE',  ( 146.0739611433025686, 245.9548013555409796, -4.594050593750042211 ) ) ;
#15593=CARTESIAN_POINT ( 'NONE',  ( 14.65434579541623172, 189.2677522451419065, -5.000000000000047962 ) ) ;
#15595=CARTESIAN_POINT ( 'NONE',  ( -4.215479392844351914, 156.8262482093458061, -4.415768667553307481E-15 ) ) ;
#15596=CARTESIAN_POINT ( 'NONE',  ( 149.1939152435731728, 272.2355539484436235, -11.44223522189843933 ) ) ;
#15598=CARTESIAN_POINT ( 'NONE',  ( 59.55217677675724275, 211.3149278399160949, -9.188101187500095079 ) ) ;
#15602=CARTESIAN_POINT ( 'NONE',  ( 198.2040940955416488, 287.3474340887963763, 16.95806375232200480 ) ) ;
#15604=CARTESIAN_POINT ( 'NONE',  ( 153.2966090711206846, 276.8115077458087399, 7.191393513384046088 ) ) ;
#15605=AXIS2_PLACEMENT_3D ( 'NONE', #84424, #14970, #45857 ) ;
#15608=CARTESIAN_POINT ( 'NONE',  ( 110.9455453822464790, 234.8615022471902591, -10.00000000000009592 ) ) ;
#15609=CARTESIAN_POINT ( 'NONE',  ( 200.6800100461949228, 283.0590218669948399, 18.32402613046234308 ) ) ;
#15610=CARTESIAN_POINT ( 'NONE',  ( 164.3706594650489023, 245.9486618633701482, -1.665857659249071698 ) ) ;
#15611=ORIENTED_EDGE ( 'NONE', *, *, #38962, .F. ) ;
#15613=CARTESIAN_POINT ( 'NONE',  ( 200.2093391412865060, 269.7417714514684803, 10.46510648850140157 ) ) ;
#15615=CARTESIAN_POINT ( 'NONE',  ( 206.2313482792274328, 273.4438219973828268, -9.403385562213845361 ) ) ;
#15616=CARTESIAN_POINT ( 'NONE',  ( 193.6523268064705974, 293.2313262976975352, 15.26490498002906193 ) ) ;
#15619=CARTESIAN_POINT ( 'NONE',  ( 173.3120886762449686, 251.6182065839331301, 0.03490652146819783752 ) ) ;
#15622=CARTESIAN_POINT ( 'NONE',  ( 147.9133274879049793, 274.4535970048112290, -9.359166267164972908 ) ) ;
#15623=FACE_OUTER_BOUND ( 'NONE', #6696, .T. ) ;
#15627=CARTESIAN_POINT ( 'NONE',  ( 156.9763224152064822, 271.9908631200777904, -15.29896765642516776 ) ) ;
#15628=CARTESIAN_POINT ( 'NONE',  ( 6.406750531224583156, 186.0530062829863027, -4.648177544792955347E-16 ) ) ;
#15632=CARTESIAN_POINT ( 'NONE',  ( 140.3904091109174317, 241.8615022471902023, 5.000000000000051514 ) ) ;
#15634=ORIENTED_EDGE ( 'NONE', *, *, #93815, .F. ) ;
#15635=EDGE_CURVE ( 'NONE', #4619, #11450, #78327, .T. ) ;
#15636=CARTESIAN_POINT ( 'NONE',  ( 172.1836633629298206, 284.9661130839314751, 10.60870986581373820 ) ) ;
#15640=CARTESIAN_POINT ( 'NONE',  ( 163.9942050550062049, 246.6007000282974673, 5.791111691696777974 ) ) ;
#15641=CARTESIAN_POINT ( 'NONE',  ( 187.1243084772174825, 293.7649743884641111, -10.81561194776973700 ) ) ;
#15642=CARTESIAN_POINT ( 'NONE',  ( 164.3068057902571582, 265.7701674460021195, -17.51175939818463334 ) ) ;
#15643=CARTESIAN_POINT ( 'NONE',  ( 140.2550926398021147, 251.7833772461660544, -9.188101187500095079 ) ) ;
#15644=EDGE_CURVE ( 'NONE', #90262, #94724, #57851, .T. ) ;
#15646=CARTESIAN_POINT ( 'NONE',  ( 179.3255745279743394, 258.5940977613889231, 9.670503133756291447 ) ) ;
#15647=CARTESIAN_POINT ( 'NONE',  ( 66.23672358827711548, 218.2369531367911293, -4.594050593750048428 ) ) ;
#15649=CARTESIAN_POINT ( 'NONE',  ( 151.0715479399129606, 268.9833987204304435, 14.24612252017116987 ) ) ;
#15653=ORIENTED_EDGE ( 'NONE', *, *, #2576, .T. ) ;
#15654=CARTESIAN_POINT ( 'NONE',  ( 157.4139724630872195, 257.9979972031215425, -18.09067551972931653 ) ) ;
#15655=AXIS2_PLACEMENT_3D ( 'NONE', #48174, #25897, #56263 ) ;
#15656=ORIENTED_EDGE ( 'NONE', *, *, #56489, .F. ) ;
#15657=ORIENTED_EDGE ( 'NONE', *, *, #16416, .F. ) ;
#15658=EDGE_CURVE ( 'NONE', #21882, #85237, #52365, .T. ) ;
#15661=CARTESIAN_POINT ( 'NONE',  ( 197.8751239397817301, 286.8074493601922654, 16.93281720670876922 ) ) ;
#15662=CARTESIAN_POINT ( 'NONE',  ( 191.1192699377806719, 299.6187094927299199, -9.526914969203620132 ) ) ;
#15667=CARTESIAN_POINT ( 'NONE',  ( 81.01380268399661588, 208.3923013555409796, 4.594050593750050204 ) ) ;
#15675=CARTESIAN_POINT ( 'NONE',  ( 164.4573439719129340, 245.7985198932525748, 1.541132361166968501 ) ) ;
#15678=CARTESIAN_POINT ( 'NONE',  ( 207.3895038639124095, 270.9794483157102150, -1.916867053770541007 ) ) ;
#15679=CARTESIAN_POINT ( 'NONE',  ( 147.4771145948261051, 275.6046598944997186, -0.0007385123558252784009 ) ) ;
#15680=VERTEX_POINT ( 'NONE', #11406 ) ;
#15683=CARTESIAN_POINT ( 'NONE',  ( 185.3858643910043327, 260.1458795028655118, 6.052290864491880029 ) ) ;
#15685=CARTESIAN_POINT ( 'NONE',  ( 153.3859906278383676, 264.9746663937372091, -17.41799046551451013 ) ) ;
#15686=AXIS2_PLACEMENT_3D ( 'NONE', #27385, #58270, #89246 ) ;
#15690=CARTESIAN_POINT ( 'NONE',  ( 147.7917198021585534, 275.6304213403500398, -3.790807063116589770 ) ) ;
#15692=CARTESIAN_POINT ( 'NONE',  ( 188.2520712372829621, 265.6420100395978920, -13.17850047611677766 ) ) ;
#15695=EDGE_LOOP ( 'NONE', ( #10930, #76813, #79490, #432 ) ) ;
#15697=EDGE_CURVE ( 'NONE', #19691, #53889, #56599, .T. ) ;
#15698=CARTESIAN_POINT ( 'NONE',  ( 157.8043799545718286, 257.3217915922150496, -17.97575562758749257 ) ) ;
#15699=CARTESIAN_POINT ( 'NONE',  ( 155.6276701977099890, 261.0919634844306643, 17.49722577287685255 ) ) ;
#15701=CARTESIAN_POINT ( 'NONE',  ( 60.28305926085675992, 215.6115022471903160, -5.000000000000047962 ) ) ;
#15706=CARTESIAN_POINT ( 'NONE',  ( 192.2580028094575653, 262.1757339090664800, 3.009676160147899182 ) ) ;
#15707=CARTESIAN_POINT ( 'NONE',  ( -10.94779052401099051, 173.6744531367911293, 4.594050593750047540 ) ) ;
#15708=CARTESIAN_POINT ( 'NONE',  ( 191.6148588865760871, 296.7603242537468873, -11.89382487812838995 ) ) ;
#15709=VERTEX_POINT ( 'NONE', #10389 ) ;
#15710=EDGE_CURVE ( 'NONE', #41871, #16265, #9413, .T. ) ;
#15711=CARTESIAN_POINT ( 'NONE',  ( 174.8527186269040783, 255.3323168797083156, 8.645391441763411677 ) ) ;
#15714=CARTESIAN_POINT ( 'NONE',  ( 28.21305602519035460, 187.0958772461660544, -9.188101187500095079 ) ) ;
#15717=CARTESIAN_POINT ( 'NONE',  ( 181.9564645032531018, 275.7194610820193361, -16.43226933849268789 ) ) ;
#15719=CARTESIAN_POINT ( 'NONE',  ( 125.2349645446897171, 243.1115022471902591, 10.00000000000009592 ) ) ;
#15720=CARTESIAN_POINT ( 'NONE',  ( 170.1675564235169418, 270.7386499948772780, -16.98440315941436651 ) ) ;
#15722=CARTESIAN_POINT ( 'NONE',  ( 138.0629658346988151, 250.5177522451418213, -10.00000000000009592 ) ) ;
#15725=CARTESIAN_POINT ( 'NONE',  ( 164.5546760946605787, 285.7985264595317290, -4.260912962880108346 ) ) ;
#15728=CARTESIAN_POINT ( 'NONE',  ( 68.07728789491670796, 220.1115022471903160, -5.000000000000047962 ) ) ;
#15729=CYLINDRICAL_SURFACE ( 'NONE', #33679, 17.82106496071139645 ) ;
#15730=CARTESIAN_POINT ( 'NONE',  ( 35.46636587765004123, 179.0327760586659736, 1.948934522072303157E-15 ) ) ;
#15733=CARTESIAN_POINT ( 'NONE',  ( 151.4428545556028780, 268.3402767968688067, -15.03309903163500749 ) ) ;
#15735=CARTESIAN_POINT ( 'NONE',  ( 162.5812779487254147, 280.2977391392396953, -9.910640860102120087 ) ) ;
#15736=CARTESIAN_POINT ( 'NONE',  ( 163.7166294601506991, 282.3380383384618995, 10.03031969300557513 ) ) ;
#15738=CARTESIAN_POINT ( 'NONE',  ( 190.2476911738421848, 301.1283281946692796, -1.360079143321618611 ) ) ;
#15740=CARTESIAN_POINT ( 'NONE',  ( 188.8132345201846931, 270.2707858497124676, -15.13545237428995094 ) ) ;
#15741=EDGE_LOOP ( 'NONE', ( #2451, #44939, #62871, #19315 ) ) ;
#15745=CARTESIAN_POINT ( 'NONE',  ( 198.4097421844162170, 265.0824675037606539, -3.039349057205883664 ) ) ;
#15748=CARTESIAN_POINT ( 'NONE',  ( 161.3261849411383650, 273.2032229615781489, 15.91718547624222957 ) ) ;
#15751=CARTESIAN_POINT ( 'NONE',  ( 172.0418500013140033, 261.1904116954747224, 16.05919355830004847 ) ) ;
#15754=EDGE_LOOP ( 'NONE', ( #86624, #73741, #30060, #69024 ) ) ;
#15755=VERTEX_POINT ( 'NONE', #26588 ) ;
#15758=CARTESIAN_POINT ( 'NONE',  ( 202.0119585509590934, 280.0399447494788205, 15.93797677053798623 ) ) ;
#15761=CARTESIAN_POINT ( 'NONE',  ( 201.4066285247549786, 281.8004817444100354, -17.79749223817309201 ) ) ;
#15765=ORIENTED_EDGE ( 'NONE', *, *, #37760, .F. ) ;
#15766=CARTESIAN_POINT ( 'NONE',  ( 189.8171280724701546, 301.8740853621098950, -0.4360232994423257624 ) ) ;
#15770=CARTESIAN_POINT ( 'NONE',  ( 195.8248271798537417, 291.4684452715354155, 17.35175160929494709 ) ) ;
#15771=EDGE_CURVE ( 'NONE', #30236, #68451, #3523, .T. ) ;
#15772=CARTESIAN_POINT ( 'NONE',  ( 164.2090401137261892, 246.2285947913476889, -5.787448100099915393 ) ) ;
#15779=CARTESIAN_POINT ( 'NONE',  ( 159.7588695950563817, 254.4119446770600064, 15.33386816469749903 ) ) ;
#15782=ORIENTED_EDGE ( 'NONE', *, *, #99902, .F. ) ;
#15786=CARTESIAN_POINT ( 'NONE',  ( 190.4750160083620472, 300.7345900314585947, -1.159659205620361400 ) ) ;
#15788=EDGE_LOOP ( 'NONE', ( #84141, #91108, #7710 ) ) ;
#15789=CARTESIAN_POINT ( 'NONE',  ( 149.6896757981861583, 271.3768714794653647, 12.49809796062302603 ) ) ;
#15790=CARTESIAN_POINT ( 'NONE',  ( 170.7330658761331676, 275.4497203906630602, -16.60568353338077685 ) ) ;
#15791=CARTESIAN_POINT ( 'NONE',  ( 161.8935665241663457, 250.2391126920490194, -13.69501063978231770 ) ) ;
#15792=CARTESIAN_POINT ( 'NONE',  ( 147.5749551500760788, 275.0396750858066639, -4.254929048021584670 ) ) ;
#15793=CARTESIAN_POINT ( 'NONE',  ( 161.3390181621638533, 256.5413485146231096, 15.77656010779211826 ) ) ;
#15796=CARTESIAN_POINT ( 'NONE',  ( 88.35671610020233402, 228.4865022471903160, 10.00000000000009415 ) ) ;
#15801=CARTESIAN_POINT ( 'NONE',  ( 115.8441751185107478, 231.5643266524159856, 9.188101187500095079 ) ) ;
#15802=ORIENTED_EDGE ( 'NONE', *, *, #61947, .F. ) ;
#15803=CARTESIAN_POINT ( 'NONE',  ( 191.1747001918821525, 299.5227014763493116, -9.654804683100723040 ) ) ;
#15809=CARTESIAN_POINT ( 'NONE',  ( 167.1442095974935569, 284.0302014969162769, -8.032154302468351048 ) ) ;
#15812=AXIS2_PLACEMENT_3D ( 'NONE', #74680, #57950, #5256 ) ;
#15814=CARTESIAN_POINT ( 'NONE',  ( 44.53222222597941027, 196.5177522451418781, -10.00000000000009592 ) ) ;
#15815=CARTESIAN_POINT ( 'NONE',  ( 134.5719744753492364, 242.3768266524160140, -9.188101187500093303 ) ) ;
#15816=CARTESIAN_POINT ( 'NONE',  ( 189.7493380202622291, 294.8126471784881915, -12.68491631734921299 ) ) ;
#15818=CARTESIAN_POINT ( 'NONE',  ( 186.1974923302803973, 296.9264864461521256, 4.665697376584795109 ) ) ;
#15819=CARTESIAN_POINT ( 'NONE',  ( 187.6338304778425936, 281.4993805173464807, -17.52881113060309204 ) ) ;
#15821=CARTESIAN_POINT ( 'NONE',  ( 52.54321753458319932, 191.9548013555410080, -4.594050593750042211 ) ) ;
#15827=CARTESIAN_POINT ( 'NONE',  ( 155.8152618860606253, 260.7670451491295012, 0.000000000000000000 ) ) ;
#15829=CARTESIAN_POINT ( 'NONE',  ( 151.3159053224887600, 278.6181574046168521, -1.690837018209672582 ) ) ;
#15830=CARTESIAN_POINT ( 'NONE',  ( 183.5794699052420071, 296.1068241588955061, -6.177496795926971984 ) ) ;
#15831=CARTESIAN_POINT ( 'NONE',  ( 178.4121483706975653, 261.1686503152587875, 12.25625725717337744 ) ) ;
#15833=CARTESIAN_POINT ( 'NONE',  ( 115.9793180381956716, 227.7677522451417929, -5.000000000000041744 ) ) ;
#15834=DIRECTION ( 'NONE',  ( 0.5000000000000048850, -0.8660254037844358210, 0.000000000000000000 ) ) ;
#15837=CARTESIAN_POINT ( 'NONE',  ( 202.4017613376760494, 280.0768611521521620, 15.73960524502980540 ) ) ;
#15839=CARTESIAN_POINT ( 'NONE',  ( 38.38920161542251464, 180.7202760586659451, -5.415160957724236172E-17 ) ) ;
#15844=CARTESIAN_POINT ( 'NONE',  ( 195.1280934431195249, 275.0822181618672175, -16.22170959459208461 ) ) ;
#15845=CARTESIAN_POINT ( 'NONE',  ( 67.34675250658217749, 203.5643266524159856, -9.188101187500093303 ) ) ;
#15846=CARTESIAN_POINT ( 'NONE',  ( 161.0952649348064938, 251.6218116045831437, 13.81854265722852482 ) ) ;
#15848=ADVANCED_FACE ( 'NONE', ( #67060 ), #55811, .F. ) ;
#15851=( BOUNDED_CURVE ( )  B_SPLINE_CURVE ( 2, ( #50532, #26752, #33875, #56128, #95198, #11567, #81489, #72880, #34349 ),
 .UNSPECIFIED., .F., .T. ) 
 B_SPLINE_CURVE_WITH_KNOTS ( ( 3, 2, 2, 2, 3 ),
 ( 0.3830645161290322509, 0.3844086021505376261, 0.3870967741935483764, 0.3897849462365591267, 0.3911290322580645018 ),
 .UNSPECIFIED. ) 
 CURVE ( )  GEOMETRIC_REPRESENTATION_ITEM ( )  RATIONAL_B_SPLINE_CURVE ( ( 0.9330127018922194093, 0.9330127018922194093, 1.000000000000000000, 0.8660254037844387076, 1.000000000000000000, 0.8660254037844387076, 1.000000000000000000, 0.9330127018922194093, 0.9330127018922194093 ) ) 
 REPRESENTATION_ITEM ( '' )  );
#15853=ADVANCED_FACE ( 'NONE', ( #41515 ), #91905, .T. ) ;
#15854=CARTESIAN_POINT ( 'NONE',  ( 164.5236374827232169, 268.7060415519879371, 16.63096613792822254 ) ) ;
#15855=CARTESIAN_POINT ( 'NONE',  ( 38.12724268070496692, 179.4865022471901455, 1.119607411625061291E-15 ) ) ;
#15856=CARTESIAN_POINT ( 'NONE',  ( 163.0309151244508712, 248.2691671304387739, 11.27270415168660200 ) ) ;
#15857=CARTESIAN_POINT ( 'NONE',  ( 147.8871150585349881, 250.0643266524159287, -9.188101187500093303 ) ) ;
#15859=CARTESIAN_POINT ( 'NONE',  ( 164.0938789702753411, 260.4145277690955140, -16.14174696660529307 ) ) ;
#15860=CARTESIAN_POINT ( 'NONE',  ( 188.9667663523237024, 261.8616926428981628, 6.534948879020797463 ) ) ;
#15861=CARTESIAN_POINT ( 'NONE',  ( 164.5648480107187197, 245.6123174360222094, 3.015887571020871238 ) ) ;
#15867=CARTESIAN_POINT ( 'NONE',  ( 149.7543087857887656, 247.2677522451417929, -5.000000000000041744 ) ) ;
#15868=CARTESIAN_POINT ( 'NONE',  ( -27.42236680055714260, 166.5217562850347406, 1.224646799147364892E-15 ) ) ;
#15870=ORIENTED_EDGE ( 'NONE', *, *, #22958, .T. ) ;
#15871=CARTESIAN_POINT ( 'NONE',  ( 206.9645602195919025, 272.1738616639552220, 7.969428354269253667 ) ) ;
#15874=CARTESIAN_POINT ( 'NONE',  ( 152.8107382695299918, 265.9710327055011589, 16.32045346488711246 ) ) ;
#15875=FACE_OUTER_BOUND ( 'NONE', #41022, .T. ) ;
#15876=CARTESIAN_POINT ( 'NONE',  ( 163.4218292706009095, 247.5920839679097014, -10.44611490715852042 ) ) ;
#15877=CARTESIAN_POINT ( 'NONE',  ( 200.9061540366740246, 282.6673289856585143, -18.13083321883407351 ) ) ;
#15878=ORIENTED_EDGE ( 'NONE', *, *, #69578, .T. ) ;
#15881=ADVANCED_FACE ( 'NONE', ( #49136 ), #56676, .F. ) ;
#15884=ORIENTED_EDGE ( 'NONE', *, *, #22472, .T. ) ;
#15896=CARTESIAN_POINT ( 'NONE',  ( 203.6828132253460240, 277.8580141955760041, 15.80358291857228359 ) ) ;
#15897=CARTESIAN_POINT ( 'NONE',  ( 137.7923328995641157, 240.3615022471902023, 5.000000000000051514 ) ) ;
#15898=CARTESIAN_POINT ( 'NONE',  ( 191.5544531425776427, 298.8649500714207647, 8.366689293739112188 ) ) ;
#15899=CARTESIAN_POINT ( 'NONE',  ( 102.3056452726415984, 218.3262482093457493, 3.021315404115420679E-15 ) ) ;
#15903=EDGE_LOOP ( 'NONE', ( #74102, #22754, #32143, #46101 ) ) ;
#15904=EDGE_LOOP ( 'NONE', ( #34238, #21935, #8811, #86497 ) ) ;
#15906=VERTEX_POINT ( 'NONE', #82072 ) ;
#15909=CARTESIAN_POINT ( 'NONE',  ( 208.0045976720423084, 270.3724639545367836, 2.002128742561712471 ) ) ;
#15912=CARTESIAN_POINT ( 'NONE',  ( 165.0407670381244145, 270.9616198530111433, 16.81988890767253864 ) ) ;
#15913=DIRECTION ( 'NONE',  ( 0.4999999999999998890, -0.8660254037844385966, 0.000000000000000000 ) ) ;
#15914=CARTESIAN_POINT ( 'NONE',  ( 148.2352135776142177, 273.8960739431854563, -9.245976304249309052 ) ) ;
#15915=CARTESIAN_POINT ( 'NONE',  ( 174.6053779230379632, 290.0266613665239106, 6.313546118724348233 ) ) ;
#15916=CARTESIAN_POINT ( 'NONE',  ( 158.9428945936735715, 255.3498263921298985, -17.51518199015400512 ) ) ;
#15920=FACE_OUTER_BOUND ( 'NONE', #45808, .T. ) ;
#15922=CARTESIAN_POINT ( 'NONE',  ( 198.3449891235413531, 287.1033967417670283, 16.95540786497457120 ) ) ;
#15924=CARTESIAN_POINT ( 'NONE',  ( 191.1269952354458610, 299.6053288846700866, 6.026773553208284007 ) ) ;
#15926=CARTESIAN_POINT ( 'NONE',  ( 159.5221561062548972, 254.3465160214695118, -16.91023001054109542 ) ) ;
#15927=DIRECTION ( 'NONE',  ( 0.4999999999999998890, -0.8660254037844385966, 0.000000000000000000 ) ) ;
#15930=CARTESIAN_POINT ( 'NONE',  ( 170.8004095096928836, 255.2646207969754357, 11.24633423646908703 ) ) ;
#15931=CARTESIAN_POINT ( 'NONE',  ( 159.4594236750365326, 281.8839243825340191, 2.078914130625487910 ) ) ;
#15933=CARTESIAN_POINT ( 'NONE',  ( 155.7713280489876695, 260.8431407871109968, -18.06005460683174491 ) ) ;
#15934=CARTESIAN_POINT ( 'NONE',  ( -22.42236680055709641, 157.8615022471902591, 0.000000000000000000 ) ) ;
#15935=DIRECTION ( 'NONE',  ( 0.4999999999999992784, -0.8660254037844390407, 0.000000000000000000 ) ) ;
#15937=CARTESIAN_POINT ( 'NONE',  ( 3.035171627975005837, 185.8927522451419350, 2.944929066748280225E-16 ) ) ;
#15938=CARTESIAN_POINT ( 'NONE',  ( 91.59511671678144751, 229.8149278399160949, 9.188101187500093303 ) ) ;
#15941=DIRECTION ( 'NONE',  ( -0.8660254037844392627, -0.4999999999999987232, 0.000000000000000000 ) ) ;
#15942=CARTESIAN_POINT ( 'NONE',  ( 164.0095377641384857, 246.5741429970625802, -8.745455945562961020 ) ) ;
#15945=CARTESIAN_POINT ( 'NONE',  ( 5.858601742122021783, 180.3149278399161233, 9.188101187500093303 ) ) ;
#15947=CARTESIAN_POINT ( 'NONE',  ( 181.4577051398952108, 255.5722452524177299, 4.229640769421640911 ) ) ;
#15952=CARTESIAN_POINT ( 'NONE',  ( 201.3212028412432062, 267.0810577319301160, -3.784738031960614091 ) ) ;
#15953=DIRECTION ( 'NONE',  ( 0.4999999999999998890, -0.8660254037844385966, 0.000000000000000000 ) ) ;
#15954=CARTESIAN_POINT ( 'NONE',  ( 202.7185166046502331, 279.5282249361877120, -16.86058306256609640 ) ) ;
#15956=CARTESIAN_POINT ( 'NONE',  ( 94.62744204236609846, 213.8932355074535394, -2.679491924311248496 ) ) ;
#15957=CARTESIAN_POINT ( 'NONE',  ( 169.8466615877324841, 251.3021325278160134, 9.294982655322041154 ) ) ;
#15958=CARTESIAN_POINT ( 'NONE',  ( 35.03300607999280913, 191.0333772461660544, 9.188101187500095079 ) ) ;
#15959=CARTESIAN_POINT ( 'NONE',  ( 122.7720312530212396, 247.8149278399160949, 9.188101187500093303 ) ) ;
#15961=ORIENTED_EDGE ( 'NONE', *, *, #18900, .T. ) ;
#15962=CARTESIAN_POINT ( 'NONE',  ( 150.4814168194272099, 271.9348575896366924, -11.67596527614399982 ) ) ;
#15963=FACE_OUTER_BOUND ( 'NONE', #69956, .T. ) ;
#15965=CARTESIAN_POINT ( 'NONE',  ( 170.3178023250738420, 289.0326318653803241, -4.561300590322002080 ) ) ;
#15967=CARTESIAN_POINT ( 'NONE',  ( 193.9844289374573520, 294.6561085335266625, 15.49818881749970245 ) ) ;
#15968=CARTESIAN_POINT ( 'NONE',  ( 207.8232941427535536, 270.6864908788566026, -6.505149060073906142 ) ) ;
#15969=CARTESIAN_POINT ( 'NONE',  ( 194.3442947553755005, 294.0328026529847421, -15.97648891113594871 ) ) ;
#15970=CARTESIAN_POINT ( 'NONE',  ( 148.3874010092782498, 273.6324775792697892, -8.328854486678444857 ) ) ;
#15973=CARTESIAN_POINT ( 'NONE',  ( -22.42236680055709641, 157.8615022471902591, 0.000000000000000000 ) ) ;
#15974=ADVANCED_FACE ( 'NONE', ( #47011 ), #54585, .T. ) ;
#15976=CARTESIAN_POINT ( 'NONE',  ( 190.0515794655415789, 301.4680036374047063, -1.296825456579539626 ) ) ;
#15977=B_SPLINE_CURVE_WITH_KNOTS ( 'NONE', 3,
 ( #12803, #43667, #19421, #35073, #65480, #65979, #58369, #2707, #56873, #87857, #49783, #49292, #80231, #89345, #72616, #95937 ),
 .UNSPECIFIED., .F., .F.,
 ( 4, 2, 2, 2, 2, 2, 2, 4 ),
 ( 0.000000000000000000, 0.0003786681000626436911, 0.0007573362001252873822, 0.001136004300187931073, 0.001514672400250574764, 0.001893340500313218456, 0.002272008600375862147, 0.003029344800501141289 ),
 .UNSPECIFIED. ) ;
#15979=CARTESIAN_POINT ( 'NONE',  ( 152.7901873964250115, 266.7870861983042801, -15.84272339013448949 ) ) ;
#15981=CARTESIAN_POINT ( 'NONE',  ( 163.7085541710205234, 247.0954618725873217, -6.713544974106887331 ) ) ;
#15982=CARTESIAN_POINT ( 'NONE',  ( 182.6387802082273879, 268.5597891637301586, 15.04617342855019047 ) ) ;
#15984=CARTESIAN_POINT ( 'NONE',  ( 112.6237299221286321, 226.6423013555409796, -4.594050593750043987 ) ) ;
#15986=CARTESIAN_POINT ( 'NONE',  ( 191.5451565139252068, 298.8810523045859213, 7.782291334092181323 ) ) ;
#15989=CARTESIAN_POINT ( 'NONE',  ( 193.7944905295941567, 278.3514127848527551, 16.31057853467515173 ) ) ;
#15990=CARTESIAN_POINT ( 'NONE',  ( 190.8671785295675818, 300.0553446199063501, -7.998068249277817898 ) ) ;
#15991=B_SPLINE_CURVE_WITH_KNOTS ( 'NONE', 3,
 ( #56987, #95565, #9404, #80348 ),
 .UNSPECIFIED., .F., .F.,
 ( 4, 4 ),
 ( 0.007815255211040535860, 0.01599263494101685681 ),
 .UNSPECIFIED. ) ;
#15992=CARTESIAN_POINT ( 'NONE',  ( 150.7133245577828689, 269.6038598187387834, -14.58664962216439598 ) ) ;
#15993=CARTESIAN_POINT ( 'NONE',  ( 142.1224599184862711, 252.8615022471902307, -10.00000000000009592 ) ) ;
#15998=CARTESIAN_POINT ( 'NONE',  ( 192.9843945815383108, 267.1901746418614039, 11.24122804034830203 ) ) ;
#16001=ORIENTED_EDGE ( 'NONE', *, *, #17356, .F. ) ;
#16003=CARTESIAN_POINT ( 'NONE',  ( 183.2250948126493881, 264.4847478218908918, -13.17622970261022530 ) ) ;
#16008=CARTESIAN_POINT ( 'NONE',  ( 187.2487605686656309, 278.8013110013918094, 17.16344444290080418 ) ) ;
#16009=AXIS2_PLACEMENT_3D ( 'NONE', #66538, #12354, #34638 ) ;
#16011=VERTEX_POINT ( 'NONE', #55586 ) ;
#16012=CARTESIAN_POINT ( 'NONE',  ( 167.6769706185343409, 249.8146627436505867, 6.781605082613990199 ) ) ;
#16013=ADVANCED_FACE ( 'NONE', ( #86570 ), #7499, .T. ) ;
#16014=FACE_OUTER_BOUND ( 'NONE', #48619, .T. ) ;
#16018=CARTESIAN_POINT ( 'NONE',  ( 159.1305474299093135, 255.0248021455850846, 16.88467499060716648 ) ) ;
#16019=CYLINDRICAL_SURFACE ( 'NONE', #31565, 17.82106496071139645 ) ;
#16021=VECTOR ( 'NONE', #7734, 1000.000000000000000 ) ;
#16024=CARTESIAN_POINT ( 'NONE',  ( 148.1316126177475496, 276.0755160693871630, 5.020219949272568094 ) ) ;
#16026=CARTESIAN_POINT ( 'NONE',  ( 162.6619436536031174, 249.4045681345386072, 10.74432698607139614 ) ) ;
#16030=CARTESIAN_POINT ( 'NONE',  ( 169.8597199083751832, 269.3794817305624747, 17.64580905768150032 ) ) ;
#16033=ORIENTED_EDGE ( 'NONE', *, *, #3619, .F. ) ;
#16035=CARTESIAN_POINT ( 'NONE',  ( 206.3559632282955647, 273.2279825742143089, -11.28941701449801904 ) ) ;
#16036=CARTESIAN_POINT ( 'NONE',  ( 190.4649878924934683, 300.7519592376469291, 1.979076455900417919 ) ) ;
#16037=CARTESIAN_POINT ( 'NONE',  ( 190.0340467409721441, 301.4983712071542641, 4.077645795029533282 ) ) ;
#16039=CARTESIAN_POINT ( 'NONE',  ( 170.8196951477767982, 250.8282041339933244, -5.540778955988154841 ) ) ;
#16041=CARTESIAN_POINT ( 'NONE',  ( 183.4484973779139523, 284.6930032971759488, -15.01462800346279280 ) ) ;
#16042=B_SPLINE_CURVE_WITH_KNOTS ( 'NONE', 3,
 ( #37945, #52160, #68856, #83108 ),
 .UNSPECIFIED., .F., .F.,
 ( 4, 4 ),
 ( 8.774936542010898348E-05, 0.008022331835684331364 ),
 .UNSPECIFIED. ) ;
#16043=CARTESIAN_POINT ( 'NONE',  ( 130.0524911732904343, 236.7048013555409796, 4.594050593750051981 ) ) ;
#16044=CARTESIAN_POINT ( 'NONE',  ( 186.9756763787170257, 262.2700035475498339, -10.24646055643486520 ) ) ;
#16045=CARTESIAN_POINT ( 'NONE',  ( 161.2265274951298863, 283.7633814984351375, 2.173529036228213140 ) ) ;
#16046=CARTESIAN_POINT ( 'NONE',  ( 180.5872800571609389, 291.4665845829162549, -9.750679543141076877 ) ) ;
#16050=CARTESIAN_POINT ( 'NONE',  ( 200.0716132454348894, 273.8135256567975375, 13.71647348634510877 ) ) ;
#16051=CARTESIAN_POINT ( 'NONE',  ( 178.8491990207230344, 254.9654333574110012, 1.324507615027452845 ) ) ;
#16053=CARTESIAN_POINT ( 'NONE',  ( 206.7325995683429767, 270.5756292972641859, -5.459556455514786855 ) ) ;
#16055=CARTESIAN_POINT ( 'NONE',  ( 201.1388841337167435, 282.2642286331299601, -18.17233400608081340 ) ) ;
#16058=CARTESIAN_POINT ( 'NONE',  ( 156.0507216674837707, 279.5060275253360373, 7.618106348741741307 ) ) ;
#16060=CARTESIAN_POINT ( 'NONE',  ( 194.6310785344323904, 293.5360785768717165, -14.54510914272505495 ) ) ;
#16061=CARTESIAN_POINT ( 'NONE',  ( 152.8623378685196030, 273.8643641423199711, 12.12982893395569306 ) ) ;
#16063=CARTESIAN_POINT ( 'NONE',  ( 188.0407104400106846, 266.0414501920158727, -11.72547689681096905 ) ) ;
#16064=CARTESIAN_POINT ( 'NONE',  ( 156.9004364869687436, 276.5848328012408501, 10.23493742149738672 ) ) ;
#16065=CARTESIAN_POINT ( 'NONE',  ( 195.7309803721981609, 265.3211447974111934, 4.250103213233941801 ) ) ;
#16066=CARTESIAN_POINT ( 'NONE',  ( 190.0340467409721441, 301.4983712071542641, 4.077645795029533282 ) ) ;
#16067=CARTESIAN_POINT ( 'NONE',  ( 204.6508828921556074, 273.0178721416635881, -9.847606913800847295 ) ) ;
#16068=CARTESIAN_POINT ( 'NONE',  ( 164.2092836438689005, 283.3451842658567443, -6.697959257182540149 ) ) ;
#16069=CARTESIAN_POINT ( 'NONE',  ( 151.4352391397386555, 275.0282326485918247, -9.505706171079989275 ) ) ;
#16070=CARTESIAN_POINT ( 'NONE',  ( 200.9521687275011175, 282.5876292032514243, -18.16013154125647944 ) ) ;
#16072=CARTESIAN_POINT ( 'NONE',  ( 204.8438479865957333, 272.6835259793063528, -9.477213056041572159 ) ) ;
#16074=CARTESIAN_POINT ( 'NONE',  ( 186.7654524502822539, 262.6710075733441272, -8.886537497778370209 ) ) ;
#16075=CARTESIAN_POINT ( 'NONE',  ( 192.3193821777917947, 275.6344104414516778, -15.92451825442405955 ) ) ;
#16077=CARTESIAN_POINT ( 'NONE',  ( 162.5887743522035294, 284.9919049736276975, -2.844505511527740005 ) ) ;
#16078=CARTESIAN_POINT ( 'NONE',  ( 153.1164404339926080, 265.4415410246681972, 16.15325778160653414 ) ) ;
#16079=CARTESIAN_POINT ( 'NONE',  ( 201.5036534377215958, 270.3153034880852488, -10.25451236307256409 ) ) ;
#16083=CARTESIAN_POINT ( 'NONE',  ( 89.53865347855843027, 216.3768266524159856, 9.188101187500098632 ) ) ;
#16085=CARTESIAN_POINT ( 'NONE',  ( 193.1444937042664094, 296.1109190324805240, -12.15243020627156767 ) ) ;
#16086=CARTESIAN_POINT ( 'NONE',  ( 163.3939361803663246, 247.6403962173759226, -10.78041711314006790 ) ) ;
#16088=CARTESIAN_POINT ( 'NONE',  ( 155.4495868485232108, 261.4004128932040203, -18.48326470492642315 ) ) ;
#16095=CARTESIAN_POINT ( 'NONE',  ( 161.7570549189561859, 250.4755577280957652, 14.23709397115338682 ) ) ;
#16096=CARTESIAN_POINT ( 'NONE',  ( 196.9080397933726942, 269.7016881256661804, 12.39056067425276630 ) ) ;
#16097=CARTESIAN_POINT ( 'NONE',  ( 205.0902471979347581, 275.4202670467537359, -13.79912452887783303 ) ) ;
#16099=CARTESIAN_POINT ( 'NONE',  ( 196.1241105319816143, 290.9500712997905794, 15.97146679939154268 ) ) ;
#16100=CARTESIAN_POINT ( 'NONE',  ( 190.1321413272149812, 298.8808762037565430, -8.148410351609143731 ) ) ;
#16101=CARTESIAN_POINT ( 'NONE',  ( 161.5757715694810770, 250.7895496999525449, -14.51803553215175135 ) ) ;
#16102=ADVANCED_FACE ( 'NONE', ( #54089 ), #17616, .T. ) ;
#16104=CARTESIAN_POINT ( 'NONE',  ( 29.07873433320978052, 199.8464784336661353, 1.353441290958777327E-15 ) ) ;
#16106=CARTESIAN_POINT ( 'NONE',  ( 60.25564886944957976, 217.8464784336661637, 1.353441290958777327E-15 ) ) ;
#16110=CARTESIAN_POINT ( 'NONE',  ( 146.6963301283313967, 249.3768266524160140, 9.188101187500098632 ) ) ;
#16116=CARTESIAN_POINT ( 'NONE',  ( 136.7639277290221855, 239.7677522451417929, -5.000000000000041744 ) ) ;
#16119=CARTESIAN_POINT ( 'NONE',  ( 63.01627839189497138, 213.3149278399160949, 9.188101187500093303 ) ) ;
#16121=DIRECTION ( 'NONE',  ( -0.8660254037844387076, -0.4999999999999998890, -0.000000000000000000 ) ) ;
#16122=CARTESIAN_POINT ( 'NONE',  ( 159.5764336135613632, 254.2525046211064819, 15.32981087583629076 ) ) ;
#16124=CARTESIAN_POINT ( 'NONE',  ( 201.4731444478667015, 281.6852727860684240, 16.40638429239196938 ) ) ;
#16126=CARTESIAN_POINT ( 'NONE',  ( 108.4196379545419120, 226.7365022471902307, -10.00000000000009059 ) ) ;
#16127=CARTESIAN_POINT ( 'NONE',  ( 181.7815785431583038, 276.1505370498239813, -17.81783396216490445 ) ) ;
#16128=CARTESIAN_POINT ( 'NONE',  ( 207.6727254509676186, 270.9472835030587703, 7.315149605389819953 ) ) ;
#16133=CARTESIAN_POINT ( 'NONE',  ( 206.8791291248445532, 272.3218326606039454, -10.16823074922856840 ) ) ;
#16134=CARTESIAN_POINT ( 'NONE',  ( 190.1532766730107085, 279.2606816812074726, -17.72189159620656440 ) ) ;
#16137=CARTESIAN_POINT ( 'NONE',  ( 173.4291969867144587, 251.4074785162788714, 0.3572428630574652209 ) ) ;
#16138=VERTEX_POINT ( 'NONE', #64721 ) ;
#16140=CARTESIAN_POINT ( 'NONE',  ( 194.7576540903134799, 293.3168432830895540, -14.62421624641040196 ) ) ;
#16145=CARTESIAN_POINT ( 'NONE',  ( 100.8442274002074441, 217.4824982072973683, 3.021315404115420679E-15 ) ) ;
#16149=B_SPLINE_CURVE_WITH_KNOTS ( 'NONE', 3,
 ( #20719, #45483, #44485, #76418 ),
 .UNSPECIFIED., .F., .F.,
 ( 4, 4 ),
 ( 0.01434568471657762107, 0.02303913993019953560 ),
 .UNSPECIFIED. ) ;
#16150=CARTESIAN_POINT ( 'NONE',  ( -11.77978294824862893, 175.5530062829863311, 1.347971487989956912E-14 ) ) ;
#16153=( BOUNDED_CURVE ( )  B_SPLINE_CURVE ( 2, ( #62072, #94532, #55965, #16983, #53973, #55472, #86458, #47874, #1806 ),
 .UNSPECIFIED., .F., .T. ) 
 B_SPLINE_CURVE_WITH_KNOTS ( ( 3, 2, 2, 2, 3 ),
 ( 0.6169354838709677491, 0.6182795698924731242, 0.6209677419354838745, 0.6236559139784946248, 0.6250000000000000000 ),
 .UNSPECIFIED. ) 
 CURVE ( )  GEOMETRIC_REPRESENTATION_ITEM ( )  RATIONAL_B_SPLINE_CURVE ( ( 0.9330127018922194093, 0.9330127018922194093, 1.000000000000000000, 0.8660254037844387076, 1.000000000000000000, 0.8660254037844387076, 1.000000000000000000, 0.9330127018922194093, 0.9330127018922194093 ) ) 
 REPRESENTATION_ITEM ( '' )  );
#16157=CARTESIAN_POINT ( 'NONE',  ( 164.3010377730689981, 246.0692501711882869, 7.247566249275159578 ) ) ;
#16159=CARTESIAN_POINT ( 'NONE',  ( 157.0887340267001946, 258.5613266995183039, -17.61824281915036394 ) ) ;
#16160=CARTESIAN_POINT ( 'NONE',  ( 133.0017827873424494, 259.8464784336661637, 1.353441290958777525E-15 ) ) ;
#16162=CARTESIAN_POINT ( 'NONE',  ( 206.4680688164142168, 270.6138877121450150, 2.724256221002448797 ) ) ;
#16163=CARTESIAN_POINT ( 'NONE',  ( 182.0101398577191958, 260.3743076433015062, 9.429781970683626113 ) ) ;
#16164=CARTESIAN_POINT ( 'NONE',  ( 87.45434598099585344, 230.4869531367911293, 4.594050593750046652 ) ) ;
#16166=CARTESIAN_POINT ( 'NONE',  ( 190.9501423151522772, 299.9116471280854626, 8.746938802470586083 ) ) ;
#16170=CARTESIAN_POINT ( 'NONE',  ( 195.8309633264585727, 291.4578171538532274, -15.70624013417040743 ) ) ;
#16174=CARTESIAN_POINT ( 'NONE',  ( 193.2980202556421432, 268.5488920227266476, -13.18347973120535599 ) ) ;
#16175=CARTESIAN_POINT ( 'NONE',  ( 146.9235493515124062, 276.1679430252639804, 0.7994986043261682607 ) ) ;
#16177=CARTESIAN_POINT ( 'NONE',  ( 52.32645086003936541, 201.0177522451418497, -10.00000000000009592 ) ) ;
#16178=CARTESIAN_POINT ( 'NONE',  ( -22.42236680055709641, 157.8615022471902591, 0.000000000000000000 ) ) ;
#16179=CARTESIAN_POINT ( 'NONE',  ( 80.33713356334875755, 211.0643266524159856, -9.188101187500093303 ) ) ;
#16180=ORIENTED_EDGE ( 'NONE', *, *, #41613, .F. ) ;
#16184=B_SPLINE_SURFACE_WITH_KNOTS ( 'NONE', 3, 1, ( 
 ( #17666, #87637 ),
 ( #17151, #47055 ),
 ( #71376, #86123 ),
 ( #57141, #88122 ),
 ( #48564, #24751 ),
 ( #40441, #95208 ),
 ( #56652, #25253 ),
 ( #55632, #32850 ),
 ( #70350, #31838 ),
 ( #55138, #1965 ),
 ( #64768, #77969 ),
 ( #62741, #40931 ),
 ( #9577, #79505 ),
 ( #18165, #86617 ),
 ( #962, #63759 ),
 ( #25777, #94692 ),
 ( #56136, #1474 ),
 ( #26265, #49065 ),
 ( #79999, #10568 ),
 ( #10066, #48049 ),
 ( #2476, #41443 ),
 ( #24260, #72383 ),
 ( #8564, #47548 ),
 ( #33357, #64257 ),
 ( #2993, #33883 ),
 ( #78475, #95717 ),
 ( #9062, #39929 ),
 ( #70866, #32355 ),
 ( #63256, #4449 ),
 ( #42922, #19679 ),
 ( #67242, #36340 ),
 ( #42434, #80504 ),
 ( #43442, #27264 ),
 ( #35349, #50540 ) ),
 .UNSPECIFIED., .T., .F., .F.,
 ( 4, 2, 2, 2, 2, 2, 2, 2, 2, 2, 2, 2, 2, 2, 2, 2, 4 ),
 ( 2, 2 ),
 ( 0.000000000000000000, 0.06250000000000000000, 0.1250000000000000000, 0.1875000000000000000, 0.2500000000000000000, 0.3125000000000000000, 0.3750000000000000000, 0.4375000000000000000, 0.5000000000000000000, 0.5625000000000000000, 0.6250000000000000000, 0.6875000000000000000, 0.7500000000000000000, 0.8125000000000000000, 0.8750000000000000000, 0.9375000000000000000, 1.000000000000000000 ),
 ( 0.000000000000000000, 1.000000000000000000 ),
 .UNSPECIFIED. ) ;
#16185=CARTESIAN_POINT ( 'NONE',  ( 200.9211856235105529, 282.6412935135391535, -18.21488537951028519 ) ) ;
#16190=CARTESIAN_POINT ( 'NONE',  ( 206.9678007395010013, 269.7219839212710326, -0.02000383387707006105 ) ) ;
#16192=CARTESIAN_POINT ( 'NONE',  ( 160.9324095734352511, 260.4995019621508163, 16.69280320549395924 ) ) ;
#16194=CARTESIAN_POINT ( 'NONE',  ( 192.5672132233574700, 296.7161803602032819, 11.26440590052197521 ) ) ;
#16197=CARTESIAN_POINT ( 'NONE',  ( 152.8651171364917900, 265.8768457450651113, -16.25664868183201861 ) ) ;
#16199=CARTESIAN_POINT ( 'NONE',  ( 138.9086373102437051, 262.5530062829863027, -4.648177544792955347E-16 ) ) ;
#16200=ORIENTED_EDGE ( 'NONE', *, *, #98920, .T. ) ;
#16201=CARTESIAN_POINT ( 'NONE',  ( 195.8856561536922811, 265.4848694841979864, 4.430043780811904419 ) ) ;
#16202=CARTESIAN_POINT ( 'NONE',  ( 85.30758498749676733, 213.3927522451418213, 10.00000000000009948 ) ) ;
#16204=CARTESIAN_POINT ( 'NONE',  ( 187.8780304577002198, 266.2815348468194543, -12.02982252659589868 ) ) ;
#16205=CARTESIAN_POINT ( 'NONE',  ( 198.5685943996323886, 266.1185824620975495, 1.314686358112626685 ) ) ;
#16206=CARTESIAN_POINT ( 'NONE',  ( 156.8545567402366316, 272.5222548076167755, 14.36144970815616695 ) ) ;
#16209=CARTESIAN_POINT ( 'NONE',  ( 202.4017613376760494, 280.0768611521521620, 15.73960524502980540 ) ) ;
#16210=CARTESIAN_POINT ( 'NONE',  ( 198.2505066714982149, 285.2670451491296149, 0.000000000000000000 ) ) ;
#16211=CARTESIAN_POINT ( 'NONE',  ( 177.6568436143930967, 264.5527407949075496, -15.77239500404458283 ) ) ;
#16213=CARTESIAN_POINT ( 'NONE',  ( 199.2490371652133945, 281.9579806773367068, -16.60615833393185525 ) ) ;
#16216=CARTESIAN_POINT ( 'NONE',  ( 172.3003440879262484, 275.1291536054555422, 16.73320108566939268 ) ) ;
#16217=CARTESIAN_POINT ( 'NONE',  ( 166.0707157462996406, 285.6421157637285546, -3.164261021881538571 ) ) ;
#16218=CARTESIAN_POINT ( 'NONE',  ( 126.4618338667176403, 250.4865022471902876, -10.00000000000009592 ) ) ;
#16219=CARTESIAN_POINT ( 'NONE',  ( 191.8419389717784327, 261.4849666034271536, 3.078932809042389529 ) ) ;
#16221=CARTESIAN_POINT ( 'NONE',  ( -4.696256414383327638, 180.3464784336661637, 1.353441290958777327E-15 ) ) ;
#16222=CARTESIAN_POINT ( 'NONE',  ( 73.84070662262635665, 224.9860189848785126, -2.679491924311252493 ) ) ;
#16223=ORIENTED_EDGE ( 'NONE', *, *, #21918, .T. ) ;
#16224=ADVANCED_FACE ( 'NONE', ( #18627 ), #71231, .F. ) ;
#16227=DIRECTION ( 'NONE',  ( 0.4999999999999998890, -0.8660254037844385966, 0.000000000000000000 ) ) ;
#16229=CYLINDRICAL_SURFACE ( 'NONE', #89078, 17.82106496071139645 ) ;
#16230=CARTESIAN_POINT ( 'NONE',  ( 12.11013585174968554, 186.9869531367911293, 4.594050593750046652 ) ) ;
#16234=CARTESIAN_POINT ( 'NONE',  ( 147.2937583206075942, 275.5267222813735088, 0.1877253132609109920 ) ) ;
#16236=CARTESIAN_POINT ( 'NONE',  ( 190.2350275263131607, 261.6741793222014962, -0.7552779011735962778 ) ) ;
#16238=CARTESIAN_POINT ( 'NONE',  ( 69.44849478424205813, 224.2365022471903160, 2.944929066748280225E-16 ) ) ;
#16240=CARTESIAN_POINT ( 'NONE',  ( 203.3784415195017061, 270.0710565943527399, 6.595345848229188235 ) ) ;
#16241=CARTESIAN_POINT ( 'NONE',  ( 20.95974617273066443, 195.1589784336661637, -6.496448406907675876E-16 ) ) ;
#16243=CARTESIAN_POINT ( 'NONE',  ( 127.3278592705020742, 250.9865022471903160, 10.00000000000009415 ) ) ;
#16244=CARTESIAN_POINT ( 'NONE',  ( 164.5139018292655919, 259.6662038739244736, -17.01387605652571366 ) ) ;
#16245=CARTESIAN_POINT ( 'NONE',  ( 150.9003228897357189, 269.2799692068659283, -14.30003212299500781 ) ) ;
#16247=CARTESIAN_POINT ( 'NONE',  ( 155.3738696901333469, 261.5315588585399951, 17.02116401938635804 ) ) ;
#16249=CARTESIAN_POINT ( 'NONE',  ( 163.1096457525017627, 281.1598135738970541, -10.26398345759424657 ) ) ;
#16252=CARTESIAN_POINT ( 'NONE',  ( 162.8037981520209314, 248.6625452659484381, 9.809699077002424161 ) ) ;
#16253=CARTESIAN_POINT ( 'NONE',  ( 185.9817139542059579, 267.6581844819601770, -14.98798611928668301 ) ) ;
#16255=CARTESIAN_POINT ( 'NONE',  ( 185.3296124515819372, 291.1871008657900006, 13.45743802455416827 ) ) ;
#16265=VERTEX_POINT ( 'NONE', #78807 ) ;
#16266=CARTESIAN_POINT ( 'NONE',  ( 189.5147274052520174, 274.6873094654737315, -16.11146568285224134 ) ) ;
#16269=CARTESIAN_POINT ( 'NONE',  ( 151.4281781455628675, 268.3656970847310390, 15.24742929158552585 ) ) ;
#16273=CARTESIAN_POINT ( 'NONE',  ( 190.4281805785508084, 300.8157113754859893, -1.233909217199055774 ) ) ;
#16274=CARTESIAN_POINT ( 'NONE',  ( 149.2593905435863348, 272.1221474021800759, -12.98626158366800176 ) ) ;
#16275=CARTESIAN_POINT ( 'NONE',  ( 180.4421801628115816, 287.0161100701561736, -13.61753346319509639 ) ) ;
#16276=EDGE_CURVE ( 'NONE', #47888, #17056, #83011, .T. ) ;
#16277=EDGE_LOOP ( 'NONE', ( #83135, #13444, #82374, #93054, #60738, #76939, #68674, #10080, #79877, #64648, #24374, #52130, #10825, #93028, #37621, #78797, #58298, #31817, #52377, #80992, #88709, #42275, #16409, #85900, #1738, #70330, #85131, #60510, #99747, #66854, #66621, #74758, #30408, #86994, #51289, #23484, #42067, #74603, #51418, #81899, #69105, #25516, #70136, #63413, #93769, #90995, #94210, #15508, #23396, #16921, #74011, #60497, #16033 ) ) ;
#16282=CARTESIAN_POINT ( 'NONE',  ( 159.4285914931787431, 254.5085746851079023, 15.41072477910873673 ) ) ;
#16285=CARTESIAN_POINT ( 'NONE',  ( 66.20992061623260838, 209.0333772461660544, 9.188101187500095079 ) ) ;
#16288=CARTESIAN_POINT ( 'NONE',  ( 159.6684720758726144, 254.4985299059416377, 15.35327236017407948 ) ) ;
#16289=CARTESIAN_POINT ( 'NONE',  ( 98.13012578506970840, 215.9155109091896065, 2.679491924311254714 ) ) ;
#16290=CARTESIAN_POINT ( 'NONE',  ( 173.0447734647070206, 271.2248508029067011, 16.42412328953864886 ) ) ;
#16293=CYLINDRICAL_SURFACE ( 'NONE', #10869, 17.82106496071139645 ) ;
#16294=CARTESIAN_POINT ( 'NONE',  ( 190.4240181651484818, 300.8229208869809668, -4.214281362166949485 ) ) ;
#16295=CARTESIAN_POINT ( 'NONE',  ( 148.0389988358468827, 274.2359278451201590, 7.783622668412842671 ) ) ;
#16297=CARTESIAN_POINT ( 'NONE',  ( 148.9232972370683399, 272.7042780851529642, 12.27045554427055940 ) ) ;
#16299=EDGE_CURVE ( 'NONE', #39606, #43165, #99014, .T. ) ;
#16301=CARTESIAN_POINT ( 'NONE',  ( 147.5381343315788172, 275.1034506142203782, -4.056595942992749393 ) ) ;
#16303=CARTESIAN_POINT ( 'NONE',  ( 160.2788325581946083, 255.7866659750827694, 16.08102370418938065 ) ) ;
#16306=CARTESIAN_POINT ( 'NONE',  ( 164.2897805489690768, 249.8104079013010335, 11.36607573508163505 ) ) ;
#16307=CARTESIAN_POINT ( 'NONE',  ( 198.2505066714982149, 285.2670451491296149, 0.000000000000000000 ) ) ;
#16309=CARTESIAN_POINT ( 'NONE',  ( 112.1907172202364080, 226.3923013555410080, 4.594050593750050204 ) ) ;
#16311=CARTESIAN_POINT ( 'NONE',  ( 191.8000917695741805, 298.4394914891611847, -9.452573400474340914 ) ) ;
#16313=CARTESIAN_POINT ( 'NONE',  ( 191.2002274372966610, 261.5526795057712661, 5.342804824337664016 ) ) ;
#16314=ADVANCED_FACE ( 'NONE', ( #42273 ), #11421, .T. ) ;
#16315=CARTESIAN_POINT ( 'NONE',  ( 203.5477091018662748, 278.0920214017542662, -16.09930363698006062 ) ) ;
#16316=EDGE_CURVE ( 'NONE', #67853, #25891, #11754, .T. ) ;
#16317=CARTESIAN_POINT ( 'NONE',  ( 204.5133713884061706, 276.4194452585140311, 14.87364779308245843 ) ) ;
#16318=FACE_OUTER_BOUND ( 'NONE', #43917, .T. ) ;
#16320=CARTESIAN_POINT ( 'NONE',  ( 168.9493557510702146, 284.9254214029872401, -7.956471245316214969 ) ) ;
#16322=CARTESIAN_POINT ( 'NONE',  ( 207.7837159184916231, 270.7550423741513441, -2.369602332675663448 ) ) ;
#16324=CARTESIAN_POINT ( 'NONE',  ( 165.0831640657340529, 244.7145676943567878, -1.661138566959525775 ) ) ;
#16325=CARTESIAN_POINT ( 'NONE',  ( 125.6409139509397050, 243.3458772461660544, 9.188101187500095079 ) ) ;
#16326=DIRECTION ( 'NONE',  ( 0.8660254037844395958, 0.4999999999999985567, 0.000000000000000000 ) ) ;
#16328=CARTESIAN_POINT ( 'NONE',  ( 188.0361769804965206, 281.7550819701144746, -17.70093714309158983 ) ) ;
#16330=CARTESIAN_POINT ( 'NONE',  ( 50.64826632015721231, 209.2369531367911293, -4.594050593750048428 ) ) ;
#16331=FACE_OUTER_BOUND ( 'NONE', #13177, .T. ) ;
#16332=VERTEX_POINT ( 'NONE', #17490 ) ;
#16334=CARTESIAN_POINT ( 'NONE',  ( 196.3249884498792994, 275.2518087180711177, 16.06659936265807431 ) ) ;
#16335=EDGE_CURVE ( 'NONE', #86137, #6903, #20609, .T. ) ;
#16339=B_SPLINE_CURVE_WITH_KNOTS ( 'NONE', 3,
 ( #1110, #92835, #31988, #23386, #93849, #15790, #24403, #78619, #40079, #14799, #38078, #22893, #71024, #32510, #91842, #85245, #22403, #15282, #68991, #92344, #46177, #7699, #77097, #69497, #110, #30995, #61880, #54276, #94836, #88263, #64405, #4094, #56287, #87285, #10214, #18315, #10712, #17816, #25399, #2114, #34496, #33509, #95854, #48717, #32996, #72016, #26411, #11226, #3617, #72530 ),
 .UNSPECIFIED., .F., .F.,
 ( 4, 2, 2, 2, 2, 2, 2, 2, 2, 2, 2, 2, 2, 2, 2, 2, 2, 2, 2, 2, 2, 2, 2, 2, 4 ),
 ( 0.0001408704111295071184, 0.001152638629686134064, 0.001658522738964416082, 0.001784993766284012282, 0.001911464793603608048, 0.002037935820923203814, 0.002164406848242800014, 0.002417348902882022772, 0.002670290957521245529, 0.003176175066799552700, 0.004187943285356238166, 0.005199711503912924498, 0.005705595613191308431, 0.005958537667830458330, 0.006211479722469609964, 0.006274715236129331519, 0.006337950749789053075, 0.006401186263448773762, 0.006464421777108495318, 0.006717363831747565420, 0.007223247941025566846, 0.007476189995664625672, 0.007729132050303684498, 0.007982074104942744192, 0.008235016159581802150 ),
 .UNSPECIFIED. ) ;
#16340=CARTESIAN_POINT ( 'NONE',  ( 154.8579861482817535, 262.4250953638155011, -17.69813260923097786 ) ) ;
#16341=CARTESIAN_POINT ( 'NONE',  ( 155.7075129258784614, 270.0159152318828433, -14.86779825989652259 ) ) ;
#16343=CARTESIAN_POINT ( 'NONE',  ( 115.9793180381955580, 247.7677522451419065, -5.000000000000047962 ) ) ;
#16344=CARTESIAN_POINT ( 'NONE',  ( 194.6516423578734702, 293.0856640331928702, -14.71461979434458200 ) ) ;
#16345=ORIENTED_EDGE ( 'NONE', *, *, #7583, .F. ) ;
#16347=CARTESIAN_POINT ( 'NONE',  ( 162.6626107288841467, 248.9070890562113902, 10.12509462564867313 ) ) ;
#16349=CARTESIAN_POINT ( 'NONE',  ( 16.08835327644320401, 192.3464784336661637, 1.353441290958777327E-15 ) ) ;
#16351=CARTESIAN_POINT ( 'NONE',  ( -17.42236680055705023, 149.2012482093457777, 0.000000000000000000 ) ) ;
#16354=EDGE_CURVE ( 'NONE', #86855, #23257, #9058, .T. ) ;
#16356=CARTESIAN_POINT ( 'NONE',  ( 60.25564886944957976, 217.8464784336661637, 1.353441290958777327E-15 ) ) ;
#16357=CARTESIAN_POINT ( 'NONE',  ( 174.1648641962809450, 288.5940705739083683, 7.621244220064776087 ) ) ;
#16358=CARTESIAN_POINT ( 'NONE',  ( 184.7539679289934611, 257.4663050619941487, 1.389359455806087995 ) ) ;
#16360=CARTESIAN_POINT ( 'NONE',  ( 161.6505112061591376, 251.4379174015757883, -12.98887274494184041 ) ) ;
#16362=B_SPLINE_CURVE_WITH_KNOTS ( 'NONE', 3,
 ( #13850, #28544, #38998, #23803, #46599, #5259, #5747, #35656, #36141, #59426, #20472, #43239, #90903, #20980, #90404, #44727, #51862, #97484, #29550, #98967, #82801, #67543, #44235, #75661, #75173, #68045, #6245, #37143, #98474, #21453, #91381, #23301, #54190, #85155, #77532, #74182, #69904, #517, #31405, #54692, #12374, #28049, #89895, #86671, #71428, #24318, #25307, #25833, #39988, #55684, #85676, #55193 ),
 .UNSPECIFIED., .F., .F.,
 ( 4, 2, 2, 2, 2, 2, 2, 2, 2, 2, 2, 2, 2, 2, 2, 2, 2, 2, 2, 2, 2, 2, 2, 2, 2, 4 ),
 ( 0.0001758988993951120044, 0.0006622138821329520090, 0.001148528864870791959, 0.001391686356239734161, 0.001513265101924233125, 0.001634843847608731873, 0.001756422593293230621, 0.001878001338977729586, 0.002121158830346824876, 0.002607473813085065331, 0.003093788795823305786, 0.004066418761299786695, 0.005039048726776266737, 0.005525363709514587857, 0.005768521200883747549, 0.005890099946568327395, 0.006011678692252908109, 0.006072468065095169842, 0.006133257437937432444, 0.006254836183622050454, 0.006497993674991226626, 0.006741151166360403665, 0.006984308657729579838, 0.007227466149098756877, 0.007470623640467933917, 0.007956938623206325292 ),
 .UNSPECIFIED. ) ;
#16363=CARTESIAN_POINT ( 'NONE',  ( 162.6576765882541054, 267.6039545257508507, 16.48102639217245624 ) ) ;
#16364=CARTESIAN_POINT ( 'NONE',  ( 18.20865839366279459, 187.9865022471902876, 10.00000000000009237 ) ) ;
#16365=CARTESIAN_POINT ( 'NONE',  ( 146.4255236417662616, 255.3458772461660260, 9.188101187500095079 ) ) ;
#16366=CARTESIAN_POINT ( 'NONE',  ( 202.8499463704053198, 279.3005819042728604, 17.04674939340617001 ) ) ;
#16367=CARTESIAN_POINT ( 'NONE',  ( -14.92600794870451253, 168.3149278399160664, 9.188101187500093303 ) ) ;
#16370=CARTESIAN_POINT ( 'NONE',  ( 188.7194914702840549, 261.8282078956012242, 6.495625297079970828 ) ) ;
#16371=CARTESIAN_POINT ( 'NONE',  ( 74.74743988288986429, 202.4155109091896065, 2.679491924311254714 ) ) ;
#16372=CARTESIAN_POINT ( 'NONE',  ( 185.9427433571077586, 257.7868782628476083, -2.501399907045548598 ) ) ;
#16376=CARTESIAN_POINT ( 'NONE',  ( 184.5944248404513246, 287.4419850773005010, 15.55097255147333435 ) ) ;
#16377=CARTESIAN_POINT ( 'NONE',  ( 181.3234608124392366, 287.3713783320475841, 13.33777075617584984 ) ) ;
#16378=CARTESIAN_POINT ( 'NONE',  ( 196.6472778906841086, 289.6559313043970860, 16.38098019016104345 ) ) ;
#16380=CARTESIAN_POINT ( 'NONE',  ( 160.4502686134403007, 252.7389780038842844, 16.14074205763531111 ) ) ;
#16384=CARTESIAN_POINT ( 'NONE',  ( 191.6256142097132908, 298.3549236037118817, 8.658380026548993413 ) ) ;
#16385=CARTESIAN_POINT ( 'NONE',  ( 163.3020905273760093, 247.7994775548095845, -11.05431316445765155 ) ) ;
#16387=CARTESIAN_POINT ( 'NONE',  ( 162.7020145476934090, 284.0983276010327359, 6.051621772638641872 ) ) ;
#16390=CARTESIAN_POINT ( 'NONE',  ( 155.8021524857682039, 277.1561808410325511, -10.39920598458100542 ) ) ;
#16392=VERTEX_POINT ( 'NONE', #27102 ) ;
#16398=CARTESIAN_POINT ( 'NONE',  ( 188.3784916956350344, 286.3721210266486992, -16.81851773412965301 ) ) ;
#16401=EDGE_LOOP ( 'NONE', ( #16887, #11710, #47561, #60855 ) ) ;
#16403=CARTESIAN_POINT ( 'NONE',  ( 190.7779368023172708, 300.2099158256590385, 8.142228434510803581 ) ) ;
#16407=ORIENTED_EDGE ( 'NONE', *, *, #34981, .F. ) ;
#16409=ORIENTED_EDGE ( 'NONE', *, *, #56772, .F. ) ;
#16410=CARTESIAN_POINT ( 'NONE',  ( 183.2186634280558053, 270.7509055985178179, 17.09995095404208953 ) ) ;
#16412=CARTESIAN_POINT ( 'NONE',  ( 164.4963285489318991, 245.7309966251440301, -6.672251175510283794 ) ) ;
#16414=CARTESIAN_POINT ( 'NONE',  ( 169.9746517273565871, 283.3628436921554226, 12.55872587313221445 ) ) ;
#16416=EDGE_CURVE ( 'NONE', #31700, #48297, #38264, .T. ) ;
#16418=CARTESIAN_POINT ( 'NONE',  ( 197.7365809935693051, 288.1571905346162339, -17.55295824978644958 ) ) ;
#16420=B_SPLINE_CURVE_WITH_KNOTS ( 'NONE', 3,
 ( #99580, #30672, #14477, #13493 ),
 .UNSPECIFIED., .F., .F.,
 ( 4, 4 ),
 ( 0.000000000000000000, 0.006832007640786700794 ),
 .UNSPECIFIED. ) ;
#16422=CARTESIAN_POINT ( 'NONE',  ( 198.3572878714705610, 277.3135066751846125, -15.31504719882579302 ) ) ;
#16423=CARTESIAN_POINT ( 'NONE',  ( 191.6434079017471959, 298.2851893172241944, -8.812442504271411181 ) ) ;
#16424=CARTESIAN_POINT ( 'NONE',  ( 206.7596416265183734, 271.4678399409689291, 6.202658291405857227 ) ) ;
#16425=ORIENTED_EDGE ( 'NONE', *, *, #59885, .F. ) ;
#16426=CARTESIAN_POINT ( 'NONE',  ( 155.8152618860606253, 260.7670451491295012, 0.000000000000000000 ) ) ;
#16427=CARTESIAN_POINT ( 'NONE',  ( 159.7132918459648181, 254.0154592091499239, -16.90058287995827158 ) ) ;
#16429=CARTESIAN_POINT ( 'NONE',  ( -22.42236680055709641, 157.8615022471902591, 0.000000000000000000 ) ) ;
#16432=CARTESIAN_POINT ( 'NONE',  ( 161.5504728662519369, 250.8333683393111926, 12.94300825113363373 ) ) ;
#16433=CARTESIAN_POINT ( 'NONE',  ( 191.2038183216754987, 261.2453028453169281, -0.002002736021087949715 ) ) ;
#16434=( BOUNDED_CURVE ( )  B_SPLINE_CURVE ( 2, ( #42567, #89734, #50186, #5579, #73500, #82137, #97807, #90736, #51694 ),
 .UNSPECIFIED., .F., .T. ) 
 B_SPLINE_CURVE_WITH_KNOTS ( ( 3, 2, 2, 2, 3 ),
 ( 0.1975806451612903136, 0.1989247311827956888, 0.2016129032258064391, 0.2043010752688172171, 0.2056451612903225923 ),
 .UNSPECIFIED. ) 
 CURVE ( )  GEOMETRIC_REPRESENTATION_ITEM ( )  RATIONAL_B_SPLINE_CURVE ( ( 0.9330127018922194093, 0.9330127018922194093, 1.000000000000000000, 0.8660254037844387076, 1.000000000000000000, 0.8660254037844387076, 1.000000000000000000, 0.9330127018922194093, 0.9330127018922194093 ) ) 
 REPRESENTATION_ITEM ( '' )  );
#16435=ORIENTED_EDGE ( 'NONE', *, *, #57421, .T. ) ;
#16436=CARTESIAN_POINT ( 'NONE',  ( 155.3935616475962149, 261.4974513877137952, -18.59422973016237890 ) ) ;
#16438=CYLINDRICAL_SURFACE ( 'NONE', #20874, 10.00000000000010658 ) ;
#16439=CARTESIAN_POINT ( 'NONE',  ( 5.633247839328319628, 187.3927522451419634, 2.944929066748280225E-16 ) ) ;
#16440=CARTESIAN_POINT ( 'NONE',  ( 91.51436070488293240, 214.4548013555409796, -4.594050593750042211 ) ) ;
#16443=CARTESIAN_POINT ( 'NONE',  ( 167.0158807670456440, 278.2951364720916558, -13.37185693470555137 ) ) ;
#16444=CARTESIAN_POINT ( 'NONE',  ( 12.46239254174337852, 171.8768266524160140, -9.188101187500091527 ) ) ;
#16446=CARTESIAN_POINT ( 'NONE',  ( 161.2313178023453588, 251.3861611254901618, 13.12937145726518473 ) ) ;
#16448=ORIENTED_EDGE ( 'NONE', *, *, #67714, .F. ) ;
#16449=FACE_OUTER_BOUND ( 'NONE', #37908, .T. ) ;
#16450=( BOUNDED_CURVE ( )  B_SPLINE_CURVE ( 2, ( #30543, #8247, #37625, #91375, #640, #85282, #92380, #38626, #7229 ),
 .UNSPECIFIED., .F., .T. ) 
 B_SPLINE_CURVE_WITH_KNOTS ( ( 3, 2, 2, 2, 3 ),
 ( 0.2137096774193548432, 0.2150537634408602183, 0.2177419354838709686, 0.2204301075268817189, 0.2217741935483870941 ),
 .UNSPECIFIED. ) 
 CURVE ( )  GEOMETRIC_REPRESENTATION_ITEM ( )  RATIONAL_B_SPLINE_CURVE ( ( 0.9330127018922194093, 0.9330127018922194093, 1.000000000000000000, 0.8660254037844387076, 1.000000000000000000, 0.8660254037844387076, 1.000000000000000000, 0.9330127018922194093, 0.9330127018922194093 ) ) 
 REPRESENTATION_ITEM ( '' )  );
#16453=CIRCLE ( 'NONE', #74703, 17.82106496071138935 ) ;
#16454=CARTESIAN_POINT ( 'NONE',  ( 207.8718670335145475, 270.6023601641878713, -6.322166851501095586 ) ) ;
#16455=CARTESIAN_POINT ( 'NONE',  ( 90.16093569141993669, 222.8615022471902591, -10.00000000000009592 ) ) ;
#16458=CARTESIAN_POINT ( 'NONE',  ( 40.22915850269944116, 194.0333772461660544, 9.188101187500095079 ) ) ;
#16459=CARTESIAN_POINT ( 'NONE',  ( 199.7050857508973536, 277.1576266663558386, 15.11540184541819976 ) ) ;
#16461=CARTESIAN_POINT ( 'NONE',  ( 152.9972683157861013, 273.5452038669419608, -11.80502568439283095 ) ) ;
#16463=EDGE_CURVE ( 'NONE', #32845, #71681, #58906, .T. ) ;
#16464=CARTESIAN_POINT ( 'NONE',  ( 175.2015549758991426, 281.4682759215078249, -14.19524567657169634 ) ) ;
#16465=CARTESIAN_POINT ( 'NONE',  ( 196.0034224882197975, 291.1591091234520263, 17.53794140922627776 ) ) ;
#16467=CARTESIAN_POINT ( 'NONE',  ( 67.64427519302456915, 199.8615022471901739, 5.000000000000051514 ) ) ;
#16468=CARTESIAN_POINT ( 'NONE',  ( 186.2100982136382186, 283.2556687510013944, 16.40921232443700717 ) ) ;
#16469=CARTESIAN_POINT ( 'NONE',  ( 194.4826705584825390, 293.7931287314651740, -16.11258321617245315 ) ) ;
#16472=CARTESIAN_POINT ( 'NONE',  ( 189.4853509765368926, 263.0536865835545086, 7.945816303330112795 ) ) ;
#16473=CARTESIAN_POINT ( 'NONE',  ( 168.6336870076176808, 278.4479093902589284, 14.14941165673452161 ) ) ;
#16476=CARTESIAN_POINT ( 'NONE',  ( 190.3144310910409445, 301.0127312671879167, -1.334877248546042949 ) ) ;
#16480=CARTESIAN_POINT ( 'NONE',  ( 163.7038023771459052, 247.1036922210055025, -6.448491958542482472 ) ) ;
#16481=CARTESIAN_POINT ( 'NONE',  ( 181.3555717946182426, 267.9129953831518378, 15.03121414418437141 ) ) ;
#16482=CARTESIAN_POINT ( 'NONE',  ( 120.4179585561885659, 231.1423013555409796, -4.594050593750043987 ) ) ;
#16484=CARTESIAN_POINT ( 'NONE',  ( 191.1489696025915919, 299.5672681643093256, 8.892130899335590755 ) ) ;
#16486=FACE_OUTER_BOUND ( 'NONE', #37660, .T. ) ;
#16487=CARTESIAN_POINT ( 'NONE',  ( 194.4026365859849932, 278.7051034128888318, 16.29805033731604169 ) ) ;
#16488=CARTESIAN_POINT ( 'NONE',  ( 204.2346432313999571, 272.7292428585745370, -9.744538825520306702 ) ) ;
#16489=CARTESIAN_POINT ( 'NONE',  ( 191.3704903915450188, 262.8878367245375784, -4.354269820778342570 ) ) ;
#16491=CARTESIAN_POINT ( 'NONE',  ( 106.0200258946745322, 242.0177522451419350, 5.000000000000046185 ) ) ;
#16494=CARTESIAN_POINT ( 'NONE',  ( 192.4371825538271992, 267.1441898236624297, 11.03930663723062011 ) ) ;
#16495=AXIS2_PLACEMENT_3D ( 'NONE', #19555, #72760, #50415 ) ;
#16499=B_SPLINE_SURFACE_WITH_KNOTS ( 'NONE', 3, 1, ( 
 ( #23909, #8224 ),
 ( #85786, #70512 ),
 ( #24419, #63913 ),
 ( #33524, #55296 ),
 ( #62913, #2131 ),
 ( #62396, #93352 ),
 ( #16317, #40602 ),
 ( #41097, #55786 ),
 ( #86276, #9220 ),
 ( #56304, #39591 ),
 ( #94852, #86779 ),
 ( #56809, #78133 ),
 ( #48217, #71038 ),
 ( #25412, #18335 ),
 ( #16812, #40096 ),
 ( #43601, #90258 ),
 ( #97338, #49712 ),
 ( #4109, #74538 ),
 ( #20326, #42107 ),
 ( #59280, #11731 ),
 ( #89758, #50212 ),
 ( #81653, #73041 ),
 ( #72547, #88278 ),
 ( #81165, #65414 ),
 ( #51196, #74028 ),
 ( #18831, #34514 ),
 ( #95870, #41604 ),
 ( #80667, #11244 ),
 ( #58303, #96357 ),
 ( #4616, #89279 ),
 ( #5116, #73527 ),
 ( #64925, #65904 ),
 ( #12226, #19828 ),
 ( #35997, #43085 ) ),
 .UNSPECIFIED., .T., .F., .F.,
 ( 4, 2, 2, 2, 2, 2, 2, 2, 2, 2, 2, 2, 2, 2, 2, 2, 4 ),
 ( 2, 2 ),
 ( 0.000000000000000000, 0.06250000000000000000, 0.1250000000000000000, 0.1875000000000000000, 0.2500000000000000000, 0.3125000000000000000, 0.3750000000000000000, 0.4375000000000000000, 0.5000000000000000000, 0.5625000000000000000, 0.6250000000000000000, 0.6875000000000000000, 0.7500000000000000000, 0.8125000000000000000, 0.8750000000000000000, 0.9375000000000000000, 1.000000000000000000 ),
 ( 0.000000000000000000, 1.000000000000000000 ),
 .UNSPECIFIED. ) ;
#16501=CARTESIAN_POINT ( 'NONE',  ( 180.2632815608440637, 290.9457125825060189, -11.14479853889756988 ) ) ;
#16505=ORIENTED_EDGE ( 'NONE', *, *, #9431, .T. ) ;
#16506=CARTESIAN_POINT ( 'NONE',  ( 184.9912140082997780, 297.8717511433786171, -3.135484508529590819 ) ) ;
#16510=EDGE_CURVE ( 'NONE', #2250, #25608, #33443, .T. ) ;
#16512=CARTESIAN_POINT ( 'NONE',  ( 199.0226767019651106, 265.2340503415149442, -1.818814813163766475 ) ) ;
#16515=CARTESIAN_POINT ( 'NONE',  ( 159.9040744856012850, 255.4269131533854420, 16.38690128260775936 ) ) ;
#16516=CARTESIAN_POINT ( 'NONE',  ( 204.1780753366177237, 277.0001950557890495, 14.05599973203924158 ) ) ;
#16518=CARTESIAN_POINT ( 'NONE',  ( 172.0910100529608258, 260.0785035667472584, 15.53398388876759206 ) ) ;
#16520=CARTESIAN_POINT ( 'NONE',  ( 203.3684377202211522, 278.4025285431072803, -16.56116267537666076 ) ) ;
#16523=CARTESIAN_POINT ( 'NONE',  ( 195.9433989068402298, 290.8109596964202979, 15.97351100229838039 ) ) ;
#16531=CARTESIAN_POINT ( 'NONE',  ( 164.2904957002474191, 246.0875095769322911, -1.594749884056509748 ) ) ;
#16532=CARTESIAN_POINT ( 'NONE',  ( 189.9106593378625689, 301.7120844583541839, 2.757488645815840744 ) ) ;
#16535=CARTESIAN_POINT ( 'NONE',  ( 167.6408814478219256, 249.1979298630905362, -5.423656658118427565 ) ) ;
#16538=CARTESIAN_POINT ( 'NONE',  ( 154.2046094046408768, 279.5503029169213391, 2.157256874705086869 ) ) ;
#16539=CARTESIAN_POINT ( 'NONE',  ( 125.6409139509397050, 243.3458772461660544, 9.188101187500095079 ) ) ;
#16541=CARTESIAN_POINT ( 'NONE',  ( 183.8986139101176036, 260.8653061663941912, -9.197505754419971424 ) ) ;
#16543=ORIENTED_EDGE ( 'NONE', *, *, #80813, .F. ) ;
#16544=CARTESIAN_POINT ( 'NONE',  ( 155.3053666857671260, 275.9298431561234111, 11.76907774355536418 ) ) ;
#16545=CARTESIAN_POINT ( 'NONE',  ( 200.1572343898514816, 273.9495814528414144, 13.62147189966721683 ) ) ;
#16546=CARTESIAN_POINT ( 'NONE',  ( 177.5773431977876839, 253.6316530246629952, 1.366461747843389807 ) ) ;
#16547=CARTESIAN_POINT ( 'NONE',  ( 174.2556954761228383, 290.5492199356207834, -4.866737863781906981 ) ) ;
#16548=CARTESIAN_POINT ( 'NONE',  ( 192.7328199212471134, 296.8239589408137249, 11.25304608637181225 ) ) ;
#16550=EDGE_CURVE ( 'NONE', #23594, #32604, #93962, .T. ) ;
#16552=CARTESIAN_POINT ( 'NONE',  ( 173.4599143460859239, 287.1962067271440446, -9.656697716713990687 ) ) ;
#16553=CARTESIAN_POINT ( 'NONE',  ( 194.7368014691935514, 293.3529610823404710, 16.16394032022910920 ) ) ;
#16554=EDGE_CURVE ( 'NONE', #76220, #37198, #72232, .T. ) ;
#16555=CARTESIAN_POINT ( 'NONE',  ( 183.6215648671697522, 257.5753772875778509, -6.308267261209747012 ) ) ;
#16557=ORIENTED_EDGE ( 'NONE', *, *, #91175, .F. ) ;
#16559=CARTESIAN_POINT ( 'NONE',  ( 151.0149486366368023, 272.2794807016773575, 11.70507281214681861 ) ) ;
#16562=B_SPLINE_CURVE_WITH_KNOTS ( 'NONE', 3,
 ( #55524, #16544, #56544, #94091 ),
 .UNSPECIFIED., .F., .F.,
 ( 4, 4 ),
 ( 0.006736008396846960601, 0.01176074928893414140 ),
 .UNSPECIFIED. ) ;
#16564=CARTESIAN_POINT ( 'NONE',  ( 191.6240736048601718, 298.7443638935011450, -10.89653124444694932 ) ) ;
#16565=CARTESIAN_POINT ( 'NONE',  ( 190.1751179328237242, 301.2540287353828035, 3.252640783176552475 ) ) ;
#16567=CARTESIAN_POINT ( 'NONE',  ( 161.8372659878727973, 281.7041345820564970, -6.599806340034523267 ) ) ;
#16568=CARTESIAN_POINT ( 'NONE',  ( 154.7234497803183331, 277.1669817346232207, -8.779482032178238526 ) ) ;
#16569=CARTESIAN_POINT ( 'NONE',  ( 152.6740002182599767, 266.2078699576288159, -17.16212636348624088 ) ) ;
#16570=ORIENTED_EDGE ( 'NONE', *, *, #14398, .F. ) ;
#16571=CARTESIAN_POINT ( 'NONE',  ( 146.8358616138309571, 276.3198226421291679, 4.054088818585255716 ) ) ;
#16572=CARTESIAN_POINT ( 'NONE',  ( 164.3663504224794565, 247.9561253440330972, -9.019399920391260039 ) ) ;
#16575=CARTESIAN_POINT ( 'NONE',  ( 188.5957227590319292, 298.5807065412511179, -4.256663340113655103 ) ) ;
#16576=CARTESIAN_POINT ( 'NONE',  ( 192.1640094933931096, 297.8091675017319062, 12.36911124822534447 ) ) ;
#16577=CARTESIAN_POINT ( 'NONE',  ( 204.7200661083698776, 274.0614395018808978, 12.25436898028725530 ) ) ;
#16581=B_SPLINE_CURVE_WITH_KNOTS ( 'NONE', 3,
 ( #40853, #71799, #10484, #26186, #41362, #70778, #2911, #70267, #94614, #47960, #64179, #78902, #33804, #64687, #95637, #63174, #95127, #47471, #16075, #875, #25693, #62660, #93612, #86539, #55062, #78394, #9489, #8975, #80427, #73784, #89057, #11991, #19608, #28171, #36263, #5377, #34767, #4374, #57565, #20586, #82435, #67164, #28663, #72814, #58076, #18594, #49472, #65667 ),
 .UNSPECIFIED., .F., .F.,
 ( 4, 2, 2, 2, 2, 2, 2, 2, 2, 2, 2, 2, 2, 2, 2, 2, 2, 2, 2, 2, 2, 2, 2, 4 ),
 ( 0.0005625401255440777831, 0.0009993461653160591509, 0.001217749185202049618, 0.001326950695145041490, 0.001436152205088033363, 0.001545353715031025236, 0.001654555224974016891, 0.001872958244859952498, 0.002309764284631770151, 0.003183376364175405891, 0.004056988443719042499, 0.004930600523262678239, 0.005367406563034496543, 0.005585809582920406129, 0.005695011092863360921, 0.005749611847834837017, 0.005804212602806313979, 0.005858813357777790942, 0.005913414112749267905, 0.006022615622692071777, 0.006241018642577681255, 0.006677824682348895008, 0.007114630722120110495, 0.007551436761891325115 ),
 .UNSPECIFIED. ) ;
#16582=CARTESIAN_POINT ( 'NONE',  ( 0.9064528339360315989, 162.1423013555410080, -4.594050593750043987 ) ) ;
#16583=CARTESIAN_POINT ( 'NONE',  ( 99.30858933894288043, 218.9548013555409511, -4.594050593750042211 ) ) ;
#16585=CARTESIAN_POINT ( 'NONE',  ( 146.9370072200009645, 276.1446333132804511, -3.799807221059707363 ) ) ;
#16587=CARTESIAN_POINT ( 'NONE',  ( 154.9048824156581361, 262.3438686460345366, -17.40627786727128168 ) ) ;
#16589=CARTESIAN_POINT ( 'NONE',  ( 161.8882824960653579, 250.2482648971885340, -13.83574485983625557 ) ) ;
#16590=CARTESIAN_POINT ( 'NONE',  ( 163.0683798854284703, 248.2042762609320903, 11.26611642476872710 ) ) ;
#16593=CARTESIAN_POINT ( 'NONE',  ( 180.2909215930809523, 290.7362029762227849, 9.342184055492005257 ) ) ;
#16594=CARTESIAN_POINT ( 'NONE',  ( 169.2536829177031450, 252.1151759106098211, -8.809847033144830419 ) ) ;
#16595=CARTESIAN_POINT ( 'NONE',  ( 164.3239256700930468, 246.0296071706643772, -4.221892678519003184 ) ) ;
#16596=CARTESIAN_POINT ( 'NONE',  ( 196.0355168007595523, 291.1035201434990540, 17.55377893960077884 ) ) ;
#16598=CARTESIAN_POINT ( 'NONE',  ( 207.7296438747196134, 270.8486979012336633, -6.692930657757584001 ) ) ;
#16599=CARTESIAN_POINT ( 'NONE',  ( 33.89617418964321871, 196.5024278399160949, -9.188101187500093303 ) ) ;
#16600=CARTESIAN_POINT ( 'NONE',  ( 71.67687952550437558, 206.0643266524160140, 9.188101187500095079 ) ) ;
#16601=CARTESIAN_POINT ( 'NONE',  ( 66.04860371747962233, 197.3932355074535678, -2.679491924311248496 ) ) ;
#16603=CARTESIAN_POINT ( 'NONE',  ( 101.8522786425098730, 229.6115022471902307, 10.00000000000009592 ) ) ;
#16606=B_SPLINE_CURVE_WITH_KNOTS ( 'NONE', 3,
 ( #51893, #35690, #81338, #19020 ),
 .UNSPECIFIED., .F., .F.,
 ( 4, 4 ),
 ( 0.009370377214594900056, 0.01414487375777262641 ),
 .UNSPECIFIED. ) ;
#16608=CARTESIAN_POINT ( 'NONE',  ( 196.2367626659915345, 269.4862306000135845, -10.76191796027563896 ) ) ;
#16610=CARTESIAN_POINT ( 'NONE',  ( 198.6363782946250183, 286.5986958926748116, -18.50260615857378355 ) ) ;
#16611=CARTESIAN_POINT ( 'NONE',  ( 196.3286486926436680, 290.5958008134369948, -16.58330917766970458 ) ) ;
#16613=CARTESIAN_POINT ( 'NONE',  ( 67.69866210081085001, 200.7048013555409796, 4.594050593750051981 ) ) ;
#16614=CARTESIAN_POINT ( 'NONE',  ( 170.7953178271928039, 255.2457615276028093, -12.92277808742838374 ) ) ;
#16615=CARTESIAN_POINT ( 'NONE',  ( 202.8151641853381477, 279.3608264160075692, -16.28741359973609448 ) ) ;
#16616=CARTESIAN_POINT ( 'NONE',  ( 197.8809552785519656, 287.9071269377202498, 17.61728046362068412 ) ) ;
#16618=CARTESIAN_POINT ( 'NONE',  ( 198.9738057768446993, 281.0626889417751499, 17.36572826697628003 ) ) ;
#16621=CARTESIAN_POINT ( 'NONE',  ( 104.8833675557553704, 241.3615022471903160, 5.000000000000046185 ) ) ;
#16622=CARTESIAN_POINT ( 'NONE',  ( 161.8662906133268393, 250.2863559554455719, 14.03735902266321744 ) ) ;
#16623=CARTESIAN_POINT ( 'NONE',  ( 164.9779129355220562, 244.8968679994381148, -1.771286574179712803 ) ) ;
#16626=CARTESIAN_POINT ( 'NONE',  ( 187.3515396730908265, 272.9474742628501645, 15.64971660612648030 ) ) ;
#16628=CARTESIAN_POINT ( 'NONE',  ( 206.8851632406098702, 272.3113812655195716, -9.957011741946159233 ) ) ;
#16629=CARTESIAN_POINT ( 'NONE',  ( 190.1002787791093738, 279.3508125853905426, -17.07129022450704525 ) ) ;
#16632=CARTESIAN_POINT ( 'NONE',  ( 173.2992619767147744, 251.6738639471601857, -0.1807056420497624716 ) ) ;
#16635=CARTESIAN_POINT ( 'NONE',  ( 194.9385458806846430, 293.0035295114944347, -15.70518692812489192 ) ) ;
#16636=DIRECTION ( 'NONE',  ( -0.8660254037844387076, -0.4999999999999998890, -0.000000000000000000 ) ) ;
#16638=ORIENTED_EDGE ( 'NONE', *, *, #1993, .F. ) ;
#16640=CARTESIAN_POINT ( 'NONE',  ( 26.34568874650619463, 186.0177522451418497, -10.00000000000009592 ) ) ;
#16644=ORIENTED_EDGE ( 'NONE', *, *, #65419, .F. ) ;
#16646=B_SPLINE_CURVE_WITH_KNOTS ( 'NONE', 3,
 ( #42539, #18773, #25880, #18276, #27856, #64360, #10172, #49171, #80106, #57246, #19291, #80608, #96296, #41548, #41039, #11185, #71975, #72987, #89227, #3095, #88721, #3578, #19776, #50158, #34459, #73472, #26865, #4055, #81110, #57744, #65842, #96806, #27365, #58248, #81597, #12166, #98272, #68836, #59222, #20268, #90198, #97775, #91681, #12677, #14152, #7041, #52633, #60718, #59738, #44031 ),
 .UNSPECIFIED., .F., .F.,
 ( 4, 2, 2, 2, 2, 2, 2, 2, 2, 2, 2, 2, 2, 2, 2, 2, 2, 2, 2, 2, 2, 2, 2, 2, 4 ),
 ( 0.0005940201049859090802, 0.001027528587323273124, 0.001244282828491905489, 0.001352659949076183941, 0.001461037069660462394, 0.001569414190244740846, 0.001677791310829019299, 0.001894545551997614367, 0.002328054034334755065, 0.003195070999009091972, 0.004062087963683428879, 0.004929104928357765786, 0.005362613410694924698, 0.005579367651863502420, 0.005687744772447786076, 0.005741933332739927037, 0.005796121893032067998, 0.005850310453324208959, 0.005904499013616349920, 0.006012876134200668271, 0.006229630375369433343, 0.006663138857707095325, 0.006879893098875905499, 0.007096647340044715674, 0.007530155822382190306 ),
 .UNSPECIFIED. ) ;
#16647=CARTESIAN_POINT ( 'NONE',  ( 160.1795347027651815, 282.8633239002924711, 5.491715875156680582 ) ) ;
#16649=CARTESIAN_POINT ( 'NONE',  ( 170.8148024314547797, 284.7141682455830960, 10.99588700018169618 ) ) ;
#16652=CARTESIAN_POINT ( 'NONE',  ( 163.4178923001155681, 247.5989030008181260, -10.38047187240561442 ) ) ;
#16653=CARTESIAN_POINT ( 'NONE',  ( 185.2391986358457530, 295.7873944733689768, 8.585680893828113724 ) ) ;
#16655=CARTESIAN_POINT ( 'NONE',  ( 157.3661765229227285, 258.0807821998820373, -18.27254492731150748 ) ) ;
#16656=CARTESIAN_POINT ( 'NONE',  ( 147.8871150585349881, 250.0643266524159571, -9.188101187500093303 ) ) ;
#16657=CARTESIAN_POINT ( 'NONE',  ( 206.4855316718497704, 270.5831568970470471, 2.844589147210771163 ) ) ;
#16660=CARTESIAN_POINT ( 'NONE',  ( 89.53865347855843027, 216.3768266524159856, 9.188101187500098632 ) ) ;
#16662=CARTESIAN_POINT ( 'NONE',  ( 191.3638605175971747, 299.1950661814348678, 7.382965314423603154 ) ) ;
#16665=CARTESIAN_POINT ( 'NONE',  ( 195.3366900501289081, 292.3139235812797097, -16.23544628325368677 ) ) ;
#16670=B_SPLINE_CURVE_WITH_KNOTS ( 'NONE', 3,
 ( #26984, #58842, #65971, #20890 ),
 .UNSPECIFIED., .F., .F.,
 ( 4, 4 ),
 ( 0.01149519226291654053, 0.01747808870979753251 ),
 .UNSPECIFIED. ) ;
#16674=EDGE_CURVE ( 'NONE', #35319, #1341, #29585, .T. ) ;
#16675=CYLINDRICAL_SURFACE ( 'NONE', #22056, 17.82106496071139645 ) ;
#16676=CARTESIAN_POINT ( 'NONE',  ( 85.69549220138247847, 220.2833772461660544, -9.188101187500095079 ) ) ;
#16677=ORIENTED_EDGE ( 'NONE', *, *, #2397, .F. ) ;
#16678=EDGE_CURVE ( 'NONE', #47832, #39418, #67354, .T. ) ;
#16679=ORIENTED_EDGE ( 'NONE', *, *, #63333, .F. ) ;
#16680=CARTESIAN_POINT ( 'NONE',  ( 208.0006710756887287, 270.3792650189220126, -0.8737665032493013850 ) ) ;
#16682=ORIENTED_EDGE ( 'NONE', *, *, #60800, .T. ) ;
#16683=B_SPLINE_CURVE_WITH_KNOTS ( 'NONE', 3,
 ( #27791, #59662, #27296, #88652 ),
 .UNSPECIFIED., .F., .F.,
 ( 4, 4 ),
 ( 0.003490422054099921560, 0.008938099447508861262 ),
 .UNSPECIFIED. ) ;
#16687=CARTESIAN_POINT ( 'NONE',  ( 198.4864866673927963, 270.7146468523363865, -12.49260379043138158 ) ) ;
#16688=CARTESIAN_POINT ( 'NONE',  ( 182.6190391695882624, 260.4331822435277104, -11.41224075906783497 ) ) ;
#16691=CARTESIAN_POINT ( 'NONE',  ( 189.3799976626108048, 295.0441500152971344, 11.39732311151665733 ) ) ;
#16692=CARTESIAN_POINT ( 'NONE',  ( 185.8665295013605601, 259.3226075094696057, 5.962194205549277370 ) ) ;
#16693=CARTESIAN_POINT ( 'NONE',  ( 206.2809287719926488, 273.3579460648492159, -10.70911012174624588 ) ) ;
#16694=CARTESIAN_POINT ( 'NONE',  ( 147.7893382324786273, 275.1191502349608982, -4.499236673701186184 ) ) ;
#16697=CARTESIAN_POINT ( 'NONE',  ( 195.6914848190668863, 279.7035040353765680, -17.46620344769279853 ) ) ;
#16700=CARTESIAN_POINT ( 'NONE',  ( 161.2799361541916028, 251.3019516699124836, 14.40628917569557110 ) ) ;
#16702=CARTESIAN_POINT ( 'NONE',  ( 187.4537318743986987, 265.8610463774303980, -11.83450410342445736 ) ) ;
#16703=CARTESIAN_POINT ( 'NONE',  ( 199.0746189151364831, 265.2438329385483939, 1.559867394473611002 ) ) ;
#16706=CARTESIAN_POINT ( 'NONE',  ( 202.4323889586180201, 280.0238125565655878, 15.69595176008160919 ) ) ;
#16708=CARTESIAN_POINT ( 'NONE',  ( 207.1601050488701503, 271.8351680844880889, 6.320235450527015075 ) ) ;
#16709=CARTESIAN_POINT ( 'NONE',  ( 177.4388027723078665, 264.4896303202365857, -15.65959907089493619 ) ) ;
#16711=CARTESIAN_POINT ( 'NONE',  ( 199.1807827224510845, 281.9190771098037658, -16.60222886460724112 ) ) ;
#16713=CARTESIAN_POINT ( 'NONE',  ( 172.0224699280288974, 275.0334117845947617, 16.95724843200788712 ) ) ;
#16714=CARTESIAN_POINT ( 'NONE',  ( 163.3157238902107906, 283.7599821633143051, -3.437047550650083938 ) ) ;
#16716=CARTESIAN_POINT ( 'NONE',  ( 192.0091641151854844, 261.6684110230355600, 3.065581067129474757 ) ) ;
#16717=CARTESIAN_POINT ( 'NONE',  ( 186.5128128464827455, 296.3652354721813822, -8.829210103799347564 ) ) ;
#16718=CARTESIAN_POINT ( 'NONE',  ( 4.614210867829412699, 161.2202760586659451, -5.415160957724236172E-17 ) ) ;
#16723=CARTESIAN_POINT ( 'NONE',  ( 175.2285374422532414, 254.6787769949789322, 9.431799880968993577 ) ) ;
#16724=CARTESIAN_POINT ( 'NONE',  ( 203.5726949774746117, 269.0034548673361883, -6.096665150295551783 ) ) ;
#16726=CARTESIAN_POINT ( 'NONE',  ( 27.18482440607883888, 180.3768266524160140, 9.188101187500096856 ) ) ;
#16731=CARTESIAN_POINT ( 'NONE',  ( 146.8859094598974480, 276.2331372299326517, -0.7994986043261681496 ) ) ;
#16732=CARTESIAN_POINT ( 'NONE',  ( 14.08707949041329144, 167.3932355074535394, -2.679491924311274254 ) ) ;
#16733=B_SPLINE_SURFACE_WITH_KNOTS ( 'NONE', 3, 1, ( 
 ( #54997, #7923 ),
 ( #62088, #30717 ),
 ( #47399, #311 ),
 ( #78325, #61598 ),
 ( #39774, #91548 ),
 ( #77315, #84946 ),
 ( #53008, #83959 ),
 ( #45405, #76336 ),
 ( #6909, #37797 ),
 ( #38798, #92067 ),
 ( #92549, #7402 ),
 ( #15490, #46390 ),
 ( #69703, #31198 ),
 ( #16997, #73224 ),
 ( #49407, #71228 ),
 ( #94049, #18523 ),
 ( #9925, #63603 ),
 ( #40786, #78828 ),
 ( #32703, #65108 ),
 ( #47886, #57493 ),
 ( #86974, #48918 ),
 ( #1820, #86470 ),
 ( #80354, #25097 ),
 ( #94543, #56502 ),
 ( #19035, #3336 ),
 ( #56994, #2837 ),
 ( #32201, #72230 ),
 ( #95572, #26615 ),
 ( #26117, #49907 ),
 ( #34213, #55483 ),
 ( #87976, #2327 ),
 ( #88473, #9410 ),
 ( #55979, #17506 ),
 ( #48412, #95056 ) ),
 .UNSPECIFIED., .T., .F., .F.,
 ( 4, 2, 2, 2, 2, 2, 2, 2, 2, 2, 2, 2, 2, 2, 2, 2, 4 ),
 ( 2, 2 ),
 ( 0.000000000000000000, 0.06250000000000000000, 0.1250000000000000000, 0.1875000000000000000, 0.2500000000000000000, 0.3125000000000000000, 0.3750000000000000000, 0.4375000000000000000, 0.5000000000000000000, 0.5625000000000000000, 0.6250000000000000000, 0.6875000000000000000, 0.7500000000000000000, 0.8125000000000000000, 0.8750000000000000000, 0.9375000000000000000, 1.000000000000000000 ),
 ( 0.000000000000000000, 1.000000000000000000 ),
 .UNSPECIFIED. ) ;
#16734=CARTESIAN_POINT ( 'NONE',  ( 186.9002619757878279, 295.9402723794265171, -7.697862465556936762 ) ) ;
#16737=CARTESIAN_POINT ( 'NONE',  ( 60.71607196274899110, 215.8615022471903160, 5.000000000000046185 ) ) ;
#16738=( BOUNDED_CURVE ( )  B_SPLINE_CURVE ( 2, ( #23305, #78536, #47110, #93764, #77010, #16218, #54194, #24322, #86181 ),
 .UNSPECIFIED., .F., .T. ) 
 B_SPLINE_CURVE_WITH_KNOTS ( ( 3, 2, 2, 2, 3 ),
 ( 0.8830645161290322509, 0.8844086021505376261, 0.8870967741935483764, 0.8897849462365591267, 0.8911290322580645018 ),
 .UNSPECIFIED. ) 
 CURVE ( )  GEOMETRIC_REPRESENTATION_ITEM ( )  RATIONAL_B_SPLINE_CURVE ( ( 0.9330127018922194093, 0.9330127018922194093, 1.000000000000000000, 0.8660254037844387076, 1.000000000000000000, 0.8660254037844387076, 1.000000000000000000, 0.9330127018922194093, 0.9330127018922194093 ) ) 
 REPRESENTATION_ITEM ( '' )  );
#16740=CARTESIAN_POINT ( 'NONE',  ( 203.5026800799811895, 269.8567082039247111, 6.928182654214480429 ) ) ;
#16741=CARTESIAN_POINT ( 'NONE',  ( 41.71789998727770410, 185.7048013555409796, 4.594050593750051981 ) ) ;
#16744=CARTESIAN_POINT ( 'NONE',  ( 204.5222561433589021, 270.7959794724876588, -6.481264364560415103 ) ) ;
#16745=CARTESIAN_POINT ( 'NONE',  ( 175.8062715677771166, 253.2953273735088544, -6.838868645307838001 ) ) ;
#16747=CARTESIAN_POINT ( 'NONE',  ( 6.060800048784472871, 162.7592609112380444, 2.679491924311254714 ) ) ;
#16748=CARTESIAN_POINT ( 'NONE',  ( 202.8902555442842868, 278.4536566332962479, -15.11955846344091547 ) ) ;
#16751=CARTESIAN_POINT ( 'NONE',  ( 203.0535368433499457, 278.9479528611958585, 16.46202213522710167 ) ) ;
#16752=CARTESIAN_POINT ( 'NONE',  ( 149.4171629335945681, 271.8488776066536730, -11.42564036194071520 ) ) ;
#16753=CARTESIAN_POINT ( 'NONE',  ( 186.7162059521595836, 267.9499891762567358, -15.17631223955298303 ) ) ;
#16758=CARTESIAN_POINT ( 'NONE',  ( 23.45662567177863167, 195.8967562850347122, -4.648177544792955347E-16 ) ) ;
#16760=CARTESIAN_POINT ( 'NONE',  ( 190.7779368023172708, 300.2099158256590385, 8.142228434510803581 ) ) ;
#16761=CARTESIAN_POINT ( 'NONE',  ( 178.8559941927174748, 256.9455126458981340, -7.290009489429222889 ) ) ;
#16762=ORIENTED_EDGE ( 'NONE', *, *, #64850, .F. ) ;
#16763=VERTEX_POINT ( 'NONE', #62155 ) ;
#16771=CARTESIAN_POINT ( 'NONE',  ( 148.0389988358468827, 274.2359278451201590, 7.783622668412842671 ) ) ;
#16772=CARTESIAN_POINT ( 'NONE',  ( 196.2421909983451940, 290.7455499326673021, -17.31908925000307065 ) ) ;
#16773=CARTESIAN_POINT ( 'NONE',  ( 181.1477013271936016, 287.8971774238942203, -14.15342935774602218 ) ) ;
#16780=EDGE_CURVE ( 'NONE', #63237, #15171, #19450, .T. ) ;
#16781=CARTESIAN_POINT ( 'NONE',  ( 198.2040940955416488, 287.3474340887963763, 16.95806375232200480 ) ) ;
#16783=CARTESIAN_POINT ( 'NONE',  ( 56.60219097117523290, 212.6744531367911293, 4.594050593750047540 ) ) ;
#16784=EDGE_LOOP ( 'NONE', ( #10998, #40926, #11071, #97205 ) ) ;
#16787=CARTESIAN_POINT ( 'NONE',  ( 197.9637121306999461, 287.7637878651254937, 17.83088679657193865 ) ) ;
#16788=CARTESIAN_POINT ( 'NONE',  ( 176.3169295130042258, 273.0865261982322636, 16.85758906909942567 ) ) ;
#16789=ORIENTED_EDGE ( 'NONE', *, *, #82260, .F. ) ;
#16790=AXIS2_PLACEMENT_3D ( 'NONE', #72998, #57258, #34955 ) ;
#16791=CARTESIAN_POINT ( 'NONE',  ( 190.5346086712997078, 299.7911943260875205, 5.206985090025521679 ) ) ;
#16796=CARTESIAN_POINT ( 'NONE',  ( 110.0998739067015606, 222.8262482093458061, 3.021315404115420679E-15 ) ) ;
#16797=CARTESIAN_POINT ( 'NONE',  ( 175.6063544791335573, 254.0105997054014040, 8.344378697908656051 ) ) ;
#16798=CARTESIAN_POINT ( 'NONE',  ( 161.4816992964961742, 250.9524876563463067, -12.92750327687364198 ) ) ;
#16800=CARTESIAN_POINT ( 'NONE',  ( 147.1603453755519695, 275.7578002805973370, -5.230822882238410187 ) ) ;
#16801=CARTESIAN_POINT ( 'NONE',  ( 190.8153366230912411, 300.1451374358846920, 3.771947273125533684 ) ) ;
#16802=CARTESIAN_POINT ( 'NONE',  ( 180.5734370714514228, 271.1176088554109356, 17.19503379674203103 ) ) ;
#16803=CARTESIAN_POINT ( 'NONE',  ( 164.3493441216711517, 245.9855811210807417, 1.722120810491653664 ) ) ;
#16805=CARTESIAN_POINT ( 'NONE',  ( 154.8782533782051871, 264.3899914918594050, -17.45241046926759765 ) ) ;
#16806=CARTESIAN_POINT ( 'NONE',  ( -22.42236680055709641, 157.8615022471902591, 0.000000000000000000 ) ) ;
#16807=CARTESIAN_POINT ( 'NONE',  ( 117.3868696429430258, 229.3923013555409796, 4.594050593750050204 ) ) ;
#16809=CARTESIAN_POINT ( 'NONE',  ( 191.3610003135137276, 299.2000202002271294, -9.855749861282104618 ) ) ;
#16811=CARTESIAN_POINT ( 'NONE',  ( 202.8151641853381477, 279.3608264160075692, -16.28741359973609448 ) ) ;
#16812=CARTESIAN_POINT ( 'NONE',  ( 204.2133777088835700, 276.9390495533970693, 13.75768580338462144 ) ) ;
#16814=CARTESIAN_POINT ( 'NONE',  ( 174.8285612161963058, 252.5975812908445732, 5.144082065870574816 ) ) ;
#16815=ORIENTED_EDGE ( 'NONE', *, *, #57491, .F. ) ;
#16816=CARTESIAN_POINT ( 'NONE',  ( 163.3939361803663246, 247.6403962173759226, -10.78041711314006790 ) ) ;
#16818=CARTESIAN_POINT ( 'NONE',  ( 24.59328401069779346, 196.5530062829863311, -4.648177544792955347E-16 ) ) ;
#16819=CARTESIAN_POINT ( 'NONE',  ( 206.2536424468873406, 272.9128265684719281, 8.671401193505188232 ) ) ;
#16820=CARTESIAN_POINT ( 'NONE',  ( 136.3040252829181327, 243.3768266524160140, 9.188101187500096856 ) ) ;
#16821=CARTESIAN_POINT ( 'NONE',  ( 198.5970767652345899, 286.6667681383942181, -17.17073100918929640 ) ) ;
#16822=CARTESIAN_POINT ( 'NONE',  ( 185.3345560757713315, 297.6803563334680689, 4.160651365811766311 ) ) ;
#16823=CARTESIAN_POINT ( 'NONE',  ( 187.4269513160483314, 281.3598214497520189, -17.37670249948783763 ) ) ;
#16825=CARTESIAN_POINT ( 'NONE',  ( 55.49285624440017273, 202.8458772461660260, 9.188101187500095079 ) ) ;
#16829=CARTESIAN_POINT ( 'NONE',  ( 181.8509774751104544, 266.9677320091309412, 16.09658033613713712 ) ) ;
#16830=B_SPLINE_CURVE_WITH_KNOTS ( 'NONE', 3,
 ( #44546, #98287, #35960, #29373, #36958, #75995, #30361 ),
 .UNSPECIFIED., .F., .F.,
 ( 4, 3, 4 ),
 ( 0.000000000000000000, 0.001498044977020785264, 0.001890351849317388738 ),
 .UNSPECIFIED. ) ;
#16833=CARTESIAN_POINT ( 'NONE',  ( 151.3082152111609844, 278.3337183599618356, -1.667790407313227918 ) ) ;
#16835=CARTESIAN_POINT ( 'NONE',  ( 178.8406662910292084, 261.3676314715743274, 12.21613212044301022 ) ) ;
#16836=CARTESIAN_POINT ( 'NONE',  ( 114.7524487161675779, 250.3927522451419634, 2.944929066748280225E-16 ) ) ;
#16838=VERTEX_POINT ( 'NONE', #2396 ) ;
#16839=CARTESIAN_POINT ( 'NONE',  ( 163.1014434023538513, 248.1470085697407058, 9.692260209037655727 ) ) ;
#16841=EDGE_CURVE ( 'NONE', #54426, #49659, #63566, .T. ) ;
#16842=CARTESIAN_POINT ( 'NONE',  ( 24.91150772114469092, 179.0643266524160140, 9.188101187500095079 ) ) ;
#16844=CARTESIAN_POINT ( 'NONE',  ( 188.7579712926501543, 290.5937008958214847, -14.99838659903155325 ) ) ;
#16848=CARTESIAN_POINT ( 'NONE',  ( 51.02741275436266477, 210.2677522451419350, -5.000000000000047962 ) ) ;
#16849=EDGE_CURVE ( 'NONE', #95819, #95312, #17859, .T. ) ;
#16850=CARTESIAN_POINT ( 'NONE',  ( 173.2055275001436314, 289.0856056677645824, 8.083435772122928853 ) ) ;
#16851=CARTESIAN_POINT ( 'NONE',  ( 163.2029997909485814, 256.0468373663799753, -14.94059154133669587 ) ) ;
#16852=CARTESIAN_POINT ( 'NONE',  ( 204.6149525604204769, 276.2435015074934199, -13.22810747389629960 ) ) ;
#16853=CARTESIAN_POINT ( 'NONE',  ( 162.2496630651073701, 251.8436134512154183, -12.97535039530458967 ) ) ;
#16856=CARTESIAN_POINT ( 'NONE',  ( 161.8567175149206321, 267.2024831904969346, 16.48631320651076848 ) ) ;
#16857=CARTESIAN_POINT ( 'NONE',  ( 21.74492879244924382, 193.3615022471903160, 5.000000000000046185 ) ) ;
#16858=DIRECTION ( 'NONE',  ( 0.8660254037844395958, 0.4999999999999985567, 0.000000000000000000 ) ) ;
#16859=CARTESIAN_POINT ( 'NONE',  ( 202.2603678735342214, 280.3217618159037556, 16.49712126737133744 ) ) ;
#16860=CARTESIAN_POINT ( 'NONE',  ( -6.590166341514275494, 160.8768266524160140, 9.188101187500098632 ) ) ;
#16862=CARTESIAN_POINT ( 'NONE',  ( 164.5093404746413910, 259.6730185065525802, -16.72720059574769991 ) ) ;
#16863=CARTESIAN_POINT ( 'NONE',  ( 200.2141246490667754, 282.1197396120186909, 17.30140834831486529 ) ) ;
#16865=CARTESIAN_POINT ( 'NONE',  ( 185.5400204171384075, 259.9029772015394428, 7.379271805359726599 ) ) ;
#16866=CARTESIAN_POINT ( 'NONE',  ( 206.4537138826727301, 273.0586734743599209, 11.45643784582899016 ) ) ;
#16868=CARTESIAN_POINT ( 'NONE',  ( 186.6238840102718086, 259.3006934494294455, -2.364174896264719994 ) ) ;
#16872=CARTESIAN_POINT ( 'NONE',  ( 179.8194114752668042, 286.2860187198718904, 13.09292147992676902 ) ) ;
#16873=CARTESIAN_POINT ( 'NONE',  ( 154.6671547551263757, 278.4911608342019349, -5.208367705655446045 ) ) ;
#16875=CARTESIAN_POINT ( 'NONE',  ( 207.2585079244812221, 271.6647293043187688, 8.480643094032153328 ) ) ;
#16876=CARTESIAN_POINT ( 'NONE',  ( 206.4484807199597753, 273.0677375780628608, -9.220527398138528952 ) ) ;
#16879=CARTESIAN_POINT ( 'NONE',  ( 80.61430232155159104, 228.8967562850347122, -4.648177544792955347E-16 ) ) ;
#16880=CARTESIAN_POINT ( 'NONE',  ( 191.4732661803433018, 298.1837965232045349, 9.193897954715051668 ) ) ;
#16881=CARTESIAN_POINT ( 'NONE',  ( 207.9743173328493526, 270.4249110404894054, -2.481515874287090639 ) ) ;
#16882=CARTESIAN_POINT ( 'NONE',  ( 154.9455285025717615, 262.2734675583710100, 18.28470720339922551 ) ) ;
#16885=DIRECTION ( 'NONE',  ( -0.8660254037844359321, -0.5000000000000051070, -0.000000000000000000 ) ) ;
#16886=CARTESIAN_POINT ( 'NONE',  ( 89.54518929453067244, 234.0530062829863027, -4.648177544792955347E-16 ) ) ;
#16887=ORIENTED_EDGE ( 'NONE', *, *, #86343, .T. ) ;
#16888=CARTESIAN_POINT ( 'NONE',  ( 188.8891845508813390, 297.3683201713357107, 7.792454418634450874 ) ) ;
#16889=EDGE_LOOP ( 'NONE', ( #45028, #39770, #78188, #29137 ) ) ;
#16890=DIRECTION ( 'NONE',  ( 0.4999999999999992784, -0.8660254037844390407, 0.000000000000000000 ) ) ;
#16893=ORIENTED_EDGE ( 'NONE', *, *, #6915, .T. ) ;
#16894=CARTESIAN_POINT ( 'NONE',  ( 200.4592688079413847, 283.4413569069752725, 18.39277739746426832 ) ) ;
#16896=CARTESIAN_POINT ( 'NONE',  ( 191.4484954869714954, 299.0484741143815199, 8.684991747358081327 ) ) ;
#16897=CARTESIAN_POINT ( 'NONE',  ( 149.4284094220488157, 274.0275188989749040, -8.736341709343308892 ) ) ;
#16898=ORIENTED_EDGE ( 'NONE', *, *, #80886, .F. ) ;
#16899=EDGE_CURVE ( 'NONE', #65652, #62907, #86335, .T. ) ;
#16901=CARTESIAN_POINT ( 'NONE',  ( 170.6773407966179263, 255.4795565429710678, -11.51496627275842144 ) ) ;
#16903=ORIENTED_EDGE ( 'NONE', *, *, #26150, .F. ) ;
#16905=ORIENTED_EDGE ( 'NONE', *, *, #6844, .T. ) ;
#16906=CARTESIAN_POINT ( 'NONE',  ( 149.4596969528118393, 273.7752065243203106, 10.43958276706939614 ) ) ;
#16910=CARTESIAN_POINT ( 'NONE',  ( 168.8745654493266102, 272.6928345997080783, 16.05439322531100999 ) ) ;
#16911=CARTESIAN_POINT ( 'NONE',  ( 164.4068639292406715, 270.3611440525622811, 17.36650109901806971 ) ) ;
#16912=CARTESIAN_POINT ( 'NONE',  ( 194.5252985417586729, 293.7192948986070178, -14.54632727629426370 ) ) ;
#16914=EDGE_CURVE ( 'NONE', #79192, #13224, #16581, .T. ) ;
#16915=CARTESIAN_POINT ( 'NONE',  ( 197.7164576114591341, 288.1920452548512230, -17.18932158603989180 ) ) ;
#16916=B_SPLINE_CURVE_WITH_KNOTS ( 'NONE', 3,
 ( #8036, #32318, #63219, #38407 ),
 .UNSPECIFIED., .F., .F.,
 ( 4, 4 ),
 ( 0.01205678105519798413, 0.01821341545976904938 ),
 .UNSPECIFIED. ) ;
#16917=CARTESIAN_POINT ( 'NONE',  ( 166.8603047740130876, 247.0964243085869896, 1.925065518075911530 ) ) ;
#16919=CARTESIAN_POINT ( 'NONE',  ( 164.7297297678022403, 245.3267338555121455, 3.020078936458732599 ) ) ;
#16920=CARTESIAN_POINT ( 'NONE',  ( 197.8977219949227049, 287.8780861330898801, 17.48564646125164046 ) ) ;
#16921=ORIENTED_EDGE ( 'NONE', *, *, #69116, .F. ) ;
#16924=EDGE_CURVE ( 'NONE', #80622, #74751, #70959, .T. ) ;
#16925=CARTESIAN_POINT ( 'NONE',  ( 206.7680519836501958, 272.5142239127119979, -10.57935479673322021 ) ) ;
#16928=FACE_OUTER_BOUND ( 'NONE', #74031, .T. ) ;
#16929=CARTESIAN_POINT ( 'NONE',  ( 190.9750074087093026, 262.0973604801322381, -0.7408433392359728975 ) ) ;
#16930=EDGE_LOOP ( 'NONE', ( #83711, #76580, #66767, #78715 ) ) ;
#16933=CARTESIAN_POINT ( 'NONE',  ( 207.6007741873543750, 271.0719067473055475, 7.587922723682903658 ) ) ;
#16934=CARTESIAN_POINT ( 'NONE',  ( 13.28313890609088688, 185.1427522451419350, -10.00000000000009415 ) ) ;
#16935=CARTESIAN_POINT ( 'NONE',  ( 86.66977078063996487, 220.8458772461660544, 9.188101187500095079 ) ) ;
#16939=CARTESIAN_POINT ( 'NONE',  ( 167.0011108565465747, 278.0668406281866396, -14.45516252385082900 ) ) ;
#16940=CARTESIAN_POINT ( 'NONE',  ( 2.232293911657190488, 172.0958772461660544, -9.188101187500095079 ) ) ;
#16942=CARTESIAN_POINT ( 'NONE',  ( 161.1238074876215478, 251.5723744529297505, 13.42537408252843179 ) ) ;
#16946=CARTESIAN_POINT ( 'NONE',  ( 198.1198657144259982, 265.9800056028663562, -2.879908836942639105 ) ) ;
#16948=CARTESIAN_POINT ( 'NONE',  ( 33.84893051719189572, 201.8967562850347122, -4.648177544792955347E-16 ) ) ;
#16949=CARTESIAN_POINT ( 'NONE',  ( 156.6543370668840680, 266.2741171134555316, 17.28817642186849213 ) ) ;
#16950=CARTESIAN_POINT ( 'NONE',  ( 167.3110317288038686, 250.1317611871268696, 9.699734311170200129 ) ) ;
#16951=CARTESIAN_POINT ( 'NONE',  ( 33.21950506899538880, 199.1744531367911293, 4.594050593750047540 ) ) ;
#16952=CARTESIAN_POINT ( 'NONE',  ( 199.8327978920034411, 276.9379622803334087, 15.19750203934660249 ) ) ;
#16955=CARTESIAN_POINT ( 'NONE',  ( 175.2786348600535860, 281.1565833761089266, -15.16109458501749607 ) ) ;
#16958=CARTESIAN_POINT ( 'NONE',  ( -13.03140383004354241, 163.2833772461660544, -9.188101187500095079 ) ) ;
#16960=CARTESIAN_POINT ( 'NONE',  ( 154.9683083969241011, 262.2340116239618055, 18.33261662430134109 ) ) ;
#16961=CARTESIAN_POINT ( 'NONE',  ( 198.7829547491859330, 286.3448180261817129, -18.59838968157616179 ) ) ;
#16962=CYLINDRICAL_SURFACE ( 'NONE', #72682, 17.82106496071139645 ) ;
#16963=CARTESIAN_POINT ( 'NONE',  ( 147.8308140999695866, 274.5965143850199865, -7.866624397492971710 ) ) ;
#16965=CARTESIAN_POINT ( 'NONE',  ( 192.5271661211833703, 265.1515744257078495, 7.739560070318121987 ) ) ;
#16966=CARTESIAN_POINT ( 'NONE',  ( 163.7010375032499212, 247.1084811230698506, 6.649922295230481950 ) ) ;
#16968=CARTESIAN_POINT ( 'NONE',  ( 191.1687199697037443, 299.5330595250031820, -8.491751560014430211 ) ) ;
#16969=CARTESIAN_POINT ( 'NONE',  ( 190.6084209867335915, 300.5035258309363826, -0.5505750481748228342 ) ) ;
#16970=ORIENTED_EDGE ( 'NONE', *, *, #27535, .F. ) ;
#16971=CARTESIAN_POINT ( 'NONE',  ( 152.5423653171682474, 268.4358682943698682, -15.78187745328793490 ) ) ;
#16973=CARTESIAN_POINT ( 'NONE',  ( 108.5372593219620683, 221.2202760586659167, -5.415160957724236172E-17 ) ) ;
#16976=EDGE_CURVE ( 'NONE', #37468, #28879, #60795, .T. ) ;
#16978=CARTESIAN_POINT ( 'NONE',  ( 191.5612668698545633, 276.9093416755657699, 16.88675210317316910 ) ) ;
#16979=CARTESIAN_POINT ( 'NONE',  ( 191.3465768251321890, 299.2250024149264505, -6.938973362607056217 ) ) ;
#16980=B_SPLINE_CURVE_WITH_KNOTS ( 'NONE', 3,
 ( #75879, #6457, #66261, #58635 ),
 .UNSPECIFIED., .F., .F.,
 ( 4, 4 ),
 ( 0.01344258228325481003, 0.02205949149894677330 ),
 .UNSPECIFIED. ) ;
#16982=CARTESIAN_POINT ( 'NONE',  ( 149.2923684163597784, 272.0650280510108701, -12.99082738998495756 ) ) ;
#16983=CARTESIAN_POINT ( 'NONE',  ( 83.16056367749568778, 225.4865022471902876, 10.00000000000009415 ) ) ;
#16984=CARTESIAN_POINT ( 'NONE',  ( 173.1636647817533685, 289.7167559925995874, -1.225364899902585902 ) ) ;
#16987=CARTESIAN_POINT ( 'NONE',  ( 130.9983832723993089, 257.9860189848785694, -2.679491924311252493 ) ) ;
#16988=CARTESIAN_POINT ( 'NONE',  ( 175.8776426353156523, 278.6924052921702923, 15.46313303699034059 ) ) ;
#16991=VERTEX_POINT ( 'NONE', #99083 ) ;
#16992=EDGE_CURVE ( 'NONE', #42801, #100197, #5626, .T. ) ;
#16995=FACE_OUTER_BOUND ( 'NONE', #48074, .T. ) ;
#16996=CARTESIAN_POINT ( 'NONE',  ( 194.3094773688834778, 284.8302703302293253, 17.74979085435418469 ) ) ;
#16997=CARTESIAN_POINT ( 'NONE',  ( 192.5254593562406171, 297.1831179748913314, 11.00703791256144015 ) ) ;
#16999=CARTESIAN_POINT ( 'NONE',  ( 191.2585535523842850, 280.2024068932645378, 17.45594619081192889 ) ) ;
#17000=B_SPLINE_SURFACE_WITH_KNOTS ( 'NONE', 3, 1, ( 
 ( #19848, #57324 ),
 ( #58319, #88800 ),
 ( #74557, #97846 ),
 ( #58805, #43616 ),
 ( #97356, #64943 ),
 ( #11748, #11261 ),
 ( #66916, #82179 ),
 ( #50226, #20848 ),
 ( #81670, #42124 ),
 ( #4633, #89294 ),
 ( #50716, #81181 ),
 ( #5133, #66428 ),
 ( #27922, #36015 ),
 ( #95888, #51739 ),
 ( #28415, #27445 ),
 ( #96371, #89769 ),
 ( #42611, #73542 ),
 ( #10746, #59295 ),
 ( #65921, #26449 ),
 ( #41622, #35019 ),
 ( #88296, #3168 ),
 ( #12243, #43102 ),
 ( #72564, #74045 ),
 ( #18852, #73055 ),
 ( #49733, #80686 ),
 ( #35528, #20340 ),
 ( #34530, #65430 ),
 ( #51212, #90276 ),
 ( #26937, #91255 ),
 ( #83158, #68412 ),
 ( #59810, #84654 ),
 ( #98343, #99339 ),
 ( #23303, #67415 ),
 ( #13248, #44105 ) ),
 .UNSPECIFIED., .T., .F., .F.,
 ( 4, 2, 2, 2, 2, 2, 2, 2, 2, 2, 2, 2, 2, 2, 2, 2, 4 ),
 ( 2, 2 ),
 ( 0.000000000000000000, 0.06250000000000000000, 0.1250000000000000000, 0.1875000000000000000, 0.2500000000000000000, 0.3125000000000000000, 0.3750000000000000000, 0.4375000000000000000, 0.5000000000000000000, 0.5625000000000000000, 0.6250000000000000000, 0.6875000000000000000, 0.7500000000000000000, 0.8125000000000000000, 0.8750000000000000000, 0.9375000000000000000, 1.000000000000000000 ),
 ( 0.000000000000000000, 1.000000000000000000 ),
 .UNSPECIFIED. ) ;
#17002=CARTESIAN_POINT ( 'NONE',  ( 176.7804342879712465, 274.6069073446109883, -17.51127113154074522 ) ) ;
#17004=CARTESIAN_POINT ( 'NONE',  ( 167.6448875122848108, 280.9501575304901735, 11.66831761562362857 ) ) ;
#17005=CARTESIAN_POINT ( 'NONE',  ( 147.9133274879049793, 274.4535970048112290, -9.359166267164972908 ) ) ;
#17010=CARTESIAN_POINT ( 'NONE',  ( 71.37900974329706116, 202.0177522451417929, 5.000000000000051514 ) ) ;
#17014=CARTESIAN_POINT ( 'NONE',  ( 155.5587153255869453, 261.2113968263770971, -18.30500480654006878 ) ) ;
#17018=CARTESIAN_POINT ( 'NONE',  ( 95.62772104926125394, 236.0177522451419350, 5.000000000000046185 ) ) ;
#17019=ORIENTED_EDGE ( 'NONE', *, *, #21292, .F. ) ;
#17021=ORIENTED_EDGE ( 'NONE', *, *, #64757, .T. ) ;
#17023=CARTESIAN_POINT ( 'NONE',  ( 203.3349860717029571, 278.4604684979374838, -16.59553970625579566 ) ) ;
#17027=CARTESIAN_POINT ( 'NONE',  ( 205.9334673742153257, 273.9597668594684023, -10.28447216160094158 ) ) ;
#17028=CARTESIAN_POINT ( 'NONE',  ( 190.2767435973494798, 301.0780079210716735, 3.520490206057748317 ) ) ;
#17029=CARTESIAN_POINT ( 'NONE',  ( 156.6812872898450735, 261.2670451491295012, 0.000000000000000000 ) ) ;
#17031=CARTESIAN_POINT ( 'NONE',  ( 167.6860649869540509, 249.0846947427896509, -5.222016127407463237 ) ) ;
#17034=CARTESIAN_POINT ( 'NONE',  ( 153.8583843864966241, 279.6722161493621570, 2.192119895967011622 ) ) ;
#17036=CARTESIAN_POINT ( 'NONE',  ( 134.1932619090760568, 236.0327760586659736, 1.948934522072303157E-15 ) ) ;
#17037=CARTESIAN_POINT ( 'NONE',  ( 186.6308142930050735, 262.8605285626102841, -9.271754035113762171 ) ) ;
#17038=VERTEX_POINT ( 'NONE', #30156 ) ;
#17043=CARTESIAN_POINT ( 'NONE',  ( 200.0693866756322734, 273.7496136914496674, 13.78539325936003657 ) ) ;
#17044=CARTESIAN_POINT ( 'NONE',  ( 180.7525632646832321, 256.2381716922662918, 1.265208511841812600 ) ) ;
#17045=CARTESIAN_POINT ( 'NONE',  ( 174.0979558812879304, 290.0036607898268244, -4.751154830586174604 ) ) ;
#17046=CARTESIAN_POINT ( 'NONE',  ( 192.0448397941376584, 298.0155754755651287, 11.82564086563478156 ) ) ;
#17047=DIRECTION ( 'NONE',  ( -0.8660254037844387076, -0.4999999999999998890, -0.000000000000000000 ) ) ;
#17050=( BOUNDED_CURVE ( )  B_SPLINE_CURVE ( 2, ( #4323, #98039, #29134, #43814, #90478, #75239, #36212, #35224, #89962 ),
 .UNSPECIFIED., .F., .T. ) 
 B_SPLINE_CURVE_WITH_KNOTS ( ( 3, 2, 2, 2, 3 ),
 ( 0.02016129032258064807, 0.02150537634408602322, 0.02419354838709677352, 0.02688172043010752729, 0.02822580645161290591 ),
 .UNSPECIFIED. ) 
 CURVE ( )  GEOMETRIC_REPRESENTATION_ITEM ( )  RATIONAL_B_SPLINE_CURVE ( ( 0.9330127018922192983, 0.9330127018922194093, 1.000000000000000000, 0.8660254037844387076, 1.000000000000000000, 0.8660254037844387076, 1.000000000000000000, 0.9330127018922191873, 0.9330127018922192983 ) ) 
 REPRESENTATION_ITEM ( '' )  );
#17051=CARTESIAN_POINT ( 'NONE',  ( 173.2412943989675398, 277.7050541934257240, 16.79641741871846250 ) ) ;
#17052=CARTESIAN_POINT ( 'NONE',  ( 177.2220074482157770, 256.0735339440234952, -7.327850677533820800 ) ) ;
#17054=CARTESIAN_POINT ( 'NONE',  ( 194.4666154385731431, 293.8209370148700827, -14.56896502715340702 ) ) ;
#17055=CARTESIAN_POINT ( 'NONE',  ( 166.9178459015252542, 248.1196852899930718, -6.726913786253128080 ) ) ;
#17056=VERTEX_POINT ( 'NONE', #21574 ) ;
#17058=CARTESIAN_POINT ( 'NONE',  ( 158.0274747602609580, 277.2166826364630197, 10.25079899571118602 ) ) ;
#17059=CARTESIAN_POINT ( 'NONE',  ( 151.9376213889835299, 267.4833155035536265, -16.92460756927863130 ) ) ;
#17061=CARTESIAN_POINT ( 'NONE',  ( 202.9216520459657147, 279.1763840310111391, 15.75371595331685803 ) ) ;
#17062=CARTESIAN_POINT ( 'NONE',  ( 161.4315010361464431, 281.4375180470930218, -6.688515640316089694 ) ) ;
#17063=CARTESIAN_POINT ( 'NONE',  ( 154.5109925159944169, 277.6691952191739574, -9.102046555125145488 ) ) ;
#17064=CARTESIAN_POINT ( 'NONE',  ( 200.0792105639032172, 267.3392562440996585, 6.292352169839691811 ) ) ;
#17066=CARTESIAN_POINT ( 'NONE',  ( 205.0054711740847608, 272.4066460739620084, -9.410916817109468369 ) ) ;
#17067=B_SPLINE_CURVE_WITH_KNOTS ( 'NONE', 3,
 ( #87487, #26613, #26115, #65106, #25094, #56992, #55977, #64104, #49905, #18520, #18023, #19033, #48916, #10922 ),
 .UNSPECIFIED., .F., .F.,
 ( 4, 2, 2, 2, 2, 2, 4 ),
 ( 0.001295899257826045765, 0.001512579950660447722, 0.001729260643494849679, 0.001945941336329251635, 0.002162622029163653592, 0.002595983414832457505, 0.003029344800501261419 ),
 .UNSPECIFIED. ) ;
#17068=CARTESIAN_POINT ( 'NONE',  ( 186.8071600733163393, 262.5868003515040527, -8.808218396323256982 ) ) ;
#17070=CARTESIAN_POINT ( 'NONE',  ( 73.95673202641080479, 225.0530062829863311, -4.648177544792955347E-16 ) ) ;
#17071=CARTESIAN_POINT ( 'NONE',  ( 200.0313018224816801, 276.5939864008022369, 15.71640468486303099 ) ) ;
#17073=CARTESIAN_POINT ( 'NONE',  ( 153.2712411579340426, 265.1734183057532732, 16.26687330118495467 ) ) ;
#17074=LINE ( 'NONE', #86543, #57597 ) ;
#17077=CARTESIAN_POINT ( 'NONE',  ( -3.667330603741788320, 162.5643266524160140, 9.188101187500095079 ) ) ;
#17078=CARTESIAN_POINT ( 'NONE',  ( 87.02133327910362937, 230.2369531367911009, -4.594050593750048428 ) ) ;
#17079=CARTESIAN_POINT ( 'NONE',  ( 203.4696564630250464, 278.2272125378923988, -16.38980782817167636 ) ) ;
#17081=DIRECTION ( 'NONE',  ( -0.8660254037844387076, -0.4999999999999998890, -0.000000000000000000 ) ) ;
#17083=CARTESIAN_POINT ( 'NONE',  ( 154.9903553346911735, 262.1958252075976361, -18.39016733948542637 ) ) ;
#17089=CARTESIAN_POINT ( 'NONE',  ( 162.0191462209216979, 250.0216022768697144, 13.77935367201302341 ) ) ;
#17090=CARTESIAN_POINT ( 'NONE',  ( -9.297732140679750401, 176.9860189848785410, -2.679491924311252493 ) ) ;
#17091=CARTESIAN_POINT ( 'NONE',  ( 164.7508860646548783, 245.2900900744633930, -5.203382148009804808 ) ) ;
#17092=CARTESIAN_POINT ( 'NONE',  ( 157.8763546842245376, 257.1971277035954699, 17.68444922773363004 ) ) ;
#17094=CARTESIAN_POINT ( 'NONE',  ( 47.23881193640350062, 188.8923013555410080, 4.594050593750050204 ) ) ;
#17095=CARTESIAN_POINT ( 'NONE',  ( 61.36533069198963375, 215.4244531367911293, -4.594050593750046652 ) ) ;
#17101=CARTESIAN_POINT ( 'NONE',  ( 184.8670040873090841, 279.3961096007919878, 17.75634087450649190 ) ) ;
#17102=DIRECTION ( 'NONE',  ( -0.8660254037844387076, -0.4999999999999998890, -0.000000000000000000 ) ) ;
#17103=CARTESIAN_POINT ( 'NONE',  ( 181.8129518053731033, 270.5384970965435514, -17.23398818032472946 ) ) ;
#17106=CARTESIAN_POINT ( 'NONE',  ( 150.7850480413316632, 269.4796311011364764, -14.43114374163211089 ) ) ;
#17107=CARTESIAN_POINT ( 'NONE',  ( 148.9194629746633893, 272.7109192224475009, -12.27648025871169679 ) ) ;
#17109=CARTESIAN_POINT ( 'NONE',  ( 69.24135662524314228, 198.5327760586659451, 1.948934522072302763E-15 ) ) ;
#17110=CARTESIAN_POINT ( 'NONE',  ( 97.16130770534415717, 220.2365022471902023, 10.00000000000009948 ) ) ;
#17111=CARTESIAN_POINT ( 'NONE',  ( 202.7754741559590173, 279.4295715634463022, -15.65855077192107636 ) ) ;
#17112=CARTESIAN_POINT ( 'NONE',  ( 198.6587626159274294, 286.5599251108861267, 17.99840276545888784 ) ) ;
#17113=DIRECTION ( 'NONE',  ( -0.4999999999999987788, 0.8660254037844392627, 0.000000000000000000 ) ) ;
#17114=CARTESIAN_POINT ( 'NONE',  ( 201.6407369932504992, 281.3949939824937019, 16.25974739329136298 ) ) ;
#17120=CARTESIAN_POINT ( 'NONE',  ( 117.4407359106297264, 248.6115022471903160, -5.000000000000047962 ) ) ;
#17122=CARTESIAN_POINT ( 'NONE',  ( 207.4764081617721843, 271.2873150223495600, 6.359972247200924578 ) ) ;
#17123=ORIENTED_EDGE ( 'NONE', *, *, #62303, .F. ) ;
#17125=CARTESIAN_POINT ( 'NONE',  ( 184.8398010511286316, 271.1657223325220798, 16.51723966498060037 ) ) ;
#17127=CARTESIAN_POINT ( 'NONE',  ( 159.2186641046529303, 254.8721795879351646, -15.96198087403305443 ) ) ;
#17132=VERTEX_POINT ( 'NONE', #53933 ) ;
#17134=CARTESIAN_POINT ( 'NONE',  ( 167.3947881066641514, 247.6242492910987778, 3.581681636340571018 ) ) ;
#17135=CARTESIAN_POINT ( 'NONE',  ( 148.4951514626549738, 273.8415162155406506, 8.072631028758147309 ) ) ;
#17136=ORIENTED_EDGE ( 'NONE', *, *, #24480, .F. ) ;
#17143=FACE_OUTER_BOUND ( 'NONE', #46675, .T. ) ;
#17146=CARTESIAN_POINT ( 'NONE',  ( 183.2164173712471040, 295.8027025434371922, 1.003979349283407707 ) ) ;
#17147=ADVANCED_FACE ( 'NONE', ( #92016 ), #52959, .T. ) ;
#17151=CARTESIAN_POINT ( 'NONE',  ( 193.8913555215501390, 294.8173164187117550, 15.40725395879721837 ) ) ;
#17152=CARTESIAN_POINT ( 'NONE',  ( 185.4383826630807448, 292.6325493778165310, -10.71708923905308986 ) ) ;
#17153=CARTESIAN_POINT ( 'NONE',  ( 157.7733463334721478, 257.3755434007023268, -16.94489513499352995 ) ) ;
#17154=CARTESIAN_POINT ( 'NONE',  ( 135.2211464324225858, 255.0024278399161517, -9.188101187500093303 ) ) ;
#17157=CARTESIAN_POINT ( 'NONE',  ( 88.48327179163739231, 212.7048013555409796, 4.594050593750051981 ) ) ;
#17159=CARTESIAN_POINT ( 'NONE',  ( 150.7530568467738590, 269.5350414755053521, 15.60317050893315916 ) ) ;
#17161=ORIENTED_EDGE ( 'NONE', *, *, #1452, .F. ) ;
#17162=CARTESIAN_POINT ( 'NONE',  ( 157.1602365732760802, 258.4374806559784474, -16.85676213245926292 ) ) ;
#17163=VERTEX_POINT ( 'NONE', #53446 ) ;
#17167=CARTESIAN_POINT ( 'NONE',  ( 191.0481192767711036, 299.7419460525905492, -9.103377665618040737 ) ) ;
#17168=CARTESIAN_POINT ( 'NONE',  ( 163.8402655714165519, 249.7793471524227868, 10.22989909625667693 ) ) ;
#17170=CARTESIAN_POINT ( 'NONE',  ( 162.5429104506708597, 249.1144160197565043, 10.44355587256373674 ) ) ;
#17171=CARTESIAN_POINT ( 'NONE',  ( 88.13136219740870558, 215.5643266524159571, -9.188101187500093303 ) ) ;
#17174=CARTESIAN_POINT ( 'NONE',  ( 208.3863431123642727, 269.7112614563416173, -1.693909372230378851 ) ) ;
#17178=CARTESIAN_POINT ( 'NONE',  ( 161.5852327833977142, 283.9684635997116970, 0.5249851707666771672 ) ) ;
#17184=CARTESIAN_POINT ( 'NONE',  ( 206.0870578475358172, 273.6937403561189512, -10.07771901274806581 ) ) ;
#17185=CARTESIAN_POINT ( 'NONE',  ( 155.7501102573973526, 262.3711424935290211, -17.08610291111812529 ) ) ;
#17186=CARTESIAN_POINT ( 'NONE',  ( 174.5965431966999120, 283.7287010187061469, 13.61117779920129323 ) ) ;
#17187=CARTESIAN_POINT ( 'NONE',  ( 198.9920886056412144, 285.3025922593915311, -17.15779807132265944 ) ) ;
#17188=EDGE_CURVE ( 'NONE', #66481, #85402, #88961, .T. ) ;
#17189=CARTESIAN_POINT ( 'NONE',  ( 141.4548986661878303, 259.1427522451419350, 10.00000000000009415 ) ) ;
#17191=CARTESIAN_POINT ( 'NONE',  ( -1.637757109730603178, 179.8615022471903444, 5.000000000000046185 ) ) ;
#17192=CARTESIAN_POINT ( 'NONE',  ( 200.2690241097007799, 283.7708703901988656, 16.96680019208369927 ) ) ;
#17194=CARTESIAN_POINT ( 'NONE',  ( 186.6676767428766937, 265.3792542468744386, -11.85556035995023905 ) ) ;
#17196=CARTESIAN_POINT ( 'NONE',  ( 174.9406376537963297, 290.1712607282375984, -6.365627776605657040 ) ) ;
#17197=ADVANCED_FACE ( 'NONE', ( #9357, #16449 ), #47348, .F. ) ;
#17198=CARTESIAN_POINT ( 'NONE',  ( 156.6677280378305284, 272.7060788182535020, 14.73662401990965876 ) ) ;
#17202=CARTESIAN_POINT ( 'NONE',  ( 179.9792551569844363, 266.4521290304439276, -14.77927586968167617 ) ) ;
#17204=CARTESIAN_POINT ( 'NONE',  ( 183.2562432415718092, 256.2013173691302086, 2.311692295278971798 ) ) ;
#17206=CARTESIAN_POINT ( 'NONE',  ( 181.8559320684326224, 273.7276056269956257, 17.73031764801637067 ) ) ;
#17207=CARTESIAN_POINT ( 'NONE',  ( 175.7622132985686392, 274.0430017844784629, -17.75579533532145504 ) ) ;
#17209=CARTESIAN_POINT ( 'NONE',  ( 195.0382653549689280, 265.8412794934087628, -7.320742485009862577 ) ) ;
#17210=CARTESIAN_POINT ( 'NONE',  ( -3.153561889951042474, 178.1744531367911577, 4.594050593750047540 ) ) ;
#17212=ORIENTED_EDGE ( 'NONE', *, *, #22528, .F. ) ;
#17213=CARTESIAN_POINT ( 'NONE',  ( 161.3981413584396876, 253.0972142504356270, -15.11937522241654719 ) ) ;
#17215=CARTESIAN_POINT ( 'NONE',  ( 203.7676226056132691, 275.1754274059050545, -12.67277803424182281 ) ) ;
#17217=CARTESIAN_POINT ( 'NONE',  ( 26.91401791951368949, 186.3458772461660544, 9.188101187500095079 ) ) ;
#17218=CARTESIAN_POINT ( 'NONE',  ( 66.77824978924009258, 209.3615022471902591, -10.00000000000009592 ) ) ;
#17220=CARTESIAN_POINT ( 'NONE',  ( 178.6803586118992939, 291.7013059717194210, 6.068282667768776228 ) ) ;
#17221=CARTESIAN_POINT ( 'NONE',  ( 191.8329718516215223, 298.3825415164982928, -8.871589506312979267 ) ) ;
#17222=CARTESIAN_POINT ( 'NONE',  ( 149.6891899025559383, 271.3777130753837241, 11.83206864037965289 ) ) ;
#17227=EDGE_CURVE ( 'NONE', #49678, #50293, #42920, .T. ) ;
#17228=EDGE_CURVE ( 'NONE', #54644, #46249, #29671, .T. ) ;
#17229=CARTESIAN_POINT ( 'NONE',  ( 73.27344031762343946, 203.1115022471901739, -5.000000000000041744 ) ) ;
#17231=CARTESIAN_POINT ( 'NONE',  ( 185.6221575045317138, 277.7868078161695280, -17.14424904577442277 ) ) ;
#17232=CARTESIAN_POINT ( 'NONE',  ( 149.9899443387552083, 245.8567911112850481, 0.000000000000000000 ) ) ;
#17234=CARTESIAN_POINT ( 'NONE',  ( 38.06444208900335013, 180.5327760586659451, 1.948934522072303157E-15 ) ) ;
#17235=CARTESIAN_POINT ( 'NONE',  ( 159.2876523829509665, 254.7526883847961017, 15.64395448151312351 ) ) ;
#17237=CARTESIAN_POINT ( 'NONE',  ( 203.1584666061235396, 270.1366466773015986, -6.432727867013968925 ) ) ;
#17239=DIRECTION ( 'NONE',  ( -0.8660254037844359321, -0.5000000000000051070, -0.000000000000000000 ) ) ;
#17242=CARTESIAN_POINT ( 'NONE',  ( -8.223158621222619757, 159.3927522451418213, 10.00000000000009948 ) ) ;
#17244=B_SPLINE_CURVE_WITH_KNOTS ( 'NONE', 3,
 ( #20241, #35919, #82582, #5037, #27830, #44508, #45508, #28316, #98751, #12649, #51115, #14128, #45010, #90171, #99236, #44002, #75438, #83061, #60197, #66820, #13145, #75955, #97748, #14628, #67830, #6532, #58706, #37407, #20744, #90679, #43518, #51630, #74944, #5528, #89680, #29331, #76440, #36412, #21723, #74457, #67316, #68313, #98244, #28832, #52114, #21235, #52607, #13634, #29822, #60696 ),
 .UNSPECIFIED., .F., .F.,
 ( 4, 2, 2, 2, 2, 2, 2, 2, 2, 2, 2, 2, 2, 2, 2, 2, 2, 2, 2, 2, 2, 2, 2, 2, 4 ),
 ( 0.0003547852092621711076, 0.001373122238808988701, 0.001882290753582355376, 0.002009582882275727511, 0.002136875010969099646, 0.002264167139662471781, 0.002391459268355844350, 0.002646043525742580813, 0.002900627783129316843, 0.003409796297902792806, 0.004428133327449595112, 0.005446470356996396985, 0.005955638871769835217, 0.006210223129156513568, 0.006464807386543191051, 0.006528453450889841990, 0.006592099515236493797, 0.006655745579583143869, 0.006719391643929794808, 0.006973975901316441933, 0.007483144416089663326, 0.007737728673476274022, 0.007992312930862884718, 0.008246897188249495414, 0.008501481445636106110 ),
 .UNSPECIFIED. ) ;
#17245=CARTESIAN_POINT ( 'NONE',  ( 201.6504829983214222, 272.7620465441235638, 12.67600476192259507 ) ) ;
#17247=CARTESIAN_POINT ( 'NONE',  ( 202.9093905060991005, 279.1976216410395182, 16.97070083370504179 ) ) ;
#17248=CARTESIAN_POINT ( 'NONE',  ( 196.9728329903666122, 289.4800408803428695, -17.53478045286815856 ) ) ;
#17250=CARTESIAN_POINT ( 'NONE',  ( 186.0548307059467277, 267.6833961656038241, -15.01235236491201164 ) ) ;
#17258=CARTESIAN_POINT ( 'NONE',  ( 183.6018926243820601, 279.6860137177432080, 17.64978500148036389 ) ) ;
#17259=CARTESIAN_POINT ( 'NONE',  ( 178.7278109544135134, 282.3134984357692474, 15.46213385585119404 ) ) ;
#17262=CARTESIAN_POINT ( 'NONE',  ( 177.5672598793707948, 256.2453929386242066, -7.265003576077156744 ) ) ;
#17263=CARTESIAN_POINT ( 'NONE',  ( 149.6676065383367416, 271.4150965588098074, 11.80358707172367261 ) ) ;
#17267=CARTESIAN_POINT ( 'NONE',  ( 189.5365842474118665, 274.1395708678550704, -15.66050912157280983 ) ) ;
#17270=CARTESIAN_POINT ( 'NONE',  ( 152.8328714238065515, 265.9326969577624027, -16.29536156676786263 ) ) ;
#17274=CARTESIAN_POINT ( 'NONE',  ( 157.6668627405778409, 257.5599783937680058, -16.78811156090270629 ) ) ;
#17275=CARTESIAN_POINT ( 'NONE',  ( 105.9391831106087096, 219.7202760586659167, -5.415160957724236172E-17 ) ) ;
#17277=VERTEX_POINT ( 'NONE', #91373 ) ;
#17279=CARTESIAN_POINT ( 'NONE',  ( 208.2555382576270233, 269.9378221106229034, 3.215405476967123199 ) ) ;
#17282=CARTESIAN_POINT ( 'NONE',  ( 198.0858447170796524, 287.5522480202560018, 18.44384186289807559 ) ) ;
#17284=CARTESIAN_POINT ( 'NONE',  ( 61.01376819352597636, 206.0333772461660544, 9.188101187500095079 ) ) ;
#17287=CARTESIAN_POINT ( 'NONE',  ( 197.9988809731023025, 287.7028736432410483, 18.08661327024293897 ) ) ;
#17288=CARTESIAN_POINT ( 'NONE',  ( 176.6106934046284493, 273.2656583511206918, 17.19257000985071215 ) ) ;
#17289=VECTOR ( 'NONE', #69219, 1000.000000000000000 ) ;
#17293=CARTESIAN_POINT ( 'NONE',  ( 177.3243750670959287, 288.8712866368100549, 11.28047403827316764 ) ) ;
#17296=CARTESIAN_POINT ( 'NONE',  ( 101.2828866085936852, 240.8297689869268936, -2.679491924311252493 ) ) ;
#17298=CARTESIAN_POINT ( 'NONE',  ( 207.3646600298985447, 271.4808684644054324, -5.284084612275558257 ) ) ;
#17299=CARTESIAN_POINT ( 'NONE',  ( 146.8153075009282134, 276.3554234099810287, -4.113808735271278216 ) ) ;
#17300=CARTESIAN_POINT ( 'NONE',  ( 149.6036070299368532, 271.5259469590175740, 11.63513718912356865 ) ) ;
#17301=B_SPLINE_CURVE_WITH_KNOTS ( 'NONE', 3,
 ( #31386, #62270, #3028, #64805 ),
 .UNSPECIFIED., .F., .F.,
 ( 4, 4 ),
 ( 0.03832837999546955671, 0.04687175281637306901 ),
 .UNSPECIFIED. ) ;
#17303=CARTESIAN_POINT ( 'NONE',  ( 180.7592890006537800, 271.2502507736807047, 17.08356462066134540 ) ) ;
#17306=CARTESIAN_POINT ( 'NONE',  ( 154.0654594722044521, 264.2254380362395523, -16.58972724529802889 ) ) ;
#17308=CARTESIAN_POINT ( 'NONE',  ( 111.6762543149156386, 235.2833772461660544, -9.188101187500095079 ) ) ;
#17309=ORIENTED_EDGE ( 'NONE', *, *, #18403, .T. ) ;
#17310=CARTESIAN_POINT ( 'NONE',  ( 191.5324528500417216, 298.9030556958743432, -8.286652526617016790 ) ) ;
#17312=CARTESIAN_POINT ( 'NONE',  ( 202.9881971861223917, 279.0611244672630278, -15.16231470264511927 ) ) ;
#17313=CARTESIAN_POINT ( 'NONE',  ( 192.5198628683430684, 296.3988585064753352, 11.83524212884658411 ) ) ;
#17315=CARTESIAN_POINT ( 'NONE',  ( 178.2401400375956939, 255.0819166014324821, 4.396970161736177829 ) ) ;
#17316=ORIENTED_EDGE ( 'NONE', *, *, #55165, .T. ) ;
#17318=CARTESIAN_POINT ( 'NONE',  ( 154.6982851380984130, 273.6571292083216349, -13.42362762759460892 ) ) ;
#17320=CARTESIAN_POINT ( 'NONE',  ( 206.6961830126489303, 272.6387046219738295, -10.22526498917591375 ) ) ;
#17321=CARTESIAN_POINT ( 'NONE',  ( 134.1932619090760568, 236.0327760586659736, 1.948934522072302763E-15 ) ) ;
#17322=CARTESIAN_POINT ( 'NONE',  ( 198.4522155198218059, 286.9176751754968109, -17.57438352224490075 ) ) ;
#17323=CARTESIAN_POINT ( 'NONE',  ( 190.2428527899854487, 298.9129196009670864, -8.201882143933323377 ) ) ;
#17324=CARTESIAN_POINT ( 'NONE',  ( 188.0035612729766115, 279.2325960380115362, 17.82077010991123700 ) ) ;
#17325=CARTESIAN_POINT ( 'NONE',  ( 47.96943409690536697, 192.3768266524160140, 9.188101187500098632 ) ) ;
#17329=CARTESIAN_POINT ( 'NONE',  ( 189.6134825805156368, 259.7924916801782160, -1.707211797017506472 ) ) ;
#17332=CARTESIAN_POINT ( 'NONE',  ( 171.1789833775259808, 259.9602249310370894, 14.90491122363313004 ) ) ;
#17333=CARTESIAN_POINT ( 'NONE',  ( 151.8566147802715705, 278.2686478900306497, -1.635913686782525911 ) ) ;
#17335=CARTESIAN_POINT ( 'NONE',  ( 155.6281496932864457, 261.0911329737299980, -18.07904265579665548 ) ) ;
#17336=CARTESIAN_POINT ( 'NONE',  ( 17.70578863690133886, 169.4824982072973967, 3.021315404115420679E-15 ) ) ;
#17338=CARTESIAN_POINT ( 'NONE',  ( 119.0104069514411123, 249.5177522451419065, 5.000000000000046185 ) ) ;
#17340=EDGE_LOOP ( 'NONE', ( #35689, #46157, #62714, #6021 ) ) ;
#17341=CARTESIAN_POINT ( 'NONE',  ( 147.6220714307702622, 274.9580672937808572, 8.392894244419288441 ) ) ;
#17343=CARTESIAN_POINT ( 'NONE',  ( 20.90579313287664576, 189.0024278399160949, -9.188101187500093303 ) ) ;
#17346=CARTESIAN_POINT ( 'NONE',  ( 80.11143256479013530, 210.3927522451418213, 10.00000000000009948 ) ) ;
#17347=CARTESIAN_POINT ( 'NONE',  ( 146.9324727656309335, 276.1524872186338371, 3.813717745456558728 ) ) ;
#17349=CARTESIAN_POINT ( 'NONE',  ( 152.8593402092683959, 275.2840601128194749, 10.96293945604634068 ) ) ;
#17350=CARTESIAN_POINT ( 'NONE',  ( 60.12067949409930634, 205.5177522451418497, -10.00000000000009592 ) ) ;
#17352=CARTESIAN_POINT ( 'NONE',  ( 163.2088130023161057, 256.0821108490627580, -14.95559493010926921 ) ) ;
#17356=EDGE_CURVE ( 'NONE', #56036, #56410, #65909, .T. ) ;
#17357=CARTESIAN_POINT ( 'NONE',  ( 19.94070920123167312, 188.9865022471903160, -10.00000000000009415 ) ) ;
#17358=CARTESIAN_POINT ( 'NONE',  ( 32.27148724097330756, 200.9860189848785410, -2.679491924311252493 ) ) ;
#17360=CARTESIAN_POINT ( 'NONE',  ( 202.8211298556536804, 279.3504935719197988, 17.07914446815911447 ) ) ;
#17361=CARTESIAN_POINT ( 'NONE',  ( -5.047471817081990331, 158.7048013555409796, 4.594050593750051981 ) ) ;
#17363=CARTESIAN_POINT ( 'NONE',  ( 164.1994273494235301, 252.5555082259370181, 13.35012251226196867 ) ) ;
#17364=CARTESIAN_POINT ( 'NONE',  ( 199.9134407114337364, 283.6250491837689651, 17.05367660732407842 ) ) ;
#17366=CARTESIAN_POINT ( 'NONE',  ( 22.11123320312891849, 195.1199935810940929, 2.679491924311251605 ) ) ;
#17368=B_SPLINE_CURVE_WITH_KNOTS ( 'NONE', 3,
 ( #45934, #53547, #61142, #53055 ),
 .UNSPECIFIED., .F., .F.,
 ( 4, 4 ),
 ( 2.602085213965210642E-18, 0.003217767275339507987 ),
 .UNSPECIFIED. ) ;
#17369=CARTESIAN_POINT ( 'NONE',  ( 164.4261001824251878, 245.8526357240660900, 1.583002802772015549 ) ) ;
#17370=CARTESIAN_POINT ( 'NONE',  ( 183.2458657411818308, 257.8356223092092705, -2.282625027615983182 ) ) ;
#17373=CARTESIAN_POINT ( 'NONE',  ( 196.9098758191317700, 289.5890858996224324, -16.54412079817003800 ) ) ;
#17374=CARTESIAN_POINT ( 'NONE',  ( 177.9925615710933755, 254.8251403409008731, -7.350624415798725053 ) ) ;
#17376=CARTESIAN_POINT ( 'NONE',  ( 153.2873167144811646, 277.6669624900651456, -5.602515137802061673 ) ) ;
#17378=CARTESIAN_POINT ( 'NONE',  ( 160.5729363862711523, 252.5265111888899696, 15.95386353709229965 ) ) ;
#17380=EDGE_LOOP ( 'NONE', ( #7564, #23813, #29276, #53758 ) ) ;
#17381=CARTESIAN_POINT ( 'NONE',  ( 192.4202172926039793, 297.3654025762033370, 10.98569444949570872 ) ) ;
#17382=CARTESIAN_POINT ( 'NONE',  ( 207.3502731283117555, 271.5057873089173768, 6.280625384230454245 ) ) ;
#17383=CARTESIAN_POINT ( 'NONE',  ( 190.9015239950540206, 298.2326252366660810, 9.554377282061516041 ) ) ;
#17385=CARTESIAN_POINT ( 'NONE',  ( 193.9204722154232741, 294.7668848255750049, 15.43855698596013859 ) ) ;
#17386=EDGE_LOOP ( 'NONE', ( #98495, #43804, #90688, #95184, #41189, #37176, #96293, #24532, #79479, #96522, #22625, #15144, #46163, #28980, #68972, #44801, #59095, #13705, #68474, #1063 ) ) ;
#17390=ORIENTED_EDGE ( 'NONE', *, *, #14602, .T. ) ;
#17392=CARTESIAN_POINT ( 'NONE',  ( 188.5527807511783180, 297.9505215649899696, 7.797827009507764195 ) ) ;
#17399=CARTESIAN_POINT ( 'NONE',  ( 173.7019467158212933, 267.2044448140225086, 16.95278284378356659 ) ) ;
#17400=CARTESIAN_POINT ( 'NONE',  ( 180.3089020998223475, 294.4768193211729681, -5.541584815692371713 ) ) ;
#17402=CARTESIAN_POINT ( 'NONE',  ( 127.4956995296957416, 255.9637435831425023, 2.679491924311251605 ) ) ;
#17403=CARTESIAN_POINT ( 'NONE',  ( 191.5766842709549280, 298.8264446275616137, 8.039910086100929831 ) ) ;
#17404=CARTESIAN_POINT ( 'NONE',  ( 151.4143897794357088, 274.9824025847329949, -8.616620037206830673 ) ) ;
#17406=CARTESIAN_POINT ( 'NONE',  ( 170.7449765318682466, 255.6388512455198736, -11.59872511109924709 ) ) ;
#17408=VERTEX_POINT ( 'NONE', #16334 ) ;
#17415=CARTESIAN_POINT ( 'NONE',  ( 167.3899042128373651, 272.0936304241042194, 16.05079403648893788 ) ) ;
#17417=CARTESIAN_POINT ( 'NONE',  ( 147.8819534105757043, 274.5079385007862811, -9.338341377131436971 ) ) ;
#17425=CARTESIAN_POINT ( 'NONE',  ( 164.2801755739368446, 246.1053845600426087, 2.518777461081745717 ) ) ;
#17426=CARTESIAN_POINT ( 'NONE',  ( 205.7576124508049418, 274.2643565215761328, 10.88614016733041545 ) ) ;
#17427=CARTESIAN_POINT ( 'NONE',  ( 196.4628211408765139, 276.9783169463397030, -16.67918425853740771 ) ) ;
#17431=CARTESIAN_POINT ( 'NONE',  ( 190.6843051365801784, 300.3720906279131100, 5.205712306949425106 ) ) ;
#17433=CARTESIAN_POINT ( 'NONE',  ( 206.7893622945242385, 272.4773133715531230, -10.52881283832460291 ) ) ;
#17436=CARTESIAN_POINT ( 'NONE',  ( 161.3193951073452581, 251.2336067582368742, 13.01220207292984377 ) ) ;
#17437=CARTESIAN_POINT ( 'NONE',  ( 190.8369279865719932, 261.8867820640782043, -0.3648464445779296406 ) ) ;
#17438=ORIENTED_EDGE ( 'NONE', *, *, #63482, .T. ) ;
#17439=CARTESIAN_POINT ( 'NONE',  ( 167.2609760701786570, 252.9900861492237425, -12.15359341202019117 ) ) ;
#17445=CARTESIAN_POINT ( 'NONE',  ( 23.67544375150423619, 171.1427522451417644, 1.119607411625061291E-15 ) ) ;
#17446=CARTESIAN_POINT ( 'NONE',  ( 95.22211873877631660, 213.5327760586659451, 1.948934522072302763E-15 ) ) ;
#17449=CARTESIAN_POINT ( 'NONE',  ( 169.8363984463651377, 280.1429775057247298, -13.61031055851517557 ) ) ;
#17450=CARTESIAN_POINT ( 'NONE',  ( 5.777845730223497789, 164.9548013555410080, -4.594050593750042211 ) ) ;
#17452=CARTESIAN_POINT ( 'NONE',  ( 161.2799361541916028, 251.3019516699124836, 14.40628917569557110 ) ) ;
#17455=CARTESIAN_POINT ( 'NONE',  ( 200.2433557449332682, 267.4156030511788344, -2.849737501924599403 ) ) ;
#17458=CARTESIAN_POINT ( 'NONE',  ( 40.86965645935567437, 187.7365022471901739, -10.00000000000009237 ) ) ;
#17461=CARTESIAN_POINT ( 'NONE',  ( 28.53781555160951555, 187.2833772461660544, -9.188101187500095079 ) ) ;
#17462=CARTESIAN_POINT ( 'NONE',  ( 81.77131458871032521, 208.0177522451417929, 5.000000000000051514 ) ) ;
#17467=DIRECTION ( 'NONE',  ( 0.8660254037844303809, 0.5000000000000144329, 0.000000000000000000 ) ) ;
#17469=CARTESIAN_POINT ( 'NONE',  ( -4.722712290662820500, 158.8923013555410080, 4.594050593750050204 ) ) ;
#17472=CARTESIAN_POINT ( 'NONE',  ( 207.1211793645798878, 271.9025893473983047, -6.294110402770905388 ) ) ;
#17474=CARTESIAN_POINT ( 'NONE',  ( 194.3708539535661259, 293.9868007723104029, -16.01585187499628304 ) ) ;
#17476=DIRECTION ( 'NONE',  ( -0.4999999999999987788, 0.8660254037844392627, 0.000000000000000000 ) ) ;
#17477=CARTESIAN_POINT ( 'NONE',  ( 164.2059258710715994, 246.2339888178522926, 7.329631442356459914 ) ) ;
#17478=CARTESIAN_POINT ( 'NONE',  ( 191.0478321355427624, 299.7424433957868928, -9.006798842970001218 ) ) ;
#17479=CARTESIAN_POINT ( 'NONE',  ( 148.0427192501136062, 274.2294838985851015, 9.385226820296049155 ) ) ;
#17482=CARTESIAN_POINT ( 'NONE',  ( 208.1757572214753793, 270.0760069187178374, 2.172546422564154867 ) ) ;
#17483=CARTESIAN_POINT ( 'NONE',  ( 110.3772162092389948, 234.5333772461660828, 9.188101187500095079 ) ) ;
#17489=CARTESIAN_POINT ( 'NONE',  ( 157.0957870390718369, 258.5491105237443321, 17.69218919045495397 ) ) ;
#17490=CARTESIAN_POINT ( 'NONE',  ( 200.1133476818314705, 272.1141633677412415, 12.87458617912082914 ) ) ;
#17491=CARTESIAN_POINT ( 'NONE',  ( 204.5028199768381398, 272.8749048982307954, -9.750091098900030673 ) ) ;
#17492=B_SPLINE_CURVE_WITH_KNOTS ( 'NONE', 3,
 ( #99386, #55242, #15751, #30958 ),
 .UNSPECIFIED., .F., .F.,
 ( 4, 4 ),
 ( 0.008069797487559298571, 0.01626517688446255105 ),
 .UNSPECIFIED. ) ;
#17493=CARTESIAN_POINT ( 'NONE',  ( -22.42236680055709641, 157.8615022471902591, 0.000000000000000000 ) ) ;
#17494=CARTESIAN_POINT ( 'NONE',  ( 196.2293283710122012, 290.7678286567270902, -17.07152402978540096 ) ) ;
#17496=CARTESIAN_POINT ( 'NONE',  ( 172.6105268277075311, 290.6563111985113892, -1.849890294009189251 ) ) ;
#17501=CARTESIAN_POINT ( 'NONE',  ( 189.5599828453989346, 263.0657735508838186, -9.804501003715218488 ) ) ;
#17502=ORIENTED_EDGE ( 'NONE', *, *, #26815, .F. ) ;
#17506=CARTESIAN_POINT ( 'NONE',  ( 152.7314557461996571, 266.1083540640618708, 17.39314074348802208 ) ) ;
#17509=CARTESIAN_POINT ( 'NONE',  ( 163.2523617031003482, 269.8851863420952668, -17.32811968646028689 ) ) ;
#17511=CARTESIAN_POINT ( 'NONE',  ( 195.3339445956660256, 290.3114242235789675, -16.63067108908084535 ) ) ;
#17513=CARTESIAN_POINT ( 'NONE',  ( 163.7954642885384544, 279.4399783988836248, 12.25154076785413082 ) ) ;
#17515=CARTESIAN_POINT ( 'NONE',  ( 20.87890338866488804, 172.8615022471901739, 5.000000000000051514 ) ) ;
#17518=CARTESIAN_POINT ( 'NONE',  ( 188.7491163893556347, 293.7278928144251040, 12.91049369769965516 ) ) ;
#17522=CARTESIAN_POINT ( 'NONE',  ( 155.0304386007204016, 262.1263989543018056, -17.12961552904782181 ) ) ;
#17523=ORIENTED_EDGE ( 'NONE', *, *, #63482, .F. ) ;
#17524=VERTEX_POINT ( 'NONE', #1145 ) ;
#17531=ORIENTED_EDGE ( 'NONE', *, *, #20706, .T. ) ;
#17533=CARTESIAN_POINT ( 'NONE',  ( 206.7127649687076314, 272.6099838315917623, -10.35326570309970506 ) ) ;
#17534=CARTESIAN_POINT ( 'NONE',  ( 190.5255224008060395, 300.6471103936386271, 2.040674304113719639 ) ) ;
#17536=CARTESIAN_POINT ( 'NONE',  ( 192.4172326059820648, 297.3705722050773943, -12.52563289807247848 ) ) ;
#17538=CARTESIAN_POINT ( 'NONE',  ( 201.1755594471486859, 282.2007051268825535, -18.15567516623250910 ) ) ;
#17541=CARTESIAN_POINT ( 'NONE',  ( 157.8706589075648310, 280.9451892264036132, 2.094144116980718451 ) ) ;
#17542=CARTESIAN_POINT ( 'NONE',  ( 123.8274129399422918, 251.4869531367911577, 4.594050593750046652 ) ) ;
#17550=ORIENTED_EDGE ( 'NONE', *, *, #781, .F. ) ;
#17551=CARTESIAN_POINT ( 'NONE',  ( 203.6078461682101590, 276.3159402255348027, 13.42158206181595048 ) ) ;
#17552=CARTESIAN_POINT ( 'NONE',  ( 177.8946713442994678, 253.3491511510508190, 1.398846671321700486 ) ) ;
#17554=CARTESIAN_POINT ( 'NONE',  ( 172.6012549852709412, 290.2025030293380610, -5.021894074213228087 ) ) ;
#17555=CARTESIAN_POINT ( 'NONE',  ( 192.8302070313391141, 296.6552795181322608, 12.00067902349765880 ) ) ;
#17558=CARTESIAN_POINT ( 'NONE',  ( 176.7740879285838389, 288.5420746471101552, -9.314761950507488564 ) ) ;
#17559=CARTESIAN_POINT ( 'NONE',  ( 193.4225248517565774, 292.8543354191958201, -14.39945119728164435 ) ) ;
#17560=CARTESIAN_POINT ( 'NONE',  ( 177.2273226362962362, 256.0984073744629086, -7.379249422943265024 ) ) ;
#17561=ORIENTED_EDGE ( 'NONE', *, *, #56103, .T. ) ;
#17562=CARTESIAN_POINT ( 'NONE',  ( 148.0346525705264469, 274.2434557974783615, -9.381294579651672905 ) ) ;
#17565=CARTESIAN_POINT ( 'NONE',  ( 163.0656072001963537, 277.9852329471388543, 13.74753899820123415 ) ) ;
#17568=CARTESIAN_POINT ( 'NONE',  ( 192.1435947104413913, 297.8445269430296776, -9.754524473716664090 ) ) ;
#17569=CARTESIAN_POINT ( 'NONE',  ( 148.9230895364621574, 272.7046378331555161, 12.20434325797056019 ) ) ;
#17570=CARTESIAN_POINT ( 'NONE',  ( 162.6626107288841467, 248.9070890562113902, 10.12509462564867313 ) ) ;
#17571=CARTESIAN_POINT ( 'NONE',  ( 153.4735438756679002, 270.0204785379407326, 14.29634556544180235 ) ) ;
#17572=CARTESIAN_POINT ( 'NONE',  ( 160.5520610138454458, 282.2019950894995759, 6.659617355605994327 ) ) ;
#17573=CARTESIAN_POINT ( 'NONE',  ( 152.7729059155601021, 266.0365602647466972, -17.50667083025758686 ) ) ;
#17575=CARTESIAN_POINT ( 'NONE',  ( 163.1033070407499110, 249.6811796723388852, -11.57508889205896274 ) ) ;
#17576=PRODUCT_DEFINITION_SHAPE ( 'NONE', 'NONE',  #3701 ) ;
#17577=CARTESIAN_POINT ( 'NONE',  ( 186.9555558246591431, 262.3224090832389379, -8.686013347077395252 ) ) ;
#17578=DIRECTION ( 'NONE',  ( 0.5000000000000048850, -0.8660254037844358210, 0.000000000000000000 ) ) ;
#17579=CARTESIAN_POINT ( 'NONE',  ( -22.42236680055709641, 157.8615022471902591, 0.000000000000000000 ) ) ;
#17580=EDGE_CURVE ( 'NONE', #68024, #20256, #37022, .T. ) ;
#17581=CARTESIAN_POINT ( 'NONE',  ( 184.6438136528588529, 297.2564992327004916, -4.482047658127568113 ) ) ;
#17582=EDGE_CURVE ( 'NONE', #1108, #53329, #84083, .T. ) ;
#17583=CARTESIAN_POINT ( 'NONE',  ( 201.1893450866852504, 280.1768276987904756, -16.82388990131531870 ) ) ;
#17585=CARTESIAN_POINT ( 'NONE',  ( -11.23620533500811725, 170.9865022471903444, -10.00000000000009592 ) ) ;
#17587=CARTESIAN_POINT ( 'NONE',  ( -6.265406815095104776, 161.0643266524159856, 9.188101187500095079 ) ) ;
#17588=CARTESIAN_POINT ( 'NONE',  ( 88.48327179163739231, 212.7048013555409796, 4.594050593750051981 ) ) ;
#17589=CARTESIAN_POINT ( 'NONE',  ( 26.05470188313195123, 197.3967562850347122, -4.648177544792955347E-16 ) ) ;
#17591=CARTESIAN_POINT ( 'NONE',  ( 182.8190671368951428, 294.1949347170434521, -7.963347553794334566 ) ) ;
#17592=CARTESIAN_POINT ( 'NONE',  ( -12.03006195514386434, 173.8615022471903160, 5.000000000000046185 ) ) ;
#17597=CARTESIAN_POINT ( 'NONE',  ( 161.9469964850341626, 250.1465692851796518, 14.00188699914706092 ) ) ;
#17598=EDGE_CURVE ( 'NONE', #97734, #29236, #1873, .T. ) ;
#17599=CARTESIAN_POINT ( 'NONE',  ( 169.2574381869089564, 252.1335231699163160, -8.836137456772515719 ) ) ;
#17600=CARTESIAN_POINT ( 'NONE',  ( 164.3378896953848596, 246.0054207693806063, -5.823270600575261469 ) ) ;
#17606=CARTESIAN_POINT ( 'NONE',  ( 30.18841615574984516, 197.4244531367911293, -4.594050593750046652 ) ) ;
#17607=CARTESIAN_POINT ( 'NONE',  ( 175.1616093908759240, 264.7739651183366618, -16.67648531822408486 ) ) ;
#17609=CARTESIAN_POINT ( 'NONE',  ( 64.39641960523518094, 217.1744531367911293, 4.594050593750047540 ) ) ;
#17610=CARTESIAN_POINT ( 'NONE',  ( 164.5641499066685469, 246.8022252770303169, -5.664862832761055955 ) ) ;
#17612=AXIS2_PLACEMENT_3D ( 'NONE', #87460, #26085, #10387 ) ;
#17613=EDGE_CURVE ( 'NONE', #92966, #56021, #61048, .T. ) ;
#17614=CARTESIAN_POINT ( 'NONE',  ( 166.2779816807986322, 259.4367366842961360, 15.68628669229216932 ) ) ;
#17616=CYLINDRICAL_SURFACE ( 'NONE', #15037, 17.82106496071139645 ) ;
#17618=CARTESIAN_POINT ( 'NONE',  ( 176.5628964405708530, 270.0282015820967558, -17.29816915654511078 ) ) ;
#17619=EDGE_CURVE ( 'NONE', #92966, #61965, #19991, .T. ) ;
#17622=CARTESIAN_POINT ( 'NONE',  ( 148.9322735291567597, 272.6887306911919495, -12.40988026045598858 ) ) ;
#17625=CARTESIAN_POINT ( 'NONE',  ( 71.43287601098374751, 221.2369531367911293, -4.594050593750048428 ) ) ;
#17627=AXIS2_PLACEMENT_3D ( 'NONE', #51528, #28225, #92074 ) ;
#17628=CARTESIAN_POINT ( 'NONE',  ( 172.6035724952978967, 290.6552710437545670, -0.3907579110097771369 ) ) ;
#17630=CARTESIAN_POINT ( 'NONE',  ( 154.0650720908321034, 263.7984627973538068, 16.93260884073979966 ) ) ;
#17631=EDGE_CURVE ( 'NONE', #54122, #49104, #18939, .T. ) ;
#17633=CARTESIAN_POINT ( 'NONE',  ( 168.2820353728258738, 287.7095463320123940, -5.019694092131335772 ) ) ;
#17636=CARTESIAN_POINT ( 'NONE',  ( 126.4618338667177113, 230.4865022471901170, 1.119607411625061291E-15 ) ) ;
#17637=( BOUNDED_CURVE ( )  B_SPLINE_CURVE ( 2, ( #44872, #90033, #97622, #59062, #29689, #52479, #6396, #74326, #36782 ),
 .UNSPECIFIED., .F., .T. ) 
 B_SPLINE_CURVE_WITH_KNOTS ( ( 3, 2, 2, 2, 3 ),
 ( 0.4556451612903225645, 0.4569892473118279397, 0.4596774193548386900, 0.4623655913978494403, 0.4637096774193548154 ),
 .UNSPECIFIED. ) 
 CURVE ( )  GEOMETRIC_REPRESENTATION_ITEM ( )  RATIONAL_B_SPLINE_CURVE ( ( 0.9330127018922194093, 0.9330127018922194093, 1.000000000000000000, 0.8660254037844387076, 1.000000000000000000, 0.8660254037844387076, 1.000000000000000000, 0.9330127018922194093, 0.9330127018922194093 ) ) 
 REPRESENTATION_ITEM ( '' )  );
#17638=CARTESIAN_POINT ( 'NONE',  ( 15.95338390109293059, 180.0177522451418497, -10.00000000000009592 ) ) ;
#17643=CARTESIAN_POINT ( 'NONE',  ( 202.3425522658138505, 280.1794142728863903, 15.86053073629060961 ) ) ;
#17644=CARTESIAN_POINT ( 'NONE',  ( -22.42236680055709641, 157.8615022471902591, 0.000000000000000000 ) ) ;
#17645=CYLINDRICAL_SURFACE ( 'NONE', #59607, 17.82106496071139645 ) ;
#17647=CARTESIAN_POINT ( 'NONE',  ( 175.9795468396543185, 253.0532177342393254, -0.2546238855235851140 ) ) ;
#17650=CARTESIAN_POINT ( 'NONE',  ( 170.6815359018025333, 250.4067295894952281, 3.251190589082308513 ) ) ;
#17651=CARTESIAN_POINT ( 'NONE',  ( 148.5271690325042186, 274.6709829484061061, 7.673052289842670071 ) ) ;
#17658=CARTESIAN_POINT ( 'NONE',  ( 167.9209307024295583, 276.8122465436554762, 15.57331525377104775 ) ) ;
#17662=CARTESIAN_POINT ( 'NONE',  ( 183.3830520126487329, 295.9076832148600147, 1.011780174870672511 ) ) ;
#17664=CARTESIAN_POINT ( 'NONE',  ( 147.9500839974939197, 274.3899328626944225, -9.375093207164509224 ) ) ;
#17666=CARTESIAN_POINT ( 'NONE',  ( 193.9204722154232741, 294.7668848255750049, 15.43855698596013859 ) ) ;
#17668=CARTESIAN_POINT ( 'NONE',  ( 205.4103625296683617, 274.8658110279089897, -13.38953657917851814 ) ) ;
#17669=CARTESIAN_POINT ( 'NONE',  ( 208.0418200135015923, 270.3079929679526572, -4.942760474469149123 ) ) ;
#17670=CARTESIAN_POINT ( 'NONE',  ( 206.4325537506903459, 270.6027761474677504, 2.448701755339154129 ) ) ;
#17672=CARTESIAN_POINT ( 'NONE',  ( 77.06204113558260360, 224.4869531367911293, 4.594050593750046652 ) ) ;
#17674=CARTESIAN_POINT ( 'NONE',  ( 151.4384131719918685, 268.3479694989391078, 14.98299707687648841 ) ) ;
#17677=CARTESIAN_POINT ( 'NONE',  ( 195.4464213238641150, 292.1238634399910552, -17.06481037329052342 ) ) ;
#17682=CARTESIAN_POINT ( 'NONE',  ( 191.5893301551938350, 298.8045413135534432, -8.323356515452589477 ) ) ;
#17685=CARTESIAN_POINT ( 'NONE',  ( 208.0366075493969902, 270.3170212206142082, 1.570844709476715284 ) ) ;
#17686=CARTESIAN_POINT ( 'NONE',  ( 99.63334886536203783, 219.1423013555409796, -4.594050593750043987 ) ) ;
#17689=CARTESIAN_POINT ( 'NONE',  ( 162.7459776558209228, 248.7626933030860812, -9.895605163646791880 ) ) ;
#17690=ORIENTED_EDGE ( 'NONE', *, *, #21120, .F. ) ;
#17696=CARTESIAN_POINT ( 'NONE',  ( -16.08955603893133812, 171.5177522451419350, 5.000000000000046185 ) ) ;
#17700=CARTESIAN_POINT ( 'NONE',  ( 204.4329329219251861, 276.5587687693421799, 13.28840463846547948 ) ) ;
#17702=CARTESIAN_POINT ( 'NONE',  ( 159.8188415394622268, 253.8326417772889840, -15.43862849427313222 ) ) ;
#17705=EDGE_CURVE ( 'NONE', #78457, #47416, #40608, .T. ) ;
#17708=CARTESIAN_POINT ( 'NONE',  ( -22.42236680055709641, 157.8615022471902591, 0.000000000000000000 ) ) ;
#17712=CARTESIAN_POINT ( 'NONE',  ( 161.6707029936031574, 250.6251236501384483, 14.45053103226186231 ) ) ;
#17714=CARTESIAN_POINT ( 'NONE',  ( 170.4700060268252457, 251.4149474771376731, 7.010157526727356370 ) ) ;
#17716=CARTESIAN_POINT ( 'NONE',  ( 200.9741374040782489, 267.1036203943184546, 5.055124302673880798 ) ) ;
#17719=VECTOR ( 'NONE', #89921, 1000.000000000000000 ) ;
#17720=B_SPLINE_CURVE_WITH_KNOTS ( 'NONE', 3,
 ( #85485, #22644, #29744, #45428, #46417, #31226, #84970, #14553, #92578, #24138, #61122, #77852 ),
 .UNSPECIFIED., .F., .F.,
 ( 4, 2, 2, 2, 2, 4 ),
 ( 0.000000000000000000, 0.0004691669264628405001, 0.0009383338529256810001, 0.001407500779388521717, 0.001642084242619940015, 0.001876667705851358314 ),
 .UNSPECIFIED. ) ;
#17721=CARTESIAN_POINT ( 'NONE',  ( 164.2672861321391053, 246.1277097281173667, -2.417001679502223777 ) ) ;
#17723=CARTESIAN_POINT ( 'NONE',  ( 199.2695128734261516, 281.5989303855700996, -16.59789331015314318 ) ) ;
#17724=B_SPLINE_CURVE_WITH_KNOTS ( 'NONE', 3,
 ( #21587, #23050, #51986, #45846, #74812, #76298, #30678, #92027, #76768, #52470, #5883, #7362, #60553, #61558, #92505, #13985, #82924, #82447, #29680, #13011, #43870, #5392, #44371, #67175, #83417, #98099, #75302, #75802, #36770, #98610, #29192, #99094, #70663, #16464, #79323, #47846, #78785, #40250, #86937, #33170, #55443, #71190, #15446, #7880, #94009, #9371, #16955, #46346, #69661, #63565, #54439, #64072 ),
 .UNSPECIFIED., .F., .F.,
 ( 4, 2, 2, 2, 2, 2, 2, 2, 2, 2, 2, 2, 2, 2, 2, 2, 2, 2, 2, 2, 2, 2, 2, 2, 2, 4 ),
 ( 9.939757338935888544E-05, 0.001109022545050053358, 0.001361428787965241480, 0.001613835030880429603, 0.001740038152338023447, 0.001866241273795617509, 0.001992444395253211570, 0.002118647516710805197, 0.002371053759626150313, 0.002623460002541494994, 0.003128272488372348288, 0.004137897460034054876, 0.005147522431695762332, 0.005652334917526606953, 0.005904741160442065692, 0.006030944281899838430, 0.006157147403357612035, 0.006220248964086553915, 0.006283350524815494928, 0.006409553646273225165, 0.006661959889188582423, 0.006914366132103938814, 0.007166772375019295205, 0.007419178617934651596, 0.007671584860850008854, 0.008176397346680856076 ),
 .UNSPECIFIED. ) ;
#17726=CARTESIAN_POINT ( 'NONE',  ( 192.1640094933931096, 297.8091675017319062, 12.36911124822534447 ) ) ;
#17727=CARTESIAN_POINT ( 'NONE',  ( 170.9335546628262534, 274.1512530509741055, 16.08033032509779758 ) ) ;
#17729=CARTESIAN_POINT ( 'NONE',  ( 161.0344790431144304, 273.4108582822469771, -15.37894900309793655 ) ) ;
#17730=CARTESIAN_POINT ( 'NONE',  ( 188.6052575583571524, 261.0271860406964493, 2.867474821217330661 ) ) ;
#17731=CARTESIAN_POINT ( 'NONE',  ( 161.8668411317136986, 250.2854024296290447, -13.43522912998426655 ) ) ;
#17733=CARTESIAN_POINT ( 'NONE',  ( 5.155129649429669669, 173.7833772461660828, -9.188101187500095079 ) ) ;
#17735=ORIENTED_EDGE ( 'NONE', *, *, #56543, .F. ) ;
#17736=CARTESIAN_POINT ( 'NONE',  ( 160.1510049008126089, 253.7907123372172862, -14.98674719755693729 ) ) ;
#17739=CARTESIAN_POINT ( 'NONE',  ( 204.6350011963004647, 275.7068757420208271, -12.64342396695018245 ) ) ;
#17741=CARTESIAN_POINT ( 'NONE',  ( 13.65283037618196893, 184.8149278399161233, 9.188101187500093303 ) ) ;
#17742=CARTESIAN_POINT ( 'NONE',  ( 161.4726291907278721, 250.9681975403669867, 14.52346149734912117 ) ) ;
#17745=CARTESIAN_POINT ( 'NONE',  ( 181.7908406276906703, 294.3191638571922226, 6.361577546909467529 ) ) ;
#17746=CARTESIAN_POINT ( 'NONE',  ( 173.5944101645363844, 272.6791245995305530, -16.35745397706937609 ) ) ;
#17747=CARTESIAN_POINT ( 'NONE',  ( 149.6461826035522904, 271.4522039023545972, 11.73164196682384386 ) ) ;
#17750=EDGE_CURVE ( 'NONE', #40534, #5726, #30920, .T. ) ;
#17751=CARTESIAN_POINT ( 'NONE',  ( 190.0398248856338057, 298.8169614316505545, -8.166243001185458539 ) ) ;
#17753=CARTESIAN_POINT ( 'NONE',  ( 84.09875786492884231, 229.3615022471903160, 5.000000000000046185 ) ) ;
#17755=CARTESIAN_POINT ( 'NONE',  ( 203.7311721596700238, 270.2501766899930544, 6.028001199396760157 ) ) ;
#17756=CARTESIAN_POINT ( 'NONE',  ( 40.68897417663616523, 203.4869531367911293, 4.594050593750046652 ) ) ;
#17757=CARTESIAN_POINT ( 'NONE',  ( 194.3094773688834778, 284.8302703302293253, 17.74979085435418469 ) ) ;
#17760=CARTESIAN_POINT ( 'NONE',  ( 146.8358616138309571, 276.3198226421291679, 4.054088818585255716 ) ) ;
#17764=CARTESIAN_POINT ( 'NONE',  ( 89.19923881209058436, 210.7592609112379876, 2.679491924311254714 ) ) ;
#17766=DIRECTION ( 'NONE',  ( -0.8660254037844387076, -0.4999999999999998890, -0.000000000000000000 ) ) ;
#17767=CARTESIAN_POINT ( 'NONE',  ( 206.6679807590241467, 270.3735744487264583, -1.305484171715150854 ) ) ;
#17769=CARTESIAN_POINT ( 'NONE',  ( 202.6560281492536717, 279.6364581158209717, 17.15553667345918853 ) ) ;
#17770=CARTESIAN_POINT ( 'NONE',  ( 149.7200635338602410, 271.3242383773507527, -12.12223662813266500 ) ) ;
#17771=CARTESIAN_POINT ( 'NONE',  ( 157.4627203480516755, 258.4629190429250798, 16.86169483958236626 ) ) ;
#17772=ORIENTED_EDGE ( 'NONE', *, *, #21270, .T. ) ;
#17774=B_SPLINE_CURVE_WITH_KNOTS ( 'NONE', 3,
 ( #80751, #96939, #35587, #20908, #12303, #66972, #57883, #51795, #66482, #74103, #51270, #19427, #42667, #27505, #5189, #73600 ),
 .UNSPECIFIED., .F., .F.,
 ( 4, 2, 2, 2, 2, 2, 2, 4 ),
 ( 0.000000000000000000, 0.0003044019995352871002, 0.0006088039990705742003, 0.0009132059986058614631, 0.001217607998141148401, 0.001522009997676435555, 0.001826411997211722926, 0.002435215996282302873 ),
 .UNSPECIFIED. ) ;
#17778=CARTESIAN_POINT ( 'NONE',  ( 179.6077830788075005, 283.1794306977752171, 16.12751113146045867 ) ) ;
#17779=CARTESIAN_POINT ( 'NONE',  ( 150.6431064791187850, 269.7254810985950257, 15.11064854015152470 ) ) ;
#17780=CARTESIAN_POINT ( 'NONE',  ( 182.1439385020048860, 290.0253507885926183, 13.01467259685074573 ) ) ;
#17783=AXIS2_PLACEMENT_3D ( 'NONE', #100092, #6868, #52971 ) ;
#17784=ORIENTED_EDGE ( 'NONE', *, *, #95834, .T. ) ;
#17785=CARTESIAN_POINT ( 'NONE',  ( 189.6669961101834190, 274.2288721523702861, -15.66740572939721154 ) ) ;
#17788=CARTESIAN_POINT ( 'NONE',  ( 200.9521687275011175, 282.5876292032514243, -18.16013154125647944 ) ) ;
#17792=EDGE_CURVE ( 'NONE', #23912, #54506, #98602, .T. ) ;
#17793=CARTESIAN_POINT ( 'NONE',  ( 157.8239779013331372, 257.2878469527003062, -17.92251383114021479 ) ) ;
#17794=CARTESIAN_POINT ( 'NONE',  ( 101.7984123748231298, 220.3923013555410080, 4.594050593750050204 ) ) ;
#17795=VECTOR ( 'NONE', #21141, 1000.000000000000000 ) ;
#17796=CARTESIAN_POINT ( 'NONE',  ( 87.96987174722529801, 210.0494855054051584, -2.679491924311248496 ) ) ;
#17798=FACE_OUTER_BOUND ( 'NONE', #63296, .T. ) ;
#17803=CARTESIAN_POINT ( 'NONE',  ( 57.65757265809627796, 216.3464784336661637, 1.353441290958777525E-15 ) ) ;
#17805=CARTESIAN_POINT ( 'NONE',  ( 191.5451565139252068, 298.8810523045859213, 7.782291334092181323 ) ) ;
#17806=CARTESIAN_POINT ( 'NONE',  ( 198.1915864813676933, 287.3690979120270867, 17.02875488965938189 ) ) ;
#17807=CARTESIAN_POINT ( 'NONE',  ( 174.6077656993458902, 272.0895251850873251, 16.48419557227402521 ) ) ;
#17812=CARTESIAN_POINT ( 'NONE',  ( 178.0498610173981433, 288.8670518452568672, 10.97635994419254324 ) ) ;
#17815=CARTESIAN_POINT ( 'NONE',  ( 172.0900369064530082, 258.7028160241414412, -13.89453031103171909 ) ) ;
#17816=CARTESIAN_POINT ( 'NONE',  ( 174.2114552513667434, 277.4090650679840451, -15.60050915102441849 ) ) ;
#17817=CARTESIAN_POINT ( 'NONE',  ( 161.0974665087481981, 251.6179983666593216, -13.69252715295363210 ) ) ;
#17818=CARTESIAN_POINT ( 'NONE',  ( 71.90223342829800401, 218.9865022471902876, -10.00000000000009592 ) ) ;
#17820=CARTESIAN_POINT ( 'NONE',  ( 149.6700657135140489, 271.4108371424580355, 12.58635654151485284 ) ) ;
#17822=CARTESIAN_POINT ( 'NONE',  ( 206.4768661561222984, 273.0185725604343361, 11.39716120335626925 ) ) ;
#17824=CARTESIAN_POINT ( 'NONE',  ( 164.1198370452240454, 253.9973699534765501, 14.40966736368955026 ) ) ;
#17825=FACE_OUTER_BOUND ( 'NONE', #24765, .T. ) ;
#17826=CARTESIAN_POINT ( 'NONE',  ( 102.3121810886138832, 236.0024278399160949, 9.188101187500095079 ) ) ;
#17828=CARTESIAN_POINT ( 'NONE',  ( 191.4082244002820516, 299.1182256826033949, -8.271837126846561361 ) ) ;
#17830=CARTESIAN_POINT ( 'NONE',  ( 203.3684377202211522, 278.4025285431072803, -16.56116267537666076 ) ) ;
#17832=FACE_OUTER_BOUND ( 'NONE', #17950, .T. ) ;
#17835=CARTESIAN_POINT ( 'NONE',  ( 174.8082613492344706, 252.7768654443898697, 5.092377277474876784 ) ) ;
#17836=ORIENTED_EDGE ( 'NONE', *, *, #94713, .F. ) ;
#17840=CARTESIAN_POINT ( 'NONE',  ( 184.5707630536305714, 261.7313796936621770, 9.605701619106270073 ) ) ;
#17841=CARTESIAN_POINT ( 'NONE',  ( 164.4575000359379828, 245.7982495824318505, -1.032884424947213997 ) ) ;
#17842=CARTESIAN_POINT ( 'NONE',  ( 134.2197177853555843, 257.4869531367911577, 4.594050593750046652 ) ) ;
#17843=CARTESIAN_POINT ( 'NONE',  ( 150.9584389135710865, 269.1793093008492406, -15.82751450793727699 ) ) ;
#17845=CARTESIAN_POINT ( 'NONE',  ( 187.6000567067785596, 297.9053677150377553, 4.710378011297792433 ) ) ;
#17847=CARTESIAN_POINT ( 'NONE',  ( 57.82012596918833935, 210.3149278399160664, 9.188101187500093303 ) ) ;
#17849=CARTESIAN_POINT ( 'NONE',  ( 171.0605077851577391, 249.7720551134824802, 4.373113433538289740 ) ) ;
#17851=CARTESIAN_POINT ( 'NONE',  ( 174.8228812346009420, 261.7023400441105991, 14.27858715412817681 ) ) ;
#17855=AXIS2_PLACEMENT_3D ( 'NONE', #64300, #94731, #95756 ) ;
#17856=CARTESIAN_POINT ( 'NONE',  ( 193.2148890581035516, 289.1379580677868830, 16.18061100571382838 ) ) ;
#17858=CARTESIAN_POINT ( 'NONE',  ( 123.2683651867145898, 248.6427522451419350, 10.00000000000009237 ) ) ;
#17859=B_SPLINE_CURVE_WITH_KNOTS ( 'NONE', 3,
 ( #79924, #55555, #39845, #32271 ),
 .UNSPECIFIED., .F., .F.,
 ( 4, 4 ),
 ( 0.004970936986721591171, 0.01054214532650148139 ),
 .UNSPECIFIED. ) ;
#17862=VERTEX_POINT ( 'NONE', #84050 ) ;
#17863=CARTESIAN_POINT ( 'NONE',  ( 190.6084209867335915, 300.5035258309363826, -0.5505750481748228342 ) ) ;
#17865=CARTESIAN_POINT ( 'NONE',  ( 50.26990084964904071, 190.6423013555410080, -4.594050593750043987 ) ) ;
#17866=B_SPLINE_CURVE_WITH_KNOTS ( 'NONE', 3,
 ( #37996, #31902, #77009, #62806, #30915, #84655, #99834, #54696, #23807, #85680, #22317, #9120, #24321, #84171, #61802, #32419, #85158, #93252, #53699, #68909, #16217, #7112, #30418, #55196, #7615, #86180, #23304, #15200, #61308, #47109, #78029, #8621, #92270, #46604, #46096, #38503, #70414, #1537, #16714, #47607, #69418, #62295, #45601, #39992, #54193, #70931, #22818, #8127 ),
 .UNSPECIFIED., .F., .F.,
 ( 4, 2, 2, 2, 2, 2, 2, 2, 2, 2, 2, 2, 2, 2, 2, 2, 2, 2, 2, 2, 2, 2, 2, 4 ),
 ( 0.0006475970585499132631, 0.001633499019554147860, 0.001879974509805226648, 0.002126450000056305436, 0.002249687745181803630, 0.002372925490307301391, 0.002496163235432799152, 0.002619400980558297346, 0.002865876470809139778, 0.003112351961059982210, 0.003605302941561666641, 0.004591204902565082339, 0.005577106863568498905, 0.006070057844070207188, 0.006563008824571915471, 0.006686246569697319557, 0.006747865442260097060, 0.006809484314822874564, 0.006932722059948418294, 0.007055959805073961158, 0.007302435295325071171, 0.007548910785576180317, 0.008041861766078397741, 0.008534812746580616033 ),
 .UNSPECIFIED. ) ;
#17868=CARTESIAN_POINT ( 'NONE',  ( 191.2966886305924277, 269.6700499042153751, 14.73436473925947254 ) ) ;
#17869=CARTESIAN_POINT ( 'NONE',  ( 73.90491717100159974, 220.1427522451418781, 10.00000000000009415 ) ) ;
#17870=CARTESIAN_POINT ( 'NONE',  ( 190.9586609929293104, 299.8968923453624598, -4.970176667899034229 ) ) ;
#17872=CARTESIAN_POINT ( 'NONE',  ( 198.1299909997756572, 277.6936685613563327, -16.45399728936175521 ) ) ;
#17873=CARTESIAN_POINT ( 'NONE',  ( 60.98670489788378291, 196.0177522451417929, 5.000000000000051514 ) ) ;
#17875=CARTESIAN_POINT ( 'NONE',  ( 181.0163322597064735, 256.3998266669695454, 1.320919897633525686 ) ) ;
#17876=CARTESIAN_POINT ( 'NONE',  ( 157.8043799545718286, 257.3217915922150496, -17.97575562758749257 ) ) ;
#17879=CARTESIAN_POINT ( 'NONE',  ( 51.11762373747155408, 186.9865022471901455, 1.119607411625061291E-15 ) ) ;
#17880=CARTESIAN_POINT ( 'NONE',  ( 184.6791799238867213, 294.3958812847097875, 10.00409762499635846 ) ) ;
#17881=CARTESIAN_POINT ( 'NONE',  ( 208.3132655666949233, 269.8378354783333180, 2.688523655043302707 ) ) ;
#17882=CARTESIAN_POINT ( 'NONE',  ( 4.830370123010505168, 173.5958772461660828, -9.188101187500095079 ) ) ;
#17884=CARTESIAN_POINT ( 'NONE',  ( 163.8743436044941006, 247.1942500250122237, 6.352646675549487476 ) ) ;
#17885=CARTESIAN_POINT ( 'NONE',  ( 185.0827326577621932, 267.3863886128668241, -15.44458570467620007 ) ) ;
#17886=CARTESIAN_POINT ( 'NONE',  ( 192.0963028965829551, 297.9264387674147656, 11.34530024772836754 ) ) ;
#17888=CARTESIAN_POINT ( 'NONE',  ( 155.7565973091642491, 261.3698664144865802, -17.06302194855465970 ) ) ;
#17893=CARTESIAN_POINT ( 'NONE',  ( 150.3919553510150138, 271.7028101267143256, -12.69180684425547234 ) ) ;
#17897=CARTESIAN_POINT ( 'NONE',  ( 153.3438016572222296, 277.7235982778221342, -5.222468100669257041 ) ) ;
#17899=CARTESIAN_POINT ( 'NONE',  ( 207.2372516306344608, 271.7015462852415908, 9.113068844475435526 ) ) ;
#17904=CARTESIAN_POINT ( 'NONE',  ( 207.4764081617721843, 271.2873150223495600, 6.359972247200924578 ) ) ;
#17905=CARTESIAN_POINT ( 'NONE',  ( 191.6375357288227121, 298.3185633171067934, 8.736688151381864387 ) ) ;
#17907=CARTESIAN_POINT ( 'NONE',  ( 194.3252252352508265, 294.0658320307167628, 14.07225870721148731 ) ) ;
#17908=ORIENTED_EDGE ( 'NONE', *, *, #52945, .F. ) ;
#17909=ORIENTED_EDGE ( 'NONE', *, *, #58316, .F. ) ;
#17910=CARTESIAN_POINT ( 'NONE',  ( 159.2882649660388097, 278.2295398647215166, -9.800005944379622136 ) ) ;
#17914=CARTESIAN_POINT ( 'NONE',  ( 188.9259862807830928, 297.2999610039981917, 7.833423077949829505 ) ) ;
#17921=CARTESIAN_POINT ( 'NONE',  ( 161.4844649541891499, 250.9476973967054789, 12.93553496455142415 ) ) ;
#17922=CARTESIAN_POINT ( 'NONE',  ( 166.1882723046687715, 274.1880526520006356, -15.18604489847817440 ) ) ;
#17926=CYLINDRICAL_SURFACE ( 'NONE', #86027, 10.00000000000010658 ) ;
#17931=ORIENTED_EDGE ( 'NONE', *, *, #28146, .F. ) ;
#17934=ORIENTED_EDGE ( 'NONE', *, *, #90245, .F. ) ;
#17935=B_SPLINE_CURVE_WITH_KNOTS ( 'NONE', 3,
 ( #92927, #53877, #22003, #75726, #8307, #52401 ),
 .UNSPECIFIED., .F., .F.,
 ( 4, 2, 4 ),
 ( 0.02140010735210632134, 0.02598537340429217871, 0.03057063945647803607 ),
 .UNSPECIFIED. ) ;
#17936=CARTESIAN_POINT ( 'NONE',  ( 158.8610524726626352, 259.9521463235002443, 17.06794338822354007 ) ) ;
#17937=CARTESIAN_POINT ( 'NONE',  ( 147.5402343333208819, 275.0998133045071086, 7.426466083746204205 ) ) ;
#17938=CARTESIAN_POINT ( 'NONE',  ( 180.3607121444757695, 291.6144073518768209, -9.916234337600110749 ) ) ;
#17940=CARTESIAN_POINT ( 'NONE',  ( 152.6945189806187955, 266.1723304187151484, 16.62409282110771613 ) ) ;
#17946=CARTESIAN_POINT ( 'NONE',  ( 205.8379285891498682, 274.1252448892948905, 10.44730901608240181 ) ) ;
#17947=CARTESIAN_POINT ( 'NONE',  ( 190.8615153089693877, 298.2432307714133799, -9.563193282498932746 ) ) ;
#17948=CARTESIAN_POINT ( 'NONE',  ( 159.2876523829509665, 254.7526883847961017, 15.64395448151312351 ) ) ;
#17950=EDGE_LOOP ( 'NONE', ( #24492, #77620, #11504 ) ) ;
#17951=CARTESIAN_POINT ( 'NONE',  ( 191.0347634949463895, 299.7650789452856657, 5.488533456550475087 ) ) ;
#17955=B_SPLINE_CURVE_WITH_KNOTS ( 'NONE', 3,
 ( #58224, #81571, #73941, #96273, #43522, #41524, #74461, #5040, #66823, #3073, #4527, #35430, #11652, #97266, #27833, #64844, #95792, #26346, #57719, #11163, #42030, #3556, #34435, #26841, #23580, #298, #15480, #6024, #46897, #21238, #67833, #52610, #5532, #21726, #59717, #39274, #28835, #52117, #82585, #83568, #83064, #13638, #98754, #90682, #13149, #31185, #91161, #36920 ),
 .UNSPECIFIED., .F., .F.,
 ( 4, 2, 2, 2, 2, 2, 2, 2, 2, 2, 2, 2, 2, 2, 2, 2, 2, 2, 2, 2, 2, 2, 2, 4 ),
 ( 0.002832262493831907979, 0.003034780587620233231, 0.003237298681408558049, 0.003338557728302722193, 0.003439816775196886337, 0.003541075822091050047, 0.003642334868985214191, 0.003844852962773611868, 0.004047371056562009545, 0.004452407244138802296, 0.005262479619292319277, 0.006072551994445837126, 0.006882624369599354974, 0.007692696744752871955, 0.007793955791646984925, 0.007844585315093993705, 0.007895214838541001617, 0.007945844361988012999, 0.007996473885435020912, 0.008097732932329217148, 0.008300251026117758807, 0.008502769119906296996, 0.008907805307483380314, 0.009312841495060458427 ),
 .UNSPECIFIED. ) ;
#17957=CARTESIAN_POINT ( 'NONE',  ( 161.0952649348064938, 251.6218116045831437, 13.81854265722852482 ) ) ;
#17961=FACE_OUTER_BOUND ( 'NONE', #96703, .T. ) ;
#17963=CARTESIAN_POINT ( 'NONE',  ( 51.91943859288068097, 212.3297689869269220, -2.679491924311252493 ) ) ;
#17965=CARTESIAN_POINT ( 'NONE',  ( 192.1902081399911708, 278.5511368846052846, 17.60910353013618490 ) ) ;
#17967=CARTESIAN_POINT ( 'NONE',  ( 26.27351996285754510, 172.6427522451417929, 1.119607411625061291E-15 ) ) ;
#17968=CARTESIAN_POINT ( 'NONE',  ( 104.5047417616495125, 221.9548013555409511, -4.594050593750042211 ) ) ;
#17970=DIRECTION ( 'NONE',  ( 0.4999999999999992784, -0.8660254037844390407, 0.000000000000000000 ) ) ;
#17971=CARTESIAN_POINT ( 'NONE',  ( 170.0778888726681259, 280.3528892525189917, -13.69567824744189011 ) ) ;
#17972=CARTESIAN_POINT ( 'NONE',  ( 16.87327557256410060, 189.7369531367911293, -4.594050593750048428 ) ) ;
#17973=CARTESIAN_POINT ( 'NONE',  ( 200.3414094930810165, 283.6454952284590263, 16.87912319229835489 ) ) ;
#17977=CARTESIAN_POINT ( 'NONE',  ( 200.9301851018323930, 267.7613211563358391, -3.272224760724934622 ) ) ;
#17979=CARTESIAN_POINT ( 'NONE',  ( 190.2629546459234859, 273.4080951500121159, -16.67925241984795903 ) ) ;
#17980=DIRECTION ( 'NONE',  ( -0.8660254037844387076, -0.4999999999999998890, -0.000000000000000000 ) ) ;
#17981=CARTESIAN_POINT ( 'NONE',  ( 207.7836085030675690, 270.7552284231231852, -5.468305433308493058 ) ) ;
#17982=CARTESIAN_POINT ( 'NONE',  ( 184.4613657420405559, 285.4439036850075695, 15.12519662030571510 ) ) ;
#17984=CARTESIAN_POINT ( 'NONE',  ( 42.04265951369687571, 185.8923013555410080, 4.594050593750050204 ) ) ;
#17985=CARTESIAN_POINT ( 'NONE',  ( 83.50336539627915045, 219.0177522451418497, -10.00000000000009592 ) ) ;
#17988=CARTESIAN_POINT ( 'NONE',  ( 178.9277264332957316, 259.3186642429575386, -10.30312369890718571 ) ) ;
#17989=CARTESIAN_POINT ( 'NONE',  ( 0.9872088458345583684, 177.5024278399160949, 9.188101187500095079 ) ) ;
#17991=CARTESIAN_POINT ( 'NONE',  ( 161.1750406344237661, 251.4836360396366501, -14.21198410781773802 ) ) ;
#17992=DIRECTION ( 'NONE',  ( -0.8660254037844387076, -0.4999999999999998890, -0.000000000000000000 ) ) ;
#17993=CARTESIAN_POINT ( 'NONE',  ( 192.9523350703175311, 296.4437475495926719, -13.35611922184540923 ) ) ;
#17994=CARTESIAN_POINT ( 'NONE',  ( 193.2752197284765998, 263.9480352582601768, 7.898392093415175452 ) ) ;
#17995=CARTESIAN_POINT ( 'NONE',  ( 171.5690451057043617, 279.9092378594070851, 15.19443294771788189 ) ) ;
#17996=CARTESIAN_POINT ( 'NONE',  ( 147.1259762202154207, 275.8173294038533641, -0.6716460511724978710 ) ) ;
#17997=CARTESIAN_POINT ( 'NONE',  ( 206.9676408587583296, 272.1685258403992975, 7.544050792475608169 ) ) ;
#17998=ORIENTED_EDGE ( 'NONE', *, *, #21952, .F. ) ;
#17999=AXIS2_PLACEMENT_3D ( 'NONE', #8281, #31559, #72093 ) ;
#18000=CARTESIAN_POINT ( 'NONE',  ( 164.4963285489318991, 245.7309966251440301, -6.672251175510283794 ) ) ;
#18001=CARTESIAN_POINT ( 'NONE',  ( -9.359816960141781550, 158.7365022471902023, 10.00000000000009592 ) ) ;
#18003=CARTESIAN_POINT ( 'NONE',  ( 102.9345500736427113, 239.4244531367911293, -4.594050593750046652 ) ) ;
#18006=CARTESIAN_POINT ( 'NONE',  ( 151.2671975087473015, 270.6445237267302559, 14.15418255155509542 ) ) ;
#18007=CARTESIAN_POINT ( 'NONE',  ( 195.8449251089225811, 291.4336346372613775, 16.14492769602857081 ) ) ;
#18009=CARTESIAN_POINT ( 'NONE',  ( 204.6262888618301190, 272.9406470939589440, -9.753183039192979464 ) ) ;
#18011=CARTESIAN_POINT ( 'NONE',  ( 190.5804445141703241, 262.3181372627366841, -4.380721925984095932 ) ) ;
#18012=CARTESIAN_POINT ( 'NONE',  ( 149.1486417047969155, 272.3139700178423368, -11.47583619705022606 ) ) ;
#18014=CARTESIAN_POINT ( 'NONE',  ( 190.5052505396941740, 300.1343187134208392, 3.427856936506675556 ) ) ;
#18015=CARTESIAN_POINT ( 'NONE',  ( 176.0802790653596048, 291.8812439832981909, -1.090742048283624088 ) ) ;
#18019=CARTESIAN_POINT ( 'NONE',  ( 178.2382707639212356, 285.7843550335422833, 14.43266090959460435 ) ) ;
#18020=CARTESIAN_POINT ( 'NONE',  ( 165.3873398078029595, 269.6810096676893522, -16.29630396821910310 ) ) ;
#18022=CARTESIAN_POINT ( 'NONE',  ( 199.2993768369113354, 272.2699461441282551, 12.30839096982038505 ) ) ;
#18023=CARTESIAN_POINT ( 'NONE',  ( 156.3272571654081275, 261.0848386047626377, 17.42342629828958067 ) ) ;
#18025=CARTESIAN_POINT ( 'NONE',  ( 148.4345653551533815, 274.8385398012493965, 7.278542558485217917 ) ) ;
#18026=ORIENTED_EDGE ( 'NONE', *, *, #1004, .F. ) ;
#18027=CARTESIAN_POINT ( 'NONE',  ( 190.8877596188617645, 280.8087401328753003, 16.64766537405279223 ) ) ;
#18029=CARTESIAN_POINT ( 'NONE',  ( 195.3658642540283950, 290.3602234657191730, -16.70539931202024775 ) ) ;
#18031=CARTESIAN_POINT ( 'NONE',  ( 167.7652100969719413, 280.9220867458556654, 12.66497483005768210 ) ) ;
#18033=CARTESIAN_POINT ( 'NONE',  ( 147.6095889327917803, 274.9796876144846465, -8.460961150142429332 ) ) ;
#18034=CARTESIAN_POINT ( 'NONE',  ( 165.3053181839423473, 245.9328214431010338, -1.040564150934635057 ) ) ;
#18037=FACE_OUTER_BOUND ( 'NONE', #87443, .T. ) ;
#18040=CARTESIAN_POINT ( 'NONE',  ( 189.4949498660852214, 300.2643150046559413, 3.278686253974624432 ) ) ;
#18041=CARTESIAN_POINT ( 'NONE',  ( 155.5322964227545413, 261.2571557083629159, -18.35853982030605280 ) ) ;
#18044=CARTESIAN_POINT ( 'NONE',  ( 179.0484917649878298, 259.9789987921100192, 12.89662402083353854 ) ) ;
#18052=B_SPLINE_CURVE_WITH_KNOTS ( 'NONE', 3,
 ( #48906, #72219, #33195, #3322 ),
 .UNSPECIFIED., .F., .F.,
 ( 4, 4 ),
 ( 0.02444194389405377615, 0.03368619770401917735 ),
 .UNSPECIFIED. ) ;
#18053=CARTESIAN_POINT ( 'NONE',  ( 147.1889317863637530, 275.7082871646651370, -6.244700368100694732 ) ) ;
#18054=CARTESIAN_POINT ( 'NONE',  ( 192.3030664838027519, 265.4539026115626257, 10.80274721496235735 ) ) ;
#18056=CARTESIAN_POINT ( 'NONE',  ( 152.7375212135632125, 266.0978483664162582, -16.47968945089317572 ) ) ;
#18058=CARTESIAN_POINT ( 'NONE',  ( 154.1353700909746181, 279.5493911791057826, 2.161561130678962606 ) ) ;
#18059=CARTESIAN_POINT ( 'NONE',  ( 136.7913381204293728, 237.5327760586659736, 1.948934522072303157E-15 ) ) ;
#18064=CARTESIAN_POINT ( 'NONE',  ( 203.5186246619243207, 276.4695941624181046, 13.73756916699280417 ) ) ;
#18065=ADVANCED_FACE ( 'NONE', ( #35663 ), #9766, .F. ) ;
#18066=CARTESIAN_POINT ( 'NONE',  ( 179.6182561431837428, 255.5231795168529345, 1.315866801863230240 ) ) ;
#18067=CARTESIAN_POINT ( 'NONE',  ( 172.5766600205861607, 288.7097676792643028, -4.646140225306805149 ) ) ;
#18069=CARTESIAN_POINT ( 'NONE',  ( 157.3706863651409549, 280.2504512272545867, -7.019172882110545686 ) ) ;
#18073=AXIS2_PLACEMENT_3D ( 'NONE', #2328, #72746, #3339 ) ;
#18074=CARTESIAN_POINT ( 'NONE',  ( 195.1239386621870437, 291.9024892941676512, 15.58172254008325019 ) ) ;
#18076=CARTESIAN_POINT ( 'NONE',  ( 195.3887114072277882, 286.2014090520565901, -17.68059800431107220 ) ) ;
#18077=CARTESIAN_POINT ( 'NONE',  ( 152.7506372714153713, 273.5640845184121872, 11.93689953919982649 ) ) ;
#18081=CARTESIAN_POINT ( 'NONE',  ( 204.2869422847054182, 269.1846276741756014, -2.932770657268202630 ) ) ;
#18082=CARTESIAN_POINT ( 'NONE',  ( 191.4039669030298967, 299.1255998841573387, -10.25374536856971019 ) ) ;
#18084=CARTESIAN_POINT ( 'NONE',  ( 202.8787628851569593, 279.2506702366259788, 17.01435431865322556 ) ) ;
#18085=CARTESIAN_POINT ( 'NONE',  ( 164.5423507617603320, 283.6868644380134583, -6.754471756332288024 ) ) ;
#18086=CARTESIAN_POINT ( 'NONE',  ( 151.4858105020860251, 274.9918459198586902, -8.658055901311536573 ) ) ;
#18087=CARTESIAN_POINT ( 'NONE',  ( -22.42236680055709641, 157.8615022471902591, 0.000000000000000000 ) ) ;
#18091=CARTESIAN_POINT ( 'NONE',  ( 15.10771242554802463, 167.9824982072973967, -5.229199737892075682E-14 ) ) ;
#18092=CARTESIAN_POINT ( 'NONE',  ( 192.1859061758433143, 297.7712413352111298, 11.15082371775444336 ) ) ;
#18095=CARTESIAN_POINT ( 'NONE',  ( -3.938137090306929711, 168.5333772461660828, 9.188101187500095079 ) ) ;
#18098=LINE ( 'NONE', #97136, #12433 ) ;
#18101=CARTESIAN_POINT ( 'NONE',  ( 163.3065739647292673, 284.2937766533170247, 6.003775226036714763 ) ) ;
#18103=CARTESIAN_POINT ( 'NONE',  ( 163.1096928939807924, 248.1327200311062882, -9.690381021358412283 ) ) ;
#18104=CARTESIAN_POINT ( 'NONE',  ( 207.7730309186906084, 270.7735493366856190, 6.335709893618091115 ) ) ;
#18106=CARTESIAN_POINT ( 'NONE',  ( 168.3557124657904467, 273.6222795104500278, 17.14480014634877136 ) ) ;
#18108=LINE ( 'NONE', #97142, #18909 ) ;
#18110=CARTESIAN_POINT ( 'NONE',  ( 48.37494963522306080, 207.9244531367911293, -4.594050593750046652 ) ) ;
#18112=CARTESIAN_POINT ( 'NONE',  ( 76.25066296318219372, 205.6423013555409796, -4.594050593750043987 ) ) ;
#18113=CARTESIAN_POINT ( 'NONE',  ( 207.7836085030675690, 270.7552284231231852, -5.468305433308493058 ) ) ;
#18117=CARTESIAN_POINT ( 'NONE',  ( 152.1020077497548755, 267.1985899746260316, 15.41056800135520710 ) ) ;
#18119=EDGE_CURVE ( 'NONE', #90508, #90974, #73298, .T. ) ;
#18125=CARTESIAN_POINT ( 'NONE',  ( 78.09096694622414248, 206.7048013555409796, 4.594050593750051981 ) ) ;
#18129=CARTESIAN_POINT ( 'NONE',  ( 154.1134794093426592, 263.7146188622353407, 17.41994999336771244 ) ) ;
#18130=EDGE_CURVE ( 'NONE', #48457, #82532, #76182, .T. ) ;
#18132=CARTESIAN_POINT ( 'NONE',  ( 191.0557287345794180, 287.0893601664016614, 16.13915540770992152 ) ) ;
#18133=CARTESIAN_POINT ( 'NONE',  ( 136.0806360202347491, 237.8262482093457493, 3.021315404115420679E-15 ) ) ;
#18135=CARTESIAN_POINT ( 'NONE',  ( 129.0599100780710558, 231.9865022471901455, 1.119607411625061291E-15 ) ) ;
#18140=ORIENTED_EDGE ( 'NONE', *, *, #3900, .T. ) ;
#18141=CARTESIAN_POINT ( 'NONE',  ( 163.1014434023538513, 248.1470085697407058, 9.692260209037655727 ) ) ;
#18144=CARTESIAN_POINT ( 'NONE',  ( 149.8050492866161392, 271.5723974896224604, -11.69608657949948061 ) ) ;
#18147=VERTEX_POINT ( 'NONE', #70541 ) ;
#18149=CARTESIAN_POINT ( 'NONE',  ( 147.8505793332463725, 274.5622799967613332, -9.317516487097901035 ) ) ;
#18150=CARTESIAN_POINT ( 'NONE',  ( 148.5802502259396647, 273.7349012789782137, 8.359561399005384530 ) ) ;
#18151=VERTEX_POINT ( 'NONE', #41126 ) ;
#18156=CARTESIAN_POINT ( 'NONE',  ( 168.0771236874269334, 276.6984061524693175, 15.22277158092185978 ) ) ;
#18157=ADVANCED_FACE ( 'NONE', ( #23938 ), #32552, .T. ) ;
#18160=ORIENTED_EDGE ( 'NONE', *, *, #23514, .F. ) ;
#18161=CARTESIAN_POINT ( 'NONE',  ( 183.0745236532343370, 295.8212215650241887, 0.6855209140772098309 ) ) ;
#18162=CARTESIAN_POINT ( 'NONE',  ( 164.0741338217690668, 246.4622593432776796, 7.359073626423302983 ) ) ;
#18163=CARTESIAN_POINT ( 'NONE',  ( 147.9133274879049793, 274.4535970048112290, -9.359166267164972908 ) ) ;
#18164=CARTESIAN_POINT ( 'NONE',  ( 207.9743173328493526, 270.4249110404894054, -2.481515874287090639 ) ) ;
#18165=CARTESIAN_POINT ( 'NONE',  ( 194.1011995340913074, 294.4538559273262877, 13.93949783759920713 ) ) ;
#18166=CARTESIAN_POINT ( 'NONE',  ( 185.2119534494709967, 292.8366621963887724, -11.93359106299072359 ) ) ;
#18167=CARTESIAN_POINT ( 'NONE',  ( 157.6500260163024620, 257.5891404556457474, -18.23450497588216379 ) ) ;
#18168=CARTESIAN_POINT ( 'NONE',  ( 207.3563322976324912, 271.4952925198022058, -4.480576336268985216 ) ) ;
#18169=CARTESIAN_POINT ( 'NONE',  ( 166.3373473137807252, 265.5045842688243738, 16.55012934221398169 ) ) ;
#18171=CARTESIAN_POINT ( 'NONE',  ( 90.40467888234286420, 216.8768266524159856, -9.188101187500091527 ) ) ;
#18173=CARTESIAN_POINT ( 'NONE',  ( 150.1167764007130643, 271.3850789835987030, 12.27179235466227603 ) ) ;
#18177=CARTESIAN_POINT ( 'NONE',  ( 168.2073321238995049, 267.1113765662216792, -17.52088750715768484 ) ) ;
#18178=ORIENTED_EDGE ( 'NONE', *, *, #32022, .T. ) ;
#18182=ADVANCED_FACE ( 'NONE', ( #47731 ), #1158, .T. ) ;
#18183=CARTESIAN_POINT ( 'NONE',  ( 84.00308638938395234, 207.7592609112379876, 2.679491924311254714 ) ) ;
#18184=CARTESIAN_POINT ( 'NONE',  ( 191.0702043019150835, 299.7036936669546776, -8.800021049343948576 ) ) ;
#18185=B_SPLINE_SURFACE_WITH_KNOTS ( 'NONE', 3, 1, ( 
 ( #43318, #82876 ),
 ( #50923, #21056 ),
 ( #74264, #81873 ),
 ( #51935, #34729 ),
 ( #73742, #36716 ),
 ( #58034, #59002 ),
 ( #98552, #82390 ),
 ( #29141, #35733 ),
 ( #66630, #60010 ),
 ( #20549, #90975 ),
 ( #51427, #21535 ),
 ( #43821, #52417 ),
 ( #65628, #27149 ),
 ( #4333, #13875 ),
 ( #12907, #59958 ),
 ( #37654, #43265 ),
 ( #50875, #74210 ),
 ( #90930, #43766 ),
 ( #21480, #5773 ),
 ( #81824, #19996 ),
 ( #58948, #60453 ),
 ( #83814, #74710 ),
 ( #75689, #58468 ),
 ( #28572, #4800 ),
 ( #21971, #14381 ),
 ( #52368, #36662 ),
 ( #35681, #36166 ),
 ( #76199, #51371 ),
 ( #90433, #59452 ),
 ( #21005, #83313 ),
 ( #13395, #44756 ),
 ( #51886, #66583 ),
 ( #6775, #82827 ),
 ( #82339, #67569 ) ),
 .UNSPECIFIED., .T., .F., .F.,
 ( 4, 2, 2, 2, 2, 2, 2, 2, 2, 2, 2, 2, 2, 2, 2, 2, 4 ),
 ( 2, 2 ),
 ( 0.000000000000000000, 0.06250000000000000000, 0.1250000000000000000, 0.1875000000000000000, 0.2500000000000000000, 0.3125000000000000000, 0.3750000000000000000, 0.4375000000000000000, 0.5000000000000000000, 0.5625000000000000000, 0.6250000000000000000, 0.6875000000000000000, 0.7500000000000000000, 0.8125000000000000000, 0.8750000000000000000, 0.9375000000000000000, 1.000000000000000000 ),
 ( 0.000000000000000000, 1.000000000000000000 ),
 .UNSPECIFIED. ) ;
#18188=CARTESIAN_POINT ( 'NONE',  ( 162.4993287900620942, 249.1899016702093661, 10.54298717179175071 ) ) ;
#18189=CARTESIAN_POINT ( 'NONE',  ( 102.2314250767153538, 220.6423013555409796, -4.594050593750043987 ) ) ;
#18192=ORIENTED_EDGE ( 'NONE', *, *, #95990, .F. ) ;
#18193=CARTESIAN_POINT ( 'NONE',  ( 118.5773942495489166, 239.2677522451418497, 10.00000000000009592 ) ) ;
#18194=CARTESIAN_POINT ( 'NONE',  ( 162.7070706717508699, 248.8300821762643693, -9.986337079333621247 ) ) ;
#18195=ORIENTED_EDGE ( 'NONE', *, *, #26405, .T. ) ;
#18198=FACE_OUTER_BOUND ( 'NONE', #58373, .T. ) ;
#18203=CARTESIAN_POINT ( 'NONE',  ( 204.6163864379986705, 276.2410179586759682, 14.66911174422491726 ) ) ;
#18205=CARTESIAN_POINT ( 'NONE',  ( 160.6175188173358492, 275.6489243641970575, 12.85245945024576564 ) ) ;
#18207=EDGE_CURVE ( 'NONE', #23003, #65011, #30936, .T. ) ;
#18208=CARTESIAN_POINT ( 'NONE',  ( 188.8357241328549492, 269.5691870241041102, 14.73685245099255958 ) ) ;
#18209=CARTESIAN_POINT ( 'NONE',  ( 183.3702726886198491, 288.7829620135148048, 14.41901549737766253 ) ) ;
#18211=CARTESIAN_POINT ( 'NONE',  ( 147.6497331045811734, 249.4111022060903622, 10.00000000000009770 ) ) ;
#18212=ORIENTED_EDGE ( 'NONE', *, *, #57306, .F. ) ;
#18213=CARTESIAN_POINT ( 'NONE',  ( 149.0580910181880654, 274.3322375007426217, 9.004245725843048831 ) ) ;
#18214=CARTESIAN_POINT ( 'NONE',  ( 161.4469036912142599, 251.0127554125742222, 12.93933463576739307 ) ) ;
#18216=CARTESIAN_POINT ( 'NONE',  ( 167.9211111253673323, 249.4040118433879627, 8.061254949035708606 ) ) ;
#18218=CARTESIAN_POINT ( 'NONE',  ( 176.7048560268192716, 290.6280913003972728, -6.170303688665058850 ) ) ;
#18219=CARTESIAN_POINT ( 'NONE',  ( 162.9935763125246240, 248.3338398497890580, -10.29128364753544034 ) ) ;
#18220=ORIENTED_EDGE ( 'NONE', *, *, #12183, .F. ) ;
#18221=CARTESIAN_POINT ( 'NONE',  ( 164.9779129355220562, 244.8968679994381148, -1.771286574179712803 ) ) ;
#18222=CARTESIAN_POINT ( 'NONE',  ( 179.1221870662444928, 265.9242797405647138, -14.83509186512012867 ) ) ;
#18223=CARTESIAN_POINT ( 'NONE',  ( 184.6099029562445253, 266.0940484426244552, 13.19535090614431816 ) ) ;
#18226=CARTESIAN_POINT ( 'NONE',  ( 192.2943420783192323, 297.5834248427583475, 12.53393473147773562 ) ) ;
#18231=( BOUNDED_CURVE ( )  B_SPLINE_CURVE ( 2, ( #659, #84798, #45742, #84307, #22949, #76192, #69051, #85305, #70046 ),
 .UNSPECIFIED., .F., .T. ) 
 B_SPLINE_CURVE_WITH_KNOTS ( ( 3, 2, 2, 2, 3 ),
 ( 0.3911290322580645018, 0.3924731182795698770, 0.3951612903225806273, 0.3978494623655913776, 0.3991935483870967527 ),
 .UNSPECIFIED. ) 
 CURVE ( )  GEOMETRIC_REPRESENTATION_ITEM ( )  RATIONAL_B_SPLINE_CURVE ( ( 0.9330127018922194093, 0.9330127018922194093, 1.000000000000000000, 0.8660254037844387076, 1.000000000000000000, 0.8660254037844387076, 1.000000000000000000, 0.9330127018922194093, 0.9330127018922194093 ) ) 
 REPRESENTATION_ITEM ( '' )  );
#18232=CARTESIAN_POINT ( 'NONE',  ( 10.86574497745707646, 167.8923013555410080, 4.594050593750050204 ) ) ;
#18233=B_SPLINE_CURVE_WITH_KNOTS ( 'NONE', 3,
 ( #13991, #66687, #36780, #74819, #83425, #52477, #52979, #22581, #6877, #67182, #45372, #4907, #98617, #13507, #67688, #44377, #76305, #61065, #30177, #59568 ),
 .UNSPECIFIED., .F., .F.,
 ( 4, 2, 2, 2, 2, 2, 2, 2, 2, 4 ),
 ( 0.003620162585681084913, 0.003755372724757697310, 0.003890582863834310141, 0.004025793002910922971, 0.004161003141987535368, 0.004431423420140844296, 0.004701843698294154092, 0.005242684254600804040, 0.005783524810907454856, 0.007946887036134204704 ),
 .UNSPECIFIED. ) ;
#18237=PLANE ( 'NONE',  #77460 ) ;
#18238=CARTESIAN_POINT ( 'NONE',  ( 202.9461111005703913, 274.5853058359568308, -12.78354684315880618 ) ) ;
#18240=CARTESIAN_POINT ( 'NONE',  ( 34.35668405510998724, 181.4548013555409796, -4.594050593750042211 ) ) ;
#18242=AXIS2_PLACEMENT_3D ( 'NONE', #67945, #98865, #61323 ) ;
#18243=CARTESIAN_POINT ( 'NONE',  ( 200.4403816905005158, 283.4740703539914648, 16.81798557643505987 ) ) ;
#18246=CARTESIAN_POINT ( 'NONE',  ( 181.3918697797460311, 294.4956595908585086, 6.501009157982572617 ) ) ;
#18247=FACE_OUTER_BOUND ( 'NONE', #12844, .T. ) ;
#18249=CARTESIAN_POINT ( 'NONE',  ( 165.8975677354378035, 271.5909624305264174, 17.28637137770206067 ) ) ;
#18253=CARTESIAN_POINT ( 'NONE',  ( 95.28491933047791917, 212.4865022471901455, 1.119607411625061291E-15 ) ) ;
#18254=CARTESIAN_POINT ( 'NONE',  ( 164.6319316456770139, 246.1186112673341597, 1.146231737620790891 ) ) ;
#18255=CARTESIAN_POINT ( 'NONE',  ( 183.3350989353408806, 260.3215222104232680, -10.84733429619501699 ) ) ;
#18256=CARTESIAN_POINT ( 'NONE',  ( 39.14627965220388006, 205.6589784336661637, -6.496448406907675876E-16 ) ) ;
#18257=DIRECTION ( 'NONE',  ( 0.4999999999999992784, -0.8660254037844390407, 0.000000000000000000 ) ) ;
#18260=CARTESIAN_POINT ( 'NONE',  ( 147.5813496936708020, 275.0285994114094592, 4.516581957185684004 ) ) ;
#18265=CARTESIAN_POINT ( 'NONE',  ( 168.7715202826167911, 285.3210262249357356, 7.552708256878819526 ) ) ;
#18266=CARTESIAN_POINT ( 'NONE',  ( 168.0576292222695542, 281.8341897004820567, -11.13511954253887914 ) ) ;
#18267=DIRECTION ( 'NONE',  ( 0.4999999999999998890, -0.8660254037844385966, 0.000000000000000000 ) ) ;
#18268=CARTESIAN_POINT ( 'NONE',  ( 86.83108767939293671, 232.4860189848785410, -2.679491924311252493 ) ) ;
#18270=CARTESIAN_POINT ( 'NONE',  ( 163.2835940097493790, 247.8315144631017404, 11.08416305054517359 ) ) ;
#18271=CARTESIAN_POINT ( 'NONE',  ( 149.3141802193904368, 272.0272488999566463, -11.40332369054239336 ) ) ;
#18272=CARTESIAN_POINT ( 'NONE',  ( 171.3930954440937739, 255.6893612109813034, 11.28323771083614524 ) ) ;
#18276=CARTESIAN_POINT ( 'NONE',  ( 171.8875188505430458, 252.3843871569532098, 8.791676787938541793 ) ) ;
#18280=CARTESIAN_POINT ( 'NONE',  ( 179.1455725186695815, 282.4470739261427639, 15.26283603612785988 ) ) ;
#18287=CARTESIAN_POINT ( 'NONE',  ( 188.5138031843794124, 273.5367886141518738, -15.67519387171974543 ) ) ;
#18289=CARTESIAN_POINT ( 'NONE',  ( 149.3629284598386278, 271.9428144707212027, -12.99253781774931049 ) ) ;
#18290=VERTEX_POINT ( 'NONE', #50708 ) ;
#18292=CARTESIAN_POINT ( 'NONE',  ( 191.6399467885100876, 261.9049270161082177, -5.586019516979663813 ) ) ;
#18296=CARTESIAN_POINT ( 'NONE',  ( 116.7102005222951817, 232.0643266524159856, -9.188101187500093303 ) ) ;
#18297=CARTESIAN_POINT ( 'NONE',  ( 80.83312040127709963, 224.1427522451419065, -10.00000000000009592 ) ) ;
#18299=CARTESIAN_POINT ( 'NONE',  ( 163.8398374448017591, 246.8680725722146008, -5.948785025486735378 ) ) ;
#18300=ORIENTED_EDGE ( 'NONE', *, *, #5026, .F. ) ;
#18303=CARTESIAN_POINT ( 'NONE',  ( 204.8009505137602844, 275.5216285192182113, -12.34812582524854285 ) ) ;
#18304=CARTESIAN_POINT ( 'NONE',  ( 62.47501251452969484, 213.0024278399160949, -9.188101187500093303 ) ) ;
#18307=CARTESIAN_POINT ( 'NONE',  ( 183.9509481277042937, 296.4026742571778641, 5.972361342789342942 ) ) ;
#18308=CARTESIAN_POINT ( 'NONE',  ( 173.2210010745182842, 271.2950951356299925, 16.42349981143101090 ) ) ;
#18309=VERTEX_POINT ( 'NONE', #81661 ) ;
#18312=CARTESIAN_POINT ( 'NONE',  ( 169.3571508527084291, 283.0956279022483955, 12.63651818596384935 ) ) ;
#18314=CARTESIAN_POINT ( 'NONE',  ( 172.2467550100553808, 258.4300157609564508, -14.58559033337875377 ) ) ;
#18315=CARTESIAN_POINT ( 'NONE',  ( 174.2667842284330675, 277.2948997594879756, -15.61071884909420682 ) ) ;
#18316=CARTESIAN_POINT ( 'NONE',  ( 161.5083988044524119, 250.9062427520286178, -14.53522982831775856 ) ) ;
#18317=CARTESIAN_POINT ( 'NONE',  ( 206.5157691485259761, 270.5309844673936368, 2.116125166999188068 ) ) ;
#18319=EDGE_CURVE ( 'NONE', #30468, #20065, #68233, .T. ) ;
#18320=CARTESIAN_POINT ( 'NONE',  ( 148.9719199701866899, 272.6200610409887872, 12.59512981512031438 ) ) ;
#18322=CARTESIAN_POINT ( 'NONE',  ( 32.13723363786251497, 199.3615022471903160, 5.000000000000046185 ) ) ;
#18325=CARTESIAN_POINT ( 'NONE',  ( 164.4513687979423082, 254.3942805075391504, 14.15307082335797695 ) ) ;
#18326=CARTESIAN_POINT ( 'NONE',  ( 208.2777459429579210, 269.8993572713111462, 3.129643751043610589 ) ) ;
#18327=EDGE_CURVE ( 'NONE', #17163, #80346, #97345, .T. ) ;
#18328=CARTESIAN_POINT ( 'NONE',  ( 121.1210835531159091, 249.9244531367911293, -4.594050593750046652 ) ) ;
#18333=ADVANCED_FACE ( 'NONE', ( #8609 ), #78019, .T. ) ;
#18334=CARTESIAN_POINT ( 'NONE',  ( 171.0677017869332417, 283.0637397488268334, -13.46002028830316988 ) ) ;
#18335=CARTESIAN_POINT ( 'NONE',  ( 163.7729086741176161, 246.9839966035275438, 6.099406794390714204 ) ) ;
#18337=CARTESIAN_POINT ( 'NONE',  ( 174.8587845204546056, 252.5724801960949151, 5.155470236899263092 ) ) ;
#18340=CARTESIAN_POINT ( 'NONE',  ( 158.4705108345335987, 275.1496518313210231, -12.42170905744487364 ) ) ;
#18341=CARTESIAN_POINT ( 'NONE',  ( 183.6436237883546880, 261.3127158997198762, 9.534748110082331252 ) ) ;
#18342=CARTESIAN_POINT ( 'NONE',  ( 34.13991738056614622, 190.5177522451418497, -10.00000000000009592 ) ) ;
#18343=CARTESIAN_POINT ( 'NONE',  ( 141.9874905431360332, 240.5327760586659451, 1.948934522072302763E-15 ) ) ;
#18344=CARTESIAN_POINT ( 'NONE',  ( 188.5502890729128183, 299.8136175509387726, -3.629854520258569028 ) ) ;
#18346=DIRECTION ( 'NONE',  ( 0.4999999999999998890, -0.8660254037844385966, 0.000000000000000000 ) ) ;
#18348=CARTESIAN_POINT ( 'NONE',  ( 67.02199298016300588, 203.3768266524159856, -9.188101187500091527 ) ) ;
#18349=CARTESIAN_POINT ( 'NONE',  ( 170.7729407420521284, 250.5257104363971621, 3.420218544161329532 ) ) ;
#18351=CARTESIAN_POINT ( 'NONE',  ( 155.4174679471833826, 279.7120021735884166, -1.458095568104960549 ) ) ;
#18352=CARTESIAN_POINT ( 'NONE',  ( 172.5808743809259909, 287.8688692445808215, -8.370650701620615308 ) ) ;
#18353=CARTESIAN_POINT ( 'NONE',  ( 155.1865148098964937, 261.8560670301561686, -16.99758927948949605 ) ) ;
#18355=CARTESIAN_POINT ( 'NONE',  ( 125.0004159942834860, 249.6427522451419065, -10.00000000000009415 ) ) ;
#18357=ORIENTED_EDGE ( 'NONE', *, *, #8336, .F. ) ;
#18359=CARTESIAN_POINT ( 'NONE',  ( 148.2267527339363369, 273.9107285543102535, 7.913369084260907016 ) ) ;
#18360=CARTESIAN_POINT ( 'NONE',  ( -15.41332078621576329, 174.1589784336661921, -6.496448406907676862E-16 ) ) ;
#18361=CARTESIAN_POINT ( 'NONE',  ( 37.90188877791127453, 186.5643266524160424, 9.188101187500095079 ) ) ;
#18365=CARTESIAN_POINT ( 'NONE',  ( 190.1542208370626099, 290.9744051383607371, -14.40790947658664400 ) ) ;
#18366=CARTESIAN_POINT ( 'NONE',  ( 190.6218339396177441, 300.4802939150614520, -4.178005820806754755 ) ) ;
#18369=CARTESIAN_POINT ( 'NONE',  ( 56.22356517706933943, 203.2677522451418781, 10.00000000000009592 ) ) ;
#18370=CARTESIAN_POINT ( 'NONE',  ( -17.42236680055705023, 149.2012482093457777, 0.000000000000000000 ) ) ;
#18371=CARTESIAN_POINT ( 'NONE',  ( 163.1660858168057473, 256.0097020245835893, -14.93562900060027765 ) ) ;
#18372=CARTESIAN_POINT ( 'NONE',  ( -0.8439004895948557516, 176.9865022471903160, -10.00000000000009592 ) ) ;
#18374=CARTESIAN_POINT ( 'NONE',  ( 179.2814824751584695, 294.6666816158376605, 1.075539458643513191 ) ) ;
#18375=CARTESIAN_POINT ( 'NONE',  ( 30.47735161394232151, 201.7365022471903444, 2.944929066748280225E-16 ) ) ;
#18376=CARTESIAN_POINT ( 'NONE',  ( 185.1158323825266052, 294.3144650231332662, 9.807602087358677778 ) ) ;
#18377=CARTESIAN_POINT ( 'NONE',  ( 202.8787628851569593, 279.2506702366259788, 17.01435431865322556 ) ) ;
#18378=CARTESIAN_POINT ( 'NONE',  ( 0.1751364819041374699, 183.1589784336661637, -6.496448406907675876E-16 ) ) ;
#18381=CARTESIAN_POINT ( 'NONE',  ( 152.6992418905140028, 266.1641500988167763, 17.27767170937316621 ) ) ;
#18383=CARTESIAN_POINT ( 'NONE',  ( 206.3106310032756596, 273.3065002911688453, 10.17860425536756175 ) ) ;
#18385=CARTESIAN_POINT ( 'NONE',  ( 186.3729170633118599, 259.2531417649982473, -2.352328541926433925 ) ) ;
#18388=CARTESIAN_POINT ( 'NONE',  ( 176.9834359889674715, 260.3444538793796141, -13.76265079422755377 ) ) ;
#18392=CARTESIAN_POINT ( 'NONE',  ( 74.64464720694877542, 207.2365022471902023, -10.00000000000009237 ) ) ;
#18393=AXIS2_PLACEMENT_3D ( 'NONE', #67711, #60087, #91050 ) ;
#18394=CARTESIAN_POINT ( 'NONE',  ( 153.2412541709487357, 277.6964940543419971, -5.155127835892409749 ) ) ;
#18396=CARTESIAN_POINT ( 'NONE',  ( 159.8188415394622268, 253.8326417772889840, -15.43862849427313222 ) ) ;
#18397=CYLINDRICAL_SURFACE ( 'NONE', #60873, 10.00000000000010658 ) ;
#18399=ORIENTED_EDGE ( 'NONE', *, *, #73975, .T. ) ;
#18400=CARTESIAN_POINT ( 'NONE',  ( -22.42236680055709641, 157.8615022471902591, 0.000000000000000000 ) ) ;
#18401=CARTESIAN_POINT ( 'NONE',  ( 207.6727254509676186, 270.9472835030587703, 7.315149605389819953 ) ) ;
#18403=EDGE_CURVE ( 'NONE', #44538, #28481, #42970, .T. ) ;
#18405=VECTOR ( 'NONE', #29368, 1000.000000000000000 ) ;
#18406=CARTESIAN_POINT ( 'NONE',  ( 193.7999837595647250, 294.9755769528473479, 15.24609078262870199 ) ) ;
#18408=VERTEX_POINT ( 'NONE', #35395 ) ;
#18414=CARTESIAN_POINT ( 'NONE',  ( 155.4612256362409255, 261.7625261697407950, -16.98072832849991443 ) ) ;
#18420=VERTEX_POINT ( 'NONE', #74919 ) ;
#18421=CARTESIAN_POINT ( 'NONE',  ( 173.7157974438445081, 267.2565184175704758, 16.75892562235658900 ) ) ;
#18422=CARTESIAN_POINT ( 'NONE',  ( 169.5377272533189625, 276.4473244127411249, -15.81453032960868832 ) ) ;
#18424=B_SPLINE_SURFACE_WITH_KNOTS ( 'NONE', 3, 1, ( 
 ( #25529, #56417 ),
 ( #61997, #8328 ),
 ( #85370, #15916 ),
 ( #24017, #54915 ),
 ( #71145, #85894 ),
 ( #16418, #47313 ),
 ( #78239, #8820 ),
 ( #16915, #78737 ),
 ( #64530, #35111 ),
 ( #3740, #66021 ),
 ( #18441, #12843 ),
 ( #18945, #73629 ),
 ( #50314, #89382 ),
 ( #73144, #57916 ),
 ( #43196, #58888 ),
 ( #3253, #34135 ),
 ( #10834, #2747 ),
 ( #51298, #66516 ),
 ( #88896, #12332 ),
 ( #19935, #20432 ),
 ( #27538, #27032 ),
 ( #33637, #41712 ),
 ( #74140, #95488 ),
 ( #89857, #96971 ),
 ( #88391, #42698 ),
 ( #11355, #58407 ),
 ( #34617, #72658 ),
 ( #95974, #50808 ),
 ( #80781, #26040 ),
 ( #4215, #42209 ),
 ( #4733, #49823 ),
 ( #81758, #43704 ),
 ( #57410, #65517 ),
 ( #97441, #28012 ) ),
 .UNSPECIFIED., .T., .F., .F.,
 ( 4, 2, 2, 2, 2, 2, 2, 2, 2, 2, 2, 2, 2, 2, 2, 2, 4 ),
 ( 2, 2 ),
 ( 0.000000000000000000, 0.06250000000000000000, 0.1250000000000000000, 0.1875000000000000000, 0.2500000000000000000, 0.3125000000000000000, 0.3750000000000000000, 0.4375000000000000000, 0.5000000000000000000, 0.5625000000000000000, 0.6250000000000000000, 0.6875000000000000000, 0.7500000000000000000, 0.8125000000000000000, 0.8750000000000000000, 0.9375000000000000000, 1.000000000000000000 ),
 ( 0.000000000000000000, 1.000000000000000000 ),
 .UNSPECIFIED. ) ;
#18426=CARTESIAN_POINT ( 'NONE',  ( 171.1865699020292766, 254.5746376615227291, -11.62694971751192519 ) ) ;
#18427=CARTESIAN_POINT ( 'NONE',  ( 202.7599932440484451, 279.4563852894229967, 15.58249343055423353 ) ) ;
#18428=ORIENTED_EDGE ( 'NONE', *, *, #89685, .F. ) ;
#18429=ORIENTED_EDGE ( 'NONE', *, *, #57491, .T. ) ;
#18430=CARTESIAN_POINT ( 'NONE',  ( 160.0914855916899171, 268.6372815687846014, -16.51133705495732684 ) ) ;
#18432=CARTESIAN_POINT ( 'NONE',  ( 179.7646977617114601, 254.2800489533466077, -2.868012902750119331 ) ) ;
#18436=CARTESIAN_POINT ( 'NONE',  ( 147.9292452580141912, 274.4260266182387227, 6.430851193091030815 ) ) ;
#18437=CARTESIAN_POINT ( 'NONE',  ( 180.0253394064914119, 291.5621715643180778, -10.00052010529626934 ) ) ;
#18439=CARTESIAN_POINT ( 'NONE',  ( 192.0712386031329686, 297.9698513971258649, 12.12276320360788873 ) ) ;
#18441=CARTESIAN_POINT ( 'NONE',  ( 197.5503536138679976, 288.4797458180196372, -16.78011540949930946 ) ) ;
#18445=CARTESIAN_POINT ( 'NONE',  ( 205.8610808625997208, 274.0851439753691920, 10.38803237360972531 ) ) ;
#18447=CARTESIAN_POINT ( 'NONE',  ( 164.3939401533646958, 245.9083385283718712, 2.844462461176849200 ) ) ;
#18451=CARTESIAN_POINT ( 'NONE',  ( 187.5612807588072428, 277.0616058210526944, 17.40194786215237244 ) ) ;
#18454=CARTESIAN_POINT ( 'NONE',  ( 164.3523996349191805, 247.8276598175897902, 8.684433193650701099 ) ) ;
#18456=CARTESIAN_POINT ( 'NONE',  ( 160.5437591895810954, 252.5770475759798046, -16.01484307027506304 ) ) ;
#18460=CARTESIAN_POINT ( 'NONE',  ( 60.73642589098854216, 194.3262482093457777, 3.021315404115420679E-15 ) ) ;
#18461=CARTESIAN_POINT ( 'NONE',  ( 206.9676408587583296, 272.1685258403992975, 7.544050792475608169 ) ) ;
#18462=CARTESIAN_POINT ( 'NONE',  ( 27.21171415029068186, 176.5177522451417929, 5.000000000000051514 ) ) ;
#18463=CARTESIAN_POINT ( 'NONE',  ( 95.76303752037657091, 226.0958772461660260, -9.188101187500095079 ) ) ;
#18464=CARTESIAN_POINT ( 'NONE',  ( 180.7944058683433752, 294.0821055505414279, -2.743935788258776487 ) ) ;
#18466=CARTESIAN_POINT ( 'NONE',  ( 207.9312334543074599, 270.4995345071110933, 1.552289074598145469 ) ) ;
#18468=CARTESIAN_POINT ( 'NONE',  ( 26.91401791951368949, 186.3458772461660544, 9.188101187500095079 ) ) ;
#18469=CYLINDRICAL_SURFACE ( 'NONE', #99670, 10.00000000000010658 ) ;
#18471=EDGE_LOOP ( 'NONE', ( #85514, #25127, #41454, #49928 ) ) ;
#18472=CARTESIAN_POINT ( 'NONE',  ( 185.1499092832424651, 259.9585293422515520, -5.749318524461872748 ) ) ;
#18475=CARTESIAN_POINT ( 'NONE',  ( 192.9818866559145931, 263.7816602304387175, -4.162437127754325061 ) ) ;
#18477=CARTESIAN_POINT ( 'NONE',  ( 161.1747502674735415, 251.4841389699472529, -13.25152330924089839 ) ) ;
#18480=CARTESIAN_POINT ( 'NONE',  ( 49.83688814775681664, 190.3923013555410080, 4.594050593750050204 ) ) ;
#18481=CARTESIAN_POINT ( 'NONE',  ( 80.90528918492583443, 217.5177522451418497, -10.00000000000009592 ) ) ;
#18483=EDGE_CURVE ( 'NONE', #18408, #81112, #32114, .T. ) ;
#18486=CARTESIAN_POINT ( 'NONE',  ( 157.7632566947985708, 282.3764601569879460, -1.694678876849560645 ) ) ;
#18487=CARTESIAN_POINT ( 'NONE',  ( 0.4734401320438119676, 161.8923013555410080, 4.594050593750050204 ) ) ;
#18489=CARTESIAN_POINT ( 'NONE',  ( 151.1699610800269511, 268.8129421616204695, -14.28929860221299286 ) ) ;
#18490=CARTESIAN_POINT ( 'NONE',  ( 186.1126677289907434, 283.4250391647574929, 17.12934966007601645 ) ) ;
#18491=CARTESIAN_POINT ( 'NONE',  ( 147.3379027498079381, 275.4502618871274535, -3.695260257281167249 ) ) ;
#18493=CARTESIAN_POINT ( 'NONE',  ( 204.6427704787179493, 276.1953194596412118, 13.28850621060895953 ) ) ;
#18494=CARTESIAN_POINT ( 'NONE',  ( 146.5157004908022031, 276.8743579738231233, -0.1877253132609108255 ) ) ;
#18495=CARTESIAN_POINT ( 'NONE',  ( 164.3138894970802824, 246.0469903322357368, -2.642126690130961020 ) ) ;
#18498=CARTESIAN_POINT ( 'NONE',  ( -6.040052912301486110, 173.9865022471903160, -10.00000000000009415 ) ) ;
#18499=CARTESIAN_POINT ( 'NONE',  ( 181.1462475035585271, 268.2071771633989670, 15.44497821374024049 ) ) ;
#18500=CARTESIAN_POINT ( 'NONE',  ( 112.2171730965159071, 247.8464784336661353, 1.353441290958777327E-15 ) ) ;
#18503=CYLINDRICAL_SURFACE ( 'NONE', #71102, 17.82106496071139645 ) ;
#18504=CARTESIAN_POINT ( 'NONE',  ( 157.0935036675524827, 258.5530654392286465, 17.32636058289560665 ) ) ;
#18505=CARTESIAN_POINT ( 'NONE',  ( 185.5122157014849336, 288.1045496927467866, 15.02337816592467057 ) ) ;
#18507=ORIENTED_EDGE ( 'NONE', *, *, #10713, .T. ) ;
#18508=CARTESIAN_POINT ( 'NONE',  ( 193.1827667186879864, 263.4048335427814322, -5.307581698297376249 ) ) ;
#18509=CARTESIAN_POINT ( 'NONE',  ( 196.8435556370661459, 289.7039558245273838, -16.43899056939217118 ) ) ;
#18510=CARTESIAN_POINT ( 'NONE',  ( 189.8641800978502658, 300.0801047183622359, 4.769842506271963600 ) ) ;
#18511=CARTESIAN_POINT ( 'NONE',  ( 176.2543089179515619, 292.5905172262055203, -1.124657176953766102 ) ) ;
#18515=CARTESIAN_POINT ( 'NONE',  ( 175.1327937842674771, 279.3162497976952636, 15.76955821438891903 ) ) ;
#18518=B_SPLINE_CURVE_WITH_KNOTS ( 'NONE', 3,
 ( #9409, #8904, #1317, #40284 ),
 .UNSPECIFIED., .F., .F.,
 ( 4, 4 ),
 ( 0.009203791814746210831, 0.01435997971314354436 ),
 .UNSPECIFIED. ) ;
#18520=CARTESIAN_POINT ( 'NONE',  ( 156.2139277615245589, 261.1003705204080916, 17.33299519700502245 ) ) ;
#18523=CARTESIAN_POINT ( 'NONE',  ( 153.3703256797887775, 265.0017988796566897, 16.44314709207578318 ) ) ;
#18525=CARTESIAN_POINT ( 'NONE',  ( 164.4854433269806577, 246.2060377238486808, -1.879056492287135116 ) ) ;
#18526=EDGE_CURVE ( 'NONE', #9601, #77760, #96109, .T. ) ;
#18528=CARTESIAN_POINT ( 'NONE',  ( 175.0209189270691184, 273.4799616097778880, -16.39738812790832867 ) ) ;
#18532=CARTESIAN_POINT ( 'NONE',  ( 148.3629184514745987, 273.6748826132846375, -8.219814532462343948 ) ) ;
#18533=CARTESIAN_POINT ( 'NONE',  ( -22.42236680055709641, 157.8615022471902591, 0.000000000000000000 ) ) ;
#18534=ORIENTED_EDGE ( 'NONE', *, *, #34080, .F. ) ;
#18537=CARTESIAN_POINT ( 'NONE',  ( 151.1926529451685326, 268.7736386982768408, 14.30343427984827365 ) ) ;
#18539=CARTESIAN_POINT ( 'NONE',  ( 189.8233477357014465, 300.2304324313545294, 3.241907359326032356 ) ) ;
#18540=CARTESIAN_POINT ( 'NONE',  ( 203.5555343017997529, 278.0784677578903370, -15.71723084798551362 ) ) ;
#18541=EDGE_LOOP ( 'NONE', ( #73972, #16001, #12949, #9944 ) ) ;
#18543=ORIENTED_EDGE ( 'NONE', *, *, #54380, .F. ) ;
#18544=DIRECTION ( 'NONE',  ( 0.4999999999999998890, -0.8660254037844385966, 0.000000000000000000 ) ) ;
#18546=CARTESIAN_POINT ( 'NONE',  ( 193.2749530133065150, 294.1419888553381838, 14.05938658124414431 ) ) ;
#18548=ORIENTED_EDGE ( 'NONE', *, *, #63474, .F. ) ;
#18552=CARTESIAN_POINT ( 'NONE',  ( 185.5632263566141944, 282.0228027493975560, -16.47564400571021181 ) ) ;
#18553=B_SPLINE_CURVE_WITH_KNOTS ( 'NONE', 3,
 ( #14625, #96902, #27474, #50739 ),
 .UNSPECIFIED., .F., .F.,
 ( 4, 4 ),
 ( 0.02891663082521821887, 0.03807346097812620150 ),
 .UNSPECIFIED. ) ;
#18556=CARTESIAN_POINT ( 'NONE',  ( 197.3327212804159103, 267.5970440452412049, 9.861675131224707513 ) ) ;
#18557=CARTESIAN_POINT ( 'NONE',  ( 193.2100161762185735, 295.9974307820218087, -12.46499585622781758 ) ) ;
#18558=CARTESIAN_POINT ( 'NONE',  ( 201.3505934466285510, 281.8975373467312693, -16.83770227898004279 ) ) ;
#18561=CARTESIAN_POINT ( 'NONE',  ( 131.6216415740022398, 255.9869531367911009, 4.594050593750046652 ) ) ;
#18565=VERTEX_POINT ( 'NONE', #66304 ) ;
#18569=CARTESIAN_POINT ( 'NONE',  ( 202.5511585997265911, 279.8180975037686835, 17.12781264818056925 ) ) ;
#18572=CARTESIAN_POINT ( 'NONE',  ( 153.4850820818235491, 276.9265329172790757, 7.161006446225682609 ) ) ;
#18575=B_SPLINE_CURVE_WITH_KNOTS ( 'NONE', 3,
 ( #34371, #49566, #5470, #42449, #81028, #97691, #74887 ),
 .UNSPECIFIED., .F., .F.,
 ( 4, 3, 4 ),
 ( 0.000000000000000000, 0.001498044977024529231, 0.003064388198862243000 ),
 .UNSPECIFIED. ) ;
#18576=CARTESIAN_POINT ( 'NONE',  ( 170.9494504878256294, 280.9963802879100285, 14.66202574695598138 ) ) ;
#18582=CARTESIAN_POINT ( 'NONE',  ( 162.6380106777187962, 276.9062633384314722, 12.86980460176377150 ) ) ;
#18583=B_SPLINE_CURVE_WITH_KNOTS ( 'NONE', 3,
 ( #6478, #81645, #26912, #57792, #49701, #12216, #50203, #3144, #81154, #11722, #42584, #29770 ),
 .UNSPECIFIED., .F., .F.,
 ( 4, 2, 2, 2, 2, 4 ),
 ( 0.001861292369029458101, 0.001963120261722284526, 0.002064948154415110516, 0.002268603939800654078, 0.002675915510571577269, 0.003490538652113424952 ),
 .UNSPECIFIED. ) ;
#18584=CARTESIAN_POINT ( 'NONE',  ( 201.0217745861505705, 267.6100443300385336, -2.437338837632460287 ) ) ;
#18585=CARTESIAN_POINT ( 'NONE',  ( 191.6373630319821473, 298.7213459305223182, -9.457989462015230941 ) ) ;
#18586=CARTESIAN_POINT ( 'NONE',  ( 149.6071296322179194, 271.5198456328920997, 12.75640156477042453 ) ) ;
#18588=CARTESIAN_POINT ( 'NONE',  ( 202.3894997978090373, 280.0980987621804275, 16.95659012541789323 ) ) ;
#18591=CYLINDRICAL_SURFACE ( 'NONE', #64076, 17.82106496071139645 ) ;
#18592=ORIENTED_EDGE ( 'NONE', *, *, #73643, .T. ) ;
#18594=CARTESIAN_POINT ( 'NONE',  ( 190.2932943857919099, 273.3550103105087601, -16.39709156336667206 ) ) ;
#18596=CARTESIAN_POINT ( 'NONE',  ( 195.3624787578944222, 290.3824063481519602, -16.76522224015156226 ) ) ;
#18598=CYLINDRICAL_SURFACE ( 'NONE', #85560, 17.82106496071139645 ) ;
#18599=CARTESIAN_POINT ( 'NONE',  ( 202.2603678735342214, 280.3217618159037556, 16.49712126737133744 ) ) ;
#18600=CARTESIAN_POINT ( 'NONE',  ( -13.03140383004354241, 163.2833772461660544, -9.188101187500095079 ) ) ;
#18601=CARTESIAN_POINT ( 'NONE',  ( 101.5001087246834857, 241.6589784336661637, -6.496448406907675876E-16 ) ) ;
#18602=CARTESIAN_POINT ( 'NONE',  ( 155.1398527401465230, 261.9368881057492899, -17.02245700497956449 ) ) ;
#18604=CARTESIAN_POINT ( 'NONE',  ( 164.9009427471078766, 270.4319544559331234, -17.40525121274953335 ) ) ;
#18607=CARTESIAN_POINT ( 'NONE',  ( 195.9879163382961735, 284.2697365227047044, 17.81990856217999664 ) ) ;
#18608=CARTESIAN_POINT ( 'NONE',  ( 163.7707745167360258, 284.3866919517458314, 5.949292284668742603 ) ) ;
#18609=CYLINDRICAL_SURFACE ( 'NONE', #37048, 10.00000000000010658 ) ;
#18611=CARTESIAN_POINT ( 'NONE',  ( 207.3943894158706485, 271.4293756574240888, 4.935128030509036812 ) ) ;
#18613=CARTESIAN_POINT ( 'NONE',  ( 7.429509195272512301, 163.5494855054051868, -2.679491924311248496 ) ) ;
#18615=CARTESIAN_POINT ( 'NONE',  ( 166.1440757875318468, 253.4574300428235176, -13.57559907896235707 ) ) ;
#18618=B_SPLINE_CURVE_WITH_KNOTS ( 'NONE', 3,
 ( #32038, #10264, #655, #71074 ),
 .UNSPECIFIED., .F., .F.,
 ( 4, 4 ),
 ( 0.01369033625325341563, 0.02232895555845127236 ),
 .UNSPECIFIED. ) ;
#18619=CARTESIAN_POINT ( 'NONE',  ( 46.20988612576196175, 206.6744531367911009, 4.594050593750047540 ) ) ;
#18620=DIRECTION ( 'NONE',  ( 0.4999999999999998890, -0.8660254037844385966, 0.000000000000000000 ) ) ;
#18621=CARTESIAN_POINT ( 'NONE',  ( 85.53328598605538957, 214.0643266524159856, -9.188101187500093303 ) ) ;
#18622=CARTESIAN_POINT ( 'NONE',  ( 207.4541616930702617, 271.3258470364304458, -6.834942797545373594 ) ) ;
#18625=CARTESIAN_POINT ( 'NONE',  ( 163.2099281326308073, 258.2947298600615227, 16.26832179941359158 ) ) ;
#18627=FACE_OUTER_BOUND ( 'NONE', #86251, .T. ) ;
#18628=CARTESIAN_POINT ( 'NONE',  ( 176.7395174816466579, 270.1897220922618317, -16.92019873687963738 ) ) ;
#18631=CARTESIAN_POINT ( 'NONE',  ( -1.439292958244568821, 176.6427522451419065, 10.00000000000009415 ) ) ;
#18633=CARTESIAN_POINT ( 'NONE',  ( 76.00665944866153723, 220.8149278399160664, 9.188101187500093303 ) ) ;
#18635=CARTESIAN_POINT ( 'NONE',  ( 198.9721957120447655, 281.0613474150461570, 17.36564602955951386 ) ) ;
#18637=CARTESIAN_POINT ( 'NONE',  ( 153.6273456746711759, 264.5566271899593858, 16.53755489349362051 ) ) ;
#18640=CARTESIAN_POINT ( 'NONE',  ( 189.9423737135788031, 286.7344497837455037, 16.91658226365147755 ) ) ;
#18642=CARTESIAN_POINT ( 'NONE',  ( 129.9981042655041392, 235.8615022471901739, 5.000000000000051514 ) ) ;
#18643=CARTESIAN_POINT ( 'NONE',  ( 157.8239779013331372, 257.2878469527003062, -17.92251383114021479 ) ) ;
#18646=CARTESIAN_POINT ( 'NONE',  ( 168.9664584017443190, 248.6242280028398000, -1.894951047014129752 ) ) ;
#18648=CARTESIAN_POINT ( 'NONE',  ( 202.7599932440484451, 279.4563852894229967, 15.58249343055423353 ) ) ;
#18649=CARTESIAN_POINT ( 'NONE',  ( 207.1609884636329184, 269.8336379652346295, -0.06011041530970540059 ) ) ;
#18650=CARTESIAN_POINT ( 'NONE',  ( 149.8778024318413316, 271.4674628212321750, -11.84461879799805750 ) ) ;
#18651=ADVANCED_FACE ( 'NONE', ( #23176 ), #32383, .F. ) ;
#18652=ORIENTED_EDGE ( 'NONE', *, *, #28093, .F. ) ;
#18653=CARTESIAN_POINT ( 'NONE',  ( 173.8149039564748648, 250.7382744391995004, 0.4725378802161041558 ) ) ;
#18654=ORIENTED_EDGE ( 'NONE', *, *, #20721, .T. ) ;
#18656=CARTESIAN_POINT ( 'NONE',  ( 167.5081569794162135, 288.0162707042766783, 1.593351152410132698 ) ) ;
#18657=CARTESIAN_POINT ( 'NONE',  ( 193.9195169834368073, 280.6179910428906510, -17.69857902634443292 ) ) ;
#18658=CARTESIAN_POINT ( 'NONE',  ( 192.1486163249491312, 296.6222505933895377, -11.73513860937963571 ) ) ;
#18667=CARTESIAN_POINT ( 'NONE',  ( 198.2831132362969413, 286.4402291352642465, 17.17725333493805095 ) ) ;
#18668=CARTESIAN_POINT ( 'NONE',  ( 163.7729086741176161, 246.9839966035275438, 6.099406794390714204 ) ) ;
#18669=CARTESIAN_POINT ( 'NONE',  ( 148.3025927079438304, 273.7793698660844939, -8.046026357031887954 ) ) ;
#18670=CARTESIAN_POINT ( 'NONE',  ( 186.8123841630082040, 258.3999256946553942, 3.104652050626591553 ) ) ;
#18671=FACE_OUTER_BOUND ( 'NONE', #74142, .T. ) ;
#18672=CARTESIAN_POINT ( 'NONE',  ( 205.2121761402296443, 275.2090799237855094, -14.05269615702442465 ) ) ;
#18673=CARTESIAN_POINT ( 'NONE',  ( 207.8174097099488620, 270.6966830154477748, -3.591979512285951692 ) ) ;
#18674=CARTESIAN_POINT ( 'NONE',  ( 166.0516328627014104, 265.6217384291983876, 16.61431992032753868 ) ) ;
#18676=CARTESIAN_POINT ( 'NONE',  ( 98.90203251333015544, 240.1589784336661637, -6.496448406907675876E-16 ) ) ;
#18677=VERTEX_POINT ( 'NONE', #72822 ) ;
#18678=CARTESIAN_POINT ( 'NONE',  ( 150.1524654112955659, 271.3963926634256723, 12.33079788649884456 ) ) ;
#18679=CARTESIAN_POINT ( 'NONE',  ( 164.5817713503295181, 277.0414339631335565, -13.52591915174977366 ) ) ;
#18680=VERTEX_POINT ( 'NONE', #3415 ) ;
#18683=CARTESIAN_POINT ( 'NONE',  ( 28.65277809448527080, 198.8967562850347122, -4.648177544792955347E-16 ) ) ;
#18685=CARTESIAN_POINT ( 'NONE',  ( 206.1405152101578437, 273.6011494880188479, -9.618815605734603480 ) ) ;
#18686=CARTESIAN_POINT ( 'NONE',  ( 206.8073682671177664, 270.4461261121818438, -4.970999383176901709 ) ) ;
#18687=CARTESIAN_POINT ( 'NONE',  ( 98.52366704282199805, 221.5643266524159856, -9.188101187500093303 ) ) ;
#18688=ORIENTED_EDGE ( 'NONE', *, *, #26842, .T. ) ;
#18695=CARTESIAN_POINT ( 'NONE',  ( 154.1034206470755805, 265.3711135606169478, 16.96274506973287544 ) ) ;
#18696=EDGE_CURVE ( 'NONE', #99795, #71782, #23542, .T. ) ;
#18698=CARTESIAN_POINT ( 'NONE',  ( 129.0235653626489238, 254.4869531367911577, 4.594050593750046652 ) ) ;
#18703=CARTESIAN_POINT ( 'NONE',  ( 156.8296764551412537, 259.0100275755436883, 18.25869368615038013 ) ) ;
#18706=CARTESIAN_POINT ( 'NONE',  ( 188.8869121454080755, 269.5302090799899020, 14.83494772155178332 ) ) ;
#18707=CARTESIAN_POINT ( 'NONE',  ( 188.7930588916510999, 290.9633865388665299, 14.97457979531618832 ) ) ;
#18711=CARTESIAN_POINT ( 'NONE',  ( 203.0105432934428507, 277.9143972074624571, -15.01251885043221002 ) ) ;
#18712=CARTESIAN_POINT ( 'NONE',  ( 161.6673510627899191, 250.6309293646106653, 13.01175935005004192 ) ) ;
#18716=CARTESIAN_POINT ( 'NONE',  ( 175.7882114856885210, 291.4026636951798537, -6.622811550496607857 ) ) ;
#18725=CARTESIAN_POINT ( 'NONE',  ( 203.2732885619977026, 278.5673317194472247, -16.64305493556850024 ) ) ;
#18726=CARTESIAN_POINT ( 'NONE',  ( 180.4323844735881437, 272.9924779018138565, 16.99013570338881252 ) ) ;
#18729=CARTESIAN_POINT ( 'NONE',  ( 205.9915890110450505, 273.4897725707952532, -9.552466559589154471 ) ) ;
#18730=CARTESIAN_POINT ( 'NONE',  ( 16.57566611395445477, 186.5024278399161233, 9.188101187500095079 ) ) ;
#18731=LINE ( 'NONE', #70937, #33912 ) ;
#18734=CARTESIAN_POINT ( 'NONE',  ( 206.1585898378126274, 271.5698433145930721, 8.212139725584252758 ) ) ;
#18735=CARTESIAN_POINT ( 'NONE',  ( 208.2555382576270233, 269.9378221106229034, 3.215405476967123199 ) ) ;
#18737=CARTESIAN_POINT ( 'NONE',  ( 32.46173284068399312, 198.7369531367911293, -4.594050593750048428 ) ) ;
#18739=CARTESIAN_POINT ( 'NONE',  ( 190.1813752874636805, 301.2431906792259042, -4.710625539811892359 ) ) ;
#18741=CARTESIAN_POINT ( 'NONE',  ( 181.7166236227738239, 294.4692410469801302, 6.427997548790919780 ) ) ;
#18744=CARTESIAN_POINT ( 'NONE',  ( 148.9739782091477309, 272.6164960665341823, 12.45483701539941457 ) ) ;
#18745=CARTESIAN_POINT ( 'NONE',  ( 179.6158688349506463, 278.5679919970204423, -16.38266072639121518 ) ) ;
#18751=AXIS2_PLACEMENT_3D ( 'NONE', #81060, #98600, #29182 ) ;
#18752=CARTESIAN_POINT ( 'NONE',  ( 94.05805000844996755, 215.1115022471902023, -5.000000000000041744 ) ) ;
#18754=CARTESIAN_POINT ( 'NONE',  ( 161.9062657679373842, 267.9766905929743643, -17.48695504021573655 ) ) ;
#18755=CARTESIAN_POINT ( 'NONE',  ( 46.91405240998433612, 188.7048013555409796, 4.594050593750051981 ) ) ;
#18758=CARTESIAN_POINT ( 'NONE',  ( 150.7133245577828689, 269.6038598187387834, -14.58664962216439598 ) ) ;
#18759=CARTESIAN_POINT ( 'NONE',  ( 181.9559929377375056, 291.6402902057536721, -11.43735378946719372 ) ) ;
#18760=EDGE_CURVE ( 'NONE', #33613, #82781, #82783, .T. ) ;
#18762=CARTESIAN_POINT ( 'NONE',  ( 170.9671437369523517, 287.2122471754595949, 8.607527358884711433 ) ) ;
#18763=CARTESIAN_POINT ( 'NONE',  ( 207.4826643481121664, 271.2764789897469768, 7.783310782367018454 ) ) ;
#18764=B_SPLINE_CURVE_WITH_KNOTS ( 'NONE', 3,
 ( #84526, #38870, #45959, #60660 ),
 .UNSPECIFIED., .F., .F.,
 ( 4, 4 ),
 ( 0.008512387967132429428, 0.01362662226579259422 ),
 .UNSPECIFIED. ) ;
#18765=CARTESIAN_POINT ( 'NONE',  ( 167.0271109968743417, 287.8086958075197686, 0.5416428030073258126 ) ) ;
#18767=CARTESIAN_POINT ( 'NONE',  ( 189.7194741408086429, 264.5021160184427913, 10.84982732454233911 ) ) ;
#18769=CARTESIAN_POINT ( 'NONE',  ( 204.4345574087956550, 276.5559550755466489, 14.49589339982634861 ) ) ;
#18770=ORIENTED_EDGE ( 'NONE', *, *, #3999, .T. ) ;
#18772=EDGE_CURVE ( 'NONE', #13470, #83200, #75639, .T. ) ;
#18773=CARTESIAN_POINT ( 'NONE',  ( 172.2368248080031492, 252.4453057155697877, 8.861972572817373717 ) ) ;
#18776=EDGE_LOOP ( 'NONE', ( #89628, #69350, #95942 ) ) ;
#18777=CARTESIAN_POINT ( 'NONE',  ( 179.2225705765399084, 282.9028557827877535, 16.02728324287294370 ) ) ;
#18778=CARTESIAN_POINT ( 'NONE',  ( 191.5544531425776427, 298.8649500714207647, 8.366689293739112188 ) ) ;
#18780=DIRECTION ( 'NONE',  ( 0.4999999999999998890, -0.8660254037844385966, 0.000000000000000000 ) ) ;
#18781=ORIENTED_EDGE ( 'NONE', *, *, #77601, .F. ) ;
#18782=ORIENTED_EDGE ( 'NONE', *, *, #45353, .F. ) ;
#18783=CARTESIAN_POINT ( 'NONE',  ( 207.5462191418491500, 271.1663988579299485, -5.239401497773396699 ) ) ;
#18784=CARTESIAN_POINT ( 'NONE',  ( -22.42236680055709641, 157.8615022471902591, 0.000000000000000000 ) ) ;
#18785=CARTESIAN_POINT ( 'NONE',  ( 149.2765980486851731, 272.0923431290771646, -11.40617906909507973 ) ) ;
#18788=CARTESIAN_POINT ( 'NONE',  ( 198.2819808855875863, 287.2125302111982705, 18.53535247371401695 ) ) ;
#18791=CARTESIAN_POINT ( 'NONE',  ( 157.2104826425669728, 258.3504519110855995, -16.92635148710569482 ) ) ;
#18792=CARTESIAN_POINT ( 'NONE',  ( 118.1714448432989144, 239.0333772461660544, 9.188101187500095079 ) ) ;
#18795=CARTESIAN_POINT ( 'NONE',  ( 164.1821508476733698, 246.2751683663292397, -7.347745041495428175 ) ) ;
#18796=ORIENTED_EDGE ( 'NONE', *, *, #50025, .T. ) ;
#18800=CARTESIAN_POINT ( 'NONE',  ( 63.96340690334295687, 216.9244531367911293, -4.594050593750046652 ) ) ;
#18802=CARTESIAN_POINT ( 'NONE',  ( 150.8359915840788688, 269.3913942967808453, 15.73449616766854575 ) ) ;
#18803=CARTESIAN_POINT ( 'NONE',  ( 150.8613910702043768, 269.3474010963252567, 15.19517615056406612 ) ) ;
#18804=AXIS2_PLACEMENT_3D ( 'NONE', #58676, #19721, #58193 ) ;
#18808=CARTESIAN_POINT ( 'NONE',  ( 191.2649737798357705, 297.3663430354321235, 11.06343876070684296 ) ) ;
#18810=CARTESIAN_POINT ( 'NONE',  ( 172.2332593386741735, 258.4530275332109568, -14.26710149980596576 ) ) ;
#18814=CARTESIAN_POINT ( 'NONE',  ( 148.9517569034208009, 272.6549844970639924, 12.50737104496728236 ) ) ;
#18815=CARTESIAN_POINT ( 'NONE',  ( 180.7461886851734789, 271.3453486839773063, 16.63588864205645379 ) ) ;
#18819=CARTESIAN_POINT ( 'NONE',  ( 164.2695167311736668, 253.9159192467835169, 14.61855453912878211 ) ) ;
#18821=CARTESIAN_POINT ( 'NONE',  ( 164.3890147726454813, 245.9168695380243435, -6.010262808998044548 ) ) ;
#18822=CARTESIAN_POINT ( 'NONE',  ( 117.9006383567337792, 245.0024278399160949, 9.188101187500095079 ) ) ;
#18824=VECTOR ( 'NONE', #58652, 999.9999999999998863 ) ;
#18828=EDGE_CURVE ( 'NONE', #90614, #4734, #52467, .T. ) ;
#18829=CARTESIAN_POINT ( 'NONE',  ( 155.5066938333533528, 261.3015006940112244, -18.40036130547566273 ) ) ;
#18831=CARTESIAN_POINT ( 'NONE',  ( 204.9103773355753617, 275.7318107871104189, 13.62808820451859937 ) ) ;
#18833=CARTESIAN_POINT ( 'NONE',  ( 178.0467360553784033, 255.3817929127459934, 4.775061655386900306 ) ) ;
#18834=ORIENTED_EDGE ( 'NONE', *, *, #66450, .F. ) ;
#18837=CARTESIAN_POINT ( 'NONE',  ( 158.5141842721128285, 275.0039168403922645, -12.51588967219915816 ) ) ;
#18840=CARTESIAN_POINT ( 'NONE',  ( 164.4306612431381325, 245.8447357351751066, -2.314684942147286595 ) ) ;
#18841=CARTESIAN_POINT ( 'NONE',  ( 142.5284093247362591, 253.0958772461660544, -9.188101187500095079 ) ) ;
#18843=CARTESIAN_POINT ( 'NONE',  ( 189.0276693039769498, 300.1137990693615620, -3.525949465148791262 ) ) ;
#18844=LINE ( 'NONE', #19838, #7703 ) ;
#18845=CARTESIAN_POINT ( 'NONE',  ( 150.5438776023515004, 278.3016033182416322, -9.804454847755098641E-05 ) ) ;
#18846=CARTESIAN_POINT ( 'NONE',  ( 72.21814540286966633, 206.3768266524159856, -9.188101187500091527 ) ) ;
#18847=CARTESIAN_POINT ( 'NONE',  ( 157.8429099974857195, 257.2550556002704525, -17.85752049034686095 ) ) ;
#18848=CARTESIAN_POINT ( 'NONE',  ( 174.6639587582037620, 252.0453782210719282, 3.541528378334539262 ) ) ;
#18852=CARTESIAN_POINT ( 'NONE',  ( 190.6661865267473104, 300.4034729807058852, 4.523489664447863490 ) ) ;
#18853=CARTESIAN_POINT ( 'NONE',  ( 155.3925584512507498, 279.7696002511819415, -1.290171526702664995 ) ) ;
#18854=CARTESIAN_POINT ( 'NONE',  ( 172.5626239099614168, 287.5492475841473379, -8.221891676024617013 ) ) ;
#18855=CARTESIAN_POINT ( 'NONE',  ( 203.0026270830780675, 279.0361311525880978, -16.61345826058821373 ) ) ;
#18856=CARTESIAN_POINT ( 'NONE',  ( 193.5438442197551296, 288.5803156727525902, 16.04593160988459033 ) ) ;
#18857=CARTESIAN_POINT ( 'NONE',  ( 126.8046355855010603, 254.0177522451418781, 5.000000000000046185 ) ) ;
#18860=CARTESIAN_POINT ( 'NONE',  ( 157.8092552871339365, 257.3133472685137235, 17.04082256169242626 ) ) ;
#18861=CARTESIAN_POINT ( 'NONE',  ( 158.8266160086023149, 257.5512268093053194, -17.29683829744028856 ) ) ;
#18862=CARTESIAN_POINT ( 'NONE',  ( -5.724140937729832679, 161.3768266524159856, -9.188101187500093303 ) ) ;
#18864=CARTESIAN_POINT ( 'NONE',  ( 45.07374842694240868, 187.6423013555410080, -4.594050593750043987 ) ) ;
#18865=CARTESIAN_POINT ( 'NONE',  ( 175.3888197414261185, 256.6087255675022902, -10.77910597738013898 ) ) ;
#18868=CARTESIAN_POINT ( 'NONE',  ( 157.8429099974857195, 257.2550556002704525, -17.85752049034686095 ) ) ;
#18869=CARTESIAN_POINT ( 'NONE',  ( 192.0603001030472683, 293.3461588932823929, -14.68827779892621344 ) ) ;
#18870=CARTESIAN_POINT ( 'NONE',  ( 190.6954410837624607, 300.3528026016029457, -5.728531842148099962 ) ) ;
#18872=EDGE_CURVE ( 'NONE', #59884, #49538, #7765, .T. ) ;
#18873=CARTESIAN_POINT ( 'NONE',  ( 67.04888272437477781, 219.5177522451419065, 5.000000000000046185 ) ) ;
#18874=CARTESIAN_POINT ( 'NONE',  ( 47.20246722098136871, 211.3927522451419350, 2.944929066748280225E-16 ) ) ;
#18875=CARTESIAN_POINT ( 'NONE',  ( 181.3255421082058376, 255.3544676688379127, 2.128643196724650632 ) ) ;
#18876=CARTESIAN_POINT ( 'NONE',  ( 205.2391015854675516, 275.1624436846170738, -14.01434138479280911 ) ) ;
#18880=CARTESIAN_POINT ( 'NONE',  ( 161.7323330629232316, 267.3777249680341015, 16.49771666234070366 ) ) ;
#18881=CARTESIAN_POINT ( 'NONE',  ( 53.71569994882487009, 188.4865022471901455, 1.119607411625061291E-15 ) ) ;
#18882=CARTESIAN_POINT ( 'NONE',  ( 183.4669127592752034, 292.6857018627941898, 9.408060097649215692 ) ) ;
#18884=CARTESIAN_POINT ( 'NONE',  ( -2.963858511049441979, 169.0958772461660544, -9.188101187500095079 ) ) ;
#18887=CARTESIAN_POINT ( 'NONE',  ( 30.74798454907712042, 181.8927522451418497, 10.00000000000009948 ) ) ;
#18889=CARTESIAN_POINT ( 'NONE',  ( 165.0020474182383339, 244.8550658491588479, 1.825383354618924425 ) ) ;
#18890=CARTESIAN_POINT ( 'NONE',  ( 182.6449127974795203, 278.5736680211113594, 16.63823239613948601 ) ) ;
#18892=DIRECTION ( 'NONE',  ( -0.8660254037844387076, -0.4999999999999998890, -0.000000000000000000 ) ) ;
#18894=CARTESIAN_POINT ( 'NONE',  ( 176.5378754974050821, 260.2610757822269534, -13.57310438010597586 ) ) ;
#18897=CARTESIAN_POINT ( 'NONE',  ( 153.2955602623325149, 277.6818314479798460, -5.275435393451455290 ) ) ;
#18899=CARTESIAN_POINT ( 'NONE',  ( 158.3828892404620490, 259.0189987438004096, 16.74082065088548177 ) ) ;
#18900=EDGE_CURVE ( 'NONE', #54972, #16763, #12632, .T. ) ;
#18901=CARTESIAN_POINT ( 'NONE',  ( 193.7999837595647250, 294.9755769528473479, 15.24609078262870199 ) ) ;
#18905=CARTESIAN_POINT ( 'NONE',  ( 206.1405152101578437, 273.6011494880188479, -9.618815605734603480 ) ) ;
#18908=CARTESIAN_POINT ( 'NONE',  ( 164.7243055739305078, 245.3361288348881999, -1.445094907380085170 ) ) ;
#18909=VECTOR ( 'NONE', #10012, 1000.000000000000000 ) ;
#18910=B_SPLINE_CURVE_WITH_KNOTS ( 'NONE', 3,
 ( #75822, #38274, #21609, #5900, #100115, #30700, #52489, #84927, #37291, #37781, #76317, #60575, #291, #91531, #99615, #30193, #61079, #15473, #67703, #52992, #14003, #98630, #6409, #16488, #40768, #33192, #17491, #71212, #87475, #18009, #70177, #39267, #85442, #48397 ),
 .UNSPECIFIED., .F., .F.,
 ( 4, 2, 2, 2, 2, 2, 2, 2, 2, 2, 2, 2, 2, 2, 2, 2, 4 ),
 ( 0.003332772792290249371, 0.003484938153222827580, 0.003637103514155405788, 0.003713186194621726551, 0.003789268875088047314, 0.003941434236020691442, 0.004245764957886018730, 0.004550095679751345150, 0.005158757123481937275, 0.005767418567212528532, 0.006984741454673737068, 0.007593402898404376031, 0.007897733620269692043, 0.008049898981202348314, 0.008125981661668640887, 0.008164023001901790644, 0.008202064342134938665 ),
 .UNSPECIFIED. ) ;
#18915=CARTESIAN_POINT ( 'NONE',  ( 159.6998082543438500, 278.4571990200508935, -9.779246870798463220 ) ) ;
#18916=CARTESIAN_POINT ( 'NONE',  ( 63.51261232558832859, 214.1427522451419350, 10.00000000000009415 ) ) ;
#18920=CARTESIAN_POINT ( 'NONE',  ( 199.0746189151364831, 265.2438329385483939, 1.559867394473611002 ) ) ;
#18924=B_SPLINE_CURVE_WITH_KNOTS ( 'NONE', 3,
 ( #98568, #62004, #92955, #60022, #23508, #86893, #8825, #24023, #40715, #24524, #33129, #54921, #62502, #47319, #94466, #33645, #85899, #16424 ),
 .UNSPECIFIED., .F., .F.,
 ( 4, 2, 2, 2, 2, 2, 2, 2, 4 ),
 ( 6.399695615700000250E-17, 0.0002914903321845351307, 0.0005829806643690061850, 0.0008744709965534773477, 0.001165961328737948402, 0.001457451660922419456, 0.001748941993106890727, 0.002040432325291361999, 0.002331922657475833053 ),
 .UNSPECIFIED. ) ;
#18926=ORIENTED_EDGE ( 'NONE', *, *, #20845, .F. ) ;
#18927=CARTESIAN_POINT ( 'NONE',  ( 174.8111530639320108, 267.9940263390942619, 16.29984105809692707 ) ) ;
#18928=CARTESIAN_POINT ( 'NONE',  ( 166.1857273590558179, 273.8697761094379644, -16.44210238554618897 ) ) ;
#18930=EDGE_LOOP ( 'NONE', ( #38992, #72664 ) ) ;
#18931=DIRECTION ( 'NONE',  ( 0.4999999999999992784, -0.8660254037844390407, 0.000000000000000000 ) ) ;
#18932=CARTESIAN_POINT ( 'NONE',  ( 163.1332433029523372, 248.0919295262283981, 11.24052392390482957 ) ) ;
#18933=ORIENTED_EDGE ( 'NONE', *, *, #36758, .T. ) ;
#18935=ORIENTED_EDGE ( 'NONE', *, *, #85133, .F. ) ;
#18936=CARTESIAN_POINT ( 'NONE',  ( 157.5954339963122663, 268.8483900235063402, 15.63267351098963154 ) ) ;
#18939=B_SPLINE_CURVE_WITH_KNOTS ( 'NONE', 3,
 ( #79682, #10244, #60786, #75532, #20844, #75042, #76045, #43614, #98339, #90775, #90273, #30415, #45598, #91751, #20337, #28932, #99829, #52206, #60292, #51737, #5129, #22314, #29421, #51210, #59806, #21326, #82175, #83154, #37012, #13721, #12751, #13244, #28413, #89767, #29916, #44597, #6626, #98842, #59292, #74553, #36012, #53217, #66914, #6116, #67921, #91251, #21815, #84168, #37992, #7109 ),
 .UNSPECIFIED., .F., .F.,
 ( 4, 2, 2, 2, 2, 2, 2, 2, 2, 2, 2, 2, 2, 2, 2, 2, 2, 2, 2, 2, 2, 2, 2, 2, 4 ),
 ( 0.001915670005683367365, 0.002365191695059523820, 0.002589952539747623732, 0.002814713384435723210, 0.002927093806779732400, 0.003039474229123741589, 0.003151854651467750346, 0.003264235073811759969, 0.003488995918499739751, 0.003713756763187719100, 0.004163278452563567641, 0.004612800141939415316, 0.005511843520691112400, 0.006410886899442808616, 0.006860408588818692720, 0.007309930278194576823, 0.007422310700538548717, 0.007478500911710535097, 0.007534691122882520610, 0.007647071545226449135, 0.007759451967570377660, 0.008208973656945820277, 0.008658495346321262026, 0.008883256191009034075, 0.009108017035696806124 ),
 .UNSPECIFIED. ) ;
#18940=CARTESIAN_POINT ( 'NONE',  ( 147.3627346024176461, 275.4072518567613201, 7.337996838423670454 ) ) ;
#18941=DIRECTION ( 'NONE',  ( 0.4999999999999992784, -0.8660254037844390407, 0.000000000000000000 ) ) ;
#18943=CARTESIAN_POINT ( 'NONE',  ( 193.6023084030469761, 294.8553025941217243, 13.33578009685492560 ) ) ;
#18944=CARTESIAN_POINT ( 'NONE',  ( 178.5465195133704981, 291.5681621643464041, 6.587540641832299038 ) ) ;
#18945=CARTESIAN_POINT ( 'NONE',  ( 197.4356762619225663, 288.6783728180664070, -16.68343683487013962 ) ) ;
#18950=CARTESIAN_POINT ( 'NONE',  ( 165.0020474182383339, 244.8550658491588479, 1.825383354618924425 ) ) ;
#18951=CARTESIAN_POINT ( 'NONE',  ( 198.6742831389107096, 286.5330427765190393, 17.60232614297041565 ) ) ;
#18955=CARTESIAN_POINT ( 'NONE',  ( 190.8281514355135187, 300.1229415296796788, 6.778607853984104814 ) ) ;
#18956=CARTESIAN_POINT ( 'NONE',  ( 171.5651214720799373, 259.5975988575258953, -15.07810809630464099 ) ) ;
#18957=CARTESIAN_POINT ( 'NONE',  ( 163.9564365344733687, 247.8982689250301235, 8.517658320392268223 ) ) ;
#18959=B_SPLINE_CURVE_WITH_KNOTS ( 'NONE', 3,
 ( #54165, #69390, #67901, #98821 ),
 .UNSPECIFIED., .F., .F.,
 ( 4, 4 ),
 ( 0.000000000000000000, 0.005725910648720425322 ),
 .UNSPECIFIED. ) ;
#18960=CARTESIAN_POINT ( 'NONE',  ( 47.74604483422196921, 186.8262482093457777, 3.021315404115420679E-15 ) ) ;
#18961=CARTESIAN_POINT ( 'NONE',  ( 148.7072594763547215, 273.0784664630622274, -9.449416077291342475 ) ) ;
#18966=CARTESIAN_POINT ( 'NONE',  ( 47.13029843733273339, 198.0177522451418781, -10.00000000000009592 ) ) ;
#18968=CARTESIAN_POINT ( 'NONE',  ( 196.4287751515431921, 269.1031666285815618, -12.09581130873691279 ) ) ;
#18969=CARTESIAN_POINT ( 'NONE',  ( 34.06774859691741142, 197.1427522451419350, -10.00000000000009415 ) ) ;
#18970=CARTESIAN_POINT ( 'NONE',  ( 102.6097905472235539, 239.2369531367911009, -4.594050593750048428 ) ) ;
#18972=CARTESIAN_POINT ( 'NONE',  ( 181.3921258689275646, 294.4728088502279775, -2.647902565978816014 ) ) ;
#18973=B_SPLINE_CURVE_WITH_KNOTS ( 'NONE', 3,
 ( #52690, #83651, #14210, #76992, #46583, #38986, #15, #45588, #76514, #46081, #6614, #37979, #84157, #76036, #30900, #7098, #60775, #7599, #30400, #37487, #68397, #31392, #86165, #38486, #61788, #16201, #39471, #91739, #503, #47093, #68890, #69400, #99323, #14703, #29902, #92734, #92256, #99817, #84640, #61292, #8112, #22805, #53683, #22302, #53202, #78014, #8605, #15180 ),
 .UNSPECIFIED., .F., .F.,
 ( 4, 2, 2, 2, 2, 2, 2, 2, 2, 2, 2, 2, 2, 2, 2, 2, 2, 2, 2, 2, 2, 2, 2, 4 ),
 ( 0.0006084983335041455922, 0.001036156343644727140, 0.001249985348714947007, 0.001356899851249977144, 0.001463814353785007280, 0.001677643358855142146, 0.001891472363925276795, 0.002319130374065546743, 0.003174446394346166437, 0.004029762414626786998, 0.004885078434907406258, 0.005312736445047754053, 0.005526565450117964379, 0.005633479952653145870, 0.005686937203920737482, 0.005740394455188327361, 0.005793851706455918973, 0.005847308957723510586, 0.005954223460258693812, 0.006168052465329072406, 0.006595710475469845208, 0.007023368485610619744, 0.007237197490680984460, 0.007451026495751349177 ),
 .UNSPECIFIED. ) ;
#18975=CARTESIAN_POINT ( 'NONE',  ( 162.4419666585835387, 249.2892557963607203, 10.75794555938079711 ) ) ;
#18976=CARTESIAN_POINT ( 'NONE',  ( 14.70821206310299978, 188.4869531367911293, 4.594050593750046652 ) ) ;
#18977=CARTESIAN_POINT ( 'NONE',  ( 161.6707029936031574, 250.6251236501384483, 14.45053103226186231 ) ) ;
#18980=VERTEX_POINT ( 'NONE', #33546 ) ;
#18981=CARTESIAN_POINT ( 'NONE',  ( 185.1894006957831778, 259.9970902747327841, -5.780845478426857476 ) ) ;
#18982=ADVANCED_FACE ( 'NONE', ( #79687 ), #13725, .T. ) ;
#18985=CARTESIAN_POINT ( 'NONE',  ( 190.2510882691990730, 301.1224442529128851, -5.480893437181090455 ) ) ;
#18986=CARTESIAN_POINT ( 'NONE',  ( 192.9730208252800594, 263.8306068669091360, -4.263488463504454096 ) ) ;
#18987=CARTESIAN_POINT ( 'NONE',  ( 161.6923300915171922, 250.5876644177310482, -14.43081872899884566 ) ) ;
#18988=CARTESIAN_POINT ( 'NONE',  ( 185.8754509513723576, 286.6007344811247890, 15.75805532497020423 ) ) ;
#18989=CARTESIAN_POINT ( 'NONE',  ( 99.88567928453475986, 235.1427522451419065, 10.00000000000009415 ) ) ;
#18990=CARTESIAN_POINT ( 'NONE',  ( 49.32242524243604720, 199.2833772461660828, -9.188101187500095079 ) ) ;
#18991=CARTESIAN_POINT ( 'NONE',  ( 79.10106959370823176, 223.1427522451419065, 10.00000000000009237 ) ) ;
#18992=ORIENTED_EDGE ( 'NONE', *, *, #25243, .F. ) ;
#18994=CARTESIAN_POINT ( 'NONE',  ( 158.0503757190722354, 282.4476557944344108, -1.686668573986806585 ) ) ;
#18995=CARTESIAN_POINT ( 'NONE',  ( -3.667330603741788320, 162.5643266524160140, 9.188101187500095079 ) ) ;
#18996=B_SPLINE_CURVE_WITH_KNOTS ( 'NONE', 3,
 ( #54341, #70561, #99990, #60957, #61459, #91916, #23958, #99490, #85839, #38663, #69566, #9275, #173, #31057, #92898, #8275, #47260, #78181, #84806, #8770, #76674, #22471, #14862, #53365, #84315, #45749, #92409, #39639, #15346, #32052, #62964, #77692, #78686, #7261, #38144, #85313, #15859, #93914, #22957, #39140, #46766, #668, #86325, #16862, #53846, #46242 ),
 .UNSPECIFIED., .F., .F.,
 ( 4, 2, 2, 2, 2, 2, 2, 2, 2, 2, 2, 2, 2, 2, 2, 2, 2, 2, 2, 2, 2, 2, 4 ),
 ( 0.002366943055100816529, 0.002788261558867141145, 0.002998920810750290225, 0.003104250436691864332, 0.003209580062633438872, 0.003314909688575013412, 0.003420239314516587952, 0.003630898566399730527, 0.004052217070165960167, 0.004894854077698489701, 0.005737491085231020971, 0.006580128092763551373, 0.007001446596529816574, 0.007422765100296080040, 0.007528094726237586493, 0.007580759539208290279, 0.007633424352178995800, 0.007686089165149699587, 0.007738753978120403373, 0.007844083604061628801, 0.008265402107826599898, 0.008686720611591570995, 0.009108039115356540358 ),
 .UNSPECIFIED. ) ;
#18998=CARTESIAN_POINT ( 'NONE',  ( 199.0773057068961123, 285.8349872121713702, -17.17316764978006560 ) ) ;
#19000=CARTESIAN_POINT ( 'NONE',  ( 192.8607783413999073, 296.6023284558532396, -11.80574095728561446 ) ) ;
#19002=CARTESIAN_POINT ( 'NONE',  ( 164.1224127655298730, 246.3786377597482158, 7.356982420601481998 ) ) ;
#19003=CARTESIAN_POINT ( 'NONE',  ( 191.6823192895500370, 298.6434794082964572, -8.424208857102787107 ) ) ;
#19004=CARTESIAN_POINT ( 'NONE',  ( 164.4440639631384045, 245.8215215431751233, -2.910115319305802029 ) ) ;
#19006=B_SPLINE_CURVE_WITH_KNOTS ( 'NONE', 3,
 ( #29740, #62613, #22641, #60614 ),
 .UNSPECIFIED., .F., .F.,
 ( 4, 4 ),
 ( 2.422837424025932118E-15, 0.002968769119667788274 ),
 .UNSPECIFIED. ) ;
#19007=EDGE_CURVE ( 'NONE', #64907, #86118, #43618, .T. ) ;
#19008=CARTESIAN_POINT ( 'NONE',  ( 208.0692320075777957, 270.2605140014760536, 2.043861372130216569 ) ) ;
#19009=CARTESIAN_POINT ( 'NONE',  ( -1.637757109730603178, 179.8615022471903444, 5.000000000000046185 ) ) ;
#19011=CARTESIAN_POINT ( 'NONE',  ( 125.2075541532825014, 255.3464784336661353, 1.353441290958777327E-15 ) ) ;
#19014=CARTESIAN_POINT ( 'NONE',  ( 37.53185021205516847, 199.1427522451419065, 10.00000000000009415 ) ) ;
#19016=CARTESIAN_POINT ( 'NONE',  ( 185.7458139929641732, 288.0803647735083928, 14.78940038638959997 ) ) ;
#19020=CARTESIAN_POINT ( 'NONE',  ( 193.9979983253333842, 262.2552985615510579, -0.8131695963413709816 ) ) ;
#19021=CARTESIAN_POINT ( 'NONE',  ( 149.3801359649374092, 271.9130101976182914, -11.41245530317637424 ) ) ;
#19024=CARTESIAN_POINT ( 'NONE',  ( 173.2640678248423569, 289.7688146612205742, -1.079593490584200177 ) ) ;
#19028=CARTESIAN_POINT ( 'NONE',  ( 168.9077028164640240, 271.8916309642168585, -16.88789700254694992 ) ) ;
#19030=B_SPLINE_SURFACE_WITH_KNOTS ( 'NONE', 3, 1, ( 
 ( #56007, #31709 ),
 ( #17023, #25647 ),
 ( #1846, #26143 ),
 ( #47425, #39800 ),
 ( #95083, #94569 ),
 ( #56529, #48438 ),
 ( #62614, #25126 ),
 ( #2864, #33754 ),
 ( #73740, #59000 ),
 ( #49934, #98044 ),
 ( #11463, #42319 ),
 ( #42807, #65133 ),
 ( #10953, #82388 ),
 ( #65626, #66628 ),
 ( #5337, #26640 ),
 ( #66131, #4850 ),
 ( #72771, #89015 ),
 ( #88002, #19060 ),
 ( #80383, #96583 ),
 ( #80895, #73248 ),
 ( #12448, #3842 ),
 ( #81382, #3364 ),
 ( #35229, #50921 ),
 ( #88498, #12957 ),
 ( #49430, #27147 ),
 ( #34727, #41824 ),
 ( #51425, #43316 ),
 ( #58032, #19566 ),
 ( #28622, #50425 ),
 ( #4331, #43819 ),
 ( #74757, #36218 ),
 ( #97559, #81871 ),
 ( #97080, #11949 ),
 ( #67120, #27650 ) ),
 .UNSPECIFIED., .T., .F., .F.,
 ( 4, 2, 2, 2, 2, 2, 2, 2, 2, 2, 2, 2, 2, 2, 2, 2, 4 ),
 ( 2, 2 ),
 ( 0.000000000000000000, 0.06250000000000000000, 0.1250000000000000000, 0.1875000000000000000, 0.2500000000000000000, 0.3125000000000000000, 0.3750000000000000000, 0.4375000000000000000, 0.5000000000000000000, 0.5625000000000000000, 0.6250000000000000000, 0.6875000000000000000, 0.7500000000000000000, 0.8125000000000000000, 0.8750000000000000000, 0.9375000000000000000, 1.000000000000000000 ),
 ( 0.000000000000000000, 1.000000000000000000 ),
 .UNSPECIFIED. ) ;
#19032=CARTESIAN_POINT ( 'NONE',  ( 196.5114978539924095, 270.9775588704130769, 12.02747001956845985 ) ) ;
#19033=CARTESIAN_POINT ( 'NONE',  ( 156.5453005749562294, 261.0928181209063155, 17.61606195476766956 ) ) ;
#19035=CARTESIAN_POINT ( 'NONE',  ( 192.7693357657653053, 296.7607116428271183, 12.22606306887835714 ) ) ;
#19038=CARTESIAN_POINT ( 'NONE',  ( 194.5559179531667553, 283.0183282092541504, 17.56514686992159469 ) ) ;
#19040=CARTESIAN_POINT ( 'NONE',  ( 173.7983950520408882, 272.6079108873909149, -16.38292534526199518 ) ) ;
#19042=CARTESIAN_POINT ( 'NONE',  ( 163.8626652770474266, 279.3816800765269477, 12.16740215884250631 ) ) ;
#19043=CARTESIAN_POINT ( 'NONE',  ( 194.6782745185928434, 293.4543327343926080, -14.56555309295305634 ) ) ;
#19044=CARTESIAN_POINT ( 'NONE',  ( 159.5606259118165724, 264.0648208006689401, -17.79391822139266566 ) ) ;
#19045=ORIENTED_EDGE ( 'NONE', *, *, #12881, .F. ) ;
#19047=CARTESIAN_POINT ( 'NONE',  ( 185.3238942230333919, 291.2129889426717568, 12.00891028115657555 ) ) ;
#19052=CARTESIAN_POINT ( 'NONE',  ( 185.0431258460432957, 259.9412888983961238, -5.848330788044057371 ) ) ;
#19053=ORIENTED_EDGE ( 'NONE', *, *, #80391, .T. ) ;
#19055=CARTESIAN_POINT ( 'NONE',  ( 178.4748507201557004, 260.9579597201419006, 12.09575687999501881 ) ) ;
#19060=CARTESIAN_POINT ( 'NONE',  ( 154.9792334219179679, 262.2150889255981951, -17.21325849938693153 ) ) ;
#19064=CARTESIAN_POINT ( 'NONE',  ( 189.9926605375425481, 301.5700542142271843, 2.240758812287489743 ) ) ;
#19065=CARTESIAN_POINT ( 'NONE',  ( 161.6007233961445309, 277.4982682042578404, -13.28202216465472674 ) ) ;
#19066=CARTESIAN_POINT ( 'NONE',  ( 147.5749551500760788, 275.0396750858066639, -4.254929048021584670 ) ) ;
#19067=CARTESIAN_POINT ( 'NONE',  ( 153.4613150239306094, 264.8442007126561748, -16.86932470306368259 ) ) ;
#19071=CARTESIAN_POINT ( 'NONE',  ( 141.9874905431360332, 240.5327760586659451, 1.948934522072303157E-15 ) ) ;
#19072=ORIENTED_EDGE ( 'NONE', *, *, #26316, .T. ) ;
#19076=CARTESIAN_POINT ( 'NONE',  ( 203.8368721788344544, 271.7098658965333584, 9.656807015386196014 ) ) ;
#19078=CARTESIAN_POINT ( 'NONE',  ( -5.238238056892285499, 179.3297689869269504, -2.679491924311240503 ) ) ;
#19080=CARTESIAN_POINT ( 'NONE',  ( 170.9867886428140196, 287.8958644575130279, -5.368964696424015415 ) ) ;
#19081=CARTESIAN_POINT ( 'NONE',  ( 152.8260228566844603, 277.7352812325914329, 6.769763962897619614 ) ) ;
#19083=CARTESIAN_POINT ( 'NONE',  ( 178.6026051973306323, 254.4708812555809345, 5.813106864979912913 ) ) ;
#19086=ORIENTED_EDGE ( 'NONE', *, *, #26286, .T. ) ;
#19087=CARTESIAN_POINT ( 'NONE',  ( 185.0052077488253417, 273.1271762488819377, -16.58638918698247977 ) ) ;
#19091=CARTESIAN_POINT ( 'NONE',  ( 164.0768433133964095, 278.1026867120588122, 13.25608502235604647 ) ) ;
#19093=CARTESIAN_POINT ( 'NONE',  ( 164.1339789967515514, 246.3586044596203521, -8.192084292517387567 ) ) ;
#19094=CARTESIAN_POINT ( 'NONE',  ( 149.2561433752359505, 272.1277716627430436, 12.99353668144589946 ) ) ;
#19096=CARTESIAN_POINT ( 'NONE',  ( 202.2712651538608668, 280.3028871727136675, 16.13191389836473988 ) ) ;
#19097=CARTESIAN_POINT ( 'NONE',  ( 161.4345289443906779, 281.4097987515496015, -6.805021284559834349 ) ) ;
#19099=DIRECTION ( 'NONE',  ( -0.8660254037844387076, -0.4999999999999998890, -0.000000000000000000 ) ) ;
#19106=CARTESIAN_POINT ( 'NONE',  ( 153.4289928607825573, 264.9001843414388873, 17.27358709529985958 ) ) ;
#19110=CARTESIAN_POINT ( 'NONE',  ( 192.4240881988952196, 286.9807864659827032, 17.27280571159278466 ) ) ;
#19112=CARTESIAN_POINT ( 'NONE',  ( 10.35128207213630169, 176.7833772461660544, -9.188101187500095079 ) ) ;
#19113=CARTESIAN_POINT ( 'NONE',  ( 106.1553423657898492, 232.0958772461660260, -9.188101187500095079 ) ) ;
#19114=CARTESIAN_POINT ( 'NONE',  ( 203.3205561747472814, 278.4854618126124706, -15.14439614831292147 ) ) ;
#19116=CARTESIAN_POINT ( 'NONE',  ( 186.6044737300459246, 296.1965008795603467, -7.321969523639923594 ) ) ;
#19120=CARTESIAN_POINT ( 'NONE',  ( 172.4746793654577743, 290.6488618360747864, 2.762989037780315904 ) ) ;
#19122=CARTESIAN_POINT ( 'NONE',  ( 148.1829914015846157, 273.9865254053503349, -9.304102644963160529 ) ) ;
#19123=CARTESIAN_POINT ( 'NONE',  ( 181.6983192186336566, 291.5179062160608510, 9.337665102737071621 ) ) ;
#19124=CARTESIAN_POINT ( 'NONE',  ( 178.0782606409264304, 276.0678601331425739, -17.70468353419743579 ) ) ;
#19125=CARTESIAN_POINT ( 'NONE',  ( 205.5005536374337112, 274.7095954468686045, -13.54891840104049194 ) ) ;
#19126=CARTESIAN_POINT ( 'NONE',  ( -0.9341114727036623488, 180.2677522451419350, -5.000000000000047962 ) ) ;
#19128=DIRECTION ( 'NONE',  ( -0.4999999999999987232, 0.8660254037844394848, 0.000000000000000000 ) ) ;
#19130=B_SPLINE_CURVE_WITH_KNOTS ( 'NONE', 3,
 ( #59461, #14390, #66592, #59967 ),
 .UNSPECIFIED., .F., .F.,
 ( 4, 4 ),
 ( 0.01142038051278651892, 0.01737621679390735294 ),
 .UNSPECIFIED. ) ;
#19131=CARTESIAN_POINT ( 'NONE',  ( 175.6683667130938034, 265.4573993361621547, -15.76779689782518368 ) ) ;
#19132=CARTESIAN_POINT ( 'NONE',  ( 82.58295308470839302, 227.6744531367911293, 4.594050593750047540 ) ) ;
#19133=CARTESIAN_POINT ( 'NONE',  ( 161.8668411317136986, 250.2854024296290447, -13.43522912998426655 ) ) ;
#19137=CARTESIAN_POINT ( 'NONE',  ( 151.7315266105576939, 267.8402821309618957, 15.96020185843874373 ) ) ;
#19138=FACE_OUTER_BOUND ( 'NONE', #81135, .T. ) ;
#19139=CARTESIAN_POINT ( 'NONE',  ( 176.7306370342185460, 270.1477411634788268, -17.15222723775526603 ) ) ;
#19145=CARTESIAN_POINT ( 'NONE',  ( 77.41429782557628414, 209.3768266524159571, -9.188101187500093303 ) ) ;
#19146=DIRECTION ( 'NONE',  ( -0.8660254037844387076, -0.4999999999999998890, -0.000000000000000000 ) ) ;
#19148=CARTESIAN_POINT ( 'NONE',  ( 191.4405189358380426, 288.5485936597882528, -15.93201744756964722 ) ) ;
#19149=( BOUNDED_CURVE ( )  B_SPLINE_CURVE ( 2, ( #3997, #73660, #40730, #95515, #48865, #86911, #80293, #87923, #26561 ),
 .UNSPECIFIED., .F., .T. ) 
 B_SPLINE_CURVE_WITH_KNOTS ( ( 3, 2, 2, 2, 3 ),
 ( 0.6653225806451612545, 0.6666666666666666297, 0.6693548387096773800, 0.6720430107526881303, 0.6733870967741935054 ),
 .UNSPECIFIED. ) 
 CURVE ( )  GEOMETRIC_REPRESENTATION_ITEM ( )  RATIONAL_B_SPLINE_CURVE ( ( 0.9330127018922194093, 0.9330127018922194093, 1.000000000000000000, 0.8660254037844387076, 1.000000000000000000, 0.8660254037844387076, 1.000000000000000000, 0.9330127018922194093, 0.9330127018922194093 ) ) 
 REPRESENTATION_ITEM ( '' )  );
#19153=CARTESIAN_POINT ( 'NONE',  ( 122.1317068477954422, 247.9865022471903160, 10.00000000000009237 ) ) ;
#19154=CARTESIAN_POINT ( 'NONE',  ( 13.51768745649706993, 188.6115022471903160, -5.000000000000047962 ) ) ;
#19158=CARTESIAN_POINT ( 'NONE',  ( 165.5769259146263437, 246.9434120422340868, -1.858383500763620910 ) ) ;
#19159=ORIENTED_EDGE ( 'NONE', *, *, #37993, .T. ) ;
#19160=CARTESIAN_POINT ( 'NONE',  ( 162.9466247808429102, 248.4151622881552441, 11.25765811906727443 ) ) ;
#19167=CARTESIAN_POINT ( 'NONE',  ( 189.0455566057698604, 290.5252480108450186, 14.38176501911003236 ) ) ;
#19168=CARTESIAN_POINT ( 'NONE',  ( 170.1131776778324820, 289.4493487920391317, 2.171624877603286485 ) ) ;
#19169=CARTESIAN_POINT ( 'NONE',  ( 194.0402169394646137, 280.7468621445926829, -17.21104619501045363 ) ) ;
#19170=CARTESIAN_POINT ( 'NONE',  ( 191.8781672928813293, 296.7077321713139213, -11.78931491291747768 ) ) ;
#19173=CARTESIAN_POINT ( 'NONE',  ( 111.8115707860309556, 225.3615022471902023, 5.000000000000051514 ) ) ;
#19177=CARTESIAN_POINT ( 'NONE',  ( 164.2085977011741988, 275.1762843307250819, 14.84329694928079491 ) ) ;
#19178=CARTESIAN_POINT ( 'NONE',  ( 186.0348036264326481, 259.0250182415348945, 6.435743254585703177 ) ) ;
#19179=VERTEX_POINT ( 'NONE', #76050 ) ;
#19180=VERTEX_POINT ( 'NONE', #68414 ) ;
#19181=CARTESIAN_POINT ( 'NONE',  ( 185.2974406820879096, 297.2943441938441538, 1.030251969549985880 ) ) ;
#19183=CARTESIAN_POINT ( 'NONE',  ( 204.2556901454867955, 276.8657622634082713, 13.61111001399713949 ) ) ;
#19184=CARTESIAN_POINT ( 'NONE',  ( 194.3541845315608612, 294.0156730581561533, -14.67567721756631016 ) ) ;
#19186=CARTESIAN_POINT ( 'NONE',  ( -22.42236680055709641, 157.8615022471902591, 0.000000000000000000 ) ) ;
#19188=CARTESIAN_POINT ( 'NONE',  ( 157.6921299354026189, 257.5162143285667753, -18.18720974599499840 ) ) ;
#19189=CARTESIAN_POINT ( 'NONE',  ( 208.0925911829191932, 270.2200547229618337, -3.965170738876734546 ) ) ;
#19190=CARTESIAN_POINT ( 'NONE',  ( 191.8986733338516331, 296.2687432111309249, 12.49828825629462337 ) ) ;
#19191=AXIS2_PLACEMENT_3D ( 'NONE', #93966, #71650, #39688 ) ;
#19192=CARTESIAN_POINT ( 'NONE',  ( 181.4842875826702482, 256.0790464748339446, 5.242542569475632241 ) ) ;
#19193=CARTESIAN_POINT ( 'NONE',  ( 100.9591899430832029, 229.0958772461660260, -9.188101187500095079 ) ) ;
#19194=VERTEX_POINT ( 'NONE', #5622 ) ;
#19196=CARTESIAN_POINT ( 'NONE',  ( 118.5773942495489592, 229.2677522451417929, -5.000000000000041744 ) ) ;
#19198=B_SPLINE_CURVE_WITH_KNOTS ( 'NONE', 3,
 ( #59192, #90168, #36914, #29329, #83562, #20741, #38906, #45505, #93658, #60694, #53604, #61703, #47018, #92655, #30321, #99734 ),
 .UNSPECIFIED., .F., .F.,
 ( 4, 2, 2, 2, 2, 2, 2, 4 ),
 ( 0.000000000000000000, 0.0003786681000626416311, 0.0007573362001252832622, 0.001136004300187924785, 0.001514672400250566524, 0.001893340500313208264, 0.002272008600375849570, 0.003029344800501268357 ),
 .UNSPECIFIED. ) ;
#19201=CARTESIAN_POINT ( 'NONE',  ( 176.8376293082206701, 292.8516012225593386, -2.786154410470390363 ) ) ;
#19203=CARTESIAN_POINT ( 'NONE',  ( 159.9997000813754084, 253.5193855937126841, -16.28798248637880519 ) ) ;
#19205=CARTESIAN_POINT ( 'NONE',  ( 96.60225995211651195, 217.3923013555410080, 4.594050593750050204 ) ) ;
#19211=CARTESIAN_POINT ( 'NONE',  ( 192.4325953160755773, 264.9157042485226725, -7.801807992731872865 ) ) ;
#19212=CARTESIAN_POINT ( 'NONE',  ( 18.71383987920374992, 181.6115022471902591, 10.00000000000009592 ) ) ;
#19213=AXIS2_PLACEMENT_3D ( 'NONE', #5013, #44480, #21210 ) ;
#19215=CARTESIAN_POINT ( 'NONE',  ( 136.8177939967088435, 258.9869531367911009, 4.594050593750046652 ) ) ;
#19218=CARTESIAN_POINT ( 'NONE',  ( 166.8083734521890449, 257.5796782931630560, -15.79284703031436798 ) ) ;
#19220=CARTESIAN_POINT ( 'NONE',  ( 156.7854950622006527, 259.0865519928661911, 18.17819951099994213 ) ) ;
#19221=CARTESIAN_POINT ( 'NONE',  ( 160.5517938760779089, 275.6377758284635888, 12.83436562505768741 ) ) ;
#19223=CARTESIAN_POINT ( 'NONE',  ( 189.7737856813211579, 269.7866060870444471, 15.20194579022378889 ) ) ;
#19230=CARTESIAN_POINT ( 'NONE',  ( 153.6596595523362794, 266.9882342533689439, 16.60685250298524807 ) ) ;
#19231=CARTESIAN_POINT ( 'NONE',  ( 206.7596416265183734, 271.4678399409689291, 6.202658291405857227 ) ) ;
#19233=CARTESIAN_POINT ( 'NONE',  ( 206.8775514429320026, 272.3245652858344670, -9.838455694836268250 ) ) ;
#19235=CARTESIAN_POINT ( 'NONE',  ( 162.8223739550644211, 248.6303710312858186, -11.16939803179192658 ) ) ;
#19242=CARTESIAN_POINT ( 'NONE',  ( 177.5616848261300902, 264.8410986875884419, -15.15881583357887585 ) ) ;
#19243=B_SPLINE_CURVE_WITH_KNOTS ( 'NONE', 3,
 ( #25909, #87764, #3605, #42081, #18303, #63387, #49201, #72518, #82133, #50670, #66871, #4081 ),
 .UNSPECIFIED., .F., .F.,
 ( 4, 2, 2, 2, 2, 4 ),
 ( 0.001172129118361127592, 0.001404330768412652593, 0.001636532418464177593, 0.002100935718567244724, 0.002565339018670311638, 0.003029742318773378552 ),
 .UNSPECIFIED. ) ;
#19245=B_SPLINE_CURVE_WITH_KNOTS ( 'NONE', 3,
 ( #64049, #72170, #3276, #65051 ),
 .UNSPECIFIED., .F., .F.,
 ( 4, 4 ),
 ( 0.01672295409251149667, 0.02560742481406136015 ),
 .UNSPECIFIED. ) ;
#19248=CARTESIAN_POINT ( 'NONE',  ( 92.68684311912451790, 230.9865022471902876, -10.00000000000009592 ) ) ;
#19249=CARTESIAN_POINT ( 'NONE',  ( 155.4810912439522212, 261.3458456796594760, -18.44218279064527266 ) ) ;
#19252=CARTESIAN_POINT ( 'NONE',  ( 6.183361268541195166, 180.5024278399160949, 9.188101187500095079 ) ) ;
#19258=CARTESIAN_POINT ( 'NONE',  ( 32.38097682878547090, 183.3768266524160140, 9.188101187500096856 ) ) ;
#19260=CARTESIAN_POINT ( 'NONE',  ( 161.4726291907278721, 250.9681975403669867, 14.52346149734912117 ) ) ;
#19261=CARTESIAN_POINT ( 'NONE',  ( 147.4368675721658519, 275.2788497866417288, 5.050119523016719292 ) ) ;
#19263=CARTESIAN_POINT ( 'NONE',  ( 178.6323251955368505, 291.6746863476311660, 6.062186576083094636 ) ) ;
#19264=CARTESIAN_POINT ( 'NONE',  ( 177.9425575674935374, 293.7981536106174758, 2.760600958814514616 ) ) ;
#19265=CARTESIAN_POINT ( 'NONE',  ( 179.0121081408051396, 278.3636465084506426, -16.96624558982258080 ) ) ;
#19268=CARTESIAN_POINT ( 'NONE',  ( 84.23301146803963491, 230.9860189848785410, -2.679491924311252493 ) ) ;
#19271=CARTESIAN_POINT ( 'NONE',  ( 88.42888488385111145, 211.8615022471902023, 5.000000000000051514 ) ) ;
#19273=CARTESIAN_POINT ( 'NONE',  ( 181.4204268205617154, 259.5203828285251006, -11.17471347674236348 ) ) ;
#19274=CARTESIAN_POINT ( 'NONE',  ( 38.76756708593069334, 199.3149278399161233, -9.188101187500095079 ) ) ;
#19277=CARTESIAN_POINT ( 'NONE',  ( 198.7829547491859330, 286.3448180261817129, -18.59838968157616179 ) ) ;
#19279=ORIENTED_EDGE ( 'NONE', *, *, #68824, .T. ) ;
#19280=CARTESIAN_POINT ( 'NONE',  ( 171.2251843287659483, 286.5252364908957929, 7.482153322356102088 ) ) ;
#19281=CARTESIAN_POINT ( 'NONE',  ( 207.6007741873543750, 271.0719067473055475, 7.587922723682903658 ) ) ;
#19284=CARTESIAN_POINT ( 'NONE',  ( 189.0887393702818997, 265.5389857731253187, 10.68645298647155784 ) ) ;
#19285=CARTESIAN_POINT ( 'NONE',  ( 196.4808189786114951, 290.3322341467384717, -17.84817245450773271 ) ) ;
#19286=EDGE_CURVE ( 'NONE', #80986, #13784, #45261, .T. ) ;
#19287=CARTESIAN_POINT ( 'NONE',  ( 175.1555329544323172, 257.3877955703446787, 11.56198837495037068 ) ) ;
#19291=CARTESIAN_POINT ( 'NONE',  ( 171.6221518209352439, 252.5826950423761161, 8.616696649246458506 ) ) ;
#19292=CARTESIAN_POINT ( 'NONE',  ( 14.02286894203806433, 172.2365022471902307, 10.00000000000009948 ) ) ;
#19293=EDGE_LOOP ( 'NONE', ( #22638, #27043, #93492, #67858 ) ) ;
#19295=CARTESIAN_POINT ( 'NONE',  ( 191.4484954869714954, 299.0484741143815199, 8.684991747358081327 ) ) ;
#19297=CARTESIAN_POINT ( 'NONE',  ( 166.7686158928260909, 246.5184119549025752, 0.4773397470127070386 ) ) ;
#19301=CARTESIAN_POINT ( 'NONE',  ( 161.8935665241663457, 250.2391126920490194, -13.69501063978231770 ) ) ;
#19303=CARTESIAN_POINT ( 'NONE',  ( 196.4808189786114951, 290.3322341467384717, -17.84817245450773271 ) ) ;
#19307=CARTESIAN_POINT ( 'NONE',  ( 197.8809552785519656, 287.9071269377202498, 17.61728046362068412 ) ) ;
#19311=CARTESIAN_POINT ( 'NONE',  ( 205.3943609285979051, 274.8935266139653777, -13.14270440534009943 ) ) ;
#19312=CARTESIAN_POINT ( 'NONE',  ( 112.2171730965159071, 247.8464784336661353, 1.353441290958777525E-15 ) ) ;
#19314=CARTESIAN_POINT ( 'NONE',  ( 34.21208616421488102, 183.8927522451417929, -10.00000000000009237 ) ) ;
#19315=ORIENTED_EDGE ( 'NONE', *, *, #61391, .F. ) ;
#19317=CARTESIAN_POINT ( 'NONE',  ( 208.1757572214753793, 270.0760069187178374, 2.172546422564154867 ) ) ;
#19320=CARTESIAN_POINT ( 'NONE',  ( 159.9671766634011192, 253.5757178060795809, 16.49140845334465411 ) ) ;
#19322=CARTESIAN_POINT ( 'NONE',  ( 72.16419236301562989, 200.2202760586659736, -5.415160957724236172E-17 ) ) ;
#19323=ORIENTED_EDGE ( 'NONE', *, *, #781, .T. ) ;
#19324=FACE_OUTER_BOUND ( 'NONE', #53272, .T. ) ;
#19325=CARTESIAN_POINT ( 'NONE',  ( 150.8167050463783312, 269.4247995599803289, 14.38040671671637938 ) ) ;
#19326=CARTESIAN_POINT ( 'NONE',  ( 168.9285091408607684, 266.8905904589466900, 17.77692745299157195 ) ) ;
#19327=CARTESIAN_POINT ( 'NONE',  ( 172.6353124949622213, 276.9286716572659657, 15.75460722331730246 ) ) ;
#19332=CARTESIAN_POINT ( 'NONE',  ( 203.5080190724872011, 278.1607665491929993, -15.47044080916498743 ) ) ;
#19338=CARTESIAN_POINT ( 'NONE',  ( 177.0481772032109120, 269.7367243736813975, 17.49060471085816815 ) ) ;
#19342=CARTESIAN_POINT ( 'NONE',  ( 153.8374836801523315, 264.9808921322257902, -16.57868851438277957 ) ) ;
#19344=CARTESIAN_POINT ( 'NONE',  ( 10.02758540662582654, 165.0494855054052437, -2.679491924311248496 ) ) ;
#19345=CARTESIAN_POINT ( 'NONE',  ( 126.2364799639240260, 237.5643266524160140, 9.188101187500095079 ) ) ;
#19350=CARTESIAN_POINT ( 'NONE',  ( 163.2708734627827312, 285.5880326804372089, 1.431608037597408289 ) ) ;
#19353=CARTESIAN_POINT ( 'NONE',  ( 178.6690291948835068, 254.3411016048053170, 4.509037496016676805 ) ) ;
#19354=ORIENTED_EDGE ( 'NONE', *, *, #97840, .T. ) ;
#19358=EDGE_CURVE ( 'NONE', #83021, #6447, #16738, .T. ) ;
#19364=CARTESIAN_POINT ( 'NONE',  ( 157.1850763439666139, 258.3944569110938687, -16.98181238659443437 ) ) ;
#19365=CARTESIAN_POINT ( 'NONE',  ( 174.5802574196832779, 252.1115117894923117, 3.521029629026526386 ) ) ;
#19367=FACE_OUTER_BOUND ( 'NONE', #26874, .T. ) ;
#19369=CARTESIAN_POINT ( 'NONE',  ( 169.3955309194774372, 285.1200513657703937, -8.058459443620145990 ) ) ;
#19370=FACE_OUTER_BOUND ( 'NONE', #19739, .T. ) ;
#19371=CARTESIAN_POINT ( 'NONE',  ( 157.5112492719526642, 271.0101375079576655, -14.70005484135263529 ) ) ;
#19372=CARTESIAN_POINT ( 'NONE',  ( 134.5988642195610225, 258.5177522451419350, 5.000000000000046185 ) ) ;
#19376=CARTESIAN_POINT ( 'NONE',  ( 157.4177733328310467, 257.9914139036126812, 18.29188238796808363 ) ) ;
#19377=CARTESIAN_POINT ( 'NONE',  ( 190.5726849661229210, 300.5654224342945326, -0.2192718484028965964 ) ) ;
#19378=CARTESIAN_POINT ( 'NONE',  ( -7.645548028435306342, 157.2048013555409796, 4.594050593750051981 ) ) ;
#19379=CARTESIAN_POINT ( 'NONE',  ( 39.47103917862304456, 205.8464784336661637, 1.353441290958777327E-15 ) ) ;
#19384=CARTESIAN_POINT ( 'NONE',  ( 157.2777284163744582, 258.2339788142568864, -16.82360006463426316 ) ) ;
#19385=CARTESIAN_POINT ( 'NONE',  ( 189.0965068574246573, 290.5071001834722892, -14.60706148674475280 ) ) ;
#19386=CARTESIAN_POINT ( 'NONE',  ( 146.8058449195592061, 276.3718130816831149, 4.181814292810413392 ) ) ;
#19388=CARTESIAN_POINT ( 'NONE',  ( 167.6973146981588911, 256.6379102646401975, 13.70945070367496754 ) ) ;
#19389=CARTESIAN_POINT ( 'NONE',  ( 77.51335635343681929, 208.8927522451417929, 10.00000000000009592 ) ) ;
#19393=VECTOR ( 'NONE', #85460, 1000.000000000000000 ) ;
#19394=CARTESIAN_POINT ( 'NONE',  ( 49.45774171355136417, 189.3615022471902023, 5.000000000000051514 ) ) ;
#19395=CARTESIAN_POINT ( 'NONE',  ( 181.9890126569457891, 291.7084811444626666, 9.326053301564767750 ) ) ;
#19396=CARTESIAN_POINT ( 'NONE',  ( 163.1691520398773321, 248.0297337694385931, 11.21816141384514331 ) ) ;
#19397=CARTESIAN_POINT ( 'NONE',  ( 12.08367997547019002, 165.5327760586659451, 1.948934522072303157E-15 ) ) ;
#19399=DIRECTION ( 'NONE',  ( 0.4999999999999998890, -0.8660254037844385966, 0.000000000000000000 ) ) ;
#19400=CARTESIAN_POINT ( 'NONE',  ( 192.1396999271463812, 297.8512729055811974, 12.32430960859512403 ) ) ;
#19402=CARTESIAN_POINT ( 'NONE',  ( 156.2909461963670310, 261.2938674384161004, -17.49506900824429323 ) ) ;
#19403=CARTESIAN_POINT ( 'NONE',  ( 179.3884211033321492, 277.5219014342368951, 16.65719480442988498 ) ) ;
#19408=CARTESIAN_POINT ( 'NONE',  ( 124.2787281577965075, 235.8927522451418213, 10.00000000000009948 ) ) ;
#19411=CARTESIAN_POINT ( 'NONE',  ( 159.3316980867583368, 259.1362291154864010, 16.70884618213627348 ) ) ;
#19413=CARTESIAN_POINT ( 'NONE',  ( 154.8556227199321427, 262.4291889417971788, 17.77326384500479861 ) ) ;
#19414=VERTEX_POINT ( 'NONE', #70932 ) ;
#19416=CARTESIAN_POINT ( 'NONE',  ( 206.4640281786353171, 273.0408085897082060, -10.81921452789957883 ) ) ;
#19419=B_SPLINE_CURVE_WITH_KNOTS ( 'NONE', 3,
 ( #78558, #8146, #78053, #32444, #8642, #85703, #18254, #49150, #25859, #9664, #86200, #95303 ),
 .UNSPECIFIED., .F., .F.,
 ( 4, 2, 2, 2, 2, 4 ),
 ( 0.001153997166473859142, 0.001388415620727351078, 0.001622834074980843014, 0.002091670983487826235, 0.002560507891994809240, 0.003029344800501792244 ),
 .UNSPECIFIED. ) ;
#19420=ORIENTED_EDGE ( 'NONE', *, *, #93934, .T. ) ;
#19421=CARTESIAN_POINT ( 'NONE',  ( 152.5758826934612955, 268.0217239346885094, 15.77428039732272858 ) ) ;
#19422=CARTESIAN_POINT ( 'NONE',  ( 207.1122325394003951, 271.9180857031755636, 7.794245785756032774 ) ) ;
#19427=CARTESIAN_POINT ( 'NONE',  ( 164.1356542478074516, 246.7701760825098916, -4.987495687701697378 ) ) ;
#19428=CARTESIAN_POINT ( 'NONE',  ( 204.7986527064648214, 275.9253235211867263, 14.74587861556245905 ) ) ;
#19429=CARTESIAN_POINT ( 'NONE',  ( 192.5254593562406171, 297.1831179748913314, 11.00703791256144015 ) ) ;
#19432=CARTESIAN_POINT ( 'NONE',  ( 174.9783775354441104, 262.5161152102281221, 14.35741776163894734 ) ) ;
#19435=DIRECTION ( 'NONE',  ( 0.4999999999999998890, -0.8660254037844385966, 0.000000000000000000 ) ) ;
#19440=CARTESIAN_POINT ( 'NONE',  ( 169.4433785151117036, 276.3082714494867105, -15.64270847926871966 ) ) ;
#19443=CARTESIAN_POINT ( 'NONE',  ( 175.2041007476701111, 277.6819973178614305, -15.66111034898646359 ) ) ;
#19445=EDGE_CURVE ( 'NONE', #37697, #11680, #66971, .T. ) ;
#19446=CARTESIAN_POINT ( 'NONE',  ( 156.9458340580773665, 266.2207217376895869, -16.53175181285456219 ) ) ;
#19447=VERTEX_POINT ( 'NONE', #48113 ) ;
#19450=( BOUNDED_CURVE ( )  B_SPLINE_CURVE ( 2, ( #54549, #85533, #74033, #27911, #20331, #51202, #1392, #24180, #46977 ),
 .UNSPECIFIED., .F., .T. ) 
 B_SPLINE_CURVE_WITH_KNOTS ( ( 3, 2, 2, 2, 3 ),
 ( 0.8427419354838709964, 0.8440860215053763715, 0.8467741935483871218, 0.8494623655913978721, 0.8508064516129032473 ),
 .UNSPECIFIED. ) 
 CURVE ( )  GEOMETRIC_REPRESENTATION_ITEM ( )  RATIONAL_B_SPLINE_CURVE ( ( 0.9330127018922194093, 0.9330127018922194093, 1.000000000000000000, 0.8660254037844387076, 1.000000000000000000, 0.8660254037844387076, 1.000000000000000000, 0.9330127018922194093, 0.9330127018922194093 ) ) 
 REPRESENTATION_ITEM ( '' )  );
#19452=CARTESIAN_POINT ( 'NONE',  ( 193.5623078039747895, 295.3872437836667473, 14.88922347750675712 ) ) ;
#19457=CARTESIAN_POINT ( 'NONE',  ( 178.4143452015725870, 291.8002240674260861, 6.990295570472018660 ) ) ;
#19458=CARTESIAN_POINT ( 'NONE',  ( 191.1000148935602567, 299.6520602076213891, -9.462302242170249400 ) ) ;
#19462=CARTESIAN_POINT ( 'NONE',  ( 149.2923684163597784, 272.0650280510108701, -12.99082738998495756 ) ) ;
#19464=CARTESIAN_POINT ( 'NONE',  ( 198.3523905153085423, 287.0905771551796306, 18.52598547438866206 ) ) ;
#19467=CARTESIAN_POINT ( 'NONE',  ( 146.6807985088175030, 276.5883998183917925, -3.564129467591749201 ) ) ;
#19469=CARTESIAN_POINT ( 'NONE',  ( 171.5055362605466485, 259.4143056590929746, -13.88236582212129377 ) ) ;
#19470=DIRECTION ( 'NONE',  ( 0.4999999999999998890, -0.8660254037844385966, 0.000000000000000000 ) ) ;
#19472=CARTESIAN_POINT ( 'NONE',  ( 199.1649783209272471, 285.6831337902369228, -18.56878453077520774 ) ) ;
#19473=CARTESIAN_POINT ( 'NONE',  ( 190.2679671178493095, 301.0932092294775089, 0.1305210825167657518 ) ) ;
#19476=CARTESIAN_POINT ( 'NONE',  ( 167.3627897228288077, 252.8219202345026702, -12.34552495514862613 ) ) ;
#19478=CARTESIAN_POINT ( 'NONE',  ( 132.0729567918564555, 240.3927522451418213, 10.00000000000009948 ) ) ;
#19479=CARTESIAN_POINT ( 'NONE',  ( 165.0437781805843258, 244.7827860485373606, -2.050141714668513693 ) ) ;
#19480=CARTESIAN_POINT ( 'NONE',  ( 36.81016237556818993, 185.3927522451417929, -10.00000000000009059 ) ) ;
#19481=CARTESIAN_POINT ( 'NONE',  ( 103.7194723697636221, 236.8149278399160949, -9.188101187500095079 ) ) ;
#19482=CARTESIAN_POINT ( 'NONE',  ( 183.6574624063936483, 296.2739094579258676, -2.715018486543457676 ) ) ;
#19486=CARTESIAN_POINT ( 'NONE',  ( 162.4263297320084121, 249.3163397476629086, 11.18012070315788087 ) ) ;
#19487=CARTESIAN_POINT ( 'NONE',  ( 24.58674819472551931, 178.8768266524160140, 9.188101187500098632 ) ) ;
#19493=CARTESIAN_POINT ( 'NONE',  ( 147.4771206202524354, 275.6046823160672830, -0.001107820683494442279 ) ) ;
#19496=CARTESIAN_POINT ( 'NONE',  ( 147.2494378675467033, 275.6034875578896504, 3.639370109197119341 ) ) ;
#19497=CARTESIAN_POINT ( 'NONE',  ( 192.9905603666904881, 263.7646147800884933, -4.130271572274535785 ) ) ;
#19499=CARTESIAN_POINT ( 'NONE',  ( 185.8711499578670043, 286.5456327281862627, 15.65987533235325202 ) ) ;
#19501=CARTESIAN_POINT ( 'NONE',  ( 43.61180991440864574, 205.1744531367911293, 4.594050593750047540 ) ) ;
#19502=CARTESIAN_POINT ( 'NONE',  ( 93.82350145804376496, 211.6427522451417644, 1.119607411625061291E-15 ) ) ;
#19504=CARTESIAN_POINT ( 'NONE',  ( 179.0002306397571488, 259.3607547712236965, -10.30360065349030307 ) ) ;
#19505=CARTESIAN_POINT ( 'NONE',  ( -2.476892769303202790, 175.5024278399161233, -9.188101187500093303 ) ) ;
#19507=CARTESIAN_POINT ( 'NONE',  ( 198.4522155198218059, 286.9176751754968109, -17.57438352224490075 ) ) ;
#19508=CYLINDRICAL_SURFACE ( 'NONE', #3119, 17.82106496071139645 ) ;
#19509=CARTESIAN_POINT ( 'NONE',  ( 192.4172326059820648, 297.3705722050773943, -12.52563289807247848 ) ) ;
#19511=CARTESIAN_POINT ( 'NONE',  ( 203.6831990939301420, 276.1885599565742382, 13.29506139827553390 ) ) ;
#19514=ORIENTED_EDGE ( 'NONE', *, *, #50979, .T. ) ;
#19515=CARTESIAN_POINT ( 'NONE',  ( 0.5273063997304934247, 181.1115022471903444, -5.000000000000047962 ) ) ;
#19516=CARTESIAN_POINT ( 'NONE',  ( 196.8708119716154954, 268.3476497963631573, -11.07389558091716708 ) ) ;
#19517=CARTESIAN_POINT ( 'NONE',  ( 120.7695210546522446, 240.5333772461660544, 9.188101187500095079 ) ) ;
#19525=ORIENTED_EDGE ( 'NONE', *, *, #52335, .T. ) ;
#19526=CARTESIAN_POINT ( 'NONE',  ( 151.0099717111976076, 269.0900518771037468, 15.84752309685681659 ) ) ;
#19527=CARTESIAN_POINT ( 'NONE',  ( 207.6502225385047780, 270.9862596907630063, -1.369768233574514271 ) ) ;
#19528=CARTESIAN_POINT ( 'NONE',  ( 187.9019955452718023, 260.0457317612239194, -6.306085470763082235 ) ) ;
#19529=CARTESIAN_POINT ( 'NONE',  ( 172.7307785454424618, 267.9789046868485229, -16.30596211021181219 ) ) ;
#19533=CARTESIAN_POINT ( 'NONE',  ( 165.6138761065251970, 269.2084108731353354, -16.71299972576612802 ) ) ;
#19536=CARTESIAN_POINT ( 'NONE',  ( 182.5990217920488590, 295.0943774630480902, 4.729822608770373193 ) ) ;
#19539=CARTESIAN_POINT ( 'NONE',  ( 150.6825202918323612, 277.8236102357049049, -1.156507784398024520E-06 ) ) ;
#19540=CARTESIAN_POINT ( 'NONE',  ( 193.7492780744840957, 282.5563289966625575, 17.04412244182808678 ) ) ;
#19542=CARTESIAN_POINT ( 'NONE',  ( 195.3480551831553385, 290.3289108874006388, -16.65360927049558981 ) ) ;
#19543=EDGE_LOOP ( 'NONE', ( #48985, #90563, #27878, #68756, #64756, #66023, #53904, #39775, #16570, #78314, #55541, #57151, #69658, #10410, #97110, #55371, #20797, #29002, #89464 ) ) ;
#19544=DIRECTION ( 'NONE',  ( -0.8660254037844387076, -0.4999999999999998890, -0.000000000000000000 ) ) ;
#19545=CARTESIAN_POINT ( 'NONE',  ( 194.8708600166808651, 293.1207648669033006, -14.79199694356877970 ) ) ;
#19546=CARTESIAN_POINT ( 'NONE',  ( 156.0722444812057574, 261.8173697120565180, -16.98794231501332419 ) ) ;
#19547=ORIENTED_EDGE ( 'NONE', *, *, #21918, .F. ) ;
#19552=ORIENTED_EDGE ( 'NONE', *, *, #67306, .T. ) ;
#19553=CARTESIAN_POINT ( 'NONE',  ( 83.25962220535622293, 225.0024278399160949, -9.188101187500093303 ) ) ;
#19555=CARTESIAN_POINT ( 'NONE',  ( -22.42236680055709641, 157.8615022471902591, 0.000000000000000000 ) ) ;
#19556=DIRECTION ( 'NONE',  ( -0.8660254037844387076, -0.4999999999999998890, -0.000000000000000000 ) ) ;
#19558=EDGE_CURVE ( 'NONE', #53564, #86106, #64466, .T. ) ;
#19563=CARTESIAN_POINT ( 'NONE',  ( 179.7609715772761376, 289.9450057921314965, -11.88024692884158462 ) ) ;
#19566=CARTESIAN_POINT ( 'NONE',  ( 155.1601726304954809, 261.9016930232608615, -18.56587418422714464 ) ) ;
#19567=ORIENTED_EDGE ( 'NONE', *, *, #541, .T. ) ;
#19568=CARTESIAN_POINT ( 'NONE',  ( 182.9467913113457769, 279.7477425878400368, -16.58815582825729962 ) ) ;
#19571=DIRECTION ( 'NONE',  ( 0.4999999999999988343, -0.8660254037844393737, 0.000000000000000000 ) ) ;
#19572=CARTESIAN_POINT ( 'NONE',  ( 153.4361244163197000, 264.8878321249116539, -17.23169627811277493 ) ) ;
#19574=CARTESIAN_POINT ( 'NONE',  ( 8.826716519331432309, 169.2365022471902307, 10.00000000000009948 ) ) ;
#19575=CARTESIAN_POINT ( 'NONE',  ( 145.1264855360895751, 254.5958772461660544, -9.188101187500095079 ) ) ;
#19580=VERTEX_POINT ( 'NONE', #36395 ) ;
#19583=CARTESIAN_POINT ( 'NONE',  ( 125.0725847779322351, 243.0177522451418497, -10.00000000000009592 ) ) ;
#19584=CARTESIAN_POINT ( 'NONE',  ( 156.7469768102917271, 279.2875448729189429, 7.364017834103635529 ) ) ;
#19585=CARTESIAN_POINT ( 'NONE',  ( 165.5287013238079794, 246.9198946887887871, -1.935065831620633503 ) ) ;
#19586=CARTESIAN_POINT ( 'NONE',  ( 172.0841359714602561, 280.2593053177052980, 13.89066565685676480 ) ) ;
#19590=CARTESIAN_POINT ( 'NONE',  ( 184.9091135615353494, 272.9493583962221805, -17.03684365370855858 ) ) ;
#19593=VERTEX_POINT ( 'NONE', #76425 ) ;
#19594=CARTESIAN_POINT ( 'NONE',  ( 194.2914079707598773, 293.7378065512926923, -14.23787508785857270 ) ) ;
#19597=CARTESIAN_POINT ( 'NONE',  ( 205.0753842767173580, 269.1534704228733403, -3.005433063649942671 ) ) ;
#19598=B_SPLINE_CURVE_WITH_KNOTS ( 'NONE', 3,
 ( #66892, #20313, #98318, #59783 ),
 .UNSPECIFIED., .F., .F.,
 ( 4, 4 ),
 ( 0.02408851552819888178, 0.03332966919768538122 ),
 .UNSPECIFIED. ) ;
#19599=CARTESIAN_POINT ( 'NONE',  ( 203.6564843095729316, 277.9036172154027327, -14.39421774622613803 ) ) ;
#19600=CARTESIAN_POINT ( 'NONE',  ( 149.3883679478359454, 271.8987519849911223, 12.99187507659642371 ) ) ;
#19601=CARTESIAN_POINT ( 'NONE',  ( 162.0222989613219227, 273.0741124436839868, 15.00522561680813283 ) ) ;
#19604=CARTESIAN_POINT ( 'NONE',  ( 203.3788045512062865, 270.0447488680846391, 5.971987935157939020 ) ) ;
#19605=ORIENTED_EDGE ( 'NONE', *, *, #97446, .T. ) ;
#19608=CARTESIAN_POINT ( 'NONE',  ( 189.8237993498458138, 274.2492852631884830, -15.65096844494817674 ) ) ;
#19609=ADVANCED_FACE ( 'NONE', ( #66314 ), #78824, .F. ) ;
#19611=CARTESIAN_POINT ( 'NONE',  ( 192.8132846206021611, 296.6845899933152850, 11.53748932578252351 ) ) ;
#19615=CARTESIAN_POINT ( 'NONE',  ( 12.94935828348961593, 178.2833772461660544, -9.188101187500095079 ) ) ;
#19616=CARTESIAN_POINT ( 'NONE',  ( 107.4543804714665072, 232.8458772461660544, 9.188101187500095079 ) ) ;
#19617=CARTESIAN_POINT ( 'NONE',  ( 203.0862352702880003, 278.8913175244117610, -15.09542727681365015 ) ) ;
#19619=CARTESIAN_POINT ( 'NONE',  ( 181.2455912396057727, 255.1350553628389832, -2.495996851558535123 ) ) ;
#19620=B_SPLINE_CURVE_WITH_KNOTS ( 'NONE', 3,
 ( #48114, #79056, #18729, #35408, #33941, #34900, #5022, #80564, #41506, #27325 ),
 .UNSPECIFIED., .F., .F.,
 ( 4, 2, 2, 2, 4 ),
 ( 0.001327043042251581763, 0.001752654217620215225, 0.002178265392988848470, 0.002603876568357481932, 0.003029487743726115394 ),
 .UNSPECIFIED. ) ;
#19622=CARTESIAN_POINT ( 'NONE',  ( 197.8980529691977779, 285.8775128688180871, 17.80711829255526979 ) ) ;
#19623=CARTESIAN_POINT ( 'NONE',  ( 155.5085848088033345, 279.2288744083967345, -7.567598119550592806 ) ) ;
#19624=CARTESIAN_POINT ( 'NONE',  ( 194.8598199529639317, 293.1398868181796615, -15.91766051364927570 ) ) ;
#19627=CARTESIAN_POINT ( 'NONE',  ( 166.2219174074001273, 253.6012899646903236, -13.47457580965214419 ) ) ;
#19628=CARTESIAN_POINT ( 'NONE',  ( 174.8830188891286639, 265.0810552416202768, -15.58703472796680600 ) ) ;
#19630=CARTESIAN_POINT ( 'NONE',  ( 79.55186417146283873, 225.9244531367911293, -4.594050593750046652 ) ) ;
#19631=CARTESIAN_POINT ( 'NONE',  ( 161.3773209892555371, 251.1332761876949746, -14.50043705923759241 ) ) ;
#19633=CARTESIAN_POINT ( 'NONE',  ( 196.3720681610792553, 290.5205960880691691, 16.18360420724715354 ) ) ;
#19634=CARTESIAN_POINT ( 'NONE',  ( 199.7305354183539521, 284.7035601629126518, 18.18279833004080004 ) ) ;
#19635=CARTESIAN_POINT ( 'NONE',  ( 151.3124059063077311, 268.5662204852269497, -14.45542936000225609 ) ) ;
#19636=CARTESIAN_POINT ( 'NONE',  ( 173.5541795782666838, 267.4165219661629180, -17.04824448052345431 ) ) ;
#19642=CARTESIAN_POINT ( 'NONE',  ( 173.1278816705146539, 289.7173446917369120, -0.9128981044102878473 ) ) ;
#19644=CARTESIAN_POINT ( 'NONE',  ( 191.5982176700465800, 288.2760343549104505, -15.80419025984858195 ) ) ;
#19650=CARTESIAN_POINT ( 'NONE',  ( 131.8023238567216708, 260.2365022471903444, 2.944929066748280225E-16 ) ) ;
#19651=CARTESIAN_POINT ( 'NONE',  ( 157.6036818288543486, 257.6694109429415107, -16.73826488331764395 ) ) ;
#19653=VERTEX_POINT ( 'NONE', #95148 ) ;
#19654=CARTESIAN_POINT ( 'NONE',  ( 169.2826475696182058, 248.6736941890546291, -1.907850670695832473 ) ) ;
#19656=CARTESIAN_POINT ( 'NONE',  ( 203.0398866899141126, 278.9715956204779559, 16.57839218037009132 ) ) ;
#19662=CARTESIAN_POINT ( 'NONE',  ( 158.6857353490262881, 255.7952392694948287, 17.63394428141803871 ) ) ;
#19663=CARTESIAN_POINT ( 'NONE',  ( 158.8266160086023149, 257.5512268093053194, -17.29683829744028856 ) ) ;
#19668=CARTESIAN_POINT ( 'NONE',  ( 176.8917175299031896, 289.5346434493817469, -10.53293604869262978 ) ) ;
#19669=EDGE_CURVE ( 'NONE', #51125, #56410, #97167, .T. ) ;
#19672=ORIENTED_EDGE ( 'NONE', *, *, #26302, .T. ) ;
#19673=AXIS2_PLACEMENT_3D ( 'NONE', #33494, #56273, #79132 ) ;
#19674=ORIENTED_EDGE ( 'NONE', *, *, #43566, .T. ) ;
#19676=CARTESIAN_POINT ( 'NONE',  ( 204.7986527064648214, 275.9253235211867263, 14.74587861556245905 ) ) ;
#19677=CARTESIAN_POINT ( 'NONE',  ( 165.9227384538158105, 274.2955112070876567, -15.12533405962566846 ) ) ;
#19679=CARTESIAN_POINT ( 'NONE',  ( 155.1376601545389917, 261.9406857754215707, 18.55063430030667959 ) ) ;
#19680=CARTESIAN_POINT ( 'NONE',  ( 153.6323727466833873, 269.3172676078306154, -15.66543061290010641 ) ) ;
#19681=CARTESIAN_POINT ( 'NONE',  ( 180.0662822340164269, 262.4007578510376675, -14.24330825748563534 ) ) ;
#19682=CARTESIAN_POINT ( 'NONE',  ( 164.4860472601134802, 245.7488043397450781, 5.786386706270143954 ) ) ;
#19683=CARTESIAN_POINT ( 'NONE',  ( 168.9819228013596728, 267.0053382609680170, 16.74345436343837790 ) ) ;
#19684=CARTESIAN_POINT ( 'NONE',  ( 182.0074952572218194, 256.7411546301147496, 5.145569241165440566 ) ) ;
#19685=CARTESIAN_POINT ( 'NONE',  ( 90.05242219234915524, 231.9869531367911293, 4.594050593750046652 ) ) ;
#19687=CARTESIAN_POINT ( 'NONE',  ( 149.8528230149711646, 271.4847137799879988, 11.79734874491912322 ) ) ;
#19689=CARTESIAN_POINT ( 'NONE',  ( 166.2705977412429661, 279.3148818941612035, -14.08247858441158940 ) ) ;
#19691=VERTEX_POINT ( 'NONE', #72832 ) ;
#19694=CARTESIAN_POINT ( 'NONE',  ( 157.3412122618683497, 258.1240215684019290, 16.75554199904894048 ) ) ;
#19696=CARTESIAN_POINT ( 'NONE',  ( 206.8383266605359552, 270.5703304059348397, -4.969267838202788390 ) ) ;
#19697=CARTESIAN_POINT ( 'NONE',  ( 91.05385083941617097, 229.5024278399160949, -9.188101187500093303 ) ) ;
#19699=ORIENTED_EDGE ( 'NONE', *, *, #26079, .F. ) ;
#19701=CARTESIAN_POINT ( 'NONE',  ( 162.6757594134126350, 248.8843148665554281, -10.86406770146305867 ) ) ;
#19702=ORIENTED_EDGE ( 'NONE', *, *, #30515, .F. ) ;
#19703=CARTESIAN_POINT ( 'NONE',  ( 194.7838651859529477, 266.2706033605068114, -8.657540068871613315 ) ) ;
#19704=CARTESIAN_POINT ( 'NONE',  ( 153.4111665582887838, 266.7507244080648547, 16.54171954082816853 ) ) ;
#19706=CARTESIAN_POINT ( 'NONE',  ( 128.5905526607566856, 254.2369531367911293, -4.594050593750048428 ) ) ;
#19708=CARTESIAN_POINT ( 'NONE',  ( -12.55328564014489245, 176.8927522451419350, 2.944929066748280225E-16 ) ) ;
#19710=ORIENTED_EDGE ( 'NONE', *, *, #18872, .F. ) ;
#19711=CARTESIAN_POINT ( 'NONE',  ( 157.4493702961534609, 257.9366863577731124, 17.30941950273115637 ) ) ;
#19718=CARTESIAN_POINT ( 'NONE',  ( 195.6983338289388712, 279.8441605301517257, -16.88118927210886255 ) ) ;
#19719=CYLINDRICAL_SURFACE ( 'NONE', #96493, 17.82106496071139645 ) ;
#19721=DIRECTION ( 'NONE',  ( -0.8660254037844387076, -0.4999999999999998890, -0.000000000000000000 ) ) ;
#19722=CARTESIAN_POINT ( 'NONE',  ( 167.8549298750992307, 249.5183355316891038, 8.029450975726973638 ) ) ;
#19724=CARTESIAN_POINT ( 'NONE',  ( 163.2742264920156572, 247.8477394797576778, -9.850275379362519956 ) ) ;
#19726=EDGE_CURVE ( 'NONE', #16763, #38435, #69301, .T. ) ;
#19729=CARTESIAN_POINT ( 'NONE',  ( 165.9091197491159164, 246.2627970730538323, -2.747640711776688338 ) ) ;
#19732=( BOUNDED_CURVE ( )  B_SPLINE_CURVE ( 2, ( #2166, #95413, #34069, #88817, #88313, #72067, #2667, #40635, #25969 ),
 .UNSPECIFIED., .F., .T. ) 
 B_SPLINE_CURVE_WITH_KNOTS ( ( 3, 2, 2, 2, 3 ),
 ( 0.3104838709677419373, 0.3118279569892473124, 0.3145161290322580627, 0.3172043010752688130, 0.3185483870967741882 ),
 .UNSPECIFIED. ) 
 CURVE ( )  GEOMETRIC_REPRESENTATION_ITEM ( )  RATIONAL_B_SPLINE_CURVE ( ( 0.9330127018922194093, 0.9330127018922194093, 1.000000000000000000, 0.8660254037844387076, 1.000000000000000000, 0.8660254037844387076, 1.000000000000000000, 0.9330127018922194093, 0.9330127018922194093 ) ) 
 REPRESENTATION_ITEM ( '' )  );
#19734=CARTESIAN_POINT ( 'NONE',  ( 159.6773882672717946, 272.2419546184144110, -14.76404975350964044 ) ) ;
#19736=CARTESIAN_POINT ( 'NONE',  ( 207.1211793645798878, 271.9025893473983047, -6.294110402770905388 ) ) ;
#19737=CARTESIAN_POINT ( 'NONE',  ( 10.51348828746337638, 183.0024278399160949, -9.188101187500093303 ) ) ;
#19739=EDGE_LOOP ( 'NONE', ( #48544, #6554, #63263, #17690 ) ) ;
#19743=CARTESIAN_POINT ( 'NONE',  ( 38.60536087060361154, 193.0958772461660544, -9.188101187500095079 ) ) ;
#19744=CARTESIAN_POINT ( 'NONE',  ( 200.6800100461949228, 283.0590218669948399, 18.32402613046234308 ) ) ;
#19745=CARTESIAN_POINT ( 'NONE',  ( 190.9586609929293104, 299.8968923453624598, -4.970176667899034229 ) ) ;
#19747=CARTESIAN_POINT ( 'NONE',  ( 182.4004271739244700, 284.1903799708203451, 16.39187655311515002 ) ) ;
#19748=CARTESIAN_POINT ( 'NONE',  ( 146.5046981847821428, 276.8934145268504494, 0.02269072295920678689 ) ) ;
#19755=CARTESIAN_POINT ( 'NONE',  ( 91.02696109520442747, 213.3615022471902023, 5.000000000000051514 ) ) ;
#19757=LINE ( 'NONE', #64341, #20730 ) ;
#19758=ORIENTED_EDGE ( 'NONE', *, *, #16554, .T. ) ;
#19759=CARTESIAN_POINT ( 'NONE',  ( 41.36564329728401646, 200.8149278399160664, -9.188101187500095079 ) ) ;
#19760=EDGE_LOOP ( 'NONE', ( #49969, #90731, #63613, #81526 ) ) ;
#19762=CARTESIAN_POINT ( 'NONE',  ( 147.4811722709131914, 275.2021117973970377, 3.890385073228495916 ) ) ;
#19764=ORIENTED_EDGE ( 'NONE', *, *, #65996, .F. ) ;
#19765=CARTESIAN_POINT ( 'NONE',  ( 171.3468567556325297, 286.5349138614378148, 7.626544187982161382 ) ) ;
#19766=CARTESIAN_POINT ( 'NONE',  ( 164.9586510554008782, 244.9302305544571823, -1.717556444319656039 ) ) ;
#19769=CARTESIAN_POINT ( 'NONE',  ( 187.4166251561426293, 263.4339899954952102, 11.64397722261905166 ) ) ;
#19771=CARTESIAN_POINT ( 'NONE',  ( 171.5786706455526485, 255.3236219728620711, 12.51996115914846364 ) ) ;
#19776=CARTESIAN_POINT ( 'NONE',  ( 173.8867782663501487, 254.5903856161964995, 8.266592030789951195 ) ) ;
#19778=ORIENTED_EDGE ( 'NONE', *, *, #36453, .T. ) ;
#19779=CARTESIAN_POINT ( 'NONE',  ( 182.3393106838078666, 284.1038920326962511, 14.96556368581471830 ) ) ;
#19780=EDGE_CURVE ( 'NONE', #82018, #55876, #67326, .T. ) ;
#19781=CYLINDRICAL_SURFACE ( 'NONE', #96989, 17.82106496071139645 ) ;
#19782=CARTESIAN_POINT ( 'NONE',  ( -17.42236680055705023, 149.2012482093457777, 0.000000000000000000 ) ) ;
#19784=VERTEX_POINT ( 'NONE', #66199 ) ;
#19785=CARTESIAN_POINT ( 'NONE',  ( 207.4218731373931632, 271.3817724553659332, -5.249531240730909154 ) ) ;
#19786=CARTESIAN_POINT ( 'NONE',  ( 196.6288634187112052, 290.0758136547079289, -16.31544900032282186 ) ) ;
#19787=EDGE_LOOP ( 'NONE', ( #8, #62217, #80012, #53185 ) ) ;
#19788=FACE_OUTER_BOUND ( 'NONE', #39999, .T. ) ;
#19790=CARTESIAN_POINT ( 'NONE',  ( -22.42236680055709641, 157.8615022471902591, 0.000000000000000000 ) ) ;
#19793=CARTESIAN_POINT ( 'NONE',  ( 198.0003830832412461, 286.7757149588804850, 16.94998330638511419 ) ) ;
#19795=CARTESIAN_POINT ( 'NONE',  ( 110.7287787077026451, 243.9244531367911293, -4.594050593750046652 ) ) ;
#19796=CARTESIAN_POINT ( 'NONE',  ( -22.42236680055709641, 157.8615022471902591, 0.000000000000000000 ) ) ;
#19797=CARTESIAN_POINT ( 'NONE',  ( 66.16250339235085676, 220.5530062829863027, -4.648177544792955347E-16 ) ) ;
#19798=ORIENTED_EDGE ( 'NONE', *, *, #89326, .F. ) ;
#19799=CARTESIAN_POINT ( 'NONE',  ( 207.5792673731680793, 271.1091576421853233, 2.359198794924813214 ) ) ;
#19800=VERTEX_POINT ( 'NONE', #42867 ) ;
#19804=CARTESIAN_POINT ( 'NONE',  ( 74.35571174875622091, 222.9244531367911293, -4.594050593750046652 ) ) ;
#19806=CARTESIAN_POINT ( 'NONE',  ( 174.1477614194014336, 281.2887866680289335, 15.61518462008415042 ) ) ;
#19807=CARTESIAN_POINT ( 'NONE',  ( 154.9226727788713731, 262.3130548330639726, 18.22497199616848818 ) ) ;
#19808=CARTESIAN_POINT ( 'NONE',  ( 175.8169107895047034, 278.1165438142045332, 15.85296464203584499 ) ) ;
#19809=VERTEX_POINT ( 'NONE', #43879 ) ;
#19812=CARTESIAN_POINT ( 'NONE',  ( 203.5258219653775313, 278.1299310341851765, -16.21052911601769608 ) ) ;
#19814=CARTESIAN_POINT ( 'NONE',  ( 148.1803270710863103, 273.9911401611413453, 8.879999584410908753 ) ) ;
#19815=CARTESIAN_POINT ( 'NONE',  ( -12.62545442379354554, 163.5177522451418781, -10.00000000000009592 ) ) ;
#19816=CARTESIAN_POINT ( 'NONE',  ( 207.5785076975260779, 271.1104734389944042, -6.824813054587777650 ) ) ;
#19817=CARTESIAN_POINT ( 'NONE',  ( 206.4728825436989155, 270.6102857768882473, 2.384334928751958405 ) ) ;
#19820=CARTESIAN_POINT ( 'NONE',  ( 206.5508451493652444, 272.8904371854448527, 11.05407534521577695 ) ) ;
#19822=CARTESIAN_POINT ( 'NONE',  ( 164.3602934812760452, 245.9666162739349318, -7.171958108566009571 ) ) ;
#19823=CARTESIAN_POINT ( 'NONE',  ( 130.8102634016018442, 237.1423013555409796, -4.594050593750043987 ) ) ;
#19826=CARTESIAN_POINT ( 'NONE',  ( 82.63733999249467388, 228.5177522451419350, 5.000000000000046185 ) ) ;
#19827=CARTESIAN_POINT ( 'NONE',  ( 203.1526193585190470, 278.7763369107815379, -16.67658907091021447 ) ) ;
#19828=CARTESIAN_POINT ( 'NONE',  ( 164.3010377730689981, 246.0692501711882869, 7.247566249275159578 ) ) ;
#19835=CARTESIAN_POINT ( 'NONE',  ( 164.3625597711517230, 265.6729452914248668, -17.82104740451561753 ) ) ;
#19837=CARTESIAN_POINT ( 'NONE',  ( 195.3688130124408531, 263.4455885837858204, 0.8642261836844156164 ) ) ;
#19838=CARTESIAN_POINT ( 'NONE',  ( -13.51183432020139819, 142.4280072687214442, 0.000000000000000000 ) ) ;
#19841=B_SPLINE_CURVE_WITH_KNOTS ( 'NONE', 3,
 ( #94875, #93379, #25437, #55809, #23931, #86802, #71061, #70535, #86301, #54829, #1662, #85813, #16341, #7744, #32546, #63445, #79187, #9764, #40625, #71561, #31035, #80690, #65434, #35023, #19371, #87816, #97360, #42128, #12248, #11752, #58324, #80185, #64444, #49247, #96376, #35531, #56830, #25959 ),
 .UNSPECIFIED., .F., .F.,
 ( 4, 2, 2, 2, 2, 2, 2, 2, 2, 2, 2, 2, 2, 2, 2, 2, 2, 2, 4 ),
 ( 0.0009274247721126415529, 0.001022860814635683565, 0.001118296857158725469, 0.001309168942204771329, 0.001690913112296865868, 0.002454401452480929179, 0.003981378132849053633, 0.004744866473033152940, 0.005126610643125203461, 0.005317482728171264716, 0.005412918770694336544, 0.005508354813217409239, 0.005556072834478982016, 0.005603790855740555660, 0.005699226898263672590, 0.005890098983310050433, 0.006271843153402804384, 0.006653587323495560070, 0.007035331493588314021 ),
 .UNSPECIFIED. ) ;
#19844=CARTESIAN_POINT ( 'NONE',  ( 192.4434358697015739, 296.8713576677063770, 11.08430769131553895 ) ) ;
#19848=CARTESIAN_POINT ( 'NONE',  ( 190.0445576990143195, 301.4801656937889902, 4.140328216824785912 ) ) ;
#19850=CARTESIAN_POINT ( 'NONE',  ( 169.4526480808381450, 285.1936639049519044, -7.980504902024926572 ) ) ;
#19851=CARTESIAN_POINT ( 'NONE',  ( 203.1988451939495235, 268.1137895879253961, -4.180311155435266990 ) ) ;
#19852=CARTESIAN_POINT ( 'NONE',  ( 193.4499168429655924, 288.7348347244117690, 16.02611495321234258 ) ) ;
#19853=CARTESIAN_POINT ( 'NONE',  ( 131.5677753063155251, 246.7677522451418497, 10.00000000000009592 ) ) ;
#19854=CARTESIAN_POINT ( 'NONE',  ( 183.2152767118556085, 278.9959196896102753, 17.30803618819086864 ) ) ;
#19855=ORIENTED_EDGE ( 'NONE', *, *, #6142, .T. ) ;
#19858=CARTESIAN_POINT ( 'NONE',  ( 196.3021893095863959, 290.6416298092292436, 17.45656988653421138 ) ) ;
#19859=CARTESIAN_POINT ( 'NONE',  ( 190.5674408456512765, 300.5745055173924811, -0.9151048603553563199 ) ) ;
#19860=CARTESIAN_POINT ( 'NONE',  ( -8.322217149083147802, 159.8768266524159856, -9.188101187500093303 ) ) ;
#19861=CARTESIAN_POINT ( 'NONE',  ( 39.44458330234355969, 184.3923013555410080, 4.594050593750050204 ) ) ;
#19862=CARTESIAN_POINT ( 'NONE',  ( 175.7888789257961832, 257.1435258631530019, -10.56737597936652584 ) ) ;
#19865=CARTESIAN_POINT ( 'NONE',  ( 205.2937235227012707, 275.0678357141204629, -12.80017165135291535 ) ) ;
#19866=CARTESIAN_POINT ( 'NONE',  ( 192.2926338600964584, 292.9423151340307641, -14.26349443232093961 ) ) ;
#19867=CARTESIAN_POINT ( 'NONE',  ( 147.5693121967435957, 275.0494489676833041, 4.210973343677100189 ) ) ;
#19870=CARTESIAN_POINT ( 'NONE',  ( 63.51261232558833569, 214.1427522451419065, 10.00000000000009237 ) ) ;
#19873=CARTESIAN_POINT ( 'NONE',  ( 150.2452556859942376, 270.4145788861182496, 14.49525683977126533 ) ) ;
#19874=CARTESIAN_POINT ( 'NONE',  ( 38.27158024800227309, 206.2365022471903160, 2.944929066748280225E-16 ) ) ;
#19875=CARTESIAN_POINT ( 'NONE',  ( 182.1377600559704035, 291.7984100848548792, 9.332931847923262580 ) ) ;
#19876=CARTESIAN_POINT ( 'NONE',  ( 163.2442700311756596, 247.8996255919473697, 11.14021925110252020 ) ) ;
#19877=CARTESIAN_POINT ( 'NONE',  ( -1.935626891937928917, 175.8149278399160664, 9.188101187500093303 ) ) ;
#19878=CARTESIAN_POINT ( 'NONE',  ( 168.1818879105967710, 286.4694436765728938, 4.832144866178585296 ) ) ;
#19882=CARTESIAN_POINT ( 'NONE',  ( 165.0308887387863876, 244.8051112166122891, 1.948365933089477808 ) ) ;
#19883=CARTESIAN_POINT ( 'NONE',  ( 183.1920691253360474, 278.9237338132715536, 16.88618025906524167 ) ) ;
#19891=CARTESIAN_POINT ( 'NONE',  ( 153.2378184573828150, 277.6881940163261788, -5.169838279812049464 ) ) ;
#19892=ORIENTED_EDGE ( 'NONE', *, *, #18327, .T. ) ;
#19893=CARTESIAN_POINT ( 'NONE',  ( 112.8139755218393532, 224.3932355074535394, -2.679491924311248496 ) ) ;
#19894=CARTESIAN_POINT ( 'NONE',  ( 206.5237403681858552, 272.9373840435757188, -10.81420335655575116 ) ) ;
#19895=EDGE_CURVE ( 'NONE', #16991, #27498, #41485, .T. ) ;
#19898=CARTESIAN_POINT ( 'NONE',  ( 153.0070714074088016, 265.6309737354857248, 17.74442213480098474 ) ) ;
#19902=ORIENTED_EDGE ( 'NONE', *, *, #40211, .F. ) ;
#19905=CARTESIAN_POINT ( 'NONE',  ( 163.7136804588959649, 247.0865828815331042, 6.783386239354816105 ) ) ;
#19906=CARTESIAN_POINT ( 'NONE',  ( 192.8010417052266234, 296.7057953447782097, 12.10593424093686643 ) ) ;
#19907=ORIENTED_EDGE ( 'NONE', *, *, #13054, .F. ) ;
#19909=CARTESIAN_POINT ( 'NONE',  ( 177.7843144939522517, 263.4642486473027816, 15.38512530093995956 ) ) ;
#19914=AXIS2_PLACEMENT_3D ( 'NONE', #39353, #94118, #56052 ) ;
#19917=CARTESIAN_POINT ( 'NONE',  ( 202.9887705438587773, 268.0958564390360834, 2.511777696352780254 ) ) ;
#19918=CARTESIAN_POINT ( 'NONE',  ( 166.1715776501828543, 274.1767206847245006, -15.18696448220450534 ) ) ;
#19920=ORIENTED_EDGE ( 'NONE', *, *, #25233, .F. ) ;
#19921=CARTESIAN_POINT ( 'NONE',  ( 175.9279835239203180, 278.1198263924018192, -15.71133404561638969 ) ) ;
#19922=CARTESIAN_POINT ( 'NONE',  ( 169.1667396529449263, 261.6176701127336628, -15.97132217662409381 ) ) ;
#19925=CARTESIAN_POINT ( 'NONE',  ( 158.7680870133227700, 267.7863907316387326, -16.24686683248629038 ) ) ;
#19929=CARTESIAN_POINT ( 'NONE',  ( 158.9949979552652621, 259.7205239824713203, 16.79231500460955573 ) ) ;
#19930=CARTESIAN_POINT ( 'NONE',  ( 193.2853656402591014, 295.8669216819805001, 14.14801835725165091 ) ) ;
#19931=CARTESIAN_POINT ( 'NONE',  ( 188.6236154063645643, 298.5688366442050210, -4.386709406375833176 ) ) ;
#19933=CARTESIAN_POINT ( 'NONE',  ( 192.6773196027083372, 296.9200883123592689, 11.15745042875121484 ) ) ;
#19934=CARTESIAN_POINT ( 'NONE',  ( 177.6619337662969258, 291.1046247341686239, 6.079945615520735203 ) ) ;
#19935=CARTESIAN_POINT ( 'NONE',  ( 196.9886126479698305, 289.4527097116482537, -17.08115356036521604 ) ) ;
#19939=CARTESIAN_POINT ( 'NONE',  ( 173.9076247008792393, 277.9417859016587045, -16.84130823774900776 ) ) ;
#19940=DIRECTION ( 'NONE',  ( 0.4999999999999992784, -0.8660254037844390407, 0.000000000000000000 ) ) ;
#19943=CARTESIAN_POINT ( 'NONE',  ( 184.7289685188066528, 275.5467696374773254, 16.39282505805186574 ) ) ;
#19944=CARTESIAN_POINT ( 'NONE',  ( 171.5470852890824744, 259.4466874145439306, -13.88548382802202319 ) ) ;
#19945=CARTESIAN_POINT ( 'NONE',  ( 187.1602505332256214, 299.4194354331692693, 0.8643973265446426302 ) ) ;
#19946=CARTESIAN_POINT ( 'NONE',  ( 173.4026771546767804, 273.2456497557084845, -17.70700034978624515 ) ) ;
#19947=CARTESIAN_POINT ( 'NONE',  ( 159.9741193159504746, 253.5636927791250059, -15.97707229450967503 ) ) ;
#19948=CARTESIAN_POINT ( 'NONE',  ( 190.3209390717459542, 301.0014591139522508, -1.435067967167677594 ) ) ;
#19950=CARTESIAN_POINT ( 'NONE',  ( 169.4525966125490584, 254.8330656995144636, -11.66724334959756604 ) ) ;
#19952=CARTESIAN_POINT ( 'NONE',  ( 128.9696990949622091, 245.2677522451418497, 10.00000000000009592 ) ) ;
#19953=CARTESIAN_POINT ( 'NONE',  ( 164.3138894970802824, 246.0469903322357368, -2.642126690130961020 ) ) ;
#19954=CARTESIAN_POINT ( 'NONE',  ( 22.88158713136840561, 194.0177522451419350, 5.000000000000046185 ) ) ;
#19955=CARTESIAN_POINT ( 'NONE',  ( 94.81556191316359161, 234.7369531367911009, -4.594050593750048428 ) ) ;
#19957=CARTESIAN_POINT ( 'NONE',  ( 162.9352708800131779, 249.6521066053614391, -11.39866856991230293 ) ) ;
#19959=CARTESIAN_POINT ( 'NONE',  ( 207.8018416422513894, 270.7236476996756664, 1.610379135119299754 ) ) ;
#19960=CARTESIAN_POINT ( 'NONE',  ( 31.32559514186443295, 179.7048013555409796, 4.594050593750051981 ) ) ;
#19962=CARTESIAN_POINT ( 'NONE',  ( 172.7519013077862269, 288.3158815880753423, -8.994867566259873826 ) ) ;
#19966=CARTESIAN_POINT ( 'NONE',  ( 147.4872062048032433, 275.6374356566055326, -0.2721491379029486457 ) ) ;
#19969=DIRECTION ( 'NONE',  ( 0.4999999999999998335, -0.8660254037844388186, 0.000000000000000000 ) ) ;
#19970=CARTESIAN_POINT ( 'NONE',  ( 161.3145230519951951, 251.2420454056404822, -14.44869077440025151 ) ) ;
#19973=CARTESIAN_POINT ( 'NONE',  ( 53.49034604603116350, 195.5643266524159856, 9.188101187500095079 ) ) ;
#19974=CARTESIAN_POINT ( 'NONE',  ( 86.89529822776817980, 227.6427522451419065, 10.00000000000009237 ) ) ;
#19976=ADVANCED_FACE ( 'NONE', ( #13992 ), #60561, .T. ) ;
#19977=CARTESIAN_POINT ( 'NONE',  ( 198.0324241745848042, 267.8073025728403422, -7.956821422782448749 ) ) ;
#19978=B_SPLINE_CURVE_WITH_KNOTS ( 'NONE', 3,
 ( #19663, #59104, #96183, #97179, #57124, #42904, #3465, #89590, #5441, #36324, #4434, #35332, #13060, #74371 ),
 .UNSPECIFIED., .F., .F.,
 ( 4, 2, 2, 2, 2, 2, 4 ),
 ( 2.941618428806969512E-15, 0.0005114949209976904715, 0.001022989841992439286, 0.001278737302489847466, 0.001534484762987255646, 0.001790232223484663826, 0.002045979683982072223 ),
 .UNSPECIFIED. ) ;
#19979=CARTESIAN_POINT ( 'NONE',  ( 3.462723837431157747, 161.2592609112380160, 2.679491924311254714 ) ) ;
#19980=CARTESIAN_POINT ( 'NONE',  ( 5.669592554750444435, 164.8923013555410080, 4.594050593750050204 ) ) ;
#19981=CARTESIAN_POINT ( 'NONE',  ( 181.7327785741209141, 287.1345269289352586, -14.84312672137237143 ) ) ;
#19983=CARTESIAN_POINT ( 'NONE',  ( 193.2100161762185735, 295.9974307820218087, -12.46499585622781758 ) ) ;
#19984=CARTESIAN_POINT ( 'NONE',  ( 163.7323023463233937, 247.0543288263758086, -6.244751637846886361 ) ) ;
#19987=CARTESIAN_POINT ( 'NONE',  ( 164.3706594650489023, 245.9486618633701482, -1.665857659249071698 ) ) ;
#19988=EDGE_CURVE ( 'NONE', #62997, #28370, #94598, .T. ) ;
#19990=CARTESIAN_POINT ( 'NONE',  ( -1.565588326081831072, 163.2365022471902023, 10.00000000000009592 ) ) ;
#19991=B_SPLINE_CURVE_WITH_KNOTS ( 'NONE', 3,
 ( #72562, #56825, #33541, #64940, #81667, #95885, #65427, #3646, #26446, #35524, #18848, #88797, #19365, #50224, #81179, #11745, #80684, #87809, #42608, #74042, #11259, #96874, #12241, #35017, #42121, #97354, #73053, #43099, #18349, #49242, #65918, #34528, #41619, #10743, #80177, #58803, #27442, #3166, #58317, #4630, #66424, #34051, #17849, #48750 ),
 .UNSPECIFIED., .F., .F.,
 ( 4, 2, 2, 2, 2, 2, 2, 2, 2, 2, 2, 2, 2, 2, 2, 2, 2, 2, 2, 2, 2, 4 ),
 ( 0.002247607324231777268, 0.002678942405538197770, 0.002894609946191499528, 0.003002443716518150407, 0.003110277486844801285, 0.003218111257171452164, 0.003325945027498102610, 0.003541612568151359264, 0.003972947649457884284, 0.004835617812070935190, 0.005698287974683985228, 0.006560958137297035267, 0.006992293218603561587, 0.007423628299910086173, 0.007531462070236681974, 0.007585378955399979008, 0.007639295840563276908, 0.007747129610889857097, 0.007854963381216436419, 0.008286298462522705133, 0.008717633543828975581, 0.009148968625135313684 ),
 .UNSPECIFIED. ) ;
#19994=CARTESIAN_POINT ( 'NONE',  ( 123.0967907794404113, 248.0024278399161517, 9.188101187500095079 ) ) ;
#19996=CARTESIAN_POINT ( 'NONE',  ( 164.3429939525221926, 245.9965799366839008, 1.284743659783852188 ) ) ;
#19997=CARTESIAN_POINT ( 'NONE',  ( 181.5281250038626979, 294.0940755821732751, -7.844796568590651553 ) ) ;
#19999=CARTESIAN_POINT ( 'NONE',  ( 196.4351339088274813, 290.4113630087520050, 17.20526457544535504 ) ) ;
#20003=CARTESIAN_POINT ( 'NONE',  ( 150.6931560952953646, 269.6387926204777727, 14.65021044537114037 ) ) ;
#20004=CARTESIAN_POINT ( 'NONE',  ( 163.8130561957613338, 246.9144590562426629, 7.378237555415944726 ) ) ;
#20012=ADVANCED_FACE ( 'NONE', ( #84422 ), #52831, .F. ) ;
#20015=CARTESIAN_POINT ( 'NONE',  ( 196.7494297999078867, 271.1026102776716016, 12.03499651395464376 ) ) ;
#20016=CARTESIAN_POINT ( 'NONE',  ( 181.9526327277720839, 295.0417315924539707, 4.810195558377932556 ) ) ;
#20019=EDGE_CURVE ( 'NONE', #75682, #35189, #49665, .T. ) ;
#20020=( BOUNDED_CURVE ( )  B_SPLINE_CURVE ( 2, ( #37995, #61801, #68908, #15199, #99833, #30417, #61307, #92269, #22817 ),
 .UNSPECIFIED., .F., .T. ) 
 B_SPLINE_CURVE_WITH_KNOTS ( ( 3, 2, 2, 2, 3 ),
 ( 0.2217741935483870941, 0.2231182795698924692, 0.2258064516129032195, 0.2284946236559139698, 0.2298387096774193450 ),
 .UNSPECIFIED. ) 
 CURVE ( )  GEOMETRIC_REPRESENTATION_ITEM ( )  RATIONAL_B_SPLINE_CURVE ( ( 0.9330127018922194093, 0.9330127018922194093, 1.000000000000000000, 0.8660254037844387076, 1.000000000000000000, 0.8660254037844387076, 1.000000000000000000, 0.9330127018922194093, 0.9330127018922194093 ) ) 
 REPRESENTATION_ITEM ( '' )  );
#20022=DIRECTION ( 'NONE',  ( 0.4999999999999998890, -0.8660254037844385966, 0.000000000000000000 ) ) ;
#20024=CARTESIAN_POINT ( 'NONE',  ( 192.0180279664021157, 287.5583705255741052, -16.23921153416872087 ) ) ;
#20026=CARTESIAN_POINT ( 'NONE',  ( -22.42236680055709641, 157.8615022471902591, 0.000000000000000000 ) ) ;
#20027=CARTESIAN_POINT ( 'NONE',  ( 147.6508870500795467, 274.9081571770856272, -8.950912509993816712 ) ) ;
#20028=CARTESIAN_POINT ( 'NONE',  ( 156.3551087084618700, 261.3239775484371989, -17.56576820129662053 ) ) ;
#20030=FACE_OUTER_BOUND ( 'NONE', #22685, .T. ) ;
#20031=EDGE_CURVE ( 'NONE', #85466, #46359, #84829, .T. ) ;
#20033=B_SPLINE_CURVE_WITH_KNOTS ( 'NONE', 3,
 ( #59553, #15957, #16950, #47839 ),
 .UNSPECIFIED., .F., .F.,
 ( 4, 4 ),
 ( 0.03953143252384128115, 0.04799691715800366576 ),
 .UNSPECIFIED. ) ;
#20034=DIRECTION ( 'NONE',  ( 0.4999999999999998890, -0.8660254037844385966, 0.000000000000000000 ) ) ;
#20035=ORIENTED_EDGE ( 'NONE', *, *, #38829, .T. ) ;
#20036=CARTESIAN_POINT ( 'NONE',  ( 79.98487687335507701, 226.1744531367911293, 4.594050593750047540 ) ) ;
#20037=CARTESIAN_POINT ( 'NONE',  ( 202.9996883242178569, 279.0412212322449932, 16.31748462427307089 ) ) ;
#20039=CARTESIAN_POINT ( 'NONE',  ( 185.0987280534011177, 259.9520638838685613, -6.416371529008482177 ) ) ;
#20043=ORIENTED_EDGE ( 'NONE', *, *, #62049, .F. ) ;
#20044=CARTESIAN_POINT ( 'NONE',  ( 207.3873553355473121, 271.0594493704188039, 2.178264502744591269 ) ) ;
#20045=VERTEX_POINT ( 'NONE', #27595 ) ;
#20046=CARTESIAN_POINT ( 'NONE',  ( 192.6299325303148464, 294.0530281384722002, 14.39848446519248704 ) ) ;
#20047=VERTEX_POINT ( 'NONE', #51879 ) ;
#20053=CARTESIAN_POINT ( 'NONE',  ( 152.1113819699424425, 268.9580029282372493, 15.28343548679968933 ) ) ;
#20057=CARTESIAN_POINT ( 'NONE',  ( 136.3847812948166336, 258.7369531367911009, -4.594050593750048428 ) ) ;
#20065=VERTEX_POINT ( 'NONE', #36158 ) ;
#20067=CARTESIAN_POINT ( 'NONE',  ( 181.8509774751104544, 266.9677320091309412, 16.09658033613713712 ) ) ;
#20068=CARTESIAN_POINT ( 'NONE',  ( 120.6060784269860449, 251.9860189848785410, -2.679491924311252493 ) ) ;
#20079=EDGE_LOOP ( 'NONE', ( #64489, #56886, #60875, #34331, #6430, #15961, #54366, #62151, #52164, #31867, #25494, #91192, #83650, #29870, #30095, #23626, #74244, #26299, #71852, #19798, #79958, #55050 ) ) ;
#20080=CARTESIAN_POINT ( 'NONE',  ( 159.9983927609781063, 276.8049897941343716, 13.27407150049416806 ) ) ;
#20084=CARTESIAN_POINT ( 'NONE',  ( 164.7647380297938184, 248.9862001899016946, 10.10785415616959071 ) ) ;
#20085=CARTESIAN_POINT ( 'NONE',  ( 164.6081132108126326, 274.3788087673100904, 14.77367721212278084 ) ) ;
#20086=CARTESIAN_POINT ( 'NONE',  ( 161.2908438277387972, 281.6436246679302258, -7.517958113851705981 ) ) ;
#20089=CARTESIAN_POINT ( 'NONE',  ( 160.1764156583825525, 261.1444413449148101, 17.72707215100685829 ) ) ;
#20091=B_SPLINE_SURFACE_WITH_KNOTS ( 'NONE', 3, 1, ( 
 ( #97178, #51022 ),
 ( #65723, #21154 ),
 ( #42419, #73844 ),
 ( #80995, #19662 ),
 ( #27745, #67225 ),
 ( #58614, #52033 ),
 ( #98152, #28735 ),
 ( #20154, #13548 ),
 ( #67733, #89589 ),
 ( #82973, #81974 ),
 ( #91072, #27248 ),
 ( #44420, #12551 ),
 ( #51532, #43424 ),
 ( #58131, #98656 ),
 ( #75350, #73352 ),
 ( #74370, #4953 ),
 ( #5930, #20644 ),
 ( #13059, #59609 ),
 ( #97661, #28229 ),
 ( #59103, #3940 ),
 ( #50524, #90075 ),
 ( #29240, #43919 ),
 ( #60106, #74858 ),
 ( #92561, #77326 ),
 ( #44911, #45895 ),
 ( #22627, #62601 ),
 ( #38305, #16018 ),
 ( #37315, #93555 ),
 ( #69713, #38807 ),
 ( #7933, #30728 ),
 ( #92079, #321 ),
 ( #31211, #62097 ),
 ( #815, #53513 ),
 ( #23600, #8422 ) ),
 .UNSPECIFIED., .T., .F., .F.,
 ( 4, 2, 2, 2, 2, 2, 2, 2, 2, 2, 2, 2, 2, 2, 2, 2, 4 ),
 ( 2, 2 ),
 ( 0.000000000000000000, 0.06250000000000000000, 0.1250000000000000000, 0.1875000000000000000, 0.2500000000000000000, 0.3125000000000000000, 0.3750000000000000000, 0.4375000000000000000, 0.5000000000000000000, 0.5625000000000000000, 0.6250000000000000000, 0.6875000000000000000, 0.7500000000000000000, 0.8125000000000000000, 0.8750000000000000000, 0.9375000000000000000, 1.000000000000000000 ),
 ( 0.000000000000000000, 1.000000000000000000 ),
 .UNSPECIFIED. ) ;
#20097=CARTESIAN_POINT ( 'NONE',  ( 184.6885808911535207, 260.6528513612950064, 10.31057805081157852 ) ) ;
#20100=CARTESIAN_POINT ( 'NONE',  ( 12.78715206816254302, 172.0643266524160140, -9.188101187500093303 ) ) ;
#20101=CARTESIAN_POINT ( 'NONE',  ( 102.5290345353249961, 223.8768266524159856, 9.188101187500098632 ) ) ;
#20102=CARTESIAN_POINT ( 'NONE',  ( 155.1601726304954809, 261.9016930232608615, -18.56587418422714464 ) ) ;
#20103=CARTESIAN_POINT ( 'NONE',  ( 40.63510790894940072, 204.2677522451419350, -5.000000000000047962 ) ) ;
#20104=CARTESIAN_POINT ( 'NONE',  ( 186.7158489563707064, 295.8341147379624090, -7.679202307086533175 ) ) ;
#20105=EDGE_CURVE ( 'NONE', #62030, #56261, #18231, .T. ) ;
#20109=CARTESIAN_POINT ( 'NONE',  ( 147.6054094044680198, 274.9869267698931594, -8.596541856229405809 ) ) ;
#20113=CARTESIAN_POINT ( 'NONE',  ( 166.1070111784138703, 253.4115428555481344, -13.60050710122670559 ) ) ;
#20116=CARTESIAN_POINT ( 'NONE',  ( 72.86731735994297310, 219.0024278399160664, -9.188101187500093303 ) ) ;
#20117=CARTESIAN_POINT ( 'NONE',  ( 161.8150574665248200, 250.3750943687383881, -13.25074899737357903 ) ) ;
#20119=CARTESIAN_POINT ( 'NONE',  ( 195.7578697689113199, 291.5844189092309193, 17.18796537138345215 ) ) ;
#20121=CARTESIAN_POINT ( 'NONE',  ( 199.1867231605587278, 285.6454706231928071, -17.41989184023605475 ) ) ;
#20130=CARTESIAN_POINT ( 'NONE',  ( 57.17980156396255609, 210.4865022471903160, 10.00000000000009415 ) ) ;
#20134=AXIS2_PLACEMENT_3D ( 'NONE', #96404, #34562, #19399 ) ;
#20135=CARTESIAN_POINT ( 'NONE',  ( 157.5205412249731012, 268.7636797464979281, 15.65110165726261293 ) ) ;
#20136=CARTESIAN_POINT ( 'NONE',  ( 189.5059428776464756, 300.4130739301078279, -3.423561384717671796 ) ) ;
#20138=CARTESIAN_POINT ( 'NONE',  ( 131.6579862894242865, 253.4865022471903444, -10.00000000000009415 ) ) ;
#20139=CARTESIAN_POINT ( 'NONE',  ( 157.4211152037729562, 257.9856256133486454, -16.71526195140576831 ) ) ;
#20144=CARTESIAN_POINT ( 'NONE',  ( 188.7258768753199831, 272.5327203015561395, 16.40358330166877465 ) ) ;
#20146=CARTESIAN_POINT ( 'NONE',  ( 196.4030970371012472, 264.3490001850324234, -4.693669024083267693 ) ) ;
#20148=VERTEX_POINT ( 'NONE', #7760 ) ;
#20151=VERTEX_POINT ( 'NONE', #24458 ) ;
#20152=CARTESIAN_POINT ( 'NONE',  ( 192.8546065288647924, 292.4362985693752535, 15.15881306499927916 ) ) ;
#20154=CARTESIAN_POINT ( 'NONE',  ( 205.5299317431642692, 274.6587110751127625, 11.78078220685493882 ) ) ;
#20155=CARTESIAN_POINT ( 'NONE',  ( 148.9967968810750563, 247.6423013555410080, -4.594050593750043987 ) ) ;
#20156=CARTESIAN_POINT ( 'NONE',  ( 204.8874959148301400, 273.6675085671400325, 10.84287252419124492 ) ) ;
#20157=CARTESIAN_POINT ( 'NONE',  ( 153.2583947049096764, 265.1956690150883560, -17.64103123457563882 ) ) ;
#20161=CARTESIAN_POINT ( 'NONE',  ( 176.3865323452404823, 258.8737835494043225, 13.24306684835586623 ) ) ;
#20162=CARTESIAN_POINT ( 'NONE',  ( 173.9008529106967558, 272.4049662731551962, -17.79092985220220058 ) ) ;
#20165=CARTESIAN_POINT ( 'NONE',  ( 183.0159800400793983, 295.9215593239155169, 0.5241057615201285547 ) ) ;
#20167=CARTESIAN_POINT ( 'NONE',  ( 163.7239493340838123, 247.0687966679708438, 6.286946239157660266 ) ) ;
#20168=CARTESIAN_POINT ( 'NONE',  ( 162.8751945631634612, 272.8900720096677333, -16.40198242748087054 ) ) ;
#20170=CARTESIAN_POINT ( 'NONE',  ( 166.4873690803768795, 248.5196436787675225, -7.973532822608550674 ) ) ;
#20171=CARTESIAN_POINT ( 'NONE',  ( 159.9449220377261440, 283.7382459705826818, 0.01809001837185298528 ) ) ;
#20174=CARTESIAN_POINT ( 'NONE',  ( 169.8297681824042513, 267.4479351203237911, 17.31714983691947651 ) ) ;
#20175=CARTESIAN_POINT ( 'NONE',  ( 181.9516171695871378, 256.9925793098663007, 5.069001809681082271 ) ) ;
#20176=CARTESIAN_POINT ( 'NONE',  ( 97.06207562605321471, 226.8458772461660544, 9.188101187500095079 ) ) ;
#20180=CARTESIAN_POINT ( 'NONE',  ( 163.0851559127074495, 276.7488112146713206, -14.21592638994824576 ) ) ;
#20182=ORIENTED_EDGE ( 'NONE', *, *, #56931, .F. ) ;
#20184=CARTESIAN_POINT ( 'NONE',  ( 178.7254881896226948, 292.9730135732680765, -2.650317027749069076 ) ) ;
#20185=CARTESIAN_POINT ( 'NONE',  ( 157.2333142128019858, 258.3109064714224132, 16.87956768598436597 ) ) ;
#20189=VERTEX_POINT ( 'NONE', #94894 ) ;
#20190=CARTESIAN_POINT ( 'NONE',  ( 184.7531445739716105, 265.1985052118166095, -14.31512252865175050 ) ) ;
#20193=CARTESIAN_POINT ( 'NONE',  ( 194.4117352900907747, 266.1848707878391451, -7.745729181019060938 ) ) ;
#20194=CARTESIAN_POINT ( 'NONE',  ( 23.47697960001819695, 174.3615022471901739, 5.000000000000051514 ) ) ;
#20196=CARTESIAN_POINT ( 'NONE',  ( 130.0789470495699618, 258.1589784336661637, -6.496448406907675876E-16 ) ) ;
#20199=VERTEX_POINT ( 'NONE', #71579 ) ;
#20200=CARTESIAN_POINT ( 'NONE',  ( 190.3286155001717930, 300.9881631498979004, -5.624828231725103045 ) ) ;
#20203=CARTESIAN_POINT ( 'NONE',  ( 170.2114099174445698, 248.6575072932782575, -0.2697646958337756029 ) ) ;
#20206=CARTESIAN_POINT ( 'NONE',  ( 195.5083716432090171, 279.7078053236261894, -16.99617889076117905 ) ) ;
#20207=CARTESIAN_POINT ( 'NONE',  ( -22.42236680055709641, 157.8615022471902591, 0.000000000000000000 ) ) ;
#20209=CARTESIAN_POINT ( 'NONE',  ( 206.7852059338757158, 271.6495446167011778, 6.263730558154075645 ) ) ;
#20210=CARTESIAN_POINT ( 'NONE',  ( 159.6962080797732710, 254.0450491601782232, -15.33973334987084947 ) ) ;
#20212=CARTESIAN_POINT ( 'NONE',  ( 207.5886452961740076, 271.0929146030698007, -1.661373005306138184 ) ) ;
#20214=EDGE_CURVE ( 'NONE', #48247, #54626, #59626, .T. ) ;
#20215=B_SPLINE_CURVE_WITH_KNOTS ( 'NONE', 3,
 ( #60565, #38773, #53963, #45860, #76784, #83933, #15465, #29691, #45379, #21600, #30185, #30692, #77288, #7378, #14497, #283, #69679, #37284, #61572, #38265, #6884, #91522, #39258, #93010, #15982, #23564, #29204, #52482, #13995, #44875, #75815, #37773, #6399, #99605, #61071, #92041, #16481, #94522, #26095, #63081, #64594, #25074, #18499, #55954, #80330, #63580, #33185, #78300, #64085, #78800, #79828, #87467 ),
 .UNSPECIFIED., .F., .F.,
 ( 4, 2, 2, 2, 2, 2, 2, 2, 2, 2, 2, 2, 2, 2, 2, 2, 2, 2, 2, 2, 2, 2, 2, 2, 2, 4 ),
 ( 0.0001011000311972802914, 0.001124998771331816661, 0.001380973456365458627, 0.001636948141399100377, 0.001764935483915945754, 0.001892922826432790915, 0.002020910168949636293, 0.002148897511466481454, 0.002404872196500165270, 0.002660846881533849954, 0.003172796251601219322, 0.004196694991736034386, 0.005220593731870849449, 0.005732543101938256114, 0.005988517786971918680, 0.006116505129488747361, 0.006244492472005574307, 0.006308486143264019873, 0.006372479814522463704, 0.006500467157039355702, 0.006756441842073139699, 0.007012416527106922828, 0.007268391212140705958, 0.007524365897174489087, 0.007780340582208273084, 0.008292289952275735260 ),
 .UNSPECIFIED. ) ;
#20218=CARTESIAN_POINT ( 'NONE',  ( 185.8360385916904534, 265.6419344405306902, 13.25022526328142902 ) ) ;
#20220=ADVANCED_FACE ( 'NONE', ( #1679 ), #37462, .F. ) ;
#20223=CARTESIAN_POINT ( 'NONE',  ( -22.42236680055709641, 157.8615022471902591, 0.000000000000000000 ) ) ;
#20226=EDGE_CURVE ( 'NONE', #86016, #67131, #18553, .T. ) ;
#20227=CARTESIAN_POINT ( 'NONE',  ( 8.294124642383250645, 187.8464784336662206, 1.353441290958777327E-15 ) ) ;
#20228=CARTESIAN_POINT ( 'NONE',  ( 42.77981749017101976, 207.0530062829863311, -4.648177544792955347E-16 ) ) ;
#20233=CARTESIAN_POINT ( 'NONE',  ( 29.51209413086700906, 187.8458772461660544, 9.188101187500095079 ) ) ;
#20237=CARTESIAN_POINT ( 'NONE',  ( 190.7403173041394950, 300.2750747078583800, -4.254144485856557800 ) ) ;
#20239=CARTESIAN_POINT ( 'NONE',  ( 200.2679923989394695, 268.3464411988675238, -6.479517804580061657 ) ) ;
#20240=CARTESIAN_POINT ( 'NONE',  ( 178.8232363120552009, 293.8514986339519055, 2.698715758866663705 ) ) ;
#20241=CARTESIAN_POINT ( 'NONE',  ( 177.5665759502285539, 275.7863988818428993, 17.69313789786682989 ) ) ;
#20242=CARTESIAN_POINT ( 'NONE',  ( 181.3268249587086416, 279.4937579209391743, -16.12903209385025249 ) ) ;
#20244=CARTESIAN_POINT ( 'NONE',  ( 92.59663213601581333, 214.2677522451417929, -5.000000000000041744 ) ) ;
#20245=CARTESIAN_POINT ( 'NONE',  ( 155.6413013457028001, 278.6139379961560394, 8.732707396284567380 ) ) ;
#20246=CARTESIAN_POINT ( 'NONE',  ( 100.4810717531845654, 215.4865022471901455, 1.119607411625061291E-15 ) ) ;
#20249=CARTESIAN_POINT ( 'NONE',  ( 161.6503117857367329, 267.7950018264848495, -17.32522542692637657 ) ) ;
#20251=CARTESIAN_POINT ( 'NONE',  ( 58.09093245575348874, 204.3458772461660544, 9.188101187500095079 ) ) ;
#20253=CARTESIAN_POINT ( 'NONE',  ( 177.1347673595945764, 262.9921672455169528, 15.53478677465993485 ) ) ;
#20256=VERTEX_POINT ( 'NONE', #22724 ) ;
#20258=CARTESIAN_POINT ( 'NONE',  ( 164.9836323268835940, 244.8869617230113249, -2.696511969808454534 ) ) ;
#20262=CARTESIAN_POINT ( 'NONE',  ( 185.7308318325395646, 263.1015815296372011, 11.16513425297995177 ) ) ;
#20264=CARTESIAN_POINT ( 'NONE',  ( 205.0957184426459321, 275.4107905729332515, 13.78964280781899632 ) ) ;
#20268=CARTESIAN_POINT ( 'NONE',  ( 175.0005702576303008, 255.0550677227203948, 8.001073647505871023 ) ) ;
#20273=CARTESIAN_POINT ( 'NONE',  ( 150.7530568467738590, 269.5350414755053521, 15.60317050893315916 ) ) ;
#20274=CARTESIAN_POINT ( 'NONE',  ( 159.2186641046529303, 254.8721795879351646, -15.96198087403305443 ) ) ;
#20277=CARTESIAN_POINT ( 'NONE',  ( 161.1093323826042933, 251.5974460702646809, -13.93502574894237078 ) ) ;
#20279=CARTESIAN_POINT ( 'NONE',  ( 149.2223635749290622, 272.1862799931444670, -12.97307652490353647 ) ) ;
#20282=CARTESIAN_POINT ( 'NONE',  ( 197.8977219949227049, 287.8780861330898801, 17.48564646125164046 ) ) ;
#20283=CARTESIAN_POINT ( 'NONE',  ( 204.6785851723931557, 274.1332865905380913, -12.34137688749581407 ) ) ;
#20285=CARTESIAN_POINT ( 'NONE',  ( 112.6237299221286321, 226.6423013555409796, -4.594050593750043987 ) ) ;
#20286=CARTESIAN_POINT ( 'NONE',  ( 122.2038756314442054, 231.3615022471901739, 5.000000000000051514 ) ) ;
#20287=CARTESIAN_POINT ( 'NONE',  ( 117.0077232087375734, 228.3615022471901739, 5.000000000000051514 ) ) ;
#20289=CARTESIAN_POINT ( 'NONE',  ( 207.5195222358739784, 271.2126392554839640, 2.810970398613041432 ) ) ;
#20293=LINE ( 'NONE', #28373, #64481 ) ;
#20294=CARTESIAN_POINT ( 'NONE',  ( 67.67116493723634107, 216.0024278399160380, -9.188101187500093303 ) ) ;
#20299=CARTESIAN_POINT ( 'NONE',  ( 172.4859759874162819, 276.8588516960780339, 15.79461614666721658 ) ) ;
#20302=( BOUNDED_CURVE ( )  B_SPLINE_CURVE ( 2, ( #92010, #59541, #92488, #82909, #67661, #14467, #53928, #13967, #13481 ),
 .UNSPECIFIED., .F., .T. ) 
 B_SPLINE_CURVE_WITH_KNOTS ( ( 3, 2, 2, 2, 3 ),
 ( 0.2137096774193548432, 0.2150537634408602183, 0.2177419354838709686, 0.2204301075268817189, 0.2217741935483870941 ),
 .UNSPECIFIED. ) 
 CURVE ( )  GEOMETRIC_REPRESENTATION_ITEM ( )  RATIONAL_B_SPLINE_CURVE ( ( 0.9330127018922194093, 0.9330127018922194093, 1.000000000000000000, 0.8660254037844387076, 1.000000000000000000, 0.8660254037844387076, 1.000000000000000000, 0.9330127018922194093, 0.9330127018922194093 ) ) 
 REPRESENTATION_ITEM ( '' )  );
#20305=CARTESIAN_POINT ( 'NONE',  ( 153.4495116231415750, 264.8646448025247082, -16.73555355292144498 ) ) ;
#20306=CARTESIAN_POINT ( 'NONE',  ( 155.2922060645262263, 261.6730044072216401, -16.98884022075611355 ) ) ;
#20310=CARTESIAN_POINT ( 'NONE',  ( 163.7477501808002103, 260.3652044488483739, -16.17942866797859836 ) ) ;
#20312=CARTESIAN_POINT ( 'NONE',  ( 178.3623428208658197, 294.2551730570217501, -1.850815590806885735 ) ) ;
#20313=CARTESIAN_POINT ( 'NONE',  ( 188.5189276119756698, 259.3703232174731852, -3.088365542045595991 ) ) ;
#20315=CARTESIAN_POINT ( 'NONE',  ( 148.9285945872975390, 272.6951028054104427, -12.01265727652413240 ) ) ;
#20318=CARTESIAN_POINT ( 'NONE',  ( 164.4698008747318738, 245.7769439046653019, -6.272955660526681854 ) ) ;
#20319=CARTESIAN_POINT ( 'NONE',  ( 125.2075541532825014, 255.3464784336661353, 1.353441290958777327E-15 ) ) ;
#20326=CARTESIAN_POINT ( 'NONE',  ( 204.3574891606595827, 276.6894411969685166, 13.41627538812899978 ) ) ;
#20329=ORIENTED_EDGE ( 'NONE', *, *, #541, .F. ) ;
#20331=CARTESIAN_POINT ( 'NONE',  ( 123.7735466722555628, 242.2677522451418497, 10.00000000000009592 ) ) ;
#20334=CARTESIAN_POINT ( 'NONE',  ( 198.5140642857193711, 266.2478974292683915, 0.8911030639010785181 ) ) ;
#20336=CARTESIAN_POINT ( 'NONE',  ( 175.1250016605062285, 291.8388325744778058, -4.493358603852836808 ) ) ;
#20337=CARTESIAN_POINT ( 'NONE',  ( 192.8304677249058727, 268.4476542952539262, 12.38602397553101397 ) ) ;
#20338=EDGE_CURVE ( 'NONE', #60492, #23235, #49936, .T. ) ;
#20340=CARTESIAN_POINT ( 'NONE',  ( 149.2561433752359505, 272.1277716627430436, 12.99353668144589946 ) ) ;
#20341=CYLINDRICAL_SURFACE ( 'NONE', #32104, 10.00000000000010658 ) ;
#20343=CARTESIAN_POINT ( 'NONE',  ( 203.2369479875374623, 278.6302754407888074, -16.66242713208754367 ) ) ;
#20345=CARTESIAN_POINT ( 'NONE',  ( 161.3777720748676643, 251.1324948844963387, 14.05949999684680307 ) ) ;
#20346=CARTESIAN_POINT ( 'NONE',  ( 135.3927208396968354, 235.6427522451417360, 1.119607411625061291E-15 ) ) ;
#20347=EDGE_CURVE ( 'NONE', #28481, #82871, #98428, .T. ) ;
#20348=CARTESIAN_POINT ( 'NONE',  ( 172.3600298132898843, 283.6594854551991034, -12.44358114520080960 ) ) ;
#20349=VERTEX_POINT ( 'NONE', #29876 ) ;
#20350=EDGE_CURVE ( 'NONE', #36629, #9601, #22116, .T. ) ;
#20353=CARTESIAN_POINT ( 'NONE',  ( 199.0363797504450929, 285.9058730480928716, -17.12190301149298222 ) ) ;
#20354=CARTESIAN_POINT ( 'NONE',  ( 0.9332558059805314832, 171.3458772461660544, 9.188101187500095079 ) ) ;
#20355=CARTESIAN_POINT ( 'NONE',  ( 59.55252387252222945, 199.0643266524159856, -9.188101187500093303 ) ) ;
#20359=CARTESIAN_POINT ( 'NONE',  ( 157.1269483542914998, 258.4951375425532092, -17.15328932028234377 ) ) ;
#20362=CARTESIAN_POINT ( 'NONE',  ( 167.5986172622920662, 256.5940544082843644, 13.72151094899553847 ) ) ;
#20363=CARTESIAN_POINT ( 'NONE',  ( 180.9290680551475532, 256.0398517639778220, 1.989246424408670499 ) ) ;
#20364=CARTESIAN_POINT ( 'NONE',  ( 198.6859012307616581, 286.5129196511462624, 18.23225590904412030 ) ) ;
#20365=CARTESIAN_POINT ( 'NONE',  ( 179.1279496731769996, 294.4181628194133395, 1.067429419934537105 ) ) ;
#20366=CARTESIAN_POINT ( 'NONE',  ( 52.48883062679681899, 211.1115022471903444, -5.000000000000047962 ) ) ;
#20367=FACE_OUTER_BOUND ( 'NONE', #84589, .T. ) ;
#20368=EDGE_CURVE ( 'NONE', #2785, #35157, #81010, .T. ) ;
#20370=CARTESIAN_POINT ( 'NONE',  ( 147.6430623265936219, 274.9217099957185155, 8.258152514891218487 ) ) ;
#20371=CARTESIAN_POINT ( 'NONE',  ( 19.47135178391741661, 191.2369531367911293, -4.594050593750048428 ) ) ;
#20373=CARTESIAN_POINT ( 'NONE',  ( 192.6224552386041182, 297.0151161785129261, 12.49354144254605181 ) ) ;
#20376=CARTESIAN_POINT ( 'NONE',  ( 164.8670003495851404, 245.0889742334797177, -1.557028074864921674 ) ) ;
#20377=CARTESIAN_POINT ( 'NONE',  ( 175.1378461883211912, 279.3152656845848583, 16.63146252814350134 ) ) ;
#20378=CARTESIAN_POINT ( 'NONE',  ( 176.3865323452404823, 258.8737835494043225, 13.24306684835586623 ) ) ;
#20379=LINE ( 'NONE', #64983, #21240 ) ;
#20388=B_SPLINE_CURVE_WITH_KNOTS ( 'NONE', 3,
 ( #24733, #1458, #1950, #63744 ),
 .UNSPECIFIED., .F., .F.,
 ( 4, 4 ),
 ( 0.007614618424699901196, 0.01267886371662555085 ),
 .UNSPECIFIED. ) ;
#20389=CYLINDRICAL_SURFACE ( 'NONE', #22110, 17.82106496071139645 ) ;
#20394=CARTESIAN_POINT ( 'NONE',  ( 192.6224552386041182, 297.0151161785129261, 12.49354144254605181 ) ) ;
#20398=CARTESIAN_POINT ( 'NONE',  ( 203.4357368910538355, 278.2859629599173559, -16.45855118664066197 ) ) ;
#20401=CARTESIAN_POINT ( 'NONE',  ( 159.7607676839680835, 278.6090423769052222, -9.664001967995806908 ) ) ;
#20402=CARTESIAN_POINT ( 'NONE',  ( 164.3330377059402849, 246.0138246616164110, 7.208046019122525294 ) ) ;
#20403=CARTESIAN_POINT ( 'NONE',  ( 153.3920560952016956, 264.9641606960921649, 16.50453917291963535 ) ) ;
#20404=ORIENTED_EDGE ( 'NONE', *, *, #80391, .F. ) ;
#20407=CARTESIAN_POINT ( 'NONE',  ( 177.3985541943506803, 263.1773983921460740, 15.48418877813238481 ) ) ;
#20408=ORIENTED_EDGE ( 'NONE', *, *, #22000, .T. ) ;
#20411=CARTESIAN_POINT ( 'NONE',  ( 197.0184425104562820, 289.4010428742387262, -16.90752553128928426 ) ) ;
#20412=EDGE_CURVE ( 'NONE', #90974, #25829, #37687, .T. ) ;
#20414=CARTESIAN_POINT ( 'NONE',  ( 164.5648480107187197, 245.6123174360222094, 3.015887571020871238 ) ) ;
#20418=CARTESIAN_POINT ( 'NONE',  ( 177.3086487836147285, 279.3000926714664160, -16.75854559346873884 ) ) ;
#20419=CARTESIAN_POINT ( 'NONE',  ( 172.2724355110944146, 263.6426226643334303, -15.46355804232799258 ) ) ;
#20421=CARTESIAN_POINT ( 'NONE',  ( 186.0942368718926332, 293.1614520422483565, 12.28461848767796560 ) ) ;
#20424=CARTESIAN_POINT ( 'NONE',  ( 158.0081726929925594, 269.0575936612110013, 15.62741947982547508 ) ) ;
#20427=CARTESIAN_POINT ( 'NONE',  ( 190.4976253092930278, 300.6954295735222900, -5.764807383508308902 ) ) ;
#20429=CARTESIAN_POINT ( 'NONE',  ( -27.42236680055714260, 166.5217562850347406, 1.224646799147364892E-15 ) ) ;
#20430=CARTESIAN_POINT ( 'NONE',  ( 153.4578721839791342, 264.8501638863745029, 16.85421393845643223 ) ) ;
#20431=CARTESIAN_POINT ( 'NONE',  ( 178.2182531100257279, 291.4184198334916687, 6.077856116893014082 ) ) ;
#20432=CARTESIAN_POINT ( 'NONE',  ( 158.4500152958133015, 256.2035183780225793, -16.27180754986873268 ) ) ;
#20433=ORIENTED_EDGE ( 'NONE', *, *, #26815, .T. ) ;
#20436=CARTESIAN_POINT ( 'NONE',  ( 165.0308887387863876, 244.8051112166122891, 1.948365933089477808 ) ) ;
#20437=CARTESIAN_POINT ( 'NONE',  ( 34.75566377745538205, 179.3262482093457493, 3.021315404115420679E-15 ) ) ;
#20438=ORIENTED_EDGE ( 'NONE', *, *, #98662, .F. ) ;
#20441=ORIENTED_EDGE ( 'NONE', *, *, #47542, .T. ) ;
#20444=CARTESIAN_POINT ( 'NONE',  ( 189.6768609436964539, 274.4077930505946483, -17.07046811116321550 ) ) ;
#20445=B_SPLINE_CURVE_WITH_KNOTS ( 'NONE', 3,
 ( #68849, #92213, #20787, #13189, #84599, #22767, #61246, #75480, #28875, #66862, #60239, #98791, #6572, #53644, #59238, #53160, #15137, #59751, #68354, #99770, #51678, #74985, #36456, #84115, #67359, #91200, #52647, #91694, #14667, #46034, #90722, #21277, #76475, #76951, #45543, #82627, #44045, #52154, #83103, #6064, #21760, #70868, #39931, #15642, #463, #54133, #61746, #7551 ),
 .UNSPECIFIED., .F., .F.,
 ( 4, 2, 2, 2, 2, 2, 2, 2, 2, 2, 2, 2, 2, 2, 2, 2, 2, 2, 2, 2, 2, 2, 2, 4 ),
 ( 0.0008122609998851836348, 0.001014663487969617254, 0.001115864732011832058, 0.001217065976054046861, 0.001318267220096261882, 0.001419468464138476903, 0.001621870952222960720, 0.002026675928391991673, 0.002431480904561022626, 0.003241090856899082797, 0.004050700809237142534, 0.004860310761575202705, 0.005265115737744153861, 0.005467518225828587805, 0.005568719469870849446, 0.005619320091892030140, 0.005669920713913210834, 0.005771121957955572222, 0.005872323201997933610, 0.006074725690082618222, 0.006479530666252108877, 0.006884335642421599531, 0.007086738130506338787, 0.007289140618591078910 ),
 .UNSPECIFIED. ) ;
#20446=CARTESIAN_POINT ( 'NONE',  ( 159.9972970628961377, 253.5235477438103544, -14.85214688666258809 ) ) ;
#20447=CARTESIAN_POINT ( 'NONE',  ( 102.3056452726415984, 218.3262482093457493, 3.021315404115420679E-15 ) ) ;
#20449=CARTESIAN_POINT ( 'NONE',  ( 163.2256942281324541, 247.9317998266098471, -9.780520296312531059 ) ) ;
#20451=CARTESIAN_POINT ( 'NONE',  ( 201.0732166862245549, 282.3779679885897167, -18.18766936363638820 ) ) ;
#20452=CARTESIAN_POINT ( 'NONE',  ( 207.6860335175200589, 270.9242332556395922, 6.913225035677485586 ) ) ;
#20453=CARTESIAN_POINT ( 'NONE',  ( 31.46967238556409896, 195.6427522451418781, -10.00000000000009415 ) ) ;
#20454=CARTESIAN_POINT ( 'NONE',  ( 121.7437996339097310, 241.0958772461660544, -9.188101187500095079 ) ) ;
#20456=CARTESIAN_POINT ( 'NONE',  ( 164.9401169542619243, 280.4943389099253181, -11.14461050731500436 ) ) ;
#20457=CARTESIAN_POINT ( 'NONE',  ( 195.7617614321055157, 291.5776783508526364, 16.33009124109666033 ) ) ;
#20458=CARTESIAN_POINT ( 'NONE',  ( 208.3408670980087152, 269.7900282237308147, 2.175586895783760077 ) ) ;
#20459=CARTESIAN_POINT ( 'NONE',  ( 35.49282175392953320, 200.4869531367911293, 4.594050593750046652 ) ) ;
#20461=ORIENTED_EDGE ( 'NONE', *, *, #60741, .F. ) ;
#20463=CARTESIAN_POINT ( 'NONE',  ( -22.42236680055709641, 157.8615022471902591, 0.000000000000000000 ) ) ;
#20464=CARTESIAN_POINT ( 'NONE',  ( 185.2758064758799890, 259.6671588269117592, -5.400835621108775797 ) ) ;
#20469=CARTESIAN_POINT ( 'NONE',  ( 97.33941792859064890, 238.5530062829863027, -4.648177544792955347E-16 ) ) ;
#20470=CARTESIAN_POINT ( 'NONE',  ( 161.5757715694810770, 250.7895496999525449, -14.51803553215175135 ) ) ;
#20472=CARTESIAN_POINT ( 'NONE',  ( 179.3343052093286758, 287.9874940019028031, -12.72641108234611096 ) ) ;
#20474=CARTESIAN_POINT ( 'NONE',  ( 101.6177300921037130, 216.1427522451417929, 1.119607411625061291E-15 ) ) ;
#20477=CARTESIAN_POINT ( 'NONE',  ( 194.8868098799860888, 266.4408012034644457, -7.738736915655594295 ) ) ;
#20479=CARTESIAN_POINT ( 'NONE',  ( 162.8996025780091941, 248.4966071325470125, 11.23567065566008516 ) ) ;
#20480=CARTESIAN_POINT ( 'NONE',  ( 208.3226489551340990, 269.8215829728092103, -1.240262689467544366 ) ) ;
#20481=CARTESIAN_POINT ( 'NONE',  ( 20.58138070222249638, 176.5643266524160140, -9.188101187500093303 ) ) ;
#20487=B_SPLINE_CURVE_WITH_KNOTS ( 'NONE', 3,
 ( #21027, #44288, #27124, #11926, #65601, #73226, #19038, #98524, #50897, #58490, #49910, #58006, #11440, #88986, #34700, #81846, #19540, #42782, #35705, #66603, #92433, #76221, #30597, #61483, #99512, #22980, #70077, #22494, #60474, #53869, #38168, #691, #84831, #68589, #52392, #61967, #15369, #30096, #23473, #92920, #6797, #46267, #77190, #31574, #7797, #45287, #37677, #46794, #38682, #69586, #54364, #90951, #69086, #85337 ),
 .UNSPECIFIED., .F., .F.,
 ( 4, 2, 2, 2, 2, 2, 2, 2, 2, 2, 2, 2, 2, 2, 2, 2, 2, 2, 2, 2, 2, 2, 2, 2, 2, 2, 4 ),
 ( 0.0008054865245305401020, 0.001006788277830038053, 0.001107439154479787028, 0.001208090031129536003, 0.001308740907779284979, 0.001409391784429033737, 0.001610693537728460564, 0.002013297044327447358, 0.002415900550926434152, 0.003221107564124476262, 0.004026314577322517504, 0.004831521590520558747, 0.005234125097119579802, 0.005435426850419054767, 0.005536077727068828246, 0.005586403165393787409, 0.005636728603718745706, 0.005687054042043704870, 0.005737379480368664034, 0.005838030357018627464, 0.006039332110318513559, 0.006240633863618400522, 0.006441935616918286617, 0.006643237370218172712, 0.006844539123518058807, 0.007045840876817945769, 0.007247142630117831864 ),
 .UNSPECIFIED. ) ;
#20488=CARTESIAN_POINT ( 'NONE',  ( 55.81761577081934433, 203.0333772461660544, 9.188101187500095079 ) ) ;
#20495=CARTESIAN_POINT ( 'NONE',  ( -2.070769811622824363, 179.6115022471903160, -5.000000000000047962 ) ) ;
#20497=CARTESIAN_POINT ( 'NONE',  ( 133.4083396129551602, 238.6423013555409796, -4.594050593750043987 ) ) ;
#20501=CARTESIAN_POINT ( 'NONE',  ( 196.0355168007595523, 291.1035201434990540, 17.55377893960077884 ) ) ;
#20503=CARTESIAN_POINT ( 'NONE',  ( 150.5052742266933876, 269.9642135627172479, -13.76496694288080391 ) ) ;
#20505=CARTESIAN_POINT ( 'NONE',  ( 151.3589047706063582, 268.4856820897672378, 14.56544807350869419 ) ) ;
#20506=CARTESIAN_POINT ( 'NONE',  ( 207.8730126074944451, 270.6003759718510651, -1.781618945033869306 ) ) ;
#20508=CARTESIAN_POINT ( 'NONE',  ( 169.7497442303230173, 266.0831907009023212, -17.38058090311056603 ) ) ;
#20509=CARTESIAN_POINT ( 'NONE',  ( 197.2070174366134836, 273.4893232311666793, -14.13887660181231709 ) ) ;
#20513=CARTESIAN_POINT ( 'NONE',  ( 169.5642877124303709, 282.9217698259369058, -10.96075264092123902 ) ) ;
#20516=CARTESIAN_POINT ( 'NONE',  ( 185.7432137520750359, 296.9624951973794396, 5.510464551842103376 ) ) ;
#20517=CARTESIAN_POINT ( 'NONE',  ( 148.9549916732168811, 245.2592609112379876, 2.679491924311254714 ) ) ;
#20518=CARTESIAN_POINT ( 'NONE',  ( 148.4905408331877084, 273.9803389716664697, -7.981520963315253070 ) ) ;
#20519=CARTESIAN_POINT ( 'NONE',  ( -22.42236680055709641, 157.8615022471902591, 0.000000000000000000 ) ) ;
#20527=CARTESIAN_POINT ( 'NONE',  ( 191.6723191112861855, 298.6608002251342100, -9.737039817265848995 ) ) ;
#20528=CARTESIAN_POINT ( 'NONE',  ( 185.5314771523295292, 291.0755628727823705, 12.15834007696259711 ) ) ;
#20529=CARTESIAN_POINT ( 'NONE',  ( 204.4325665793906524, 276.5594032932251594, 13.33817701435311598 ) ) ;
#20534=CARTESIAN_POINT ( 'NONE',  ( 84.12564760914067108, 225.5024278399160949, 9.188101187500095079 ) ) ;
#20535=CARTESIAN_POINT ( 'NONE',  ( 154.9899569171280973, 262.1965152870598104, 17.85248177135828485 ) ) ;
#20537=CARTESIAN_POINT ( 'NONE',  ( 181.1762993832780353, 271.6239722135371721, -17.18960871778338273 ) ) ;
#20540=ORIENTED_EDGE ( 'NONE', *, *, #8290, .F. ) ;
#20546=CARTESIAN_POINT ( 'NONE',  ( 159.4159393015865476, 258.5086116838130010, 17.42071531078585522 ) ) ;
#20549=CARTESIAN_POINT ( 'NONE',  ( 206.9526720368717463, 272.1944526004363070, -6.912324681932258130 ) ) ;
#20550=DIRECTION ( 'NONE',  ( 0.4999999999999998890, -0.8660254037844385966, 0.000000000000000000 ) ) ;
#20553=CARTESIAN_POINT ( 'NONE',  ( 148.0826818691893152, 274.1602666119424043, -9.371267383421741926 ) ) ;
#20555=CARTESIAN_POINT ( 'NONE',  ( 165.1083560551384721, 265.3609356111044804, -16.61290852168901822 ) ) ;
#20558=ORIENTED_EDGE ( 'NONE', *, *, #3944, .F. ) ;
#20560=CARTESIAN_POINT ( 'NONE',  ( 195.6491688553082611, 270.3377900390409536, -13.51386470325394917 ) ) ;
#20561=CARTESIAN_POINT ( 'NONE',  ( 199.9472389266075254, 270.2118812112473165, 9.338481273082759770 ) ) ;
#20563=CARTESIAN_POINT ( 'NONE',  ( 162.9466247808429102, 248.4151622881552441, 11.25765811906727443 ) ) ;
#20564=CARTESIAN_POINT ( 'NONE',  ( 191.2190380946134951, 260.9445496458436651, 3.106810577783889915 ) ) ;
#20565=CARTESIAN_POINT ( 'NONE',  ( 149.1167591741855745, 276.2932744649320966, -5.492527394273915675 ) ) ;
#20568=CARTESIAN_POINT ( 'NONE',  ( 192.6560265352977410, 292.3260843751113498, -14.38534841386452534 ) ) ;
#20569=CARTESIAN_POINT ( 'NONE',  ( 168.0406546387621631, 252.9712069534065222, 11.80637672277989481 ) ) ;
#20572=CARTESIAN_POINT ( 'NONE',  ( 155.5889810493316929, 261.1589750551232214, -18.49677816280062714 ) ) ;
#20574=ORIENTED_EDGE ( 'NONE', *, *, #83531, .T. ) ;
#20575=CARTESIAN_POINT ( 'NONE',  ( 190.1774295428112396, 299.2500249094251217, 7.542682482482700124 ) ) ;
#20576=CARTESIAN_POINT ( 'NONE',  ( 172.6505904036989136, 280.8448313155626579, -15.39888677054324440 ) ) ;
#20577=CARTESIAN_POINT ( 'NONE',  ( 164.1338920432579300, 246.3587550674890565, -8.095503919041194152 ) ) ;
#20578=CARTESIAN_POINT ( 'NONE',  ( 190.6661865267473104, 300.4034729807058852, 4.523489664447863490 ) ) ;
#20579=CARTESIAN_POINT ( 'NONE',  ( 164.7829470492978601, 274.1661399048329031, 15.02517063526678420 ) ) ;
#20580=CARTESIAN_POINT ( 'NONE',  ( 161.4353714413109344, 281.4025874958057329, -6.883957629530069511 ) ) ;
#20582=CARTESIAN_POINT ( 'NONE',  ( 200.0915598631207786, 267.8243757013111690, 6.133940993518010920 ) ) ;
#20583=VERTEX_POINT ( 'NONE', #55646 ) ;
#20586=CARTESIAN_POINT ( 'NONE',  ( 189.9388136067621531, 273.9745203768302986, -15.62273351239337416 ) ) ;
#20588=CARTESIAN_POINT ( 'NONE',  ( 186.6544709008256575, 298.6510803302452359, 3.914313306637340339 ) ) ;
#20589=CARTESIAN_POINT ( 'NONE',  ( 192.7507137768506880, 296.7929658737652971, 11.30364540927242345 ) ) ;
#20591=CARTESIAN_POINT ( 'NONE',  ( 191.0453904752189089, 285.8430533356794285, 17.34534042816491350 ) ) ;
#20592=CARTESIAN_POINT ( 'NONE',  ( 7.753205860782987457, 175.2833772461660544, -9.188101187500095079 ) ) ;
#20593=CARTESIAN_POINT ( 'NONE',  ( 96.79126913948807953, 232.8149278399160949, 9.188101187500093303 ) ) ;
#20594=CARTESIAN_POINT ( 'NONE',  ( 36.33098132476075648, 203.3297689869269220, -2.679491924311201423 ) ) ;
#20595=CARTESIAN_POINT ( 'NONE',  ( 185.4201904309665281, 295.0767498550951586, -7.685989019839836622 ) ) ;
#20599=CARTESIAN_POINT ( 'NONE',  ( -22.42236680055709641, 157.8615022471902591, 0.000000000000000000 ) ) ;
#20601=CARTESIAN_POINT ( 'NONE',  ( 164.7873404923249154, 250.7312283864773690, -12.00200811739543383 ) ) ;
#20602=CARTESIAN_POINT ( 'NONE',  ( 180.5563687299889182, 273.0276302482951110, 17.30336775547517547 ) ) ;
#20603=CARTESIAN_POINT ( 'NONE',  ( 194.8067605455144076, 293.2317884077015151, -16.00245909155922774 ) ) ;
#20605=CARTESIAN_POINT ( 'NONE',  ( 195.9602617257426402, 266.6740640884384561, 8.002040582201244590 ) ) ;
#20607=CARTESIAN_POINT ( 'NONE',  ( 183.1426684129219780, 267.5694331394444703, -16.03671021927237206 ) ) ;
#20608=VECTOR ( 'NONE', #76987, 1000.000000000000000 ) ;
#20609=( BOUNDED_CURVE ( )  B_SPLINE_CURVE ( 2, ( #64600, #3802, #49391, #71211, #48900 ),
 .UNSPECIFIED., .F., .T. ) 
 B_SPLINE_CURVE_WITH_KNOTS ( ( 3, 2, 3 ),
 ( 0.9784858563273379772, 0.9784946236559139976, 0.9798387096774193727 ),
 .UNSPECIFIED. ) 
 CURVE ( )  GEOMETRIC_REPRESENTATION_ITEM ( )  RATIONAL_B_SPLINE_CURVE ( ( 0.9991289483004428540, 0.9995630490582195771, 1.000000000000000000, 0.9330127018922194093, 0.9330127018922194093 ) ) 
 REPRESENTATION_ITEM ( '' )  );
#20611=CARTESIAN_POINT ( 'NONE',  ( 77.90126356732251622, 215.7833772461660544, -9.188101187500095079 ) ) ;
#20613=FACE_OUTER_BOUND ( 'NONE', #39175, .T. ) ;
#20615=CARTESIAN_POINT ( 'NONE',  ( 157.2464636617698375, 258.2881309577184652, 18.14284729738657731 ) ) ;
#20616=CARTESIAN_POINT ( 'NONE',  ( 200.4189218502630467, 283.5112398876054272, 18.06577013929910791 ) ) ;
#20618=CARTESIAN_POINT ( 'NONE',  ( 173.5450725454375061, 267.4326936521503058, -17.29647674659017298 ) ) ;
#20620=CARTESIAN_POINT ( 'NONE',  ( 147.5540328368684300, 275.0759135952944234, -4.750028533202499403 ) ) ;
#20621=DIRECTION ( 'NONE',  ( -0.8660254037844387076, -0.4999999999999998890, -0.000000000000000000 ) ) ;
#20622=ORIENTED_EDGE ( 'NONE', *, *, #47907, .T. ) ;
#20624=CARTESIAN_POINT ( 'NONE',  ( 177.1347673595945764, 262.9921672455169528, 15.53478677465993485 ) ) ;
#20625=CARTESIAN_POINT ( 'NONE',  ( 193.0142717932987182, 296.3364699985351081, -13.30037542329744937 ) ) ;
#20628=B_SPLINE_CURVE_WITH_KNOTS ( 'NONE', 3,
 ( #34487, #65388, #26900, #81142 ),
 .UNSPECIFIED., .F., .F.,
 ( 4, 4 ),
 ( 0.001193343334414101150, 0.009119723292965509209 ),
 .UNSPECIFIED. ) ;
#20631=CARTESIAN_POINT ( 'NONE',  ( 156.9010835643442192, 268.4413441992039111, 15.68067955713730122 ) ) ;
#20633=CARTESIAN_POINT ( 'NONE',  ( 138.2253456014563255, 250.6115022471902591, 10.00000000000009592 ) ) ;
#20635=VECTOR ( 'NONE', #2295, 1000.000000000000114 ) ;
#20636=ORIENTED_EDGE ( 'NONE', *, *, #85891, .T. ) ;
#20637=CARTESIAN_POINT ( 'NONE',  ( 190.3167824967908643, 299.0086585129598689, -8.112609889089975823 ) ) ;
#20638=ORIENTED_EDGE ( 'NONE', *, *, #34687, .T. ) ;
#20644=CARTESIAN_POINT ( 'NONE',  ( 158.5882721812411376, 255.9640504279652760, 16.09668399467820166 ) ) ;
#20645=CARTESIAN_POINT ( 'NONE',  ( 194.0724203524910365, 280.7181176903307005, -17.60110234268010032 ) ) ;
#20646=CARTESIAN_POINT ( 'NONE',  ( 193.1336260368645981, 296.1297423845801404, -13.41923397934924367 ) ) ;
#20647=CARTESIAN_POINT ( 'NONE',  ( 153.3859906278383676, 264.9746663937372091, -17.41799046551451013 ) ) ;
#20648=EDGE_CURVE ( 'NONE', #5726, #29964, #24630, .T. ) ;
#20652=CARTESIAN_POINT ( 'NONE',  ( 166.7213618741906771, 275.6891020104532117, 14.83267127466106139 ) ) ;
#20654=VERTEX_POINT ( 'NONE', #12462 ) ;
#20657=CARTESIAN_POINT ( 'NONE',  ( 164.4864504671816690, 245.7481059646165704, 6.337356894698421783 ) ) ;
#20658=CARTESIAN_POINT ( 'NONE',  ( 147.8819534105757043, 274.5079385007862811, -9.338341377131436971 ) ) ;
#20663=CARTESIAN_POINT ( 'NONE',  ( 170.9173439896608500, 287.6710870028733211, -4.607079402279047997 ) ) ;
#20668=CARTESIAN_POINT ( 'NONE',  ( 148.0446189821823282, 274.7176051505724104, -6.028654458819870499 ) ) ;
#20669=CARTESIAN_POINT ( 'NONE',  ( 166.4520249213679790, 277.9984640549334358, -13.37092130267346057 ) ) ;
#20671=ORIENTED_EDGE ( 'NONE', *, *, #54849, .T. ) ;
#20672=AXIS2_PLACEMENT_3D ( 'NONE', #66722, #74364, #13542 ) ;
#20679=CARTESIAN_POINT ( 'NONE',  ( 164.4909307685898341, 249.4621815394609143, 9.893007727036904342 ) ) ;
#20682=EDGE_CURVE ( 'NONE', #73019, #7170, #53503, .T. ) ;
#20683=ORIENTED_EDGE ( 'NONE', *, *, #52910, .T. ) ;
#20686=ORIENTED_EDGE ( 'NONE', *, *, #23089, .F. ) ;
#20688=CARTESIAN_POINT ( 'NONE',  ( 191.6065101195901832, 264.2025560880797457, -7.910045257811711750 ) ) ;
#20691=CARTESIAN_POINT ( 'NONE',  ( 135.7624123097878623, 255.3149278399160949, 9.188101187500093303 ) ) ;
#20699=CARTESIAN_POINT ( 'NONE',  ( 190.5742268578622145, 264.3298435039872061, -9.417883106533958326 ) ) ;
#20700=CARTESIAN_POINT ( 'NONE',  ( 170.0560250869938841, 248.9713545018433649, -0.2644624926305505497 ) ) ;
#20701=CARTESIAN_POINT ( 'NONE',  ( 172.6689194511114920, 286.8832926196414519, 10.78400060168022989 ) ) ;
#20702=B_SPLINE_CURVE_WITH_KNOTS ( 'NONE', 3,
 ( #93187, #70867, #33358, #70351 ),
 .UNSPECIFIED., .F., .F.,
 ( 4, 4 ),
 ( 0.006445490163176449683, 0.01145963672390969655 ),
 .UNSPECIFIED. ) ;
#20704=CARTESIAN_POINT ( 'NONE',  ( 199.0069894091751905, 281.8216829437676552, -16.59361213652569589 ) ) ;
#20705=CARTESIAN_POINT ( 'NONE',  ( 122.6368883333363584, 251.6115022471903160, -5.000000000000047962 ) ) ;
#20706=EDGE_CURVE ( 'NONE', #100197, #30881, #30548, .T. ) ;
#20710=CARTESIAN_POINT ( 'NONE',  ( 64.04520420253651025, 195.5327760586659736, 1.948934522072303157E-15 ) ) ;
#20712=CARTESIAN_POINT ( 'NONE',  ( 197.2094417012475560, 287.4525406113273220, 17.46401919701611760 ) ) ;
#20714=EDGE_CURVE ( 'NONE', #76357, #8790, #35390, .T. ) ;
#20715=DIRECTION ( 'NONE',  ( 0.4999999999999998890, -0.8660254037844385966, 0.000000000000000000 ) ) ;
#20716=ADVANCED_FACE ( 'NONE', ( #30128 ), #31608, .T. ) ;
#20719=CARTESIAN_POINT ( 'NONE',  ( 160.0166746459236435, 283.6086068001695253, 2.232576205374148248 ) ) ;
#20721=EDGE_CURVE ( 'NONE', #95964, #99288, #15407, .T. ) ;
#20727=CARTESIAN_POINT ( 'NONE',  ( 15.38522827951586081, 173.5643266524160140, -9.188101187500093303 ) ) ;
#20729=VERTEX_POINT ( 'NONE', #93468 ) ;
#20730=VECTOR ( 'NONE', #4037, 1000.000000000000000 ) ;
#20731=CARTESIAN_POINT ( 'NONE',  ( 182.6063025987909327, 258.0860380675601391, -8.404863973281287315 ) ) ;
#20732=CARTESIAN_POINT ( 'NONE',  ( 201.0466602553734106, 278.3904726219785744, 15.32208466927121293 ) ) ;
#20735=CARTESIAN_POINT ( 'NONE',  ( 51.59574192737019160, 200.5958772461660544, -9.188101187500095079 ) ) ;
#20737=CARTESIAN_POINT ( 'NONE',  ( 200.6129772034685175, 283.1751261563724142, 18.36811917402039640 ) ) ;
#20738=CARTESIAN_POINT ( 'NONE',  ( 199.0363797504450929, 285.9058730480928716, -17.12190301149298222 ) ) ;
#20739=CARTESIAN_POINT ( 'NONE',  ( 190.1696443193688708, 301.2635093119881162, -4.804312979389741223 ) ) ;
#20741=CARTESIAN_POINT ( 'NONE',  ( 159.1856415905643303, 255.7098345965759734, -16.10742115897274829 ) ) ;
#20742=CARTESIAN_POINT ( 'NONE',  ( 177.7369556440871463, 292.4164984073148617, 2.588529651253329789 ) ) ;
#20744=CARTESIAN_POINT ( 'NONE',  ( 179.5538644306811022, 276.7319085261062241, 16.30229987282069004 ) ) ;
#20747=CARTESIAN_POINT ( 'NONE',  ( 107.8477481777883469, 244.6199935810940929, 2.679491924311251605 ) ) ;
#20751=CARTESIAN_POINT ( 'NONE',  ( 101.8522786425098730, 229.6115022471902307, 10.00000000000009592 ) ) ;
#20753=CARTESIAN_POINT ( 'NONE',  ( 194.7393124278854657, 285.6008549388717483, -17.52668146566740148 ) ) ;
#20755=CARTESIAN_POINT ( 'NONE',  ( 57.30635725539759306, 194.7048013555409796, 4.594050593750051981 ) ) ;
#20757=CARTESIAN_POINT ( 'NONE',  ( 166.5660256732271591, 264.7075128827775075, 17.06110633390546027 ) ) ;
#20759=CARTESIAN_POINT ( 'NONE',  ( -22.42236680055709641, 157.8615022471902591, 0.000000000000000000 ) ) ;
#20760=ORIENTED_EDGE ( 'NONE', *, *, #57869, .F. ) ;
#20763=CARTESIAN_POINT ( 'NONE',  ( 207.6628070930962906, 270.9644626028195376, 7.378217122120054761 ) ) ;
#20764=CARTESIAN_POINT ( 'NONE',  ( 159.9304399683796589, 266.3231526470470385, -17.61295603372380825 ) ) ;
#20766=CARTESIAN_POINT ( 'NONE',  ( 186.4093957424555583, 263.0584473022519774, 11.49005727324106374 ) ) ;
#20768=CARTESIAN_POINT ( 'NONE',  ( 204.5773065883323056, 276.3087062438502812, 13.12907315817041187 ) ) ;
#20769=ORIENTED_EDGE ( 'NONE', *, *, #80453, .T. ) ;
#20774=ORIENTED_EDGE ( 'NONE', *, *, #27456, .T. ) ;
#20775=CARTESIAN_POINT ( 'NONE',  ( 180.0052941831603732, 282.8434537829564874, 15.07745545751880911 ) ) ;
#20776=CARTESIAN_POINT ( 'NONE',  ( 166.9663977217517470, 261.3869414865291674, 16.80305011033491169 ) ) ;
#20777=CARTESIAN_POINT ( 'NONE',  ( 206.2313482792274328, 273.4438219973828268, -9.403385562213845361 ) ) ;
#20778=ORIENTED_EDGE ( 'NONE', *, *, #5651, .F. ) ;
#20779=AXIS2_PLACEMENT_3D ( 'NONE', #13052, #66721, #52027 ) ;
#20780=CARTESIAN_POINT ( 'NONE',  ( 160.5702328569162489, 282.4873091647734213, -3.166141603222274448 ) ) ;
#20785=CARTESIAN_POINT ( 'NONE',  ( 198.2414483977475754, 287.2827345394944700, 16.94931984969033678 ) ) ;
#20786=CARTESIAN_POINT ( 'NONE',  ( 186.0348036264326481, 259.0250182415348945, 6.435743254585703177 ) ) ;
#20787=CARTESIAN_POINT ( 'NONE',  ( 161.1469752488031588, 263.0258888816042031, -17.74540750750012919 ) ) ;
#20788=CARTESIAN_POINT ( 'NONE',  ( 124.5044291563551440, 236.5643266524160424, -9.188101187500093303 ) ) ;
#20789=EDGE_CURVE ( 'NONE', #42330, #92664, #25682, .T. ) ;
#20791=CARTESIAN_POINT ( 'NONE',  ( 170.1571642572108658, 264.1681567744807353, 16.32371355451207151 ) ) ;
#20792=CARTESIAN_POINT ( 'NONE',  ( 73.18322933451462120, 206.3927522451418497, -10.00000000000009237 ) ) ;
#20795=CARTESIAN_POINT ( 'NONE',  ( 148.8217493443905255, 275.2952789360765564, 7.685775767636982003 ) ) ;
#20797=ORIENTED_EDGE ( 'NONE', *, *, #60241, .F. ) ;
#20798=CARTESIAN_POINT ( 'NONE',  ( 198.4334039703542771, 286.9502577349437615, 18.47706603442866680 ) ) ;
#20800=CARTESIAN_POINT ( 'NONE',  ( 82.55649720842890815, 206.2202760586659167, -5.415160957724236172E-17 ) ) ;
#20801=ADVANCED_FACE ( 'NONE', ( #15920 ), #22927, .F. ) ;
#20804=CARTESIAN_POINT ( 'NONE',  ( 175.3946993052283005, 278.3949788008520159, 15.46601621310474250 ) ) ;
#20810=CARTESIAN_POINT ( 'NONE',  ( 153.2513309553138470, 265.2079037882803618, -16.24091495603130397 ) ) ;
#20816=CARTESIAN_POINT ( 'NONE',  ( 174.3136715079830026, 253.2187907930447750, -7.762168257024684159 ) ) ;
#20819=CARTESIAN_POINT ( 'NONE',  ( 164.6241018286200699, 245.5096868128744632, 3.031483545445131433 ) ) ;
#20824=CARTESIAN_POINT ( 'NONE',  ( 136.7095408212358052, 258.9244531367911577, -4.594050593750046652 ) ) ;
#20826=CARTESIAN_POINT ( 'NONE',  ( -7.266922234329455499, 176.6115022471903160, -5.000000000000047962 ) ) ;
#20828=CARTESIAN_POINT ( 'NONE',  ( 168.8563211758018099, 286.0187424789903048, -9.056861680415359217 ) ) ;
#20832=ORIENTED_EDGE ( 'NONE', *, *, #68260, .T. ) ;
#20835=CARTESIAN_POINT ( 'NONE',  ( 182.1058308719148613, 275.7167741723378072, -16.43330782191204520 ) ) ;
#20837=CARTESIAN_POINT ( 'NONE',  ( 167.5923213779273340, 249.2094892142539493, -5.528754456902119863 ) ) ;
#20839=CARTESIAN_POINT ( 'NONE',  ( 200.4669192785465839, 267.1762403986572281, 0.8314407050123316933 ) ) ;
#20840=CARTESIAN_POINT ( 'NONE',  ( 199.1041333440138317, 265.1832257255362038, 0.2027868546939186056 ) ) ;
#20841=CARTESIAN_POINT ( 'NONE',  ( 190.1635032421960148, 301.2741459696644029, -5.047660290019184259 ) ) ;
#20843=CARTESIAN_POINT ( 'NONE',  ( 184.5366411851703390, 281.4491850268337885, 16.25207963496568908 ) ) ;
#20844=CARTESIAN_POINT ( 'NONE',  ( 193.2770523687239859, 268.3139821420764406, 12.74059143256334359 ) ) ;
#20845=EDGE_CURVE ( 'NONE', #65280, #13449, #70334, .T. ) ;
#20847=B_SPLINE_CURVE_WITH_KNOTS ( 'NONE', 3,
 ( #40413, #42777, #71347, #1938, #32824, #63732, #45767, #90946, #61477, #6295, #6791, #45281, #37186, #77182, #68087, #37672 ),
 .UNSPECIFIED., .F., .F.,
 ( 4, 2, 2, 2, 2, 2, 2, 4 ),
 ( 0.000000000000000000, 0.0005218775415615029088, 0.0007828163123422070919, 0.001043755083122911275, 0.001304693853903615567, 0.001565632624684319641, 0.001826571395465023933, 0.002087510166245728008 ),
 .UNSPECIFIED. ) ;
#20848=CARTESIAN_POINT ( 'NONE',  ( 149.1856130393175306, 272.2499337880290682, 11.44243872309708188 ) ) ;
#20849=CARTESIAN_POINT ( 'NONE',  ( 59.82969263072505584, 216.8967562850347122, -4.648177544792955347E-16 ) ) ;
#20851=CARTESIAN_POINT ( 'NONE',  ( 198.4772197948566372, 286.8743665007300478, 18.43646439804394532 ) ) ;
#20853=CARTESIAN_POINT ( 'NONE',  ( 138.0629658346988151, 250.5177522451418213, -10.00000000000009592 ) ) ;
#20854=CARTESIAN_POINT ( 'NONE',  ( 172.4124261811984127, 284.1103845159578896, -12.83577416862662979 ) ) ;
#20855=ORIENTED_EDGE ( 'NONE', *, *, #74554, .F. ) ;
#20857=CARTESIAN_POINT ( 'NONE',  ( 199.1944722252943905, 285.6320488493591938, -18.17555833707144686 ) ) ;
#20858=CARTESIAN_POINT ( 'NONE',  ( 18.76822678699008051, 172.4548013555409796, -4.594050593750042211 ) ) ;
#20860=CARTESIAN_POINT ( 'NONE',  ( 179.6016093521815264, 274.3055133302825084, -17.77051425966819664 ) ) ;
#20863=CARTESIAN_POINT ( 'NONE',  ( 157.0978663001774862, 258.5455091378672137, -17.31223197570816552 ) ) ;
#20865=CARTESIAN_POINT ( 'NONE',  ( 149.7854447168632817, 277.1467554076948545, 4.663160563959508842 ) ) ;
#20866=B_SPLINE_CURVE_WITH_KNOTS ( 'NONE', 3,
 ( #53557, #1378, #46964, #7978, #84508, #15052, #30265, #77375, #100189, #76390, #6964, #54042, #45943, #47456, #8468, #62142, #68757, #86034, #78383, #37850, #862, #92603, #94107, #69260, #24658, #8964, #7458, #39833, #31742, #368, #31255, #30773, #62644, #61655, #84998, #99682, #46443, #16063, #93600, #93089, #38853, #55542, #61154, #86526, #23646, #85518, #22677, #45456, #92125, #72293 ),
 .UNSPECIFIED., .F., .F.,
 ( 4, 2, 2, 2, 2, 2, 2, 2, 2, 2, 2, 2, 2, 2, 2, 2, 2, 2, 2, 2, 2, 2, 2, 2, 4 ),
 ( 0.0002086497370388745807, 0.0006900493116877915497, 0.001171448886336708302, 0.001412148673661194108, 0.001532498567323459671, 0.001652848460985725234, 0.001773198354647990797, 0.001893548248310256360, 0.002134248035634715712, 0.002615647610283591482, 0.003097047184932467251, 0.004059846334230156339, 0.005022645483527845428, 0.005504045058176613645, 0.005744744845501038519, 0.005865094739163214527, 0.005985444632825390535, 0.006045619579656511498, 0.006105794526487632462, 0.006226144420149894339, 0.006466844207474383398, 0.006948243782123404017, 0.007188943569447914760, 0.007429643356772425503, 0.007911042931421497296 ),
 .UNSPECIFIED. ) ;
#20867=CARTESIAN_POINT ( 'NONE',  ( 182.2373335159190901, 280.9600371166583841, -17.30031729693378040 ) ) ;
#20868=CARTESIAN_POINT ( 'NONE',  ( 178.6317619811870259, 253.9327355832967612, -4.167451725846189170 ) ) ;
#20869=CARTESIAN_POINT ( 'NONE',  ( 150.9950855294679570, 269.1158355001903715, 14.12809338255366320 ) ) ;
#20870=CARTESIAN_POINT ( 'NONE',  ( 179.3203272704038795, 294.0804011742710031, 1.043687953058034301 ) ) ;
#20871=CARTESIAN_POINT ( 'NONE',  ( 61.65426615018220957, 199.7365022471902023, -10.00000000000009059 ) ) ;
#20872=CARTESIAN_POINT ( 'NONE',  ( 185.0103834951779334, 294.0474252827615373, 9.686088409191285109 ) ) ;
#20874=AXIS2_PLACEMENT_3D ( 'NONE', #39217, #45338, #15935 ) ;
#20875=CARTESIAN_POINT ( 'NONE',  ( 19.90436448580963713, 191.4869531367911293, 4.594050593750046652 ) ) ;
#20876=CARTESIAN_POINT ( 'NONE',  ( 168.0283599306779649, 286.1692283979162426, 4.090021465173546034 ) ) ;
#20878=CARTESIAN_POINT ( 'NONE',  ( 8.321535033790485869, 175.6115022471902307, 10.00000000000009592 ) ) ;
#20880=CARTESIAN_POINT ( 'NONE',  ( 145.0115229932138163, 242.9824982072973683, 3.021315404115420679E-15 ) ) ;
#20882=CARTESIAN_POINT ( 'NONE',  ( 179.7935361763625224, 276.9290168454140257, 16.29839862902545988 ) ) ;
#20883=CARTESIAN_POINT ( 'NONE',  ( 185.5167212227024436, 266.6325209536038869, 13.19601323185720254 ) ) ;
#20884=CARTESIAN_POINT ( 'NONE',  ( 125.5723057710370085, 231.7592609112379876, 2.679491924311254714 ) ) ;
#20885=CARTESIAN_POINT ( 'NONE',  ( 164.0674942879805371, 281.5465086372613541, 8.868535044241015797 ) ) ;
#20890=CARTESIAN_POINT ( 'NONE',  ( 187.4676533354318906, 272.4601757945604845, -16.88503403312462936 ) ) ;
#20891=CARTESIAN_POINT ( 'NONE',  ( -27.42236680055714260, 166.5217562850347406, 1.224646799147364892E-15 ) ) ;
#20895=CARTESIAN_POINT ( 'NONE',  ( 156.5940896385898213, 276.3990306459002682, 10.26584805396775479 ) ) ;
#20899=CARTESIAN_POINT ( 'NONE',  ( 156.4935365524153497, 263.7981763440885175, 17.67496387420143833 ) ) ;
#20902=CARTESIAN_POINT ( 'NONE',  ( 204.6785851723931557, 274.1332865905380913, -12.34137688749581407 ) ) ;
#20903=CARTESIAN_POINT ( 'NONE',  ( 202.7602807045765019, 279.4558873931827065, -15.90558713185497020 ) ) ;
#20906=( BOUNDED_CURVE ( )  B_SPLINE_CURVE ( 2, ( #71105, #9808, #41165, #94921, #70575, #32069, #62980, #33593, #79730 ),
 .UNSPECIFIED., .F., .T. ) 
 B_SPLINE_CURVE_WITH_KNOTS ( ( 3, 2, 2, 2, 3 ),
 ( 0.4475806451612903136, 0.4489247311827956888, 0.4516129032258064391, 0.4543010752688171894, 0.4556451612903225645 ),
 .UNSPECIFIED. ) 
 CURVE ( )  GEOMETRIC_REPRESENTATION_ITEM ( )  RATIONAL_B_SPLINE_CURVE ( ( 0.9330127018922194093, 0.9330127018922194093, 1.000000000000000000, 0.8660254037844387076, 1.000000000000000000, 0.8660254037844387076, 1.000000000000000000, 0.9330127018922194093, 0.9330127018922194093 ) ) 
 REPRESENTATION_ITEM ( '' )  );
#20908=CARTESIAN_POINT ( 'NONE',  ( 164.9274015170355767, 246.4109339568823600, -4.339738877753560153 ) ) ;
#20909=CARTESIAN_POINT ( 'NONE',  ( 164.2712161151136172, 246.1209027979328710, 7.276091357954241445 ) ) ;
#20910=CARTESIAN_POINT ( 'NONE',  ( 192.3606619183491091, 297.4685555102766443, 10.99569063633359889 ) ) ;
#20911=ORIENTED_EDGE ( 'NONE', *, *, #34437, .F. ) ;
#20912=CARTESIAN_POINT ( 'NONE',  ( 191.2645787786270262, 299.3670271975948367, 7.309947121636420242 ) ) ;
#20915=VERTEX_POINT ( 'NONE', #88900 ) ;
#20918=B_SPLINE_CURVE_WITH_KNOTS ( 'NONE', 3,
 ( #89641, #28788, #36881, #98205, #20203, #28278, #29783, #21689, #44469, #90125, #82035, #20700, #52568, #14088, #99694, #44973, #43968, #74906, #45468, #75911, #6491, #5985, #12611, #66785, #76403, #5491, #51589, #37370, #68275, #60655, #43475, #83026, #13108, #59668, #97711, #36374, #67786, #84031, #14590, #90642, #21202, #98712, #37861, #52081, #68770, #13595, #39354, #100201, #1889, #381 ),
 .UNSPECIFIED., .F., .F.,
 ( 4, 2, 2, 2, 2, 2, 2, 2, 2, 2, 2, 2, 2, 2, 2, 2, 2, 2, 2, 2, 2, 2, 2, 2, 4 ),
 ( 0.0007717967845395873154, 0.0009775820906090470185, 0.001080474743643774268, 0.001183367396678501734, 0.001286260049713228984, 0.001389152702747956450, 0.001594938008817510479, 0.002006508620956503827, 0.002418079233095497826, 0.003241220457373425977, 0.004064361681651354127, 0.004887502905929283145, 0.005299073518068247654, 0.005504858824137695214, 0.005607751477172462362, 0.005659197803689845069, 0.005710644130207229510, 0.005813536783242036557, 0.005916429436276843604, 0.006122214742346457697, 0.006533785354485663333, 0.006739570660555331202, 0.006945355966624997338, 0.007151141272694665207, 0.007356926578764333077 ),
 .UNSPECIFIED. ) ;
#20919=CARTESIAN_POINT ( 'NONE',  ( 196.7823306783968746, 289.8100005636337073, -17.85370042640856170 ) ) ;
#20922=CARTESIAN_POINT ( 'NONE',  ( 206.5117639185820906, 272.9581278627833285, 11.28485531511759099 ) ) ;
#20924=B_SPLINE_SURFACE_WITH_KNOTS ( 'NONE', 3, 1, ( 
 ( #12915, #13883 ),
 ( #82347, #73702 ),
 ( #35184, #67078 ),
 ( #51379, #97514 ),
 ( #5295, #59966 ),
 ( #57991, #4285 ),
 ( #3806, #65588 ),
 ( #44765, #51894 ),
 ( #34686, #13404 ),
 ( #35691, #81339 ),
 ( #96536, #82835 ),
 ( #66093, #28581 ),
 ( #58956, #27106 ),
 ( #88972, #11913 ),
 ( #19527, #59460 ),
 ( #36175, #29100 ),
 ( #36670, #42769 ),
 ( #97041, #89928 ),
 ( #21013, #27609 ),
 ( #20506, #12407 ),
 ( #89448, #44275 ),
 ( #74719, #75205 ),
 ( #50883, #43774 ),
 ( #5782, #20004 ),
 ( #81831, #43273 ),
 ( #67578, #98510 ),
 ( #74220, #90938 ),
 ( #4809, #21488 ),
 ( #52379, #66591 ),
 ( #68077, #37662 ),
 ( #22480, #61954 ),
 ( #84815, #14870 ),
 ( #68573, #92906 ),
 ( #181, #46775 ) ),
 .UNSPECIFIED., .T., .F., .F.,
 ( 4, 2, 2, 2, 2, 2, 2, 2, 2, 2, 2, 2, 2, 2, 2, 2, 4 ),
 ( 2, 2 ),
 ( 0.000000000000000000, 0.06250000000000000000, 0.1250000000000000000, 0.1875000000000000000, 0.2500000000000000000, 0.3125000000000000000, 0.3750000000000000000, 0.4375000000000000000, 0.5000000000000000000, 0.5625000000000000000, 0.6250000000000000000, 0.6875000000000000000, 0.7500000000000000000, 0.8125000000000000000, 0.8750000000000000000, 0.9375000000000000000, 1.000000000000000000 ),
 ( 0.000000000000000000, 1.000000000000000000 ),
 .UNSPECIFIED. ) ;
#20925=ORIENTED_EDGE ( 'NONE', *, *, #45457, .T. ) ;
#20926=CARTESIAN_POINT ( 'NONE',  ( 177.8254925427601449, 279.4843545943256231, -16.44570388904381986 ) ) ;
#20927=CARTESIAN_POINT ( 'NONE',  ( 172.3690860356537655, 263.8130983119961570, -15.50581088013947273 ) ) ;
#20930=CARTESIAN_POINT ( 'NONE',  ( 94.39539123479723060, 213.7592609112380160, 2.679491924311254714 ) ) ;
#20931=CARTESIAN_POINT ( 'NONE',  ( 147.0456760057551833, 275.9564134551570760, -3.678503029046952033 ) ) ;
#20932=ORIENTED_EDGE ( 'NONE', *, *, #49251, .T. ) ;
#20936=CARTESIAN_POINT ( 'NONE',  ( 169.0812390597727131, 272.3489582993335603, 16.78971480844334963 ) ) ;
#20937=CARTESIAN_POINT ( 'NONE',  ( 190.9498149295421570, 299.9122141765958531, -5.138500224925297566 ) ) ;
#20938=CARTESIAN_POINT ( 'NONE',  ( 188.5431557236284448, 298.7030506545673347, -4.948255474722738079 ) ) ;
#20939=CARTESIAN_POINT ( 'NONE',  ( 143.8748646542946972, 242.3262482093457777, 3.021315404115420679E-15 ) ) ;
#20940=CARTESIAN_POINT ( 'NONE',  ( 192.8010417052266234, 296.7057953447782097, 12.10593424093686643 ) ) ;
#20941=CARTESIAN_POINT ( 'NONE',  ( 191.8416637716208299, 298.3674866694441334, 8.941921481404037308 ) ) ;
#20942=CARTESIAN_POINT ( 'NONE',  ( 146.5310397537613483, 276.8477895910274356, -0.2793038414862049068 ) ) ;
#20945=CARTESIAN_POINT ( 'NONE',  ( 197.0184425104562820, 289.4010428742387262, -16.90752553128928426 ) ) ;
#20946=CARTESIAN_POINT ( 'NONE',  ( 205.8610808625997208, 274.0851439753691920, 10.38803237360972531 ) ) ;
#20950=CARTESIAN_POINT ( 'NONE',  ( 101.4461556848294492, 235.5024278399160949, -9.188101187500093303 ) ) ;
#20951=VERTEX_POINT ( 'NONE', #47197 ) ;
#20952=CARTESIAN_POINT ( 'NONE',  ( 190.2557389001687511, 301.1143891237862817, -3.302524770651862784 ) ) ;
#20954=DIRECTION ( 'NONE',  ( -0.8660254037844387076, -0.4999999999999998890, -0.000000000000000000 ) ) ;
#20956=CARTESIAN_POINT ( 'NONE',  ( 160.4869048512927918, 252.6755221785256822, -16.09843817406293809 ) ) ;
#20957=CARTESIAN_POINT ( 'NONE',  ( 147.9236371514436996, 274.4357401437532076, -9.513995150070424955 ) ) ;
#20959=CARTESIAN_POINT ( 'NONE',  ( 170.5132574684816120, 255.5220156066502852, -11.62455434932883769 ) ) ;
#20962=CARTESIAN_POINT ( 'NONE',  ( 206.9026071836525205, 272.2811674698855313, 7.240992997279449561 ) ) ;
#20963=CARTESIAN_POINT ( 'NONE',  ( 34.21208616421487392, 183.8927522451417929, -10.00000000000009059 ) ) ;
#20964=CARTESIAN_POINT ( 'NONE',  ( 121.2028808523094767, 228.5327760586659451, 1.948934522072302763E-15 ) ) ;
#20966=AXIS2_PLACEMENT_3D ( 'NONE', #60573, #61578, #92528 ) ;
#20967=CARTESIAN_POINT ( 'NONE',  ( 163.3740049908953438, 249.6749180501957710, -11.76522313559978627 ) ) ;
#20968=CARTESIAN_POINT ( 'NONE',  ( 105.0197468877793625, 219.8932355074535678, -2.679491924311248496 ) ) ;
#20969=CARTESIAN_POINT ( 'NONE',  ( 174.9435373006569421, 253.2161234547149604, -3.877573368771597195 ) ) ;
#20970=CARTESIAN_POINT ( 'NONE',  ( 44.74898890052324418, 187.4548013555409796, -4.594050593750042211 ) ) ;
#20975=CARTESIAN_POINT ( 'NONE',  ( 180.8664914282228722, 267.5501807654961226, 15.00410415709774270 ) ) ;
#20978=CARTESIAN_POINT ( 'NONE',  ( 161.8750289368003621, 250.2712207352165592, -13.97436367953006098 ) ) ;
#20980=CARTESIAN_POINT ( 'NONE',  ( 179.4151417752438817, 287.8800236340311471, -12.58290191272617520 ) ) ;
#20982=CARTESIAN_POINT ( 'NONE',  ( 93.96783902534107824, 238.3927522451419350, 2.944929066748280225E-16 ) ) ;
#20985=CARTESIAN_POINT ( 'NONE',  ( 194.8262681699237930, 266.4033461770301869, -7.730570064367828564 ) ) ;
#20986=CARTESIAN_POINT ( 'NONE',  ( 202.3421728196210552, 280.1800714929709670, 16.85915999540957344 ) ) ;
#20987=CARTESIAN_POINT ( 'NONE',  ( 154.2853090730916676, 265.4170011543745886, 17.16471700533586642 ) ) ;
#20990=CARTESIAN_POINT ( 'NONE',  ( 15.38522827951586081, 173.5643266524160140, -9.188101187500093303 ) ) ;
#20995=CARTESIAN_POINT ( 'NONE',  ( 50.35065686154756293, 206.0024278399160949, 9.188101187500095079 ) ) ;
#20996=CARTESIAN_POINT ( 'NONE',  ( 163.7012083107868534, 247.1081852757374975, -6.544933039329257518 ) ) ;
#20997=CARTESIAN_POINT ( 'NONE',  ( 203.6965450807731770, 276.1611523005571485, 13.27569016410228109 ) ) ;
#20999=CARTESIAN_POINT ( 'NONE',  ( 207.6918009085542849, 270.9142438413412037, 7.009114282139513818 ) ) ;
#21000=ORIENTED_EDGE ( 'NONE', *, *, #18207, .T. ) ;
#21001=CARTESIAN_POINT ( 'NONE',  ( 10.41442975960284834, 183.4865022471903160, 10.00000000000009237 ) ) ;
#21003=CARTESIAN_POINT ( 'NONE',  ( 139.3076170325891212, 260.4244531367911577, -4.594050593750046652 ) ) ;
#21005=CARTESIAN_POINT ( 'NONE',  ( 207.5820376350654612, 271.1043594078285537, -7.625615357094640778 ) ) ;
#21008=CARTESIAN_POINT ( 'NONE',  ( 196.3519702320103590, 290.5554067223432639, 17.39042812051341969 ) ) ;
#21009=CARTESIAN_POINT ( 'NONE',  ( 188.7211440809105341, 289.5549014049189509, 14.43271874758353235 ) ) ;
#21012=CARTESIAN_POINT ( 'NONE',  ( 191.4484954869714954, 299.0484741143815199, 8.684991747358081327 ) ) ;
#21013=CARTESIAN_POINT ( 'NONE',  ( 207.7972699113062731, 270.7315661699511224, -1.706133800161685476 ) ) ;
#21015=CARTESIAN_POINT ( 'NONE',  ( 169.6032317452356324, 266.0645475789909824, -16.96121667089491325 ) ) ;
#21021=CARTESIAN_POINT ( 'NONE',  ( 196.2244288253768048, 270.9124372856092577, 12.11018688171617619 ) ) ;
#21022=CARTESIAN_POINT ( 'NONE',  ( 183.7603294395054832, 295.5481930741308929, 4.675700597948987181 ) ) ;
#21024=CARTESIAN_POINT ( 'NONE',  ( 150.7575236960178700, 277.9469932911979981, -5.090193068913281593E-05 ) ) ;
#21026=ORIENTED_EDGE ( 'NONE', *, *, #53690, .F. ) ;
#21027=CARTESIAN_POINT ( 'NONE',  ( 194.3413770922408617, 282.8930799310762723, 17.82077676852630077 ) ) ;
#21033=CARTESIAN_POINT ( 'NONE',  ( 159.4145189439792887, 263.9450760762234722, -17.23651461227130710 ) ) ;
#21036=CARTESIAN_POINT ( 'NONE',  ( 191.8000917695741805, 298.4394914891611847, -9.452573400474340914 ) ) ;
#21037=LINE ( 'NONE', #27133, #5516 ) ;
#21038=CARTESIAN_POINT ( 'NONE',  ( 204.8284483594339065, 275.8737159363993214, 14.69997973035875383 ) ) ;
#21039=CARTESIAN_POINT ( 'NONE',  ( 49.89075441544350298, 209.6115022471903160, -5.000000000000047962 ) ) ;
#21040=ORIENTED_EDGE ( 'NONE', *, *, #82849, .T. ) ;
#21041=CARTESIAN_POINT ( 'NONE',  ( 86.23641098298273278, 232.8464784336661353, 1.353441290958777525E-15 ) ) ;
#21044=CARTESIAN_POINT ( 'NONE',  ( 181.8616327328832085, 257.2205658361911560, -6.091144281000731020 ) ) ;
#21046=ORIENTED_EDGE ( 'NONE', *, *, #39023, .T. ) ;
#21047=ADVANCED_FACE ( 'NONE', ( #76612 ), #38082, .T. ) ;
#21048=CARTESIAN_POINT ( 'NONE',  ( 207.2939815914345161, 270.5662793833256501, 1.732060402802277022 ) ) ;
#21054=AXIS2_PLACEMENT_3D ( 'NONE', #71697, #86431, #24561 ) ;
#21055=VERTEX_POINT ( 'NONE', #86767 ) ;
#21056=CARTESIAN_POINT ( 'NONE',  ( 165.0728672701316100, 244.7324022674953312, 1.876804411200113210 ) ) ;
#21061=CARTESIAN_POINT ( 'NONE',  ( 18.71383987920379255, 171.6115022471901739, -5.000000000000041744 ) ) ;
#21062=B_SPLINE_CURVE_WITH_KNOTS ( 'NONE', 3,
 ( #13790, #6190, #98416, #68476 ),
 .UNSPECIFIED., .F., .F.,
 ( 4, 4 ),
 ( 0.002244590204956481774, 0.004621833422667826624 ),
 .UNSPECIFIED. ) ;
#21064=CARTESIAN_POINT ( 'NONE',  ( 164.7521862919904549, 265.1279320591024202, -16.62063656794546418 ) ) ;
#21068=VERTEX_POINT ( 'NONE', #2625 ) ;
#21070=CARTESIAN_POINT ( 'NONE',  ( 165.4473470637335879, 246.0837842385732301, 3.196113342258863899 ) ) ;
#21071=CARTESIAN_POINT ( 'NONE',  ( 199.9558687439891855, 270.1792697243771499, 10.11239592992032144 ) ) ;
#21073=LINE ( 'NONE', #30640, #57693 ) ;
#21074=CARTESIAN_POINT ( 'NONE',  ( 159.9997000813754084, 253.5193855937126841, -16.28798248637880519 ) ) ;
#21075=CARTESIAN_POINT ( 'NONE',  ( 149.9429820946090217, 276.2925415708097034, -5.357056126780523009 ) ) ;
#21076=CARTESIAN_POINT ( 'NONE',  ( 165.1821270928554952, 246.6881764609589425, -1.872407309469820813 ) ) ;
#21081=FACE_OUTER_BOUND ( 'NONE', #88630, .T. ) ;
#21086=CARTESIAN_POINT ( 'NONE',  ( 174.9842232683056409, 281.3912648188263006, -14.16965494358151290 ) ) ;
#21087=CARTESIAN_POINT ( 'NONE',  ( 204.0342455540030926, 277.2493155469190356, -14.37282112774435028 ) ) ;
#21089=CARTESIAN_POINT ( 'NONE',  ( 104.9037214839949002, 219.8262482093457777, 3.021315404115420679E-15 ) ) ;
#21090=CARTESIAN_POINT ( 'NONE',  ( -3.126064726376516667, 162.8768266524159856, -9.188101187500091527 ) ) ;
#21091=CARTESIAN_POINT ( 'NONE',  ( 115.4120517331926408, 225.8932355074535678, -2.679491924311248496 ) ) ;
#21092=CARTESIAN_POINT ( 'NONE',  ( 188.9023514920928619, 296.9480906869840737, 8.133443239242762246 ) ) ;
#21093=ORIENTED_EDGE ( 'NONE', *, *, #52522, .T. ) ;
#21095=LINE ( 'NONE', #83908, #66220 ) ;
#21101=CARTESIAN_POINT ( 'NONE',  ( 149.7728113105055172, 277.1702417969415251, 3.080250329875358961 ) ) ;
#21102=CARTESIAN_POINT ( 'NONE',  ( 26.88721494746919660, 177.1423013555409796, -4.594050593750043987 ) ) ;
#21104=CARTESIAN_POINT ( 'NONE',  ( 186.2154994046558159, 296.8723033710291475, -7.399325338573278010 ) ) ;
#21108=EDGE_CURVE ( 'NONE', #65984, #16838, #11145, .T. ) ;
#21109=CARTESIAN_POINT ( 'NONE',  ( 190.7618201014540773, 299.8460682594623563, -4.647714112044580403 ) ) ;
#21111=CARTESIAN_POINT ( 'NONE',  ( 207.8718670335145475, 270.6023601641878713, -6.322166851501095586 ) ) ;
#21112=CARTESIAN_POINT ( 'NONE',  ( 194.3442947553755005, 294.0328026529847421, -15.97648891113594871 ) ) ;
#21115=CARTESIAN_POINT ( 'NONE',  ( 172.5891611840680469, 287.6914292476137689, -9.739357961162628641 ) ) ;
#21116=CARTESIAN_POINT ( 'NONE',  ( 162.6382063110229410, 251.1910714611167919, -12.78875127087469998 ) ) ;
#21117=CARTESIAN_POINT ( 'NONE',  ( 51.53259423990365207, 193.8927522451418213, 10.00000000000009948 ) ) ;
#21119=CARTESIAN_POINT ( 'NONE',  ( 172.8718622337294732, 262.9888249722745286, -15.65873574236441357 ) ) ;
#21120=EDGE_CURVE ( 'NONE', #15680, #8119, #72705, .T. ) ;
#21121=CARTESIAN_POINT ( 'NONE',  ( 102.2314250767153538, 220.6423013555409796, -4.594050593750043987 ) ) ;
#21124=CARTESIAN_POINT ( 'NONE',  ( 157.3412122618683497, 258.1240215684019290, 16.75554199904894048 ) ) ;
#21125=CARTESIAN_POINT ( 'NONE',  ( 200.4541693463981744, 283.4501894334596841, 17.82706366043037960 ) ) ;
#21126=CARTESIAN_POINT ( 'NONE',  ( 149.6746633631864825, 271.4028737796298856, 12.81448833497433881 ) ) ;
#21127=CARTESIAN_POINT ( 'NONE',  ( 151.1811967613751335, 268.7934813906678642, -15.79361349403328418 ) ) ;
#21130=CARTESIAN_POINT ( 'NONE',  ( 147.2567621633200474, 275.5908015054806128, -3.647191014543873955 ) ) ;
#21135=CARTESIAN_POINT ( 'NONE',  ( 193.2100161762185735, 295.9974307820218087, -12.46499585622781758 ) ) ;
#21137=ORIENTED_EDGE ( 'NONE', *, *, #31757, .T. ) ;
#21139=CARTESIAN_POINT ( 'NONE',  ( 159.4889735931715222, 254.4039898200529706, 16.88104032092801887 ) ) ;
#21140=CARTESIAN_POINT ( 'NONE',  ( 193.8324327182400282, 288.0664881071944023, 17.07309623557379297 ) ) ;
#21141=DIRECTION ( 'NONE',  ( -0.8660254037844387076, -0.4999999999999998890, -0.000000000000000000 ) ) ;
#21143=CARTESIAN_POINT ( 'NONE',  ( 135.6272693901030095, 249.1115022471902591, 10.00000000000009592 ) ) ;
#21150=ORIENTED_EDGE ( 'NONE', *, *, #59561, .T. ) ;
#21151=CARTESIAN_POINT ( 'NONE',  ( 181.4476193698807549, 290.8642548751454342, -11.08784992509195000 ) ) ;
#21153=CARTESIAN_POINT ( 'NONE',  ( 164.7124890890957545, 259.3090575768129042, 16.88404478802990738 ) ) ;
#21154=CARTESIAN_POINT ( 'NONE',  ( 158.8074094763257449, 255.5844934990455499, 17.62168084431520043 ) ) ;
#21155=CARTESIAN_POINT ( 'NONE',  ( 190.7959044753356181, 278.1545862522023640, -16.79819019203270969 ) ) ;
#21156=CARTESIAN_POINT ( 'NONE',  ( 153.8428010968516162, 264.1834474519768605, -18.07686942510439110 ) ) ;
#21157=CARTESIAN_POINT ( 'NONE',  ( 201.1060504099706350, 282.3210983108598384, -18.18000168485860257 ) ) ;
#21160=EDGE_CURVE ( 'NONE', #20583, #81472, #66752, .T. ) ;
#21163=EDGE_LOOP ( 'NONE', ( #40925, #66595, #78013, #23768, #54126, #58653, #54028, #7796, #35081, #82983, #84493, #54529, #78136, #69192, #12026, #44690, #68321, #69259, #58393, #585, #53764, #68096, #30974, #75224, #22864, #31810, #98451, #62256, #79617, #15498, #28649, #98146, #81282, #29006, #24781, #79127, #94297, #99261, #31084, #36565, #267, #92704, #61875, #51069, #40839, #45924, #73343, #25878, #85832, #10819, #27226, #66995, #10321, #51176 ) ) ;
#21166=CARTESIAN_POINT ( 'NONE',  ( 204.9427641582406636, 275.6757151647582305, 14.40446820030680897 ) ) ;
#21168=CARTESIAN_POINT ( 'NONE',  ( 199.3225951545807106, 279.5975192435293479, 16.97220939274292206 ) ) ;
#21169=CARTESIAN_POINT ( 'NONE',  ( 197.4063992150350373, 273.1943876493294852, -13.35659089524287602 ) ) ;
#21172=CARTESIAN_POINT ( 'NONE',  ( 171.0233422444486280, 287.7839941292462527, -4.495013932621471753 ) ) ;
#21173=EDGE_CURVE ( 'NONE', #20256, #85118, #19598, .T. ) ;
#21175=CARTESIAN_POINT ( 'NONE',  ( 178.1648171342568219, 255.5065660826824114, 4.897822005985157823 ) ) ;
#21176=CARTESIAN_POINT ( 'NONE',  ( 116.7098534265301595, 244.3149278399160949, -9.188101187500095079 ) ) ;
#21177=ORIENTED_EDGE ( 'NONE', *, *, #12730, .F. ) ;
#21178=CARTESIAN_POINT ( 'NONE',  ( 148.0632853866802350, 275.0336310366062094, -5.814038160505428543 ) ) ;
#21179=CARTESIAN_POINT ( 'NONE',  ( 187.1789365411204926, 291.3781964708418286, -14.15416893886036220 ) ) ;
#21182=CARTESIAN_POINT ( 'NONE',  ( 184.5564966555429862, 297.9066928836515444, -1.116615600582069101 ) ) ;
#21183=CARTESIAN_POINT ( 'NONE',  ( 180.7178857814544699, 294.1703499652309119, -2.354211428759664493 ) ) ;
#21184=CARTESIAN_POINT ( 'NONE',  ( 157.8562613713738472, 257.2319303423452652, 17.81420683562559404 ) ) ;
#21185=CARTESIAN_POINT ( 'NONE',  ( 159.9647205790309101, 253.5799718689968927, -16.48298384325780219 ) ) ;
#21188=AXIS2_PLACEMENT_3D ( 'NONE', #38049, #38557, #52272 ) ;
#21189=ORIENTED_EDGE ( 'NONE', *, *, #7613, .F. ) ;
#21193=CARTESIAN_POINT ( 'NONE',  ( -7.429302001086912632, 166.5177522451418781, -10.00000000000009592 ) ) ;
#21195=CARTESIAN_POINT ( 'NONE',  ( 198.0482269745670862, 285.9982792772420908, 17.61538258229827747 ) ) ;
#21197=CARTESIAN_POINT ( 'NONE',  ( 200.9445292274600092, 282.6008612054670266, -16.62830946367346741 ) ) ;
#21199=CARTESIAN_POINT ( 'NONE',  ( 157.1187995864133882, 258.5092516225370218, 18.42986330599266509 ) ) ;
#21200=CARTESIAN_POINT ( 'NONE',  ( 174.5885488454506174, 256.4458599265808516, 12.05082362884263425 ) ) ;
#21201=CARTESIAN_POINT ( 'NONE',  ( 189.8223291672571236, 263.2674012269775972, -9.776181882378969235 ) ) ;
#21202=CARTESIAN_POINT ( 'NONE',  ( 173.4224352300193175, 251.4084521971564072, -0.8939200208722334340 ) ) ;
#21203=CARTESIAN_POINT ( 'NONE',  ( 178.1545585138619572, 285.2582789952114126, 13.03273863630066209 ) ) ;
#21206=FACE_OUTER_BOUND ( 'NONE', #74359, .T. ) ;
#21208=CARTESIAN_POINT ( 'NONE',  ( 55.84441874286383722, 212.2369531367911293, -4.594050593750048428 ) ) ;
#21209=CARTESIAN_POINT ( 'NONE',  ( 159.2186641046529303, 254.8721795879351646, -15.96198087403305443 ) ) ;
#21210=DIRECTION ( 'NONE',  ( 0.5000000000000001110, -0.8660254037844387076, 0.000000000000000000 ) ) ;
#21211=CARTESIAN_POINT ( 'NONE',  ( 162.9111474110223412, 248.4766108952035211, -9.702990628959184960 ) ) ;
#21214=CARTESIAN_POINT ( 'NONE',  ( 207.2337123599961899, 271.7076764818092443, -5.443417788256701861 ) ) ;
#21217=CARTESIAN_POINT ( 'NONE',  ( 111.7912168577913974, 246.8967562850347122, -4.648177544792955347E-16 ) ) ;
#21220=CYLINDRICAL_SURFACE ( 'NONE', #43364, 17.82106496071139645 ) ;
#21228=CARTESIAN_POINT ( 'NONE',  ( 47.42782112377506820, 204.3149278399161233, 9.188101187500093303 ) ) ;
#21230=DIRECTION ( 'NONE',  ( 0.8660254037844395958, 0.4999999999999985567, 0.000000000000000000 ) ) ;
#21231=CARTESIAN_POINT ( 'NONE',  ( 149.6230451358742926, 271.4922791719315001, -12.72565967355361671 ) ) ;
#21233=CARTESIAN_POINT ( 'NONE',  ( 198.0457135053186448, 287.1931070555794463, 16.94346135465734449 ) ) ;
#21234=CARTESIAN_POINT ( 'NONE',  ( 175.6626792159711670, 291.0177071100450235, 2.486975767635404733 ) ) ;
#21235=CARTESIAN_POINT ( 'NONE',  ( 180.0647771456566204, 276.3369416177878293, 17.44453780294904632 ) ) ;
#21238=CARTESIAN_POINT ( 'NONE',  ( 163.3406587279032181, 256.0941660840857139, -14.91928245677631004 ) ) ;
#21240=VECTOR ( 'NONE', #27486, 1000.000000000000000 ) ;
#21242=CARTESIAN_POINT ( 'NONE',  ( 99.25420243115651431, 238.1115022471902876, -5.000000000000047962 ) ) ;
#21243=CARTESIAN_POINT ( 'NONE',  ( 200.5621507313343557, 283.2631601884785368, 16.81037192529623425 ) ) ;
#21244=CARTESIAN_POINT ( 'NONE',  ( 164.8669435086126498, 270.4944952562744334, -16.92984481350135084 ) ) ;
#21246=CARTESIAN_POINT ( 'NONE',  ( 56.62968813474974894, 197.3768266524160140, -9.188101187500091527 ) ) ;
#21249=CARTESIAN_POINT ( 'NONE',  ( 146.8000281410530192, 276.3818880375922049, 4.652863924796177386 ) ) ;
#21251=VERTEX_POINT ( 'NONE', #4606 ) ;
#21255=CARTESIAN_POINT ( 'NONE',  ( 177.1935088715161157, 274.8242815821236036, -17.29576750977079769 ) ) ;
#21256=CARTESIAN_POINT ( 'NONE',  ( 206.6389649419900536, 271.5030152196637800, -6.665702415263554670 ) ) ;
#21257=CARTESIAN_POINT ( 'NONE',  ( 204.6861706212249885, 276.1201482077632363, 14.69005155300678922 ) ) ;
#21258=VERTEX_POINT ( 'NONE', #35496 ) ;
#21261=CARTESIAN_POINT ( 'NONE',  ( 190.7404869014439726, 298.2747809567102308, -9.591077548819823662 ) ) ;
#21262=CARTESIAN_POINT ( 'NONE',  ( 175.0387250457744983, 253.3993311541219953, -7.863511161993287146 ) ) ;
#21263=ADVANCED_FACE ( 'NONE', ( #66400 ), #55316, .F. ) ;
#21267=CARTESIAN_POINT ( 'NONE',  ( 166.9356869029893460, 261.4657499883571177, 16.52387450907458799 ) ) ;
#21268=CARTESIAN_POINT ( 'NONE',  ( 206.0870578475358172, 273.6937403561189512, -10.07771901274806581 ) ) ;
#21269=ORIENTED_EDGE ( 'NONE', *, *, #57284, .T. ) ;
#21270=EDGE_CURVE ( 'NONE', #79646, #73728, #73859, .T. ) ;
#21272=DIRECTION ( 'NONE',  ( 0.4999999999999992784, -0.8660254037844390407, 0.000000000000000000 ) ) ;
#21273=CARTESIAN_POINT ( 'NONE',  ( 207.6523394534040392, 270.9825930866021508, -2.115019688068903392 ) ) ;
#21275=CARTESIAN_POINT ( 'NONE',  ( 188.4688990864094080, 295.3997683978527675, -11.43812978727723717 ) ) ;
#21277=CARTESIAN_POINT ( 'NONE',  ( 164.6182694729110949, 265.1159723368043615, -16.62666970452827186 ) ) ;
#21278=CARTESIAN_POINT ( 'NONE',  ( 130.8102634016018442, 237.1423013555409796, -4.594050593750043987 ) ) ;
#21279=ADVANCED_FACE ( 'NONE', ( #82535 ), #43959, .T. ) ;
#21280=B_SPLINE_CURVE_WITH_KNOTS ( 'NONE', 3,
 ( #77394, #45474, #39357, #92140 ),
 .UNSPECIFIED., .F., .F.,
 ( 4, 4 ),
 ( 0.03072821384799830427, 0.03979477762634543725 ),
 .UNSPECIFIED. ) ;
#21284=DIRECTION ( 'NONE',  ( 0.4999999999999998890, -0.8660254037844385966, 0.000000000000000000 ) ) ;
#21286=CARTESIAN_POINT ( 'NONE',  ( 201.2310239275262518, 281.6122570310417359, 16.42038788625619716 ) ) ;
#21287=ORIENTED_EDGE ( 'NONE', *, *, #21108, .F. ) ;
#21290=CARTESIAN_POINT ( 'NONE',  ( 149.3118911495987788, 247.0312136851381126, 5.028230608967417581 ) ) ;
#21292=EDGE_CURVE ( 'NONE', #1341, #69600, #6283, .T. ) ;
#21293=CARTESIAN_POINT ( 'NONE',  ( 191.0050299662194107, 260.5068323652516824, -0.1977049704586299195 ) ) ;
#21296=CARTESIAN_POINT ( 'NONE',  ( 155.3738696901333469, 261.5315588585399951, 17.02116401938635804 ) ) ;
#21300=CARTESIAN_POINT ( 'NONE',  ( 152.6873874250818517, 266.1846826352417565, -16.66598363829485763 ) ) ;
#21302=ORIENTED_EDGE ( 'NONE', *, *, #4908, .T. ) ;
#21304=CARTESIAN_POINT ( 'NONE',  ( 174.7528540796445213, 253.3049902866633261, -7.833201063209856763 ) ) ;
#21305=CARTESIAN_POINT ( 'NONE',  ( 164.3090168944849836, 246.0554299274959931, 2.641760039552302430 ) ) ;
#21306=CARTESIAN_POINT ( 'NONE',  ( 198.9892818938948551, 281.0772271664100117, 17.34293942954158751 ) ) ;
#21307=CARTESIAN_POINT ( 'NONE',  ( 164.1821508476733698, 246.2751683663292397, -7.347745041495428175 ) ) ;
#21308=CARTESIAN_POINT ( 'NONE',  ( 133.4890956248536895, 254.0024278399161233, 9.188101187500095079 ) ) ;
#21309=ORIENTED_EDGE ( 'NONE', *, *, #48446, .F. ) ;
#21318=CARTESIAN_POINT ( 'NONE',  ( 182.2771148168560842, 275.8536480385645291, -16.43645293322504486 ) ) ;
#21319=CARTESIAN_POINT ( 'NONE',  ( 165.3447893439585243, 247.5681563451806824, -5.571162280481247286 ) ) ;
#21321=CARTESIAN_POINT ( 'NONE',  ( 202.3532268619428862, 267.6858343578610402, 0.8563957037533130867 ) ) ;
#21322=CARTESIAN_POINT ( 'NONE',  ( 190.1693911629507738, 301.2639477917662703, -5.112716700269980485 ) ) ;
#21323=CARTESIAN_POINT ( 'NONE',  ( 183.4588200504678355, 280.8776272736768647, 16.45139132406686144 ) ) ;
#21325=CARTESIAN_POINT ( 'NONE',  ( 204.6713671561005299, 276.1457885614869951, -12.94307097876490431 ) ) ;
#21326=CARTESIAN_POINT ( 'NONE',  ( 194.8104010662821111, 269.9905278424700441, 12.02357665573980405 ) ) ;
#21331=CARTESIAN_POINT ( 'NONE',  ( 159.9628729326222754, 253.5831720864507588, 15.75051413866357386 ) ) ;
#21332=CARTESIAN_POINT ( 'NONE',  ( 161.2816932310574884, 251.2989083235077032, 13.15717084518158764 ) ) ;
#21333=CARTESIAN_POINT ( 'NONE',  ( 147.1562325744354212, 255.7677522451418781, 10.00000000000009592 ) ) ;
#21334=CARTESIAN_POINT ( 'NONE',  ( 172.2123999945063417, 283.8628369387304815, -12.71294468390556887 ) ) ;
#21336=EDGE_CURVE ( 'NONE', #25811, #26754, #91335, .T. ) ;
#21339=CARTESIAN_POINT ( 'NONE',  ( 150.9115585710837877, 269.2605084359132093, -15.80434701481532578 ) ) ;
#21340=CARTESIAN_POINT ( 'NONE',  ( 6.400214715252306341, 168.3768266524160140, 9.188101187500096856 ) ) ;
#21342=CARTESIAN_POINT ( 'NONE',  ( 181.6561284561640832, 276.3695326334836295, -16.98996653829426862 ) ) ;
#21348=CARTESIAN_POINT ( 'NONE',  ( 150.1387292596415648, 276.5099847689000967, 3.745717586651703179 ) ) ;
#21349=CARTESIAN_POINT ( 'NONE',  ( 196.2467569046250162, 269.4493588965917183, -10.72705572559448761 ) ) ;
#21350=CARTESIAN_POINT ( 'NONE',  ( 74.41009865654258704, 203.7677522451417929, -5.000000000000041744 ) ) ;
#21351=CARTESIAN_POINT ( 'NONE',  ( 176.3344142305265905, 254.0447395692417842, -3.866504412443106276 ) ) ;
#21352=EDGE_CURVE ( 'NONE', #84236, #60492, #27987, .T. ) ;
#21353=CARTESIAN_POINT ( 'NONE',  ( 198.5799742811345823, 286.6963905097911152, 17.08859794237710261 ) ) ;
#21355=CARTESIAN_POINT ( 'NONE',  ( 64.10800479423814124, 194.4865022471901739, 1.119607411625061291E-15 ) ) ;
#21357=CARTESIAN_POINT ( 'NONE',  ( 190.4750160083620472, 300.7345900314585947, -1.159659205620361400 ) ) ;
#21358=CARTESIAN_POINT ( 'NONE',  ( 21.36630299834339652, 173.9548013555409796, -4.594050593750042211 ) ) ;
#21359=CARTESIAN_POINT ( 'NONE',  ( 167.6841820197852257, 287.3320466105657260, 4.942676059668591471 ) ) ;
#21362=CARTESIAN_POINT ( 'NONE',  ( 202.1695757186951994, 279.6930204168322689, -15.81993831395799077 ) ) ;
#21363=DIRECTION ( 'NONE',  ( -0.8660254037844387076, -0.4999999999999998890, -0.000000000000000000 ) ) ;
#21364=CARTESIAN_POINT ( 'NONE',  ( 185.1889932722985748, 266.7802408231123081, 13.62321108638839462 ) ) ;
#21368=CARTESIAN_POINT ( 'NONE',  ( 165.4973148452406804, 285.5633041981129736, -0.04349354715313477615 ) ) ;
#21369=CYLINDRICAL_SURFACE ( 'NONE', #75888, 10.00000000000010658 ) ;
#21372=ORIENTED_EDGE ( 'NONE', *, *, #62001, .T. ) ;
#21373=CARTESIAN_POINT ( 'NONE',  ( 183.9962501225037101, 290.1813357568594824, 12.16961482813081474 ) ) ;
#21381=CARTESIAN_POINT ( 'NONE',  ( 155.6066474290145720, 261.1283759879266881, -18.16552045242181279 ) ) ;
#21386=LINE ( 'NONE', #52273, #44259 ) ;
#21387=ORIENTED_EDGE ( 'NONE', *, *, #77658, .T. ) ;
#21392=ORIENTED_EDGE ( 'NONE', *, *, #82260, .T. ) ;
#21395=EDGE_CURVE ( 'NONE', #11048, #2437, #52203, .T. ) ;
#21396=CARTESIAN_POINT ( 'NONE',  ( 43.68655075043449898, 184.4824982072973967, 3.021315404115420679E-15 ) ) ;
#21397=ORIENTED_EDGE ( 'NONE', *, *, #64850, .T. ) ;
#21398=CARTESIAN_POINT ( 'NONE',  ( 164.2572333502590709, 246.1451216570909253, 2.155809084027023204 ) ) ;
#21401=ORIENTED_EDGE ( 'NONE', *, *, #34080, .T. ) ;
#21402=CARTESIAN_POINT ( 'NONE',  ( 175.6393304058065610, 277.9438274558168018, -15.68642701745271495 ) ) ;
#21403=CARTESIAN_POINT ( 'NONE',  ( 172.1807612816075448, 264.1729231858467983, -16.32128620121408957 ) ) ;
#21406=CARTESIAN_POINT ( 'NONE',  ( 158.6328712587097414, 275.0136024797188270, -12.55550228384817757 ) ) ;
#21409=VERTEX_POINT ( 'NONE', #69763 ) ;
#21412=CARTESIAN_POINT ( 'NONE',  ( 147.5693121967435957, 275.0494489676833041, 4.210973343677100189 ) ) ;
#21415=CARTESIAN_POINT ( 'NONE',  ( 153.4477557824949940, 264.8676860077344486, 17.16010094972647693 ) ) ;
#21416=CARTESIAN_POINT ( 'NONE',  ( 147.0160867267995854, 276.0076635896675725, 0.7715638482002742382 ) ) ;
#21417=CARTESIAN_POINT ( 'NONE',  ( 191.8232488616404225, 298.3993822291468518, -9.342381338555176384 ) ) ;
#21424=CARTESIAN_POINT ( 'NONE',  ( 167.1547084800286882, 256.3859753943238502, -15.10362562340490911 ) ) ;
#21425=VERTEX_POINT ( 'NONE', #44963 ) ;
#21426=CARTESIAN_POINT ( 'NONE',  ( 149.0943192338760070, 272.4080592974699471, -12.87526400066115606 ) ) ;
#21428=CARTESIAN_POINT ( 'NONE',  ( 148.7903119393423026, 273.3731287249261186, 9.064500856912474092 ) ) ;
#21430=CARTESIAN_POINT ( 'NONE',  ( 182.8912941787172315, 284.3928553195365794, -14.99677252371531289 ) ) ;
#21433=CARTESIAN_POINT ( 'NONE',  ( 170.5605287177041305, 255.6265081261690568, -11.70025675400036747 ) ) ;
#21435=CARTESIAN_POINT ( 'NONE',  ( 164.7694554770609159, 245.2579269087094076, -3.003635650077957742 ) ) ;
#21436=EDGE_CURVE ( 'NONE', #705, #37573, #83660, .T. ) ;
#21437=CARTESIAN_POINT ( 'NONE',  ( 36.66582480827072743, 198.6427522451419350, -10.00000000000009415 ) ) ;
#21438=CARTESIAN_POINT ( 'NONE',  ( 109.7816501962546454, 240.3149278399160949, 9.188101187500093303 ) ) ;
#21439=CARTESIAN_POINT ( 'NONE',  ( 177.5665759502285539, 275.7863988818428993, 17.69313789786682989 ) ) ;
#21442=CARTESIAN_POINT ( 'NONE',  ( 195.9713281756800427, 291.2146981034049418, 17.52210387885178022 ) ) ;
#21443=CARTESIAN_POINT ( 'NONE',  ( 172.4017459954111473, 250.5914637853330476, -4.115793628843052332 ) ) ;
#21444=CARTESIAN_POINT ( 'NONE',  ( 39.90439897628026955, 193.8458772461660544, 9.188101187500095079 ) ) ;
#21445=CARTESIAN_POINT ( 'NONE',  ( 147.6215775367315644, 275.3445823649863087, -3.142877717583205222 ) ) ;
#21448=CARTESIAN_POINT ( 'NONE',  ( 179.5196496019146650, 266.1175816663657656, 16.29367087753972498 ) ) ;
#21449=CARTESIAN_POINT ( 'NONE',  ( 30.58014428988347788, 176.9155109091896634, 2.679491924311254714 ) ) ;
#21450=CARTESIAN_POINT ( 'NONE',  ( 147.5492216329511166, 275.0842468449245644, 4.751613690710122739 ) ) ;
#21452=CARTESIAN_POINT ( 'NONE',  ( 166.6288018012914449, 255.3266329142646498, -14.67773939159194896 ) ) ;
#21453=CARTESIAN_POINT ( 'NONE',  ( 176.3126652553115150, 285.5045246447724594, -12.04976978329188242 ) ) ;
#21454=CARTESIAN_POINT ( 'NONE',  ( 164.2885300478071144, 250.0642274256680366, 10.21650006632281205 ) ) ;
#21455=CARTESIAN_POINT ( 'NONE',  ( 87.40047971330913867, 221.2677522451418497, 10.00000000000009592 ) ) ;
#21457=CARTESIAN_POINT ( 'NONE',  ( 195.3926592889443157, 266.7123800746668962, -7.757725527663858145 ) ) ;
#21458=EDGE_CURVE ( 'NONE', #77337, #6621, #96948, .T. ) ;
#21459=CARTESIAN_POINT ( 'NONE',  ( 158.7932562801271104, 282.3814901877906891, -1.645599008796116314 ) ) ;
#21461=CARTESIAN_POINT ( 'NONE',  ( 19.09298631340924501, 172.6423013555409796, -4.594050593750043987 ) ) ;
#21466=CARTESIAN_POINT ( 'NONE',  ( 194.7211787970855141, 275.0175511178182433, -15.89236621824491635 ) ) ;
#21467=CARTESIAN_POINT ( 'NONE',  ( 63.26028190641562787, 198.1423013555410080, -4.594050593750043987 ) ) ;
#21468=CARTESIAN_POINT ( 'NONE',  ( 163.9910908123517288, 246.6060940548019289, -7.333295033952830444 ) ) ;
#21470=EDGE_CURVE ( 'NONE', #77729, #15709, #38913, .T. ) ;
#21472=CARTESIAN_POINT ( 'NONE',  ( 164.9779129355220562, 244.8968679994381148, -1.771286574179712803 ) ) ;
#21473=ORIENTED_EDGE ( 'NONE', *, *, #25618, .F. ) ;
#21475=( BOUNDED_CURVE ( )  B_SPLINE_CURVE ( 2, ( #52085, #50584, #89646, #65784, #59672, #11617, #20705, #75406, #27305 ),
 .UNSPECIFIED., .F., .T. ) 
 B_SPLINE_CURVE_WITH_KNOTS ( ( 3, 2, 2, 2, 3 ),
 ( 0.8669354838709677491, 0.8682795698924731242, 0.8709677419354838745, 0.8736559139784946248, 0.8750000000000000000 ),
 .UNSPECIFIED. ) 
 CURVE ( )  GEOMETRIC_REPRESENTATION_ITEM ( )  RATIONAL_B_SPLINE_CURVE ( ( 0.9330127018922194093, 0.9330127018922194093, 1.000000000000000000, 0.8660254037844387076, 1.000000000000000000, 0.8660254037844387076, 1.000000000000000000, 0.9330127018922194093, 0.9330127018922194093 ) ) 
 REPRESENTATION_ITEM ( '' )  );
#21476=CARTESIAN_POINT ( 'NONE',  ( 14.88889434582242544, 192.7365022471903444, 2.944929066748280225E-16 ) ) ;
#21477=CARTESIAN_POINT ( 'NONE',  ( 208.2939409893161553, 269.8713066281881083, 2.523744790997269227 ) ) ;
#21478=CARTESIAN_POINT ( 'NONE',  ( 134.8967340017684080, 242.5643266524159856, -9.188101187500093303 ) ) ;
#21480=CARTESIAN_POINT ( 'NONE',  ( 206.8583977782397483, 272.3577404062329492, -8.036528591665119237 ) ) ;
#21481=CARTESIAN_POINT ( 'NONE',  ( 202.4560076411394220, 279.0611292670678267, 15.58065739802832717 ) ) ;
#21482=CARTESIAN_POINT ( 'NONE',  ( 194.4090165346928529, 280.7843443599479656, -17.71307557792658116 ) ) ;
#21487=CARTESIAN_POINT ( 'NONE',  ( 166.1047324428320167, 246.6357536469371610, 3.930903826211260998 ) ) ;
#21488=CARTESIAN_POINT ( 'NONE',  ( 164.1057330408499411, 246.4075278903502237, 7.856393496352101380 ) ) ;
#21491=CARTESIAN_POINT ( 'NONE',  ( 169.9474419461124626, 266.2972067178577049, -16.74373953161226325 ) ) ;
#21492=CARTESIAN_POINT ( 'NONE',  ( 195.2321946600270337, 271.9407588785367125, -13.42877009059527538 ) ) ;
#21496=B_SPLINE_CURVE_WITH_KNOTS ( 'NONE', 3,
 ( #71492, #94807, #36450, #67353 ),
 .UNSPECIFIED., .F., .F.,
 ( 4, 4 ),
 ( 0.01205011342145419564, 0.02055108600438866617 ),
 .UNSPECIFIED. ) ;
#21499=B_SPLINE_SURFACE_WITH_KNOTS ( 'NONE', 3, 1, ( 
 ( #74330, #28699 ),
 ( #5407, #59576 ),
 ( #75318, #98114 ),
 ( #13999, #91037 ),
 ( #82941, #67697 ),
 ( #6403, #22590 ),
 ( #51494, #37287 ),
 ( #13025, #68182 ),
 ( #68679, #29694 ),
 ( #60075, #92046 ),
 ( #99111, #21605 ),
 ( #43888, #91527 ),
 ( #22090, #76313 ),
 ( #37777, #99611 ),
 ( #30188, #61074 ),
 ( #81938, #12516 ),
 ( #43388, #24083 ),
 ( #23072, #45863 ),
 ( #15986, #24580 ),
 ( #55463, #78303 ),
 ( #92526, #46885 ),
 ( #62563, #1799 ),
 ( #53966, #84923 ),
 ( #31667, #85437 ),
 ( #69682, #15469 ),
 ( #77810, #31174 ),
 ( #69181, #70173 ),
 ( #16484, #93526 ),
 ( #78803, #62064 ),
 ( #286, #47379 ),
 ( #8393, #85958 ),
 ( #9391, #46364 ),
 ( #93013, #23568 ),
 ( #54459, #77293 ) ),
 .UNSPECIFIED., .T., .F., .F.,
 ( 4, 2, 2, 2, 2, 2, 2, 2, 2, 2, 2, 2, 2, 2, 2, 2, 4 ),
 ( 2, 2 ),
 ( 0.000000000000000000, 0.06250000000000000000, 0.1250000000000000000, 0.1875000000000000000, 0.2500000000000000000, 0.3125000000000000000, 0.3750000000000000000, 0.4375000000000000000, 0.5000000000000000000, 0.5625000000000000000, 0.6250000000000000000, 0.6875000000000000000, 0.7500000000000000000, 0.8125000000000000000, 0.8750000000000000000, 0.9375000000000000000, 1.000000000000000000 ),
 ( 0.000000000000000000, 1.000000000000000000 ),
 .UNSPECIFIED. ) ;
#21500=B_SPLINE_CURVE_WITH_KNOTS ( 'NONE', 3,
 ( #71792, #31261, #95121, #1882, #87038, #56566, #23651, #8474, #93094, #64173, #46970, #39345, #56046, #868, #70770, #24664, #63669, #25686, #18085, #31747, #24173, #16068, #48981, #69765, #62652, #54542, #9481, #55056, #85525, #86039, #16567, #40352, #47463, #78388, #39839, #32265, #63168, #94112, #86532, #17062, #28164, #35266, #19097, #20580, #57058, #50957, #72298, #73779, #66662, #11985, #20086, #49975, #3398, #42841, #58069, #4368 ),
 .UNSPECIFIED., .F., .F.,
 ( 4, 2, 2, 2, 2, 2, 2, 2, 2, 2, 2, 2, 2, 2, 2, 2, 2, 2, 2, 2, 2, 2, 2, 2, 2, 2, 2, 4 ),
 ( 0.001001512342791581987, 0.001483580493562128202, 0.001965648644332674416, 0.002206682719717947307, 0.002447716795103221064, 0.002568233832795857510, 0.002688750870488493955, 0.002809267908181130400, 0.002929784945873766845, 0.003170819021259039736, 0.003411853096644312192, 0.003893921247414742614, 0.004858057548955562258, 0.005822193850496381468, 0.006304262001266755511, 0.006545296076651900032, 0.006786330152037044552, 0.006846588670883270618, 0.006906847189729496683, 0.006967105708575722749, 0.007027364227421947947, 0.007147881265114443446, 0.007268398302806938945, 0.007509432378191927340, 0.007750466453576916603, 0.007991500528961904132, 0.008232534604346893395, 0.008714602755116832022 ),
 .UNSPECIFIED. ) ;
#21503=CARTESIAN_POINT ( 'NONE',  ( 182.1922674602477628, 295.0151143605804691, 4.768981532823296732 ) ) ;
#21504=CARTESIAN_POINT ( 'NONE',  ( 163.4178923001155681, 247.5989030008181260, -10.38047187240561442 ) ) ;
#21510=EDGE_LOOP ( 'NONE', ( #87645, #15656, #78158, #54352, #79247, #90492, #97311, #11443, #66606, #63395, #78640, #20329, #14404, #5096, #41205, #60846, #2217, #3402, #19699, #24105, #77317, #16679, #54545, #17161, #65989, #28052, #13084, #92255, #8081, #47041, #38786, #13408, #92325, #24559, #68367, #19902, #65161, #73630, #8559, #24387, #5238, #22982, #94922, #34764, #23478, #51668, #36876, #72994, #63277, #5264, #32528 ) ) ;
#21514=ORIENTED_EDGE ( 'NONE', *, *, #79736, .T. ) ;
#21515=CARTESIAN_POINT ( 'NONE',  ( 191.5324528500417216, 298.9030556958743432, -8.286652526617016790 ) ) ;
#21518=CARTESIAN_POINT ( 'NONE',  ( 204.9103773355753617, 275.7318107871104189, 13.62808820451859937 ) ) ;
#21520=CARTESIAN_POINT ( 'NONE',  ( 194.3413770922408617, 282.8930799310762723, 17.82077676852630077 ) ) ;
#21522=CARTESIAN_POINT ( 'NONE',  ( 95.05956542768423390, 219.5643266524160140, 9.188101187500095079 ) ) ;
#21523=CARTESIAN_POINT ( 'NONE',  ( 155.1614028326249866, 261.8995622506689074, 18.45604204116099822 ) ) ;
#21524=CARTESIAN_POINT ( 'NONE',  ( 181.2000081644680733, 271.5771930539713708, -17.25712798740391563 ) ) ;
#21526=B_SPLINE_SURFACE_WITH_KNOTS ( 'NONE', 3, 1, ( 
 ( #51850, #67030 ),
 ( #21442, #43226 ),
 ( #68528, #75646 ),
 ( #4760, #35642 ),
 ( #82299, #98460 ),
 ( #83269, #13837 ),
 ( #29539, #14337 ),
 ( #37127, #66543 ),
 ( #58432, #68034 ),
 ( #52820, #89883 ),
 ( #20457, #12869 ),
 ( #83776, #30027 ),
 ( #46723, #31020 ),
 ( #32015, #84279 ),
 ( #70017, #93363 ),
 ( #61912, #77651 ),
 ( #84770, #137 ),
 ( #15306, #70522 ),
 ( #632, #30532 ),
 ( #71050, #38105 ),
 ( #85798, #78648 ),
 ( #69018, #22919 ),
 ( #14824, #60911 ),
 ( #92860, #7729 ),
 ( #99948, #91878 ),
 ( #62924, #46205 ),
 ( #40111, #45713 ),
 ( #31512, #55307 ),
 ( #93875, #76636 ),
 ( #38617, #8237 ),
 ( #69526, #62407 ),
 ( #85272, #77122 ),
 ( #86289, #23920 ),
 ( #61419, #22431 ) ),
 .UNSPECIFIED., .T., .F., .F.,
 ( 4, 2, 2, 2, 2, 2, 2, 2, 2, 2, 2, 2, 2, 2, 2, 2, 4 ),
 ( 2, 2 ),
 ( 0.000000000000000000, 0.06250000000000000000, 0.1250000000000000000, 0.1875000000000000000, 0.2500000000000000000, 0.3125000000000000000, 0.3750000000000000000, 0.4375000000000000000, 0.5000000000000000000, 0.5625000000000000000, 0.6250000000000000000, 0.6875000000000000000, 0.7500000000000000000, 0.8125000000000000000, 0.8750000000000000000, 0.9375000000000000000, 1.000000000000000000 ),
 ( 0.000000000000000000, 1.000000000000000000 ),
 .UNSPECIFIED. ) ;
#21529=EDGE_LOOP ( 'NONE', ( #20636, #26507, #62655, #3294 ) ) ;
#21533=CARTESIAN_POINT ( 'NONE',  ( 158.6496056213609904, 257.8578177934796258, 17.38082990300775776 ) ) ;
#21534=VERTEX_POINT ( 'NONE', #8472 ) ;
#21535=CARTESIAN_POINT ( 'NONE',  ( 164.4989919961878684, 245.7263833991736988, 2.405231973350729024 ) ) ;
#21540=CARTESIAN_POINT ( 'NONE',  ( 165.0694571955912409, 264.4563124879717293, -17.70034357220088950 ) ) ;
#21542=CARTESIAN_POINT ( 'NONE',  ( 192.0969986600162827, 271.0201763999182845, -15.22553433325905736 ) ) ;
#21546=CARTESIAN_POINT ( 'NONE',  ( 164.2602539243905539, 281.6793576088280133, 8.832505592777787129 ) ) ;
#21547=CARTESIAN_POINT ( 'NONE',  ( 9.004826742577897392, 187.5530062829863027, -4.648177544792955347E-16 ) ) ;
#21549=CARTESIAN_POINT ( 'NONE',  ( 163.1014434023538513, 248.1470085697407058, 9.692260209037655727 ) ) ;
#21550=CARTESIAN_POINT ( 'NONE',  ( 185.1754690811580701, 257.9748643125362264, 3.025625122693937463 ) ) ;
#21551=CARTESIAN_POINT ( 'NONE',  ( 160.8824536440269526, 282.3397334439140423, -6.171673602401500425 ) ) ;
#21553=CARTESIAN_POINT ( 'NONE',  ( 158.5586670023323563, 257.8002292186573072, 17.26955892278689220 ) ) ;
#21555=CARTESIAN_POINT ( 'NONE',  ( 200.3134965941964651, 283.6938417875134064, 18.29802468362849766 ) ) ;
#21556=CARTESIAN_POINT ( 'NONE',  ( 194.7554030189934622, 263.4159149995173266, -0.7846879789437617436 ) ) ;
#21557=VERTEX_POINT ( 'NONE', #55546 ) ;
#21558=CARTESIAN_POINT ( 'NONE',  ( 93.48865797453373716, 236.3297689869269220, -2.679491924311252493 ) ) ;
#21560=CARTESIAN_POINT ( 'NONE',  ( 9.692741923115875124, 169.7365022471902023, -10.00000000000009237 ) ) ;
#21562=CARTESIAN_POINT ( 'NONE',  ( 12.56145106960391011, 171.3927522451418213, 10.00000000000009592 ) ) ;
#21564=CARTESIAN_POINT ( 'NONE',  ( 174.9738539119461223, 281.6573486160436346, -14.08158005805571023 ) ) ;
#21565=CARTESIAN_POINT ( 'NONE',  ( 203.4569662549483837, 278.2491926230401305, -15.13189527399345913 ) ) ;
#21567=CARTESIAN_POINT ( 'NONE',  ( 164.8513470711439197, 274.0536041136784888, 15.36431698690459058 ) ) ;
#21568=CARTESIAN_POINT ( 'NONE',  ( -0.3657822996961275219, 170.5958772461660544, -9.188101187500095079 ) ) ;
#21570=CARTESIAN_POINT ( 'NONE',  ( 163.5322132292002095, 248.5708327738595926, 9.747496234835503870 ) ) ;
#21571=ORIENTED_EDGE ( 'NONE', *, *, #56679, .T. ) ;
#21574=CARTESIAN_POINT ( 'NONE',  ( 195.6664450926536460, 278.3245960621525796, 17.18455885460583232 ) ) ;
#21575=CARTESIAN_POINT ( 'NONE',  ( 171.9934119896647644, 289.4116381468080021, 2.632332000678004658 ) ) ;
#21577=CARTESIAN_POINT ( 'NONE',  ( 201.9489429292733291, 280.8611656421081193, -16.76649152307749091 ) ) ;
#21579=CARTESIAN_POINT ( 'NONE',  ( 153.3817192398776683, 279.2928347461563590, 3.875170408332509808 ) ) ;
#21580=CARTESIAN_POINT ( 'NONE',  ( 22.80074434730262567, 171.7202760586659736, -5.415160957724236172E-17 ) ) ;
#21581=CARTESIAN_POINT ( 'NONE',  ( 119.1457234225564008, 239.5958772461660544, -9.188101187500095079 ) ) ;
#21587=CARTESIAN_POINT ( 'NONE',  ( 176.9878821292914211, 283.3466992399841615, -15.40003107629192769 ) ) ;
#21589=FACE_OUTER_BOUND ( 'NONE', #85651, .T. ) ;
#21590=CARTESIAN_POINT ( 'NONE',  ( 184.0471386986133098, 274.9938889884007267, 16.36334711905761097 ) ) ;
#21594=CARTESIAN_POINT ( 'NONE',  ( 192.9213923665448931, 265.3941825485875370, 7.787462690985773150 ) ) ;
#21596=CARTESIAN_POINT ( 'NONE',  ( 55.08690683815022027, 192.6115022471902023, -5.000000000000041744 ) ) ;
#21597=CARTESIAN_POINT ( 'NONE',  ( 182.3156994963505042, 267.7668330571380011, -14.83048941619937011 ) ) ;
#21599=ADVANCED_FACE ( 'NONE', ( #62649 ), #23761, .F. ) ;
#21600=CARTESIAN_POINT ( 'NONE',  ( 185.1025075027767457, 269.5733332805129976, 15.84353680425453703 ) ) ;
#21603=CARTESIAN_POINT ( 'NONE',  ( 103.7198194655286017, 224.5643266524159856, -9.188101187500093303 ) ) ;
#21604=CARTESIAN_POINT ( 'NONE',  ( 161.8408514536557163, 250.3304178724980318, -14.12919723462510646 ) ) ;
#21605=CARTESIAN_POINT ( 'NONE',  ( 151.0715479399129606, 268.9833987204304435, 14.24612252017116987 ) ) ;
#21607=CARTESIAN_POINT ( 'NONE',  ( 196.2255671652529259, 290.7743432561995860, 16.01325193769018185 ) ) ;
#21608=CARTESIAN_POINT ( 'NONE',  ( 200.4562370433687875, 283.4466080772515966, 17.70760574868393533 ) ) ;
#21609=CARTESIAN_POINT ( 'NONE',  ( 201.4059013154023603, 270.3081817402440947, -10.22446195156602400 ) ) ;
#21613=CARTESIAN_POINT ( 'NONE',  ( 192.8607783413999073, 296.6023284558532396, -11.80574095728561446 ) ) ;
#21618=CARTESIAN_POINT ( 'NONE',  ( 193.1444937042664094, 296.1109190324805240, -12.15243020627156767 ) ) ;
#21619=CARTESIAN_POINT ( 'NONE',  ( 196.8104339078508076, 289.7613243423628546, -16.40335862274955403 ) ) ;
#21622=CARTESIAN_POINT ( 'NONE',  ( 198.3523905153085423, 287.0905771551796306, 18.52598547438866206 ) ) ;
#21623=CARTESIAN_POINT ( 'NONE',  ( 156.3558586708529106, 268.1492557597510427, 15.72842580066797780 ) ) ;
#21625=CARTESIAN_POINT ( 'NONE',  ( 134.4004000680749300, 261.7365022471904012, 2.944929066748280225E-16 ) ) ;
#21628=ORIENTED_EDGE ( 'NONE', *, *, #14654, .F. ) ;
#21632=CARTESIAN_POINT ( 'NONE',  ( 185.0948665225164120, 293.0251998113765808, -10.41559016972385798 ) ) ;
#21636=CARTESIAN_POINT ( 'NONE',  ( 190.7742855516683278, 278.1955315082693687, -16.74573926298076998 ) ) ;
#21637=CARTESIAN_POINT ( 'NONE',  ( 153.7958926348061368, 264.2646952915446263, -18.09980811596817318 ) ) ;
#21638=CARTESIAN_POINT ( 'NONE',  ( 152.7729059155601021, 266.0365602647466972, -17.50667083025758686 ) ) ;
#21643=CARTESIAN_POINT ( 'NONE',  ( 189.5078380459772802, 300.6522465952268135, 0.4004850747286866630 ) ) ;
#21645=AXIS2_PLACEMENT_3D ( 'NONE', #14163, #6059, #21272 ) ;
#21646=ORIENTED_EDGE ( 'NONE', *, *, #75470, .T. ) ;
#21647=CARTESIAN_POINT ( 'NONE',  ( 157.7847820078105201, 257.3557362317297361, -18.02899742403477035 ) ) ;
#21648=CARTESIAN_POINT ( 'NONE',  ( 182.5291792280718823, 296.7636338796572204, 0.3805386115670883473 ) ) ;
#21649=CARTESIAN_POINT ( 'NONE',  ( 164.4294002498235159, 245.8469198396639399, 6.098783631055905374 ) ) ;
#21650=CARTESIAN_POINT ( 'NONE',  ( 165.9477391530904242, 274.0934507990922384, -15.17489481902206272 ) ) ;
#21651=CARTESIAN_POINT ( 'NONE',  ( 206.6395994010593427, 272.7367103121227387, -10.00948282007047219 ) ) ;
#21652=CARTESIAN_POINT ( 'NONE',  ( 201.1327128468116143, 274.8997197801397192, -13.94580791315554613 ) ) ;
#21654=CARTESIAN_POINT ( 'NONE',  ( 147.8465295590381743, 274.5692944114487091, 9.322947948439978205 ) ) ;
#21655=CARTESIAN_POINT ( 'NONE',  ( 170.3109497006183801, 287.3311160575474332, -4.623670106724921069 ) ) ;
#21657=AXIS2_PLACEMENT_3D ( 'NONE', #45413, #91556, #54492 ) ;
#21658=CARTESIAN_POINT ( 'NONE',  ( 186.3952907517880817, 286.6368042130659433, -15.42260794059327900 ) ) ;
#21659=CARTESIAN_POINT ( 'NONE',  ( 115.6001716039901055, 246.7369531367911009, -4.594050593750048428 ) ) ;
#21661=CARTESIAN_POINT ( 'NONE',  ( 183.9106092447611900, 260.0878217146031375, -9.644928028340759241 ) ) ;
#21662=B_SPLINE_CURVE_WITH_KNOTS ( 'NONE', 3,
 ( #77756, #54408, #69129, #99552 ),
 .UNSPECIFIED., .F., .F.,
 ( 4, 4 ),
 ( 0.003612368519395985772, 0.01157920093718791538 ),
 .UNSPECIFIED. ) ;
#21664=CARTESIAN_POINT ( 'NONE',  ( 191.1174571109413591, 274.9979070728601869, 15.98165944953893991 ) ) ;
#21666=ORIENTED_EDGE ( 'NONE', *, *, #87917, .F. ) ;
#21668=CARTESIAN_POINT ( 'NONE',  ( 164.5824376406421266, 246.2431216187744667, -2.547103021557204805 ) ) ;
#21669=CARTESIAN_POINT ( 'NONE',  ( 157.0935036675524827, 258.5530654392286465, 17.32636058289560665 ) ) ;
#21671=CYLINDRICAL_SURFACE ( 'NONE', #90081, 17.82106496071139645 ) ;
#21673=CARTESIAN_POINT ( 'NONE',  ( 148.6214941521368758, 273.2270163621349752, 10.16346731517885082 ) ) ;
#21677=EDGE_CURVE ( 'NONE', #66481, #68024, #64240, .T. ) ;
#21679=CARTESIAN_POINT ( 'NONE',  ( 193.7609008727193043, 262.8443104439116951, 4.759103018491034121 ) ) ;
#21680=CARTESIAN_POINT ( 'NONE',  ( 158.3972311956721342, 263.3721427664003727, 17.45954809345846215 ) ) ;
#21684=CARTESIAN_POINT ( 'NONE',  ( 201.4520623681621316, 281.7217880192456505, -17.56577389517433119 ) ) ;
#21685=ORIENTED_EDGE ( 'NONE', *, *, #54704, .T. ) ;
#21689=CARTESIAN_POINT ( 'NONE',  ( 170.0607343483624447, 248.7358776599870964, -0.2674079240231920784 ) ) ;
#21690=CARTESIAN_POINT ( 'NONE',  ( 189.0380684747346152, 269.9222665765973943, -14.01655753500979351 ) ) ;
#21694=CARTESIAN_POINT ( 'NONE',  ( 191.1921138502980568, 283.4129728893950073, -16.58386050240950027 ) ) ;
#21696=CARTESIAN_POINT ( 'NONE',  ( 67.34640541081718368, 215.8149278399160949, -9.188101187500095079 ) ) ;
#21697=CARTESIAN_POINT ( 'NONE',  ( 159.5050723400634638, 254.3761059724978679, -15.34938048045353298 ) ) ;
#21700=CARTESIAN_POINT ( 'NONE',  ( 207.2683629543511756, 271.6476598918739001, -6.694388351944108528 ) ) ;
#21702=CARTESIAN_POINT ( 'NONE',  ( 108.6384560342674064, 221.9824982072974251, 3.021315404115420679E-15 ) ) ;
#21712=CARTESIAN_POINT ( 'NONE',  ( 199.3058668659812724, 277.8561274100368905, 16.30908028197919535 ) ) ;
#21713=CARTESIAN_POINT ( 'NONE',  ( 147.8505793332463725, 274.5622799967613332, -9.317516487097901035 ) ) ;
#21715=CARTESIAN_POINT ( 'NONE',  ( 46.23738328933649200, 191.3768266524159856, -9.188101187500093303 ) ) ;
#21717=CARTESIAN_POINT ( 'NONE',  ( 151.4188942279983223, 268.3817773016460251, -14.77302265413830895 ) ) ;
#21718=CARTESIAN_POINT ( 'NONE',  ( 149.3629284598386278, 271.9428144707212027, -12.99253781774931049 ) ) ;
#21720=CARTESIAN_POINT ( 'NONE',  ( 157.3029956111992362, 258.1902147490555421, -18.22269824972649843 ) ) ;
#21722=CARTESIAN_POINT ( 'NONE',  ( 175.6422712798515420, 291.0239839832145208, 2.433063146221782436 ) ) ;
#21723=CARTESIAN_POINT ( 'NONE',  ( 179.9202220416364355, 276.5770508256506446, 16.41260542237966646 ) ) ;
#21725=CARTESIAN_POINT ( 'NONE',  ( 149.1653648461108617, 275.5304674000249179, 7.618651205328232479 ) ) ;
#21726=CARTESIAN_POINT ( 'NONE',  ( 163.2804934380540658, 256.0196637926906078, -14.90650773794625472 ) ) ;
#21729=CARTESIAN_POINT ( 'NONE',  ( 97.16130770534417138, 220.2365022471902023, 10.00000000000009592 ) ) ;
#21730=CARTESIAN_POINT ( 'NONE',  ( 161.2799361541916028, 251.3019516699124836, 14.40628917569557110 ) ) ;
#21732=ORIENTED_EDGE ( 'NONE', *, *, #82817, .T. ) ;
#21733=CARTESIAN_POINT ( 'NONE',  ( 58.87550765610937731, 213.9869531367911009, 4.594050593750046652 ) ) ;
#21735=CARTESIAN_POINT ( 'NONE',  ( 184.1612352507079322, 265.5980064862902168, 14.76078110080899641 ) ) ;
#21736=CARTESIAN_POINT ( 'NONE',  ( 161.6369034275210481, 251.0970872729290591, 12.75120819296054009 ) ) ;
#21740=CARTESIAN_POINT ( 'NONE',  ( 207.6860335175200589, 270.9242332556395922, 6.913225035677485586 ) ) ;
#21742=DIRECTION ( 'NONE',  ( -0.8660254037844387076, -0.4999999999999998890, -0.000000000000000000 ) ) ;
#21743=CARTESIAN_POINT ( 'NONE',  ( 206.8776226275057297, 271.8386879954387609, -6.083657955821966112 ) ) ;
#21744=CARTESIAN_POINT ( 'NONE',  ( 157.4243923570103050, 257.9799494174374104, 18.06359219958597606 ) ) ;
#21745=EDGE_LOOP ( 'NONE', ( #72301, #4485, #72292 ) ) ;
#21756=CARTESIAN_POINT ( 'NONE',  ( 162.6341128535665064, 248.9564488241690299, -10.63508949045170660 ) ) ;
#21757=CARTESIAN_POINT ( 'NONE',  ( 204.5730103890532519, 276.3161474792809145, 14.88139715235883109 ) ) ;
#21758=CARTESIAN_POINT ( 'NONE',  ( 188.5952966566430860, 295.4055683097271867, -11.38938388239568056 ) ) ;
#21760=CARTESIAN_POINT ( 'NONE',  ( 164.3743206631776275, 265.6518399700423174, -16.94241144619603290 ) ) ;
#21761=CARTESIAN_POINT ( 'NONE',  ( 128.2929432021470575, 251.0024278399160949, 9.188101187500095079 ) ) ;
#21762=CARTESIAN_POINT ( 'NONE',  ( 160.0364848823596731, 255.1851680591929892, -16.26533138570701809 ) ) ;
#21763=CARTESIAN_POINT ( 'NONE',  ( 83.72013207082297015, 209.9548013555409796, -4.594050593750042211 ) ) ;
#21764=VERTEX_POINT ( 'NONE', #20084 ) ;
#21765=CARTESIAN_POINT ( 'NONE',  ( 171.9709265855787521, 264.6047551489337479, 15.86023412204940897 ) ) ;
#21766=CARTESIAN_POINT ( 'NONE',  ( 204.6282099259498182, 271.7394219149207970, 9.770859781323483872 ) ) ;
#21768=VERTEX_POINT ( 'NONE', #93868 ) ;
#21769=CARTESIAN_POINT ( 'NONE',  ( 160.7611904649662051, 253.0402142913282830, 14.60361351347018477 ) ) ;
#21770=ORIENTED_EDGE ( 'NONE', *, *, #47859, .T. ) ;
#21774=CARTESIAN_POINT ( 'NONE',  ( 194.3094773688834778, 284.8302703302293253, 17.74979085435418469 ) ) ;
#21775=CARTESIAN_POINT ( 'NONE',  ( 191.7741832257749195, 298.4843664033717801, -8.615487418695501276 ) ) ;
#21778=CARTESIAN_POINT ( 'NONE',  ( 194.4459411895494725, 293.8567458645873103, 14.31012567920753042 ) ) ;
#21780=CARTESIAN_POINT ( 'NONE',  ( 182.0092902691650920, 257.1508607890800135, -6.141684172092635841 ) ) ;
#21783=EDGE_CURVE ( 'NONE', #38435, #91209, #36404, .T. ) ;
#21784=B_SPLINE_SURFACE_WITH_KNOTS ( 'NONE', 3, 1, ( 
 ( #78722, #69603 ),
 ( #55874, #9311 ),
 ( #40184, #1728 ),
 ( #78221, #93446 ),
 ( #16403, #92449 ),
 ( #84846, #22995 ),
 ( #54897, #15384 ),
 ( #100028, #23998 ),
 ( #46281, #53886 ),
 ( #77209, #32607 ),
 ( #70601, #63004 ),
 ( #47296, #1214 ),
 ( #62481, #207 ),
 ( #86870, #8312 ),
 ( #8805, #63504 ),
 ( #7812, #94442 ),
 ( #38697, #93949 ),
 ( #54376, #24503 ),
 ( #61980, #55382 ),
 ( #23487, #9829 ),
 ( #17403, #86366 ),
 ( #85351, #24997 ),
 ( #15898, #46805 ),
 ( #77727, #39177 ),
 ( #16896, #48313 ),
 ( #79258, #30614 ),
 ( #40690, #61499 ),
 ( #2729, #87394 ),
 ( #51161, #4576 ),
 ( #97306, #27383 ),
 ( #82125, #25509 ),
 ( #67361, #51681 ),
 ( #59240, #66864 ),
 ( #56399, #12697 ) ),
 .UNSPECIFIED., .T., .F., .F.,
 ( 4, 2, 2, 2, 2, 2, 2, 2, 2, 2, 2, 2, 2, 2, 2, 2, 4 ),
 ( 2, 2 ),
 ( 0.000000000000000000, 0.06250000000000000000, 0.1250000000000000000, 0.1875000000000000000, 0.2500000000000000000, 0.3125000000000000000, 0.3750000000000000000, 0.4375000000000000000, 0.5000000000000000000, 0.5625000000000000000, 0.6250000000000000000, 0.6875000000000000000, 0.7500000000000000000, 0.8125000000000000000, 0.8750000000000000000, 0.9375000000000000000, 1.000000000000000000 ),
 ( 0.000000000000000000, 1.000000000000000000 ),
 .UNSPECIFIED. ) ;
#21785=CARTESIAN_POINT ( 'NONE',  ( 186.5210254826074276, 287.5177492320627266, 16.01978303813461935 ) ) ;
#21786=ORIENTED_EDGE ( 'NONE', *, *, #88875, .F. ) ;
#21788=CARTESIAN_POINT ( 'NONE',  ( 163.9470117944672438, 260.6273701597328341, -16.21158959658340493 ) ) ;
#21789=CARTESIAN_POINT ( 'NONE',  ( 164.5451017335383597, 246.7547400039435956, 5.445355051732909679 ) ) ;
#21791=CARTESIAN_POINT ( 'NONE',  ( 185.1394335896403902, 275.7790610180006752, 16.42070492368160117 ) ) ;
#21792=CARTESIAN_POINT ( 'NONE',  ( 164.8616299252405213, 245.0982760813026857, 1.544363874765093625 ) ) ;
#21794=CARTESIAN_POINT ( 'NONE',  ( 195.2502824789841895, 279.2012642199275660, 16.31828257502794699 ) ) ;
#21795=CARTESIAN_POINT ( 'NONE',  ( 162.9177813375093820, 261.5106994340935671, 17.39058219678560135 ) ) ;
#21796=CARTESIAN_POINT ( 'NONE',  ( 135.0589402170954827, 248.7833772461660544, -9.188101187500095079 ) ) ;
#21805=CARTESIAN_POINT ( 'NONE',  ( 148.0770056944566022, 275.8785175959847038, -3.807152131487734348 ) ) ;
#21806=B_SPLINE_CURVE_WITH_KNOTS ( 'NONE', 3,
 ( #69417, #29, #30914, #86179, #23806, #24808, #10122, #16713, #62294, #47606, #87194, #40987, #16216, #78534, #2022, #56198, #94748, #32418, #9119, #39991, #33417, #54695, #95274, #71931, #17727, #85157, #1536, #64316, #63313, #48110, #85679, #520, #79052, #9641, #40500, #71432, #32907, #48629, #46603, #79564, #39000, #2535, #93251, #47108, #70413, #1021, #86070, #32792, #38890, #18106 ),
 .UNSPECIFIED., .F., .F.,
 ( 4, 2, 2, 2, 2, 2, 2, 2, 2, 2, 2, 2, 2, 2, 2, 2, 2, 2, 2, 2, 2, 2, 2, 2, 4 ),
 ( 0.0007103610476057106715, 0.001202613152260477609, 0.001694865256915244331, 0.001940991309242592021, 0.002187117361569939494, 0.002310180387733583741, 0.002433243413897227987, 0.002556306440060872667, 0.002679369466224516480, 0.002925495518551847040, 0.003171621570879177600, 0.003663873675533679125, 0.004648377884842772381, 0.005632882094151865637, 0.006125134198806411398, 0.006617386303460958026, 0.006740449329624556736, 0.006801980842706337009, 0.006863512355788118149, 0.006986575381951677828, 0.007109638408115237507, 0.007355764460442497377, 0.007601890512769757247, 0.008094142617424250966, 0.008586394722078742950 ),
 .UNSPECIFIED. ) ;
#21809=CARTESIAN_POINT ( 'NONE',  ( 199.1113007661987240, 266.5577079162528094, 0.8260111218802939081 ) ) ;
#21810=CARTESIAN_POINT ( 'NONE',  ( 197.6828869641981612, 265.7779761413833626, 0.8200578392135022820 ) ) ;
#21811=CARTESIAN_POINT ( 'NONE',  ( 147.0538900202505488, 275.9421863647172017, 5.192507380313251986 ) ) ;
#21812=CARTESIAN_POINT ( 'NONE',  ( 185.0761968336884138, 281.7485531843886406, 16.20522637585934689 ) ) ;
#21814=CARTESIAN_POINT ( 'NONE',  ( 164.5416088356626290, 245.6525688679454618, -1.463507744092769292 ) ) ;
#21815=CARTESIAN_POINT ( 'NONE',  ( 196.8474129767564875, 269.8048104555306281, 12.12537726023140117 ) ) ;
#21820=CARTESIAN_POINT ( 'NONE',  ( 205.1385161361615701, 274.5423688205104895, 11.59183615411821933 ) ) ;
#21822=CARTESIAN_POINT ( 'NONE',  ( 198.6012358295098750, 286.6595644277572887, 18.21911298807435386 ) ) ;
#21824=CARTESIAN_POINT ( 'NONE',  ( -5.778093977583854013, 155.2202760586659451, -5.415160957724236172E-17 ) ) ;
#21825=CARTESIAN_POINT ( 'NONE',  ( 172.5963845202620064, 283.7040405909344827, -12.35744486217303084 ) ) ;
#21830=CARTESIAN_POINT ( 'NONE',  ( 202.5011135140420606, 274.1303848594789088, -12.97262903380130261 ) ) ;
#21831=CARTESIAN_POINT ( 'NONE',  ( 198.4344074287054696, 286.9485196940960918, -17.83642855442570152 ) ) ;
#21832=CARTESIAN_POINT ( 'NONE',  ( 7.428446334363822956, 175.0958772461660544, -9.188101187500095079 ) ) ;
#21833=CARTESIAN_POINT ( 'NONE',  ( 180.7163234865986681, 274.9646179361455438, -16.46674387372169690 ) ) ;
#21836=CARTESIAN_POINT ( 'NONE',  ( 170.6324991628954990, 271.0675588811652119, -17.59648249145834953 ) ) ;
#21838=CARTESIAN_POINT ( 'NONE',  ( 150.1550056273443943, 276.5028295449805000, 3.910624302002001063 ) ) ;
#21839=EDGE_CURVE ( 'NONE', #76328, #38319, #38692, .T. ) ;
#21840=EDGE_CURVE ( 'NONE', #12202, #947, #39938, .T. ) ;
#21841=CARTESIAN_POINT ( 'NONE',  ( 175.7921476968669197, 253.7367219729100327, -3.864758291546732671 ) ) ;
#21842=CARTESIAN_POINT ( 'NONE',  ( 150.9195128607351251, 269.2467312020988857, 13.93698123781031484 ) ) ;
#21844=CARTESIAN_POINT ( 'NONE',  ( 46.06580888206220692, 210.7365022471903444, 2.944929066748280225E-16 ) ) ;
#21846=CARTESIAN_POINT ( 'NONE',  ( 190.5674408456512765, 300.5745055173924811, -0.9151048603553563199 ) ) ;
#21847=CARTESIAN_POINT ( 'NONE',  ( 20.93329029645117245, 173.7048013555409796, 4.594050593750051981 ) ) ;
#21848=CARTESIAN_POINT ( 'NONE',  ( 164.5737363065680370, 285.5024452864429918, 4.376381487704442463 ) ) ;
#21849=CARTESIAN_POINT ( 'NONE',  ( 153.3616370783189211, 265.0168479788495688, 17.48287904751960653 ) ) ;
#21851=CARTESIAN_POINT ( 'NONE',  ( 202.0661878422603763, 279.1895584290143120, -16.02388874507808225 ) ) ;
#21853=CARTESIAN_POINT ( 'NONE',  ( 206.8968397926183229, 272.2911568841838061, 7.145103750817420440 ) ) ;
#21854=CARTESIAN_POINT ( 'NONE',  ( 185.4724734968301618, 266.2864717598490643, 14.59729369397538612 ) ) ;
#21855=CARTESIAN_POINT ( 'NONE',  ( 201.5189872289815867, 266.7509884862435570, -2.318412474989284267 ) ) ;
#21856=CARTESIAN_POINT ( 'NONE',  ( 164.1744119160098023, 281.5290954411402709, 9.010387237428474805 ) ) ;
#21858=CARTESIAN_POINT ( 'NONE',  ( 190.5893431400089923, 300.5365696307625853, -0.3099240395267599535 ) ) ;
#21860=CARTESIAN_POINT ( 'NONE',  ( 201.1389011169710272, 268.2808080133845010, 7.540724018285327013 ) ) ;
#21869=CARTESIAN_POINT ( 'NONE',  ( 155.0619429961492983, 262.0718317407570339, -17.08853361476647592 ) ) ;
#21870=EDGE_LOOP ( 'NONE', ( #5628, #13645, #44353, #86256 ) ) ;
#21871=CARTESIAN_POINT ( 'NONE',  ( 186.2429809382703354, 271.9601928012535268, -16.35413080596582347 ) ) ;
#21872=CARTESIAN_POINT ( 'NONE',  ( 164.1259971043086239, 246.3724295028720519, 5.761669507629934905 ) ) ;
#21873=VERTEX_POINT ( 'NONE', #65420 ) ;
#21874=CARTESIAN_POINT ( 'NONE',  ( 201.3505934466285510, 281.8975373467312693, -16.83770227898004279 ) ) ;
#21882=VERTEX_POINT ( 'NONE', #13237 ) ;
#21883=CARTESIAN_POINT ( 'NONE',  ( 206.4695239676918845, 273.0312896038346366, 10.41704154450801667 ) ) ;
#21886=CARTESIAN_POINT ( 'NONE',  ( 149.3883679478359454, 271.8987519849911223, 12.99187507659642371 ) ) ;
#21887=CARTESIAN_POINT ( 'NONE',  ( 193.2902653713029508, 264.7699875813403310, -9.193237569391540021 ) ) ;
#21891=CARTESIAN_POINT ( 'NONE',  ( 149.0243928082760192, 274.5278390230128025, 9.115363623326919296 ) ) ;
#21898=CARTESIAN_POINT ( 'NONE',  ( 148.0427192501136062, 274.2294838985851015, 9.385226820296049155 ) ) ;
#21899=CARTESIAN_POINT ( 'NONE',  ( 149.6071296322179194, 271.5198456328920997, 12.75640156477042453 ) ) ;
#21900=CARTESIAN_POINT ( 'NONE',  ( 152.8134625983922490, 265.9663140294953791, 17.57333028169644251 ) ) ;
#21902=CARTESIAN_POINT ( 'NONE',  ( 146.5443760852173227, 276.8246903873589986, -0.3422986961735821065 ) ) ;
#21903=CARTESIAN_POINT ( 'NONE',  ( 191.0862225170008628, 299.6759493045793192, -9.402218231374108726 ) ) ;
#21906=CARTESIAN_POINT ( 'NONE',  ( 149.6890529486499872, 271.3779502865075983, -12.51465682618088593 ) ) ;
#21907=DIRECTION ( 'NONE',  ( 0.4999999999999992784, -0.8660254037844390407, 0.000000000000000000 ) ) ;
#21909=CARTESIAN_POINT ( 'NONE',  ( 168.2861312974920338, 286.3523900831025344, 3.986708875144260311 ) ) ;
#21911=CARTESIAN_POINT ( 'NONE',  ( 101.2839494695023603, 229.2833772461660544, -9.188101187500095079 ) ) ;
#21912=ORIENTED_EDGE ( 'NONE', *, *, #97112, .T. ) ;
#21913=DIRECTION ( 'NONE',  ( 0.4999999999999998890, -0.8660254037844385966, 0.000000000000000000 ) ) ;
#21915=CARTESIAN_POINT ( 'NONE',  ( 148.7795025377680815, 273.5541084840127724, 8.957187006633716919 ) ) ;
#21916=EDGE_CURVE ( 'NONE', #24285, #94448, #97346, .T. ) ;
#21918=EDGE_CURVE ( 'NONE', #89828, #2810, #30266, .T. ) ;
#21919=LINE ( 'NONE', #60900, #43428 ) ;
#21920=CARTESIAN_POINT ( 'NONE',  ( 193.0622221429366050, 289.4054684591471300, 16.71589558189321778 ) ) ;
#21921=CARTESIAN_POINT ( 'NONE',  ( 168.0580858286423052, 284.4539385443458741, -7.981534432883824692 ) ) ;
#21923=CARTESIAN_POINT ( 'NONE',  ( 170.6462599113855561, 255.5044248170252388, -12.77826996180470864 ) ) ;
#21924=CARTESIAN_POINT ( 'NONE',  ( -22.42236680055709641, 157.8615022471902591, 0.000000000000000000 ) ) ;
#21926=CARTESIAN_POINT ( 'NONE',  ( 44.46005344233076784, 183.1427522451417360, 1.119607411625061291E-15 ) ) ;
#21927=CARTESIAN_POINT ( 'NONE',  ( 122.2582625392304863, 232.2048013555409796, 4.594050593750051981 ) ) ;
#21928=CARTESIAN_POINT ( 'NONE',  ( 198.8157103782086210, 286.2880836124806478, -18.60729372713428020 ) ) ;
#21930=CARTESIAN_POINT ( 'NONE',  ( 104.9037214839949002, 219.8262482093457777, 3.021315404115420679E-15 ) ) ;
#21931=CARTESIAN_POINT ( 'NONE',  ( 174.4680951374541849, 252.9015896160454702, -3.884363688654588476 ) ) ;
#21932=CARTESIAN_POINT ( 'NONE',  ( 29.86365662933068066, 197.2369531367911293, -4.594050593750048428 ) ) ;
#21935=ORIENTED_EDGE ( 'NONE', *, *, #26555, .T. ) ;
#21936=CARTESIAN_POINT ( 'NONE',  ( 188.4805308512120234, 298.0761574053781828, 7.892637567094712203 ) ) ;
#21937=CARTESIAN_POINT ( 'NONE',  ( 179.2182182526515248, 265.9655207074544592, 16.25122323871343610 ) ) ;
#21940=CARTESIAN_POINT ( 'NONE',  ( 190.8957779480239765, 300.0058089740729770, -4.541438514207768229 ) ) ;
#21943=CARTESIAN_POINT ( 'NONE',  ( 164.2897805489690768, 249.8104079013010335, 11.36607573508163505 ) ) ;
#21945=CARTESIAN_POINT ( 'NONE',  ( 99.01965388075031171, 234.6427522451419065, -10.00000000000009415 ) ) ;
#21946=ORIENTED_EDGE ( 'NONE', *, *, #9052, .F. ) ;
#21949=CARTESIAN_POINT ( 'NONE',  ( 202.8499463704053198, 279.3005819042728604, 17.04674939340617001 ) ) ;
#21950=CARTESIAN_POINT ( 'NONE',  ( 163.2000388741132895, 247.9762362032568035, -11.19676374274550312 ) ) ;
#21952=EDGE_CURVE ( 'NONE', #59274, #80346, #73700, .T. ) ;
#21953=CARTESIAN_POINT ( 'NONE',  ( 13.97758990260114231, 185.0024278399160949, 9.188101187500095079 ) ) ;
#21958=EDGE_CURVE ( 'NONE', #93932, #43017, #49298, .T. ) ;
#21959=CARTESIAN_POINT ( 'NONE',  ( 174.0404940119542232, 287.4816634783161930, 10.83703146888826119 ) ) ;
#21960=CARTESIAN_POINT ( 'NONE',  ( 59.20026718252854891, 214.1744531367911293, 4.594050593750047540 ) ) ;
#21961=CARTESIAN_POINT ( 'NONE',  ( 207.5583741822599393, 271.1453457103705205, 3.140867606700001424 ) ) ;
#21967=CARTESIAN_POINT ( 'NONE',  ( 11.35262394703597977, 187.3615022471903160, 5.000000000000046185 ) ) ;
#21968=CARTESIAN_POINT ( 'NONE',  ( 163.7595992360150490, 247.0070492265414828, -6.976205010573520049 ) ) ;
#21969=CARTESIAN_POINT ( 'NONE',  ( 143.3676317564762144, 244.3923013555409511, 4.594050593750050204 ) ) ;
#21971=CARTESIAN_POINT ( 'NONE',  ( 207.2934053853322780, 271.6042851290696376, -8.345259833563044793 ) ) ;
#21973=CARTESIAN_POINT ( 'NONE',  ( 177.0253895856008057, 252.4355161662766420, -0.1804300260461335903 ) ) ;
#21976=CARTESIAN_POINT ( 'NONE',  ( 166.8083734521890449, 257.5796782931630560, -15.79284703031436798 ) ) ;
#21979=CARTESIAN_POINT ( 'NONE',  ( 151.9862327556172943, 268.5453780521097542, -15.09052660903973120 ) ) ;
#21980=CARTESIAN_POINT ( 'NONE',  ( 156.4002494452255689, 280.4459135353391730, -5.478302318053954956 ) ) ;
#21981=CARTESIAN_POINT ( 'NONE',  ( 195.9583358019009722, 272.3999277485804669, -13.38286462214372108 ) ) ;
#21982=ORIENTED_EDGE ( 'NONE', *, *, #76769, .F. ) ;
#21983=CARTESIAN_POINT ( 'NONE',  ( 160.1500473090515584, 253.2589765566000608, 16.19674609738075333 ) ) ;
#21984=CARTESIAN_POINT ( 'NONE',  ( 171.3259067627017487, 284.4620142900025712, -11.36310073225868500 ) ) ;
#21990=CARTESIAN_POINT ( 'NONE',  ( 149.7799119457360177, 272.8289483412673917, 11.37468589474485903 ) ) ;
#21991=CARTESIAN_POINT ( 'NONE',  ( 137.7719789713245291, 261.8967562850346553, -4.648177544792955347E-16 ) ) ;
#21992=CARTESIAN_POINT ( 'NONE',  ( 201.1060504099706350, 282.3210983108598384, -18.18000168485860257 ) ) ;
#21993=CARTESIAN_POINT ( 'NONE',  ( 97.10949284993499475, 215.3262482093457493, 3.021315404115420679E-15 ) ) ;
#21995=CARTESIAN_POINT ( 'NONE',  ( 191.9204824329850396, 287.7260408795398234, -15.99984276108531311 ) ) ;
#21997=CARTESIAN_POINT ( 'NONE',  ( 148.9517569034208009, 272.6549844970639924, 12.50737104496728236 ) ) ;
#21998=DIRECTION ( 'NONE',  ( 0.4999999999999998890, -0.8660254037844385966, 0.000000000000000000 ) ) ;
#22000=EDGE_CURVE ( 'NONE', #5671, #32845, #46391, .T. ) ;
#22002=CARTESIAN_POINT ( 'NONE',  ( 191.0862225170008628, 299.6759493045793192, -9.402218231374108726 ) ) ;
#22003=CARTESIAN_POINT ( 'NONE',  ( 183.8973593476267752, 262.2032069668072722, -12.40570899861645771 ) ) ;
#22004=CARTESIAN_POINT ( 'NONE',  ( 163.8003088823192286, 260.8948240748503054, -17.39314492925268141 ) ) ;
#22007=CARTESIAN_POINT ( 'NONE',  ( 99.71410487726059557, 234.5024278399160949, 9.188101187500095079 ) ) ;
#22008=CARTESIAN_POINT ( 'NONE',  ( 203.0794350760556028, 278.9030958063233925, 15.06053680683988638 ) ) ;
#22010=CARTESIAN_POINT ( 'NONE',  ( 179.8103815483993344, 270.2768680805289705, -16.04546734559231780 ) ) ;
#22014=VERTEX_POINT ( 'NONE', #61790 ) ;
#22015=DIRECTION ( 'NONE',  ( 0.4999999999999998890, -0.8660254037844385966, 0.000000000000000000 ) ) ;
#22024=ORIENTED_EDGE ( 'NONE', *, *, #5473, .F. ) ;
#22029=CARTESIAN_POINT ( 'NONE',  ( 9.120852146362338431, 187.6199935810941213, 2.679491924311251605 ) ) ;
#22033=CARTESIAN_POINT ( 'NONE',  ( 200.0411626275569574, 270.6720010161316736, -11.59284015024147152 ) ) ;
#22035=CARTESIAN_POINT ( 'NONE',  ( 161.3440642087019796, 281.4507293028746062, -6.554503167351243498 ) ) ;
#22039=CARTESIAN_POINT ( 'NONE',  ( 192.6527964471240750, 292.3325994180497105, -14.38016747683365359 ) ) ;
#22041=CARTESIAN_POINT ( 'NONE',  ( 168.3057934360732588, 253.3915715900249097, 11.59359703697476718 ) ) ;
#22042=CARTESIAN_POINT ( 'NONE',  ( 194.2039773765081350, 263.4403579747535105, -0.7712302936324405556 ) ) ;
#22044=CARTESIAN_POINT ( 'NONE',  ( 155.6732402535458846, 261.0130338324187846, -18.36886937783899043 ) ) ;
#22046=CARTESIAN_POINT ( 'NONE',  ( 6.427104459464150210, 164.5177522451418213, 5.000000000000051514 ) ) ;
#22048=CARTESIAN_POINT ( 'NONE',  ( 172.5784562716271466, 280.0954662991010196, -14.34707186603650442 ) ) ;
#22049=CARTESIAN_POINT ( 'NONE',  ( 163.3366259987258786, 247.7396603637682801, -8.236665301808596240 ) ) ;
#22052=CARTESIAN_POINT ( 'NONE',  ( -14.30363896367569509, 171.7369531367911293, -4.594050593750048428 ) ) ;
#22054=CARTESIAN_POINT ( 'NONE',  ( 186.5421728102579948, 295.6688228412515969, 8.171192122117640011 ) ) ;
#22056=AXIS2_PLACEMENT_3D ( 'NONE', #16178, #55650, #8585 ) ;
#22061=CARTESIAN_POINT ( 'NONE',  ( 175.0451609275794453, 292.0163007842869547, 3.353226643629469539 ) ) ;
#22063=CARTESIAN_POINT ( 'NONE',  ( -22.42236680055709641, 157.8615022471902591, 0.000000000000000000 ) ) ;
#22064=CARTESIAN_POINT ( 'NONE',  ( 202.0385627042762451, 280.7059396384401566, -16.09405805615697460 ) ) ;
#22065=( BOUNDED_CURVE ( )  B_SPLINE_CURVE ( 2, ( #42228, #10357, #26056, #72165, #18966, #3271, #10858, #26556, #41733 ),
 .UNSPECIFIED., .F., .T. ) 
 B_SPLINE_CURVE_WITH_KNOTS ( ( 3, 2, 2, 2, 3 ),
 ( 0.3669354838709677491, 0.3682795698924731242, 0.3709677419354838745, 0.3736559139784946248, 0.3750000000000000000 ),
 .UNSPECIFIED. ) 
 CURVE ( )  GEOMETRIC_REPRESENTATION_ITEM ( )  RATIONAL_B_SPLINE_CURVE ( ( 0.9330127018922194093, 0.9330127018922194093, 1.000000000000000000, 0.8660254037844387076, 1.000000000000000000, 0.8660254037844387076, 1.000000000000000000, 0.9330127018922194093, 0.9330127018922194093 ) ) 
 REPRESENTATION_ITEM ( '' )  );
#22067=CARTESIAN_POINT ( 'NONE',  ( 151.5010811193459119, 277.2876517059261232, 3.696019110083865300 ) ) ;
#22070=CARTESIAN_POINT ( 'NONE',  ( 14.24839638916628459, 179.0333772461660544, 9.188101187500095079 ) ) ;
#22071=CARTESIAN_POINT ( 'NONE',  ( 112.6505328941731108, 235.8458772461660544, 9.188101187500095079 ) ) ;
#22072=CARTESIAN_POINT ( 'NONE',  ( 181.2594824857899312, 293.4632464574068536, -6.243252836990251353 ) ) ;
#22074=CARTESIAN_POINT ( 'NONE',  ( 206.1823507212516802, 271.5286882572439140, -8.119960357998227352 ) ) ;
#22079=CARTESIAN_POINT ( 'NONE',  ( 184.4178076012347276, 274.3843162572107985, 17.30722352241574313 ) ) ;
#22080=CARTESIAN_POINT ( 'NONE',  ( 190.1225270613304588, 284.8508451989043806, 16.94479376615364075 ) ) ;
#22082=CARTESIAN_POINT ( 'NONE',  ( 170.8677527226213044, 279.5558645822755466, 13.90315963116175446 ) ) ;
#22083=CARTESIAN_POINT ( 'NONE',  ( 192.5651576355940051, 265.2377806318704643, 7.853493163364257512 ) ) ;
#22085=B_SPLINE_CURVE_WITH_KNOTS ( 'NONE', 3,
 ( #57110, #51516, #45884, #60591 ),
 .UNSPECIFIED., .F., .F.,
 ( 4, 4 ),
 ( 0.008178853229217460802, 0.01408825881594157406 ),
 .UNSPECIFIED. ) ;
#22086=CARTESIAN_POINT ( 'NONE',  ( 18.26047324907200675, 192.8967562850347122, -4.648177544792955347E-16 ) ) ;
#22088=CARTESIAN_POINT ( 'NONE',  ( 92.46148921633090367, 218.0643266524160140, 9.188101187500095079 ) ) ;
#22090=CARTESIAN_POINT ( 'NONE',  ( 191.2645787786270262, 299.3670271975948367, 7.309947121636420242 ) ) ;
#22092=CARTESIAN_POINT ( 'NONE',  ( 157.3363371328520088, 258.1324655395517311, 18.24585617226787093 ) ) ;
#22093=CARTESIAN_POINT ( 'NONE',  ( 152.2297789851355105, 266.9772837032011807, 16.97658142831851080 ) ) ;
#22094=CARTESIAN_POINT ( 'NONE',  ( 149.0866298612203593, 272.4213776815879555, 12.86424381646844495 ) ) ;
#22099=CARTESIAN_POINT ( 'NONE',  ( 192.6247335881259630, 297.0111699613833594, -13.30158778996737290 ) ) ;
#22100=CARTESIAN_POINT ( 'NONE',  ( 169.5727729373952002, 284.0798650663272156, -11.84966624384599676 ) ) ;
#22105=CARTESIAN_POINT ( 'NONE',  ( 147.1034852426517148, 275.8562849197056153, -3.648177088342072327 ) ) ;
#22106=CARTESIAN_POINT ( 'NONE',  ( 149.3253462891332219, 272.0079086998416074, -12.99539319630191336 ) ) ;
#22107=B_SPLINE_CURVE_WITH_KNOTS ( 'NONE', 3,
 ( #53421, #54919, #62003, #13941 ),
 .UNSPECIFIED., .F., .F.,
 ( 4, 4 ),
 ( 0.002635550454916707128, 0.01057756139833311744 ),
 .UNSPECIFIED. ) ;
#22108=ORIENTED_EDGE ( 'NONE', *, *, #16276, .F. ) ;
#22109=B_SPLINE_SURFACE_WITH_KNOTS ( 'NONE', 3, 1, ( 
 ( #29045, #75149 ),
 ( #75637, #59915 ),
 ( #76156, #5727 ),
 ( #36615, #66535 ),
 ( #90885, #6223 ),
 ( #37608, #83261 ),
 ( #29531, #20449 ),
 ( #51319, #52811 ),
 ( #68520, #50826 ),
 ( #74158, #74662 ),
 ( #5239, #7720 ),
 ( #15299, #39595 ),
 ( #62917, #91867 ),
 ( #31014, #53799 ),
 ( #23913, #1645 ),
 ( #38098, #54813 ),
 ( #55300, #84762 ),
 ( #22424, #62401 ),
 ( #92365, #22912 ),
 ( #71042, #70010 ),
 ( #46199, #85790 ),
 ( #61904, #40101 ),
 ( #86280, #47703 ),
 ( #16322, #625 ),
 ( #99939, #131 ),
 ( #14817, #77115 ),
 ( #54296, #23407 ),
 ( #93356, #47214 ),
 ( #60904, #69009 ),
 ( #53315, #16816 ),
 ( #61411, #84271 ),
 ( #38612, #45704 ),
 ( #69516, #30522 ),
 ( #92854, #78641 ) ),
 .UNSPECIFIED., .T., .F., .F.,
 ( 4, 2, 2, 2, 2, 2, 2, 2, 2, 2, 2, 2, 2, 2, 2, 2, 4 ),
 ( 2, 2 ),
 ( 0.000000000000000000, 0.06250000000000000000, 0.1250000000000000000, 0.1875000000000000000, 0.2500000000000000000, 0.3125000000000000000, 0.3750000000000000000, 0.4375000000000000000, 0.5000000000000000000, 0.5625000000000000000, 0.6250000000000000000, 0.6875000000000000000, 0.7500000000000000000, 0.8125000000000000000, 0.8750000000000000000, 0.9375000000000000000, 1.000000000000000000 ),
 ( 0.000000000000000000, 1.000000000000000000 ),
 .UNSPECIFIED. ) ;
#22110=AXIS2_PLACEMENT_3D ( 'NONE', #45640, #82723, #91298 ) ;
#22112=CARTESIAN_POINT ( 'NONE',  ( 159.9628729326222754, 253.5831720864507588, 15.75051413866357386 ) ) ;
#22113=CARTESIAN_POINT ( 'NONE',  ( 179.8897980908058116, 262.7712755250011014, -12.78868501294826565 ) ) ;
#22114=CARTESIAN_POINT ( 'NONE',  ( 172.8210543149999978, 253.0650713199155177, -9.347212986753337560 ) ) ;
#22115=CARTESIAN_POINT ( 'NONE',  ( 174.5899361521156266, 284.9381008987350583, -13.57821407317514684 ) ) ;
#22116=B_SPLINE_CURVE_WITH_KNOTS ( 'NONE', 3,
 ( #21774, #61260, #7069, #29387, #98300, #92230, #37954, #23259, #14186, #36972, #22781, #28889, #92709, #52664, #99787, #59766, #53657, #85110, #60255, #83618, #15154, #38458, #91711, #76968, #53177, #15661, #46556, #22273, #77491, #76010, #52167, #8085, #7568, #37459, #69372, #100291, #84132, #68862, #30875, #61761 ),
 .UNSPECIFIED., .F., .F.,
 ( 4, 2, 2, 2, 2, 2, 2, 2, 2, 2, 2, 2, 2, 2, 2, 2, 2, 2, 2, 4 ),
 ( 0.003508113122471474138, 0.003679226956315371794, 0.003764783873237320406, 0.003850340790159269451, 0.004021454624003175347, 0.004192568457847080376, 0.004534796125534887833, 0.004877023793222695289, 0.006245934463974074299, 0.007614845134725453310, 0.007957072802413343166, 0.008128186636257288961, 0.008213743553179261858, 0.008299300470101233021, 0.008320689699331723643, 0.008342078928562212531, 0.008384857387023216327, 0.008470414303945223919, 0.008641528137789279002, 0.008983755805477347534 ),
 .UNSPECIFIED. ) ;
#22117=ORIENTED_EDGE ( 'NONE', *, *, #90029, .T. ) ;
#22118=CARTESIAN_POINT ( 'NONE',  ( 187.3434644620873257, 278.8535086450150402, 17.53040139197816671 ) ) ;
#22122=CARTESIAN_POINT ( 'NONE',  ( 185.3111611773075253, 292.6075343283709458, -10.66299757420777183 ) ) ;
#22123=ORIENTED_EDGE ( 'NONE', *, *, #23692, .F. ) ;
#22124=CARTESIAN_POINT ( 'NONE',  ( 39.93146227192245590, 203.8615022471903160, 5.000000000000046185 ) ) ;
#22126=CARTESIAN_POINT ( 'NONE',  ( 190.5639199208830803, 278.8100509870810129, -16.51443528190589305 ) ) ;
#22127=CARTESIAN_POINT ( 'NONE',  ( 193.0564854987053707, 296.2633537159950379, -12.03146446119285429 ) ) ;
#22128=CARTESIAN_POINT ( 'NONE',  ( 200.6737073311291795, 283.0699384897140476, -17.61533935526990291 ) ) ;
#22132=AXIS2_PLACEMENT_3D ( 'NONE', #16806, #94350, #32518 ) ;
#22135=CARTESIAN_POINT ( 'NONE',  ( 71.18054559181101126, 205.2365022471902023, 10.00000000000009948 ) ) ;
#22137=B_SPLINE_CURVE_WITH_KNOTS ( 'NONE', 3,
 ( #99156, #21168, #54014, #67241 ),
 .UNSPECIFIED., .F., .F.,
 ( 4, 4 ),
 ( 0.000000000000000000, 0.005815978540402074078 ),
 .UNSPECIFIED. ) ;
#22140=CARTESIAN_POINT ( 'NONE',  ( 204.9463377925012253, 275.6695254486514841, -14.15865086131798378 ) ) ;
#22141=CARTESIAN_POINT ( 'NONE',  ( 169.3729277929404020, 269.0884521908612328, 17.29306383018335680 ) ) ;
#22144=CARTESIAN_POINT ( 'NONE',  ( 177.3799066019990676, 269.9615352214298127, -17.60161419056240817 ) ) ;
#22145=CARTESIAN_POINT ( 'NONE',  ( 197.4575405150459915, 273.2519002803542207, -13.37676461630871216 ) ) ;
#22147=CARTESIAN_POINT ( 'NONE',  ( 147.7870527676176948, 274.6723112360602386, 9.257357958194809555 ) ) ;
#22148=CARTESIAN_POINT ( 'NONE',  ( 167.1357220015965481, 286.2500965088896692, -4.817194026439638677 ) ) ;
#22150=CARTESIAN_POINT ( 'NONE',  ( 186.5810050528308182, 287.0653887321775528, -16.02633163178817810 ) ) ;
#22151=B_SPLINE_CURVE_WITH_KNOTS ( 'NONE', 3,
 ( #90101, #96207, #10577, #28255, #89618, #41964, #20180, #4462, #34848, #65753, #34366, #50550, #88133, #3003, #72393, #11586, #81506, #73871, #96705, #80513, #11088, #18679, #4978, #51559, #66753, #58641, #72900, #20669, #27274, #35858, #35359, #82005, #3491, #66268, #41452, #73380, #58157, #51046, #42444, #59129, #89138, #12074, #3966, #65264, #33894, #57652, #64779, #42932, #19689, #26770 ),
 .UNSPECIFIED., .F., .F.,
 ( 4, 2, 2, 2, 2, 2, 2, 2, 2, 2, 2, 2, 2, 2, 2, 2, 2, 2, 2, 2, 2, 2, 2, 2, 4 ),
 ( 0.0003075647970707622828, 0.0007717470533795799809, 0.001235929309688397733, 0.001468020437842779179, 0.001584066001920029967, 0.001700111565997280971, 0.001816157130074532193, 0.001932202694151782980, 0.002164293822306383435, 0.002628476078615583043, 0.003092658334924782652, 0.004021022847543170159, 0.004949387360161558100, 0.005413569616470791969, 0.005645660744625372908, 0.005761706308702621744, 0.005877751872779870580, 0.005935774654818462906, 0.005993797436857055232, 0.006109843000934376059, 0.006341934129088985621, 0.006806116385398164846, 0.007270298641707344939, 0.007502389769861964909, 0.007734480898016584879 ),
 .UNSPECIFIED. ) ;
#22152=CARTESIAN_POINT ( 'NONE',  ( 111.8659576938172364, 226.2048013555410080, 4.594050593750051981 ) ) ;
#22153=ORIENTED_EDGE ( 'NONE', *, *, #70166, .F. ) ;
#22154=B_SPLINE_CURVE_WITH_KNOTS ( 'NONE', 3,
 ( #14698, #59278, #83138, #90255, #51722, #29408, #36497, #67400, #60277, #98325, #48087, #38980, #47088, #32887, #17185, #2001, #25288, #78513 ),
 .UNSPECIFIED., .F., .F.,
 ( 4, 2, 2, 2, 2, 2, 2, 2, 4 ),
 ( 0.0002032915482228868484, 0.0005852909360411848042, 0.0006807907829957838977, 0.0007285407064730834445, 0.0007762906299503830997, 0.0008717904769048328987, 0.0009672903238592826976, 0.001349289711677355980, 0.001731289099495429695 ),
 .UNSPECIFIED. ) ;
#22157=CARTESIAN_POINT ( 'NONE',  ( 188.1252097491235702, 273.5990210901503019, 15.73037138839605120 ) ) ;
#22158=ORIENTED_EDGE ( 'NONE', *, *, #16899, .T. ) ;
#22160=CARTESIAN_POINT ( 'NONE',  ( 180.3896065631481065, 294.7457813050739901, -1.965667979761724915 ) ) ;
#22161=CARTESIAN_POINT ( 'NONE',  ( 196.3519702320103590, 290.5554067223432639, 17.39042812051341969 ) ) ;
#22162=CARTESIAN_POINT ( 'NONE',  ( 206.0870578475358172, 273.6937403561189512, -10.07771901274806581 ) ) ;
#22164=CARTESIAN_POINT ( 'NONE',  ( 96.65612621980328356, 216.6115022471901739, -5.000000000000041744 ) ) ;
#22165=VERTEX_POINT ( 'NONE', #3524 ) ;
#22166=CARTESIAN_POINT ( 'NONE',  ( 194.7295074538898803, 293.3655946874374081, 16.09945624218667959 ) ) ;
#22170=VERTEX_POINT ( 'NONE', #25297 ) ;
#22171=CARTESIAN_POINT ( 'NONE',  ( 206.4229368915142686, 273.1119807867502800, 10.31819530520674810 ) ) ;
#22172=CARTESIAN_POINT ( 'NONE',  ( 195.7664554078432104, 265.2673286538130810, 4.151641377481578132 ) ) ;
#22176=CARTESIAN_POINT ( 'NONE',  ( -19.92236680055706444, 153.5313752282680184, 0.000000000000000000 ) ) ;
#22177=CARTESIAN_POINT ( 'NONE',  ( 157.2948870673828026, 280.9759411348209142, 6.053012778684776940 ) ) ;
#22178=CARTESIAN_POINT ( 'NONE',  ( 152.7691010214056462, 266.0431505347400503, -16.40662330462167162 ) ) ;
#22183=CARTESIAN_POINT ( 'NONE',  ( 190.0998002681485559, 264.3044181240644548, -9.275971950984974512 ) ) ;
#22184=CARTESIAN_POINT ( 'NONE',  ( 192.3868339392006135, 271.8215131925324499, 14.10193610252311380 ) ) ;
#22185=CARTESIAN_POINT ( 'NONE',  ( 192.7248895367048362, 271.5377591740219145, -15.00482078990248169 ) ) ;
#22189=CARTESIAN_POINT ( 'NONE',  ( 24.34300500380255983, 194.8615022471903160, 5.000000000000046185 ) ) ;
#22190=ADVANCED_FACE ( 'NONE', ( #56184 ), #81536, .T. ) ;
#22192=CARTESIAN_POINT ( 'NONE',  ( 71.08131351252005459, 211.8458772461660544, 9.188101187500095079 ) ) ;
#22193=CARTESIAN_POINT ( 'NONE',  ( 206.6268150440956504, 272.7588534679261443, -10.76664753678610609 ) ) ;
#22194=CARTESIAN_POINT ( 'NONE',  ( 193.0142717932987182, 296.3364699985351081, -13.30037542329744937 ) ) ;
#22195=CARTESIAN_POINT ( 'NONE',  ( -27.42236680055714260, 166.5217562850347406, 1.224646799147364892E-15 ) ) ;
#22196=CARTESIAN_POINT ( 'NONE',  ( 161.8926315922002743, 250.2407320417157166, -13.77020595223768495 ) ) ;
#22197=CARTESIAN_POINT ( 'NONE',  ( 193.8003511027313550, 288.1208047801705447, 17.19107869180001913 ) ) ;
#22198=CONICAL_SURFACE ( 'NONE', #93472, 16.82106496071143908, 0.7853981633974241872 ) ;
#22202=CARTESIAN_POINT ( 'NONE',  ( 188.0605157086127406, 260.5832606518970920, -7.266969944812869286 ) ) ;
#22203=CARTESIAN_POINT ( 'NONE',  ( 204.9304696503118919, 275.6970098771450353, -13.62097861578000213 ) ) ;
#22204=CARTESIAN_POINT ( 'NONE',  ( 157.7045020317009403, 270.7409348844154238, -14.98380028358599603 ) ) ;
#22206=AXIS2_PLACEMENT_3D ( 'NONE', #7385, #69686, #75322 ) ;
#22207=CARTESIAN_POINT ( 'NONE',  ( 52.94873307290088604, 207.5024278399160949, 9.188101187500095079 ) ) ;
#22208=CARTESIAN_POINT ( 'NONE',  ( 157.5520850189458884, 257.7587792392113215, 16.71892742266126319 ) ) ;
#22211=CARTESIAN_POINT ( 'NONE',  ( -15.56633235393031178, 168.4865022471903160, 10.00000000000009237 ) ) ;
#22212=CARTESIAN_POINT ( 'NONE',  ( 41.36564329728400935, 200.8149278399160664, -9.188101187500095079 ) ) ;
#22215=CARTESIAN_POINT ( 'NONE',  ( 151.1811967613751335, 268.7934813906678642, -15.79361349403328418 ) ) ;
#22216=CARTESIAN_POINT ( 'NONE',  ( 149.7200635338602410, 271.3242383773507527, -12.12223662813266500 ) ) ;
#22220=CARTESIAN_POINT ( 'NONE',  ( 196.3956310503436953, 264.1850728776087180, 4.154333235580330630 ) ) ;
#22222=CARTESIAN_POINT ( 'NONE',  ( 149.3592332192440892, 275.3511165631820745, 7.499194079129854806 ) ) ;
#22224=CARTESIAN_POINT ( 'NONE',  ( 94.05805000844991071, 225.1115022471902307, 10.00000000000009592 ) ) ;
#22225=CARTESIAN_POINT ( 'NONE',  ( 200.3414094930810165, 283.6454952284590263, 16.87912319229835489 ) ) ;
#22226=CARTESIAN_POINT ( 'NONE',  ( 194.4740566694322297, 285.4027869386137581, -17.19371202535040055 ) ) ;
#22228=CARTESIAN_POINT ( 'NONE',  ( 61.04057116557046925, 215.2369531367911009, -4.594050593750048428 ) ) ;
#22229=ORIENTED_EDGE ( 'NONE', *, *, #22897, .T. ) ;
#22230=CARTESIAN_POINT ( 'NONE',  ( 179.9540635007602418, 264.0123226724073788, 15.22985420633530573 ) ) ;
#22231=CARTESIAN_POINT ( 'NONE',  ( 146.7879906441258129, 276.4027375938661635, 4.347255311287614887 ) ) ;
#22232=CARTESIAN_POINT ( 'NONE',  ( 205.2706556652093752, 273.1077904153184477, -10.97544480913108167 ) ) ;
#22233=EDGE_LOOP ( 'NONE', ( #9841, #18429, #70357, #35673 ) ) ;
#22234=CARTESIAN_POINT ( 'NONE',  ( 170.4855375986076638, 248.6613294790634541, -0.2716024841417116753 ) ) ;
#22236=CARTESIAN_POINT ( 'NONE',  ( 148.1829914015846157, 273.9865254053503349, -9.304102644963160529 ) ) ;
#22237=CARTESIAN_POINT ( 'NONE',  ( 177.1267550122267949, 274.7903246707450649, -17.34070711746236526 ) ) ;
#22239=CARTESIAN_POINT ( 'NONE',  ( 156.8572647664473152, 258.9622432186664014, 16.97926827742052325 ) ) ;
#22243=CARTESIAN_POINT ( 'NONE',  ( 169.9290877785755356, 289.3386371799751942, -2.202558799265889267 ) ) ;
#22244=CARTESIAN_POINT ( 'NONE',  ( 156.5621193438227294, 267.5160442540268946, 16.96304260999163205 ) ) ;
#22247=CARTESIAN_POINT ( 'NONE',  ( 159.2536436069973718, 254.8115933126508992, -15.76697951715411250 ) ) ;
#22251=AXIS2_PLACEMENT_3D ( 'NONE', #43492, #43980, #53092 ) ;
#22254=CARTESIAN_POINT ( 'NONE',  ( 208.1303168694798273, 270.1547119170880364, -0.9257663487928086132 ) ) ;
#22255=CARTESIAN_POINT ( 'NONE',  ( 204.8523313866422484, 275.8323493198358847, 14.65426965484541100 ) ) ;
#22256=CARTESIAN_POINT ( 'NONE',  ( 198.6742831389107096, 286.5330427765190393, 17.60232614297041565 ) ) ;
#22258=CARTESIAN_POINT ( 'NONE',  ( 131.4326323866306723, 240.5643266524160140, 9.188101187500095079 ) ) ;
#22259=CARTESIAN_POINT ( 'NONE',  ( 177.2879723884094290, 269.2816851795835191, 16.08031286173457630 ) ) ;
#22260=AXIS2_PLACEMENT_3D ( 'NONE', #42426, #3948, #81985 ) ;
#22261=CARTESIAN_POINT ( 'NONE',  ( 181.5606416776419110, 260.1619400365603383, 9.495244246682995382 ) ) ;
#22262=CARTESIAN_POINT ( 'NONE',  ( 78.87554214658000262, 216.3458772461660544, 9.188101187500095079 ) ) ;
#22264=CARTESIAN_POINT ( 'NONE',  ( 170.3127733705114224, 263.9010670580030364, 17.23448983536806622 ) ) ;
#22265=CARTESIAN_POINT ( 'NONE',  ( 182.9145022086223946, 255.8442969664664304, 0.6158721635512950376 ) ) ;
#22266=ORIENTED_EDGE ( 'NONE', *, *, #95739, .F. ) ;
#22269=VERTEX_POINT ( 'NONE', #51595 ) ;
#22273=CARTESIAN_POINT ( 'NONE',  ( 197.9272639331449284, 286.8449481112537001, 16.93522022078217404 ) ) ;
#22274=CARTESIAN_POINT ( 'NONE',  ( 191.1000148935602567, 299.6520602076213891, -9.462302242170249400 ) ) ;
#22276=CARTESIAN_POINT ( 'NONE',  ( 193.7275870247597425, 295.1009717758319084, 14.48058678254265885 ) ) ;
#22280=ORIENTED_EDGE ( 'NONE', *, *, #49800, .F. ) ;
#22281=EDGE_CURVE ( 'NONE', #15004, #65652, #70088, .T. ) ;
#22283=CARTESIAN_POINT ( 'NONE',  ( 187.9760109300380861, 288.6839808275937571, 15.87893199255275789 ) ) ;
#22288=CARTESIAN_POINT ( 'NONE',  ( 183.8409078303500621, 275.4022649685220472, 16.46562491007150442 ) ) ;
#22289=CARTESIAN_POINT ( 'NONE',  ( 206.5508451493652444, 272.8904371854448527, 11.05407534521577695 ) ) ;
#22290=CARTESIAN_POINT ( 'NONE',  ( 149.0203866098534888, 272.5361143586139860, -12.73049804737905255 ) ) ;
#22292=CARTESIAN_POINT ( 'NONE',  ( 162.7946441242182232, 261.4156790044469290, 17.51582106973610564 ) ) ;
#22293=CARTESIAN_POINT ( 'NONE',  ( 127.8056303646358032, 256.8464784336661637, 1.353441290958777327E-15 ) ) ;
#22294=ORIENTED_EDGE ( 'NONE', *, *, #31829, .T. ) ;
#22298=CARTESIAN_POINT ( 'NONE',  ( 201.1388841337167435, 282.2642286331299601, -18.17233400608081340 ) ) ;
#22301=ORIENTED_EDGE ( 'NONE', *, *, #24417, .T. ) ;
#22302=CARTESIAN_POINT ( 'NONE',  ( 196.0614467148371602, 264.7781410680017302, 5.416773119000386494 ) ) ;
#22303=CARTESIAN_POINT ( 'NONE',  ( 148.3010860587701814, 276.5068540982774721, -3.904121881399305050 ) ) ;
#22305=AXIS2_PLACEMENT_3D ( 'NONE', #78401, #71303, #48492 ) ;
#22306=CARTESIAN_POINT ( 'NONE',  ( 184.6824817629046436, 263.5711312746864792, -12.44848753094074389 ) ) ;
#22307=CARTESIAN_POINT ( 'NONE',  ( 198.6594462311236100, 266.3252094933188232, 0.8312128693835356685 ) ) ;
#22308=CARTESIAN_POINT ( 'NONE',  ( 190.7908437487391780, 300.1875603386860689, -4.317984972589949955 ) ) ;
#22309=CARTESIAN_POINT ( 'NONE',  ( 186.8917667502177267, 282.0639843911756088, 17.00272728164306457 ) ) ;
#22311=AXIS2_PLACEMENT_3D ( 'NONE', #17644, #72866, #80482 ) ;
#22313=CARTESIAN_POINT ( 'NONE',  ( 177.2604144123859271, 264.5285374513375132, -15.40663022330867271 ) ) ;
#22314=CARTESIAN_POINT ( 'NONE',  ( 193.5841046816602216, 269.1605544676620525, 12.13440722373979419 ) ) ;
#22317=CARTESIAN_POINT ( 'NONE',  ( 166.4998282923256170, 286.5300311998390725, -3.271394949006546593 ) ) ;
#22319=CARTESIAN_POINT ( 'NONE',  ( 159.3767386493506137, 254.5983864451355032, 15.47015898230477760 ) ) ;
#22321=CARTESIAN_POINT ( 'NONE',  ( -6.887775800123916881, 157.6423013555410080, -4.594050593750043987 ) ) ;
#22323=VERTEX_POINT ( 'NONE', #75918 ) ;
#22326=B_SPLINE_CURVE_WITH_KNOTS ( 'NONE', 3,
 ( #95751, #93741, #9099, #2002, #55668, #48607, #87674, #55177, #48088, #70906, #80036, #78514, #57181, #17186, #10605, #1515, #41477, #3029, #63293, #79028, #88159, #49588, #10103, #80542, #40966, #9619, #40482, #32888, #2513, #89169, #3518, #21203, #82545, #34881, #13109, #97712, #27797, #58671, #27302, #43476, #81051, #89642, #97228, #66296, #51074, #35882, #11614, #66786, #34395, #98206, #96737, #5005 ),
 .UNSPECIFIED., .F., .F.,
 ( 4, 2, 2, 2, 2, 2, 2, 2, 2, 2, 2, 2, 2, 2, 2, 2, 2, 2, 2, 2, 2, 2, 2, 2, 2, 4 ),
 ( 0.0006802182506974893640, 0.001179301278685929155, 0.001678384306674368838, 0.001927925820668672380, 0.002177467334662975488, 0.002302238091660068712, 0.002427008848657161936, 0.002551779605654255594, 0.002676550362651348818, 0.002926091876645458504, 0.003175633390639568624, 0.003674716418627863891, 0.004672882474604453558, 0.005671048530581044092, 0.006170131558569339793, 0.006419673072563446443, 0.006669214586557552227, 0.006731599965056004296, 0.006793985343554457233, 0.006856370722052909303, 0.006918756100551360505, 0.007168297614545246846, 0.007667380642533016058, 0.008166463670520785270, 0.008416005184514652529, 0.008665546698508521523 ),
 .UNSPECIFIED. ) ;
#22328=CARTESIAN_POINT ( 'NONE',  ( 151.1451503555562113, 268.8559155969762742, -15.81507177720227553 ) ) ;
#22329=CARTESIAN_POINT ( 'NONE',  ( 5.371288904610766579, 186.1589784336661637, -6.496448406907676862E-16 ) ) ;
#22331=CARTESIAN_POINT ( 'NONE',  ( 181.2988614377958356, 275.3026993373888445, -16.43866227028271965 ) ) ;
#22334=CARTESIAN_POINT ( 'NONE',  ( 72.38141447910541615, 201.0494855054051868, -2.679491924311248496 ) ) ;
#22336=CARTESIAN_POINT ( 'NONE',  ( 127.8330407560430473, 244.6115022471902591, 10.00000000000009592 ) ) ;
#22337=B_SPLINE_SURFACE_WITH_KNOTS ( 'NONE', 3, 1, ( 
 ( #42646, #64980 ),
 ( #58352, #36046 ),
 ( #95923, #57360 ),
 ( #51771, #20376 ),
 ( #65963, #66949 ),
 ( #88335, #73578 ),
 ( #74082, #28451 ),
 ( #49770, #27484 ),
 ( #50753, #81706 ),
 ( #12278, #4671 ),
 ( #35561, #66462 ),
 ( #97387, #92780 ),
 ( #29456, #61 ),
 ( #45630, #37049 ),
 ( #21853, #76558 ),
 ( #98379, #36544 ),
 ( #92295, #23333 ),
 ( #54222, #13279 ),
 ( #5655, #68442 ),
 ( #67451, #61337 ),
 ( #53729, #99370 ),
 ( #84203, #22351 ),
 ( #22846, #28968 ),
 ( #53247, #7139 ),
 ( #14257, #84688 ),
 ( #59846, #91785 ),
 ( #38536, #14749 ),
 ( #44141, #52248 ),
 ( #7645, #38026 ),
 ( #77039, #99862 ),
 ( #30447, #90809 ),
 ( #60824, #15229 ),
 ( #6155, #75566 ),
 ( #46125, #69443 ) ),
 .UNSPECIFIED., .T., .F., .F.,
 ( 4, 2, 2, 2, 2, 2, 2, 2, 2, 2, 2, 2, 2, 2, 2, 2, 4 ),
 ( 2, 2 ),
 ( 0.000000000000000000, 0.06250000000000000000, 0.1250000000000000000, 0.1875000000000000000, 0.2500000000000000000, 0.3125000000000000000, 0.3750000000000000000, 0.4375000000000000000, 0.5000000000000000000, 0.5625000000000000000, 0.6250000000000000000, 0.6875000000000000000, 0.7500000000000000000, 0.8125000000000000000, 0.8750000000000000000, 0.9375000000000000000, 1.000000000000000000 ),
 ( 0.000000000000000000, 1.000000000000000000 ),
 .UNSPECIFIED. ) ;
#22338=CARTESIAN_POINT ( 'NONE',  ( 175.5289681635948398, 253.4651622633166710, -3.633261989091086441 ) ) ;
#22339=CARTESIAN_POINT ( 'NONE',  ( 191.1394246315239229, 261.3397897443172724, -1.588466913715747442 ) ) ;
#22341=CARTESIAN_POINT ( 'NONE',  ( 52.92184332868904306, 211.3615022471903160, 5.000000000000046185 ) ) ;
#22342=CYLINDRICAL_SURFACE ( 'NONE', #99239, 17.82106496071139645 ) ;
#22344=CARTESIAN_POINT ( 'NONE',  ( 148.4016473149517594, 273.6078022540229426, 8.470066617688926769 ) ) ;
#22345=CARTESIAN_POINT ( 'NONE',  ( 26.12944271915780448, 176.7048013555409796, 4.594050593750051981 ) ) ;
#22351=CARTESIAN_POINT ( 'NONE',  ( 164.5867587387928950, 245.5743669417666126, -3.022048486790635202 ) ) ;
#22353=CARTESIAN_POINT ( 'NONE',  ( 160.5424585579978896, 278.9220658006375970, -9.787057437366879498 ) ) ;
#22356=CARTESIAN_POINT ( 'NONE',  ( 148.2267527339363369, 273.9107285543102535, 7.913369084260907016 ) ) ;
#22358=CARTESIAN_POINT ( 'NONE',  ( 194.2199708651012600, 294.2481379475345875, 15.50834247347371253 ) ) ;
#22360=CARTESIAN_POINT ( 'NONE',  ( 185.5050748790181672, 290.8734282190925455, 12.35404501033644920 ) ) ;
#22362=CARTESIAN_POINT ( 'NONE',  ( 4.715407580134756138, 161.9824982072973683, 3.021315404115420679E-15 ) ) ;
#22368=CARTESIAN_POINT ( 'NONE',  ( 154.8833801513861772, 262.3811116602312268, -17.49275566389638215 ) ) ;
#22371=DIRECTION ( 'NONE',  ( 0.4999999999999998890, -0.8660254037844385966, 0.000000000000000000 ) ) ;
#22372=CARTESIAN_POINT ( 'NONE',  ( 204.9768178125733016, 275.6167325052707611, 13.98665089523138505 ) ) ;
#22373=EDGE_LOOP ( 'NONE', ( #66873, #73886, #11808, #64545 ) ) ;
#22374=CARTESIAN_POINT ( 'NONE',  ( 150.7226148805041817, 269.5877685077668957, 15.52819754351937576 ) ) ;
#22375=AXIS2_PLACEMENT_3D ( 'NONE', #79655, #2626, #31992 ) ;
#22379=VERTEX_POINT ( 'NONE', #64693 ) ;
#22380=CARTESIAN_POINT ( 'NONE',  ( 148.2980785574368952, 273.7871886041155562, 9.134436720559454770 ) ) ;
#22381=VECTOR ( 'NONE', #88209, 1000.000000000000000 ) ;
#22384=CARTESIAN_POINT ( 'NONE',  ( 206.3106310032756596, 273.3065002911688453, 10.17860425536756175 ) ) ;
#22387=ORIENTED_EDGE ( 'NONE', *, *, #81117, .F. ) ;
#22388=EDGE_CURVE ( 'NONE', #58638, #26637, #7872, .T. ) ;
#22389=CARTESIAN_POINT ( 'NONE',  ( 149.0359194785865498, 272.5092106407810206, 12.76357969772040590 ) ) ;
#22391=VERTEX_POINT ( 'NONE', #93190 ) ;
#22400=CARTESIAN_POINT ( 'NONE',  ( 146.7845206192450007, 276.4087478532630939, 4.443586170796542945 ) ) ;
#22401=CARTESIAN_POINT ( 'NONE',  ( 147.6300909839706321, 274.9441770201837585, 8.328755691084779755 ) ) ;
#22402=CARTESIAN_POINT ( 'NONE',  ( 149.3833831332874240, 271.9073859370555510, 11.40518020539810173 ) ) ;
#22403=CARTESIAN_POINT ( 'NONE',  ( 171.0589475124673413, 275.4374387251525036, -16.05662091941493586 ) ) ;
#22405=CARTESIAN_POINT ( 'NONE',  ( 146.5163827660608433, 276.8731762384107356, -0.1825760380121486393 ) ) ;
#22406=ADVANCED_FACE ( 'NONE', ( #55141 ), #76329, .F. ) ;
#22407=CARTESIAN_POINT ( 'NONE',  ( 191.7741832257749195, 298.4843664033717801, -8.615487418695501276 ) ) ;
#22408=CARTESIAN_POINT ( 'NONE',  ( 163.5970988786415035, 257.6140216154675500, 15.49997863511091545 ) ) ;
#22412=CARTESIAN_POINT ( 'NONE',  ( 167.8632803254916723, 287.0380262542474838, 3.490854160492717462 ) ) ;
#22414=CARTESIAN_POINT ( 'NONE',  ( 106.9945647975297760, 223.3923013555410080, 4.594050593750050204 ) ) ;
#22416=CARTESIAN_POINT ( 'NONE',  ( 190.6156810949310056, 300.4909509546700974, -4.738288261098400511 ) ) ;
#22420=CARTESIAN_POINT ( 'NONE',  ( 179.9804799098377543, 283.2464424863279646, -16.00788805095805500 ) ) ;
#22422=CARTESIAN_POINT ( 'NONE',  ( 168.9026472910029213, 285.9199674911590705, -7.578321094149770509 ) ) ;
#22423=ORIENTED_EDGE ( 'NONE', *, *, #5586, .F. ) ;
#22424=CARTESIAN_POINT ( 'NONE',  ( 207.5920568422024814, 271.0870056320159165, -1.586464549033245186 ) ) ;
#22425=DIRECTION ( 'NONE',  ( -0.8660254037844387076, -0.4999999999999998890, -0.000000000000000000 ) ) ;
#22427=CARTESIAN_POINT ( 'NONE',  ( 34.21208616421480286, 203.8927522451419350, 2.944929066748280225E-16 ) ) ;
#22428=CARTESIAN_POINT ( 'NONE',  ( 107.8059429699301575, 242.2369531367911009, -4.594050593750048428 ) ) ;
#22429=CARTESIAN_POINT ( 'NONE',  ( 199.2383506163646132, 285.5560492466715345, -17.78808061564097898 ) ) ;
#22431=CARTESIAN_POINT ( 'NONE',  ( 157.2744851780909414, 258.2395962677452985, 18.17792129701959070 ) ) ;
#22432=CARTESIAN_POINT ( 'NONE',  ( 175.5508771970481803, 253.4024090357540615, -4.579646307325052845 ) ) ;
#22433=CARTESIAN_POINT ( 'NONE',  ( 38.44315465527655107, 186.8768266524159856, -9.188101187500091527 ) ) ;
#22434=VECTOR ( 'NONE', #43977, 1000.000000000000000 ) ;
#22437=CARTESIAN_POINT ( 'NONE',  ( -0.5010987708114443828, 180.5177522451419350, 5.000000000000046185 ) ) ;
#22438=CARTESIAN_POINT ( 'NONE',  ( 178.1315106821064091, 265.7600619140744129, 15.42674999082912812 ) ) ;
#22440=CARTESIAN_POINT ( 'NONE',  ( 147.4811722709131914, 275.2021117973970377, 3.890385073228495916 ) ) ;
#22442=CYLINDRICAL_SURFACE ( 'NONE', #60793, 10.00000000000010658 ) ;
#22443=CARTESIAN_POINT ( 'NONE',  ( 165.2854559968822343, 250.6596768082254414, 10.19847216201956641 ) ) ;
#22444=CARTESIAN_POINT ( 'NONE',  ( 114.7524487161676774, 230.3927522451418213, -10.00000000000009059 ) ) ;
#22447=ORIENTED_EDGE ( 'NONE', *, *, #74681, .T. ) ;
#22449=CARTESIAN_POINT ( 'NONE',  ( 163.1008115941903895, 248.1481028935802442, 11.25332017433677834 ) ) ;
#22450=CARTESIAN_POINT ( 'NONE',  ( 208.0421103033489771, 270.3074901711881353, -2.473242163239977476 ) ) ;
#22452=EDGE_CURVE ( 'NONE', #80984, #92056, #58151, .T. ) ;
#22453=CARTESIAN_POINT ( 'NONE',  ( 13.89683389070260944, 169.6423013555409796, -4.594050593750043987 ) ) ;
#22455=CARTESIAN_POINT ( 'NONE',  ( 194.3301429122894888, 273.0266408274683840, 14.32923346541002374 ) ) ;
#22458=CARTESIAN_POINT ( 'NONE',  ( 174.6713748507754929, 286.4050021081735622, 10.35879135939865847 ) ) ;
#22459=CARTESIAN_POINT ( 'NONE',  ( 66.56148311469628709, 218.4244531367911293, -4.594050593750046652 ) ) ;
#22460=EDGE_CURVE ( 'NONE', #74797, #36600, #3744, .T. ) ;
#22461=CARTESIAN_POINT ( 'NONE',  ( 208.2764314485352770, 269.9016340424377063, 2.433736665191914117 ) ) ;
#22467=CARTESIAN_POINT ( 'NONE',  ( 8.321535033790485869, 175.6115022471902307, 10.00000000000009592 ) ) ;
#22468=CARTESIAN_POINT ( 'NONE',  ( 164.3053959849042087, 246.0617015268593661, -7.251939739328854273 ) ) ;
#22469=CARTESIAN_POINT ( 'NONE',  ( 143.8006444583684242, 244.6423013555409796, -4.594050593750043987 ) ) ;
#22471=CARTESIAN_POINT ( 'NONE',  ( 165.4376610383445723, 261.3391624790643277, -16.16452297080461165 ) ) ;
#22472=EDGE_CURVE ( 'NONE', #83741, #28867, #16980, .T. ) ;
#22474=CARTESIAN_POINT ( 'NONE',  ( 195.4968220042985365, 281.1850258734705790, -17.68988808217971709 ) ) ;
#22478=ORIENTED_EDGE ( 'NONE', *, *, #32486, .T. ) ;
#22479=CARTESIAN_POINT ( 'NONE',  ( 190.8860811105559208, 300.0226043892405414, 8.636347304323541252 ) ) ;
#22480=CARTESIAN_POINT ( 'NONE',  ( 208.3738965968843502, 269.7328194535299986, -0.6978089580936264191 ) ) ;
#22481=CARTESIAN_POINT ( 'NONE',  ( 152.3249143222120381, 268.8125044657937792, -15.54600960379902297 ) ) ;
#22485=CARTESIAN_POINT ( 'NONE',  ( 160.2385711492790108, 253.1056487676453628, 14.63819537062152598 ) ) ;
#22486=DIRECTION ( 'NONE',  ( -0.8660254037844387076, -0.4999999999999998890, -0.000000000000000000 ) ) ;
#22489=DIRECTION ( 'NONE',  ( 0.4999999999999992784, -0.8660254037844390407, 0.000000000000000000 ) ) ;
#22491=CARTESIAN_POINT ( 'NONE',  ( 186.6036341826941509, 277.9756864068600635, 17.81853497364681616 ) ) ;
#22493=CARTESIAN_POINT ( 'NONE',  ( 201.4214977800931763, 281.7747274386935601, -17.04225209925078133 ) ) ;
#22494=CARTESIAN_POINT ( 'NONE',  ( 191.0170027573799700, 280.9900163574024532, 16.65089222855447204 ) ) ;
#22497=ORIENTED_EDGE ( 'NONE', *, *, #57951, .T. ) ;
#22498=CARTESIAN_POINT ( 'NONE',  ( 190.6094661480870798, 300.5017155583701083, 4.598210453186021951 ) ) ;
#22502=CARTESIAN_POINT ( 'NONE',  ( 191.3610003135137276, 299.2000202002271294, -9.855749861282104618 ) ) ;
#22504=CARTESIAN_POINT ( 'NONE',  ( 204.2457645315488719, 276.8829539310449945, 14.53406579917280261 ) ) ;
#22507=CARTESIAN_POINT ( 'NONE',  ( 104.3964885861764600, 221.8923013555410080, 4.594050593750050204 ) ) ;
#22508=CARTESIAN_POINT ( 'NONE',  ( 161.1884843536000744, 251.4603508349806873, 13.21272898143761942 ) ) ;
#22509=CARTESIAN_POINT ( 'NONE',  ( 181.3300189534027709, 271.3270077267823694, -16.02231281199806645 ) ) ;
#22520=CARTESIAN_POINT ( 'NONE',  ( 163.8455942243524248, 246.8581015375447691, -7.178103170949780676 ) ) ;
#22521=CARTESIAN_POINT ( 'NONE',  ( 165.7734550839200836, 271.2459260585341099, 16.34257236049911910 ) ) ;
#22523=B_SPLINE_CURVE_WITH_KNOTS ( 'NONE', 3,
 ( #4280, #80848, #42272, #50878 ),
 .UNSPECIFIED., .F., .F.,
 ( 4, 4 ),
 ( 0.004692142627948476911, 0.01023732688395309794 ),
 .UNSPECIFIED. ) ;
#22524=CARTESIAN_POINT ( 'NONE',  ( 167.2155108587164136, 281.8882477833899998, 11.54502438761175576 ) ) ;
#22525=CARTESIAN_POINT ( 'NONE',  ( 194.3442947553755005, 294.0328026529847421, -15.97648891113594871 ) ) ;
#22528=EDGE_CURVE ( 'NONE', #96078, #23912, #24167, .T. ) ;
#22532=CARTESIAN_POINT ( 'NONE',  ( 201.0247283420269184, 278.7743575993829950, -15.66353679845565061 ) ) ;
#22535=DIRECTION ( 'NONE',  ( -0.8660254037844387076, -0.4999999999999998890, -0.000000000000000000 ) ) ;
#22537=EDGE_CURVE ( 'NONE', #73589, #47832, #97932, .T. ) ;
#22538=CARTESIAN_POINT ( 'NONE',  ( 54.05850166760819775, 212.0177522451419065, 5.000000000000046185 ) ) ;
#22539=EDGE_CURVE ( 'NONE', #95735, #93829, #7297, .T. ) ;
#22540=CARTESIAN_POINT ( 'NONE',  ( 188.8122907880376147, 259.7915673222115061, 2.322190842852634329 ) ) ;
#22543=CARTESIAN_POINT ( 'NONE',  ( 172.0545069220451921, 254.4921861736880260, 11.48538074941503773 ) ) ;
#22544=CARTESIAN_POINT ( 'NONE',  ( 157.6090322939100474, 281.6562889287993698, 1.386678441765768932 ) ) ;
#22546=CARTESIAN_POINT ( 'NONE',  ( 102.3056452726415984, 218.3262482093457493, 3.021315404115420679E-15 ) ) ;
#22549=CARTESIAN_POINT ( 'NONE',  ( -4.759057006084942643, 181.3927522451419634, 2.944929066748280225E-16 ) ) ;
#22550=CARTESIAN_POINT ( 'NONE',  ( 196.1441694980680666, 269.5113810647022774, -10.83627284691216808 ) ) ;
#22552=CARTESIAN_POINT ( 'NONE',  ( 203.9379510532215818, 277.4161025147623718, -15.87772908648316061 ) ) ;
#22554=CARTESIAN_POINT ( 'NONE',  ( 161.9037764296581088, 250.9274884326035533, -12.69612398869453784 ) ) ;
#22555=CARTESIAN_POINT ( 'NONE',  ( -8.322217149083147802, 159.8768266524159856, -9.188101187500091527 ) ) ;
#22558=CARTESIAN_POINT ( 'NONE',  ( 163.3885797654601788, 248.6152187624725229, 9.728336025080901450 ) ) ;
#22559=ORIENTED_EDGE ( 'NONE', *, *, #11776, .F. ) ;
#22562=DIRECTION ( 'NONE',  ( -0.8660254037844387076, -0.4999999999999998890, -0.000000000000000000 ) ) ;
#22563=CARTESIAN_POINT ( 'NONE',  ( 151.2375434627641084, 277.2274377546415849, 6.632753350058649744 ) ) ;
#22565=CARTESIAN_POINT ( 'NONE',  ( 162.4372904523162902, 249.2973552232023735, -11.26290998720616621 ) ) ;
#22566=DIRECTION ( 'NONE',  ( 0.4999999999999998890, -0.8660254037844385966, 0.000000000000000000 ) ) ;
#22567=B_SPLINE_CURVE_WITH_KNOTS ( 'NONE', 3,
 ( #25007, #47305, #87887, #25519 ),
 .UNSPECIFIED., .F., .F.,
 ( 4, 4 ),
 ( 0.009431583545826283804, 0.01484449304010337575 ),
 .UNSPECIFIED. ) ;
#22568=CARTESIAN_POINT ( 'NONE',  ( 21.77181853666109745, 189.5024278399161233, 9.188101187500095079 ) ) ;
#22569=CARTESIAN_POINT ( 'NONE',  ( 116.3854409958760385, 231.8768266524160140, -9.188101187500091527 ) ) ;
#22570=CARTESIAN_POINT ( 'NONE',  ( 182.0997321953872188, 294.5560652551307044, -6.453979911311197526 ) ) ;
#22572=CARTESIAN_POINT ( 'NONE',  ( 149.9839146186740777, 271.6364095184536609, -11.71912693422898677 ) ) ;
#22577=CARTESIAN_POINT ( 'NONE',  ( 184.3226795282388650, 274.5458599865910969, 17.66928848808302988 ) ) ;
#22578=CARTESIAN_POINT ( 'NONE',  ( 188.9978738728263465, 284.0756316726331079, 16.44648605183132872 ) ) ;
#22581=CARTESIAN_POINT ( 'NONE',  ( 186.9492098651599861, 298.8821793078109295, -0.5976176902946377378 ) ) ;
#22583=CARTESIAN_POINT ( 'NONE',  ( 50.46014644935972626, 188.3932355074535963, -2.679491924311248496 ) ) ;
#22584=FACE_OUTER_BOUND ( 'NONE', #63786, .T. ) ;
#22586=CARTESIAN_POINT ( 'NONE',  ( -22.42236680055709641, 157.8615022471902591, 0.000000000000000000 ) ) ;
#22588=CARTESIAN_POINT ( 'NONE',  ( 94.78875894111908451, 225.5333772461660544, 9.188101187500095079 ) ) ;
#22590=CARTESIAN_POINT ( 'NONE',  ( 150.6931560952953646, 269.6387926204777727, 14.65021044537114037 ) ) ;
#22593=CARTESIAN_POINT ( 'NONE',  ( 171.3928239984006723, 250.3015599828365509, -5.796133048607560845 ) ) ;
#22595=CARTESIAN_POINT ( 'NONE',  ( 108.1850894041356810, 233.2677522451418497, 10.00000000000009592 ) ) ;
#22596=CARTESIAN_POINT ( 'NONE',  ( 198.2505066714982149, 285.2670451491296149, 0.000000000000000000 ) ) ;
#22597=CARTESIAN_POINT ( 'NONE',  ( 159.9950753608005130, 276.8117990079294373, 13.35014033362692487 ) ) ;
#22598=CARTESIAN_POINT ( 'NONE',  ( 138.2253456014562403, 260.6115022471903444, -5.000000000000047962 ) ) ;
#22601=CARTESIAN_POINT ( 'NONE',  ( 198.7178327464537801, 265.3776419993419040, 3.619097246555301961 ) ) ;
#22602=ORIENTED_EDGE ( 'NONE', *, *, #38592, .T. ) ;
#22605=CARTESIAN_POINT ( 'NONE',  ( 160.6332181072797312, 257.2038896978352227, 16.95477083490439441 ) ) ;
#22606=CARTESIAN_POINT ( 'NONE',  ( 200.0258286195224855, 270.0420316592483800, 9.097251813766577655 ) ) ;
#22607=B_SPLINE_CURVE_WITH_KNOTS ( 'NONE', 3,
 ( #383, #63176, #17581, #70269, #31758, #47962, #8485, #25173, #93614, #39848, #31271, #878, #30789, #46461, #100203, #39355, #23660, #62158, #9493, #32273, #69276, #94616, #85015, #69775, #16575, #56054, #7993, #38868, #93105, #62662, #70781, #86541, #61669, #54551, #85535, #46980, #54059, #78905 ),
 .UNSPECIFIED., .F., .F.,
 ( 4, 2, 2, 2, 2, 2, 2, 2, 2, 2, 2, 2, 2, 2, 2, 2, 2, 2, 4 ),
 ( 0.003133190382345474832, 0.003329911802006756648, 0.003526633221668038030, 0.003624993931498598273, 0.003723354641329158516, 0.003920076060990278569, 0.004313518900312601073, 0.004706961739634923578, 0.005493847418279567719, 0.006280733096924212729, 0.007854504454213501879, 0.008051225873874617162, 0.008100406228789911595, 0.008149586583705209497, 0.008247947293535850405, 0.008641390132858299544, 0.009034832972180748684, 0.009231554391841950702, 0.009428275811503154455 ),
 .UNSPECIFIED. ) ;
#22612=CARTESIAN_POINT ( 'NONE',  ( 198.4772197948566372, 286.8743665007300478, 18.43646439804394532 ) ) ;
#22613=CARTESIAN_POINT ( 'NONE',  ( 183.6368557740999279, 264.3442894037191309, -13.58800719496283804 ) ) ;
#22614=CARTESIAN_POINT ( 'NONE',  ( 169.6113679783735222, 252.3049375988781264, -8.761831181614468278 ) ) ;
#22617=LINE ( 'NONE', #54481, #63036 ) ;
#22619=CARTESIAN_POINT ( 'NONE',  ( 187.2446448861898318, 278.7970116248035879, 17.43233615778165202 ) ) ;
#22620=B_SPLINE_SURFACE_WITH_KNOTS ( 'NONE', 3, 1, ( 
 ( #59580, #5411 ),
 ( #48130, #25853 ),
 ( #80075, #88194 ),
 ( #32926, #12520 ),
 ( #49141, #18744 ),
 ( #2553, #50992 ),
 ( #9657, #79073 ),
 ( #64334, #56215 ),
 ( #51498, #10647 ),
 ( #63830, #81942 ),
 ( #40516, #95294 ),
 ( #3069, #41521 ),
 ( #72464, #13029 ),
 ( #36294, #56729 ),
 ( #43392, #33955 ),
 ( #74335, #67196 ),
 ( #71451, #17747 ),
 ( #87212, #17222 ),
 ( #26343, #87712 ),
 ( #4924, #35802 ),
 ( #66696, #28197 ),
 ( #98118, #94767 ),
 ( #25329, #48647 ),
 ( #79582, #10143 ),
 ( #41008, #21126 ),
 ( #31179, #6891 ),
 ( #14981, #61580 ),
 ( #45867, #29210 ),
 ( #76792, #92050 ),
 ( #38780, #92530 ),
 ( #83941, #13519 ),
 ( #36791, #23078 ),
 ( #53970, #22094 ),
 ( #68683, #90556 ) ),
 .UNSPECIFIED., .T., .F., .F.,
 ( 4, 2, 2, 2, 2, 2, 2, 2, 2, 2, 2, 2, 2, 2, 2, 2, 4 ),
 ( 2, 2 ),
 ( 0.000000000000000000, 0.06250000000000000000, 0.1250000000000000000, 0.1875000000000000000, 0.2500000000000000000, 0.3125000000000000000, 0.3750000000000000000, 0.4375000000000000000, 0.5000000000000000000, 0.5625000000000000000, 0.6250000000000000000, 0.6875000000000000000, 0.7500000000000000000, 0.8125000000000000000, 0.8750000000000000000, 0.9375000000000000000, 1.000000000000000000 ),
 ( 0.000000000000000000, 1.000000000000000000 ),
 .UNSPECIFIED. ) ;
#22623=CARTESIAN_POINT ( 'NONE',  ( 167.9675024332174473, 249.3202678378337964, 6.485191139041705632 ) ) ;
#22625=ORIENTED_EDGE ( 'NONE', *, *, #54311, .T. ) ;
#22627=CARTESIAN_POINT ( 'NONE',  ( 206.3068339233826975, 273.3130770264637590, 11.67356747362499547 ) ) ;
#22629=CARTESIAN_POINT ( 'NONE',  ( 153.6091969257113874, 264.5880617452517072, -18.08645444069259511 ) ) ;
#22630=CARTESIAN_POINT ( 'NONE',  ( 153.1961624462112752, 265.3034584490234806, -16.19494717845262954 ) ) ;
#22635=CARTESIAN_POINT ( 'NONE',  ( 156.4163639670109092, 273.5530270839410036, -14.20678783894327069 ) ) ;
#22636=VERTEX_POINT ( 'NONE', #40320 ) ;
#22637=CARTESIAN_POINT ( 'NONE',  ( 196.1009891436883379, 290.6035456363609342, 16.03271038754406419 ) ) ;
#22638=ORIENTED_EDGE ( 'NONE', *, *, #66531, .T. ) ;
#22640=CARTESIAN_POINT ( 'NONE',  ( 157.5487431480040925, 257.7645675294749594, -18.29554785922338311 ) ) ;
#22641=CARTESIAN_POINT ( 'NONE',  ( 163.5242786094305529, 253.3114143684073269, 14.53606660635604975 ) ) ;
#22642=ADVANCED_FACE ( 'NONE', ( #95602 ), #8407, .F. ) ;
#22643=CARTESIAN_POINT ( 'NONE',  ( 152.4004768191108781, 241.6816263820140307, 0.000000000000000000 ) ) ;
#22644=CARTESIAN_POINT ( 'NONE',  ( 165.2963502628107619, 246.1214967944202954, 3.165412660861774974 ) ) ;
#22645=CARTESIAN_POINT ( 'NONE',  ( 206.5266458972945429, 272.9323515195362120, -9.802257691457246125 ) ) ;
#22646=CARTESIAN_POINT ( 'NONE',  ( 197.7177225922534944, 272.6128245650874078, -13.25409340876743336 ) ) ;
#22648=CARTESIAN_POINT ( 'NONE',  ( 192.5284579606305613, 297.1779242397361713, -13.15228012403107272 ) ) ;
#22649=CARTESIAN_POINT ( 'NONE',  ( 171.1445398911689608, 250.9114044520595712, -5.572095004965957443 ) ) ;
#22650=CARTESIAN_POINT ( 'NONE',  ( 165.8412968737758888, 265.9713712601042062, 17.00718710691081981 ) ) ;
#22652=CARTESIAN_POINT ( 'NONE',  ( 183.4095142257296800, 284.6173269999417244, -15.03714304829159154 ) ) ;
#22654=CARTESIAN_POINT ( 'NONE',  ( 119.6601863278771845, 230.7048013555409796, 4.594050593750051981 ) ) ;
#22656=CARTESIAN_POINT ( 'NONE',  ( 184.5555326536461678, 260.2792554538418699, -9.747852867291117107 ) ) ;
#22658=CARTESIAN_POINT ( 'NONE',  ( 156.6812872898450735, 261.2670451491295012, 0.000000000000000000 ) ) ;
#22661=ORIENTED_EDGE ( 'NONE', *, *, #76587, .F. ) ;
#22667=CARTESIAN_POINT ( 'NONE',  ( 192.8425562372348452, 296.6338900660878721, 11.79498561092278841 ) ) ;
#22668=CARTESIAN_POINT ( 'NONE',  ( 159.5895502557670795, 254.2297859303815244, -16.92708575547316485 ) ) ;
#22669=CARTESIAN_POINT ( 'NONE',  ( 88.40853095561153907, 233.3967562850347122, -4.648177544792955347E-16 ) ) ;
#22671=CARTESIAN_POINT ( 'NONE',  ( 195.4960223750947250, 292.0379518991509258, 15.68485942957119406 ) ) ;
#22672=( BOUNDED_CURVE ( )  B_SPLINE_CURVE ( 2, ( #97798, #88741, #58756, #4577, #73491, #28367, #20287, #66376, #81132 ),
 .UNSPECIFIED., .F., .T. ) 
 B_SPLINE_CURVE_WITH_KNOTS ( ( 3, 2, 2, 2, 3 ),
 ( 0.7782258064516128782, 0.7795698924731182533, 0.7822580645161290036, 0.7849462365591397539, 0.7862903225806451291 ),
 .UNSPECIFIED. ) 
 CURVE ( )  GEOMETRIC_REPRESENTATION_ITEM ( )  RATIONAL_B_SPLINE_CURVE ( ( 0.9330127018922194093, 0.9330127018922194093, 1.000000000000000000, 0.8660254037844387076, 1.000000000000000000, 0.8660254037844387076, 1.000000000000000000, 0.9330127018922194093, 0.9330127018922194093 ) ) 
 REPRESENTATION_ITEM ( '' )  );
#22674=CARTESIAN_POINT ( 'NONE',  ( 61.87308422990769685, 194.9824982072973967, 3.021315404115420679E-15 ) ) ;
#22675=CARTESIAN_POINT ( 'NONE',  ( 196.4030970371012472, 264.3490001850324234, -4.693669024083267693 ) ) ;
#22677=CARTESIAN_POINT ( 'NONE',  ( 188.5598007550805733, 265.1235053368025092, -11.94157573910213799 ) ) ;
#22679=CARTESIAN_POINT ( 'NONE',  ( 196.3492756709495382, 264.2680142592890888, 4.029091280256919205 ) ) ;
#22682=CARTESIAN_POINT ( 'NONE',  ( 184.8269865458371726, 289.1777887761302850, -13.20314450223754754 ) ) ;
#22683=CARTESIAN_POINT ( 'NONE',  ( 156.9442477613751805, 280.6005629174807723, 5.998941275641159976 ) ) ;
#22684=CYLINDRICAL_SURFACE ( 'NONE', #86774, 17.82106496071139645 ) ;
#22685=EDGE_LOOP ( 'NONE', ( #89025, #87862, #15653, #61998, #58422 ) ) ;
#22686=CARTESIAN_POINT ( 'NONE',  ( 204.7036265338580279, 272.9347255250285684, -9.700744708777794045 ) ) ;
#22691=CARTESIAN_POINT ( 'NONE',  ( 174.1511926551437170, 259.1985027499044918, -14.38432268034557993 ) ) ;
#22693=CARTESIAN_POINT ( 'NONE',  ( 52.25428207639063061, 207.6427522451419350, -10.00000000000009592 ) ) ;
#22694=CARTESIAN_POINT ( 'NONE',  ( 155.6518451030846961, 261.0500913200531841, 17.91778754207898317 ) ) ;
#22698=CARTESIAN_POINT ( 'NONE',  ( 76.00665944866153723, 220.8149278399160664, 9.188101187500093303 ) ) ;
#22699=CARTESIAN_POINT ( 'NONE',  ( 159.7132918459648181, 254.0154592091499239, -16.90058287995827158 ) ) ;
#22700=CARTESIAN_POINT ( 'NONE',  ( 193.2140586456748679, 295.9904290195353269, -12.67640480829088823 ) ) ;
#22701=CARTESIAN_POINT ( 'NONE',  ( 163.4178923001155681, 247.5989030008181260, -10.38047187240561442 ) ) ;
#22703=CARTESIAN_POINT ( 'NONE',  ( 197.2380956165551709, 287.7323366031149021, -17.26490520431893572 ) ) ;
#22704=CARTESIAN_POINT ( 'NONE',  ( 207.1770866921659717, 271.8057550155037347, -5.569195235244989384 ) ) ;
#22706=CARTESIAN_POINT ( 'NONE',  ( 99.93749413994396491, 240.0530062829862743, -4.648177544792955347E-16 ) ) ;
#22710=CARTESIAN_POINT ( 'NONE',  ( 205.5937218600166432, 274.5482233517041095, -12.97537981636971338 ) ) ;
#22711=CARTESIAN_POINT ( 'NONE',  ( 157.2333142128019858, 258.3109064714224132, 16.87956768598436597 ) ) ;
#22713=CARTESIAN_POINT ( 'NONE',  ( 54.35637144981559743, 196.0643266524159856, -9.188101187500093303 ) ) ;
#22714=CARTESIAN_POINT ( 'NONE',  ( 157.7233946900069839, 257.4620621851055375, 16.86796251324260254 ) ) ;
#22715=CARTESIAN_POINT ( 'NONE',  ( 180.1168005803277481, 295.2192856762299016, -2.191971455912026467 ) ) ;
#22716=EDGE_CURVE ( 'NONE', #18420, #93728, #74964, .T. ) ;
#22718=CARTESIAN_POINT ( 'NONE',  ( 150.8371008641169908, 248.7048013555409511, 4.594050593750051981 ) ) ;
#22721=CARTESIAN_POINT ( 'NONE',  ( 150.6916211261701619, 269.6414512649903941, -15.44346024757110847 ) ) ;
#22722=CARTESIAN_POINT ( 'NONE',  ( 196.8104339078508076, 289.7613243423628546, -16.40335862274955403 ) ) ;
#22724=CARTESIAN_POINT ( 'NONE',  ( 185.9427433571077586, 257.7868782628476083, -2.501399907045548598 ) ) ;
#22727=CARTESIAN_POINT ( 'NONE',  ( 198.4334039703542771, 286.9502577349437615, 18.47706603442866680 ) ) ;
#22729=CARTESIAN_POINT ( 'NONE',  ( 152.3777131358734209, 276.3565970158849154, 7.198581938326709562 ) ) ;
#22734=CARTESIAN_POINT ( 'NONE',  ( 121.2656814440110935, 227.4865022471901455, 1.119607411625061291E-15 ) ) ;
#22735=CARTESIAN_POINT ( 'NONE',  ( 181.1866291719431104, 292.1633450213508922, -10.35974650001995556 ) ) ;
#22736=CARTESIAN_POINT ( 'NONE',  ( 192.9105100888655500, 284.4402630435000674, -16.74955499512010348 ) ) ;
#22740=CARTESIAN_POINT ( 'NONE',  ( 159.2289198208967775, 254.8544161663325838, -15.88961297684315888 ) ) ;
#22741=CARTESIAN_POINT ( 'NONE',  ( 187.0639549125049541, 276.7591803672281117, -16.89325600899905666 ) ) ;
#22743=ORIENTED_EDGE ( 'NONE', *, *, #49267, .T. ) ;
#22744=CARTESIAN_POINT ( 'NONE',  ( 60.71607196274899110, 215.8615022471903160, 5.000000000000046185 ) ) ;
#22746=CARTESIAN_POINT ( 'NONE',  ( 194.1852025340051284, 294.3083584634874796, -15.46421316575964688 ) ) ;
#22747=CARTESIAN_POINT ( 'NONE',  ( 177.1176718376224244, 274.7376581003516094, -16.86326964924343130 ) ) ;
#22748=DIRECTION ( 'NONE',  ( 0.4999999999999998890, -0.8660254037844385966, 0.000000000000000000 ) ) ;
#22749=ORIENTED_EDGE ( 'NONE', *, *, #82386, .F. ) ;
#22750=B_SPLINE_CURVE_WITH_KNOTS ( 'NONE', 3,
 ( #20168, #51035, #74871, #35848, #5453, #42919, #67240, #98170, #52048, #59628, #81992, #52533, #97675, #91085, #74383, #82986, #6452, #13562, #44434, #35347, #75367, #58145, #5947, #28242, #36840, #68232, #67749, #98673, #29254, #21650, #83483, #44927, #43440, #37330, #12565, #89125, #19677, #12063, #62112, #39802, #15022, #93059, #45913, #54507, #23614, #7949, #78354, #53033 ),
 .UNSPECIFIED., .F., .F.,
 ( 4, 2, 2, 2, 2, 2, 2, 2, 2, 2, 2, 2, 2, 2, 2, 2, 2, 2, 2, 2, 2, 2, 2, 4 ),
 ( 0.0004852726061935422742, 0.0009346415430110950173, 0.001159326011419822573, 0.001384010479828550128, 0.001496352714032899486, 0.001608694948237248843, 0.001833379416645954932, 0.002282748353463394646, 0.003181486227098212494, 0.004080224100733030775, 0.004978961974367849055, 0.005428330911185216996, 0.005653015379593942166, 0.005765357613798340747, 0.005821528730900540904, 0.005877699848002740195, 0.005933870965104939485, 0.005990042082207139643, 0.006102384316411719502, 0.006327068784821065703, 0.006776437721639757238, 0.007225806658458449640, 0.007450491126867776759, 0.007675175595277103878 ),
 .UNSPECIFIED. ) ;
#22752=LINE ( 'NONE', #1462, #40313 ) ;
#22754=ORIENTED_EDGE ( 'NONE', *, *, #84816, .T. ) ;
#22756=B_SPLINE_CURVE_WITH_KNOTS ( 'NONE', 3,
 ( #96056, #10924, #71732, #63104, #33207, #80865, #24602, #72745, #11439, #64616, #42291, #64106, #25617, #18025, #10418, #79854 ),
 .UNSPECIFIED., .F., .F.,
 ( 4, 2, 2, 2, 2, 2, 2, 4 ),
 ( 8.673617379884035472E-19, 0.0003786681000627679949, 0.0007573362001255351224, 0.001136004300188302304, 0.001514672400251069377, 0.001893340500313836451, 0.002272008600376603741, 0.003029344800502137888 ),
 .UNSPECIFIED. ) ;
#22757=CARTESIAN_POINT ( 'NONE',  ( -1.367124174595798713, 160.0177522451418213, 5.000000000000051514 ) ) ;
#22759=AXIS2_PLACEMENT_3D ( 'NONE', #37191, #68093, #99015 ) ;
#22760=CARTESIAN_POINT ( 'NONE',  ( 173.1024016144300504, 285.3904325752632758, 10.53327312915123493 ) ) ;
#22764=CARTESIAN_POINT ( 'NONE',  ( 162.6396274730868186, 248.9468972229755082, -10.26162218571527518 ) ) ;
#22765=CARTESIAN_POINT ( 'NONE',  ( 164.4272222519600746, 245.8506922426221593, 7.021336339662529902 ) ) ;
#22766=CARTESIAN_POINT ( 'NONE',  ( 160.0072461633487535, 253.5063153963366744, 16.23938890643736244 ) ) ;
#22767=CARTESIAN_POINT ( 'NONE',  ( 161.0258333705537552, 262.9627432743089344, -17.59774463166796465 ) ) ;
#22769=CARTESIAN_POINT ( 'NONE',  ( 177.6687795445700999, 268.6483195260574917, 16.58452684940672484 ) ) ;
#22770=CARTESIAN_POINT ( 'NONE',  ( 195.5801065724998580, 291.4439665296084740, -15.68012860244166440 ) ) ;
#22771=CARTESIAN_POINT ( 'NONE',  ( 72.21814540286966633, 206.3768266524159856, -9.188101187500091527 ) ) ;
#22772=ORIENTED_EDGE ( 'NONE', *, *, #71251, .T. ) ;
#22773=CARTESIAN_POINT ( 'NONE',  ( 170.3956142831928275, 263.8003389354304886, 15.85802135508393107 ) ) ;
#22774=CARTESIAN_POINT ( 'NONE',  ( 167.2900023830132170, 283.1360949131732809, -11.47530909209802275 ) ) ;
#22775=ORIENTED_EDGE ( 'NONE', *, *, #88991, .F. ) ;
#22780=ADVANCED_FACE ( 'NONE', ( #5340 ), #98048, .T. ) ;
#22781=CARTESIAN_POINT ( 'NONE',  ( 194.3503960779362956, 284.8058050914982573, 17.28495561203828146 ) ) ;
#22782=CARTESIAN_POINT ( 'NONE',  ( 191.3041230083617563, 299.2985345825480863, -9.819045872446528378 ) ) ;
#22784=CARTESIAN_POINT ( 'NONE',  ( 193.7114073116034945, 295.1289958610702797, 14.86160832869823345 ) ) ;
#22786=CARTESIAN_POINT ( 'NONE',  ( 79.98487687335507701, 226.1744531367911293, 4.594050593750047540 ) ) ;
#22787=EDGE_LOOP ( 'NONE', ( #76211, #50391, #14278, #90324 ) ) ;
#22788=CARTESIAN_POINT ( 'NONE',  ( 161.5034534227228562, 250.9148084044473990, -12.72651426731975732 ) ) ;
#22793=CARTESIAN_POINT ( 'NONE',  ( 206.1215120922853146, 273.6340638536760821, 10.12238414215620885 ) ) ;
#22795=CARTESIAN_POINT ( 'NONE',  ( 195.3365262966702289, 279.2463014027769646, 16.32157205693540192 ) ) ;
#22796=CARTESIAN_POINT ( 'NONE',  ( 161.1581524785962642, 260.6267798172495986, 16.70816614512294862 ) ) ;
#22797=ORIENTED_EDGE ( 'NONE', *, *, #38969, .T. ) ;
#22799=CARTESIAN_POINT ( 'NONE',  ( 156.7165066408136909, 274.2344053129649524, 13.65978042195306585 ) ) ;
#22800=CARTESIAN_POINT ( 'NONE',  ( 161.9461893331167914, 280.9078031139047198, -10.53061385661272276 ) ) ;
#22801=CARTESIAN_POINT ( 'NONE',  ( 201.3715986869907510, 281.8611552031986776, -17.89433714524984964 ) ) ;
#22805=CARTESIAN_POINT ( 'NONE',  ( 195.8898456738714060, 265.0745416412873965, 5.322143108867450678 ) ) ;
#22806=CARTESIAN_POINT ( 'NONE',  ( 181.8076198581489393, 291.5803737294537541, 10.22569155168986299 ) ) ;
#22808=CARTESIAN_POINT ( 'NONE',  ( 184.5976612927380245, 263.6176899794377846, -12.36297651287966204 ) ) ;
#22809=CARTESIAN_POINT ( 'NONE',  ( 198.9491760152053530, 265.4618440174380680, 1.652013691215429736 ) ) ;
#22810=ORIENTED_EDGE ( 'NONE', *, *, #62989, .F. ) ;
#22811=CARTESIAN_POINT ( 'NONE',  ( 190.8957779480239765, 300.0058089740729770, -4.541438514207768229 ) ) ;
#22813=DIRECTION ( 'NONE',  ( 0.5000000000000048850, -0.8660254037844358210, 0.000000000000000000 ) ) ;
#22814=CARTESIAN_POINT ( 'NONE',  ( 169.8069776206597226, 261.6727971985682757, -16.70353856883196286 ) ) ;
#22817=CARTESIAN_POINT ( 'NONE',  ( 19.39713158799116499, 193.5530062829863311, -4.648177544792955347E-16 ) ) ;
#22818=CARTESIAN_POINT ( 'NONE',  ( 162.7666423248381022, 284.7022503539437253, -3.997099778975750528 ) ) ;
#22820=CARTESIAN_POINT ( 'NONE',  ( 159.6898930778639283, 254.0559870643349143, 16.90891900388599822 ) ) ;
#22821=CARTESIAN_POINT ( 'NONE',  ( 148.3831018964633870, 243.1427522451417644, 1.119607411625061291E-15 ) ) ;
#22824=CARTESIAN_POINT ( 'NONE',  ( 178.8060443869409539, 256.5898062107611963, 8.688066605584527480 ) ) ;
#22827=CARTESIAN_POINT ( 'NONE',  ( 12.62459875707045143, 178.0958772461660544, -9.188101187500095079 ) ) ;
#22830=CARTESIAN_POINT ( 'NONE',  ( 170.0816090270627683, 270.7169371497489010, -17.26929808975160796 ) ) ;
#22831=CARTESIAN_POINT ( 'NONE',  ( 179.2598940579185580, 287.6958704249323091, 13.53542817836178003 ) ) ;
#22833=CARTESIAN_POINT ( 'NONE',  ( 191.4420812244453600, 260.8157448279923187, -1.331758356259544085 ) ) ;
#22834=ADVANCED_FACE ( 'NONE', ( #8816 ), #6823, .T. ) ;
#22836=CARTESIAN_POINT ( 'NONE',  ( 70.17018262072913615, 217.9865022471902876, 10.00000000000009237 ) ) ;
#22838=CARTESIAN_POINT ( 'NONE',  ( 148.3280470635002928, 273.7352816289870248, 9.058704604771318003 ) ) ;
#22840=CARTESIAN_POINT ( 'NONE',  ( 26.64321143294855077, 192.3149278399161233, 9.188101187500093303 ) ) ;
#22845=FACE_OUTER_BOUND ( 'NONE', #49303, .T. ) ;
#22846=CARTESIAN_POINT ( 'NONE',  ( 207.1601050488701503, 271.8351680844880889, 6.320235450527015075 ) ) ;
#22847=CARTESIAN_POINT ( 'NONE',  ( 185.8037470671009714, 266.7899001189457522, 13.20055515182332684 ) ) ;
#22848=CARTESIAN_POINT ( 'NONE',  ( 163.1981911828994498, 281.1124743395109817, -10.20120161817862581 ) ) ;
#22849=CARTESIAN_POINT ( 'NONE',  ( 160.4111170237447084, 280.0480387167077083, 9.177741064962299689 ) ) ;
#22853=CARTESIAN_POINT ( 'NONE',  ( 155.2695601165254402, 261.7122283397445131, 16.98599069618989077 ) ) ;
#22854=VERTEX_POINT ( 'NONE', #91976 ) ;
#22858=CARTESIAN_POINT ( 'NONE',  ( 158.6884840273770010, 272.1760528269434189, 15.70102783839913840 ) ) ;
#22864=ORIENTED_EDGE ( 'NONE', *, *, #98844, .F. ) ;
#22868=ORIENTED_EDGE ( 'NONE', *, *, #81465, .T. ) ;
#22869=CARTESIAN_POINT ( 'NONE',  ( 190.8860811105559208, 300.0226043892405414, 8.636347304323541252 ) ) ;
#22874=CARTESIAN_POINT ( 'NONE',  ( 147.6207754342248961, 274.9603120256437592, 8.795690793376332195 ) ) ;
#22875=VERTEX_POINT ( 'NONE', #39685 ) ;
#22877=CARTESIAN_POINT ( 'NONE',  ( 158.3316779918856696, 265.2189361393055833, 17.13948956058090545 ) ) ;
#22878=ORIENTED_EDGE ( 'NONE', *, *, #41896, .F. ) ;
#22879=CARTESIAN_POINT ( 'NONE',  ( 190.6893905452545823, 300.3632824417117604, 3.294993852933539191 ) ) ;
#22883=CARTESIAN_POINT ( 'NONE',  ( 142.9371257517045137, 259.7655487066560340, -7.305945665944389766 ) ) ;
#22886=ORIENTED_EDGE ( 'NONE', *, *, #63187, .T. ) ;
#22888=CARTESIAN_POINT ( 'NONE',  ( 190.8422434538341861, 299.4678640767844513, 6.131100907076111106 ) ) ;
#22889=DIRECTION ( 'NONE',  ( -0.8660254037844387076, -0.4999999999999998890, -0.000000000000000000 ) ) ;
#22890=CARTESIAN_POINT ( 'NONE',  ( 169.7005567072155259, 288.7155782076579271, 4.430715832634252394 ) ) ;
#22891=CARTESIAN_POINT ( 'NONE',  ( 189.9462859318020946, 301.6503773875500087, -1.164147598593831656 ) ) ;
#22892=CARTESIAN_POINT ( 'NONE',  ( 149.6036070299368532, 271.5259469590175740, 11.63513718912356865 ) ) ;
#22893=CARTESIAN_POINT ( 'NONE',  ( 170.6523519555879034, 275.2952615463115649, -16.30984520614018507 ) ) ;
#22894=CARTESIAN_POINT ( 'NONE',  ( 191.0517893919347614, 299.7355892266572255, 9.200480906495027256 ) ) ;
#22895=CARTESIAN_POINT ( 'NONE',  ( 147.1731211915891322, 275.7356719181125868, 0.5879280619134324981 ) ) ;
#22896=CARTESIAN_POINT ( 'NONE',  ( 163.2687272288607403, 257.7479913314281816, 15.56745367196672092 ) ) ;
#22897=EDGE_CURVE ( 'NONE', #6222, #32604, #100260, .T. ) ;
#22899=CARTESIAN_POINT ( 'NONE',  ( 196.6288634187112052, 290.0758136547079289, -16.31544900032282186 ) ) ;
#22904=CARTESIAN_POINT ( 'NONE',  ( 190.5823735273246200, 300.5486413540409103, -3.280301628010032111 ) ) ;
#22908=CARTESIAN_POINT ( 'NONE',  ( 179.6007985214840801, 282.9056516878069374, -15.77944700681856460 ) ) ;
#22910=CARTESIAN_POINT ( 'NONE',  ( 169.0589559950515763, 284.9876656434325355, -7.953138351973477072 ) ) ;
#22911=ORIENTED_EDGE ( 'NONE', *, *, #54935, .F. ) ;
#22912=CARTESIAN_POINT ( 'NONE',  ( 162.6425574510925003, 248.9418223522047526, -10.70838742014210077 ) ) ;
#22915=CARTESIAN_POINT ( 'NONE',  ( 52.39861964368810732, 194.3927522451417929, -10.00000000000009059 ) ) ;
#22916=CARTESIAN_POINT ( 'NONE',  ( 133.0835800865360170, 238.4548013555409796, -4.594050593750042211 ) ) ;
#22918=CARTESIAN_POINT ( 'NONE',  ( 172.9438399295877957, 262.8668947608421718, -16.49499919880818766 ) ) ;
#22919=CARTESIAN_POINT ( 'NONE',  ( 157.8740713127050981, 257.2010826190796706, 17.31862062017425075 ) ) ;
#22920=CARTESIAN_POINT ( 'NONE',  ( 176.0127109592394277, 252.6004560315867593, -4.768680066900455650 ) ) ;
#22921=CARTESIAN_POINT ( 'NONE',  ( 39.63359248971512017, 199.8149278399161233, 9.188101187500093303 ) ) ;
#22926=CARTESIAN_POINT ( 'NONE',  ( 177.9596406573189427, 265.6046161183090248, 15.53676538602235269 ) ) ;
#22927=B_SPLINE_SURFACE_WITH_KNOTS ( 'NONE', 3, 1, ( 
 ( #25017, #34621 ),
 ( #64028, #25534 ),
 ( #27037, #56422 ),
 ( #80274, #40713 ),
 ( #86386, #88395 ),
 ( #94464, #87418 ),
 ( #72148, #49334 ),
 ( #33127, #55897 ),
 ( #95979, #9331 ),
 ( #86891, #65521 ),
 ( #42213, #17425 ),
 ( #47807, #95493 ),
 ( #71656, #10839 ),
 ( #48334, #40203 ),
 ( #33642, #11359 ),
 ( #71149, #26541 ),
 ( #94970, #79777 ),
 ( #17946, #48845 ),
 ( #18445, #10342 ),
 ( #41208, #32627 ),
 ( #49828, #57414 ),
 ( #1748, #2752 ),
 ( #64534, #26044 ),
 ( #56914, #87901 ),
 ( #80785, #5713 ),
 ( #12847, #13334 ),
 ( #35620, #28016 ),
 ( #97444, #73634 ),
 ( #35115, #89861 ),
 ( #96974, #75622 ),
 ( #66519, #51302 ),
 ( #81761, #4736 ),
 ( #43200, #12335 ),
 ( #83244, #59901 ) ),
 .UNSPECIFIED., .T., .F., .F.,
 ( 4, 2, 2, 2, 2, 2, 2, 2, 2, 2, 2, 2, 2, 2, 2, 2, 4 ),
 ( 2, 2 ),
 ( 0.000000000000000000, 0.06250000000000000000, 0.1250000000000000000, 0.1875000000000000000, 0.2500000000000000000, 0.3125000000000000000, 0.3750000000000000000, 0.4375000000000000000, 0.5000000000000000000, 0.5625000000000000000, 0.6250000000000000000, 0.6875000000000000000, 0.7500000000000000000, 0.8125000000000000000, 0.8750000000000000000, 0.9375000000000000000, 1.000000000000000000 ),
 ( 0.000000000000000000, 1.000000000000000000 ),
 .UNSPECIFIED. ) ;
#22930=CARTESIAN_POINT ( 'NONE',  ( 166.0261724905091114, 252.1720833225167837, -12.65714730546942768 ) ) ;
#22933=CARTESIAN_POINT ( 'NONE',  ( 182.1964890600146987, 262.8133727455790449, 12.68220177327409637 ) ) ;
#22934=CARTESIAN_POINT ( 'NONE',  ( 112.0100349375168918, 242.1427522451419065, -10.00000000000009415 ) ) ;
#22937=CARTESIAN_POINT ( 'NONE',  ( 163.1691520398773321, 248.0297337694385931, 11.21816141384514331 ) ) ;
#22939=CARTESIAN_POINT ( 'NONE',  ( 162.8223739550644211, 248.6303710312858186, -11.16939803179192658 ) ) ;
#22940=CARTESIAN_POINT ( 'NONE',  ( 17.63104780087548562, 190.1744531367911293, 4.594050593750047540 ) ) ;
#22942=CARTESIAN_POINT ( 'NONE',  ( 196.2011903101464441, 273.6939821814302150, 14.92212602658747223 ) ) ;
#22945=CARTESIAN_POINT ( 'NONE',  ( 174.7884235540875011, 286.3353386219461640, 10.46792632123525735 ) ) ;
#22946=CARTESIAN_POINT ( 'NONE',  ( 66.96803994030899787, 197.2202760586659736, -5.415160957724236172E-17 ) ) ;
#22947=CARTESIAN_POINT ( 'NONE',  ( 208.2939409893161553, 269.8713066281881083, 2.523744790997269227 ) ) ;
#22949=CARTESIAN_POINT ( 'NONE',  ( 51.02741275436270030, 200.2677522451418781, 10.00000000000009592 ) ) ;
#22951=( BOUNDED_CURVE ( )  B_SPLINE_CURVE ( 2, ( #69868, #480, #54656, #85632, #16177, #47073, #77990, #70888, #35365 ),
 .UNSPECIFIED., .F., .T. ) 
 B_SPLINE_CURVE_WITH_KNOTS ( ( 3, 2, 2, 2, 3 ),
 ( 0.3991935483870967527, 0.4005376344086021279, 0.4032258064516128782, 0.4059139784946236285, 0.4072580645161290591 ),
 .UNSPECIFIED. ) 
 CURVE ( )  GEOMETRIC_REPRESENTATION_ITEM ( )  RATIONAL_B_SPLINE_CURVE ( ( 0.9330127018922194093, 0.9330127018922194093, 1.000000000000000000, 0.8660254037844387076, 1.000000000000000000, 0.8660254037844387076, 1.000000000000000000, 0.9330127018922179660, 0.9330127018922194093 ) ) 
 REPRESENTATION_ITEM ( '' )  );
#22953=CARTESIAN_POINT ( 'NONE',  ( 15.68275096595825246, 169.8615022471901739, 5.000000000000051514 ) ) ;
#22954=CARTESIAN_POINT ( 'NONE',  ( 207.5195222358739784, 271.2126392554839640, 2.810970398613041432 ) ) ;
#22955=CARTESIAN_POINT ( 'NONE',  ( 136.6287848093373043, 243.5643266524160140, 9.188101187500095079 ) ) ;
#22957=CARTESIAN_POINT ( 'NONE',  ( 164.1341878931737313, 260.3349919959172780, -16.13799654372055059 ) ) ;
#22958=EDGE_CURVE ( 'NONE', #24776, #39107, #28822, .T. ) ;
#22959=CARTESIAN_POINT ( 'NONE',  ( 189.1600758314701238, 261.3976643428155171, 6.743524540470962947 ) ) ;
#22960=CARTESIAN_POINT ( 'NONE',  ( 193.8652130780152731, 280.5836658925297229, -17.72338988841175933 ) ) ;
#22962=CARTESIAN_POINT ( 'NONE',  ( 185.5475819381700546, 277.7404700938030260, -17.45495574986458109 ) ) ;
#22968=CARTESIAN_POINT ( 'NONE',  ( 156.5681255643642089, 279.9925795744871948, -5.322131134865745850 ) ) ;
#22971=CARTESIAN_POINT ( 'NONE',  ( 159.9921098401940469, 253.5325322770800653, 16.01215344049969502 ) ) ;
#22972=CARTESIAN_POINT ( 'NONE',  ( 168.1981980474926104, 282.0723965943072926, -10.92329350232336260 ) ) ;
#22974=CARTESIAN_POINT ( 'NONE',  ( 200.8654040100879854, 282.2982806454822367, -16.59380369206422756 ) ) ;
#22976=CARTESIAN_POINT ( 'NONE',  ( 149.7519917370995586, 271.6399139028688410, 11.58851940123675917 ) ) ;
#22977=CARTESIAN_POINT ( 'NONE',  ( 162.7459776558209228, 248.7626933030860812, -9.895605163646791880 ) ) ;
#22978=CARTESIAN_POINT ( 'NONE',  ( 153.1961624462112752, 265.3034584490234806, -16.19494717845262954 ) ) ;
#22979=ORIENTED_EDGE ( 'NONE', *, *, #53690, .T. ) ;
#22980=CARTESIAN_POINT ( 'NONE',  ( 191.1637967482625129, 281.0701639715127271, 16.65787912226990386 ) ) ;
#22982=ORIENTED_EDGE ( 'NONE', *, *, #3450, .F. ) ;
#22983=CARTESIAN_POINT ( 'NONE',  ( 149.3883679478359454, 271.8987519849911223, 12.99187507659642371 ) ) ;
#22987=CARTESIAN_POINT ( 'NONE',  ( 146.5913834600193582, 276.7432712258716947, -0.4909717733184599253 ) ) ;
#22989=CARTESIAN_POINT ( 'NONE',  ( 149.7109319212262051, 271.3400547943878109, -12.38605961032017433 ) ) ;
#22992=ORIENTED_EDGE ( 'NONE', *, *, #61020, .F. ) ;
#22993=CARTESIAN_POINT ( 'NONE',  ( 103.8820256808556906, 230.7833772461660544, -9.188101187500095079 ) ) ;
#22994=CARTESIAN_POINT ( 'NONE',  ( 161.1089126327036354, 251.5981730984191529, 13.95161017039218976 ) ) ;
#22995=CARTESIAN_POINT ( 'NONE',  ( 150.6931560952953646, 269.6387926204777727, 14.65021044537114037 ) ) ;
#22996=CARTESIAN_POINT ( 'NONE',  ( 142.2974213780761090, 241.4155109091895781, 2.679491924311254714 ) ) ;
#23003=VERTEX_POINT ( 'NONE', #48325 ) ;
#23004=CARTESIAN_POINT ( 'NONE',  ( 207.5195222358739784, 271.2126392554839640, 2.810970398613041432 ) ) ;
#23006=CARTESIAN_POINT ( 'NONE',  ( 170.8277526913387021, 283.1399606207687043, 11.93616677736253351 ) ) ;
#23007=CARTESIAN_POINT ( 'NONE',  ( 194.2154056360670040, 294.2560451561701029, -15.66696967429384557 ) ) ;
#23010=CARTESIAN_POINT ( 'NONE',  ( 164.9582166835089367, 246.4294246379055835, 1.883828838449762566 ) ) ;
#23017=CARTESIAN_POINT ( 'NONE',  ( 162.6476498368881494, 248.9330020812748785, 10.75824100428386743 ) ) ;
#23018=CARTESIAN_POINT ( 'NONE',  ( 184.9682936869809566, 258.1092236034054395, 2.986271678517576245 ) ) ;
#23021=CARTESIAN_POINT ( 'NONE',  ( 161.4025183475459073, 251.0896330829197041, 14.50747140106038735 ) ) ;
#23022=CARTESIAN_POINT ( 'NONE',  ( 158.0246744607735252, 281.0366367605934101, 2.042212327287092233 ) ) ;
#23023=VERTEX_POINT ( 'NONE', #24515 ) ;
#23024=CARTESIAN_POINT ( 'NONE',  ( 194.5803494922524806, 293.6239438553467380, -14.52903234192032222 ) ) ;
#23026=EDGE_CURVE ( 'NONE', #85510, #39184, #30077, .T. ) ;
#23027=CARTESIAN_POINT ( 'NONE',  ( 9.963374858250592325, 169.8927522451418213, 10.00000000000009592 ) ) ;
#23029=CARTESIAN_POINT ( 'NONE',  ( 169.9469112398214747, 250.9785751410766750, -8.718312767540300712 ) ) ;
#23030=CARTESIAN_POINT ( 'NONE',  ( 169.7647569238031338, 280.6421679560587563, -14.26277949995917638 ) ) ;
#23032=CARTESIAN_POINT ( 'NONE',  ( 0.9332558059805314832, 171.3458772461660544, 9.188101187500095079 ) ) ;
#23033=CARTESIAN_POINT ( 'NONE',  ( -0.9341114727036189391, 170.2677522451418781, 10.00000000000009592 ) ) ;
#23035=ORIENTED_EDGE ( 'NONE', *, *, #24461, .T. ) ;
#23036=CARTESIAN_POINT ( 'NONE',  ( 165.6218532904677829, 246.1078588663072253, -2.807711028975429013 ) ) ;
#23038=ADVANCED_FACE ( 'NONE', ( #26036 ), #57407, .T. ) ;
#23040=FACE_OUTER_BOUND ( 'NONE', #45422, .T. ) ;
#23041=CARTESIAN_POINT ( 'NONE',  ( 201.9751774886444480, 280.8157260523632317, -16.30213982533239303 ) ) ;
#23043=CARTESIAN_POINT ( 'NONE',  ( 149.7411355705484652, 277.2267774073285977, 3.080663611250638922 ) ) ;
#23044=CARTESIAN_POINT ( 'NONE',  ( 9.403806464923315289, 185.4244531367911293, -4.594050593750046652 ) ) ;
#23045=CARTESIAN_POINT ( 'NONE',  ( 122.2582625392304863, 232.2048013555409796, 4.594050593750051981 ) ) ;
#23046=CARTESIAN_POINT ( 'NONE',  ( 203.0026270830780675, 279.0361311525880978, -16.61345826058821373 ) ) ;
#23047=CARTESIAN_POINT ( 'NONE',  ( 178.9928779471620430, 291.8529855680378660, -6.150425450240065928 ) ) ;
#23048=CARTESIAN_POINT ( 'NONE',  ( 195.8954499045513558, 275.1620197951183400, 15.78109384089318823 ) ) ;
#23049=CARTESIAN_POINT ( 'NONE',  ( 26.05470188313195123, 197.3967562850347122, -4.648177544792955347E-16 ) ) ;
#23050=CARTESIAN_POINT ( 'NONE',  ( 177.2884455301937408, 283.4926669082274771, -15.35860094086973326 ) ) ;
#23052=CARTESIAN_POINT ( 'NONE',  ( -17.68663747114990770, 172.8464784336661353, 1.353441290958777327E-15 ) ) ;
#23053=CARTESIAN_POINT ( 'NONE',  ( 157.0848929289108469, 258.5679796760466047, 17.57466231005294688 ) ) ;
#23054=CARTESIAN_POINT ( 'NONE',  ( 155.6559071247401960, 261.0430556921643870, 17.79853447468815375 ) ) ;
#23055=FACE_OUTER_BOUND ( 'NONE', #4133, .T. ) ;
#23056=CARTESIAN_POINT ( 'NONE',  ( 190.1509686661389367, 284.8912016344419840, 17.04044544971958430 ) ) ;
#23059=AXIS2_PLACEMENT_3D ( 'NONE', #84331, #84824, #46260 ) ;
#23060=CARTESIAN_POINT ( 'NONE',  ( 189.2409861230456727, 262.5526351957132078, 8.112751438749265631 ) ) ;
#23061=CARTESIAN_POINT ( 'NONE',  ( 171.4203603884429299, 279.8539503503338324, 13.89678279489301360 ) ) ;
#23063=CARTESIAN_POINT ( 'NONE',  ( 191.1192699377806719, 299.6187094927299199, -9.526914969203620132 ) ) ;
#23064=CARTESIAN_POINT ( 'NONE',  ( 190.4281805785508084, 300.8157113754859893, -1.233909217199055774 ) ) ;
#23065=CARTESIAN_POINT ( 'NONE',  ( 181.2056177239550152, 266.0170940294115098, -15.02664418762704024 ) ) ;
#23067=CARTESIAN_POINT ( 'NONE',  ( 152.3064147080143584, 267.5489654531014594, -15.38666967861120050 ) ) ;
#23069=CARTESIAN_POINT ( 'NONE',  ( 188.2735287570237688, 299.1710073388255751, -5.251721556916531419 ) ) ;
#23070=CARTESIAN_POINT ( 'NONE',  ( 93.65192705076950119, 231.0024278399160949, -9.188101187500093303 ) ) ;
#23072=CARTESIAN_POINT ( 'NONE',  ( 191.5281967176683509, 298.9104275333885994, 7.715154960566919407 ) ) ;
#23077=CARTESIAN_POINT ( 'NONE',  ( 191.8998383512474106, 277.1803453812353837, 16.60231051853036277 ) ) ;
#23078=CARTESIAN_POINT ( 'NONE',  ( 149.1140077604129885, 272.3739577691819136, 12.91581545547286503 ) ) ;
#23079=CARTESIAN_POINT ( 'NONE',  ( 150.9115585710837877, 269.2605084359132093, -15.80434701481532578 ) ) ;
#23080=CARTESIAN_POINT ( 'NONE',  ( 146.5889662694323761, 243.8932355074535678, -2.679491924311248496 ) ) ;
#23082=CARTESIAN_POINT ( 'NONE',  ( 132.1371673402316844, 235.5494855054051868, -2.679491924311248496 ) ) ;
#23084=EDGE_LOOP ( 'NONE', ( #75246, #18935, #77702, #41532 ) ) ;
#23087=CARTESIAN_POINT ( 'NONE',  ( 200.3894610702548675, 269.4183277505318301, 8.919713072033628620 ) ) ;
#23088=CARTESIAN_POINT ( 'NONE',  ( 196.9728329903666122, 289.4800408803428695, -17.53478045286815856 ) ) ;
#23089=EDGE_CURVE ( 'NONE', #25756, #44273, #88118, .T. ) ;
#23090=EDGE_CURVE ( 'NONE', #85466, #26183, #89854, .T. ) ;
#23094=CARTESIAN_POINT ( 'NONE',  ( 183.4202745723773091, 264.5322101262771639, -13.24744625114140817 ) ) ;
#23095=CARTESIAN_POINT ( 'NONE',  ( 169.3369456435013944, 252.0587115110951117, -8.674031833049340889 ) ) ;
#23097=ORIENTED_EDGE ( 'NONE', *, *, #57438, .T. ) ;
#23098=CARTESIAN_POINT ( 'NONE',  ( 188.6533994728961829, 279.6148911687740224, 16.71976415023760509 ) ) ;
#23101=CARTESIAN_POINT ( 'NONE',  ( 179.8347084456439688, 290.9760905973820968, 10.83644005890302253 ) ) ;
#23105=LINE ( 'NONE', #53018, #10381 ) ;
#23106=CARTESIAN_POINT ( 'NONE',  ( 190.5525489982964302, 278.5900507645195034, -16.51546226578511423 ) ) ;
#23107=CARTESIAN_POINT ( 'NONE',  ( 153.5731768013688736, 264.6504504307081334, -18.06482034778880674 ) ) ;
#23108=CARTESIAN_POINT ( 'NONE',  ( 185.3081074539437907, 278.3520910533009101, 17.82413638460242922 ) ) ;
#23115=CARTESIAN_POINT ( 'NONE',  ( 197.8980529691977779, 285.8775128688180871, 17.80711829255526979 ) ) ;
#23118=CARTESIAN_POINT ( 'NONE',  ( 172.9269288353417835, 271.0868964859365633, 16.42719315256508850 ) ) ;
#23120=CARTESIAN_POINT ( 'NONE',  ( 190.0466317824856048, 300.2728036453518143, -3.352836199975675058 ) ) ;
#23122=CARTESIAN_POINT ( 'NONE',  ( 198.5444618742102705, 273.8348775512076259, -13.44695229262796055 ) ) ;
#23125=CARTESIAN_POINT ( 'NONE',  ( 171.4102349331081996, 250.9416128396940735, -5.608677351237023601 ) ) ;
#23127=CARTESIAN_POINT ( 'NONE',  ( 178.3260541269674775, 254.9471070209705204, 5.880822174413203207 ) ) ;
#23128=CARTESIAN_POINT ( 'NONE',  ( 112.9213393807382886, 229.8768266524160140, 9.188101187500098632 ) ) ;
#23139=CARTESIAN_POINT ( 'NONE',  ( 205.6812242890302400, 270.0455300709248831, -5.666524662691169389 ) ) ;
#23141=CARTESIAN_POINT ( 'NONE',  ( 200.9812045408918380, 282.5373376992193926, -16.61165062382494284 ) ) ;
#23146=CARTESIAN_POINT ( 'NONE',  ( 148.2352135776142177, 273.8960739431854563, -9.245976304249309052 ) ) ;
#23148=EDGE_LOOP ( 'NONE', ( #15611, #93801, #36585 ) ) ;
#23150=ADVANCED_FACE ( 'NONE', ( #5705 ), #305, .F. ) ;
#23152=CARTESIAN_POINT ( 'NONE',  ( 159.7079830814418244, 278.3650007144455003, 10.37211021382808696 ) ) ;
#23153=CARTESIAN_POINT ( 'NONE',  ( 192.4799288706118148, 262.6369605892642767, 4.631236763554750446 ) ) ;
#23154=CARTESIAN_POINT ( 'NONE',  ( 158.2231871454910959, 263.2639962149535791, 17.34092271714001399 ) ) ;
#23156=CARTESIAN_POINT ( 'NONE',  ( 184.2460973547030392, 288.7912027798610097, -14.42049990347707222 ) ) ;
#23157=CARTESIAN_POINT ( 'NONE',  ( 157.1201528510747210, 280.1329342086722249, 5.821162413553630621 ) ) ;
#23158=CARTESIAN_POINT ( 'NONE',  ( 153.1961624462112752, 265.3034584490234806, -16.19494717845262954 ) ) ;
#23160=CARTESIAN_POINT ( 'NONE',  ( 146.7845206192450007, 276.4087478532630939, 4.443586170796542945 ) ) ;
#23161=B_SPLINE_SURFACE_WITH_KNOTS ( 'NONE', 3, 1, ( 
 ( #25866, #17760 ),
 ( #10158, #80594 ),
 ( #72974, #3565 ),
 ( #72478, #50143 ),
 ( #63843, #34445 ),
 ( #89214, #65344 ),
 ( #81584, #41024 ),
 ( #34931, #57727 ),
 ( #88208, #81097 ),
 ( #73459, #4042 ),
 ( #94782, #19762 ),
 ( #71466, #2057 ),
 ( #25341, #33971 ),
 ( #2566, #56742 ),
 ( #87724, #18260 ),
 ( #10658, #3081 ),
 ( #51646, #59208 ),
 ( #37419, #12663 ),
 ( #73953, #68325 ),
 ( #74957, #13647 ),
 ( #59726, #4539 ),
 ( #60211, #90692 ),
 ( #99251, #43532 ),
 ( #35931, #6036 ),
 ( #29836, #5541 ),
 ( #74471, #12153 ),
 ( #52620, #44520 ),
 ( #53132, #60707 ),
 ( #29346, #21249 ),
 ( #36425, #5051 ),
 ( #91668, #22231 ),
 ( #67333, #52127 ),
 ( #66833, #51129 ),
 ( #67843, #43015 ) ),
 .UNSPECIFIED., .T., .F., .F.,
 ( 4, 2, 2, 2, 2, 2, 2, 2, 2, 2, 2, 2, 2, 2, 2, 2, 4 ),
 ( 2, 2 ),
 ( 0.000000000000000000, 0.06250000000000000000, 0.1250000000000000000, 0.1875000000000000000, 0.2500000000000000000, 0.3125000000000000000, 0.3750000000000000000, 0.4375000000000000000, 0.5000000000000000000, 0.5625000000000000000, 0.6250000000000000000, 0.6875000000000000000, 0.7500000000000000000, 0.8125000000000000000, 0.8750000000000000000, 0.9375000000000000000, 1.000000000000000000 ),
 ( 0.000000000000000000, 1.000000000000000000 ),
 .UNSPECIFIED. ) ;
#23163=CARTESIAN_POINT ( 'NONE',  ( 188.8764293144468240, 259.6972905960182061, 3.583694637520717041 ) ) ;
#23164=CARTESIAN_POINT ( 'NONE',  ( 182.4203110637134273, 275.0573665403885570, -17.01792947190426020 ) ) ;
#23165=CARTESIAN_POINT ( 'NONE',  ( 76.32488315910845245, 203.3262482093458061, 3.021315404115420679E-15 ) ) ;
#23166=CARTESIAN_POINT ( 'NONE',  ( 189.1711897435683909, 270.1262327773276297, -14.07582082338928053 ) ) ;
#23168=CARTESIAN_POINT ( 'NONE',  ( 163.8758338523056182, 285.7844739252391264, -2.579456967851244897 ) ) ;
#23169=EDGE_CURVE ( 'NONE', #13784, #13192, #33683, .T. ) ;
#23172=CARTESIAN_POINT ( 'NONE',  ( 188.4805308512120234, 298.0761574053781828, 7.892637567094712203 ) ) ;
#23174=CARTESIAN_POINT ( 'NONE',  ( 77.57650404090335883, 215.5958772461660544, -9.188101187500095079 ) ) ;
#23175=CARTESIAN_POINT ( 'NONE',  ( 36.46736065678477701, 181.8615022471902023, 5.000000000000051514 ) ) ;
#23176=FACE_OUTER_BOUND ( 'NONE', #64618, .T. ) ;
#23178=CARTESIAN_POINT ( 'NONE',  ( 154.8579861482817535, 262.4250953638155011, -17.69813260923097786 ) ) ;
#23179=CARTESIAN_POINT ( 'NONE',  ( 161.8408514536557163, 250.3304178724980318, -14.12919723462510646 ) ) ;
#23180=CARTESIAN_POINT ( 'NONE',  ( 202.8211298556536804, 279.3504935719197988, 17.07914446815911447 ) ) ;
#23181=CARTESIAN_POINT ( 'NONE',  ( 163.0019261236505486, 284.2031270801829805, 6.030241692761612704 ) ) ;
#23185=EDGE_CURVE ( 'NONE', #78092, #48457, #46608, .T. ) ;
#23186=CARTESIAN_POINT ( 'NONE',  ( 166.0702642583571844, 249.2115659832978167, -9.324519184667250826 ) ) ;
#23187=CARTESIAN_POINT ( 'NONE',  ( 163.9712156549718429, 246.6405188371923600, -4.902504724781694634 ) ) ;
#23188=CARTESIAN_POINT ( 'NONE',  ( 196.2255671652529259, 290.7743432561995860, 16.01325193769018185 ) ) ;
#23189=CARTESIAN_POINT ( 'NONE',  ( -6.130263895410211994, 157.2677522451417929, -5.000000000000041744 ) ) ;
#23191=CARTESIAN_POINT ( 'NONE',  ( 58.41569198217266035, 204.5333772461660544, 9.188101187500095079 ) ) ;
#23192=CARTESIAN_POINT ( 'NONE',  ( 163.8894951723502800, 247.1650863376556231, -6.266457964612296649 ) ) ;
#23194=EDGE_CURVE ( 'NONE', #81343, #39182, #95466, .T. ) ;
#23196=CARTESIAN_POINT ( 'NONE',  ( -12.03006195514386434, 173.8615022471903160, 5.000000000000046185 ) ) ;
#23198=B_SPLINE_CURVE_WITH_KNOTS ( 'NONE', 3,
 ( #93976, #47814, #78751, #9339 ),
 .UNSPECIFIED., .F., .F.,
 ( 4, 4 ),
 ( 0.005707261542966231803, 0.01134347631022532103 ),
 .UNSPECIFIED. ) ;
#23199=CARTESIAN_POINT ( 'NONE',  ( 15.88121511744419756, 186.6427522451419350, -10.00000000000009592 ) ) ;
#23201=CARTESIAN_POINT ( 'NONE',  ( 151.0013883899287066, 269.1049186256390726, -14.25461351222133466 ) ) ;
#23202=CARTESIAN_POINT ( 'NONE',  ( 196.6317700900902139, 290.0707791521982131, -17.91116578096951883 ) ) ;
#23204=CARTESIAN_POINT ( 'NONE',  ( 63.55789136502527015, 201.3768266524160140, 9.188101187500096856 ) ) ;
#23208=CARTESIAN_POINT ( 'NONE',  ( 198.0006249058153003, 287.6998530631771587, 18.31850453277666801 ) ) ;
#23209=DIRECTION ( 'NONE',  ( 0.8660254037844395958, 0.4999999999999985567, 0.000000000000000000 ) ) ;
#23210=CARTESIAN_POINT ( 'NONE',  ( 153.4632428020424300, 264.8408617030205505, 17.93840816349579015 ) ) ;
#23213=CARTESIAN_POINT ( 'NONE',  ( 117.4407359106297406, 238.6115022471902307, 10.00000000000009592 ) ) ;
#23214=CARTESIAN_POINT ( 'NONE',  ( 200.7523954295751594, 282.9336467052548869, 18.23634913067694185 ) ) ;
#23215=CARTESIAN_POINT ( 'NONE',  ( -27.42236680055714260, 166.5217562850347406, 1.224646799147364892E-15 ) ) ;
#23220=ORIENTED_EDGE ( 'NONE', *, *, #10456, .F. ) ;
#23221=CARTESIAN_POINT ( 'NONE',  ( 159.6962080797732710, 254.0450491601782232, -15.33973334987084947 ) ) ;
#23222=CARTESIAN_POINT ( 'NONE',  ( 189.6282054824295642, 278.2883837369565754, -16.50473759827790587 ) ) ;
#23223=FACE_OUTER_BOUND ( 'NONE', #78382, .T. ) ;
#23228=CARTESIAN_POINT ( 'NONE',  ( 148.0826818691893152, 274.1602666119424043, -9.371267383421741926 ) ) ;
#23235=VERTEX_POINT ( 'NONE', #42092 ) ;
#23236=CARTESIAN_POINT ( 'NONE',  ( 183.8754313647489198, 256.5225093191261294, -2.022205659181245174 ) ) ;
#23239=CARTESIAN_POINT ( 'NONE',  ( 174.5584865442874616, 286.5715570807610106, 11.73736338454468076 ) ) ;
#23244=CARTESIAN_POINT ( 'NONE',  ( 204.3371846825755824, 276.7246095846310823, 14.72513001683937262 ) ) ;
#23245=CARTESIAN_POINT ( 'NONE',  ( 188.1399729590822858, 294.5748838946434489, -10.97770313550398669 ) ) ;
#23246=CARTESIAN_POINT ( 'NONE',  ( 204.7237927799493775, 276.0549847173622879, -12.81020997223575364 ) ) ;
#23247=CARTESIAN_POINT ( 'NONE',  ( 136.0871718362070339, 255.5024278399161233, 9.188101187500095079 ) ) ;
#23248=CARTESIAN_POINT ( 'NONE',  ( 177.5089039944837452, 268.9213076647187677, 16.19086122322285348 ) ) ;
#23249=CARTESIAN_POINT ( 'NONE',  ( 179.2327624300868365, 257.7468971898826453, 10.15833653911241186 ) ) ;
#23250=CARTESIAN_POINT ( 'NONE',  ( 67.34640541081718368, 215.8149278399160949, -9.188101187500095079 ) ) ;
#23252=FACE_OUTER_BOUND ( 'NONE', #81274, .T. ) ;
#23254=CARTESIAN_POINT ( 'NONE',  ( 156.6812872898450735, 261.2670451491295012, 0.000000000000000000 ) ) ;
#23256=CARTESIAN_POINT ( 'NONE',  ( 195.5605487959511777, 291.9261888597969232, -15.74379588760244175 ) ) ;
#23257=VERTEX_POINT ( 'NONE', #12207 ) ;
#23259=CARTESIAN_POINT ( 'NONE',  ( 194.1833477612660204, 284.7236497737663399, 17.42380001248895027 ) ) ;
#23260=CARTESIAN_POINT ( 'NONE',  ( 146.7818291168261453, 276.4134096722012828, -0.7617065417431535534 ) ) ;
#23261=FACE_OUTER_BOUND ( 'NONE', #100152, .T. ) ;
#23262=CARTESIAN_POINT ( 'NONE',  ( 155.6276701977099890, 261.0919634844306643, 17.49722577287685255 ) ) ;
#23264=CARTESIAN_POINT ( 'NONE',  ( 72.19064823929512897, 221.6744531367911293, 4.594050593750047540 ) ) ;
#23266=VERTEX_POINT ( 'NONE', #26906 ) ;
#23267=CARTESIAN_POINT ( 'NONE',  ( 200.3487535410712610, 283.6327749642065896, -17.20506751786975030 ) ) ;
#23273=CARTESIAN_POINT ( 'NONE',  ( 205.9240884482826175, 273.9760116357041966, 10.27504561427317142 ) ) ;
#23274=CARTESIAN_POINT ( 'NONE',  ( 160.4962995477943650, 275.9333967852908813, 14.18032076246626794 ) ) ;
#23276=CARTESIAN_POINT ( 'NONE',  ( 162.6191010640297065, 261.4165189579067032, 16.98501175862150347 ) ) ;
#23278=CARTESIAN_POINT ( 'NONE',  ( 188.6595133177037269, 294.9934435437166371, 11.67654844209925891 ) ) ;
#23279=CARTESIAN_POINT ( 'NONE',  ( 185.5760615167922367, 259.8211877333729376, 5.844598467702574851 ) ) ;
#23281=CARTESIAN_POINT ( 'NONE',  ( 152.6621968174709991, 266.2283140474973493, -17.02835521334403168 ) ) ;
#23284=ADVANCED_FACE ( 'NONE', ( #52553 ), #31029, .F. ) ;
#23289=CARTESIAN_POINT ( 'NONE',  ( -22.42236680055709641, 157.8615022471902591, 0.000000000000000000 ) ) ;
#23291=CARTESIAN_POINT ( 'NONE',  ( 186.3860696682239677, 265.1981530971773964, -11.87193015803705087 ) ) ;
#23293=CARTESIAN_POINT ( 'NONE',  ( 156.7306434729829903, 272.3907090408932845, 14.28438741009544977 ) ) ;
#23294=ORIENTED_EDGE ( 'NONE', *, *, #50025, .F. ) ;
#23299=CARTESIAN_POINT ( 'NONE',  ( 155.4216552449402684, 261.4487918497463284, 18.51722274565528892 ) ) ;
#23301=CARTESIAN_POINT ( 'NONE',  ( 176.2109476536867589, 285.4385534205517843, -12.05244463992889514 ) ) ;
#23303=CARTESIAN_POINT ( 'NONE',  ( 190.0550686570564949, 301.4619601804237732, 4.203010638620038542 ) ) ;
#23304=CARTESIAN_POINT ( 'NONE',  ( 164.0717493910576650, 284.1959068738492533, -3.117773458651499574 ) ) ;
#23305=CARTESIAN_POINT ( 'NONE',  ( 133.4825598088814047, 236.3262482093457493, 3.021315404115420679E-15 ) ) ;
#23306=CARTESIAN_POINT ( 'NONE',  ( 191.8140490939860285, 262.3104730638163460, 2.949596223079247626 ) ) ;
#23308=CARTESIAN_POINT ( 'NONE',  ( -4.289699588770600869, 159.1423013555410080, -4.594050593750043987 ) ) ;
#23310=ORIENTED_EDGE ( 'NONE', *, *, #66566, .F. ) ;
#23311=CYLINDRICAL_SURFACE ( 'NONE', #45977, 17.82106496071139645 ) ;
#23314=CARTESIAN_POINT ( 'NONE',  ( 138.6787122315880083, 239.3262482093457493, 3.021315404115420679E-15 ) ) ;
#23316=CARTESIAN_POINT ( 'NONE',  ( 32.86828966629671811, 177.5327760586659736, 1.948934522072302763E-15 ) ) ;
#23320=CARTESIAN_POINT ( 'NONE',  ( 170.4337869423260372, 270.9453688967402059, -17.51992477341579146 ) ) ;
#23321=CARTESIAN_POINT ( 'NONE',  ( 9.620573139467140322, 176.3615022471902307, -10.00000000000009592 ) ) ;
#23323=CARTESIAN_POINT ( 'NONE',  ( 178.9036571371011632, 255.1432592131925787, -3.948543175344032541 ) ) ;
#23324=CARTESIAN_POINT ( 'NONE',  ( 162.6991225460172927, 284.8212170328912975, -3.897741803361528756 ) ) ;
#23325=B_SPLINE_CURVE_WITH_KNOTS ( 'NONE', 3,
 ( #9277, #40150, #1690, #45750 ),
 .UNSPECIFIED., .F., .F.,
 ( 4, 4 ),
 ( 0.03903437031820212316, 0.04753079826317264944 ),
 .UNSPECIFIED. ) ;
#23326=CARTESIAN_POINT ( 'NONE',  ( 74.57247842330004062, 213.8615022471902591, -10.00000000000009592 ) ) ;
#23328=CARTESIAN_POINT ( 'NONE',  ( 203.3837935586101935, 270.0850993924222507, 6.058045230343306109 ) ) ;
#23329=CARTESIAN_POINT ( 'NONE',  ( 22.50244069716294959, 192.9869531367911293, 4.594050593750046652 ) ) ;
#23332=CARTESIAN_POINT ( 'NONE',  ( 198.8157103782086210, 286.2880836124806478, -18.60729372713428020 ) ) ;
#23333=CARTESIAN_POINT ( 'NONE',  ( 164.3138894970802824, 246.0469903322357368, -2.642126690130961020 ) ) ;
#23334=CARTESIAN_POINT ( 'NONE',  ( 155.4186054393023255, 261.4540742680644598, 17.05753227160644769 ) ) ;
#23335=CARTESIAN_POINT ( 'NONE',  ( 179.8888715531147682, 274.4711782159853328, -17.82026667163308531 ) ) ;
#23336=CARTESIAN_POINT ( 'NONE',  ( 159.8982049494451019, 278.5378777402860919, -9.810204408616700178 ) ) ;
#23337=CARTESIAN_POINT ( 'NONE',  ( 156.7442704525034571, 261.1579551113846378, 17.82061976529222846 ) ) ;
#23342=CARTESIAN_POINT ( 'NONE',  ( 186.2747035149648696, 267.7638619178059685, -15.07880563748316227 ) ) ;
#23343=ORIENTED_EDGE ( 'NONE', *, *, #79542, .T. ) ;
#23344=CARTESIAN_POINT ( 'NONE',  ( 165.0528804069804494, 264.4852527057752241, -17.76608744198970768 ) ) ;
#23352=CARTESIAN_POINT ( 'NONE',  ( 174.5432515410337544, 282.4104588529930311, -15.15290805577315680 ) ) ;
#23353=STYLED_ITEM('',(#100338),#45023);
#23354=EDGE_CURVE ( 'NONE', #29582, #35319, #68829, .T. ) ;
#23356=DIRECTION ( 'NONE',  ( -0.8660254037844387076, -0.4999999999999998890, -0.000000000000000000 ) ) ;
#23358=CARTESIAN_POINT ( 'NONE',  ( 153.3859906278383676, 264.9746663937372091, -17.41799046551451013 ) ) ;
#23364=CARTESIAN_POINT ( 'NONE',  ( 190.3691966041315311, 300.9178746160123410, 0.1783449565851275009 ) ) ;
#23366=CARTESIAN_POINT ( 'NONE',  ( 149.0598351764325002, 272.4677874370131576, -11.59078276432863674 ) ) ;
#23368=CARTESIAN_POINT ( 'NONE',  ( 174.9148042186883174, 263.6164057622452219, -16.35743113487313138 ) ) ;
#23370=ORIENTED_EDGE ( 'NONE', *, *, #44772, .T. ) ;
#23372=CARTESIAN_POINT ( 'NONE',  ( 148.9517569034208009, 272.6549844970639924, 12.50737104496728236 ) ) ;
#23376=CARTESIAN_POINT ( 'NONE',  ( 159.5956778034477281, 255.1851156857001115, 15.94425648350737745 ) ) ;
#23380=VERTEX_POINT ( 'NONE', #17051 ) ;
#23382=CARTESIAN_POINT ( 'NONE',  ( 77.00817486789590305, 205.2677522451417929, -5.000000000000041744 ) ) ;
#23383=CARTESIAN_POINT ( 'NONE',  ( 190.0515794655415789, 301.4680036374047063, -1.296825456579539626 ) ) ;
#23385=CARTESIAN_POINT ( 'NONE',  ( 190.0445576990143195, 301.4801656937889902, 4.140328216824785912 ) ) ;
#23386=CARTESIAN_POINT ( 'NONE',  ( 171.0076562725379858, 275.6637320423262736, -16.75718656872113499 ) ) ;
#23387=CARTESIAN_POINT ( 'NONE',  ( 146.5086121934486982, 276.8866352649785654, -0.04230388357226919777 ) ) ;
#23388=CARTESIAN_POINT ( 'NONE',  ( 193.1028332910263998, 296.1830769848763225, -12.04975758233223893 ) ) ;
#23389=CARTESIAN_POINT ( 'NONE',  ( 190.0259678364800493, 301.5123642802043946, 4.004183174499006626 ) ) ;
#23391=CARTESIAN_POINT ( 'NONE',  ( 96.99346744615054661, 215.2592609112380160, 2.679491924311254714 ) ) ;
#23393=CARTESIAN_POINT ( 'NONE',  ( 154.5219726700536569, 264.1077093662300399, -17.00691965702323216 ) ) ;
#23395=CARTESIAN_POINT ( 'NONE',  ( 108.1307024963493149, 242.4244531367911293, -4.594050593750046652 ) ) ;
#23396=ORIENTED_EDGE ( 'NONE', *, *, #87559, .F. ) ;
#23397=CARTESIAN_POINT ( 'NONE',  ( 191.8329718516215223, 298.3825415164982928, -8.871589506312979267 ) ) ;
#23400=CARTESIAN_POINT ( 'NONE',  ( 203.2187760522547819, 278.6617501559703101, -15.08675642319914978 ) ) ;
#23402=CARTESIAN_POINT ( 'NONE',  ( 190.9889137617930714, 298.2006275540064735, -9.555045851526354994 ) ) ;
#23403=EDGE_CURVE ( 'NONE', #4764, #61618, #48205, .T. ) ;
#23405=CARTESIAN_POINT ( 'NONE',  ( 165.8799236907572379, 283.6072792123424620, -8.180192921770395031 ) ) ;
#23407=CARTESIAN_POINT ( 'NONE',  ( 163.2000388741132895, 247.9762362032568035, -11.19676374274550312 ) ) ;
#23410=CARTESIAN_POINT ( 'NONE',  ( 51.53259423990365917, 193.8927522451418213, 10.00000000000009592 ) ) ;
#23411=CARTESIAN_POINT ( 'NONE',  ( 135.6816562978893330, 239.9548013555409796, -4.594050593750042211 ) ) ;
#23412=CARTESIAN_POINT ( 'NONE',  ( 150.8168331730346949, 269.4245776381016526, -15.71017957295074652 ) ) ;
#23413=CARTESIAN_POINT ( 'NONE',  ( 168.8785100482814698, 272.6966330010931756, 17.41127854651366391 ) ) ;
#23416=CARTESIAN_POINT ( 'NONE',  ( 52.11020483269097525, 191.7048013555409796, 4.594050593750051981 ) ) ;
#23418=ORIENTED_EDGE ( 'NONE', *, *, #46881, .T. ) ;
#23422=CARTESIAN_POINT ( 'NONE',  ( 190.9586609929293104, 299.8968923453624598, -4.970176667899034229 ) ) ;
#23426=CARTESIAN_POINT ( 'NONE',  ( 178.5107126437189038, 260.9283949996104752, 13.53338759835929395 ) ) ;
#23428=CARTESIAN_POINT ( 'NONE',  ( 105.5870131927823081, 241.7677522451419065, -5.000000000000047962 ) ) ;
#23433=CARTESIAN_POINT ( 'NONE',  ( 147.9710862514405960, 274.3535558917855042, 7.785500222159708272 ) ) ;
#23435=CARTESIAN_POINT ( 'NONE',  ( 25.77753312492912841, 179.5643266524160140, -9.188101187500093303 ) ) ;
#23440=CARTESIAN_POINT ( 'NONE',  ( 194.8648160861291103, 275.0048917464952183, -16.07792121436337851 ) ) ;
#23441=CARTESIAN_POINT ( 'NONE',  ( 61.01376819352597636, 206.0333772461660544, 9.188101187500095079 ) ) ;
#23442=CARTESIAN_POINT ( 'NONE',  ( 200.1782072557437857, 283.9281697954355650, 18.05177561285849208 ) ) ;
#23446=ORIENTED_EDGE ( 'NONE', *, *, #16924, .F. ) ;
#23447=CARTESIAN_POINT ( 'NONE',  ( 26.94108121515588294, 196.3615022471903160, 5.000000000000046185 ) ) ;
#23448=CARTESIAN_POINT ( 'NONE',  ( 208.0045976720423084, 270.3724639545367836, 2.002128742561712471 ) ) ;
#23449=CARTESIAN_POINT ( 'NONE',  ( 143.0153750664825054, 259.5024278399160949, -9.188101187500093303 ) ) ;
#23451=CARTESIAN_POINT ( 'NONE',  ( 189.1724466617436349, 261.8427108266350274, 6.584756579409549282 ) ) ;
#23452=CARTESIAN_POINT ( 'NONE',  ( 205.8610808625997208, 274.0851439753691920, 10.38803237360972531 ) ) ;
#23453=CARTESIAN_POINT ( 'NONE',  ( 202.5128468779458331, 267.1751508879428343, 0.8823122286173835649 ) ) ;
#23455=VERTEX_POINT ( 'NONE', #25673 ) ;
#23456=CARTESIAN_POINT ( 'NONE',  ( 166.8533131785278272, 247.0304541540030243, 3.784327470570368224 ) ) ;
#23457=DIRECTION ( 'NONE',  ( 1.000000000000000000, 0.000000000000000000, 0.000000000000000000 ) ) ;
#23458=EDGE_CURVE ( 'NONE', #33315, #98890, #31335, .T. ) ;
#23459=CARTESIAN_POINT ( 'NONE',  ( 178.1412175327710656, 285.9644113652241231, 12.86296424501218461 ) ) ;
#23462=VERTEX_POINT ( 'NONE', #9974 ) ;
#23465=DIRECTION ( 'NONE',  ( 0.5000000000000048850, -0.8660254037844358210, 0.000000000000000000 ) ) ;
#23466=CARTESIAN_POINT ( 'NONE',  ( 192.0332533962074706, 298.0356437054567778, 11.70630383928353346 ) ) ;
#23468=CARTESIAN_POINT ( 'NONE',  ( 181.4283053378885597, 267.7238133557910373, 16.48022347432943135 ) ) ;
#23469=CARTESIAN_POINT ( 'NONE',  ( 208.3194307158603067, 269.8271571267425770, -2.120200867047394855 ) ) ;
#23473=CARTESIAN_POINT ( 'NONE',  ( 190.7633961518363890, 281.0789110243076721, 16.67417094886322460 ) ) ;
#23474=CARTESIAN_POINT ( 'NONE',  ( 171.6334153394907389, 249.3410379734025923, 0.9431220288450494760 ) ) ;
#23478=ORIENTED_EDGE ( 'NONE', *, *, #87220, .F. ) ;
#23479=CARTESIAN_POINT ( 'NONE',  ( 146.8637854207107409, 276.2714571898724216, 0.7988785540157756770 ) ) ;
#23481=DIRECTION ( 'NONE',  ( -0.8660254037844387076, -0.4999999999999998890, -0.000000000000000000 ) ) ;
#23484=ORIENTED_EDGE ( 'NONE', *, *, #90641, .F. ) ;
#23485=CARTESIAN_POINT ( 'NONE',  ( 161.3193951073452581, 251.2336067582368742, 13.01220207292984377 ) ) ;
#23486=CARTESIAN_POINT ( 'NONE',  ( 136.1324508756439400, 242.7365022471902307, 10.00000000000009948 ) ) ;
#23487=CARTESIAN_POINT ( 'NONE',  ( 191.5694459269389824, 298.8389818071599962, 7.944420692511652504 ) ) ;
#23491=ORIENTED_EDGE ( 'NONE', *, *, #62695, .F. ) ;
#23495=DIRECTION ( 'NONE',  ( -0.8660254037844387076, -0.4999999999999998890, -0.000000000000000000 ) ) ;
#23497=CARTESIAN_POINT ( 'NONE',  ( 207.6932907333322191, 270.9116633891313199, 2.120963121341169710 ) ) ;
#23499=CARTESIAN_POINT ( 'NONE',  ( 167.0456650196674673, 282.1831978616474998, 12.11327121657329542 ) ) ;
#23500=CARTESIAN_POINT ( 'NONE',  ( 147.9791529310278122, 274.3395839928920168, -7.789432462804474433 ) ) ;
#23502=CARTESIAN_POINT ( 'NONE',  ( -22.42236680055709641, 157.8615022471902591, 0.000000000000000000 ) ) ;
#23504=CARTESIAN_POINT ( 'NONE',  ( 166.0832898494950030, 246.9231440688584769, 1.898682735395063714 ) ) ;
#23506=CARTESIAN_POINT ( 'NONE',  ( 198.4136990093444126, 277.2144854508601384, -15.28644943941467993 ) ) ;
#23508=CARTESIAN_POINT ( 'NONE',  ( 206.9275546910526486, 270.9267086679434442, 4.961599381757848981 ) ) ;
#23510=CARTESIAN_POINT ( 'NONE',  ( 147.0294190956623481, 275.9845712494116583, -4.172428427132245154 ) ) ;
#23512=CARTESIAN_POINT ( 'NONE',  ( 206.6912923161529818, 272.6471755567893638, -9.325620632947922317 ) ) ;
#23513=CARTESIAN_POINT ( 'NONE',  ( 165.5694811585547654, 246.8511483137207563, -2.318198762934976731 ) ) ;
#23514=EDGE_CURVE ( 'NONE', #6423, #48869, #49462, .T. ) ;
#23516=CARTESIAN_POINT ( 'NONE',  ( 172.0057192551458343, 254.5726738447181106, 11.30606058533757796 ) ) ;
#23518=CARTESIAN_POINT ( 'NONE',  ( 194.8319568529400385, 263.3227001520926933, -0.7902351138979081258 ) ) ;
#23521=CARTESIAN_POINT ( 'NONE',  ( 194.2565597998853377, 294.1847640534938364, -14.09590134157931374 ) ) ;
#23524=EDGE_CURVE ( 'NONE', #79763, #21882, #90612, .T. ) ;
#23525=CARTESIAN_POINT ( 'NONE',  ( 5.488910272030937065, 180.6427522451419350, -10.00000000000009415 ) ) ;
#23526=CARTESIAN_POINT ( 'NONE',  ( 83.31357524521028779, 231.1589784336661353, -6.496448406907676862E-16 ) ) ;
#23527=CARTESIAN_POINT ( 'NONE',  ( 196.1279896863303520, 269.6123170192805105, -10.99537109092639220 ) ) ;
#23528=CARTESIAN_POINT ( 'NONE',  ( 164.4568492923521887, 247.7993767033852919, 8.703614106482779889 ) ) ;
#23530=CARTESIAN_POINT ( 'NONE',  ( 8.375921941576814689, 166.4548013555410080, -4.594050593750042211 ) ) ;
#23532=CARTESIAN_POINT ( 'NONE',  ( 161.7910648966377209, 250.4166507187868831, 13.19274492748169436 ) ) ;
#23533=VERTEX_POINT ( 'NONE', #67145 ) ;
#23535=CARTESIAN_POINT ( 'NONE',  ( 197.5258556021618688, 265.2381013607024443, -2.939624273662967635 ) ) ;
#23536=( BOUNDED_CURVE ( )  B_SPLINE_CURVE ( 2, ( #94276, #95299, #24831, #86694, #71456, #87716, #95794, #26348, #57224 ),
 .UNSPECIFIED., .F., .T. ) 
 B_SPLINE_CURVE_WITH_KNOTS ( ( 3, 2, 2, 2, 3 ),
 ( 0.6250000000000000000, 0.6263440860215053752, 0.6290322580645161255, 0.6317204301075268758, 0.6330645161290322509 ),
 .UNSPECIFIED. ) 
 CURVE ( )  GEOMETRIC_REPRESENTATION_ITEM ( )  RATIONAL_B_SPLINE_CURVE ( ( 0.9330127018922194093, 0.9330127018922194093, 1.000000000000000000, 0.8660254037844387076, 1.000000000000000000, 0.8660254037844387076, 1.000000000000000000, 0.9330127018922194093, 0.9330127018922194093 ) ) 
 REPRESENTATION_ITEM ( '' )  );
#23537=CARTESIAN_POINT ( 'NONE',  ( 112.6979501180548766, 224.3262482093457777, 3.021315404115420679E-15 ) ) ;
#23539=CARTESIAN_POINT ( 'NONE',  ( 163.8835510476618254, 277.4261113242017132, -14.47671527678674330 ) ) ;
#23542=B_SPLINE_CURVE_WITH_KNOTS ( 'NONE', 3,
 ( #78916, #47970, #26688, #80438 ),
 .UNSPECIFIED., .F., .F.,
 ( 4, 4 ),
 ( 0.008386952484578737849, 0.01475959061312598006 ),
 .UNSPECIFIED. ) ;
#23543=CARTESIAN_POINT ( 'NONE',  ( 35.30381256655795852, 185.0643266524160140, 9.188101187500095079 ) ) ;
#23544=CARTESIAN_POINT ( 'NONE',  ( 119.6866422041566693, 252.1589784336661637, -6.496448406907675876E-16 ) ) ;
#23545=CARTESIAN_POINT ( 'NONE',  ( 199.3879857545408640, 277.4998007522424359, 15.19030560797578389 ) ) ;
#23546=ORIENTED_EDGE ( 'NONE', *, *, #53148, .F. ) ;
#23547=CARTESIAN_POINT ( 'NONE',  ( 153.2461334198073075, 273.7581969524157444, -11.86170745181470387 ) ) ;
#23550=CARTESIAN_POINT ( 'NONE',  ( 194.3562588153086779, 294.0120802933159325, 14.11474987148825200 ) ) ;
#23551=CARTESIAN_POINT ( 'NONE',  ( 184.5123196318015459, 277.1383014161853566, -17.82024832176989904 ) ) ;
#23554=CARTESIAN_POINT ( 'NONE',  ( 194.2223991963907963, 294.2439319543634610, -14.97294938100067441 ) ) ;
#23556=CARTESIAN_POINT ( 'NONE',  ( 163.2645943797325572, 249.2862317762373436, -10.33311602661124518 ) ) ;
#23557=CYLINDRICAL_SURFACE ( 'NONE', #5456, 10.00000000000010658 ) ;
#23559=LINE ( 'NONE', #31659, #58179 ) ;
#23564=CARTESIAN_POINT ( 'NONE',  ( 182.1962218731464134, 268.3183306110546482, 15.02138923653300218 ) ) ;
#23565=CARTESIAN_POINT ( 'NONE',  ( 121.5276403787286483, 228.7202760586659736, -5.415160957724236172E-17 ) ) ;
#23567=ORIENTED_EDGE ( 'NONE', *, *, #20031, .F. ) ;
#23568=CARTESIAN_POINT ( 'NONE',  ( 150.6655900823359389, 269.6865383554857090, 15.31288044136207205 ) ) ;
#23570=CARTESIAN_POINT ( 'NONE',  ( 195.6627736265002682, 278.3332898145053491, 16.90917068752747809 ) ) ;
#23571=CARTESIAN_POINT ( 'NONE',  ( 150.7162572431468561, 269.5987802586857924, -13.73098793484843405 ) ) ;
#23573=CARTESIAN_POINT ( 'NONE',  ( 150.7691137448031213, 269.5072301123068428, -15.63821625702598084 ) ) ;
#23576=CARTESIAN_POINT ( 'NONE',  ( 175.0296968597178306, 264.6864531019056699, -16.70299667166197466 ) ) ;
#23577=CARTESIAN_POINT ( 'NONE',  ( 146.9422184197532317, 276.1356072505412840, -5.063317562214876943 ) ) ;
#23579=ORIENTED_EDGE ( 'NONE', *, *, #52802, .F. ) ;
#23580=CARTESIAN_POINT ( 'NONE',  ( 164.3645038749433525, 256.7011479335206445, -14.91022226314676402 ) ) ;
#23581=DIRECTION ( 'NONE',  ( -0.8660254037844357100, -0.5000000000000049960, -0.000000000000000000 ) ) ;
#23583=CARTESIAN_POINT ( 'NONE',  ( 196.9976074755333286, 289.4371302133026802, -16.79549473444794216 ) ) ;
#23586=CARTESIAN_POINT ( 'NONE',  ( 180.1160312531098668, 262.9874791413300272, -12.84058704759554992 ) ) ;
#23587=EDGE_CURVE ( 'NONE', #58638, #23003, #66650, .T. ) ;
#23590=LINE ( 'NONE', #45885, #19393 ) ;
#23594=VERTEX_POINT ( 'NONE', #98067 ) ;
#23595=CARTESIAN_POINT ( 'NONE',  ( 167.5863728346707830, 249.8758218121444656, 6.940154622966127285 ) ) ;
#23596=EDGE_CURVE ( 'NONE', #28763, #15906, #51953, .T. ) ;
#23597=LINE ( 'NONE', #47405, #51537 ) ;
#23600=CARTESIAN_POINT ( 'NONE',  ( 205.9050707304272407, 274.0089512892737389, 12.32231322111777772 ) ) ;
#23601=CARTESIAN_POINT ( 'NONE',  ( 192.5381442786905666, 297.1611470447178363, -13.11433798472783074 ) ) ;
#23604=CARTESIAN_POINT ( 'NONE',  ( 119.0825757350898755, 232.8927522451418213, 10.00000000000009948 ) ) ;
#23607=CARTESIAN_POINT ( 'NONE',  ( 195.7233648222712930, 290.9602864498907593, 16.00646756461187437 ) ) ;
#23614=CARTESIAN_POINT ( 'NONE',  ( 165.4869498693733760, 275.0640536683063146, -15.87538405248356810 ) ) ;
#23616=CARTESIAN_POINT ( 'NONE',  ( 190.1364579050488430, 301.3209898677110345, 2.002245206357507357 ) ) ;
#23618=CARTESIAN_POINT ( 'NONE',  ( 192.7705129102570822, 296.7586727687594816, -13.39629674907774692 ) ) ;
#23619=CARTESIAN_POINT ( 'NONE',  ( 167.7877716316831425, 248.9074273214486368, -5.048719896133492036 ) ) ;
#23621=CARTESIAN_POINT ( 'NONE',  ( 183.5171238009618264, 284.3872251382956620, -15.26397248544439122 ) ) ;
#23622=CARTESIAN_POINT ( 'NONE',  ( 124.3418758452630613, 242.5958772461660544, -9.188101187500095079 ) ) ;
#23624=CARTESIAN_POINT ( 'NONE',  ( 160.1642720190261855, 283.6550828934768447, 2.228402901662201341 ) ) ;
#23625=CARTESIAN_POINT ( 'NONE',  ( 180.4686939987674918, 291.6062955413669329, -9.874166343425045511 ) ) ;
#23626=ORIENTED_EDGE ( 'NONE', *, *, #30863, .F. ) ;
#23631=CARTESIAN_POINT ( 'NONE',  ( 175.8027662909930484, 284.8719843250962072, 14.11304877541382119 ) ) ;
#23632=CARTESIAN_POINT ( 'NONE',  ( 174.1370939159656643, 290.5918216138747425, -4.894811010708814081 ) ) ;
#23635=CARTESIAN_POINT ( 'NONE',  ( 200.9445292274600092, 282.6008612054670266, -16.62830946367346741 ) ) ;
#23637=ORIENTED_EDGE ( 'NONE', *, *, #46067, .T. ) ;
#23639=CARTESIAN_POINT ( 'NONE',  ( 148.0129410789982103, 274.2810612039135094, 10.14596848016967279 ) ) ;
#23640=CARTESIAN_POINT ( 'NONE',  ( 174.0965047066266038, 253.2374073076369427, -7.700682943850493345 ) ) ;
#23642=FACE_OUTER_BOUND ( 'NONE', #23084, .T. ) ;
#23646=CARTESIAN_POINT ( 'NONE',  ( 188.4786970353986248, 265.2655723350032986, -11.77073285016548354 ) ) ;
#23648=CARTESIAN_POINT ( 'NONE',  ( 194.4506751305639796, 264.6470882917897711, 4.421188665544642404 ) ) ;
#23649=CARTESIAN_POINT ( 'NONE',  ( 149.6896757981861583, 271.3768714794653647, 12.49809796062302603 ) ) ;
#23650=CARTESIAN_POINT ( 'NONE',  ( 8.086986483384254853, 182.1427522451419350, -10.00000000000009592 ) ) ;
#23651=CARTESIAN_POINT ( 'NONE',  ( 164.2700632124239633, 284.1926600866962644, -7.004898476152563447 ) ) ;
#23652=FACE_OUTER_BOUND ( 'NONE', #31248, .T. ) ;
#23653=DIRECTION ( 'NONE',  ( 0.4999999999999998890, -0.8660254037844385966, 0.000000000000000000 ) ) ;
#23655=CARTESIAN_POINT ( 'NONE',  ( 147.3984236761635884, 275.3454365677582700, 5.108566646342994844 ) ) ;
#23657=CARTESIAN_POINT ( 'NONE',  ( 186.7529496275546421, 262.6979624853421456, -8.915494530226171221 ) ) ;
#23659=DIRECTION ( 'NONE',  ( 0.4999999999999992784, -0.8660254037844390407, 0.000000000000000000 ) ) ;
#23660=CARTESIAN_POINT ( 'NONE',  ( 186.0996347449242307, 297.2146404166695675, -4.282800944430866785 ) ) ;
#23661=CARTESIAN_POINT ( 'NONE',  ( 152.9920137376499838, 265.6570543845515431, 16.15798175643282164 ) ) ;
#23662=CARTESIAN_POINT ( 'NONE',  ( 37.60401899570393880, 182.5177522451417929, 5.000000000000051514 ) ) ;
#23663=CARTESIAN_POINT ( 'NONE',  ( 193.9844289374573520, 294.6561085335266625, 15.49818881749970245 ) ) ;
#23664=CARTESIAN_POINT ( 'NONE',  ( 191.4011393215214412, 282.8345302558525987, -17.71497175083820608 ) ) ;
#23666=CARTESIAN_POINT ( 'NONE',  ( 69.78227540684341079, 211.0958772461660544, -9.188101187500095079 ) ) ;
#23667=CARTESIAN_POINT ( 'NONE',  ( 178.6317619811870259, 253.9327355832967612, -4.167451725846189170 ) ) ;
#23668=CARTESIAN_POINT ( 'NONE',  ( 147.5118896528469179, 275.1489077312122049, -3.975523961781759930 ) ) ;
#23669=CARTESIAN_POINT ( 'NONE',  ( 58.19016453504443831, 197.7365022471902307, 10.00000000000009948 ) ) ;
#23670=CARTESIAN_POINT ( 'NONE',  ( 202.7973612924478743, 279.3916619310153919, -15.54732529288344089 ) ) ;
#23679=CARTESIAN_POINT ( 'NONE',  ( -0.3647194387874375665, 159.0494855054051868, -2.679491924311248496 ) ) ;
#23680=CARTESIAN_POINT ( 'NONE',  ( 164.6737691338994978, 245.4236605166554739, -4.507742726242741860 ) ) ;
#23681=CARTESIAN_POINT ( 'NONE',  ( 195.9920715006079490, 291.1787696107118677, 15.99608784761372071 ) ) ;
#23683=CARTESIAN_POINT ( 'NONE',  ( 159.9040744856012850, 255.4269131533854420, 16.38690128260775936 ) ) ;
#23684=CARTESIAN_POINT ( 'NONE',  ( 43.58535403812915376, 183.7202760586659736, -5.415160957724236172E-17 ) ) ;
#23685=CARTESIAN_POINT ( 'NONE',  ( 58.14488549560751807, 210.5024278399160949, 9.188101187500095079 ) ) ;
#23686=CARTESIAN_POINT ( 'NONE',  ( 192.4619825937016060, 278.6107209869106214, -17.59187769095188969 ) ) ;
#23689=CARTESIAN_POINT ( 'NONE',  ( -11.16403655135938955, 164.3615022471902591, -10.00000000000009592 ) ) ;
#23691=CARTESIAN_POINT ( 'NONE',  ( 200.0860664192757952, 270.7206606627561882, -11.57593477606718224 ) ) ;
#23692=EDGE_CURVE ( 'NONE', #70225, #8187, #26965, .T. ) ;
#23695=CARTESIAN_POINT ( 'NONE',  ( 137.2172943591538967, 238.4824982072973967, 3.021315404115420679E-15 ) ) ;
#23696=CARTESIAN_POINT ( 'NONE',  ( 149.0203866098534888, 272.5361143586139860, -12.73049804737905255 ) ) ;
#23698=CARTESIAN_POINT ( 'NONE',  ( 64.74832919946385346, 214.3149278399160949, -9.188101187500095079 ) ) ;
#23701=CARTESIAN_POINT ( 'NONE',  ( 159.2511875226268216, 254.8158473755685520, 15.75855490706745599 ) ) ;
#23703=CARTESIAN_POINT ( 'NONE',  ( 201.4964414552794949, 281.6449211855650674, 17.70651170561034249 ) ) ;
#23706=CARTESIAN_POINT ( 'NONE',  ( 198.2505066714982149, 285.2670451491296149, 0.000000000000000000 ) ) ;
#23707=CARTESIAN_POINT ( 'NONE',  ( 110.1516887621107514, 227.7365022471902023, 10.00000000000009592 ) ) ;
#23708=CARTESIAN_POINT ( 'NONE',  ( 188.0361769804965206, 281.7550819701144746, -17.70093714309158983 ) ) ;
#23709=CARTESIAN_POINT ( 'NONE',  ( 164.5867587387928950, 245.5743669417666126, -3.022048486790635202 ) ) ;
#23712=CARTESIAN_POINT ( 'NONE',  ( 185.8344414862758640, 272.0246830691658602, 15.77586892895689985 ) ) ;
#23713=ORIENTED_EDGE ( 'NONE', *, *, #25496, .F. ) ;
#23714=CARTESIAN_POINT ( 'NONE',  ( 206.4640281786353171, 273.0408085897082060, -10.81921452789957883 ) ) ;
#23715=CARTESIAN_POINT ( 'NONE',  ( 190.3815443110626404, 278.8296166914984155, -16.52682052525312884 ) ) ;
#23716=EDGE_CURVE ( 'NONE', #98890, #41308, #74788, .T. ) ;
#23717=DIRECTION ( 'NONE',  ( 0.4999999999999998890, -0.8660254037844385966, 0.000000000000000000 ) ) ;
#23719=CARTESIAN_POINT ( 'NONE',  ( 176.6558404752379090, 252.2237374370411942, -0.2705739152901737166 ) ) ;
#23722=CARTESIAN_POINT ( 'NONE',  ( 147.8163551302855296, 274.6215580551378821, -9.286329195885331345 ) ) ;
#23723=CARTESIAN_POINT ( 'NONE',  ( 148.5476103079700749, 274.7756356193531246, 7.667830427786927139 ) ) ;
#23724=ORIENTED_EDGE ( 'NONE', *, *, #25496, .T. ) ;
#23725=EDGE_CURVE ( 'NONE', #90439, #32720, #21662, .T. ) ;
#23732=CARTESIAN_POINT ( 'NONE',  ( 154.8192283419015212, 273.5986471974344454, 13.52555164010807864 ) ) ;
#23735=ORIENTED_EDGE ( 'NONE', *, *, #44819, .T. ) ;
#23736=CARTESIAN_POINT ( 'NONE',  ( 174.3933856302132028, 286.8564427156816237, 11.77909119299353691 ) ) ;
#23737=CARTESIAN_POINT ( 'NONE',  ( 162.8327449136414771, 284.5743273734687477, -2.483999256947636347 ) ) ;
#23740=CARTESIAN_POINT ( 'NONE',  ( 163.4084407101100851, 247.6152736349200438, -10.68829614238923931 ) ) ;
#23741=CARTESIAN_POINT ( 'NONE',  ( 204.9427641582406636, 275.6757151647582305, 14.40446820030680897 ) ) ;
#23743=CARTESIAN_POINT ( 'NONE',  ( 157.1002372043759010, 258.5414026113353430, -17.73553732786789539 ) ) ;
#23744=CARTESIAN_POINT ( 'NONE',  ( 130.4037065759891334, 258.3464784336661637, 1.353441290958777525E-15 ) ) ;
#23746=CARTESIAN_POINT ( 'NONE',  ( 181.7753553325198368, 260.2882442932133813, 9.488355369979771581 ) ) ;
#23747=CARTESIAN_POINT ( 'NONE',  ( 74.46396492422927338, 222.9869531367911293, 4.594050593750046652 ) ) ;
#23748=ORIENTED_EDGE ( 'NONE', *, *, #77498, .T. ) ;
#23749=CARTESIAN_POINT ( 'NONE',  ( 191.5694344253287511, 298.8390017285333897, 8.250976118904059575 ) ) ;
#23753=CARTESIAN_POINT ( 'NONE',  ( 157.3508622362421647, 258.1073073224944778, -17.04076575304558361 ) ) ;
#23755=VERTEX_POINT ( 'NONE', #14758 ) ;
#23757=ADVANCED_FACE ( 'NONE', ( #30458 ), #20389, .T. ) ;
#23759=CARTESIAN_POINT ( 'NONE',  ( 190.9474291326297930, 266.7645650087163745, -12.82661358031884546 ) ) ;
#23760=CARTESIAN_POINT ( 'NONE',  ( 191.1687199697037443, 299.5330595250031820, -8.491751560014430211 ) ) ;
#23761=B_SPLINE_SURFACE_WITH_KNOTS ( 'NONE', 3, 1, ( 
 ( #48476, #17569 ),
 ( #16066, #79418 ),
 ( #86037, #78893 ),
 ( #70258, #47461 ),
 ( #9479, #39837 ),
 ( #54539, #40350 ),
 ( #71287, #10477 ),
 ( #16565, #9984 ),
 ( #95119, #46968 ),
 ( #2388, #78386 ),
 ( #85522, #31745 ),
 ( #77887, #25684 ),
 ( #32761, #70767 ),
 ( #31259, #63667 ),
 ( #94606, #40843 ),
 ( #56564, #25161 ),
 ( #1383, #62146 ),
 ( #32263, #71790 ),
 ( #48978, #41354 ),
 ( #72296, #23649 ),
 ( #58552, #11499 ),
 ( #57556, #18586 ),
 ( #50955, #89523 ),
 ( #20578, #4882 ),
 ( #88533, #19600 ),
 ( #49973, #19094 ),
 ( #80930, #27179 ),
 ( #26671, #97591 ),
 ( #35764, #65165 ),
 ( #43850, #49465 ),
 ( #57056, #80420 ),
 ( #66169, #33796 ),
 ( #95630, #72807 ),
 ( #58067, #59032 ) ),
 .UNSPECIFIED., .T., .F., .F.,
 ( 4, 2, 2, 2, 2, 2, 2, 2, 2, 2, 2, 2, 2, 2, 2, 2, 4 ),
 ( 2, 2 ),
 ( 0.000000000000000000, 0.06250000000000000000, 0.1250000000000000000, 0.1875000000000000000, 0.2500000000000000000, 0.3125000000000000000, 0.3750000000000000000, 0.4375000000000000000, 0.5000000000000000000, 0.5625000000000000000, 0.6250000000000000000, 0.6875000000000000000, 0.7500000000000000000, 0.8125000000000000000, 0.8750000000000000000, 0.9375000000000000000, 1.000000000000000000 ),
 ( 0.000000000000000000, 1.000000000000000000 ),
 .UNSPECIFIED. ) ;
#23764=CARTESIAN_POINT ( 'NONE',  ( 80.66154599400290692, 223.5024278399160949, -9.188101187500093303 ) ) ;
#23765=EDGE_LOOP ( 'NONE', ( #97777, #89302, #86612, #95111 ) ) ;
#23768=ORIENTED_EDGE ( 'NONE', *, *, #55653, .F. ) ;
#23771=CARTESIAN_POINT ( 'NONE',  ( 162.0504616076140678, 249.9673624360595454, -13.49018830579758266 ) ) ;
#23772=ORIENTED_EDGE ( 'NONE', *, *, #19558, .F. ) ;
#23774=EDGE_CURVE ( 'NONE', #11960, #25891, #53045, .T. ) ;
#23777=CARTESIAN_POINT ( 'NONE',  ( 206.5280879940269756, 272.9298537347264642, 11.21709153681466731 ) ) ;
#23780=CARTESIAN_POINT ( 'NONE',  ( 147.1270795744234476, 264.4111747905818675, -1.822351119449947324E-15 ) ) ;
#23782=ORIENTED_EDGE ( 'NONE', *, *, #2012, .F. ) ;
#23784=CARTESIAN_POINT ( 'NONE',  ( 188.6651695142899143, 294.9748060149505591, 11.65985380162412710 ) ) ;
#23785=ADVANCED_FACE ( 'NONE', ( #23252 ), #45563, .F. ) ;
#23787=CARTESIAN_POINT ( 'NONE',  ( 196.6610909444931679, 276.7880959174222539, 16.58182079090270733 ) ) ;
#23788=CARTESIAN_POINT ( 'NONE',  ( 201.0844796915553161, 282.3584598911111812, -16.59562674965125950 ) ) ;
#23789=CARTESIAN_POINT ( 'NONE',  ( 102.4195449475128470, 241.4860189848785126, -2.679491924311252493 ) ) ;
#23792=CARTESIAN_POINT ( 'NONE',  ( -22.42236680055709641, 157.8615022471902591, 0.000000000000000000 ) ) ;
#23794=CARTESIAN_POINT ( 'NONE',  ( 27.87927540258908365, 180.2365022471902023, -10.00000000000009237 ) ) ;
#23797=CARTESIAN_POINT ( 'NONE',  ( 153.4175160819171708, 270.2815289807249997, 14.02256376582253061 ) ) ;
#23798=ORIENTED_EDGE ( 'NONE', *, *, #41862, .T. ) ;
#23799=CARTESIAN_POINT ( 'NONE',  ( 202.2712651538608668, 280.3028871727136675, 16.13191389836473988 ) ) ;
#23801=CARTESIAN_POINT ( 'NONE',  ( 155.1376601545389917, 261.9406857754215707, 18.55063430030667959 ) ) ;
#23803=CARTESIAN_POINT ( 'NONE',  ( 178.6256486530057259, 287.8356261986529034, -12.96677738169596061 ) ) ;
#23804=B_SPLINE_CURVE_WITH_KNOTS ( 'NONE', 3,
 ( #41356, #97117, #72809, #57559 ),
 .UNSPECIFIED., .F., .F.,
 ( 4, 4 ),
 ( 0.009127121522214379570, 0.01427955626753199883 ),
 .UNSPECIFIED. ) ;
#23806=CARTESIAN_POINT ( 'NONE',  ( 171.6010233849675330, 274.8379305346047659, 17.12104339205637871 ) ) ;
#23807=CARTESIAN_POINT ( 'NONE',  ( 166.3787229958576859, 286.5602776898857087, -3.288044247041284507 ) ) ;
#23809=CARTESIAN_POINT ( 'NONE',  ( 192.1608772079249263, 261.8654286030369462, 3.048632953649568655 ) ) ;
#23810=CARTESIAN_POINT ( 'NONE',  ( 187.9196281127333918, 297.0021197407985483, -9.095446553628486086 ) ) ;
#23811=CARTESIAN_POINT ( 'NONE',  ( 4.207654042216683266, 182.4244531367911293, -4.594050593750046652 ) ) ;
#23813=ORIENTED_EDGE ( 'NONE', *, *, #75108, .F. ) ;
#23814=CARTESIAN_POINT ( 'NONE',  ( 174.8837099083871180, 255.2975024955725303, 8.373857793136043171 ) ) ;
#23816=CARTESIAN_POINT ( 'NONE',  ( 25.10051690851626560, 194.4869531367911293, 4.594050593750046652 ) ) ;
#23817=CIRCLE ( 'NONE', #72394, 5.000000000000023981 ) ;
#23818=CARTESIAN_POINT ( 'NONE',  ( 69.44849478424214340, 204.2365022471902023, -10.00000000000009237 ) ) ;
#23821=CARTESIAN_POINT ( 'NONE',  ( 191.2111338740054975, 299.4595964878050154, -9.718193530796334301 ) ) ;
#23822=CARTESIAN_POINT ( 'NONE',  ( 5.154066788520982101, 185.3297689869269504, -2.679491924311252493 ) ) ;
#23823=CARTESIAN_POINT ( 'NONE',  ( 189.9097473895767507, 298.3003973193997354, -7.968993835093706402 ) ) ;
#23826=CARTESIAN_POINT ( 'NONE',  ( 73.77862180316432728, 206.7365022471902023, 10.00000000000009592 ) ) ;
#23827=( BOUNDED_CURVE ( )  B_SPLINE_CURVE ( 2, ( #90174, #34920, #20244, #12652, #51119, #50616, #65816, #19268, #72964 ),
 .UNSPECIFIED., .F., .T. ) 
 B_SPLINE_CURVE_WITH_KNOTS ( ( 3, 2, 2, 2, 3 ),
 ( 0.6250000000000000000, 0.6263440860215053752, 0.6290322580645161255, 0.6317204301075268758, 0.6330645161290322509 ),
 .UNSPECIFIED. ) 
 CURVE ( )  GEOMETRIC_REPRESENTATION_ITEM ( )  RATIONAL_B_SPLINE_CURVE ( ( 0.9330127018922194093, 0.9330127018922194093, 1.000000000000000000, 0.8660254037844387076, 1.000000000000000000, 0.8660254037844387076, 1.000000000000000000, 0.9330127018922194093, 0.9330127018922194093 ) ) 
 REPRESENTATION_ITEM ( '' )  );
#23829=CARTESIAN_POINT ( 'NONE',  ( 175.4967466201937611, 291.2628096033125189, 6.560984766252938805 ) ) ;
#23830=CARTESIAN_POINT ( 'NONE',  ( 31.32559514186443295, 179.7048013555409796, 4.594050593750051981 ) ) ;
#23833=CARTESIAN_POINT ( 'NONE',  ( 203.0120883329668970, 270.0550711529738237, -6.419258576597377974 ) ) ;
#23834=CARTESIAN_POINT ( 'NONE',  ( 151.4188942279983223, 268.3817773016460251, -14.77302265413830895 ) ) ;
#23838=CARTESIAN_POINT ( 'NONE',  ( 159.8915935406342612, 278.4112977589962838, -10.47619785574662998 ) ) ;
#23839=CARTESIAN_POINT ( 'NONE',  ( 205.8099205723994203, 269.1131406545866298, -1.356034389334280776 ) ) ;
#23842=CARTESIAN_POINT ( 'NONE',  ( 174.5885488454506174, 256.4458599265808516, 12.05082362884263425 ) ) ;
#23845=B_SPLINE_CURVE_WITH_KNOTS ( 'NONE', 3,
 ( #4214, #57915, #43195, #95973 ),
 .UNSPECIFIED., .F., .F.,
 ( 4, 4 ),
 ( 0.009376484201431983107, 0.01501325678996159353 ),
 .UNSPECIFIED. ) ;
#23846=B_SPLINE_CURVE_WITH_KNOTS ( 'NONE', 3,
 ( #92207, #13667, #91194, #44540 ),
 .UNSPECIFIED., .F., .F.,
 ( 4, 4 ),
 ( 0.01730275677769292988, 0.02623041320600179305 ),
 .UNSPECIFIED. ) ;
#23849=CARTESIAN_POINT ( 'NONE',  ( -2.305318362029009638, 176.1427522451419350, -10.00000000000009592 ) ) ;
#23852=CARTESIAN_POINT ( 'NONE',  ( 186.7554075434758545, 282.3000898601083577, 17.53539547572453827 ) ) ;
#23853=LINE ( 'NONE', #46657, #38446 ) ;
#23857=ORIENTED_EDGE ( 'NONE', *, *, #19286, .F. ) ;
#23862=ORIENTED_EDGE ( 'NONE', *, *, #59293, .F. ) ;
#23863=CARTESIAN_POINT ( 'NONE',  ( 201.4617167010348737, 281.7050662241970826, -17.43131506460443703 ) ) ;
#23867=CARTESIAN_POINT ( 'NONE',  ( 190.4750160083620472, 300.7345900314585947, -1.159659205620361400 ) ) ;
#23868=CARTESIAN_POINT ( 'NONE',  ( 201.9133243980324153, 266.9637997000594396, 2.242576533087043966 ) ) ;
#23871=CARTESIAN_POINT ( 'NONE',  ( 162.1260167985288376, 266.6785162637209510, 17.71249957499354366 ) ) ;
#23872=EDGE_LOOP ( 'NONE', ( #31116, #87243, #82229 ) ) ;
#23874=CARTESIAN_POINT ( 'NONE',  ( 157.6466783816650832, 259.5949387289228412, 17.71616314254395519 ) ) ;
#23876=ORIENTED_EDGE ( 'NONE', *, *, #91364, .F. ) ;
#23879=CARTESIAN_POINT ( 'NONE',  ( 97.35977185683022128, 217.0177522451417929, 5.000000000000051514 ) ) ;
#23881=ORIENTED_EDGE ( 'NONE', *, *, #69149, .T. ) ;
#23884=CARTESIAN_POINT ( 'NONE',  ( 190.9492596519850451, 299.5322795678457624, 5.766969289918903563 ) ) ;
#23885=CARTESIAN_POINT ( 'NONE',  ( 146.8000281410530192, 276.3818880375922049, 4.652863924796177386 ) ) ;
#23886=CARTESIAN_POINT ( 'NONE',  ( 148.3837145175834280, 273.6388627701866767, 8.841971351370922605 ) ) ;
#23889=CARTESIAN_POINT ( 'NONE',  ( 149.7162292714551199, 271.3308795146458010, 12.12826134257344357 ) ) ;
#23890=CARTESIAN_POINT ( 'NONE',  ( 157.2720021843916243, 259.7600564740663458, -17.50627268554094940 ) ) ;
#23892=CARTESIAN_POINT ( 'NONE',  ( 192.4172326059820648, 297.3705722050773943, -12.52563289807247848 ) ) ;
#23894=CARTESIAN_POINT ( 'NONE',  ( 148.9694607950094394, 272.6243204573405592, 11.81236034532910573 ) ) ;
#23897=CARTESIAN_POINT ( 'NONE',  ( 164.8537203408104972, 245.1119758834023230, 2.926011033004258355 ) ) ;
#23901=CARTESIAN_POINT ( 'NONE',  ( 116.8724067376222706, 238.2833772461660544, -9.188101187500095079 ) ) ;
#23903=CARTESIAN_POINT ( 'NONE',  ( 147.2937583206075942, 275.5267222813735088, 0.1877253132609109920 ) ) ;
#23907=EDGE_CURVE ( 'NONE', #13902, #96030, #50526, .T. ) ;
#23908=CARTESIAN_POINT ( 'NONE',  ( 203.4682009197399566, 278.2297336128146412, -15.36039508894693206 ) ) ;
#23909=CARTESIAN_POINT ( 'NONE',  ( 204.8523313866422484, 275.8323493198358847, 14.65426965484541100 ) ) ;
#23912=VERTEX_POINT ( 'NONE', #80007 ) ;
#23913=CARTESIAN_POINT ( 'NONE',  ( 207.6555576926778883, 270.9770189326688410, -1.235081510489080436 ) ) ;
#23917=CARTESIAN_POINT ( 'NONE',  ( 127.4544149619371609, 235.2048013555409796, 4.594050593750051981 ) ) ;
#23918=CARTESIAN_POINT ( 'NONE',  ( 150.6815632051821581, 269.6588720951601772, -14.68790257316217307 ) ) ;
#23919=CARTESIAN_POINT ( 'NONE',  ( 185.8154782850418769, 296.8462876573850053, 4.389817180861387058 ) ) ;
#23920=CARTESIAN_POINT ( 'NONE',  ( 157.3025066944120454, 258.1910615777721887, 18.21299529665260053 ) ) ;
#23921=FACE_OUTER_BOUND ( 'NONE', #33378, .T. ) ;
#23922=CARTESIAN_POINT ( 'NONE',  ( 51.75794814269728050, 206.8149278399160949, -9.188101187500095079 ) ) ;
#23928=CARTESIAN_POINT ( 'NONE',  ( 175.0126904547745994, 261.3741942827071512, 14.53273751430707428 ) ) ;
#23930=CARTESIAN_POINT ( 'NONE',  ( 202.8535267948003593, 279.2943804273081696, -15.36804658072946062 ) ) ;
#23931=CARTESIAN_POINT ( 'NONE',  ( 153.6154705056581520, 269.2265720717915087, -15.53643265229117887 ) ) ;
#23933=CARTESIAN_POINT ( 'NONE',  ( 112.0100349375169912, 222.1427522451417644, 1.119607411625061291E-15 ) ) ;
#23934=CARTESIAN_POINT ( 'NONE',  ( 171.1380476607806429, 267.8866146403163384, -17.76239963503928010 ) ) ;
#23937=CARTESIAN_POINT ( 'NONE',  ( 202.4323889586180201, 280.0238125565655878, 15.69595176008160919 ) ) ;
#23938=FACE_OUTER_BOUND ( 'NONE', #43572, .T. ) ;
#23939=CARTESIAN_POINT ( 'NONE',  ( 24.64070123457955219, 185.0333772461660544, 9.188101187500095079 ) ) ;
#23945=CARTESIAN_POINT ( 'NONE',  ( 71.40607303893924040, 212.0333772461660544, 9.188101187500095079 ) ) ;
#23946=CARTESIAN_POINT ( 'NONE',  ( 200.2690241097007799, 283.7708703901988656, 16.96680019208369927 ) ) ;
#23947=CARTESIAN_POINT ( 'NONE',  ( 174.3922364351138867, 288.8364454784203872, 7.670429905402864179 ) ) ;
#23948=CARTESIAN_POINT ( 'NONE',  ( 183.9122833166825615, 256.5348419210068300, 1.420446916831177298 ) ) ;
#23952=CARTESIAN_POINT ( 'NONE',  ( 27.80710661894035596, 186.8615022471902591, -10.00000000000009592 ) ) ;
#23954=CARTESIAN_POINT ( 'NONE',  ( 202.7041331321765938, 279.5531378413010657, 17.14708438049711248 ) ) ;
#23955=AXIS2_PLACEMENT_3D ( 'NONE', #36270, #42364, #27697 ) ;
#23956=CARTESIAN_POINT ( 'NONE',  ( -5.561934722402757991, 167.5958772461660544, -9.188101187500095079 ) ) ;
#23958=CARTESIAN_POINT ( 'NONE',  ( 167.7533332108949935, 262.4447794098586542, -16.91708224468162314 ) ) ;
#23959=CARTESIAN_POINT ( 'NONE',  ( 170.6150151926208309, 263.3591274673946145, 15.81415637510684391 ) ) ;
#23960=CARTESIAN_POINT ( 'NONE',  ( 185.5793223466652364, 259.8320106733570469, 7.401475797627644404 ) ) ;
#23961=CARTESIAN_POINT ( 'NONE',  ( 164.3022921857394749, 246.0670774647090582, 1.862798784958315856 ) ) ;
#23965=ORIENTED_EDGE ( 'NONE', *, *, #65141, .F. ) ;
#23966=B_SPLINE_CURVE_WITH_KNOTS ( 'NONE', 3,
 ( #69119, #70618, #100046, #1746 ),
 .UNSPECIFIED., .F., .F.,
 ( 4, 4 ),
 ( 0.002746326142393483178, 0.008136428815393210653 ),
 .UNSPECIFIED. ) ;
#23969=CARTESIAN_POINT ( 'NONE',  ( 178.3755071135885260, 285.5767383373634516, 12.93467627631818040 ) ) ;
#23970=CARTESIAN_POINT ( 'NONE',  ( 196.7042903992237086, 289.4290128693130555, 16.50876271461077849 ) ) ;
#23973=CARTESIAN_POINT ( 'NONE',  ( 206.7416841040605391, 272.5598944198493427, 8.000062685979553834 ) ) ;
#23974=CARTESIAN_POINT ( 'NONE',  ( 157.6921299354026189, 257.5162143285667753, -18.18720974599499840 ) ) ;
#23975=DIRECTION ( 'NONE',  ( -0.8660254037844387076, -0.4999999999999998890, -0.000000000000000000 ) ) ;
#23981=CARTESIAN_POINT ( 'NONE',  ( 162.6396274730868186, 248.9468972229755082, -10.26162218571527518 ) ) ;
#23982=CARTESIAN_POINT ( 'NONE',  ( 152.8328714238065515, 265.9326969577624027, -16.29536156676786263 ) ) ;
#23985=CARTESIAN_POINT ( 'NONE',  ( 138.6787122315880083, 239.3262482093457493, 3.021315404115420679E-15 ) ) ;
#23986=CARTESIAN_POINT ( 'NONE',  ( 164.1412601152769639, 248.5329951649505063, 9.989603322558886944 ) ) ;
#23987=VERTEX_POINT ( 'NONE', #4976 ) ;
#23994=CARTESIAN_POINT ( 'NONE',  ( 196.9431415128477170, 289.5314680279574304, -16.61413060656005669 ) ) ;
#23996=VERTEX_POINT ( 'NONE', #67251 ) ;
#23997=CARTESIAN_POINT ( 'NONE',  ( 161.4726291907278721, 250.9681975403669867, 14.52346149734912117 ) ) ;
#23998=CARTESIAN_POINT ( 'NONE',  ( 150.8167050463783312, 269.4247995599803289, 14.38040671671637938 ) ) ;
#24000=B_SPLINE_SURFACE_WITH_KNOTS ( 'NONE', 3, 1, ( 
 ( #14065, #75891 ),
 ( #90106, #82526 ),
 ( #60141, #35364 ),
 ( #96713, #91103 ),
 ( #97692, #36355 ),
 ( #43949, #27280 ),
 ( #58162, #59135 ),
 ( #36859, #21669 ),
 ( #58650, #89624 ),
 ( #52063, #52549 ),
 ( #67768, #20185 ),
 ( #83501, #19694 ),
 ( #74888, #44449 ),
 ( #83006, #5471 ),
 ( #28261, #51052 ),
 ( #34854, #65758 ),
 ( #66763, #73878 ),
 ( #81510, #4471 ),
 ( #42939, #4984 ),
 ( #82012, #66274 ),
 ( #67260, #13578 ),
 ( #35863, #98185 ),
 ( #12587, #28767 ),
 ( #59649, #43458 ),
 ( #90620, #21184 ),
 ( #75382, #98691 ),
 ( #29273, #8456 ),
 ( #22161, #69746 ),
 ( #46433, #54525 ),
 ( #38840, #31730 ),
 ( #85506, #45447 ),
 ( #30257, #61644 ),
 ( #6470, #84499 ),
 ( #77871, #77362 ) ),
 .UNSPECIFIED., .T., .F., .F.,
 ( 4, 2, 2, 2, 2, 2, 2, 2, 2, 2, 2, 2, 2, 2, 2, 2, 4 ),
 ( 2, 2 ),
 ( 0.000000000000000000, 0.06250000000000000000, 0.1250000000000000000, 0.1875000000000000000, 0.2500000000000000000, 0.3125000000000000000, 0.3750000000000000000, 0.4375000000000000000, 0.5000000000000000000, 0.5625000000000000000, 0.6250000000000000000, 0.6875000000000000000, 0.7500000000000000000, 0.8125000000000000000, 0.8750000000000000000, 0.9375000000000000000, 1.000000000000000000 ),
 ( 0.000000000000000000, 1.000000000000000000 ),
 .UNSPECIFIED. ) ;
#24003=B_SPLINE_CURVE_WITH_KNOTS ( 'NONE', 3,
 ( #85867, #18414, #77718, #32082, #48812, #2216, #47285, #33097, #8796, #94935 ),
 .UNSPECIFIED., .F., .F.,
 ( 4, 2, 2, 2, 4 ),
 ( 0.001476764202228747404, 0.001775028363004824659, 0.002073292523780901914, 0.002371556684556979169, 0.002669820845333056424 ),
 .UNSPECIFIED. ) ;
#24005=CARTESIAN_POINT ( 'NONE',  ( 160.3106292389843759, 268.8982433465296253, -16.92231543148939821 ) ) ;
#24009=CARTESIAN_POINT ( 'NONE',  ( 164.1821508476733698, 246.2751683663292397, -7.347745041495428175 ) ) ;
#24011=B_SPLINE_CURVE_WITH_KNOTS ( 'NONE', 3,
 ( #95835, #86738, #49189, #9702 ),
 .UNSPECIFIED., .F., .F.,
 ( 4, 4 ),
 ( 0.01365957469120875761, 0.02004134161460488853 ),
 .UNSPECIFIED. ) ;
#24015=CARTESIAN_POINT ( 'NONE',  ( 148.1004780136491377, 274.1294427855589788, -7.811560775291159331 ) ) ;
#24016=CARTESIAN_POINT ( 'NONE',  ( 175.4882053081535105, 290.1142015617031689, 6.168936154768994484 ) ) ;
#24017=CARTESIAN_POINT ( 'NONE',  ( 197.6892542711904071, 288.2391628223323892, -17.84453492130724683 ) ) ;
#24021=CARTESIAN_POINT ( 'NONE',  ( 163.8627344909259307, 282.1053904094392237, 8.484041907820431661 ) ) ;
#24023=CARTESIAN_POINT ( 'NONE',  ( 207.0213404229716900, 271.3941896262130626, 5.057553085821338001 ) ) ;
#24025=CARTESIAN_POINT ( 'NONE',  ( 176.4901148274036586, 293.1746585049929763, 1.855142305940338465 ) ) ;
#24026=CARTESIAN_POINT ( 'NONE',  ( 206.0930919633010774, 273.6832889610345774, -9.866500005465628220 ) ) ;
#24029=CARTESIAN_POINT ( 'NONE',  ( 161.5431944097339851, 250.8459749958011287, 14.52339846942414603 ) ) ;
#24030=CARTESIAN_POINT ( 'NONE',  ( 191.5383557437975242, 262.3965109955362891, -0.7496224257124077806 ) ) ;
#24032=CARTESIAN_POINT ( 'NONE',  ( 155.3230890646803175, 261.6195134818649422, -18.58700029486878691 ) ) ;
#24035=B_SPLINE_CURVE_WITH_KNOTS ( 'NONE', 3,
 ( #90223, #26887, #73991, #66375 ),
 .UNSPECIFIED., .F., .F.,
 ( 4, 4 ),
 ( 0.003196948845168229043, 0.006410911750259561115 ),
 .UNSPECIFIED. ) ;
#24036=CARTESIAN_POINT ( 'NONE',  ( -17.42236680055705023, 149.2012482093457777, 0.000000000000000000 ) ) ;
#24037=CARTESIAN_POINT ( 'NONE',  ( 15.15952728095722435, 172.8927522451418213, 10.00000000000009592 ) ) ;
#24038=CARTESIAN_POINT ( 'NONE',  ( 84.42325706775034178, 228.7369531367911293, -4.594050593750048428 ) ) ;
#24041=CARTESIAN_POINT ( 'NONE',  ( 175.0387250457744983, 253.3993311541219953, -7.863511161993287146 ) ) ;
#24042=CARTESIAN_POINT ( 'NONE',  ( 166.8803400540483324, 278.2769978431516051, -14.68497553134216460 ) ) ;
#24044=EDGE_CURVE ( 'NONE', #66029, #42203, #47999, .T. ) ;
#24045=CARTESIAN_POINT ( 'NONE',  ( 0.5273063997304934247, 181.1115022471903444, -5.000000000000047962 ) ) ;
#24046=CARTESIAN_POINT ( 'NONE',  ( 11.05475416482865114, 183.3149278399160664, 9.188101187500093303 ) ) ;
#24048=CARTESIAN_POINT ( 'NONE',  ( 161.4469036912142599, 251.0127554125742222, 12.93933463576739307 ) ) ;
#24053=CARTESIAN_POINT ( 'NONE',  ( 200.8652091308636614, 267.7637384965461251, -2.870084330802582073 ) ) ;
#24056=CARTESIAN_POINT ( 'NONE',  ( 207.1285138014047504, 271.8898857301724661, -5.752177443817618752 ) ) ;
#24060=CARTESIAN_POINT ( 'NONE',  ( 36.33204418566946714, 191.7833772461660544, -9.188101187500095079 ) ) ;
#24061=CARTESIAN_POINT ( 'NONE',  ( 199.9817534399692818, 276.6790051391964766, 15.46620920969797019 ) ) ;
#24064=CARTESIAN_POINT ( 'NONE',  ( 182.4076066396311546, 260.8566311360108898, -10.64103732181219009 ) ) ;
#24067=FACE_OUTER_BOUND ( 'NONE', #55863, .T. ) ;
#24068=CARTESIAN_POINT ( 'NONE',  ( 194.1153812227096864, 294.4292925221022870, 15.54001482840963710 ) ) ;
#24069=CARTESIAN_POINT ( 'NONE',  ( 172.8210543149999978, 253.0650713199155177, -9.347212986753337560 ) ) ;
#24070=CYLINDRICAL_SURFACE ( 'NONE', #17612, 10.00000000000010658 ) ;
#24071=CARTESIAN_POINT ( 'NONE',  ( 148.1004780136491377, 274.1294427855589788, -7.811560775291159331 ) ) ;
#24073=CARTESIAN_POINT ( 'NONE',  ( 165.0517352912010267, 249.7231812837857490, -10.72255941265194679 ) ) ;
#24075=CARTESIAN_POINT ( 'NONE',  ( 191.3610003135137276, 299.2000202002271294, -9.855749861282104618 ) ) ;
#24076=CARTESIAN_POINT ( 'NONE',  ( 189.9462859318020946, 301.6503773875500087, -1.164147598593831656 ) ) ;
#24077=CARTESIAN_POINT ( 'NONE',  ( 181.2024310249855148, 267.1550630910596738, -14.76750588113328355 ) ) ;
#24079=CARTESIAN_POINT ( 'NONE',  ( 152.4356527347738108, 268.2593731114180287, -15.63005607008648923 ) ) ;
#24080=CARTESIAN_POINT ( 'NONE',  ( 161.3788871511642071, 251.6867952676170148, -13.38168142625398005 ) ) ;
#24081=CARTESIAN_POINT ( 'NONE',  ( 103.3675627755349353, 239.6744531367911577, 4.594050593750047540 ) ) ;
#24083=CARTESIAN_POINT ( 'NONE',  ( 151.4159295687746294, 268.3869122420484814, 14.78076517566594106 ) ) ;
#24085=CARTESIAN_POINT ( 'NONE',  ( 137.9907970510500377, 257.1427522451419350, -10.00000000000009592 ) ) ;
#24086=CARTESIAN_POINT ( 'NONE',  ( 191.9527409762319223, 277.0321975987304768, 17.27471776080598076 ) ) ;
#24087=CARTESIAN_POINT ( 'NONE',  ( 151.0375045328015631, 269.0423636312102076, -14.70054264444876857 ) ) ;
#24088=CARTESIAN_POINT ( 'NONE',  ( 193.3455484147415859, 263.1264988859362006, -5.347548703547762905 ) ) ;
#24095=CARTESIAN_POINT ( 'NONE',  ( 179.0584195722606751, 280.7836316943931365, 16.10768272107902277 ) ) ;
#24096=CARTESIAN_POINT ( 'NONE',  ( 199.5392375079602232, 269.9326292274725461, 9.248178193193567154 ) ) ;
#24097=ORIENTED_EDGE ( 'NONE', *, *, #50313, .T. ) ;
#24100=CARTESIAN_POINT ( 'NONE',  ( 180.3398332753912712, 261.9433912727897109, -12.86148952795812228 ) ) ;
#24105=ORIENTED_EDGE ( 'NONE', *, *, #63047, .F. ) ;
#24106=CARTESIAN_POINT ( 'NONE',  ( 183.4553195968295256, 297.0403188216897661, -2.838562726794640056 ) ) ;
#24111=CARTESIAN_POINT ( 'NONE',  ( 164.4590282730455044, 247.3987909035931523, 7.224049096378683643 ) ) ;
#24114=CARTESIAN_POINT ( 'NONE',  ( 165.4408316472307376, 245.8969016233029379, -1.052724153476761959 ) ) ;
#24115=VERTEX_POINT ( 'NONE', #82520 ) ;
#24121=VECTOR ( 'NONE', #40412, 1000.000000000000000 ) ;
#24122=CARTESIAN_POINT ( 'NONE',  ( 167.5861325596884797, 256.5095974891418109, 15.03189046419509367 ) ) ;
#24126=CARTESIAN_POINT ( 'NONE',  ( 30.24280306353617576, 188.2677522451418497, 10.00000000000009592 ) ) ;
#24129=CARTESIAN_POINT ( 'NONE',  ( 162.9767404783699476, 249.5334703659529794, 11.21793991045672101 ) ) ;
#24130=EDGE_LOOP ( 'NONE', ( #45652, #88512, #19907, #28466, #14874 ) ) ;
#24133=CARTESIAN_POINT ( 'NONE',  ( 172.9470997986933583, 271.0928965516715152, 16.42712932072691956 ) ) ;
#24138=CARTESIAN_POINT ( 'NONE',  ( 164.4494270235151419, 246.2274769805200378, 2.019287977540549672 ) ) ;
#24139=CARTESIAN_POINT ( 'NONE',  ( 205.9736828131439097, 273.8901116759951719, -10.08879389214638778 ) ) ;
#24140=CARTESIAN_POINT ( 'NONE',  ( 190.4402228526265048, 300.7948535449484098, 3.477366254517368027 ) ) ;
#24141=CARTESIAN_POINT ( 'NONE',  ( 148.9498507103374152, 272.6582861203333437, 11.90061892622094852 ) ) ;
#24143=CARTESIAN_POINT ( 'NONE',  ( 171.3423592652010257, 250.9382160742572125, -5.598082297702525523 ) ) ;
#24145=CARTESIAN_POINT ( 'NONE',  ( 157.9671782409957359, 280.9922174830806512, 2.188311894391224310 ) ) ;
#24146=CARTESIAN_POINT ( 'NONE',  ( 120.7963240266967375, 249.7369531367911293, -4.594050593750048428 ) ) ;
#24150=AXIS2_PLACEMENT_3D ( 'NONE', #9392, #40765, #63584 ) ;
#24153=CARTESIAN_POINT ( 'NONE',  ( 200.2744661981036245, 273.7070197329613848, 13.96177302380764296 ) ) ;
#24155=CARTESIAN_POINT ( 'NONE',  ( 171.3481116032015450, 287.9154882923708669, -4.631609681352044205 ) ) ;
#24156=CARTESIAN_POINT ( 'NONE',  ( 192.4409507480105788, 297.3294911780226357, 11.00602545404914423 ) ) ;
#24159=CARTESIAN_POINT ( 'NONE',  ( 167.2515702596184042, 262.0622343731731689, -17.21809106051008342 ) ) ;
#24160=CARTESIAN_POINT ( 'NONE',  ( 174.3399253482853055, 282.2778084546079072, 14.88242142284587999 ) ) ;
#24161=CARTESIAN_POINT ( 'NONE',  ( 177.2207926979908450, 256.1411382841860700, -7.659123640409692513 ) ) ;
#24163=CARTESIAN_POINT ( 'NONE',  ( 200.5575725585719056, 282.8488716230692717, -16.71982794578856968 ) ) ;
#24164=CARTESIAN_POINT ( 'NONE',  ( 150.4165202980163087, 271.9204874465632997, 11.69410747874298018 ) ) ;
#24167=B_SPLINE_CURVE_WITH_KNOTS ( 'NONE', 3,
 ( #30751, #24635, #7954, #53534 ),
 .UNSPECIFIED., .F., .F.,
 ( 4, 4 ),
 ( 0.01326838758303781549, 0.01964715698747628719 ),
 .UNSPECIFIED. ) ;
#24168=CARTESIAN_POINT ( 'NONE',  ( 191.0339685792297644, 283.3628942986244397, -16.57419516574317697 ) ) ;
#24169=CARTESIAN_POINT ( 'NONE',  ( 191.9264930372023059, 298.2205580714880853, -10.94482840438815074 ) ) ;
#24172=CARTESIAN_POINT ( 'NONE',  ( 204.6283382085973699, 273.0595963888450797, -10.48110626936752610 ) ) ;
#24173=CARTESIAN_POINT ( 'NONE',  ( 164.3811851369638362, 283.5116506413451702, -6.723331180138965024 ) ) ;
#24174=CARTESIAN_POINT ( 'NONE',  ( 160.8722636754860105, 281.5937424928134760, 5.676029096099265203 ) ) ;
#24175=CYLINDRICAL_SURFACE ( 'NONE', #70506, 17.82106496071139645 ) ;
#24177=CARTESIAN_POINT ( 'NONE',  ( 190.7908437487391780, 300.1875603386860689, -4.317984972589949955 ) ) ;
#24179=CARTESIAN_POINT ( 'NONE',  ( 164.7364331287320738, 247.3151232938002693, -7.618980141130590411 ) ) ;
#24180=CARTESIAN_POINT ( 'NONE',  ( 129.3070403213095005, 233.9155109091896065, 2.679491924311254714 ) ) ;
#24181=CARTESIAN_POINT ( 'NONE',  ( 28.94376495785951775, 187.5177522451418497, -10.00000000000009592 ) ) ;
#24182=CARTESIAN_POINT ( 'NONE',  ( 167.3350697697217413, 278.0087195862697058, 15.28430507972256258 ) ) ;
#24183=CARTESIAN_POINT ( 'NONE',  ( 204.3334868499358095, 275.8344458505681018, 13.13630129970992400 ) ) ;
#24187=CARTESIAN_POINT ( 'NONE',  ( -1.340060878953613477, 170.0333772461660828, 9.188101187500095079 ) ) ;
#24188=CARTESIAN_POINT ( 'NONE',  ( 82.93486267893707975, 224.8149278399160949, -9.188101187500095079 ) ) ;
#24189=CARTESIAN_POINT ( 'NONE',  ( 155.5322964227545413, 261.2571557083629159, -18.35853982030605280 ) ) ;
#24190=CARTESIAN_POINT ( 'NONE',  ( 192.8011239859581849, 296.7056528303708660, -11.79847971295421694 ) ) ;
#24196=B_SPLINE_CURVE_WITH_KNOTS ( 'NONE', 3,
 ( #87248, #80113, #64367, #96812 ),
 .UNSPECIFIED., .F., .F.,
 ( 4, 4 ),
 ( 0.01106257217117561677, 0.01948240598213658858 ),
 .UNSPECIFIED. ) ;
#24200=CARTESIAN_POINT ( 'NONE',  ( 179.4642332055343843, 290.3349191133465865, 9.386686624933396672 ) ) ;
#24201=CARTESIAN_POINT ( 'NONE',  ( 169.0248750959679001, 251.9473120095521210, -8.780057449798482239 ) ) ;
#24202=CARTESIAN_POINT ( 'NONE',  ( 163.9989516851529174, 246.5924786237186197, -4.702898507341187084 ) ) ;
#24204=CARTESIAN_POINT ( 'NONE',  ( 157.3363371328520088, 258.1324655395517311, 18.24585617226787093 ) ) ;
#24205=FACE_OUTER_BOUND ( 'NONE', #93163, .T. ) ;
#24208=CARTESIAN_POINT ( 'NONE',  ( 38.76791418169571557, 187.0643266524159856, -9.188101187500093303 ) ) ;
#24209=CARTESIAN_POINT ( 'NONE',  ( 69.56611615166231388, 198.7202760586659736, -5.415160957724236172E-17 ) ) ;
#24210=CARTESIAN_POINT ( 'NONE',  ( 194.0787454455293641, 279.1516233421318702, -17.53274283404612888 ) ) ;
#24212=CARTESIAN_POINT ( 'NONE',  ( 166.9400527077043819, 259.7355344238575867, 15.86299304177872926 ) ) ;
#24213=CARTESIAN_POINT ( 'NONE',  ( 144.0982539169780523, 247.8768266524160140, 9.188101187500098632 ) ) ;
#24216=CARTESIAN_POINT ( 'NONE',  ( 200.1771779054008960, 271.0770489275255386, -11.35077613890620185 ) ) ;
#24219=CARTESIAN_POINT ( 'NONE',  ( 198.8570476668614049, 286.2164853282868080, -17.01721544293231858 ) ) ;
#24220=CARTESIAN_POINT ( 'NONE',  ( 149.1004267900891307, 272.3974806997987343, -12.86882154300063341 ) ) ;
#24222=CARTESIAN_POINT ( 'NONE',  ( 71.35211999908520397, 205.8768266524160424, 9.188101187500096856 ) ) ;
#24224=CARTESIAN_POINT ( 'NONE',  ( 202.7973612924478743, 279.3916619310153919, -15.54732529288344089 ) ) ;
#24225=CARTESIAN_POINT ( 'NONE',  ( 159.5284711081640125, 254.3355781173132755, 15.34104435652608522 ) ) ;
#24228=EDGE_CURVE ( 'NONE', #31200, #93443, #9454, .T. ) ;
#24230=CARTESIAN_POINT ( 'NONE',  ( 114.8426596992765099, 227.1115022471901739, -5.000000000000041744 ) ) ;
#24232=CARTESIAN_POINT ( 'NONE',  ( 206.9026071836525205, 272.2811674698855313, 7.240992997279449561 ) ) ;
#24235=CARTESIAN_POINT ( 'NONE',  ( 186.1070094314815719, 272.1961740520177955, 15.73899880559026876 ) ) ;
#24237=CARTESIAN_POINT ( 'NONE',  ( 206.6298919378964740, 272.7535241315335384, -9.267551915974392429 ) ) ;
#24238=CARTESIAN_POINT ( 'NONE',  ( 193.8280528473190998, 294.2408607629556059, 13.96266529814797330 ) ) ;
#24242=CARTESIAN_POINT ( 'NONE',  ( 173.7443271944094647, 250.8610699240076940, 0.5123999366559217616 ) ) ;
#24243=ORIENTED_EDGE ( 'NONE', *, *, #66320, .T. ) ;
#24245=CARTESIAN_POINT ( 'NONE',  ( 194.3708539535661259, 293.9868007723104029, -16.01585187499628304 ) ) ;
#24247=ORIENTED_EDGE ( 'NONE', *, *, #75542, .T. ) ;
#24249=CARTESIAN_POINT ( 'NONE',  ( 86.71718800452170228, 209.3262482093457777, 3.021315404115420679E-15 ) ) ;
#24251=ORIENTED_EDGE ( 'NONE', *, *, #18119, .F. ) ;
#24253=CARTESIAN_POINT ( 'NONE',  ( 176.4997286254413780, 263.1504487394882972, -15.79179489836881167 ) ) ;
#24254=CARTESIAN_POINT ( 'NONE',  ( 159.9770824720811220, 253.5585604421560788, -16.42166711341322483 ) ) ;
#24259=CARTESIAN_POINT ( 'NONE',  ( 165.0528804069804494, 264.4852527057752241, -17.76608744198970768 ) ) ;
#24260=CARTESIAN_POINT ( 'NONE',  ( 194.4904290197884507, 293.7796906822950973, 14.50206953321744940 ) ) ;
#24261=CARTESIAN_POINT ( 'NONE',  ( 185.2685622359955744, 292.7380640902246682, -11.87166941586229996 ) ) ;
#24262=CARTESIAN_POINT ( 'NONE',  ( 157.3198323354746435, 258.1610526871778006, -16.77630483474704093 ) ) ;
#24263=CARTESIAN_POINT ( 'NONE',  ( 207.9186838572135514, 270.5212710468924229, -3.653080245775895740 ) ) ;
#24266=CARTESIAN_POINT ( 'NONE',  ( 182.7174818772467120, 259.2068321934141295, 9.747744062958584976 ) ) ;
#24267=CARTESIAN_POINT ( 'NONE',  ( 85.91165145656356117, 232.6589784336661637, -6.496448406907675876E-16 ) ) ;
#24268=ORIENTED_EDGE ( 'NONE', *, *, #19007, .F. ) ;
#24269=CARTESIAN_POINT ( 'NONE',  ( 151.2455280670316711, 268.6820563007532314, 14.35914944935941229 ) ) ;
#24272=ORIENTED_EDGE ( 'NONE', *, *, #86416, .F. ) ;
#24281=CARTESIAN_POINT ( 'NONE',  ( 207.8616498235123231, 270.6200568910230118, 3.132900500943239130 ) ) ;
#24282=CARTESIAN_POINT ( 'NONE',  ( 77.73905735199544154, 209.5643266524159571, -9.188101187500093303 ) ) ;
#24283=ORIENTED_EDGE ( 'NONE', *, *, #68646, .F. ) ;
#24285=VERTEX_POINT ( 'NONE', #79891 ) ;
#24287=CARTESIAN_POINT ( 'NONE',  ( 161.9258069053378222, 250.1832707138045180, -14.03928993546631254 ) ) ;
#24288=VERTEX_POINT ( 'NONE', #65145 ) ;
#24290=CARTESIAN_POINT ( 'NONE',  ( 184.0509685884657642, 275.1883516303099668, 16.37021283893107793 ) ) ;
#24293=CARTESIAN_POINT ( 'NONE',  ( 161.7341544900357064, 283.8969558588514133, 0.5209753697341674705 ) ) ;
#24294=CARTESIAN_POINT ( 'NONE',  ( 207.1502663293453281, 270.3057540939174714, -2.562904251084027418 ) ) ;
#24297=CARTESIAN_POINT ( 'NONE',  ( 188.6621308970854898, 295.0522997026344569, 11.72041705296824965 ) ) ;
#24298=CARTESIAN_POINT ( 'NONE',  ( 156.8942407771241108, 274.4291350306359618, 13.75659550080370508 ) ) ;
#24299=CARTESIAN_POINT ( 'NONE',  ( 206.1408608592916494, 273.6005508061571732, -10.42739367433323494 ) ) ;
#24304=DIRECTION ( 'NONE',  ( -0.8660254037844387076, -0.4999999999999998890, -0.000000000000000000 ) ) ;
#24307=CARTESIAN_POINT ( 'NONE',  ( 200.7583183585857967, 282.9233878912788214, 16.96937806979494212 ) ) ;
#24309=CARTESIAN_POINT ( 'NONE',  ( 171.3764566354917633, 251.6546961497424491, 7.121511699425036923 ) ) ;
#24312=CARTESIAN_POINT ( 'NONE',  ( -22.42236680055709641, 157.8615022471902591, 0.000000000000000000 ) ) ;
#24315=CARTESIAN_POINT ( 'NONE',  ( 164.3774690880109119, 245.9368672504194819, -2.805681983503304000 ) ) ;
#24318=CARTESIAN_POINT ( 'NONE',  ( 176.1441259402330672, 285.2298478058193041, -12.99515216835783882 ) ) ;
#24321=CARTESIAN_POINT ( 'NONE',  ( 166.5889384249973091, 286.4434954512080935, -3.248033821752349226 ) ) ;
#24322=CARTESIAN_POINT ( 'NONE',  ( 124.6655725107735435, 254.3297689869269504, -2.679491924311252493 ) ) ;
#24325=CARTESIAN_POINT ( 'NONE',  ( -8.349714312657674498, 175.1744531367911293, 4.594050593750047540 ) ) ;
#24329=CARTESIAN_POINT ( 'NONE',  ( 176.4535474755452356, 256.1020709052521056, 8.255247991639031113 ) ) ;
#24330=CARTESIAN_POINT ( 'NONE',  ( 185.2609771608511835, 270.5205629937861431, -16.69046129513680299 ) ) ;
#24332=CARTESIAN_POINT ( 'NONE',  ( 19.47135178391741661, 191.2369531367911293, -4.594050593750048428 ) ) ;
#24336=CARTESIAN_POINT ( 'NONE',  ( 191.3041230083617563, 299.2985345825480863, -9.819045872446528378 ) ) ;
#24340=CARTESIAN_POINT ( 'NONE',  ( 186.5727140431293378, 296.2605864597566665, -8.800404970033115504 ) ) ;
#24341=CARTESIAN_POINT ( 'NONE',  ( 190.7335255870825108, 261.9646230305896779, -0.8058728106476181763 ) ) ;
#24344=CARTESIAN_POINT ( 'NONE',  ( 60.28305926085675992, 215.6115022471903160, -5.000000000000047962 ) ) ;
#24346=CARTESIAN_POINT ( 'NONE',  ( 203.4603280001158794, 270.1122314455482183, 6.026633026702996609 ) ) ;
#24347=CARTESIAN_POINT ( 'NONE',  ( 38.44315465527655107, 186.8768266524159856, -9.188101187500091527 ) ) ;
#24348=CARTESIAN_POINT ( 'NONE',  ( 193.0405099973349081, 283.7233392346411165, 17.77886865111357295 ) ) ;
#24350=CARTESIAN_POINT ( 'NONE',  ( 203.4761922537706482, 269.1684635965042958, -5.985248603416074786 ) ) ;
#24351=B_SPLINE_CURVE_WITH_KNOTS ( 'NONE', 3,
 ( #96363, #74035, #34043, #33530, #72554, #35516, #27435, #64427, #95389, #10736, #81659, #95877, #42113, #3158, #26929, #64933 ),
 .UNSPECIFIED., .F., .F.,
 ( 4, 2, 2, 2, 2, 2, 2, 4 ),
 ( 0.000000000000000000, 0.0004989544299106570078, 0.0007484316448658957397, 0.0009979088598211346885, 0.001247386074776373312, 0.001496863289731612152, 0.001746340504686851426, 0.001995817719642090267 ),
 .UNSPECIFIED. ) ;
#24352=CARTESIAN_POINT ( 'NONE',  ( 198.9225589249066957, 286.1030165008847916, -17.03502353404871883 ) ) ;
#24354=EDGE_CURVE ( 'NONE', #71770, #8790, #65069, .T. ) ;
#24355=CARTESIAN_POINT ( 'NONE',  ( 179.7389585068036979, 283.2694176073634935, 16.15404047216739514 ) ) ;
#24356=CARTESIAN_POINT ( 'NONE',  ( 202.4119438311506940, 279.2703662523446155, -15.60349858348900476 ) ) ;
#24357=CARTESIAN_POINT ( 'NONE',  ( 205.7858960462819766, 269.5612804690865687, -1.325532578154042351 ) ) ;
#24359=CARTESIAN_POINT ( 'NONE',  ( 163.3854574543125580, 247.6550818016845597, 10.82482370245618775 ) ) ;
#24360=CARTESIAN_POINT ( 'NONE',  ( 149.5390997184345281, 271.6376768999995761, -11.52989534384373016 ) ) ;
#24361=CARTESIAN_POINT ( 'NONE',  ( 175.3141911485210187, 257.2753051901946719, 11.72392066680403744 ) ) ;
#24364=ADVANCED_FACE ( 'NONE', ( #12459 ), #98562, .T. ) ;
#24369=CARTESIAN_POINT ( 'NONE',  ( 175.8132799389368017, 292.7022098518745565, -2.441052075075039518 ) ) ;
#24371=CARTESIAN_POINT ( 'NONE',  ( 150.6533415055477008, 269.7077535128032082, 14.84621632544246062 ) ) ;
#24372=CARTESIAN_POINT ( 'NONE',  ( 179.7438496854340997, 257.3540159337386513, -7.334582191190184730 ) ) ;
#24374=ORIENTED_EDGE ( 'NONE', *, *, #42172, .F. ) ;
#24375=CARTESIAN_POINT ( 'NONE',  ( 187.4378393846737367, 272.8763525007090607, -15.77460183161252516 ) ) ;
#24382=CARTESIAN_POINT ( 'NONE',  ( 190.6036479972031259, 300.5117928913073797, -0.6824572005520307405 ) ) ;
#24384=VERTEX_POINT ( 'NONE', #37227 ) ;
#24386=CARTESIAN_POINT ( 'NONE',  ( 162.1978965794471890, 266.5548187812856895, 17.22461409982334501 ) ) ;
#24387=ORIENTED_EDGE ( 'NONE', *, *, #93373, .F. ) ;
#24389=CARTESIAN_POINT ( 'NONE',  ( 159.5284711081640125, 254.3355781173132755, 15.34104435652608522 ) ) ;
#24391=CARTESIAN_POINT ( 'NONE',  ( 51.40603854846860798, 209.6744531367911293, 4.594050593750047540 ) ) ;
#24392=ORIENTED_EDGE ( 'NONE', *, *, #59171, .F. ) ;
#24394=CARTESIAN_POINT ( 'NONE',  ( 70.22199747613832699, 222.8967562850346837, -4.648177544792955347E-16 ) ) ;
#24395=CARTESIAN_POINT ( 'NONE',  ( 87.83349241520130590, 231.5177522451419350, 5.000000000000046185 ) ) ;
#24397=ORIENTED_EDGE ( 'NONE', *, *, #32916, .T. ) ;
#24399=CARTESIAN_POINT ( 'NONE',  ( 146.8881680668833951, 276.2292252078784145, 4.973452195244782104 ) ) ;
#24402=CARTESIAN_POINT ( 'NONE',  ( 174.4278075863048230, 260.9700190746071371, -14.02905432283994536 ) ) ;
#24403=CARTESIAN_POINT ( 'NONE',  ( 170.7059362337859056, 275.4258791682946139, -16.58347944357980452 ) ) ;
#24404=CARTESIAN_POINT ( 'NONE',  ( 161.8150574665248200, 250.3750943687383881, -13.25074899737357903 ) ) ;
#24405=CARTESIAN_POINT ( 'NONE',  ( 147.3715240516018810, 275.3920280842035595, -3.728968767617475866 ) ) ;
#24406=CARTESIAN_POINT ( 'NONE',  ( 148.9228818358559749, 272.7049975811580680, 12.13823097167056275 ) ) ;
#24409=CARTESIAN_POINT ( 'NONE',  ( 206.0041637419966776, 273.8373171585603814, 11.66586596407113596 ) ) ;
#24411=DIRECTION ( 'NONE',  ( -0.8660254037844359321, -0.5000000000000051070, -0.000000000000000000 ) ) ;
#24412=CARTESIAN_POINT ( 'NONE',  ( 163.7587049410067266, 247.0085981909329576, -6.137518685179130351 ) ) ;
#24413=CARTESIAN_POINT ( 'NONE',  ( 115.3025621453804490, 243.5024278399160949, 9.188101187500095079 ) ) ;
#24415=CARTESIAN_POINT ( 'NONE',  ( 148.9845638001402506, 272.5981612851071532, -12.53752629571579291 ) ) ;
#24417=EDGE_CURVE ( 'NONE', #39680, #39791, #44422, .T. ) ;
#24418=CARTESIAN_POINT ( 'NONE',  ( 154.8786460229866577, 262.3893114111486398, -18.06164891362396929 ) ) ;
#24419=CARTESIAN_POINT ( 'NONE',  ( 204.7986527064648214, 275.9253235211867263, 14.74587861556245905 ) ) ;
#24422=CARTESIAN_POINT ( 'NONE',  ( 174.8210708869210350, 252.8123362264541640, 5.084827073808857456 ) ) ;
#24426=CARTESIAN_POINT ( 'NONE',  ( 182.3683164725543691, 259.8255612630188693, 10.74697378040428752 ) ) ;
#24427=CARTESIAN_POINT ( 'NONE',  ( 206.3869432407897193, 272.3943931181467519, 8.042875945707256946 ) ) ;
#24428=CARTESIAN_POINT ( 'NONE',  ( 129.0235653626489238, 254.4869531367911577, 4.594050593750046652 ) ) ;
#24430=CARTESIAN_POINT ( 'NONE',  ( 189.7153962340875637, 294.7489371240931746, -12.64634207402519550 ) ) ;
#24431=CARTESIAN_POINT ( 'NONE',  ( 189.1446688698201513, 299.4652302210857329, 4.877423590139457588 ) ) ;
#24432=CARTESIAN_POINT ( 'NONE',  ( 187.3746306850530914, 281.3025677867038326, -17.17837978889408745 ) ) ;
#24434=CARTESIAN_POINT ( 'NONE',  ( 47.69862761034023180, 198.3458772461660544, 9.188101187500095079 ) ) ;
#24436=ORIENTED_EDGE ( 'NONE', *, *, #6261, .F. ) ;
#24444=CARTESIAN_POINT ( 'NONE',  ( 178.4695799393319078, 261.1737003364913221, 12.23121311639275888 ) ) ;
#24445=CARTESIAN_POINT ( 'NONE',  ( 118.5773942495489166, 239.2677522451418497, 10.00000000000009592 ) ) ;
#24448=CARTESIAN_POINT ( 'NONE',  ( 190.0515794655415789, 301.4680036374047063, -1.296825456579539626 ) ) ;
#24449=CARTESIAN_POINT ( 'NONE',  ( 37.27951979288245354, 183.1423013555409796, -4.594050593750043987 ) ) ;
#24454=CARTESIAN_POINT ( 'NONE',  ( 193.8354046899084153, 268.4885937380259406, 12.87375928640720524 ) ) ;
#24455=CARTESIAN_POINT ( 'NONE',  ( 62.64658692180388755, 213.6427522451419065, -10.00000000000009415 ) ) ;
#24457=CARTESIAN_POINT ( 'NONE',  ( 184.6285283030370863, 257.2480713052503916, 1.399339441625289560 ) ) ;
#24458=CARTESIAN_POINT ( 'NONE',  ( 175.1378461883211912, 279.3152656845848583, 16.63146252814350134 ) ) ;
#24459=CARTESIAN_POINT ( 'NONE',  ( 162.1895243271695790, 251.7827224420559560, -12.96073478808974144 ) ) ;
#24460=ORIENTED_EDGE ( 'NONE', *, *, #34805, .F. ) ;
#24461=EDGE_CURVE ( 'NONE', #32812, #56545, #11791, .T. ) ;
#24462=CARTESIAN_POINT ( 'NONE',  ( 161.7897299554012136, 267.2878364038729160, 16.48459245643600113 ) ) ;
#24463=CARTESIAN_POINT ( 'NONE',  ( 34.30229714732369217, 180.6115022471902023, -5.000000000000041744 ) ) ;
#24464=CARTESIAN_POINT ( 'NONE',  ( 152.3797953885492973, 246.5327760586659451, 1.948934522072303157E-15 ) ) ;
#24465=CARTESIAN_POINT ( 'NONE',  ( 202.2773826701151165, 280.2922913237452462, 16.62862787739668846 ) ) ;
#24466=CARTESIAN_POINT ( 'NONE',  ( -10.59588092978231266, 170.8149278399160949, -9.188101187500095079 ) ) ;
#24468=CARTESIAN_POINT ( 'NONE',  ( 170.3726117846000534, 263.6551374743509655, 15.82174270005026706 ) ) ;
#24469=CARTESIAN_POINT ( 'NONE',  ( 185.3682712903229515, 260.2001122261074784, 7.152103282995272870 ) ) ;
#24470=CARTESIAN_POINT ( 'NONE',  ( 164.3493441216711517, 245.9855811210807417, 1.722120810491653664 ) ) ;
#24471=CARTESIAN_POINT ( 'NONE',  ( 183.6513914873445117, 258.0677590912166579, -2.301000200388038763 ) ) ;
#24475=CARTESIAN_POINT ( 'NONE',  ( 174.6066048939933921, 262.0940252294753918, 15.79829227059981278 ) ) ;
#24477=CARTESIAN_POINT ( 'NONE',  ( 153.1483233301889015, 277.9035912389402938, -6.076691557333878002 ) ) ;
#24480=EDGE_CURVE ( 'NONE', #73115, #39719, #23966, .T. ) ;
#24481=CARTESIAN_POINT ( 'NONE',  ( 206.0870578475358172, 273.6937403561189512, -10.07771901274806581 ) ) ;
#24482=DIRECTION ( 'NONE',  ( -0.8660254037844387076, -0.4999999999999998890, -0.000000000000000000 ) ) ;
#24484=CARTESIAN_POINT ( 'NONE',  ( 191.5950718126193806, 298.2341233548021933, 8.974193154413244500 ) ) ;
#24487=CARTESIAN_POINT ( 'NONE',  ( 155.2098048002210930, 261.8157275836062468, 16.98811268941991059 ) ) ;
#24488=ORIENTED_EDGE ( 'NONE', *, *, #67135, .T. ) ;
#24492=ORIENTED_EDGE ( 'NONE', *, *, #63979, .F. ) ;
#24493=CARTESIAN_POINT ( 'NONE',  ( 162.7200750364849284, 284.8437062156138495, 3.896873972031206446 ) ) ;
#24496=FACE_OUTER_BOUND ( 'NONE', #78488, .T. ) ;
#24498=CARTESIAN_POINT ( 'NONE',  ( 196.5114383562724072, 290.2791998289336561, -17.87308875047256862 ) ) ;
#24500=ORIENTED_EDGE ( 'NONE', *, *, #68305, .F. ) ;
#24501=CARTESIAN_POINT ( 'NONE',  ( 161.1611771195837548, 251.5076483517112536, 14.17749514252127163 ) ) ;
#24503=CARTESIAN_POINT ( 'NONE',  ( 151.4327733764141612, 268.3577379114237829, 14.90862905801242100 ) ) ;
#24507=VERTEX_POINT ( 'NONE', #2749 ) ;
#24512=CARTESIAN_POINT ( 'NONE',  ( 208.3152833949211526, 269.8343404973242059, 2.763633873278860342 ) ) ;
#24514=CARTESIAN_POINT ( 'NONE',  ( 168.8557204221072539, 272.7203768975772959, 16.03607575273253971 ) ) ;
#24515=CARTESIAN_POINT ( 'NONE',  ( 205.8889072768004951, 273.5716727396786041, -9.812782715980612025 ) ) ;
#24517=CARTESIAN_POINT ( 'NONE',  ( 194.8598199529639317, 293.1398868181796615, -15.91766051364927570 ) ) ;
#24520=CARTESIAN_POINT ( 'NONE',  ( 167.1168391014803376, 246.9550111041327796, 1.953063234077585086 ) ) ;
#24522=CARTESIAN_POINT ( 'NONE',  ( 189.6768609436964539, 274.4077930505946483, -17.07046811116321550 ) ) ;
#24523=CARTESIAN_POINT ( 'NONE',  ( -22.42236680055709641, 157.8615022471902591, 0.000000000000000000 ) ) ;
#24524=CARTESIAN_POINT ( 'NONE',  ( 207.0336018875206605, 271.6198296197399031, 5.247267533735946898 ) ) ;
#24526=DIRECTION ( 'NONE',  ( -0.8660254037844387076, -0.4999999999999998890, -0.000000000000000000 ) ) ;
#24527=CARTESIAN_POINT ( 'NONE',  ( 168.2539250261779955, 257.0764780862120347, -14.46934504387492559 ) ) ;
#24528=CARTESIAN_POINT ( 'NONE',  ( 159.8946522441011382, 253.7013337850969492, -16.68230890105693121 ) ) ;
#24532=ORIENTED_EDGE ( 'NONE', *, *, #97966, .F. ) ;
#24533=CARTESIAN_POINT ( 'NONE',  ( 193.8431759644069530, 294.9007658595700150, -14.61944437866594093 ) ) ;
#24535=CARTESIAN_POINT ( 'NONE',  ( 164.9779129355220562, 244.8968679994381148, -1.771286574179712803 ) ) ;
#24536=CARTESIAN_POINT ( 'NONE',  ( 19.41748551623073027, 172.0177522451417929, 5.000000000000051514 ) ) ;
#24537=CARTESIAN_POINT ( 'NONE',  ( 83.80088808272149947, 225.3149278399160949, 9.188101187500093303 ) ) ;
#24540=CARTESIAN_POINT ( 'NONE',  ( 167.9211111253673323, 249.4040118433879627, 8.061254949035708606 ) ) ;
#24541=CARTESIAN_POINT ( 'NONE',  ( 166.9589859915207626, 278.2346298421052779, -13.39139289067553307 ) ) ;
#24542=CARTESIAN_POINT ( 'NONE',  ( 3.882894515797516988, 182.2369531367911009, -4.594050593750048428 ) ) ;
#24544=CARTESIAN_POINT ( 'NONE',  ( 161.1089126327036354, 251.5981730984191529, 13.95161017039218976 ) ) ;
#24545=EDGE_LOOP ( 'NONE', ( #81624, #4991, #12423, #59377 ) ) ;
#24548=DIRECTION ( 'NONE',  ( 0.8660254037844387076, 0.4999999999999998890, 0.000000000000000000 ) ) ;
#24556=CARTESIAN_POINT ( 'NONE',  ( 27.23877744593285755, 186.5333772461660544, 9.188101187500095079 ) ) ;
#24557=CARTESIAN_POINT ( 'NONE',  ( 75.70913676221920241, 214.5177522451418497, -10.00000000000009592 ) ) ;
#24559=ORIENTED_EDGE ( 'NONE', *, *, #83954, .F. ) ;
#24561=DIRECTION ( 'NONE',  ( 0.5000000000000048850, -0.8660254037844358210, 0.000000000000000000 ) ) ;
#24563=CARTESIAN_POINT ( 'NONE',  ( 199.0805333989439134, 267.9591265660101271, 8.967019654618759716 ) ) ;
#24564=CARTESIAN_POINT ( 'NONE',  ( 194.4889937320412230, 293.7821766735966662, 14.99892588346621380 ) ) ;
#24565=CARTESIAN_POINT ( 'NONE',  ( 161.3145230519951951, 251.2420454056404822, -14.44869077440025151 ) ) ;
#24566=CARTESIAN_POINT ( 'NONE',  ( 186.1229685699691458, 283.4085544576373081, 17.19819074553363336 ) ) ;
#24567=CARTESIAN_POINT ( 'NONE',  ( 147.9791529310278122, 274.3395839928920168, -7.789432462804474433 ) ) ;
#24568=CARTESIAN_POINT ( 'NONE',  ( 192.0985965716629096, 264.9293924627144747, 7.771810996922307702 ) ) ;
#24569=CARTESIAN_POINT ( 'NONE',  ( 171.7318633942313681, 279.6244332910715116, 14.38819572014175030 ) ) ;
#24570=CARTESIAN_POINT ( 'NONE',  ( 176.1037769756363218, 256.5739391985542852, -11.09083365203573379 ) ) ;
#24571=CARTESIAN_POINT ( 'NONE',  ( 147.3047606266276546, 275.5076657283461827, -0.02269072295920609994 ) ) ;
#24572=CARTESIAN_POINT ( 'NONE',  ( 189.8480911035503880, 301.8204558191226283, -0.8992086515915015399 ) ) ;
#24574=B_SPLINE_CURVE_WITH_KNOTS ( 'NONE', 3,
 ( #19769, #58241, #65351, #20766, #5547, #96290, #42533, #13169, #96800, #89702, #50152, #26859, #34939, #20262, #5058, #66841, #35447, #51136, #35938, #4049, #82098, #51654, #89221, #88715, #36432, #4546, #88215, #57735, #44023, #73466, #12671, #73961, #28338, #97282, #66349, #11671, #19284, #67339, #72981, #81104, #43022, #82603, #27359, #97768, #65834, #18767, #59216, #90190, #50638, #27849 ),
 .UNSPECIFIED., .F., .F.,
 ( 4, 2, 2, 2, 2, 2, 2, 2, 2, 2, 2, 2, 2, 2, 2, 2, 2, 2, 2, 2, 2, 2, 2, 2, 4 ),
 ( 0.0005972733594740094231, 0.001599206768350971541, 0.001849690120570192473, 0.002100173472789413406, 0.002225415148898984841, 0.002350656825008556276, 0.002475898501118127711, 0.002601140177227699146, 0.002851623529446945665, 0.003102106881666191751, 0.003603073586104625376, 0.004605006994981492192, 0.005606940403858359442, 0.006107907108296836869, 0.006358390460515996219, 0.006608873812735157303, 0.006671494650789984437, 0.006734115488844811571, 0.006796736326899638705, 0.006859357164954464972, 0.007109840517173513300, 0.007610807221611471177, 0.008111773926049430788, 0.008362257278268407992, 0.008612740630487385196 ),
 .UNSPECIFIED. ) ;
#24575=CARTESIAN_POINT ( 'NONE',  ( 153.1538868596604175, 267.0205913518451553, -16.30221171337800712 ) ) ;
#24576=EDGE_CURVE ( 'NONE', #99135, #45081, #1014, .T. ) ;
#24578=CARTESIAN_POINT ( 'NONE',  ( 111.6762543149156386, 235.2833772461660544, -9.188101187500095079 ) ) ;
#24580=CARTESIAN_POINT ( 'NONE',  ( 151.4384131719918685, 268.3479694989391078, 14.98299707687648841 ) ) ;
#24581=CYLINDRICAL_SURFACE ( 'NONE', #24150, 10.00000000000010658 ) ;
#24582=CARTESIAN_POINT ( 'NONE',  ( 157.8360072705708603, 257.2670114739976839, 17.12122855844125269 ) ) ;
#24583=CARTESIAN_POINT ( 'NONE',  ( 150.8312752086160344, 269.3995632987097224, -13.81131374255177491 ) ) ;
#24585=CARTESIAN_POINT ( 'NONE',  ( 149.3629284598386278, 271.9428144707212027, -12.99253781774931049 ) ) ;
#24587=CARTESIAN_POINT ( 'NONE',  ( 203.7562161628329420, 276.6852326455151569, 14.03846531369241646 ) ) ;
#24589=ORIENTED_EDGE ( 'NONE', *, *, #50395, .T. ) ;
#24590=CYLINDRICAL_SURFACE ( 'NONE', #55378, 17.82106496071139645 ) ;
#24592=CARTESIAN_POINT ( 'NONE',  ( 179.0770803138376550, 280.8245948471085285, 16.18081609326188897 ) ) ;
#24593=CARTESIAN_POINT ( 'NONE',  ( 159.3184698695538657, 279.9366817407362191, 9.858215026386687896 ) ) ;
#24596=B_SPLINE_SURFACE_WITH_KNOTS ( 'NONE', 3, 1, ( 
 ( #69130, #100059 ),
 ( #30644, #60523 ),
 ( #61531, #23021 ),
 ( #53914, #84875 ),
 ( #732, #68633 ),
 ( #21555, #13950 ),
 ( #15416, #44832 ),
 ( #75765, #38726 ),
 ( #69630, #17957 ),
 ( #25028, #86901 ),
 ( #63532, #80284 ),
 ( #33138, #94474 ),
 ( #54928, #9340 ),
 ( #94983, #17436 ),
 ( #95504, #64038 ),
 ( #49344, #48343 ),
 ( #85906, #62512 ),
 ( #1242, #16432 ),
 ( #40212, #2765 ),
 ( #2256, #47815 ),
 ( #79290, #8833 ),
 ( #9862, #40721 ),
 ( #25544, #63034 ),
 ( #56432, #71666 ),
 ( #55907, #41727 ),
 ( #87427, #39702 ),
 ( #71158, #41219 ),
 ( #1757, #78753 ),
 ( #32636, #48854 ),
 ( #33655, #78253 ),
 ( #93477, #70632 ),
 ( #32125, #24029 ),
 ( #93978, #55411 ),
 ( #79787, #10352 ) ),
 .UNSPECIFIED., .T., .F., .F.,
 ( 4, 2, 2, 2, 2, 2, 2, 2, 2, 2, 2, 2, 2, 2, 2, 2, 4 ),
 ( 2, 2 ),
 ( 0.000000000000000000, 0.06250000000000000000, 0.1250000000000000000, 0.1875000000000000000, 0.2500000000000000000, 0.3125000000000000000, 0.3750000000000000000, 0.4375000000000000000, 0.5000000000000000000, 0.5625000000000000000, 0.6250000000000000000, 0.6875000000000000000, 0.7500000000000000000, 0.8125000000000000000, 0.8750000000000000000, 0.9375000000000000000, 1.000000000000000000 ),
 ( 0.000000000000000000, 1.000000000000000000 ),
 .UNSPECIFIED. ) ;
#24597=B_SPLINE_CURVE_WITH_KNOTS ( 'NONE', 3,
 ( #97648, #73829, #80474, #35315 ),
 .UNSPECIFIED., .F., .F.,
 ( 4, 4 ),
 ( 0.005858324926681961892, 0.01085025600539994174 ),
 .UNSPECIFIED. ) ;
#24599=CARTESIAN_POINT ( 'NONE',  ( 188.8764293144468240, 259.6972905960182061, 3.583694637520717041 ) ) ;
#24602=CARTESIAN_POINT ( 'NONE',  ( 148.0649146996763363, 274.8219941347795157, 6.013499275595850513 ) ) ;
#24609=CARTESIAN_POINT ( 'NONE',  ( 164.0406800301222461, 279.3727068695090452, 12.06992682371145698 ) ) ;
#24610=FACE_OUTER_BOUND ( 'NONE', #36574, .T. ) ;
#24611=CARTESIAN_POINT ( 'NONE',  ( 11.35262394703597977, 187.3615022471903160, 5.000000000000046185 ) ) ;
#24614=CARTESIAN_POINT ( 'NONE',  ( 188.7896788447123697, 293.5392900447417333, 12.71403846335633503 ) ) ;
#24615=CARTESIAN_POINT ( 'NONE',  ( 60.96635096964421763, 217.5530062829863027, -4.648177544792955347E-16 ) ) ;
#24616=CARTESIAN_POINT ( 'NONE',  ( 165.3469776539213001, 255.6859576650746817, 15.29061740545938619 ) ) ;
#24617=CARTESIAN_POINT ( 'NONE',  ( 121.5128116872495525, 229.4155109091896065, 2.679491924311254714 ) ) ;
#24621=CARTESIAN_POINT ( 'NONE',  ( 175.2353567823311948, 258.4903666904938859, 12.97297848141165666 ) ) ;
#24624=EDGE_CURVE ( 'NONE', #33264, #38319, #4604, .T. ) ;
#24629=CARTESIAN_POINT ( 'NONE',  ( 182.7519487852241582, 280.2897188732222844, -16.10892874468358116 ) ) ;
#24630=B_SPLINE_CURVE_WITH_KNOTS ( 'NONE', 3,
 ( #23759, #16174, #20560, #89505 ),
 .UNSPECIFIED., .F., .F.,
 ( 4, 4 ),
 ( 0.03306110125414005868, 0.04197919891026069550 ),
 .UNSPECIFIED. ) ;
#24631=CARTESIAN_POINT ( 'NONE',  ( 206.1142978005191821, 273.6465593735555899, -11.17423994621995753 ) ) ;
#24632=CARTESIAN_POINT ( 'NONE',  ( 190.2843330081942099, 301.0648626758887758, 1.921572748488094229 ) ) ;
#24633=CARTESIAN_POINT ( 'NONE',  ( 196.2637273998480794, 284.5407699133422170, -17.38889955844871338 ) ) ;
#24635=CARTESIAN_POINT ( 'NONE',  ( 180.3459549195497118, 261.9372799863696741, 13.82492882169983872 ) ) ;
#24638=CARTESIAN_POINT ( 'NONE',  ( 153.9013169898294962, 279.6173177660232341, 2.183373660223292934 ) ) ;
#24639=CARTESIAN_POINT ( 'NONE',  ( 119.6866422041566693, 252.1589784336661637, -6.496448406907675876E-16 ) ) ;
#24640=CARTESIAN_POINT ( 'NONE',  ( 185.8243919191459099, 262.2525832573476237, -9.042311947975223418 ) ) ;
#24647=CARTESIAN_POINT ( 'NONE',  ( 190.4718661473337136, 300.2809275374601725, 2.324064312516258557 ) ) ;
#24649=CARTESIAN_POINT ( 'NONE',  ( 159.8822213732012756, 255.7228646850775533, -16.63148941946954196 ) ) ;
#24650=CARTESIAN_POINT ( 'NONE',  ( 173.6948184163663313, 287.1953014397127504, -9.575283291849126854 ) ) ;
#24651=B_SPLINE_CURVE_WITH_KNOTS ( 'NONE', 3,
 ( #72776, #13795, #89019, #34731, #19065, #48949, #65138, #41829, #72264, #10958, #49938, #81386, #2870, #27152, #3368, #33759, #80899, #64650, #58037, #5696, #64139, #11470, #42324, #50431, #11954, #3847, #95600, #90852, #26147, #98421, #56533, #21406, #73253, #52289, #57025, #65630, #42812, #44674, #75120, #88007, #34242, #6195, #96086, #67491, #29014, #59886, #75607, #95089 ),
 .UNSPECIFIED., .F., .F.,
 ( 4, 2, 2, 2, 2, 2, 2, 2, 2, 2, 2, 2, 2, 2, 2, 2, 2, 2, 2, 2, 2, 2, 2, 4 ),
 ( 0.001944024153977080144, 0.002388868632841927454, 0.002611290872274335713, 0.002833713111706743538, 0.002944924231422909287, 0.003056135351139075904, 0.003167346470855241652, 0.003278557590571408269, 0.003500979830003698133, 0.003723402069435987997, 0.004613091027165332203, 0.005502779984894675541, 0.006392468942624018879, 0.006837313421488733049, 0.007282157900353448086, 0.007393369020069691898, 0.007448974579927781711, 0.007504580139785870657, 0.007615791259502062427, 0.007727002379218254197, 0.008171846858083097603, 0.008394269097515514103, 0.008616691336947932336, 0.009061535815812862479 ),
 .UNSPECIFIED. ) ;
#24652=CARTESIAN_POINT ( 'NONE',  ( 174.9664910165346328, 282.3800467726322836, 14.52565441293174864 ) ) ;
#24653=CARTESIAN_POINT ( 'NONE',  ( 194.7312017232699475, 291.7187946681755761, 16.04046780675849604 ) ) ;
#24654=VERTEX_POINT ( 'NONE', #96469 ) ;
#24655=CARTESIAN_POINT ( 'NONE',  ( 148.2670916631250861, 273.8408594794321971, -7.980554973576580835 ) ) ;
#24656=CARTESIAN_POINT ( 'NONE',  ( 149.8083888948594335, 271.5779462620446338, 11.70101749353969645 ) ) ;
#24658=CARTESIAN_POINT ( 'NONE',  ( 189.1549977934801632, 266.7951475240158175, -11.86923019693644576 ) ) ;
#24659=B_SPLINE_CURVE_WITH_KNOTS ( 'NONE', 3,
 ( #22303, #38487, #47094, #68398, #37489, #84158, #30401, #85144, #38987, #21805, #14704, #15690 ),
 .UNSPECIFIED., .F., .F.,
 ( 4, 2, 2, 2, 2, 4 ),
 ( 0.001501127264142293862, 0.001572989943943600049, 0.001644852623744906019, 0.001788577983347369423, 0.002076028702552448237, 0.002650930140962551654 ),
 .UNSPECIFIED. ) ;
#24660=CARTESIAN_POINT ( 'NONE',  ( 160.0256511895230460, 279.1764180042833345, 10.79622904626536695 ) ) ;
#24661=CARTESIAN_POINT ( 'NONE',  ( 152.2282464967177873, 266.9799380510025912, -15.44817667187453658 ) ) ;
#24664=CARTESIAN_POINT ( 'NONE',  ( 164.6777298217157579, 283.8828607077460333, -6.799046367663557966 ) ) ;
#24665=CARTESIAN_POINT ( 'NONE',  ( 151.5210055037418613, 275.0213185945912642, -8.640155065745233287 ) ) ;
#24669=CARTESIAN_POINT ( 'NONE',  ( 204.6823371430232896, 272.9704135290961062, -9.754921121218281144 ) ) ;
#24670=CARTESIAN_POINT ( 'NONE',  ( 187.5160213568918834, 263.2186159667169818, -9.042077419483060652 ) ) ;
#24673=EDGE_CURVE ( 'NONE', #80596, #84236, #55354, .T. ) ;
#24674=CARTESIAN_POINT ( 'NONE',  ( 4.695053651895191749, 183.5177522451419350, 5.000000000000046185 ) ) ;
#24675=CARTESIAN_POINT ( 'NONE',  ( 152.6845319923753834, 266.1896283897672220, 17.20844521882669653 ) ) ;
#24679=CARTESIAN_POINT ( 'NONE',  ( -4.289699588770600869, 159.1423013555410080, -4.594050593750043987 ) ) ;
#24680=EDGE_CURVE ( 'NONE', #81902, #49338, #33019, .T. ) ;
#24681=CARTESIAN_POINT ( 'NONE',  ( 91.10780387927019319, 235.6589784336661353, -6.496448406907675876E-16 ) ) ;
#24684=CARTESIAN_POINT ( 'NONE',  ( 182.9336300665386830, 294.1347523882549808, -7.906671405285472076 ) ) ;
#24688=CARTESIAN_POINT ( 'NONE',  ( 38.47004439948830168, 203.0177522451419350, 5.000000000000046185 ) ) ;
#24691=CARTESIAN_POINT ( 'NONE',  ( 161.3809022727548950, 251.1270732227178826, 12.88239761679595219 ) ) ;
#24692=CARTESIAN_POINT ( 'NONE',  ( -7.501470784735642106, 173.1427522451419350, -10.00000000000009592 ) ) ;
#24694=CARTESIAN_POINT ( 'NONE',  ( 196.4677102463732012, 290.3549391369982686, 16.45225250689336249 ) ) ;
#24697=B_SPLINE_CURVE_WITH_KNOTS ( 'NONE', 3,
 ( #63210, #23691, #76902, #61697, #24705, #39883, #70819, #55097, #7500, #24216, #75062, #46493, #54588, #55588, #100232, #98365, #67434, #77429, #44619, #93652, #92649, #93141, #38900, #54090, #47012, #1427, #8027, #28953, #69311, #85570, #5639, #36532, #86084, #86571, #16608, #32308, #21349, #47504, #52234, #69804, #83178, #31303, #78431, #9011, #94152, #30817, #31793, #62191, #72340, #9532, #2946, #58105 ),
 .UNSPECIFIED., .F., .F.,
 ( 4, 2, 2, 2, 2, 2, 2, 2, 2, 2, 2, 2, 2, 2, 2, 2, 2, 2, 2, 2, 2, 2, 2, 2, 2, 4 ),
 ( 0.0007535677484271811411, 0.0009585266667888987444, 0.001061006125969736784, 0.001163485585150574823, 0.001265965044331413079, 0.001368444503512250901, 0.001573403421873828534, 0.001983321258597046249, 0.002393239095320263531, 0.003213074768766698095, 0.004032910442213133093, 0.004852746115659568524, 0.005262663952382786239, 0.005467622870744357801, 0.005570102329925144015, 0.005621342059515537122, 0.005672581789105929362, 0.005723821518696322469, 0.005775061248286715576, 0.005877540707467618884, 0.006082499625829548666, 0.006287458544191479315, 0.006492417462553409097, 0.006697376380915339746, 0.006902335299277270395, 0.007312253136001233174 ),
 .UNSPECIFIED. ) ;
#24698=CARTESIAN_POINT ( 'NONE',  ( 41.69040282370318096, 201.0024278399160664, -9.188101187500093303 ) ) ;
#24699=CARTESIAN_POINT ( 'NONE',  ( 58.76725448063633195, 213.9244531367911577, -4.594050593750046652 ) ) ;
#24702=CARTESIAN_POINT ( 'NONE',  ( 167.2670237296246114, 259.8210226229481350, 16.08327144298513289 ) ) ;
#24703=CARTESIAN_POINT ( 'NONE',  ( 198.5718581478091096, 286.2919326846333661, -17.01494721233840934 ) ) ;
#24705=CARTESIAN_POINT ( 'NONE',  ( 200.1987971015728078, 270.8785103762743915, -11.50719176782677522 ) ) ;
#24707=CARTESIAN_POINT ( 'NONE',  ( 198.5954523381739989, 286.6695817285962562, -18.45134152028667174 ) ) ;
#24710=CARTESIAN_POINT ( 'NONE',  ( 64.04520420253652446, 195.5327760586659451, 1.948934522072302763E-15 ) ) ;
#24713=CARTESIAN_POINT ( 'NONE',  ( 159.3767386493506137, 254.5983864451355032, 15.47015898230477760 ) ) ;
#24715=CARTESIAN_POINT ( 'NONE',  ( 153.7598317759031374, 264.3271545313291426, 16.52601577908147235 ) ) ;
#24717=CARTESIAN_POINT ( 'NONE',  ( 113.5436215935997808, 236.3615022471902307, -10.00000000000009592 ) ) ;
#24718=( BOUNDED_CURVE ( )  B_SPLINE_CURVE ( 2, ( #11723, #35500, #65895, #27418, #80656, #34993, #80154, #73032, #43076 ),
 .UNSPECIFIED., .F., .T. ) 
 B_SPLINE_CURVE_WITH_KNOTS ( ( 3, 2, 2, 2, 3 ),
 ( 0.8830645161290322509, 0.8844086021505376261, 0.8870967741935483764, 0.8897849462365591267, 0.8911290322580645018 ),
 .UNSPECIFIED. ) 
 CURVE ( )  GEOMETRIC_REPRESENTATION_ITEM ( )  RATIONAL_B_SPLINE_CURVE ( ( 0.9330127018922194093, 0.9330127018922194093, 1.000000000000000000, 0.8660254037844387076, 1.000000000000000000, 0.8660254037844387076, 1.000000000000000000, 0.9330127018922194093, 0.9330127018922194093 ) ) 
 REPRESENTATION_ITEM ( '' )  );
#24720=CARTESIAN_POINT ( 'NONE',  ( 164.8251969117060298, 245.1613799118173063, -1.508678420156898348 ) ) ;
#24721=ORIENTED_EDGE ( 'NONE', *, *, #8927, .F. ) ;
#24723=CARTESIAN_POINT ( 'NONE',  ( 187.7017978076716815, 273.1500586230484373, 15.64325622808618732 ) ) ;
#24725=CARTESIAN_POINT ( 'NONE',  ( 159.2536436069973718, 254.8115933126508992, -15.76697951715411250 ) ) ;
#24726=CARTESIAN_POINT ( 'NONE',  ( 186.9535536427556508, 276.6359796364028512, -17.38156364443241841 ) ) ;
#24729=CARTESIAN_POINT ( 'NONE',  ( 177.2873494991416408, 253.1734583796121854, -0.2633482349297172065 ) ) ;
#24732=CARTESIAN_POINT ( 'NONE',  ( 194.3177355571849318, 294.0788045336591381, -15.93712594727561616 ) ) ;
#24733=CARTESIAN_POINT ( 'NONE',  ( 164.3625597711517230, 265.6729452914248668, -17.82104740451561753 ) ) ;
#24739=CARTESIAN_POINT ( 'NONE',  ( 30.81219509745235285, 177.0494855054051584, -2.679491924311248496 ) ) ;
#24745=CARTESIAN_POINT ( 'NONE',  ( -11.66375754446418611, 175.6199935810941213, 2.679491924311258266 ) ) ;
#24747=CARTESIAN_POINT ( 'NONE',  ( 171.0749840207226384, 284.6259473909062194, 10.82415887584089020 ) ) ;
#24751=CARTESIAN_POINT ( 'NONE',  ( 154.8679462054080318, 262.4078440388265676, 17.98338675682672871 ) ) ;
#24752=CARTESIAN_POINT ( 'NONE',  ( 185.3899931942047772, 292.5462500827383110, -10.78127527295067800 ) ) ;
#24753=CARTESIAN_POINT ( 'NONE',  ( 157.8696211474012330, 257.2087905314882619, -17.27527248276125604 ) ) ;
#24754=CARTESIAN_POINT ( 'NONE',  ( 143.8006444583684242, 244.6423013555409796, -4.594050593750043987 ) ) ;
#24755=CARTESIAN_POINT ( 'NONE',  ( 206.4640281649579947, 270.6250285429839550, 2.495114648528401258 ) ) ;
#24758=CARTESIAN_POINT ( 'NONE',  ( 83.80088808272151368, 225.3149278399160949, 9.188101187500093303 ) ) ;
#24760=CARTESIAN_POINT ( 'NONE',  ( 151.0778907302193943, 268.9724126853576536, 15.84769371787143832 ) ) ;
#24763=CARTESIAN_POINT ( 'NONE',  ( 156.7217004655723258, 259.1970474754747897, -17.29079717987055886 ) ) ;
#24765=EDGE_LOOP ( 'NONE', ( #5711, #41744, #78602 ) ) ;
#24768=CARTESIAN_POINT ( 'NONE',  ( 191.0862225170008628, 299.6759493045793192, -9.402218231374108726 ) ) ;
#24770=CYLINDRICAL_SURFACE ( 'NONE', #33853, 17.82106496071139645 ) ;
#24771=CARTESIAN_POINT ( 'NONE',  ( 207.7117873102786518, 270.8796263780940308, 1.712754233133884085 ) ) ;
#24772=CARTESIAN_POINT ( 'NONE',  ( 74.78872445064843077, 223.1744531367911293, 4.594050593750047540 ) ) ;
#24775=CARTESIAN_POINT ( 'NONE',  ( 200.6420049547404005, 283.1248486163401594, -18.32425536722374915 ) ) ;
#24776=VERTEX_POINT ( 'NONE', #36601 ) ;
#24781=ORIENTED_EDGE ( 'NONE', *, *, #4908, .F. ) ;
#24782=CARTESIAN_POINT ( 'NONE',  ( 71.12873073640183463, 200.3262482093457777, 3.021315404115420679E-15 ) ) ;
#24783=CARTESIAN_POINT ( 'NONE',  ( 185.2393081206536181, 260.2620773806470424, 6.297851702954142539 ) ) ;
#24784=CARTESIAN_POINT ( 'NONE',  ( 159.9788992190088948, 253.5554137441726255, -15.81862932303382330 ) ) ;
#24786=CARTESIAN_POINT ( 'NONE',  ( 186.0776724513669080, 289.8818082167753118, 14.70292991719237818 ) ) ;
#24787=CARTESIAN_POINT ( 'NONE',  ( 198.9243589141082396, 285.7204137842527985, -17.01128707248632566 ) ) ;
#24788=FACE_OUTER_BOUND ( 'NONE', #97273, .T. ) ;
#24792=CARTESIAN_POINT ( 'NONE',  ( 200.3134965941964651, 283.6938417875134064, 18.29802468362849766 ) ) ;
#24794=CARTESIAN_POINT ( 'NONE',  ( 187.9029328552566369, 266.2162208350674746, -11.92715153469220368 ) ) ;
#24797=CARTESIAN_POINT ( 'NONE',  ( 153.3543035181429559, 270.2748555357131295, 14.00895239929496583 ) ) ;
#24799=ORIENTED_EDGE ( 'NONE', *, *, #56103, .F. ) ;
#24805=CARTESIAN_POINT ( 'NONE',  ( 199.1489080723098084, 281.8162475621487033, -16.58710646079551054 ) ) ;
#24808=CARTESIAN_POINT ( 'NONE',  ( 171.8134125096551372, 274.9389237379870679, 17.04720683530305791 ) ) ;
#24811=CARTESIAN_POINT ( 'NONE',  ( 192.0630564889537482, 261.7319799974739567, 3.060561036580589978 ) ) ;
#24812=CARTESIAN_POINT ( 'NONE',  ( 195.4097585203640222, 265.1988717782938920, -7.668974602499345039 ) ) ;
#24813=CARTESIAN_POINT ( 'NONE',  ( -0.04102277327696322862, 170.7833772461660828, -9.188101187500095079 ) ) ;
#24816=ORIENTED_EDGE ( 'NONE', *, *, #60291, .T. ) ;
#24818=CARTESIAN_POINT ( 'NONE',  ( 174.8770607290546764, 255.3075393699999438, 8.411851435852767622 ) ) ;
#24821=FACE_OUTER_BOUND ( 'NONE', #97431, .T. ) ;
#24822=CARTESIAN_POINT ( 'NONE',  ( 29.16053163240333745, 178.4548013555409796, -4.594050593750042211 ) ) ;
#24825=CARTESIAN_POINT ( 'NONE',  ( 181.6112919552439848, 294.4992701536799586, 6.459004801064330614 ) ) ;
#24826=CARTESIAN_POINT ( 'NONE',  ( 173.5136117908628535, 272.6171107484045137, -16.35964596981252939 ) ) ;
#24829=B_SPLINE_SURFACE_WITH_KNOTS ( 'NONE', 3, 1, ( 
 ( #1852, #45918 ),
 ( #22648, #53533 ),
 ( #100164, #92582 ),
 ( #84974, #46421 ),
 ( #69733, #93063 ),
 ( #23618, #54511 ),
 ( #5698, #72265 ),
 ( #2357, #36588 ),
 ( #48950, #66992 ),
 ( #64140, #57528 ),
 ( #88504, #26645 ),
 ( #5209, #72777 ),
 ( #59374, #19066 ),
 ( #18557, #97918 ),
 ( #33760, #94575 ),
 ( #34243, #25131 ),
 ( #57026, #96087 ),
 ( #3369, #49939 ),
 ( #13322, #80900 ),
 ( #11471, #28493 ),
 ( #88008, #65139 ),
 ( #56013, #90351 ),
 ( #42325, #20931 ),
 ( #2871, #41321 ),
 ( #79885, #49436 ),
 ( #48444, #74634 ),
 ( #10448, #87009 ),
 ( #64651, #26148 ),
 ( #17536, #79390 ),
 ( #36091, #80389 ),
 ( #51813, #95601 ),
 ( #33236, #10959 ),
 ( #82755, #9956 ),
 ( #41830, #44185 ) ),
 .UNSPECIFIED., .T., .F., .F.,
 ( 4, 2, 2, 2, 2, 2, 2, 2, 2, 2, 2, 2, 2, 2, 2, 2, 4 ),
 ( 2, 2 ),
 ( 0.000000000000000000, 0.06250000000000000000, 0.1250000000000000000, 0.1875000000000000000, 0.2500000000000000000, 0.3125000000000000000, 0.3750000000000000000, 0.4375000000000000000, 0.5000000000000000000, 0.5625000000000000000, 0.6250000000000000000, 0.6875000000000000000, 0.7500000000000000000, 0.8125000000000000000, 0.8750000000000000000, 0.9375000000000000000, 1.000000000000000000 ),
 ( 0.000000000000000000, 1.000000000000000000 ),
 .UNSPECIFIED. ) ;
#24830=CARTESIAN_POINT ( 'NONE',  ( 186.6285282465448745, 296.1616521089468392, -8.750901477337695411 ) ) ;
#24831=CARTESIAN_POINT ( 'NONE',  ( 91.45997379709665154, 213.6115022471902023, -5.000000000000041744 ) ) ;
#24832=CARTESIAN_POINT ( 'NONE',  ( 70.24235140437789937, 201.3615022471901739, 5.000000000000051514 ) ) ;
#24834=CARTESIAN_POINT ( 'NONE',  ( 185.6462244317068553, 277.7986853771898268, -17.33779381876608028 ) ) ;
#24835=CARTESIAN_POINT ( 'NONE',  ( 203.4613517861610603, 269.9235832942454749, 6.857405767031560018 ) ) ;
#24836=CARTESIAN_POINT ( 'NONE',  ( 43.26059451170998216, 183.5327760586659451, 1.948934522072303157E-15 ) ) ;
#24837=CARTESIAN_POINT ( 'NONE',  ( 159.3169041484411537, 254.7020228407560580, 16.67170756419672628 ) ) ;
#24838=CARTESIAN_POINT ( 'NONE',  ( 203.1085490052368243, 270.1107938249242579, -6.431837059875057605 ) ) ;
#24843=CARTESIAN_POINT ( 'NONE',  ( 168.0045135618281904, 281.9156128332120943, -11.93384029740529684 ) ) ;
#24844=B_SPLINE_CURVE_WITH_KNOTS ( 'NONE', 3,
 ( #44568, #22283, #21785, #75503 ),
 .UNSPECIFIED., .F., .F.,
 ( 4, 4 ),
 ( 0.005429109838488062507, 0.01103906108590186654 ),
 .UNSPECIFIED. ) ;
#24846=CARTESIAN_POINT ( 'NONE',  ( 169.5608527833963421, 251.6396950762901952, -9.960993533446050208 ) ) ;
#24848=CARTESIAN_POINT ( 'NONE',  ( 162.6264071486809542, 248.9697954965390920, 10.36322805486644683 ) ) ;
#24849=CARTESIAN_POINT ( 'NONE',  ( 149.5796913320911870, 271.5673701627850960, -12.80793412251569841 ) ) ;
#24851=CARTESIAN_POINT ( 'NONE',  ( 188.8949863289861071, 270.0988553178502798, -14.15076922796234982 ) ) ;
#24856=VERTEX_POINT ( 'NONE', #68008 ) ;
#24858=CARTESIAN_POINT ( 'NONE',  ( 179.0008080442136418, 282.3876334254374001, 15.30776276532570712 ) ) ;
#24860=CARTESIAN_POINT ( 'NONE',  ( 177.7787795431753466, 256.3680583258327488, -7.267765067160797621 ) ) ;
#24861=CARTESIAN_POINT ( 'NONE',  ( 190.2389970918280540, 301.1433867864428748, 4.601241515604689525 ) ) ;
#24863=EDGE_LOOP ( 'NONE', ( #78095, #16435, #36978, #72162 ) ) ;
#24865=CARTESIAN_POINT ( 'NONE',  ( 194.6820509838467785, 270.8910309865917156, -14.27696746312268239 ) ) ;
#24867=ORIENTED_EDGE ( 'NONE', *, *, #80337, .T. ) ;
#24868=CARTESIAN_POINT ( 'NONE',  ( 200.9812045408918380, 282.5373376992193926, -16.61165062382494284 ) ) ;
#24873=CARTESIAN_POINT ( 'NONE',  ( 204.6713671561005299, 276.1457885614869951, -12.94307097876490431 ) ) ;
#24874=CARTESIAN_POINT ( 'NONE',  ( 105.4518702730975122, 225.5643266524160140, 9.188101187500095079 ) ) ;
#24875=CARTESIAN_POINT ( 'NONE',  ( 149.0164813726494799, 272.5428784278667536, -11.67305721329070423 ) ) ;
#24877=ORIENTED_EDGE ( 'NONE', *, *, #20789, .T. ) ;
#24878=CARTESIAN_POINT ( 'NONE',  ( 208.2777459429579210, 269.8993572713111462, 3.129643751043610589 ) ) ;
#24881=CARTESIAN_POINT ( 'NONE',  ( 159.4889735931715222, 254.4039898200529706, 16.88104032092801887 ) ) ;
#24882=CARTESIAN_POINT ( 'NONE',  ( 58.41569198217266035, 204.5333772461660544, 9.188101187500095079 ) ) ;
#24884=CARTESIAN_POINT ( 'NONE',  ( 160.2827339360533188, 254.1851989922621726, 15.48500462334072658 ) ) ;
#24885=CARTESIAN_POINT ( 'NONE',  ( 150.2678036912315349, 270.3755245954375823, 14.25047800729520375 ) ) ;
#24886=CARTESIAN_POINT ( 'NONE',  ( 175.4173451253388407, 272.5932200924088420, 17.76602235907715510 ) ) ;
#24888=B_SPLINE_CURVE_WITH_KNOTS ( 'NONE', 3,
 ( #43003, #58708, #4526, #83063 ),
 .UNSPECIFIED., .F., .F.,
 ( 4, 4 ),
 ( 0.000000000000000000, 0.002003342248209785594 ),
 .UNSPECIFIED. ) ;
#24889=CARTESIAN_POINT ( 'NONE',  ( 190.2629546459234859, 273.4080951500121159, -16.67925241984795903 ) ) ;
#24891=CARTESIAN_POINT ( 'NONE',  ( 167.6146168596400514, 252.8497314824998909, -12.44459218179994231 ) ) ;
#24892=DIRECTION ( 'NONE',  ( 0.5000000000000048850, -0.8660254037844358210, 0.000000000000000000 ) ) ;
#24893=ORIENTED_EDGE ( 'NONE', *, *, #98347, .T. ) ;
#24894=CARTESIAN_POINT ( 'NONE',  ( 103.0791479645378104, 236.9865022471902876, -10.00000000000009592 ) ) ;
#24896=CARTESIAN_POINT ( 'NONE',  ( 207.4218731373931632, 271.3817724553659332, -5.249531240730909154 ) ) ;
#24897=CARTESIAN_POINT ( 'NONE',  ( 193.1649355862271591, 296.0755126543221536, -12.21556774862162698 ) ) ;
#24900=CARTESIAN_POINT ( 'NONE',  ( 42.54989241151534429, 183.8262482093457493, 3.021315404115420679E-15 ) ) ;
#24905=CARTESIAN_POINT ( 'NONE',  ( 106.4801018922090066, 232.2833772461660544, -9.188101187500095079 ) ) ;
#24907=CARTESIAN_POINT ( 'NONE',  ( 147.0276296945837373, 275.9876705829954062, 0.7617065417431535534 ) ) ;
#24908=ADVANCED_FACE ( 'NONE', ( #68994 ), #55283, .T. ) ;
#24911=CARTESIAN_POINT ( 'NONE',  ( 203.0862352702880003, 278.8913175244117610, -15.09542727681365015 ) ) ;
#24912=CARTESIAN_POINT ( 'NONE',  ( 183.1065844243434242, 285.0799303997669654, -14.93148665631748351 ) ) ;
#24914=CARTESIAN_POINT ( 'NONE',  ( 178.1205181064416081, 255.2832539585039342, 4.586525146579208290 ) ) ;
#24917=CARTESIAN_POINT ( 'NONE',  ( 158.4671134108900787, 274.9587530538368583, -12.53151093071063471 ) ) ;
#24919=CARTESIAN_POINT ( 'NONE',  ( 164.7680996532798474, 245.2602752643843189, -0.9068639473870550027 ) ) ;
#24920=CARTESIAN_POINT ( 'NONE',  ( 129.5380282679697075, 245.5958772461660544, -9.188101187500095079 ) ) ;
#24921=CARTESIAN_POINT ( 'NONE',  ( 198.4860348845112981, 286.8590983175747056, -18.20461732983060088 ) ) ;
#24922=EDGE_CURVE ( 'NONE', #30618, #84862, #3374, .T. ) ;
#24923=CARTESIAN_POINT ( 'NONE',  ( 185.3925434965363763, 297.5756078945317427, 4.115160971246430321 ) ) ;
#24924=CARTESIAN_POINT ( 'NONE',  ( 188.1708508464760712, 281.7058697880425484, -16.75825131916482391 ) ) ;
#24925=CARTESIAN_POINT ( 'NONE',  ( 147.1270795744234476, 264.4111747905818675, -1.822351119449947324E-15 ) ) ;
#24926=CARTESIAN_POINT ( 'NONE',  ( 44.82974491242176640, 202.8149278399160664, 9.188101187500093303 ) ) ;
#24929=ADVANCED_FACE ( 'NONE', ( #60885 ), #39949, .F. ) ;
#24930=CARTESIAN_POINT ( 'NONE',  ( 174.3443330002151583, 262.1300491651107905, 14.35593273800351533 ) ) ;
#24932=CARTESIAN_POINT ( 'NONE',  ( 182.0894599482799094, 294.4148934881073956, -6.407201795530185429 ) ) ;
#24934=CARTESIAN_POINT ( 'NONE',  ( 178.3097623879434934, 261.2848360722642838, 12.47870625538927669 ) ) ;
#24935=CARTESIAN_POINT ( 'NONE',  ( 117.2061873602235238, 245.1427522451419065, -10.00000000000009415 ) ) ;
#24938=CARTESIAN_POINT ( 'NONE',  ( 202.9972156839127990, 279.0455039708822937, 16.77197898838388213 ) ) ;
#24940=CARTESIAN_POINT ( 'NONE',  ( 30.97368554763575688, 182.5643266524159856, -9.188101187500093303 ) ) ;
#24942=CARTESIAN_POINT ( 'NONE',  ( 188.8280684177597664, 290.6827677694134309, -15.06566886457551568 ) ) ;
#24946=CARTESIAN_POINT ( 'NONE',  ( 63.58478110923711313, 197.5177522451417929, 5.000000000000051514 ) ) ;
#24947=CARTESIAN_POINT ( 'NONE',  ( 171.7935577790372861, 286.8752040708455411, 7.461994811497778102 ) ) ;
#24952=B_SPLINE_CURVE_WITH_KNOTS ( 'NONE', 3,
 ( #73612, #99282, #38445, #91697, #4193, #76479, #96952, #61248, #89361, #19917, #50788, #81740, #92217, #86128, #31355, #9066, #39435, #87642, #33361, #56657, #39933, #1478, #94201, #966, #8569, #85618, #17670, #64261, #93702, #1969, #62238, #32361, #24755, #40935, #77973, #70354, #16162, #16657, #38948, #69853, #31843, #63763, #2479, #70871 ),
 .UNSPECIFIED., .F., .F.,
 ( 4, 2, 2, 2, 2, 2, 2, 2, 2, 2, 2, 2, 2, 2, 2, 2, 2, 2, 2, 2, 2, 4 ),
 ( 0.003392636941779382433, 0.003583394314189582066, 0.003678773000394681449, 0.003774151686599781265, 0.003869530372804881081, 0.003964909059009980030, 0.004155666431420030477, 0.004537181176240082797, 0.004918695921060133383, 0.005681725410700300474, 0.006444754900340467565, 0.007970813879620801748, 0.008161571252030822704, 0.008185415923582036943, 0.008209260595133251182, 0.008233105266684463686, 0.008256949938235677924, 0.008352328624440510593, 0.008543085996850172462, 0.008733843369259834330, 0.009115358114079230925, 0.009496872858898627520 ),
 .UNSPECIFIED. ) ;
#24954=CARTESIAN_POINT ( 'NONE',  ( 27.01324999880465683, 179.7365022471902307, 10.00000000000009592 ) ) ;
#24955=CARTESIAN_POINT ( 'NONE',  ( 36.73799359191946934, 192.0177522451418781, -10.00000000000009592 ) ) ;
#24956=CARTESIAN_POINT ( 'NONE',  ( 162.8789161433191452, 248.5324370884573568, 9.731756914259689140 ) ) ;
#24957=CARTESIAN_POINT ( 'NONE',  ( -6.102853504003019403, 155.0327760586659451, 1.948934522072303157E-15 ) ) ;
#24959=CARTESIAN_POINT ( 'NONE',  ( 200.3625978841952531, 283.1932893211792361, 16.78850222475318432 ) ) ;
#24962=CARTESIAN_POINT ( 'NONE',  ( 164.6241018286200699, 245.5096868128744632, 3.031483545445131433 ) ) ;
#24964=CARTESIAN_POINT ( 'NONE',  ( 183.6116158731336441, 256.9743117497176854, -1.628339465941822661 ) ) ;
#24969=CARTESIAN_POINT ( 'NONE',  ( 152.8894687064977234, 278.3516875449029158, -6.243347624783317507 ) ) ;
#24971=CARTESIAN_POINT ( 'NONE',  ( 207.0170762168093859, 272.0829012885643579, 9.497721717913687911 ) ) ;
#24974=CARTESIAN_POINT ( 'NONE',  ( 159.2651917302844993, 254.7915913763855258, -16.53922207549818424 ) ) ;
#24977=CARTESIAN_POINT ( 'NONE',  ( 192.2431834237441706, 297.6720342317289578, 11.07782187406058938 ) ) ;
#24978=CYLINDRICAL_SURFACE ( 'NONE', #28775, 17.82106496071139645 ) ;
#24979=CARTESIAN_POINT ( 'NONE',  ( 163.3409975114459485, 247.7320886816312111, -10.96358124877083640 ) ) ;
#24987=CARTESIAN_POINT ( 'NONE',  ( 171.2741013746033332, 249.3936815359432728, 2.927055546763141169 ) ) ;
#24989=EDGE_CURVE ( 'NONE', #48406, #89111, #49882, .T. ) ;
#24990=CARTESIAN_POINT ( 'NONE',  ( 191.0481192767711036, 299.7419460525905492, -9.103377665618040737 ) ) ;
#24993=VERTEX_POINT ( 'NONE', #27897 ) ;
#24994=CARTESIAN_POINT ( 'NONE',  ( 161.5431944097339851, 250.8459749958011287, 14.52339846942414603 ) ) ;
#24996=B_SPLINE_CURVE_WITH_KNOTS ( 'NONE', 3,
 ( #27908, #58305, #13233, #59793 ),
 .UNSPECIFIED., .F., .F.,
 ( 4, 4 ),
 ( 0.01565730217348996339, 0.02445820785911252682 ),
 .UNSPECIFIED. ) ;
#24997=CARTESIAN_POINT ( 'NONE',  ( 151.3883635558152321, 268.4346579770563608, 15.44343517165679103 ) ) ;
#24999=ORIENTED_EDGE ( 'NONE', *, *, #52211, .F. ) ;
#25000=FACE_OUTER_BOUND ( 'NONE', #67758, .T. ) ;
#25002=EDGE_LOOP ( 'NONE', ( #281, #84149, #10325 ) ) ;
#25004=ORIENTED_EDGE ( 'NONE', *, *, #65731, .T. ) ;
#25007=CARTESIAN_POINT ( 'NONE',  ( 165.5093369583051128, 275.0219039653110258, -16.16693748275729803 ) ) ;
#25008=ORIENTED_EDGE ( 'NONE', *, *, #43057, .F. ) ;
#25011=CARTESIAN_POINT ( 'NONE',  ( 148.3253847707240141, 273.7398928553401447, -9.074433450356286457 ) ) ;
#25013=CARTESIAN_POINT ( 'NONE',  ( 187.0083344850037008, 268.0836409071914090, -15.22627500120235133 ) ) ;
#25017=CARTESIAN_POINT ( 'NONE',  ( 206.4943150373521803, 272.9883502116088039, 11.34100825923693101 ) ) ;
#25018=DIRECTION ( 'NONE',  ( -0.8660254037844387076, -0.4999999999999998890, -0.000000000000000000 ) ) ;
#25019=CARTESIAN_POINT ( 'NONE',  ( 159.4574711498080433, 254.4585536525209477, 16.86100557095418395 ) ) ;
#25020=ORIENTED_EDGE ( 'NONE', *, *, #13353, .T. ) ;
#25021=CARTESIAN_POINT ( 'NONE',  ( 146.7443032962641212, 276.4784063000103060, -3.845166261074166147 ) ) ;
#25023=CARTESIAN_POINT ( 'NONE',  ( 63.58478110923711313, 197.5177522451417929, 5.000000000000051514 ) ) ;
#25024=CARTESIAN_POINT ( 'NONE',  ( 206.0870578475358172, 273.6937403561189512, -10.07771901274806581 ) ) ;
#25026=( BOUNDED_CURVE ( )  B_SPLINE_CURVE ( 2, ( #52267, #43156, #5673, #66477, #68459, #66965, #90826, #36066, #74097 ),
 .UNSPECIFIED., .F., .T. ) 
 B_SPLINE_CURVE_WITH_KNOTS ( ( 3, 2, 2, 2, 3 ),
 ( 0.5524193548387096309, 0.5537634408602150060, 0.5564516129032257563, 0.5591397849462365066, 0.5604838709677418818 ),
 .UNSPECIFIED. ) 
 CURVE ( )  GEOMETRIC_REPRESENTATION_ITEM ( )  RATIONAL_B_SPLINE_CURVE ( ( 0.9330127018922194093, 0.9330127018922194093, 1.000000000000000000, 0.8660254037844387076, 1.000000000000000000, 0.8660254037844387076, 1.000000000000000000, 0.9330127018922194093, 0.9330127018922194093 ) ) 
 REPRESENTATION_ITEM ( '' )  );
#25028=CARTESIAN_POINT ( 'NONE',  ( 200.1103929410127762, 284.0456276340304953, 17.67835211026828901 ) ) ;
#25031=CARTESIAN_POINT ( 'NONE',  ( 155.1093231057254229, 261.9897669837033618, -17.23289009958756068 ) ) ;
#25032=EDGE_CURVE ( 'NONE', #44171, #79518, #63616, .T. ) ;
#25033=DIRECTION ( 'NONE',  ( -0.8660254037844387076, -0.4999999999999998890, -0.000000000000000000 ) ) ;
#25035=CARTESIAN_POINT ( 'NONE',  ( 12.48928228595513801, 188.0177522451419065, 5.000000000000046185 ) ) ;
#25036=CARTESIAN_POINT ( 'NONE',  ( 96.27750042569734035, 217.2048013555409796, 4.594050593750051981 ) ) ;
#25040=B_SPLINE_CURVE_WITH_KNOTS ( 'NONE', 3,
 ( #34990, #67388, #74526, #66891 ),
 .UNSPECIFIED., .F., .F.,
 ( 4, 4 ),
 ( 0.008405187511566250894, 0.01662358261992283662 ),
 .UNSPECIFIED. ) ;
#25041=CARTESIAN_POINT ( 'NONE',  ( 174.7267715799268615, 282.0933535004488135, -14.14109511867729729 ) ) ;
#25042=CARTESIAN_POINT ( 'NONE',  ( 208.0964157306580375, 270.2134304119617809, 3.093366075300640894 ) ) ;
#25043=B_SPLINE_CURVE_WITH_KNOTS ( 'NONE', 3,
 ( #13756, #52252, #99373, #68940, #53250, #51774, #75078, #99866, #59849, #64, #98382, #45149, #22849, #29952, #44144, #59333, #38540, #61340, #92299, #28971, #53732, #68445, #90812, #90313, #98879, #15232, #67959, #36547, #75569, #76088, #46128, #20885, #60333, #83194, #60828, #82715, #13283, #21856, #6158, #37052, #52737, #83700, #14259, #6662, #91788, #1057, #77568, #8156, #56240, #15736 ),
 .UNSPECIFIED., .F., .F.,
 ( 4, 2, 2, 2, 2, 2, 2, 2, 2, 2, 2, 2, 2, 2, 2, 2, 2, 2, 2, 2, 2, 2, 2, 2, 4 ),
 ( 0.0003491678432873779694, 0.0008189001457873160399, 0.001288632448287254165, 0.001523498599537288821, 0.001640931675162307342, 0.001758364750787326297, 0.001993230902037290263, 0.002228097053287254013, 0.002697829355787181513, 0.003167561658287109446, 0.004107026263287102789, 0.005046490868287095699, 0.005516223170787129884, 0.005751089322037109680, 0.005868522397662098711, 0.005927238935474593226, 0.005985955473287089476, 0.006044672011099583991, 0.006103388548912078507, 0.006220821624537024169, 0.006455687775786910290, 0.006925420078286675593, 0.007395152380786440896, 0.007630018532036412886, 0.007864884683286383141 ),
 .UNSPECIFIED. ) ;
#25044=CARTESIAN_POINT ( 'NONE',  ( 7.590652549690899420, 181.3149278399161233, -9.188101187500095079 ) ) ;
#25047=CARTESIAN_POINT ( 'NONE',  ( 161.8811854682448939, 250.2605573099562264, 13.51112293479948789 ) ) ;
#25052=CARTESIAN_POINT ( 'NONE',  ( 188.6230325960351024, 261.4887198759634543, -5.970139219065332625 ) ) ;
#25055=CARTESIAN_POINT ( 'NONE',  ( 161.8668411317136986, 250.2854024296290447, -13.43522912998426655 ) ) ;
#25057=CARTESIAN_POINT ( 'NONE',  ( 44.64073572505018461, 187.3923013555410080, 4.594050593750050204 ) ) ;
#25058=CARTESIAN_POINT ( 'NONE',  ( 78.23504418992378362, 222.6427522451418781, -10.00000000000009415 ) ) ;
#25060=ORIENTED_EDGE ( 'NONE', *, *, #61515, .F. ) ;
#25064=CARTESIAN_POINT ( 'NONE',  ( -13.54586673536430830, 172.1744531367911293, 4.594050593750047540 ) ) ;
#25066=CARTESIAN_POINT ( 'NONE',  ( 161.6923300915171922, 250.5876644177310482, -14.43081872899884566 ) ) ;
#25067=CARTESIAN_POINT ( 'NONE',  ( 187.0955991096881519, 282.9188776676083421, 16.20459510219963661 ) ) ;
#25068=CARTESIAN_POINT ( 'NONE',  ( 147.6884207308302450, 274.8431469350302336, -8.096293592099874203 ) ) ;
#25070=CARTESIAN_POINT ( 'NONE',  ( 171.6803261575313968, 279.7085677115863973, 14.16212843711857516 ) ) ;
#25071=CARTESIAN_POINT ( 'NONE',  ( 147.0276296945837373, 275.9876705829954062, 0.7617065417431535534 ) ) ;
#25072=DIRECTION ( 'NONE',  ( -0.8660254037844387076, -0.4999999999999998890, -0.000000000000000000 ) ) ;
#25073=ORIENTED_EDGE ( 'NONE', *, *, #22460, .T. ) ;
#25074=CARTESIAN_POINT ( 'NONE',  ( 181.1647404240839023, 268.1795203863183588, 15.36725951381329480 ) ) ;
#25075=CARTESIAN_POINT ( 'NONE',  ( 109.6190968851625911, 246.3464784336661353, 1.353441290958777327E-15 ) ) ;
#25079=CARTESIAN_POINT ( 'NONE',  ( 157.1338510812060747, 258.4831816688264325, 17.88958125218800888 ) ) ;
#25081=CARTESIAN_POINT ( 'NONE',  ( 191.1456801727256618, 299.5729656239652741, -6.514204219820171282 ) ) ;
#25083=CARTESIAN_POINT ( 'NONE',  ( 196.4783028304046013, 290.3365922432724346, -16.37291435488387492 ) ) ;
#25084=CARTESIAN_POINT ( 'NONE',  ( 46.83931157395847578, 209.3967562850346837, 1.101618078115930403E-13 ) ) ;
#25085=CARTESIAN_POINT ( 'NONE',  ( 174.8696466734779449, 292.3029143586743430, -1.153856708368909967 ) ) ;
#25088=CARTESIAN_POINT ( 'NONE',  ( 189.0480903703354727, 265.6948563348121866, 10.88985011883314513 ) ) ;
#25089=CARTESIAN_POINT ( 'NONE',  ( 179.4583960273904211, 270.4090523040318885, 17.47970616590194837 ) ) ;
#25090=CARTESIAN_POINT ( 'NONE',  ( 165.5845925187108492, 269.2586473770181783, -17.52824664516929332 ) ) ;
#25092=B_SPLINE_CURVE_WITH_KNOTS ( 'NONE', 3,
 ( #40916, #49049, #79985, #39914 ),
 .UNSPECIFIED., .F., .F.,
 ( 4, 4 ),
 ( 0.008247362098805164840, 0.01450959442545752057 ),
 .UNSPECIFIED. ) ;
#25094=CARTESIAN_POINT ( 'NONE',  ( 155.7144456569324973, 261.3779154106480291, 17.02946396951419672 ) ) ;
#25097=CARTESIAN_POINT ( 'NONE',  ( 153.4289928607825573, 264.9001843414388873, 17.27358709529985958 ) ) ;
#25099=CARTESIAN_POINT ( 'NONE',  ( 165.1263583288683492, 286.0211790206518003, 4.421035561736735175 ) ) ;
#25104=CARTESIAN_POINT ( 'NONE',  ( 167.7541779101917712, 280.9156681186656215, 11.77209881610279574 ) ) ;
#25105=B_SPLINE_CURVE_WITH_KNOTS ( 'NONE', 3,
 ( #42725, #79801, #19962, #3765 ),
 .UNSPECIFIED., .F., .F.,
 ( 4, 4 ),
 ( 0.008408023062891595290, 0.01478712368365756036 ),
 .UNSPECIFIED. ) ;
#25107=CARTESIAN_POINT ( 'NONE',  ( 19.21902136474470524, 175.2365022471902307, 10.00000000000009948 ) ) ;
#25111=CARTESIAN_POINT ( 'NONE',  ( 164.7495643159037684, 251.3192192419287494, 12.55862708640273695 ) ) ;
#25113=CARTESIAN_POINT ( 'NONE',  ( -22.42236680055709641, 157.8615022471902591, 0.000000000000000000 ) ) ;
#25115=CARTESIAN_POINT ( 'NONE',  ( 203.0498946958275326, 278.9542612457532869, -15.11479947333269003 ) ) ;
#25118=EDGE_CURVE ( 'NONE', #20654, #29718, #25040, .T. ) ;
#25119=VERTEX_POINT ( 'NONE', #42581 ) ;
#25120=CYLINDRICAL_SURFACE ( 'NONE', #90195, 17.82106496071139645 ) ;
#25121=EDGE_CURVE ( 'NONE', #28762, #483, #84295, .T. ) ;
#25126=CARTESIAN_POINT ( 'NONE',  ( 155.6569868912636991, 261.0411854816857158, -17.75433477650897984 ) ) ;
#25127=ORIENTED_EDGE ( 'NONE', *, *, #32566, .T. ) ;
#25128=CARTESIAN_POINT ( 'NONE',  ( 164.4118148411678817, 245.8773786609274623, -1.109947685176164045 ) ) ;
#25129=CARTESIAN_POINT ( 'NONE',  ( 190.1558484012587371, 301.2874045430920091, 3.461433172287052606 ) ) ;
#25131=CARTESIAN_POINT ( 'NONE',  ( 147.4563929227680603, 275.2450308873625886, -3.847749617713808412 ) ) ;
#25132=CARTESIAN_POINT ( 'NONE',  ( 153.0927037754837556, 265.4826541232073964, -16.15085267704102634 ) ) ;
#25134=CARTESIAN_POINT ( 'NONE',  ( 165.5752708168755305, 245.8622137986321832, -1.085626278946311585 ) ) ;
#25135=CARTESIAN_POINT ( 'NONE',  ( 126.4254891512956220, 252.9869531367911009, 4.594050593750046652 ) ) ;
#25138=EDGE_LOOP ( 'NONE', ( #76927, #5817, #36821, #58986, #27494 ) ) ;
#25139=VECTOR ( 'NONE', #96483, 1000.000000000000000 ) ;
#25142=CARTESIAN_POINT ( 'NONE',  ( 203.6293652163894023, 276.2782967254192954, 13.37813849736390814 ) ) ;
#25143=CARTESIAN_POINT ( 'NONE',  ( 174.2000522056604837, 283.5616462974032288, 14.37013614557462837 ) ) ;
#25145=CARTESIAN_POINT ( 'NONE',  ( 146.9870408876112151, 276.0579724588903332, 4.160141643933214617 ) ) ;
#25147=CARTESIAN_POINT ( 'NONE',  ( 200.2093391412865060, 269.7417714514684803, 10.46510648850140157 ) ) ;
#25148=CARTESIAN_POINT ( 'NONE',  ( 176.5581593771217399, 288.4200715899070246, -9.318063636782698111 ) ) ;
#25151=CARTESIAN_POINT ( 'NONE',  ( 194.9138646879852104, 291.7602453613734497, 15.86905368594769605 ) ) ;
#25153=CARTESIAN_POINT ( 'NONE',  ( 194.3011251241114508, 294.1075746476782342, -14.76047579547631905 ) ) ;
#25158=ADVANCED_FACE ( 'NONE', ( #23642 ), #14831, .F. ) ;
#25160=CARTESIAN_POINT ( 'NONE',  ( 152.1919794413566080, 267.0427544335294670, -15.42826099493241365 ) ) ;
#25161=CARTESIAN_POINT ( 'NONE',  ( 149.7119746935222793, 271.3382486597900538, 12.05352563709836922 ) ) ;
#25162=CARTESIAN_POINT ( 'NONE',  ( 202.4323889586180201, 280.0238125565655878, 15.69595176008160919 ) ) ;
#25163=CARTESIAN_POINT ( 'NONE',  ( 153.2732530772018151, 270.1937817606684575, 14.03420799374948480 ) ) ;
#25164=CARTESIAN_POINT ( 'NONE',  ( 154.8827976570641169, 277.6426042987627625, -8.977273693884303185 ) ) ;
#25165=LINE ( 'NONE', #70262, #39736 ) ;
#25167=CARTESIAN_POINT ( 'NONE',  ( 165.0952264510788154, 281.4963861521250124, -11.84807672454148886 ) ) ;
#25168=AXIS2_PLACEMENT_3D ( 'NONE', #13063, #37318, #81978 ) ;
#25169=CARTESIAN_POINT ( 'NONE',  ( 164.6244273547873718, 247.3313301143314789, -7.559144047185251125 ) ) ;
#25171=CARTESIAN_POINT ( 'NONE',  ( 198.2505066714982149, 285.2670451491296149, 0.000000000000000000 ) ) ;
#25172=CARTESIAN_POINT ( 'NONE',  ( 84.36939080006362701, 209.5177522451417929, 5.000000000000051514 ) ) ;
#25173=CARTESIAN_POINT ( 'NONE',  ( 184.6056068049121563, 296.8943211797820823, -4.405390306300510872 ) ) ;
#25175=CARTESIAN_POINT ( 'NONE',  ( 160.8891438268352374, 281.0495864612497599, 9.578199528566821996 ) ) ;
#25177=CARTESIAN_POINT ( 'NONE',  ( -12.46307465703608841, 173.6115022471903160, -5.000000000000047962 ) ) ;
#25179=CARTESIAN_POINT ( 'NONE',  ( -6.536213301660246167, 167.0333772461660828, 9.188101187500095079 ) ) ;
#25180=CARTESIAN_POINT ( 'NONE',  ( 91.51436070488293240, 214.4548013555409796, -4.594050593750042211 ) ) ;
#25181=CARTESIAN_POINT ( 'NONE',  ( 166.1309782654906257, 249.2029336093187339, -9.347746458946922132 ) ) ;
#25183=CARTESIAN_POINT ( 'NONE',  ( 183.1207986101861138, 294.8225010653632694, -8.165837621905515320 ) ) ;
#25186=DIRECTION ( 'NONE',  ( 0.4999999999999998890, -0.8660254037844385966, 0.000000000000000000 ) ) ;
#25190=CARTESIAN_POINT ( 'NONE',  ( 207.8741656103030664, 270.5983789124053374, 5.135401317816507216 ) ) ;
#25191=CARTESIAN_POINT ( 'NONE',  ( 165.9806062298373774, 249.4185370747466948, -9.186238584016363617 ) ) ;
#25194=CARTESIAN_POINT ( 'NONE',  ( 161.8882824960653579, 250.2482648971885340, -13.83574485983625557 ) ) ;
#25196=CARTESIAN_POINT ( 'NONE',  ( 45.69611741197122257, 191.0643266524160140, 9.188101187500095079 ) ) ;
#25197=DIRECTION ( 'NONE',  ( -0.8660254037844387076, -0.4999999999999998890, -0.000000000000000000 ) ) ;
#25199=CARTESIAN_POINT ( 'NONE',  ( 63.61184440487929947, 207.5333772461660544, 9.188101187500095079 ) ) ;
#25202=CARTESIAN_POINT ( 'NONE',  ( 104.9555363394041336, 224.7365022471902307, 10.00000000000009948 ) ) ;
#25203=CARTESIAN_POINT ( 'NONE',  ( 197.9294784878310907, 286.6389924893580883, -17.36088744678619378 ) ) ;
#25204=CARTESIAN_POINT ( 'NONE',  ( 200.1613715040462864, 283.9573301727594981, 16.94951437046174192 ) ) ;
#25205=CARTESIAN_POINT ( 'NONE',  ( 22.90194105960797089, 172.4824982072973967, 3.021315404115420679E-15 ) ) ;
#25212=CARTESIAN_POINT ( 'NONE',  ( 71.86588871287597158, 221.4869531367911293, 4.594050593750046652 ) ) ;
#25213=CARTESIAN_POINT ( 'NONE',  ( 99.70756906128829655, 216.8262482093457493, 3.021315404115420679E-15 ) ) ;
#25215=CARTESIAN_POINT ( 'NONE',  ( 170.0644797785468540, 289.4723839078269521, -1.148982712589306843 ) ) ;
#25217=CARTESIAN_POINT ( 'NONE',  ( 153.6005803596509054, 264.6029860754553056, 18.07864614867099462 ) ) ;
#25220=CARTESIAN_POINT ( 'NONE',  ( 189.8039450987227781, 286.5139521920973493, 16.53692407126337116 ) ) ;
#25221=CARTESIAN_POINT ( 'NONE',  ( 130.9362984529373080, 239.7365022471902307, 10.00000000000009592 ) ) ;
#25222=CARTESIAN_POINT ( 'NONE',  ( 161.8873598795597388, 250.2498629158519350, 13.90822209621415873 ) ) ;
#25223=CARTESIAN_POINT ( 'NONE',  ( 164.9404048476745004, 244.9618339132846074, -2.801285734921658666 ) ) ;
#25225=CARTESIAN_POINT ( 'NONE',  ( 185.1115058749157072, 271.5392633888741898, 15.95323373308776738 ) ) ;
#25227=CARTESIAN_POINT ( 'NONE',  ( 202.7041331321765938, 279.5531378413010657, 17.14708438049711248 ) ) ;
#25230=ORIENTED_EDGE ( 'NONE', *, *, #82821, .F. ) ;
#25231=CARTESIAN_POINT ( 'NONE',  ( 176.4056758504748359, 253.1994894479077800, -0.2561444540333105979 ) ) ;
#25233=EDGE_CURVE ( 'NONE', #65090, #25284, #85371, .T. ) ;
#25235=CARTESIAN_POINT ( 'NONE',  ( 167.5593980844118391, 247.9703659007788303, 3.535947377295492799 ) ) ;
#25239=AXIS2_PLACEMENT_3D ( 'NONE', #18087, #79919, #70772 ) ;
#25242=DIRECTION ( 'NONE',  ( -0.8660254037844387076, -0.4999999999999998890, -0.000000000000000000 ) ) ;
#25243=EDGE_CURVE ( 'NONE', #53811, #15709, #25677, .T. ) ;
#25244=DIRECTION ( 'NONE',  ( 0.4999999999999998890, -0.8660254037844385966, 0.000000000000000000 ) ) ;
#25249=CARTESIAN_POINT ( 'NONE',  ( 186.3701877112573300, 298.6212407368254276, 1.067666278078492459 ) ) ;
#25250=CARTESIAN_POINT ( 'NONE',  ( 163.2399645767092693, 283.8610605660015267, -2.803462861407186590 ) ) ;
#25251=CARTESIAN_POINT ( 'NONE',  ( 194.3442947553755005, 294.0328026529847421, -15.97648891113594871 ) ) ;
#25253=CARTESIAN_POINT ( 'NONE',  ( 154.8596847415876994, 262.4221533139083817, 17.65401077761399762 ) ) ;
#25255=CARTESIAN_POINT ( 'NONE',  ( 204.6470611188870521, 276.1878878528713130, -13.02652554726987866 ) ) ;
#25256=CARTESIAN_POINT ( 'NONE',  ( 163.9797515130013892, 246.6257342973991626, 4.819337769813046179 ) ) ;
#25259=CARTESIAN_POINT ( 'NONE',  ( 82.93486267893707975, 224.8149278399160949, -9.188101187500095079 ) ) ;
#25260=EDGE_LOOP ( 'NONE', ( #98465, #89446, #43307, #62489 ) ) ;
#25261=CARTESIAN_POINT ( 'NONE',  ( 191.2645787786270262, 299.3670271975948367, 7.309947121636420242 ) ) ;
#25264=B_SPLINE_CURVE_WITH_KNOTS ( 'NONE', 3,
 ( #41129, #17868, #81196, #34546 ),
 .UNSPECIFIED., .F., .F.,
 ( 4, 4 ),
 ( 0.008201218458928592747, 0.01437332038716656810 ),
 .UNSPECIFIED. ) ;
#25265=CARTESIAN_POINT ( 'NONE',  ( 195.4001060159568510, 292.2040839064547413, -16.96545459487308705 ) ) ;
#25271=DIRECTION ( 'NONE',  ( 0.4999999999999998890, -0.8660254037844385966, 0.000000000000000000 ) ) ;
#25272=CARTESIAN_POINT ( 'NONE',  ( 208.1583869480885483, 270.1060931147653719, 3.025867354224990979 ) ) ;
#25273=CARTESIAN_POINT ( 'NONE',  ( 94.78875894111908451, 225.5333772461660544, 9.188101187500095079 ) ) ;
#25277=CARTESIAN_POINT ( 'NONE',  ( 207.8136982414359579, 270.7031114674828700, -0.9536989003868096004 ) ) ;
#25278=ORIENTED_EDGE ( 'NONE', *, *, #48586, .F. ) ;
#25279=DIRECTION ( 'NONE',  ( -0.8660254037844387076, -0.4999999999999998890, -0.000000000000000000 ) ) ;
#25284=VERTEX_POINT ( 'NONE', #27677 ) ;
#25285=CARTESIAN_POINT ( 'NONE',  ( 191.9006881710348864, 296.3094005088366885, 11.25170506121845726 ) ) ;
#25287=CARTESIAN_POINT ( 'NONE',  ( 159.2102594322688844, 254.8867369075254885, -16.13039487917589199 ) ) ;
#25288=CARTESIAN_POINT ( 'NONE',  ( 155.6205867397425777, 262.5964510888063614, -17.36443500069399093 ) ) ;
#25290=B_SPLINE_CURVE_WITH_KNOTS ( 'NONE', 3,
 ( #60490, #98034, #51416, #76239, #14423, #59496, #30111, #75234, #75732, #13919, #5815, #45789, #36703, #6317, #37208, #68109, #99033, #29617, #29130, #28612, #91448, #22010, #82865, #6813, #99528, #83857, #52906, #53403, #84352, #36206, #90474, #14899, #98540, #37694, #68605, #22509, #67109, #44797, #38185, #76709, #7304, #69101, #28115, #58989, #67610, #20537, #21524, #82377, #12947, #43808 ),
 .UNSPECIFIED., .F., .F.,
 ( 4, 2, 2, 2, 2, 2, 2, 2, 2, 2, 2, 2, 2, 2, 2, 2, 2, 2, 2, 2, 2, 2, 2, 2, 4 ),
 ( 0.0002547070572390182255, 0.001273486803321399090, 0.001782876676362517721, 0.002037571612883104250, 0.002164919081143416597, 0.002292266549403729377, 0.002419614017664041723, 0.002546961485924354503, 0.002801656422445068968, 0.003311046295486411595, 0.004329826041568941158, 0.005348605787651470288, 0.005857995660692657224, 0.006112690597213250691, 0.006367385533733843292, 0.006431059267864082732, 0.006494733001994320437, 0.006558406736124559010, 0.006622080470254797582, 0.006876775406775844680, 0.007386165279818052501, 0.007640860216339145569, 0.007895555152860238637, 0.008150250089381331706, 0.008404945025902424774 ),
 .UNSPECIFIED. ) ;
#25293=CARTESIAN_POINT ( 'NONE',  ( 195.4175937697542338, 279.6204996462902272, -17.14456379506867023 ) ) ;
#25296=CARTESIAN_POINT ( 'NONE',  ( 161.1238074876215478, 251.5723744529297505, 13.42537408252843179 ) ) ;
#25297=CARTESIAN_POINT ( 'NONE',  ( 152.7730629122270898, 271.2363297891400293, 14.33490734661111610 ) ) ;
#25298=CARTESIAN_POINT ( 'NONE',  ( 187.8785148445833215, 266.1283279326300431, -11.85110462984868462 ) ) ;
#25300=CARTESIAN_POINT ( 'NONE',  ( 175.5190374892232228, 290.1926326353742525, -6.256965731148535603 ) ) ;
#25301=CARTESIAN_POINT ( 'NONE',  ( 152.7730629122270898, 271.2363297891400293, 14.33490734661111610 ) ) ;
#25302=ORIENTED_EDGE ( 'NONE', *, *, #59224, .F. ) ;
#25305=CARTESIAN_POINT ( 'NONE',  ( 164.8329445879545290, 245.1479605429143760, -2.955380775890217304 ) ) ;
#25307=CARTESIAN_POINT ( 'NONE',  ( 176.1244130302606834, 285.2676080955770885, -13.06404472828928398 ) ) ;
#25309=CARTESIAN_POINT ( 'NONE',  ( 95.35708811412658292, 225.8615022471902591, -10.00000000000009592 ) ) ;
#25310=CARTESIAN_POINT ( 'NONE',  ( 155.2193237801463113, 261.7992402267395846, -18.58295809893692407 ) ) ;
#25312=CARTESIAN_POINT ( 'NONE',  ( 160.3714828861807860, 272.7013802378941136, -14.85790459234098471 ) ) ;
#25314=CARTESIAN_POINT ( 'NONE',  ( 192.1413729726642714, 262.2891126618652606, 2.981852608854113296 ) ) ;
#25315=CARTESIAN_POINT ( 'NONE',  ( 161.6127771116929921, 250.7254542206800352, -12.96229604595372464 ) ) ;
#25317=CARTESIAN_POINT ( 'NONE',  ( 8.700681467995980967, 166.6423013555410080, -4.594050593750043987 ) ) ;
#25319=ORIENTED_EDGE ( 'NONE', *, *, #67714, .T. ) ;
#25320=CARTESIAN_POINT ( 'NONE',  ( 174.8858495065613852, 255.2716098750472042, 8.953978856888550553 ) ) ;
#25321=CARTESIAN_POINT ( 'NONE',  ( -17.42236680055705023, 149.2012482093457777, 0.000000000000000000 ) ) ;
#25322=FACE_OUTER_BOUND ( 'NONE', #13067, .T. ) ;
#25324=CARTESIAN_POINT ( 'NONE',  ( 17.82075117977708700, 181.0958772461660544, -9.188101187500095079 ) ) ;
#25327=CARTESIAN_POINT ( 'NONE',  ( 199.6968473295422939, 267.3144708874781372, -6.730990908593314614 ) ) ;
#25328=CARTESIAN_POINT ( 'NONE',  ( 191.1000148935602567, 299.6520602076213891, -9.462302242170249400 ) ) ;
#25329=CARTESIAN_POINT ( 'NONE',  ( 197.0455264951692129, 289.3541320366447280, 17.54437334811087368 ) ) ;
#25332=CARTESIAN_POINT ( 'NONE',  ( 190.0885270318794937, 298.7835894469523623, -8.138652993139137592 ) ) ;
#25334=CARTESIAN_POINT ( 'NONE',  ( 85.03695205236203947, 213.2365022471901739, -10.00000000000009059 ) ) ;
#25338=CARTESIAN_POINT ( 'NONE',  ( 37.03551627836181126, 198.3149278399160664, 9.188101187500093303 ) ) ;
#25340=CARTESIAN_POINT ( 'NONE',  ( 205.7753384153419631, 271.2832105871503927, -6.565646494404037803 ) ) ;
#25341=CARTESIAN_POINT ( 'NONE',  ( 190.8907028847385448, 300.0145992415348815, -5.421341690443150618 ) ) ;
#25343=EDGE_LOOP ( 'NONE', ( #86511, #20558, #46139, #35271 ) ) ;
#25344=CARTESIAN_POINT ( 'NONE',  ( 166.1070111784138703, 253.4115428555481344, -13.60050710122670559 ) ) ;
#25346=CARTESIAN_POINT ( 'NONE',  ( 159.5941974674867083, 278.9247971600711367, -11.03768485503293739 ) ) ;
#25349=CARTESIAN_POINT ( 'NONE',  ( 202.5511585997265911, 279.8180975037686835, 17.12781264818056925 ) ) ;
#25350=CARTESIAN_POINT ( 'NONE',  ( 149.7109319212262051, 271.3400547943878109, -12.38605961032017433 ) ) ;
#25351=CIRCLE ( 'NONE', #78812, 17.82106496071138224 ) ;
#25352=CARTESIAN_POINT ( 'NONE',  ( 185.5654499382181655, 267.7323668493922924, -14.54006482872913253 ) ) ;
#25353=ORIENTED_EDGE ( 'NONE', *, *, #7992, .T. ) ;
#25360=EDGE_CURVE ( 'NONE', #28922, #99839, #67195, .T. ) ;
#25363=CARTESIAN_POINT ( 'NONE',  ( 149.3833831332874240, 271.9073859370555510, 11.40518020539810173 ) ) ;
#25370=CARTESIAN_POINT ( 'NONE',  ( 152.8651171364917900, 265.8768457450651113, -16.25664868183201861 ) ) ;
#25372=CARTESIAN_POINT ( 'NONE',  ( 172.8964584746522917, 253.4886925110870664, 9.877074417240217841 ) ) ;
#25375=CARTESIAN_POINT ( 'NONE',  ( 204.7237927799493775, 276.0549847173622879, -12.81020997223575364 ) ) ;
#25376=EDGE_CURVE ( 'NONE', #46780, #68198, #39491, .T. ) ;
#25377=CARTESIAN_POINT ( 'NONE',  ( 99.98491136382573075, 228.5333772461660828, 9.188101187500095079 ) ) ;
#25379=ORIENTED_EDGE ( 'NONE', *, *, #12103, .F. ) ;
#25382=CARTESIAN_POINT ( 'NONE',  ( 161.6083111375297108, 266.9942300563631647, 16.50555569288089686 ) ) ;
#25385=CARTESIAN_POINT ( 'NONE',  ( 157.2985995762109042, 259.4415387207266122, 17.34027181022534947 ) ) ;
#25387=CARTESIAN_POINT ( 'NONE',  ( 58.76725448063633195, 213.9244531367911577, -4.594050593750046652 ) ) ;
#25389=CARTESIAN_POINT ( 'NONE',  ( 190.9061255863007318, 299.9878863388391892, 7.497146773253707153 ) ) ;
#25390=FACE_OUTER_BOUND ( 'NONE', #40036, .T. ) ;
#25391=LINE ( 'NONE', #47677, #12385 ) ;
#25395=CARTESIAN_POINT ( 'NONE',  ( 177.7443685448805581, 288.9686455644151124, 11.17637150946867841 ) ) ;
#25396=CARTESIAN_POINT ( 'NONE',  ( 147.6088797830324779, 274.9809158978982850, 8.531536684623960198 ) ) ;
#25397=VERTEX_POINT ( 'NONE', #59529 ) ;
#25398=CARTESIAN_POINT ( 'NONE',  ( 171.9697486346997266, 259.6717877315294345, -13.86376714732617543 ) ) ;
#25399=CARTESIAN_POINT ( 'NONE',  ( 174.1708078612628583, 277.4829975439923828, -15.60795485462966425 ) ) ;
#25400=CARTESIAN_POINT ( 'NONE',  ( 207.1770866921659717, 271.8057550155037347, -5.569195235244989384 ) ) ;
#25401=CARTESIAN_POINT ( 'NONE',  ( 193.1444937042664094, 296.1109190324805240, -12.15243020627156767 ) ) ;
#25402=CARTESIAN_POINT ( 'NONE',  ( 180.8863484661150949, 271.3550751966830603, 16.94740090253783649 ) ) ;
#25403=CARTESIAN_POINT ( 'NONE',  ( 189.7726967107949747, 264.4065126852114531, 11.24316165915873000 ) ) ;
#25405=CARTESIAN_POINT ( 'NONE',  ( 167.7102881833664014, 256.2825055472106897, 13.57817267270622885 ) ) ;
#25407=CARTESIAN_POINT ( 'NONE',  ( 108.0499464844507997, 227.0643266524160424, 9.188101187500095079 ) ) ;
#25409=CARTESIAN_POINT ( 'NONE',  ( 146.7818291168261453, 276.4134096722012828, -0.7617065417431535534 ) ) ;
#25411=CARTESIAN_POINT ( 'NONE',  ( 202.7973612924478743, 279.3916619310153919, -15.54732529288344089 ) ) ;
#25412=CARTESIAN_POINT ( 'NONE',  ( 204.1953342137782954, 276.9703018036655067, 13.84727111424505885 ) ) ;
#25414=CARTESIAN_POINT ( 'NONE',  ( 175.3043775287472101, 252.5449758547659940, 5.231882537108772269 ) ) ;
#25417=CARTESIAN_POINT ( 'NONE',  ( 154.5758520964906779, 273.3885357916005319, -13.22738657698927689 ) ) ;
#25418=CARTESIAN_POINT ( 'NONE',  ( 181.9501482740564029, 260.5583091221847098, 9.820294706648617478 ) ) ;
#25419=CARTESIAN_POINT ( 'NONE',  ( 206.6829130365991034, 272.6616888947074244, -10.15488415123734001 ) ) ;
#25420=CARTESIAN_POINT ( 'NONE',  ( 134.8963869060034142, 254.8149278399160949, -9.188101187500095079 ) ) ;
#25421=CARTESIAN_POINT ( 'NONE',  ( 191.8284704360776516, 295.3786271354495057, -12.12832068662400076 ) ) ;
#25422=CARTESIAN_POINT ( 'NONE',  ( 189.0615291916986109, 299.2959719742789275, 4.846944731644502902 ) ) ;
#25424=CARTESIAN_POINT ( 'NONE',  ( 68.75404378773190217, 204.3768266524160140, 9.188101187500098632 ) ) ;
#25426=ADVANCED_FACE ( 'NONE', ( #21081 ), #1146, .F. ) ;
#25429=CARTESIAN_POINT ( 'NONE',  ( 204.9658583905037688, 275.6357147811169170, -12.57240504404813564 ) ) ;
#25431=B_SPLINE_SURFACE_WITH_KNOTS ( 'NONE', 3, 1, ( 
 ( #55655, #31868 ),
 ( #55163, #86643 ),
 ( #17174, #71900 ),
 ( #39454, #48075 ),
 ( #70378, #9604 ),
 ( #2500, #70895 ),
 ( #72411, #87661 ),
 ( #32876, #86150 ),
 ( #48593, #32384 ),
 ( #16680, #1498 ),
 ( #3016, #95234 ),
 ( #25277, #17689 ),
 ( #56163, #18194 ),
 ( #25800, #56677 ),
 ( #33905, #64792 ),
 ( #95737, #43955 ),
 ( #12595, #97215 ),
 ( #96219, #96721 ),
 ( #11104, #42457 ),
 ( #50566, #19701 ),
 ( #81516, #26783 ),
 ( #65279, #51574 ),
 ( #13095, #4990 ),
 ( #67266, #12085 ),
 ( #82020, #28266 ),
 ( #43463, #98191 ),
 ( #42946, #97698 ),
 ( #41975, #74404 ),
 ( #50078, #73885 ),
 ( #57664, #49573 ),
 ( #73392, #81037 ),
 ( #80526, #35369 ),
 ( #4477, #36361 ),
 ( #59141, #90111 ) ),
 .UNSPECIFIED., .T., .F., .F.,
 ( 4, 2, 2, 2, 2, 2, 2, 2, 2, 2, 2, 2, 2, 2, 2, 2, 4 ),
 ( 2, 2 ),
 ( 0.000000000000000000, 0.06250000000000000000, 0.1250000000000000000, 0.1875000000000000000, 0.2500000000000000000, 0.3125000000000000000, 0.3750000000000000000, 0.4375000000000000000, 0.5000000000000000000, 0.5625000000000000000, 0.6250000000000000000, 0.6875000000000000000, 0.7500000000000000000, 0.8125000000000000000, 0.8750000000000000000, 0.9375000000000000000, 1.000000000000000000 ),
 ( 0.000000000000000000, 1.000000000000000000 ),
 .UNSPECIFIED. ) ;
#25433=CARTESIAN_POINT ( 'NONE',  ( 174.5900386765337657, 262.0875730750212824, 14.28570942272308741 ) ) ;
#25434=CARTESIAN_POINT ( 'NONE',  ( 153.5001613412225936, 278.7771225056793583, -1.599187862637977187 ) ) ;
#25435=CARTESIAN_POINT ( 'NONE',  ( 178.4254400080073424, 292.4993321051520070, -7.220885224839013183 ) ) ;
#25436=CARTESIAN_POINT ( 'NONE',  ( 155.3513572141771704, 261.5705516107003064, -17.00592413546589299 ) ) ;
#25437=CARTESIAN_POINT ( 'NONE',  ( 153.6088888397055143, 269.2756142106472339, -15.62050981732668475 ) ) ;
#25439=CARTESIAN_POINT ( 'NONE',  ( 121.1754704609021900, 250.7677522451419065, -5.000000000000047962 ) ) ;
#25442=ADVANCED_FACE ( 'NONE', ( #70635 ), #32128, .T. ) ;
#25443=CARTESIAN_POINT ( 'NONE',  ( 147.6088797830324779, 274.9809158978982850, 8.531536684623960198 ) ) ;
#25445=CARTESIAN_POINT ( 'NONE',  ( 36.33204418566946714, 191.7833772461660544, -9.188101187500095079 ) ) ;
#25449=CARTESIAN_POINT ( 'NONE',  ( 72.24503514708140983, 222.5177522451419065, 5.000000000000046185 ) ) ;
#25450=CARTESIAN_POINT ( 'NONE',  ( 147.4317198359019301, 275.2877659273946733, 3.797273160043843188 ) ) ;
#25453=CARTESIAN_POINT ( 'NONE',  ( 64.01779381112929457, 207.7677522451418497, 10.00000000000009592 ) ) ;
#25454=CARTESIAN_POINT ( 'NONE',  ( 174.3739577948688577, 289.3819840071309386, 7.916562535199481943 ) ) ;
#25455=CARTESIAN_POINT ( 'NONE',  ( 163.1346087304468142, 255.9866270473322629, -14.93535196593188275 ) ) ;
#25456=CARTESIAN_POINT ( 'NONE',  ( 5.723458822437210713, 164.1115022471902023, -5.000000000000041744 ) ) ;
#25459=CARTESIAN_POINT ( 'NONE',  ( 179.6160012257981862, 295.0481727651569486, 1.085779272287555663 ) ) ;
#25460=CARTESIAN_POINT ( 'NONE',  ( 20.08504676852905746, 195.7365022471903444, 2.944929066748280225E-16 ) ) ;
#25461=CARTESIAN_POINT ( 'NONE',  ( 142.0139464194155039, 261.9869531367911009, 4.594050593750046652 ) ) ;
#25463=CARTESIAN_POINT ( 'NONE',  ( 162.9148248802443106, 248.4702413316674381, 9.709394404200100581 ) ) ;
#25464=CARTESIAN_POINT ( 'NONE',  ( -0.9067010812963882671, 158.0327760586659451, 1.948934522072303157E-15 ) ) ;
#25466=CARTESIAN_POINT ( 'NONE',  ( 164.0724714897467607, 247.3131831635135711, 6.957961843141012181 ) ) ;
#25467=CARTESIAN_POINT ( 'NONE',  ( 200.4168219705828449, 282.9326697566199869, 16.82828662466668845 ) ) ;
#25468=CARTESIAN_POINT ( 'NONE',  ( 153.1164404339926080, 265.4415410246681972, 16.15325778160653414 ) ) ;
#25470=CARTESIAN_POINT ( 'NONE',  ( 156.0731593180878178, 261.2610882355718331, -17.28887939065674573 ) ) ;
#25471=CARTESIAN_POINT ( 'NONE',  ( 183.7664330935276951, 256.7078052723039718, -1.761079896072507145 ) ) ;
#25473=ORIENTED_EDGE ( 'NONE', *, *, #73261, .F. ) ;
#25474=CARTESIAN_POINT ( 'NONE',  ( 196.2630260332681189, 290.7094625936034049, -17.43112004684450866 ) ) ;
#25478=CARTESIAN_POINT ( 'NONE',  ( 165.8170486466665068, 285.4962505645767692, 0.4920860348752986169 ) ) ;
#25481=CARTESIAN_POINT ( 'NONE',  ( 153.7162572231245292, 275.1202623374771861, 10.51805260027509981 ) ) ;
#25483=EDGE_CURVE ( 'NONE', #23533, #90262, #10521, .T. ) ;
#25485=CARTESIAN_POINT ( 'NONE',  ( 152.7618747630824885, 266.0556667813044101, 16.41480086888796919 ) ) ;
#25486=CARTESIAN_POINT ( 'NONE',  ( 165.0532575723395041, 244.7663672603923715, -2.144843157699870773 ) ) ;
#25489=CARTESIAN_POINT ( 'NONE',  ( 155.0898745997320134, 262.0234527842152374, 17.05457557403769542 ) ) ;
#25491=ORIENTED_EDGE ( 'NONE', *, *, #29284, .F. ) ;
#25492=CARTESIAN_POINT ( 'NONE',  ( 155.7871210497565642, 277.0951557919157722, -10.36611183180045082 ) ) ;
#25494=ORIENTED_EDGE ( 'NONE', *, *, #70925, .T. ) ;
#25495=CARTESIAN_POINT ( 'NONE',  ( 193.1318887679063039, 292.6717260935084255, 15.39800915952812588 ) ) ;
#25496=EDGE_CURVE ( 'NONE', #24384, #39418, #87922, .T. ) ;
#25498=ORIENTED_EDGE ( 'NONE', *, *, #17580, .T. ) ;
#25500=ADVANCED_FACE ( 'NONE', ( #72675 ), #49347, .T. ) ;
#25503=AXIS2_PLACEMENT_3D ( 'NONE', #78022, #8612, #70403 ) ;
#25506=CARTESIAN_POINT ( 'NONE',  ( 200.7897860911934913, 282.8688841796032420, 18.17522996445731920 ) ) ;
#25507=CARTESIAN_POINT ( 'NONE',  ( 168.3012556413555387, 276.0081633973304633, -16.37610827237247335 ) ) ;
#25509=CARTESIAN_POINT ( 'NONE',  ( 150.7226148805041817, 269.5877685077668957, 15.52819754351937576 ) ) ;
#25511=B_SPLINE_CURVE_WITH_KNOTS ( 'NONE', 3,
 ( #189, #60974, #61962, #23468 ),
 .UNSPECIFIED., .F., .F.,
 ( 4, 4 ),
 ( 0.01631437863335180247, 0.02516723697892677206 ),
 .UNSPECIFIED. ) ;
#25513=CARTESIAN_POINT ( 'NONE',  ( 198.1063734369593590, 266.1900715569024669, 6.878534305327493215 ) ) ;
#25516=ORIENTED_EDGE ( 'NONE', *, *, #7280, .F. ) ;
#25517=CARTESIAN_POINT ( 'NONE',  ( 160.3554891620578076, 268.8548341825590455, -16.71133067088820567 ) ) ;
#25519=CARTESIAN_POINT ( 'NONE',  ( 160.4237162281696953, 273.2376347127639633, -15.66572034412998882 ) ) ;
#25522=CARTESIAN_POINT ( 'NONE',  ( 159.1510347580164648, 259.5013206209943064, 16.69515602809037347 ) ) ;
#25523=CARTESIAN_POINT ( 'NONE',  ( 168.6746947616884711, 272.7949930551382636, 15.97852131846135038 ) ) ;
#25524=CARTESIAN_POINT ( 'NONE',  ( 193.8013783128415639, 294.9731615157183455, 13.35591610390495632 ) ) ;
#25525=CARTESIAN_POINT ( 'NONE',  ( 192.1943038168404314, 277.1473907896511264, 17.36549850453357635 ) ) ;
#25529=CARTESIAN_POINT ( 'NONE',  ( 197.5889545809544927, 288.4128869818045473, -18.07878478781679732 ) ) ;
#25532=CARTESIAN_POINT ( 'NONE',  ( 162.7028393313443360, 279.7088927405546883, -12.24337270576748438 ) ) ;
#25534=CARTESIAN_POINT ( 'NONE',  ( 164.8849641302980444, 245.0578600525887794, 2.884140591399200648 ) ) ;
#25535=CARTESIAN_POINT ( 'NONE',  ( 191.1729615630557646, 298.6818583910219331, -8.222589559603353138 ) ) ;
#25536=CARTESIAN_POINT ( 'NONE',  ( 198.2040940955416488, 287.3474340887963763, 16.95806375232200480 ) ) ;
#25541=CARTESIAN_POINT ( 'NONE',  ( 169.6843210851487527, 258.2382094438814875, -14.02289787536656185 ) ) ;
#25543=FACE_OUTER_BOUND ( 'NONE', #55925, .T. ) ;
#25544=CARTESIAN_POINT ( 'NONE',  ( 200.7583183585857967, 282.9233878912788214, 16.96937806979494212 ) ) ;
#25545=DIRECTION ( 'NONE',  ( -0.8660254037844387076, -0.4999999999999998890, -0.000000000000000000 ) ) ;
#25547=CARTESIAN_POINT ( 'NONE',  ( 159.9882936611505500, 262.0288864495718144, -17.79556786074740415 ) ) ;
#25550=CARTESIAN_POINT ( 'NONE',  ( 134.6710330032098000, 241.8927522451418497, 10.00000000000009948 ) ) ;
#25552=CARTESIAN_POINT ( 'NONE',  ( 16.74724052122864393, 187.1427522451419065, 10.00000000000009237 ) ) ;
#25553=CARTESIAN_POINT ( 'NONE',  ( 100.4182711614829486, 216.5327760586659451, 1.948934522072302763E-15 ) ) ;
#25557=CARTESIAN_POINT ( 'NONE',  ( 170.1875097353064916, 280.4626186455269590, -13.75171363026703730 ) ) ;
#25558=CARTESIAN_POINT ( 'NONE',  ( 23.17910981781079727, 190.3149278399161233, -9.188101187500095079 ) ) ;
#25559=EDGE_CURVE ( 'NONE', #80879, #54426, #33485, .T. ) ;
#25560=CARTESIAN_POINT ( 'NONE',  ( 161.4396252346964218, 251.0253620690641299, 14.51972485405798885 ) ) ;
#25561=ORIENTED_EDGE ( 'NONE', *, *, #35687, .F. ) ;
#25563=CARTESIAN_POINT ( 'NONE',  ( 200.1200414979239213, 267.3440445008968709, -2.849651934370048600 ) ) ;
#25567=CARTESIAN_POINT ( 'NONE',  ( -22.42236680055709641, 157.8615022471902591, 0.000000000000000000 ) ) ;
#25568=CARTESIAN_POINT ( 'NONE',  ( 192.7288556637334125, 292.1918731402626577, -15.52061534916644447 ) ) ;
#25571=CARTESIAN_POINT ( 'NONE',  ( 29.83685365728618066, 188.0333772461660544, 9.188101187500095079 ) ) ;
#25572=CARTESIAN_POINT ( 'NONE',  ( 80.11143256479013530, 210.3927522451417929, 10.00000000000009592 ) ) ;
#25573=AXIS2_PLACEMENT_3D ( 'NONE', #9272, #39137, #85836 ) ;
#25574=CARTESIAN_POINT ( 'NONE',  ( 97.79278455872238851, 227.2677522451418497, 10.00000000000009592 ) ) ;
#25575=ORIENTED_EDGE ( 'NONE', *, *, #62756, .F. ) ;
#25578=CARTESIAN_POINT ( 'NONE',  ( 178.9086871400862719, 258.8446539160876796, -10.04105931206729529 ) ) ;
#25580=CARTESIAN_POINT ( 'NONE',  ( 0.1211834420501121806, 177.0024278399160949, -9.188101187500093303 ) ) ;
#25583=CARTESIAN_POINT ( 'NONE',  ( 198.9369963555428740, 286.0780101374919013, -18.58432392708837710 ) ) ;
#25584=CARTESIAN_POINT ( 'NONE',  ( 186.6165385818496247, 282.6660768309312743, 16.17880700807253191 ) ) ;
#25585=CARTESIAN_POINT ( 'NONE',  ( 147.6512387128590262, 274.9075480792844246, -8.209968531507987777 ) ) ;
#25587=CARTESIAN_POINT ( 'NONE',  ( 164.4294002498235159, 245.8469198396639399, 6.098783631055905374 ) ) ;
#25588=CARTESIAN_POINT ( 'NONE',  ( 191.5893301551938350, 298.8045413135534432, -8.323356515452589477 ) ) ;
#25590=EDGE_CURVE ( 'NONE', #27771, #60705, #99864, .T. ) ;
#25594=CARTESIAN_POINT ( 'NONE',  ( 99.22679203974932705, 240.3464784336661637, 1.353441290958777327E-15 ) ) ;
#25597=CARTESIAN_POINT ( 'NONE',  ( 35.87196818813498567, 201.5177522451419350, 5.000000000000046185 ) ) ;
#25600=CARTESIAN_POINT ( 'NONE',  ( 185.5365472822558672, 288.1719225632029406, 15.10228555286701813 ) ) ;
#25601=CARTESIAN_POINT ( 'NONE',  ( 191.0098866877199271, 299.8081668393321024, -6.439016407525185670 ) ) ;
#25603=CARTESIAN_POINT ( 'NONE',  ( 190.2102363550532118, 262.0023303024768779, -4.404598936143417909 ) ) ;
#25604=CARTESIAN_POINT ( 'NONE',  ( 149.2223635749290622, 272.1862799931444670, -12.97307652490353647 ) ) ;
#25605=CARTESIAN_POINT ( 'NONE',  ( 192.0603001030472683, 293.3461588932823929, -14.68827779892621344 ) ) ;
#25606=CARTESIAN_POINT ( 'NONE',  ( 173.1401207867795335, 289.7447317016536772, -1.382016094127694217 ) ) ;
#25608=VERTEX_POINT ( 'NONE', #65044 ) ;
#25610=CARTESIAN_POINT ( 'NONE',  ( 175.4103267356181846, 278.8476840418515508, 15.42183127757729189 ) ) ;
#25611=CARTESIAN_POINT ( 'NONE',  ( 166.1693173614613102, 270.1811453668383933, -16.28491390599275590 ) ) ;
#25614=CARTESIAN_POINT ( 'NONE',  ( 199.4244589065890523, 272.3134371430058422, 12.33418413535176761 ) ) ;
#25617=CARTESIAN_POINT ( 'NONE',  ( 148.2992785150285613, 274.6248789480700907, 6.993002833606254853 ) ) ;
#25618=EDGE_CURVE ( 'NONE', #47527, #74125, #11376, .T. ) ;
#25620=CARTESIAN_POINT ( 'NONE',  ( 191.2498569334766216, 280.2133405228250354, 17.23712193076469745 ) ) ;
#25622=CARTESIAN_POINT ( 'NONE',  ( 192.1027933011355344, 288.1354424464720410, -15.86813138701040060 ) ) ;
#25625=CARTESIAN_POINT ( 'NONE',  ( 147.9791529310278122, 274.3395839928920168, -7.789432462804474433 ) ) ;
#25631=CARTESIAN_POINT ( 'NONE',  ( 188.8123896052067607, 293.6903704042900358, 12.84215840511197193 ) ) ;
#25634=CARTESIAN_POINT ( 'NONE',  ( 198.2391837281077756, 286.3575794386269422, 17.25947343406376078 ) ) ;
#25637=CARTESIAN_POINT ( 'NONE',  ( 27.13954536664190798, 193.1427522451419065, 10.00000000000009415 ) ) ;
#25638=ADVANCED_FACE ( 'NONE', ( #17961 ), #57428, .T. ) ;
#25641=ORIENTED_EDGE ( 'NONE', *, *, #36443, .F. ) ;
#25642=CARTESIAN_POINT ( 'NONE',  ( 178.9149458720169719, 260.2138664454146806, 12.17723821761245695 ) ) ;
#25646=CARTESIAN_POINT ( 'NONE',  ( 173.3860743566676774, 270.4884716614657805, 17.09475665396154298 ) ) ;
#25647=CARTESIAN_POINT ( 'NONE',  ( 155.5322964227545413, 261.2571557083629159, -18.35853982030605280 ) ) ;
#25649=CARTESIAN_POINT ( 'NONE',  ( 186.1509274190741223, 282.5035783377156804, -17.04520025225239266 ) ) ;
#25650=CARTESIAN_POINT ( 'NONE',  ( 165.0817809681736037, 244.7169632896033136, -1.727194264083430131 ) ) ;
#25651=CARTESIAN_POINT ( 'NONE',  ( 189.9593806053207459, 301.6276967477073754, 3.110130642237009191 ) ) ;
#25655=CARTESIAN_POINT ( 'NONE',  ( 200.7484899876179441, 282.9404111291507888, -16.88964748465601673 ) ) ;
#25658=CARTESIAN_POINT ( 'NONE',  ( 155.9389183335434552, 280.0307964060903601, 2.100540160644290832 ) ) ;
#25659=CARTESIAN_POINT ( 'NONE',  ( 129.7002344832967538, 251.8149278399160949, -9.188101187500095079 ) ) ;
#25662=VECTOR ( 'NONE', #93464, 1000.000000000000000 ) ;
#25665=ORIENTED_EDGE ( 'NONE', *, *, #54183, .T. ) ;
#25666=CARTESIAN_POINT ( 'NONE',  ( 203.5059372267095625, 276.4897655546087663, 14.10020651900479294 ) ) ;
#25668=CARTESIAN_POINT ( 'NONE',  ( 173.8869354466250456, 290.5925258257277619, -4.931910953996751168 ) ) ;
#25670=CARTESIAN_POINT ( 'NONE',  ( 156.5044409881847685, 278.9616761084025143, 7.288134256061602478 ) ) ;
#25671=CARTESIAN_POINT ( 'NONE',  ( 153.0790963368640689, 265.5062228982576471, -17.74594954892339160 ) ) ;
#25673=CARTESIAN_POINT ( 'NONE',  ( 207.5270645556383329, 271.1995755744450207, 0.000000000000000000 ) ) ;
#25674=CARTESIAN_POINT ( 'NONE',  ( 155.0568450317760494, 264.0806616740677555, 17.52241723436104337 ) ) ;
#25677=LINE ( 'NONE', #34751, #12215 ) ;
#25678=CARTESIAN_POINT ( 'NONE',  ( 188.6826127332440421, 272.6057162039079458, 16.71479996418005243 ) ) ;
#25680=CARTESIAN_POINT ( 'NONE',  ( 163.6128237694224765, 277.6105145936779763, 13.01957428213605361 ) ) ;
#25681=CARTESIAN_POINT ( 'NONE',  ( 204.0366409255401834, 269.1163672225195000, -2.920898469201972159 ) ) ;
#25682=B_SPLINE_CURVE_WITH_KNOTS ( 'NONE', 3,
 ( #78242, #8823, #76257, #24522 ),
 .UNSPECIFIED., .F., .F.,
 ( 4, 4 ),
 ( 0.005090543101624064523, 0.01311434132611732917 ),
 .UNSPECIFIED. ) ;
#25683=CARTESIAN_POINT ( 'NONE',  ( 191.6828115734357425, 298.6426267475946474, -9.425347171908683208 ) ) ;
#25684=CARTESIAN_POINT ( 'NONE',  ( 149.5593209768671841, 271.6026526530012575, 11.55487339793564949 ) ) ;
#25685=CARTESIAN_POINT ( 'NONE',  ( 202.9093905060991005, 279.1976216410395182, 16.97070083370504179 ) ) ;
#25686=CARTESIAN_POINT ( 'NONE',  ( 164.5925561631139260, 283.7481285952978283, -6.766772729352702243 ) ) ;
#25687=CARTESIAN_POINT ( 'NONE',  ( 160.9037366693648039, 281.5822211133703945, 5.837102615454335286 ) ) ;
#25689=DIRECTION ( 'NONE',  ( -0.8660254037844387076, -0.4999999999999998890, -0.000000000000000000 ) ) ;
#25693=CARTESIAN_POINT ( 'NONE',  ( 191.5557312797294287, 275.2428672974049277, -15.79654600051574498 ) ) ;
#25695=CARTESIAN_POINT ( 'NONE',  ( 204.2663578856130755, 276.4680603110491575, 13.28230551973123852 ) ) ;
#25700=CARTESIAN_POINT ( 'NONE',  ( 91.08134800299070832, 214.2048013555409796, 4.594050593750051981 ) ) ;
#25701=CARTESIAN_POINT ( 'NONE',  ( 203.5477091018662748, 278.0920214017542662, -16.09930363698006062 ) ) ;
#25702=CARTESIAN_POINT ( 'NONE',  ( 146.7943851877206214, 276.3916619194686746, -4.608908220452185844 ) ) ;
#25703=LINE ( 'NONE', #71812, #4265 ) ;
#25704=EDGE_CURVE ( 'NONE', #99455, #62377, #15325, .T. ) ;
#25705=CARTESIAN_POINT ( 'NONE',  ( -22.42236680055709641, 157.8615022471902591, 0.000000000000000000 ) ) ;
#25708=CARTESIAN_POINT ( 'NONE',  ( 161.3547410062914480, 281.8923609553542065, 5.601659783808949911 ) ) ;
#25711=CARTESIAN_POINT ( 'NONE',  ( 207.4925036560929925, 271.2594368084131702, 4.868688772655199948 ) ) ;
#25712=B_SPLINE_CURVE_WITH_KNOTS ( 'NONE', 3,
 ( #28348, #90202, #43032, #88725, #95821, #20776, #82615, #26374, #57251, #88225, #44035, #21267, #28864, #98277, #59742, #83094, #74976, #5557, #90711, #52145, #93409, #94406, #62965, #33068, #8771, #55348, #669, #40149, #9791, #2185, #63470, #24468, #10278, #56356, #47261, #64473, #40652, #1689, #78182, #39640, #23959, #95433, #63962, #41148, #32053, #94904, #70562, #78687 ),
 .UNSPECIFIED., .F., .F.,
 ( 4, 2, 2, 2, 2, 2, 2, 2, 2, 2, 2, 2, 2, 2, 2, 2, 2, 2, 2, 2, 2, 2, 2, 4 ),
 ( 0.0005725079143340260123, 0.001009693989615074224, 0.001228287027255563256, 0.001337583546075807664, 0.001446880064896052288, 0.001556176583716296913, 0.001665473102536541104, 0.001884066140176979612, 0.002321252215457800250, 0.003195624366019438924, 0.004069996516581078465, 0.004944368667142717139, 0.005381554742423579410, 0.005600147780063974984, 0.005709444298884176240, 0.005764092558294238271, 0.005818740817704299434, 0.005873389077114361465, 0.005928037336524423495, 0.006037333855344682865, 0.006255926892985246707, 0.006693112968266370921, 0.007130299043547496003, 0.007567485118828620218 ),
 .UNSPECIFIED. ) ;
#25714=CARTESIAN_POINT ( 'NONE',  ( 205.1568691672349871, 275.3048744110253097, -13.82554525023989989 ) ) ;
#25717=ADVANCED_FACE ( 'NONE', ( #97461 ), #22109, .F. ) ;
#25719=CARTESIAN_POINT ( 'NONE',  ( 39.47103917862304456, 205.8464784336661637, 1.353441290958777327E-15 ) ) ;
#25722=CARTESIAN_POINT ( 'NONE',  ( 69.07880331415105957, 204.5643266524160140, 9.188101187500095079 ) ) ;
#25723=CARTESIAN_POINT ( 'NONE',  ( 164.6517207862732164, 247.1756023946066989, -7.101760799815486358 ) ) ;
#25724=CARTESIAN_POINT ( 'NONE',  ( -22.42236680055709641, 157.8615022471902591, 0.000000000000000000 ) ) ;
#25725=CARTESIAN_POINT ( 'NONE',  ( 164.1326753310708284, 258.2664819102902243, 15.54305778615748501 ) ) ;
#25732=CARTESIAN_POINT ( 'NONE',  ( 196.4783028304046013, 290.3365922432724346, -16.37291435488387492 ) ) ;
#25733=ORIENTED_EDGE ( 'NONE', *, *, #65744, .T. ) ;
#25735=CARTESIAN_POINT ( 'NONE',  ( 80.68904315757745849, 208.2048013555409796, 4.594050593750051981 ) ) ;
#25738=CARTESIAN_POINT ( 'NONE',  ( 169.3079978421220630, 288.1705777629971976, -1.100478215856383279 ) ) ;
#25740=CARTESIAN_POINT ( 'NONE',  ( 153.7968043968548386, 264.2631160733518527, 16.53979738298849611 ) ) ;
#25741=B_SPLINE_CURVE_WITH_KNOTS ( 'NONE', 3,
 ( #52315, #74656, #6218, #75144, #59400, #7208, #36610, #37602, #91861, #14811, #90376, #30012, #53309, #51837, #90880, #82777, #98447, #67517 ),
 .UNSPECIFIED., .F., .F.,
 ( 4, 2, 2, 2, 2, 2, 2, 2, 4 ),
 ( 1.387778780781445676E-17, 0.0002767872370572536196, 0.0005535744741144933614, 0.0008303617111717331032, 0.001107148948228972845, 0.001383936185286212695, 0.001660723422343452329, 0.001937510659400691962, 0.002214297896457931812 ),
 .UNSPECIFIED. ) ;
#25743=CARTESIAN_POINT ( 'NONE',  ( 189.8136429382303731, 286.6226720265459562, 16.81544881319448592 ) ) ;
#25744=CARTESIAN_POINT ( 'NONE',  ( 120.0388121219830708, 240.1115022471902307, 10.00000000000009592 ) ) ;
#25745=CARTESIAN_POINT ( 'NONE',  ( 157.6668627405778409, 257.5599783937680058, -16.78811156090270629 ) ) ;
#25749=CARTESIAN_POINT ( 'NONE',  ( 188.2088990708346614, 273.3690300468384180, 15.62809882445249876 ) ) ;
#25751=CARTESIAN_POINT ( 'NONE',  ( 159.9770824720811220, 253.5585604421560788, -16.42166711341322483 ) ) ;
#25755=CARTESIAN_POINT ( 'NONE',  ( 174.7476935608443114, 252.4984142128707845, -0.2521487975539727922 ) ) ;
#25756=VERTEX_POINT ( 'NONE', #9224 ) ;
#25757=CARTESIAN_POINT ( 'NONE',  ( 189.3112218707861700, 290.0744326881770689, 14.37879668408311495 ) ) ;
#25759=CARTESIAN_POINT ( 'NONE',  ( 50.59440005247052596, 190.0177522451418213, 5.000000000000051514 ) ) ;
#25760=B_SPLINE_CURVE_WITH_KNOTS ( 'NONE', 3,
 ( #93594, #94597, #24653, #25151, #87028, #18074, #90506, #13469, #66653, #80919, #97581, #51955, #12475, #65651, #50452, #44338 ),
 .UNSPECIFIED., .F., .F.,
 ( 4, 2, 2, 2, 2, 2, 2, 4 ),
 ( 3.103167691559091397E-17, 0.0003787177898468203126, 0.0007574355796936096171, 0.001136153369540402825, 0.001514871159387196032, 0.001893588949233989023, 0.002272306739080782664, 0.003029742318774367345 ),
 .UNSPECIFIED. ) ;
#25769=LINE ( 'NONE', #88113, #43299 ) ;
#25770=DIRECTION ( 'NONE',  ( -0.8660254037844387076, -0.4999999999999998890, -0.000000000000000000 ) ) ;
#25772=EDGE_LOOP ( 'NONE', ( #29970, #94432, #75758, #615 ) ) ;
#25773=CARTESIAN_POINT ( 'NONE',  ( 183.1259174442036510, 295.7551109177733792, 0.9378797900342676908 ) ) ;
#25775=CARTESIAN_POINT ( 'NONE',  ( 194.9636675848471441, 292.9600174435121289, -15.57898232594655319 ) ) ;
#25777=CARTESIAN_POINT ( 'NONE',  ( 194.2321518193436987, 294.2270399159019121, 13.98132384850917020 ) ) ;
#25778=CARTESIAN_POINT ( 'NONE',  ( 185.3422210113485562, 292.6085084928443507, -11.74510369913683761 ) ) ;
#25780=CARTESIAN_POINT ( 'NONE',  ( 164.0017338887578546, 246.5876597057176696, 4.694633606064320119 ) ) ;
#25783=CARTESIAN_POINT ( 'NONE',  ( 86.39896429407481548, 226.8149278399160664, 9.188101187500093303 ) ) ;
#25784=ORIENTED_EDGE ( 'NONE', *, *, #88057, .F. ) ;
#25787=ORIENTED_EDGE ( 'NONE', *, *, #5397, .T. ) ;
#25788=CARTESIAN_POINT ( 'NONE',  ( 195.5498780363893729, 291.9446711575129711, -17.20314750324050834 ) ) ;
#25789=ORIENTED_EDGE ( 'NONE', *, *, #29293, .F. ) ;
#25794=CARTESIAN_POINT ( 'NONE',  ( 206.7893622945242385, 272.4773133715531230, -10.52881283832460291 ) ) ;
#25796=CARTESIAN_POINT ( 'NONE',  ( 91.91987624320061911, 230.0024278399160949, 9.188101187500095079 ) ) ;
#25797=ORIENTED_EDGE ( 'NONE', *, *, #79029, .T. ) ;
#25800=CARTESIAN_POINT ( 'NONE',  ( 207.6837091943624785, 270.9282591014416539, -1.156610046911421552 ) ) ;
#25801=ORIENTED_EDGE ( 'NONE', *, *, #20412, .T. ) ;
#25802=EDGE_CURVE ( 'NONE', #61069, #78457, #46742, .T. ) ;
#25811=VERTEX_POINT ( 'NONE', #96361 ) ;
#25812=CARTESIAN_POINT ( 'NONE',  ( 204.3646970165318351, 276.6769568243839217, 14.33703115251539018 ) ) ;
#25814=DIRECTION ( 'NONE',  ( -0.8660254037844387076, -0.4999999999999998890, -0.000000000000000000 ) ) ;
#25815=CARTESIAN_POINT ( 'NONE',  ( 192.2600176540098857, 271.9115477842126438, 14.16314048194649544 ) ) ;
#25818=FACE_OUTER_BOUND ( 'NONE', #91358, .T. ) ;
#25820=CARTESIAN_POINT ( 'NONE',  ( 149.0764958053571263, 274.4627432579617334, 9.065804115783038242 ) ) ;
#25822=CARTESIAN_POINT ( 'NONE',  ( 161.1027382213887336, 251.6088674925233022, 13.55451100897754557 ) ) ;
#25826=CARTESIAN_POINT ( 'NONE',  ( 178.3941412731578851, 291.5035416958068595, -6.132204003346442001 ) ) ;
#25827=CARTESIAN_POINT ( 'NONE',  ( 163.1017244536801343, 248.1465217745638654, -10.44344155757014114 ) ) ;
#25828=B_SPLINE_CURVE_WITH_KNOTS ( 'NONE', 3,
 ( #16805, #9213, #31002, #40087, #92842, #23393, #9737, #55779, #86770, #54283, #17306, #71531, #41596, #56296, #64917, #57298, #19342, #4102 ),
 .UNSPECIFIED., .F., .F.,
 ( 4, 2, 2, 2, 2, 2, 2, 2, 4 ),
 ( 0.000000000000000000, 0.0002735155329757442671, 0.0005470310659514885342, 0.0008205465989272328012, 0.001094062131902977068, 0.001367577664878721335, 0.001641093197854465602, 0.001914608730830209870, 0.002188124263805954137 ),
 .UNSPECIFIED. ) ;
#25829=VERTEX_POINT ( 'NONE', #71542 ) ;
#25831=CARTESIAN_POINT ( 'NONE',  ( 164.9836323268835940, 244.8869617230113249, -2.696511969808454534 ) ) ;
#25832=CARTESIAN_POINT ( 'NONE',  ( 182.3781704481015140, 264.5827396642109193, 13.45902643938770638 ) ) ;
#25833=CARTESIAN_POINT ( 'NONE',  ( 176.0733391018527527, 285.3569424919562607, -13.18445672484209830 ) ) ;
#25836=FACE_OUTER_BOUND ( 'NONE', #16784, .T. ) ;
#25837=CARTESIAN_POINT ( 'NONE',  ( 180.4423813072727967, 272.9747474098779207, 17.19032754332442181 ) ) ;
#25838=CARTESIAN_POINT ( 'NONE',  ( 161.0025371176779174, 273.2044621363186820, -15.07898562200838199 ) ) ;
#25839=CARTESIAN_POINT ( 'NONE',  ( 150.5438776023515004, 278.3016033182416322, -9.804454847755098641E-05 ) ) ;
#25841=CARTESIAN_POINT ( 'NONE',  ( 161.8150574665248200, 250.3750943687383881, -13.25074899737357903 ) ) ;
#25842=CARTESIAN_POINT ( 'NONE',  ( -5.237175195983594378, 167.7833772461660828, -9.188101187500095079 ) ) ;
#25847=CARTESIAN_POINT ( 'NONE',  ( 40.66251830035667325, 182.0327760586659451, 1.948934522072302763E-15 ) ) ;
#25848=CARTESIAN_POINT ( 'NONE',  ( 161.4469036912142599, 251.0127554125742222, 12.93933463576739307 ) ) ;
#25852=CARTESIAN_POINT ( 'NONE',  ( 107.5017976953482446, 221.3262482093458061, 3.021315404115420679E-15 ) ) ;
#25853=CARTESIAN_POINT ( 'NONE',  ( 149.0436225622167115, 272.4958685085585444, 12.76381714291240144 ) ) ;
#25854=CARTESIAN_POINT ( 'NONE',  ( 182.3215694434810246, 280.0626234744391923, -16.09935857771849044 ) ) ;
#25856=CARTESIAN_POINT ( 'NONE',  ( 186.8734402896601807, 295.9231036555426044, -7.697649258255485627 ) ) ;
#25858=CARTESIAN_POINT ( 'NONE',  ( 83.23273246114447943, 208.8615022471902023, 5.000000000000051514 ) ) ;
#25859=CARTESIAN_POINT ( 'NONE',  ( 164.9965579215539151, 246.0088170146208597, 0.8672894934246058174 ) ) ;
#25862=CARTESIAN_POINT ( 'NONE',  ( 36.16949087457737733, 197.8149278399160949, -9.188101187500095079 ) ) ;
#25864=ORIENTED_EDGE ( 'NONE', *, *, #96849, .F. ) ;
#25866=CARTESIAN_POINT ( 'NONE',  ( 190.1693911629507738, 301.2639477917662703, -5.112716700269980485 ) ) ;
#25871=CARTESIAN_POINT ( 'NONE',  ( 168.0367729244566988, 281.8922763585110260, -11.02587170619616508 ) ) ;
#25875=CARTESIAN_POINT ( 'NONE',  ( 202.2603678735342214, 280.3217618159037556, 16.49712126737133744 ) ) ;
#25876=CARTESIAN_POINT ( 'NONE',  ( 111.2365322456207224, 223.4824982072973683, 3.021315404115420679E-15 ) ) ;
#25877=CARTESIAN_POINT ( 'NONE',  ( 204.5482460332032986, 276.3590406018296903, 14.63243279326650814 ) ) ;
#25878=ORIENTED_EDGE ( 'NONE', *, *, #68441, .F. ) ;
#25880=CARTESIAN_POINT ( 'NONE',  ( 172.0974426341863932, 252.4089283455955410, 8.839998632889988883 ) ) ;
#25883=VERTEX_POINT ( 'NONE', #98830 ) ;
#25884=CARTESIAN_POINT ( 'NONE',  ( 178.6998812467141420, 282.4658996288984554, 15.77537290851580032 ) ) ;
#25890=VECTOR ( 'NONE', #59550, 1000.000000000000000 ) ;
#25891=VERTEX_POINT ( 'NONE', #29412 ) ;
#25893=CARTESIAN_POINT ( 'NONE',  ( 150.9171781617125134, 270.0645241841637016, -13.65841583251952684 ) ) ;
#25894=CARTESIAN_POINT ( 'NONE',  ( 149.5390997184345281, 271.6376768999995761, -11.52989534384373016 ) ) ;
#25896=CARTESIAN_POINT ( 'NONE',  ( 153.2283961777204695, 265.2476279883323400, -17.66880461074566000 ) ) ;
#25897=DIRECTION ( 'NONE',  ( -0.8660254037844387076, -0.4999999999999998890, -0.000000000000000000 ) ) ;
#25900=CARTESIAN_POINT ( 'NONE',  ( 204.7519188734507622, 276.0062688943993408, -12.76027478560537531 ) ) ;
#25901=CARTESIAN_POINT ( 'NONE',  ( 122.5830220656496579, 232.3923013555409796, 4.594050593750050204 ) ) ;
#25902=EDGE_CURVE ( 'NONE', #74173, #49930, #18973, .T. ) ;
#25903=CARTESIAN_POINT ( 'NONE',  ( 180.4744007604609237, 287.0154873131820636, -13.59564979728018130 ) ) ;
#25904=EDGE_LOOP ( 'NONE', ( #3245, #5070, #84950, #12086 ) ) ;
#25905=CARTESIAN_POINT ( 'NONE',  ( 201.3171141051938378, 281.5403940053560632, 16.35011633700059974 ) ) ;
#25906=ORIENTED_EDGE ( 'NONE', *, *, #66106, .T. ) ;
#25908=CARTESIAN_POINT ( 'NONE',  ( 197.8822014719394531, 287.9049684674569676, 17.88172308374019792 ) ) ;
#25909=CARTESIAN_POINT ( 'NONE',  ( 204.6350011963004647, 275.7068757420208271, -12.64342396695018245 ) ) ;
#25910=CARTESIAN_POINT ( 'NONE',  ( 48.80796233711527776, 208.1744531367911293, 4.594050593750047540 ) ) ;
#25912=CARTESIAN_POINT ( 'NONE',  ( 151.4159295687746294, 268.3869122420484814, 14.78076517566594106 ) ) ;
#25913=CARTESIAN_POINT ( 'NONE',  ( 150.3996455637841621, 270.1471677736116703, 15.13740740754872327 ) ) ;
#25914=CARTESIAN_POINT ( 'NONE',  ( 172.6297427891187795, 271.8127495741235293, 17.53455634568126698 ) ) ;
#25916=DIRECTION ( 'NONE',  ( 0.8660254037844395958, 0.4999999999999985567, 0.000000000000000000 ) ) ;
#25918=CARTESIAN_POINT ( 'NONE',  ( 189.8147415777049218, 301.8782188922952514, -0.5019643756309712934 ) ) ;
#25920=CARTESIAN_POINT ( 'NONE',  ( 171.7130510479120744, 259.4982484653344272, -13.85566588815878752 ) ) ;
#25922=CARTESIAN_POINT ( 'NONE',  ( 160.5099781893591455, 258.1706592185460067, -17.21824937912870013 ) ) ;
#25924=CARTESIAN_POINT ( 'NONE',  ( 149.6877696051026305, 271.3801731027346591, 11.89134584187677390 ) ) ;
#25925=CARTESIAN_POINT ( 'NONE',  ( 41.66351307949141614, 184.8615022471902023, 5.000000000000051514 ) ) ;
#25928=CARTESIAN_POINT ( 'NONE',  ( 167.4563420731973338, 256.4722478396594170, 13.70524261881715589 ) ) ;
#25930=CARTESIAN_POINT ( 'NONE',  ( 134.8967340017684080, 242.5643266524159856, -9.188101187500093303 ) ) ;
#25932=CARTESIAN_POINT ( 'NONE',  ( 191.0604813119340690, 299.7205343796033503, -9.270812881586136811 ) ) ;
#25935=CARTESIAN_POINT ( 'NONE',  ( 182.7869685246910194, 285.6357107071319774, -15.76494286922655874 ) ) ;
#25937=CARTESIAN_POINT ( 'NONE',  ( 175.5249711800137220, 253.6457629656688653, 4.969749041686572610 ) ) ;
#25941=CARTESIAN_POINT ( 'NONE',  ( 158.3969645014495882, 274.9141732135112761, -12.53854624713853028 ) ) ;
#25942=CARTESIAN_POINT ( 'NONE',  ( 185.9504045463281443, 261.9056071599655411, 9.988078213316251563 ) ) ;
#25943=CARTESIAN_POINT ( 'NONE',  ( 165.0424088038023456, 244.7851578786982145, -1.332161216135762105 ) ) ;
#25944=CARTESIAN_POINT ( 'NONE',  ( 145.6409484414103588, 245.7048013555409511, 4.594050593750051981 ) ) ;
#25947=CARTESIAN_POINT ( 'NONE',  ( 185.9561589036855764, 296.7738594392127425, 4.656816216167465328 ) ) ;
#25949=B_SPLINE_CURVE_WITH_KNOTS ( 'NONE', 3,
 ( #86240, #23368, #55258, #70477 ),
 .UNSPECIFIED., .F., .F.,
 ( 4, 4 ),
 ( 0.01390897628007791570, 0.02024841952128482447 ),
 .UNSPECIFIED. ) ;
#25950=CARTESIAN_POINT ( 'NONE',  ( 59.93088934303040816, 217.6589784336661637, -6.496448406907675876E-16 ) ) ;
#25951=CARTESIAN_POINT ( 'NONE',  ( 207.6727254509676186, 270.9472835030587703, 7.315149605389819953 ) ) ;
#25952=CARTESIAN_POINT ( 'NONE',  ( 174.2379957965557651, 251.2590728793752248, 3.639292605338433795 ) ) ;
#25954=CARTESIAN_POINT ( 'NONE',  ( 171.1110197743758476, 259.7606215877287923, 15.15264976788713902 ) ) ;
#25955=CARTESIAN_POINT ( 'NONE',  ( 153.0048580355102672, 278.5866977936228182, -1.606994127711936615 ) ) ;
#25957=CARTESIAN_POINT ( 'NONE',  ( 203.0862352702880003, 278.8913175244117610, -15.09542727681365015 ) ) ;
#25958=ADVANCED_FACE ( 'NONE', ( #69891 ), #62278, .T. ) ;
#25959=CARTESIAN_POINT ( 'NONE',  ( 156.9763224152064822, 271.9908631200777904, -15.29896765642516776 ) ) ;
#25960=CARTESIAN_POINT ( 'NONE',  ( 131.5677753063155251, 236.7677522451417929, -5.000000000000041744 ) ) ;
#25961=EDGE_CURVE ( 'NONE', #59643, #50800, #78159, .T. ) ;
#25965=CARTESIAN_POINT ( 'NONE',  ( 147.9748066657072627, 274.3471119452502762, 9.387104374042873900 ) ) ;
#25966=CARTESIAN_POINT ( 'NONE',  ( 2.746756816977958593, 163.2048013555410080, 4.594050593750051981 ) ) ;
#25967=CARTESIAN_POINT ( 'NONE',  ( 49.83688814775681664, 190.3923013555410080, 4.594050593750050204 ) ) ;
#25969=CARTESIAN_POINT ( 'NONE',  ( 43.68655075043449898, 184.4824982072973967, 3.021315404115420679E-15 ) ) ;
#25972=CARTESIAN_POINT ( 'NONE',  ( 190.9380839614473473, 299.9325328093580652, -5.232187664503159752 ) ) ;
#25975=CARTESIAN_POINT ( 'NONE',  ( 67.98707691180798918, 203.3927522451418213, -10.00000000000009059 ) ) ;
#25976=CARTESIAN_POINT ( 'NONE',  ( 127.8330407560430757, 234.6115022471901739, -5.000000000000041744 ) ) ;
#25977=CARTESIAN_POINT ( 'NONE',  ( 163.1949325260522983, 256.0357984523876098, -14.93818428935952269 ) ) ;
#25978=CARTESIAN_POINT ( 'NONE',  ( 157.4211152037729562, 257.9856256133486454, -16.71526195140576831 ) ) ;
#25980=CARTESIAN_POINT ( 'NONE',  ( 40.72531889205828293, 180.9865022471901455, 1.119607411625061291E-15 ) ) ;
#25981=DIRECTION ( 'NONE',  ( 0.5000000000000048850, -0.8660254037844358210, 0.000000000000000000 ) ) ;
#25982=CARTESIAN_POINT ( 'NONE',  ( 163.1014434023538513, 248.1470085697407058, 9.692260209037655727 ) ) ;
#25983=CARTESIAN_POINT ( 'NONE',  ( 8.998290926605619688, 169.8768266524160140, 9.188101187500098632 ) ) ;
#25987=CARTESIAN_POINT ( 'NONE',  ( 152.6945189806187955, 266.1723304187151484, 16.62409282110771613 ) ) ;
#25989=CARTESIAN_POINT ( 'NONE',  ( 206.5318754762992910, 272.9232936229979032, 10.63244694018452741 ) ) ;
#25995=CARTESIAN_POINT ( 'NONE',  ( 168.8640704870188927, 288.0653526464637935, 0.5210052316872593181 ) ) ;
#25997=CARTESIAN_POINT ( 'NONE',  ( 160.5112507838001079, 252.6333537864655057, 16.06973146617909975 ) ) ;
#26000=CARTESIAN_POINT ( 'NONE',  ( 206.1615484827472358, 273.5647187912443314, -9.556459874778100883 ) ) ;
#26003=CARTESIAN_POINT ( 'NONE',  ( 152.9489295551198893, 265.7316783776963121, 17.71675637597311237 ) ) ;
#26004=CARTESIAN_POINT ( 'NONE',  ( 207.6826438088389750, 270.9301044032979462, 7.252082088659585146 ) ) ;
#26018=B_SPLINE_CURVE_WITH_KNOTS ( 'NONE', 3,
 ( #6699, #21891, #82258, #67995 ),
 .UNSPECIFIED., .F., .F.,
 ( 4, 4 ),
 ( 0.000000000000000000, 2.846293438401689159E-06 ),
 .UNSPECIFIED. ) ;
#26020=DIRECTION ( 'NONE',  ( 0.5000000000000048850, -0.8660254037844358210, 0.000000000000000000 ) ) ;
#26022=CARTESIAN_POINT ( 'NONE',  ( 173.7834928849634935, 267.2296750262562455, 17.04777296020808564 ) ) ;
#26023=CARTESIAN_POINT ( 'NONE',  ( 206.4537138826727301, 273.0586734743599209, 11.45643784582899016 ) ) ;
#26025=ORIENTED_EDGE ( 'NONE', *, *, #15196, .F. ) ;
#26026=CARTESIAN_POINT ( 'NONE',  ( 171.2743479101317234, 254.4242377521371736, -11.94796457435898951 ) ) ;
#26027=CARTESIAN_POINT ( 'NONE',  ( 163.3543347837650686, 247.7089878483399730, 10.92686688779373405 ) ) ;
#26029=EDGE_LOOP ( 'NONE', ( #10041, #83735, #90635, #29704 ) ) ;
#26030=CARTESIAN_POINT ( 'NONE',  ( 156.8155610647694687, 266.6398381445407040, -16.21946676759114325 ) ) ;
#26032=CARTESIAN_POINT ( 'NONE',  ( 160.3461653528465263, 270.4748347642712929, 15.77331661139888475 ) ) ;
#26034=CARTESIAN_POINT ( 'NONE',  ( 193.4053711441870576, 295.6590660519894982, 14.70124750960288118 ) ) ;
#26035=CARTESIAN_POINT ( 'NONE',  ( 177.4191073644459777, 288.9051419072185922, -9.334082586762583844 ) ) ;
#26036=FACE_OUTER_BOUND ( 'NONE', #45175, .T. ) ;
#26038=CARTESIAN_POINT ( 'NONE',  ( 192.0645969571214096, 297.9813550654635605, 11.46542907566974812 ) ) ;
#26039=CARTESIAN_POINT ( 'NONE',  ( 174.7547596240474377, 290.5425714371900199, 6.460816282008575939 ) ) ;
#26040=CARTESIAN_POINT ( 'NONE',  ( 158.5776461130937491, 255.9824553178812323, -17.58135378896025358 ) ) ;
#26044=CARTESIAN_POINT ( 'NONE',  ( 164.7462163020046262, 245.2981783406326599, 1.451255823150352064 ) ) ;
#26046=CARTESIAN_POINT ( 'NONE',  ( 159.7608930362198407, 253.9330115291272421, 15.38895778945778581 ) ) ;
#26048=CARTESIAN_POINT ( 'NONE',  ( 146.6797637568835171, 276.5901920613147809, -3.161329895305951876 ) ) ;
#26049=CARTESIAN_POINT ( 'NONE',  ( 171.6504431596714539, 259.4514037848667272, -15.21112824701198640 ) ) ;
#26050=CARTESIAN_POINT ( 'NONE',  ( 163.5642666985274332, 247.7300691424477179, 7.713274332594024507 ) ) ;
#26052=CARTESIAN_POINT ( 'NONE',  ( 199.3272761551183692, 285.4020256954596562, -18.33026947811089258 ) ) ;
#26053=CARTESIAN_POINT ( 'NONE',  ( 191.3546420016972434, 260.9821492784607244, -0.08077186525796756222 ) ) ;
#26054=ORIENTED_EDGE ( 'NONE', *, *, #18772, .F. ) ;
#26055=CARTESIAN_POINT ( 'NONE',  ( 152.1671311979278016, 269.0857928536317445, 15.36489295260887822 ) ) ;
#26056=CARTESIAN_POINT ( 'NONE',  ( 51.02741275436275004, 190.2677522451418213, -5.000000000000041744 ) ) ;
#26057=CARTESIAN_POINT ( 'NONE',  ( 207.0548180518391916, 272.0175305127218053, 7.721676452263806389 ) ) ;
#26058=CARTESIAN_POINT ( 'NONE',  ( 25.55183212637048840, 178.8927522451418497, 10.00000000000009592 ) ) ;
#26059=CARTESIAN_POINT ( 'NONE',  ( 99.30858933894288043, 218.9548013555409511, -4.594050593750042211 ) ) ;
#26062=CARTESIAN_POINT ( 'NONE',  ( 162.4702972292363086, 249.2401858085828508, 11.41296778546566060 ) ) ;
#26063=CARTESIAN_POINT ( 'NONE',  ( 27.18482440607884243, 180.3768266524160140, 9.188101187500098632 ) ) ;
#26064=CARTESIAN_POINT ( 'NONE',  ( 154.0986224399686648, 280.1916420498395155, 2.233781007141098396 ) ) ;
#26072=CARTESIAN_POINT ( 'NONE',  ( 207.6129110656513035, 271.0508850574501025, -5.265106572941297358 ) ) ;
#26073=CARTESIAN_POINT ( 'NONE',  ( 183.4649218511410425, 284.8064977680535890, 15.00784822088543358 ) ) ;
#26074=CARTESIAN_POINT ( 'NONE',  ( 167.2501155028055564, 251.6211038041439849, 10.31133882848387628 ) ) ;
#26075=CARTESIAN_POINT ( 'NONE',  ( 50.62146334811270521, 200.0333772461660544, 9.188101187500095079 ) ) ;
#26076=CARTESIAN_POINT ( 'NONE',  ( 84.80240350195585108, 209.7677522451417929, -5.000000000000041744 ) ) ;
#26077=ORIENTED_EDGE ( 'NONE', *, *, #48776, .T. ) ;
#26079=EDGE_CURVE ( 'NONE', #38189, #62928, #14101, .T. ) ;
#26080=B_SPLINE_CURVE_WITH_KNOTS ( 'NONE', 3,
 ( #61778, #16688, #39963, #1506, #32388, #63285 ),
 .UNSPECIFIED., .F., .F.,
 ( 4, 2, 4 ),
 ( 0.02097825722499890508, 0.02555397795540580511, 0.03012969868581270513 ),
 .UNSPECIFIED. ) ;
#26081=CARTESIAN_POINT ( 'NONE',  ( 178.7905889683881355, 259.2243177618232721, -10.28886766292962207 ) ) ;
#26082=CARTESIAN_POINT ( 'NONE',  ( -1.610867365518755978, 176.0024278399160949, 9.188101187500095079 ) ) ;
#26084=CARTESIAN_POINT ( 'NONE',  ( 198.8570476668614049, 286.2164853282868080, -17.01721544293231858 ) ) ;
#26085=DIRECTION ( 'NONE',  ( -0.8660254037844387076, -0.4999999999999998890, -0.000000000000000000 ) ) ;
#26086=CARTESIAN_POINT ( 'NONE',  ( 147.0314375879888757, 275.9810751181479986, -5.168577011192616588 ) ) ;
#26087=CARTESIAN_POINT ( 'NONE',  ( 175.1183745746886871, 267.9007702990796247, 17.47926410801357022 ) ) ;
#26088=CARTESIAN_POINT ( 'NONE',  ( 204.4781092559247782, 276.4805210635553863, 13.30606382016679490 ) ) ;
#26089=CARTESIAN_POINT ( 'NONE',  ( 147.1731211915891322, 275.7356719181125868, 0.5879280619134324981 ) ) ;
#26090=CARTESIAN_POINT ( 'NONE',  ( 164.7694554770609159, 245.2579269087094076, -3.003635650077957742 ) ) ;
#26093=CARTESIAN_POINT ( 'NONE',  ( 208.0045976720423084, 270.3724639545367836, 2.002128742561712471 ) ) ;
#26094=CARTESIAN_POINT ( 'NONE',  ( -3.297639133650707599, 162.2365022471902023, -10.00000000000009059 ) ) ;
#26095=CARTESIAN_POINT ( 'NONE',  ( 181.2928807913240234, 267.9761254251728815, 15.08543189990537137 ) ) ;
#26096=CARTESIAN_POINT ( 'NONE',  ( 127.4269177983626236, 250.5024278399160949, -9.188101187500093303 ) ) ;
#26099=CARTESIAN_POINT ( 'NONE',  ( 34.98558885611105751, 202.5530062829863027, -4.648177544792955347E-16 ) ) ;
#26102=CARTESIAN_POINT ( 'NONE',  ( 150.2943746394907691, 270.3295023630476521, -14.89639308767058701 ) ) ;
#26103=EDGE_LOOP ( 'NONE', ( #90447, #96731, #4306, #43665 ) ) ;
#26104=CARTESIAN_POINT ( 'NONE',  ( 158.2129804214947058, 265.2348010298870236, 17.61986633405762603 ) ) ;
#26105=CARTESIAN_POINT ( 'NONE',  ( 149.4908848037268001, 271.7211875819559737, -12.92288068979413573 ) ) ;
#26107=CARTESIAN_POINT ( 'NONE',  ( 175.4875483129441136, 292.5133918439943272, -1.145445019159226696 ) ) ;
#26109=ORIENTED_EDGE ( 'NONE', *, *, #85468, .T. ) ;
#26110=CARTESIAN_POINT ( 'NONE',  ( 189.0909386108920103, 265.6590948244866581, 10.80641681947311028 ) ) ;
#26111=CARTESIAN_POINT ( 'NONE',  ( 184.3226795282388650, 274.5458599865910969, 17.66928848808302988 ) ) ;
#26112=CARTESIAN_POINT ( 'NONE',  ( 168.1566130751629942, 271.3748772526728885, -16.49521172744375974 ) ) ;
#26113=CARTESIAN_POINT ( 'NONE',  ( 198.6815419560737155, 272.0295385808636297, 12.20295816876821426 ) ) ;
#26114=B_SPLINE_CURVE_WITH_KNOTS ( 'NONE', 3,
 ( #96980, #41215, #27549, #4744 ),
 .UNSPECIFIED., .F., .F.,
 ( 4, 4 ),
 ( 0.01048982011972383714, 0.01573329961111291642 ),
 .UNSPECIFIED. ) ;
#26115=CARTESIAN_POINT ( 'NONE',  ( 155.5855974046909296, 261.5528867068662180, 16.99664480632919705 ) ) ;
#26117=CARTESIAN_POINT ( 'NONE',  ( 192.4454213697443095, 297.3217478340386606, 12.58566886711101596 ) ) ;
#26119=CARTESIAN_POINT ( 'NONE',  ( 199.5332225370696904, 272.7339375561579686, -13.62198628356192565 ) ) ;
#26123=CARTESIAN_POINT ( 'NONE',  ( 167.6260565400901044, 280.9425530968866269, 11.66579211281432116 ) ) ;
#26124=CARTESIAN_POINT ( 'NONE',  ( 148.4083960970861256, 273.5961130204771052, -8.574185186226726429 ) ) ;
#26125=CARTESIAN_POINT ( 'NONE',  ( 109.4119587261635758, 240.6427522451419065, -10.00000000000009592 ) ) ;
#26129=B_SPLINE_CURVE_WITH_KNOTS ( 'NONE', 3,
 ( #43010, #73948, #18754, #80590, #4534, #97270, #20249, #35434, #66337, #11167, #27837, #58714, #51124, #12658, #3561, #33444, #95304, #34441, #65340, #67838, #53615, #35926, #5536, #36420, #67328, #75964, #45515, #13642, #83071, #15109, #44515, #75446, #98758, #14134, #91663, #74466, #76446, #5046, #51641, #6030, #98252, #66828, #28326, #82590, #28841, #37414, #21244, #29830, #68320, #83573, #84571, #59203 ),
 .UNSPECIFIED., .F., .F.,
 ( 4, 2, 2, 2, 2, 2, 2, 2, 2, 2, 2, 2, 2, 2, 2, 2, 2, 2, 2, 2, 2, 2, 2, 2, 2, 4 ),
 ( 0.0006591152314301792136, 0.0008712174001076930475, 0.001083319568785206990, 0.001189370653124002721, 0.001295421737462798453, 0.001401472821801594184, 0.001507523906140389915, 0.001719626074817925867, 0.001931728243495461819, 0.002355932580850601376, 0.003204341255560809801, 0.004052749930271017792, 0.004901158604981225783, 0.005325362942336289013, 0.005537465111013899557, 0.005643516195352659727, 0.005696541737522091420, 0.005749567279691522245, 0.005855618364030549562, 0.005961669448369576879, 0.006173771617047633248, 0.006597975954403787618, 0.006810078123081869141, 0.007022180291759949795, 0.007234282460438032185, 0.007446384629116113707 ),
 .UNSPECIFIED. ) ;
#26133=CARTESIAN_POINT ( 'NONE',  ( 187.0522961678524609, 271.2721401460262882, 16.58916046916640141 ) ) ;
#26134=CARTESIAN_POINT ( 'NONE',  ( 155.6066474290145720, 261.1283759879266881, -18.16552045242181279 ) ) ;
#26135=ORIENTED_EDGE ( 'NONE', *, *, #1124, .T. ) ;
#26137=CARTESIAN_POINT ( 'NONE',  ( 178.5732266955483567, 260.7996415306764106, 12.02568443977059331 ) ) ;
#26140=ORIENTED_EDGE ( 'NONE', *, *, #55697, .T. ) ;
#26141=EDGE_CURVE ( 'NONE', #54626, #90614, #69982, .T. ) ;
#26143=CARTESIAN_POINT ( 'NONE',  ( 155.5587153255869453, 261.2113968263770971, -18.30500480654006878 ) ) ;
#26144=ORIENTED_EDGE ( 'NONE', *, *, #43687, .T. ) ;
#26147=CARTESIAN_POINT ( 'NONE',  ( 158.8643209822442373, 275.1626068170347708, -12.53457103330068101 ) ) ;
#26148=CARTESIAN_POINT ( 'NONE',  ( 146.7842303614460207, 276.4092505945183689, -4.491116827832889236 ) ) ;
#26149=CARTESIAN_POINT ( 'NONE',  ( 201.2949053258274148, 281.9939920013367782, -18.04004790210578335 ) ) ;
#26150=EDGE_CURVE ( 'NONE', #46531, #97695, #91464, .T. ) ;
#26152=CARTESIAN_POINT ( 'NONE',  ( 183.3634088509504352, 284.6525016221286251, -16.42631288611494256 ) ) ;
#26153=CARTESIAN_POINT ( 'NONE',  ( 137.4944631173567018, 256.3149278399160380, -9.188101187500095079 ) ) ;
#26157=B_SPLINE_CURVE_WITH_KNOTS ( 'NONE', 3,
 ( #66808, #13134, #97737, #20732, #43992, #59702, #60683, #13624, #53106, #91642, #75943, #45982, #51617, #90159, #91147, #28817, #30311, #84062, #37396, #82572, #6519, #76429, #59183, #14617, #98740, #74934, #21712, #53595 ),
 .UNSPECIFIED., .F., .F.,
 ( 4, 2, 2, 2, 2, 2, 2, 2, 2, 2, 2, 2, 2, 4 ),
 ( 0.0004814462238576242893, 0.001666870227462020123, 0.002852294231066416011, 0.003445006232868651035, 0.003741362233769804542, 0.003778406733882429865, 0.003815451233995055189, 0.003852495734107680512, 0.003889540234220305401, 0.004037718234670611105, 0.004334074235571087202, 0.004630430236471567637, 0.004926786237372048072, 0.005223142238272528506 ),
 .UNSPECIFIED. ) ;
#26161=CARTESIAN_POINT ( 'NONE',  ( 202.6560281492536717, 279.6364581158209717, 17.15553667345918853 ) ) ;
#26163=CARTESIAN_POINT ( 'NONE',  ( 192.4464452833618964, 297.3199743636303083, 12.61460102250842574 ) ) ;
#26164=CARTESIAN_POINT ( 'NONE',  ( 153.3196571941631419, 276.9012595390603906, 7.065720231617055092 ) ) ;
#26165=CARTESIAN_POINT ( 'NONE',  ( 153.0308080659177392, 265.5898606369461277, -17.74682723936668438 ) ) ;
#26167=CARTESIAN_POINT ( 'NONE',  ( 171.5764408558917182, 280.0072332633130259, 13.86250607708617899 ) ) ;
#26175=CARTESIAN_POINT ( 'NONE',  ( 164.0359846223783791, 278.2138621274489765, 13.39833324297733164 ) ) ;
#26176=CARTESIAN_POINT ( 'NONE',  ( 200.9789653343762268, 267.8171911071562477, -2.834779958744446660 ) ) ;
#26177=CARTESIAN_POINT ( 'NONE',  ( 191.4160719247997804, 299.1046333714251659, -10.38740866002593677 ) ) ;
#26179=CARTESIAN_POINT ( 'NONE',  ( 202.3421728196210552, 280.1800714929709670, 16.85915999540957344 ) ) ;
#26181=CARTESIAN_POINT ( 'NONE',  ( 151.4541170308968674, 274.9972311722506220, -9.452079333234340908 ) ) ;
#26182=CARTESIAN_POINT ( 'NONE',  ( 60.04851071045058575, 212.1427522451419065, -10.00000000000009592 ) ) ;
#26183=VERTEX_POINT ( 'NONE', #64809 ) ;
#26186=CARTESIAN_POINT ( 'NONE',  ( 193.4352373529416411, 275.9703139695285472, -16.71496292338552792 ) ) ;
#26189=FACE_OUTER_BOUND ( 'NONE', #84027, .T. ) ;
#26192=CARTESIAN_POINT ( 'NONE',  ( -4.208943576872074210, 174.5024278399160949, 9.188101187500095079 ) ) ;
#26193=CARTESIAN_POINT ( 'NONE',  ( 95.92524373570365981, 232.3149278399160949, -9.188101187500095079 ) ) ;
#26194=CARTESIAN_POINT ( 'NONE',  ( 203.0498946958275326, 278.9542612457532869, -15.11479947333269003 ) ) ;
#26196=CARTESIAN_POINT ( 'NONE',  ( 147.7445507185682629, 275.1340851767408822, 4.244012899323919896 ) ) ;
#26197=CARTESIAN_POINT ( 'NONE',  ( 176.2580550267919932, 278.7780497695933946, -16.99066290002705060 ) ) ;
#26200=CARTESIAN_POINT ( 'NONE',  ( 160.5467508819430691, 282.2240450670404357, 5.086209391429217241 ) ) ;
#26201=CARTESIAN_POINT ( 'NONE',  ( 190.4356836585210431, 300.3996184492839916, -0.5836641476860114919 ) ) ;
#26202=B_SPLINE_CURVE_WITH_KNOTS ( 'NONE', 3,
 ( #15559, #71298, #24182, #55064 ),
 .UNSPECIFIED., .F., .F.,
 ( 4, 4 ),
 ( 0.01367696721474719219, 0.01995365678480425300 ),
 .UNSPECIFIED. ) ;
#26203=CARTESIAN_POINT ( 'NONE',  ( 208.3790849386676598, 269.7238329819538762, -1.525282248498321946 ) ) ;
#26205=CARTESIAN_POINT ( 'NONE',  ( 178.1725702544899264, 289.8985928146129254, 9.568895312856861679 ) ) ;
#26207=CARTESIAN_POINT ( 'NONE',  ( 7.313483791488072150, 163.4824982072973683, 3.021315404115420679E-15 ) ) ;
#26211=CARTESIAN_POINT ( 'NONE',  ( 50.89226983467786170, 194.0643266524160424, 9.188101187500095079 ) ) ;
#26213=CARTESIAN_POINT ( 'NONE',  ( 83.25962220535622293, 225.0024278399160664, -9.188101187500093303 ) ) ;
#26214=CARTESIAN_POINT ( 'NONE',  ( 207.1285138014047504, 271.8898857301724661, -5.752177443817618752 ) ) ;
#26216=CARTESIAN_POINT ( 'NONE',  ( 163.3339561395536350, 258.0835846320132418, 15.71813896107145148 ) ) ;
#26219=CARTESIAN_POINT ( 'NONE',  ( 174.4104451852509214, 268.9371725773738149, -16.32578690765196328 ) ) ;
#26223=VERTEX_POINT ( 'NONE', #58674 ) ;
#26225=CARTESIAN_POINT ( 'NONE',  ( 70.32319418844367931, 223.6589784336661637, -6.496448406907676862E-16 ) ) ;
#26227=FACE_OUTER_BOUND ( 'NONE', #32224, .T. ) ;
#26228=CARTESIAN_POINT ( 'NONE',  ( 192.6679047218190135, 296.9363953644068488, -13.34486378385621386 ) ) ;
#26231=( BOUNDED_CURVE ( )  B_SPLINE_CURVE ( 2, ( #16150, #24745, #62734, #31345, #30352, #8062, #22757, #9055, #62228 ),
 .UNSPECIFIED., .F., .T. ) 
 B_SPLINE_CURVE_WITH_KNOTS ( ( 3, 2, 2, 2, 3 ),
 ( 0.03629032258064516375, 0.03763440860215053890, 0.04032258064516128920, 0.04301075268817204644, 0.04435483870967742159 ),
 .UNSPECIFIED. ) 
 CURVE ( )  GEOMETRIC_REPRESENTATION_ITEM ( )  RATIONAL_B_SPLINE_CURVE ( ( 0.9330127018922194093, 0.9330127018922195203, 1.000000000000000000, 0.8660254037844387076, 1.000000000000000000, 0.8660254037844387076, 1.000000000000000000, 0.9330127018922194093, 0.9330127018922194093 ) ) 
 REPRESENTATION_ITEM ( '' )  );
#26236=CARTESIAN_POINT ( 'NONE',  ( 135.6272693901030379, 239.1115022471902023, -5.000000000000041744 ) ) ;
#26237=CARTESIAN_POINT ( 'NONE',  ( 157.4805323096970255, 257.8827121670497036, -16.70238855805511591 ) ) ;
#26242=CARTESIAN_POINT ( 'NONE',  ( 202.5511585997265911, 279.8180975037686835, 17.12781264818056925 ) ) ;
#26243=CARTESIAN_POINT ( 'NONE',  ( 207.3023081270791295, 270.3638296917698085, -0.1999334432952042662 ) ) ;
#26248=CARTESIAN_POINT ( 'NONE',  ( 192.8660768639943797, 292.4946550107171674, 15.23525216266379090 ) ) ;
#26249=CARTESIAN_POINT ( 'NONE',  ( 171.2207522194980811, 249.4850955738359630, 2.852778252398243453 ) ) ;
#26251=CARTESIAN_POINT ( 'NONE',  ( 192.9359148231858967, 296.1054784705493717, -12.00501928171166455 ) ) ;
#26253=EDGE_CURVE ( 'NONE', #92597, #80984, #21475, .T. ) ;
#26256=ADVANCED_FACE ( 'NONE', ( #42965 ), #19719, .T. ) ;
#26257=CARTESIAN_POINT ( 'NONE',  ( 166.7959447105422157, 276.3626885415273478, 15.91653206054683523 ) ) ;
#26258=CARTESIAN_POINT ( 'NONE',  ( -22.42236680055709641, 157.8615022471902591, 0.000000000000000000 ) ) ;
#26261=CARTESIAN_POINT ( 'NONE',  ( 188.4805308512120234, 298.0761574053781828, 7.892637567094712203 ) ) ;
#26262=CARTESIAN_POINT ( 'NONE',  ( 163.9149533033796047, 246.7379680887036670, 7.273005089308705706 ) ) ;
#26263=CARTESIAN_POINT ( 'NONE',  ( 147.8308140999695866, 274.5965143850199865, -7.866624397492971710 ) ) ;
#26265=CARTESIAN_POINT ( 'NONE',  ( 194.3252252352508265, 294.0658320307167628, 14.07225870721148731 ) ) ;
#26266=CARTESIAN_POINT ( 'NONE',  ( 147.4869352381265628, 275.6365489870674423, 0.2695896373555386472 ) ) ;
#26268=CARTESIAN_POINT ( 'NONE',  ( 164.6152412757387538, 245.5250337406482117, 4.392968637767231677 ) ) ;
#26270=CARTESIAN_POINT ( 'NONE',  ( 166.1117962628217697, 265.5293696438469624, 16.57715453726662247 ) ) ;
#26272=CARTESIAN_POINT ( 'NONE',  ( 87.42789010471635436, 209.0327760586659451, 1.948934522072303157E-15 ) ) ;
#26273=ORIENTED_EDGE ( 'NONE', *, *, #28633, .F. ) ;
#26276=AXIS2_PLACEMENT_3D ( 'NONE', #19186, #41954, #35850 ) ;
#26277=ORIENTED_EDGE ( 'NONE', *, *, #59885, .T. ) ;
#26280=ADVANCED_FACE ( 'NONE', ( #74912 ), #74424, .T. ) ;
#26281=CARTESIAN_POINT ( 'NONE',  ( 178.4456047009153110, 292.8474234380366852, -2.655382915061203608 ) ) ;
#26282=B_SPLINE_SURFACE_WITH_KNOTS ( 'NONE', 3, 1, ( 
 ( #72436, #96247 ),
 ( #49111, #50592 ),
 ( #10112, #33407 ),
 ( #44361, #75294 ),
 ( #87684, #10615 ),
 ( #4005, #34891 ),
 ( #79557, #65790 ),
 ( #36761, #3040 ),
 ( #26808, #25827 ),
 ( #64307, #18219 ),
 ( #33931, #57692 ),
 ( #64815, #14475 ),
 ( #39233, #30162 ),
 ( #45356, #38238 ),
 ( #22064, #68656 ),
 ( #31638, #76288 ),
 ( #23041, #52962 ),
 ( #84897, #83406 ),
 ( #29668, #69652 ),
 ( #261, #60545 ),
 ( #21577, #53937 ),
 ( #92986, #37261 ),
 ( #13977, #22565 ),
 ( #75792, #83912 ),
 ( #6860, #91501 ),
 ( #61044, #38748 ),
 ( #68160, #37749 ),
 ( #70141, #99578 ),
 ( #6378, #31142 ),
 ( #45836, #92019 ),
 ( #753, #53451 ),
 ( #99086, #69153 ),
 ( #76759, #84402 ),
 ( #15954, #14946 ) ),
 .UNSPECIFIED., .T., .F., .F.,
 ( 4, 2, 2, 2, 2, 2, 2, 2, 2, 2, 2, 2, 2, 2, 2, 2, 4 ),
 ( 2, 2 ),
 ( 0.000000000000000000, 0.06250000000000000000, 0.1250000000000000000, 0.1875000000000000000, 0.2500000000000000000, 0.3125000000000000000, 0.3750000000000000000, 0.4375000000000000000, 0.5000000000000000000, 0.5625000000000000000, 0.6250000000000000000, 0.6875000000000000000, 0.7500000000000000000, 0.8125000000000000000, 0.8750000000000000000, 0.9375000000000000000, 1.000000000000000000 ),
 ( 0.000000000000000000, 1.000000000000000000 ),
 .UNSPECIFIED. ) ;
#26283=CARTESIAN_POINT ( 'NONE',  ( 164.0981304475902789, 249.9383316284954333, 10.21525845096581264 ) ) ;
#26284=CARTESIAN_POINT ( 'NONE',  ( 159.2289198208967775, 254.8544161663325838, -15.88961297684315888 ) ) ;
#26285=CARTESIAN_POINT ( 'NONE',  ( 163.2124973040920111, 247.9546575695509887, 10.85238219581215269 ) ) ;
#26286=EDGE_CURVE ( 'NONE', #26637, #65011, #1372, .T. ) ;
#26287=CARTESIAN_POINT ( 'NONE',  ( 86.72372382049398709, 227.0024278399160949, 9.188101187500095079 ) ) ;
#26290=CARTESIAN_POINT ( 'NONE',  ( 161.4688978523910805, 250.9746604079464589, -14.18458049884803529 ) ) ;
#26291=ORIENTED_EDGE ( 'NONE', *, *, #51526, .F. ) ;
#26292=AXIS2_PLACEMENT_3D ( 'NONE', #16429, #47325, #15927 ) ;
#26294=DIRECTION ( 'NONE',  ( 0.4999999999999992784, -0.8660254037844390407, 0.000000000000000000 ) ) ;
#26295=CARTESIAN_POINT ( 'NONE',  ( 126.4254891512956220, 252.9869531367911009, 4.594050593750046652 ) ) ;
#26296=CARTESIAN_POINT ( 'NONE',  ( 188.6237917963981090, 260.2852467542186901, 5.911286565928174142 ) ) ;
#26297=CARTESIAN_POINT ( 'NONE',  ( 73.72680694775513643, 201.8262482093457777, 3.021315404115420679E-15 ) ) ;
#26299=ORIENTED_EDGE ( 'NONE', *, *, #84190, .F. ) ;
#26301=CARTESIAN_POINT ( 'NONE',  ( 160.5298764916272773, 275.8772147286272229, 14.16040495044419245 ) ) ;
#26302=EDGE_CURVE ( 'NONE', #45557, #24115, #81054, .T. ) ;
#26307=DIRECTION ( 'NONE',  ( -0.8660254037844387076, -0.4999999999999998890, -0.000000000000000000 ) ) ;
#26310=CARTESIAN_POINT ( 'NONE',  ( 161.4844649541891499, 250.9476973967054789, 12.93553496455142415 ) ) ;
#26314=CARTESIAN_POINT ( 'NONE',  ( 175.5461044416861114, 291.1942812272370702, -6.598926784758673669 ) ) ;
#26315=CARTESIAN_POINT ( 'NONE',  ( 200.9070263471402029, 275.2638490881122948, 14.76484851748618787 ) ) ;
#26316=EDGE_CURVE ( 'NONE', #21055, #87863, #60204, .T. ) ;
#26319=CARTESIAN_POINT ( 'NONE',  ( 207.6860335175200589, 270.9242332556395922, 6.913225035677485586 ) ) ;
#26320=CARTESIAN_POINT ( 'NONE',  ( 180.6399068022690813, 266.9789143157389617, -16.10679502715467848 ) ) ;
#26325=CARTESIAN_POINT ( 'NONE',  ( 152.9489295551198893, 265.7316783776963121, 17.71675637597311237 ) ) ;
#26326=CARTESIAN_POINT ( 'NONE',  ( 180.6524066389949326, 273.0753924814325160, 17.36873516045730170 ) ) ;
#26327=CARTESIAN_POINT ( 'NONE',  ( 160.6761024546964336, 273.3315593702743058, -15.58338923054105329 ) ) ;
#26329=CARTESIAN_POINT ( 'NONE',  ( 13.89683389070260944, 169.6423013555409796, -4.594050593750043987 ) ) ;
#26331=EDGE_LOOP ( 'NONE', ( #79882, #43733, #30131, #93736 ) ) ;
#26335=CARTESIAN_POINT ( 'NONE',  ( 42.15091268916992817, 185.9548013555409796, -4.594050593750042211 ) ) ;
#26339=CARTESIAN_POINT ( 'NONE',  ( 190.9380839614473473, 299.9325328093580652, -5.232187664503159752 ) ) ;
#26341=CARTESIAN_POINT ( 'NONE',  ( 178.8696907613845610, 291.8157686920125684, 6.076668511113703097 ) ) ;
#26342=CARTESIAN_POINT ( 'NONE',  ( 191.7187529716733820, 298.5803744197520473, -8.487597704798396592 ) ) ;
#26343=CARTESIAN_POINT ( 'NONE',  ( 197.0834897501566729, 289.2883777501857594, 16.96463043134541238 ) ) ;
#26344=CARTESIAN_POINT ( 'NONE',  ( 182.5718888600741820, 280.2395840502504143, -16.09643023696035513 ) ) ;
#26346=CARTESIAN_POINT ( 'NONE',  ( 166.4967320654721732, 257.8000681324233483, -15.13017568244432098 ) ) ;
#26348=CARTESIAN_POINT ( 'NONE',  ( 83.09635312912047311, 230.3297689869269220, -2.679491924311252493 ) ) ;
#26349=CARTESIAN_POINT ( 'NONE',  ( 76.30452923086889427, 224.8615022471903160, 5.000000000000046185 ) ) ;
#26352=CARTESIAN_POINT ( 'NONE',  ( 44.74898890052324418, 187.4548013555409796, -4.594050593750042211 ) ) ;
#26356=CARTESIAN_POINT ( 'NONE',  ( 198.5970767652345899, 286.6667681383942181, -17.17073100918929640 ) ) ;
#26357=CARTESIAN_POINT ( 'NONE',  ( 58.13834967963523326, 192.8262482093458061, 3.021315404115420679E-15 ) ) ;
#26361=CARTESIAN_POINT ( 'NONE',  ( 164.3138894970802824, 246.0469903322357368, -2.642126690130961020 ) ) ;
#26362=CARTESIAN_POINT ( 'NONE',  ( 147.1824143116938046, 275.7195757619304572, 6.276289813856542388 ) ) ;
#26366=CARTESIAN_POINT ( 'NONE',  ( 196.2379679265050925, 290.7528645076583871, -16.93678934971137906 ) ) ;
#26367=CARTESIAN_POINT ( 'NONE',  ( 172.2121928603940262, 256.1155326756577892, 11.22455358908347378 ) ) ;
#26370=CARTESIAN_POINT ( 'NONE',  ( 17.34263298987836066, 187.4865022471903444, -10.00000000000009592 ) ) ;
#26372=ORIENTED_EDGE ( 'NONE', *, *, #31070, .T. ) ;
#26374=CARTESIAN_POINT ( 'NONE',  ( 166.9004453850575374, 261.3797933789293779, 16.71428553088463431 ) ) ;
#26375=CARTESIAN_POINT ( 'NONE',  ( 177.7795532957129581, 255.1900280424794687, -6.882059445467048953 ) ) ;
#26376=CARTESIAN_POINT ( 'NONE',  ( 201.1403430031335517, 280.2617017971787732, 16.85780947333721613 ) ) ;
#26377=ORIENTED_EDGE ( 'NONE', *, *, #97112, .F. ) ;
#26379=CARTESIAN_POINT ( 'NONE',  ( 207.8984236726843164, 270.5563627158673512, -6.084369154771423815 ) ) ;
#26381=CARTESIAN_POINT ( 'NONE',  ( 196.4170778717353585, 290.4426369823788718, -17.78762421190030452 ) ) ;
#26382=ORIENTED_EDGE ( 'NONE', *, *, #21160, .T. ) ;
#26383=CARTESIAN_POINT ( 'NONE',  ( 201.0468719883840265, 282.4235983437597497, -16.59631526626950659 ) ) ;
#26384=CARTESIAN_POINT ( 'NONE',  ( 198.3449891235413531, 287.1033967417670283, 16.95540786497457120 ) ) ;
#26387=CARTESIAN_POINT ( 'NONE',  ( 157.8820657059571033, 257.1872359237914338, -17.60412210594719440 ) ) ;
#26388=CARTESIAN_POINT ( 'NONE',  ( 124.1257165900819359, 230.2202760586659736, -5.415160957724236172E-17 ) ) ;
#26391=CARTESIAN_POINT ( 'NONE',  ( 187.4166251561426293, 263.4339899954952102, 11.64397722261905166 ) ) ;
#26393=CARTESIAN_POINT ( 'NONE',  ( 207.6471633721571379, 270.9915583223058206, 2.196965492132801678 ) ) ;
#26395=B_SPLINE_CURVE_WITH_KNOTS ( 'NONE', 3,
 ( #16328, #54304, #39103, #15819, #47222, #78144, #16823, #8730, #39602, #24432, #92371, #53806, #1138, #47710, #9231, #24924, #32537, #94369, #63431, #55798, #1652, #86035, #9477, #78384, #85520, #63665, #94108, #78891, #24168, #1877, #55544, #39341, #40841, #77377, #71285, #92605, #8470, #30775, #38855, #40348, #70765, #32759 ),
 .UNSPECIFIED., .F., .F.,
 ( 4, 2, 2, 2, 2, 2, 2, 2, 2, 2, 2, 2, 2, 2, 2, 2, 2, 2, 2, 2, 4 ),
 ( 0.002222259514562908208, 0.002656659727101862243, 0.002873859833371299362, 0.003091059939640736914, 0.003199659992775469568, 0.003308260045910201789, 0.003525460152179574723, 0.003959860364718250335, 0.004828660789795527833, 0.005697461214872804464, 0.006566261639950082829, 0.007000661852488722012, 0.007435062065027361194, 0.007543662118161998872, 0.007597962144729316844, 0.007652262171296634816, 0.007760862224431298514, 0.007869462277565960479, 0.008303862490104212818, 0.008738262702642463423, 0.009172662915180715762 ),
 .UNSPECIFIED. ) ;
#26397=CARTESIAN_POINT ( 'NONE',  ( 198.4772197948566372, 286.8743665007300478, 18.43646439804394532 ) ) ;
#26399=CARTESIAN_POINT ( 'NONE',  ( 66.99449581658849695, 218.6744531367911293, 4.594050593750047540 ) ) ;
#26402=CARTESIAN_POINT ( 'NONE',  ( 190.8604783348975502, 300.0669496974951471, 7.597731640149610222 ) ) ;
#26404=CARTESIAN_POINT ( 'NONE',  ( 175.9016958582107293, 272.8421865953737324, 16.70581961971107887 ) ) ;
#26405=EDGE_CURVE ( 'NONE', #53525, #82029, #1961, .T. ) ;
#26410=CARTESIAN_POINT ( 'NONE',  ( 153.1965564441067045, 269.1488324487709178, -15.62636021046843382 ) ) ;
#26411=CARTESIAN_POINT ( 'NONE',  ( 173.8411061959160691, 278.0589164288677466, -16.53377806444067488 ) ) ;
#26412=CARTESIAN_POINT ( 'NONE',  ( 160.4278600671212303, 258.1933913629677591, -16.98986990419299659 ) ) ;
#26413=CARTESIAN_POINT ( 'NONE',  ( 70.22199747613832699, 222.8967562850346837, -4.648177544792955347E-16 ) ) ;
#26414=CARTESIAN_POINT ( 'NONE',  ( 190.6661865267473104, 300.4034729807058852, 4.523489664447863490 ) ) ;
#26416=CARTESIAN_POINT ( 'NONE',  ( 180.1766175091199216, 271.0712247103771801, 16.39758672572147091 ) ) ;
#26419=CARTESIAN_POINT ( 'NONE',  ( 164.2981700896163773, 253.9203781951923133, 14.63367134977796802 ) ) ;
#26421=CARTESIAN_POINT ( 'NONE',  ( 164.0179800784044915, 246.5595204798204065, -5.772998092557310557 ) ) ;
#26422=CARTESIAN_POINT ( 'NONE',  ( 125.1810982770029881, 233.8923013555409796, 4.594050593750050204 ) ) ;
#26424=CARTESIAN_POINT ( 'NONE',  ( 191.1687199697037443, 299.5330595250031820, -8.491751560014430211 ) ) ;
#26430=CARTESIAN_POINT ( 'NONE',  ( 176.7263968240380621, 254.5787242937214785, 4.904709157180852763 ) ) ;
#26435=CARTESIAN_POINT ( 'NONE',  ( 157.9903129722402753, 275.9952189379433776, -12.65964543032067091 ) ) ;
#26436=CARTESIAN_POINT ( 'NONE',  ( 182.0600995000775413, 260.3591856445613644, 10.51176232977279312 ) ) ;
#26437=CARTESIAN_POINT ( 'NONE',  ( 165.0477436618537865, 244.7759176335020186, -2.027991469056170448 ) ) ;
#26438=CARTESIAN_POINT ( 'NONE',  ( 141.2293712190596011, 252.3458772461660260, 9.188101187500095079 ) ) ;
#26444=CARTESIAN_POINT ( 'NONE',  ( 74.43750904794977430, 201.5327760586659167, 1.948934522072303157E-15 ) ) ;
#26445=CARTESIAN_POINT ( 'NONE',  ( 205.3465787480556344, 274.9762877783610406, -13.79319041940166279 ) ) ;
#26446=CARTESIAN_POINT ( 'NONE',  ( 174.6847557482075217, 251.9401552947160781, 3.562689555296894017 ) ) ;
#26449=CARTESIAN_POINT ( 'NONE',  ( 149.7128599965862463, 271.3367152699035501, 12.33532264622322394 ) ) ;
#26450=CARTESIAN_POINT ( 'NONE',  ( 155.3976843646185273, 279.6809108413763738, -1.548285546709123883 ) ) ;
#26451=CARTESIAN_POINT ( 'NONE',  ( 172.0998544454759838, 287.8757577825812177, -8.507407346436933082 ) ) ;
#26452=DIRECTION ( 'NONE',  ( -0.8660254037844387076, -0.4999999999999998890, -0.000000000000000000 ) ) ;
#26453=CARTESIAN_POINT ( 'NONE',  ( 193.6168471018168589, 288.5492936057587485, 16.06529688929707689 ) ) ;
#26454=CARTESIAN_POINT ( 'NONE',  ( 121.1754704609022752, 230.7677522451417929, -5.000000000000041744 ) ) ;
#26457=CARTESIAN_POINT ( 'NONE',  ( 157.8740713127050981, 257.2010826190796706, 17.31862062017425075 ) ) ;
#26458=CARTESIAN_POINT ( 'NONE',  ( 160.2313082275607599, 258.0676731373150687, -17.23155629354643281 ) ) ;
#26459=CARTESIAN_POINT ( 'NONE',  ( -10.21716836350912949, 177.1589784336661637, -6.496448406907676862E-16 ) ) ;
#26460=CARTESIAN_POINT ( 'NONE',  ( 29.07873433320978052, 199.8464784336661353, 1.353441290958777327E-15 ) ) ;
#26461=CARTESIAN_POINT ( 'NONE',  ( 175.5402865323166282, 256.4720531653651960, -10.93513971934378759 ) ) ;
#26463=CARTESIAN_POINT ( 'NONE',  ( -22.42236680055709641, 157.8615022471902591, 0.000000000000000000 ) ) ;
#26464=CARTESIAN_POINT ( 'NONE',  ( 204.7237927799493775, 276.0549847173622879, -12.81020997223575364 ) ) ;
#26465=CARTESIAN_POINT ( 'NONE',  ( 190.6163636546212103, 291.2123861011319832, -14.36794556205205176 ) ) ;
#26466=CARTESIAN_POINT ( 'NONE',  ( 190.8545714895799392, 300.0771806536980648, -5.516553996882049837 ) ) ;
#26468=CARTESIAN_POINT ( 'NONE',  ( 167.5861325596884797, 256.5095974891418109, 15.03189046419509367 ) ) ;
#26469=CARTESIAN_POINT ( 'NONE',  ( 66.18285732059042914, 199.0177522451417929, 5.000000000000051514 ) ) ;
#26471=CARTESIAN_POINT ( 'NONE',  ( 204.8385597977314490, 275.8562024115307167, -12.64672659107585240 ) ) ;
#26472=CARTESIAN_POINT ( 'NONE',  ( 162.1309243477163875, 252.0648751526918261, -13.42546355478092401 ) ) ;
#26474=CARTESIAN_POINT ( 'NONE',  ( 42.52953848327577191, 205.3615022471903160, 5.000000000000046185 ) ) ;
#26475=CARTESIAN_POINT ( 'NONE',  ( 181.4638851230621981, 292.1855915779808583, 8.982959869412693976 ) ) ;
#26476=CARTESIAN_POINT ( 'NONE',  ( 202.8499463704053198, 279.3005819042728604, 17.04674939340617001 ) ) ;
#26477=CARTESIAN_POINT ( 'NONE',  ( 6.480970727150832111, 183.7369531367911009, -4.594050593750048428 ) ) ;
#26479=CARTESIAN_POINT ( 'NONE',  ( 164.0679150660969015, 247.0361648238571490, 5.995095722802411764 ) ) ;
#26480=EDGE_CURVE ( 'NONE', #7391, #19447, #21280, .T. ) ;
#26484=CARTESIAN_POINT ( 'NONE',  ( 179.6767793656050856, 277.0380904139387326, 16.30208254225003373 ) ) ;
#26489=CARTESIAN_POINT ( 'NONE',  ( 153.7085206060443454, 277.9268386586845736, -5.206943850374270433 ) ) ;
#26492=CARTESIAN_POINT ( 'NONE',  ( 154.9226727788713731, 262.3130548330639726, 18.22497199616848818 ) ) ;
#26496=CARTESIAN_POINT ( 'NONE',  ( 153.4477557824949940, 264.8676860077344486, 17.16010094972647693 ) ) ;
#26497=CARTESIAN_POINT ( 'NONE',  ( 164.8670003495851404, 245.0889742334797177, -1.557028074864921674 ) ) ;
#26498=CARTESIAN_POINT ( 'NONE',  ( 191.5687499534637652, 298.4314963742343139, 8.517990275034220460 ) ) ;
#26499=CARTESIAN_POINT ( 'NONE',  ( 203.3041373168503299, 278.5139001086923827, -16.61929732091214973 ) ) ;
#26502=VERTEX_POINT ( 'NONE', #68279 ) ;
#26503=FACE_OUTER_BOUND ( 'NONE', #12173, .T. ) ;
#26507=ORIENTED_EDGE ( 'NONE', *, *, #98728, .T. ) ;
#26509=CARTESIAN_POINT ( 'NONE',  ( 175.4059438627250529, 262.7554929797840941, 14.36458932732593397 ) ) ;
#26517=CARTESIAN_POINT ( 'NONE',  ( 173.8773719162893769, 267.3830834928915010, 16.61494387878642698 ) ) ;
#26518=CARTESIAN_POINT ( 'NONE',  ( 166.2593844326262911, 273.7376754232747658, -16.16122191897295224 ) ) ;
#26523=CARTESIAN_POINT ( 'NONE',  ( 203.0507839702407580, 278.9527209772879814, 16.21318481136342626 ) ) ;
#26525=EDGE_CURVE ( 'NONE', #8895, #48406, #70583, .T. ) ;
#26526=CARTESIAN_POINT ( 'NONE',  ( 156.8716556710364500, 266.6757045202047038, -16.21603570256788629 ) ) ;
#26527=VERTEX_POINT ( 'NONE', #16079 ) ;
#26531=( BOUNDED_CURVE ( )  B_SPLINE_CURVE ( 2, ( #57223, #20747, #51634, #28319, #12142, #88696, #97752, #4032, #58709 ),
 .UNSPECIFIED., .F., .T. ) 
 B_SPLINE_CURVE_WITH_KNOTS ( ( 3, 2, 2, 2, 3 ),
 ( 0.7782258064516128782, 0.7795698924731182533, 0.7822580645161290036, 0.7849462365591397539, 0.7862903225806451291 ),
 .UNSPECIFIED. ) 
 CURVE ( )  GEOMETRIC_REPRESENTATION_ITEM ( )  RATIONAL_B_SPLINE_CURVE ( ( 0.9330127018922194093, 0.9330127018922194093, 1.000000000000000000, 0.8660254037844387076, 1.000000000000000000, 0.8660254037844387076, 1.000000000000000000, 0.9330127018922194093, 0.9330127018922194093 ) ) 
 REPRESENTATION_ITEM ( '' )  );
#26532=CARTESIAN_POINT ( 'NONE',  ( 147.1938706002993626, 275.6997328879997440, 7.009419768930110095 ) ) ;
#26536=CARTESIAN_POINT ( 'NONE',  ( 178.0801157186545254, 291.3379508872625365, 6.079316923194516775 ) ) ;
#26537=CARTESIAN_POINT ( 'NONE',  ( 146.6363376198206652, 276.6654083370839885, -0.5879280619134327202 ) ) ;
#26541=CARTESIAN_POINT ( 'NONE',  ( 164.3493441216711517, 245.9855811210807417, 1.722120810491653664 ) ) ;
#26547=CARTESIAN_POINT ( 'NONE',  ( 187.6674080789407242, 277.1453262015298264, 17.21093267091079682 ) ) ;
#26548=CARTESIAN_POINT ( 'NONE',  ( 171.6829532011573747, 259.3958823610213358, -15.24497651433520318 ) ) ;
#26549=CARTESIAN_POINT ( 'NONE',  ( 163.5366322716688785, 247.7755347313017467, 7.814338521876752708 ) ) ;
#26550=CARTESIAN_POINT ( 'NONE',  ( 118.0080022156327431, 250.4860189848785126, -2.679491924311252493 ) ) ;
#26551=CARTESIAN_POINT ( 'NONE',  ( 159.9160972866109205, 253.6641898818994889, -15.06183666839949709 ) ) ;
#26552=CARTESIAN_POINT ( 'NONE',  ( 148.6217150854157580, 273.2266336944707632, -9.117259336374514689 ) ) ;
#26553=ORIENTED_EDGE ( 'NONE', *, *, #77001, .T. ) ;
#26555=EDGE_CURVE ( 'NONE', #37792, #16392, #18764, .T. ) ;
#26556=CARTESIAN_POINT ( 'NONE',  ( 42.66379208638658582, 206.9860189848785410, -2.679491924311252493 ) ) ;
#26557=CARTESIAN_POINT ( 'NONE',  ( 164.4781197247689306, 245.7625352337404649, -1.511762618280499515 ) ) ;
#26558=CARTESIAN_POINT ( 'NONE',  ( 32.40786657299730678, 179.5177522451417929, 5.000000000000051514 ) ) ;
#26559=CARTESIAN_POINT ( 'NONE',  ( 101.1213961584103060, 235.3149278399160664, -9.188101187500095079 ) ) ;
#26560=CARTESIAN_POINT ( 'NONE',  ( 183.8023311956230827, 297.0733055398724787, -2.815221220798488577 ) ) ;
#26561=CARTESIAN_POINT ( 'NONE',  ( 100.8442274002074441, 217.4824982072973683, 3.021315404115420679E-15 ) ) ;
#26562=CARTESIAN_POINT ( 'NONE',  ( 208.2995279947827783, 269.8616296508574237, 2.738519832864397152 ) ) ;
#26563=CARTESIAN_POINT ( 'NONE',  ( 12.78680497239753144, 184.3149278399160949, -9.188101187500095079 ) ) ;
#26565=ORIENTED_EDGE ( 'NONE', *, *, #72185, .F. ) ;
#26566=ORIENTED_EDGE ( 'NONE', *, *, #43547, .F. ) ;
#26567=CARTESIAN_POINT ( 'NONE',  ( 147.7140364658288263, 276.4223552458277027, -0.9273017251447416287 ) ) ;
#26572=CARTESIAN_POINT ( 'NONE',  ( 176.9878821292914211, 283.3466992399841615, -15.40003107629192769 ) ) ;
#26575=CARTESIAN_POINT ( 'NONE',  ( 44.66719160132967659, 208.8464784336661637, 1.353441290958777525E-15 ) ) ;
#26576=CARTESIAN_POINT ( 'NONE',  ( 89.99855592466249732, 212.7677522451417929, -5.000000000000041744 ) ) ;
#26580=VECTOR ( 'NONE', #49419, 1000.000000000000000 ) ;
#26583=CARTESIAN_POINT ( 'NONE',  ( 0.9064528339360315989, 162.1423013555410080, -4.594050593750043987 ) ) ;
#26585=CARTESIAN_POINT ( 'NONE',  ( 151.0801312611820890, 268.9685319718947198, -15.83903210480701240 ) ) ;
#26586=CARTESIAN_POINT ( 'NONE',  ( 188.8764293144468240, 259.6972905960182061, 3.583694637520717041 ) ) ;
#26587=CARTESIAN_POINT ( 'NONE',  ( 147.0456760057551833, 275.9564134551570760, -3.678503029046952033 ) ) ;
#26588=CARTESIAN_POINT ( 'NONE',  ( 177.5337925685473408, 280.1858537220425092, 16.79564202278857721 ) ) ;
#26589=CARTESIAN_POINT ( 'NONE',  ( 171.3751619920873281, 280.2398791927632828, 15.33202389549764888 ) ) ;
#26590=CARTESIAN_POINT ( 'NONE',  ( 191.0604813119340690, 299.7205343796033503, -9.270812881586136811 ) ) ;
#26591=CARTESIAN_POINT ( 'NONE',  ( 164.8670003495851404, 245.0889742334797177, -1.557028074864921674 ) ) ;
#26593=CARTESIAN_POINT ( 'NONE',  ( 3.125382611083894702, 162.6115022471902023, -5.000000000000041744 ) ) ;
#26595=CARTESIAN_POINT ( 'NONE',  ( 121.5540962550081190, 250.1744531367911009, 4.594050593750047540 ) ) ;
#26598=CARTESIAN_POINT ( 'NONE',  ( -27.42236680055714260, 166.5217562850347406, 1.224646799147364892E-15 ) ) ;
#26599=CARTESIAN_POINT ( 'NONE',  ( 196.4677418905696129, 290.3548843276421394, 17.08610552292358520 ) ) ;
#26600=CARTESIAN_POINT ( 'NONE',  ( 185.5710010263521212, 288.0579674285398255, 14.90484884845676383 ) ) ;
#26602=CARTESIAN_POINT ( 'NONE',  ( 191.2056514706806070, 299.4690922889112699, 7.290007621276087590 ) ) ;
#26603=CARTESIAN_POINT ( 'NONE',  ( 149.7109319212262051, 271.3400547943878109, -12.38605961032017433 ) ) ;
#26604=CARTESIAN_POINT ( 'NONE',  ( 190.1308301828542824, 300.0323083375496935, 4.625340536964981375 ) ) ;
#26605=CARTESIAN_POINT ( 'NONE',  ( 203.5963693286578007, 276.4956262415219612, 14.26529644090561710 ) ) ;
#26607=VERTEX_POINT ( 'NONE', #16577 ) ;
#26608=CARTESIAN_POINT ( 'NONE',  ( 189.0562362369354048, 265.6604396169832398, 11.68942508348690268 ) ) ;
#26613=CARTESIAN_POINT ( 'NONE',  ( 155.5527680174282068, 261.6201814834243464, 16.99819418695508588 ) ) ;
#26615=CARTESIAN_POINT ( 'NONE',  ( 153.0070714074088016, 265.6309737354857248, 17.74442213480098474 ) ) ;
#26617=CARTESIAN_POINT ( 'NONE',  ( 198.2505066714982149, 285.2670451491296149, 0.000000000000000000 ) ) ;
#26619=CARTESIAN_POINT ( 'NONE',  ( 191.8474946137321524, 287.8597454743107846, -15.89771325201565233 ) ) ;
#26620=VERTEX_POINT ( 'NONE', #64182 ) ;
#26622=CARTESIAN_POINT ( 'NONE',  ( 194.1789525331299728, 294.3191837825503967, -15.34533909744314961 ) ) ;
#26623=CARTESIAN_POINT ( 'NONE',  ( 159.7423958009181320, 264.1536618208600657, -17.54225510600860716 ) ) ;
#26626=CARTESIAN_POINT ( 'NONE',  ( 204.8815496696085177, 273.0746141528632620, -9.761282367569325658 ) ) ;
#26629=CARTESIAN_POINT ( 'NONE',  ( 177.4877928417686803, 293.5951873982637608, -2.837372163671336267 ) ) ;
#26630=CARTESIAN_POINT ( 'NONE',  ( 184.4003287965598474, 259.5388931828980503, -5.814281059522229178 ) ) ;
#26632=ORIENTED_EDGE ( 'NONE', *, *, #10255, .F. ) ;
#26633=EDGE_CURVE ( 'NONE', #87662, #77729, #17074, .T. ) ;
#26636=AXIS2_PLACEMENT_3D ( 'NONE', #993, #38975, #56167 ) ;
#26637=VERTEX_POINT ( 'NONE', #12368 ) ;
#26638=EDGE_CURVE ( 'NONE', #6447, #68960, #95130, .T. ) ;
#26640=CARTESIAN_POINT ( 'NONE',  ( 155.1398527401465230, 261.9368881057492899, -17.02245700497956449 ) ) ;
#26641=ORIENTED_EDGE ( 'NONE', *, *, #98262, .F. ) ;
#26643=CARTESIAN_POINT ( 'NONE',  ( 160.4314248734274031, 254.1918255350734057, -15.30701149497589064 ) ) ;
#26645=CARTESIAN_POINT ( 'NONE',  ( 147.5749398328735822, 275.0397016159798227, -4.620786157167191099 ) ) ;
#26646=CARTESIAN_POINT ( 'NONE',  ( 153.2906404175950854, 265.1398178023911782, -17.60231834963988007 ) ) ;
#26648=CARTESIAN_POINT ( 'NONE',  ( 167.8988096083529911, 276.9559784313423165, -15.94421658709092426 ) ) ;
#26651=CARTESIAN_POINT ( 'NONE',  ( 145.6409484414103588, 245.7048013555409511, 4.594050593750051981 ) ) ;
#26654=CARTESIAN_POINT ( 'NONE',  ( 199.9521760394648027, 270.2061738998779674, 9.324312810954292985 ) ) ;
#26657=CARTESIAN_POINT ( 'NONE',  ( -6.635445380951201066, 173.6427522451419065, 10.00000000000009415 ) ) ;
#26658=CARTESIAN_POINT ( 'NONE',  ( 170.4623819437503016, 288.8056674672355939, -5.476885062779371260 ) ) ;
#26659=CARTESIAN_POINT ( 'NONE',  ( 157.3440770660893975, 280.1834744503427146, -6.999751510017727441 ) ) ;
#26660=CARTESIAN_POINT ( 'NONE',  ( 165.4921054121714121, 246.8916612925589220, -1.878118433271425136 ) ) ;
#26661=CARTESIAN_POINT ( 'NONE',  ( 192.8319713945120668, 292.4878551455605589, -14.36409660672679856 ) ) ;
#26665=CARTESIAN_POINT ( 'NONE',  ( 147.8819534105757043, 274.5079385007862811, -9.338341377131436971 ) ) ;
#26669=CARTESIAN_POINT ( 'NONE',  ( 201.1812938895721459, 267.3327365634810349, -2.234727838033611746 ) ) ;
#26671=CARTESIAN_POINT ( 'NONE',  ( 190.2935937139882299, 301.0488226629397559, 4.649863831023156813 ) ) ;
#26672=CARTESIAN_POINT ( 'NONE',  ( 163.4004183463084416, 247.6291687766210146, 10.19167732382099345 ) ) ;
#26676=FACE_OUTER_BOUND ( 'NONE', #56425, .T. ) ;
#26684=CARTESIAN_POINT ( 'NONE',  ( 163.1014434023538513, 248.1470085697407058, 9.692260209037655727 ) ) ;
#26685=CARTESIAN_POINT ( 'NONE',  ( 0.9872088458345585904, 177.5024278399160949, 9.188101187500095079 ) ) ;
#26686=CARTESIAN_POINT ( 'NONE',  ( 99.38934535084139554, 234.3149278399160949, 9.188101187500093303 ) ) ;
#26687=CARTESIAN_POINT ( 'NONE',  ( 202.8535267948003593, 279.2943804273081696, -15.36804658072946062 ) ) ;
#26688=CARTESIAN_POINT ( 'NONE',  ( 178.2543802835785698, 279.4939343734425279, -17.11033828990027672 ) ) ;
#26689=CARTESIAN_POINT ( 'NONE',  ( 182.3427999490124307, 257.2899902172831617, -2.311323497713533737 ) ) ;
#26696=CARTESIAN_POINT ( 'NONE',  ( 160.1795347027651815, 282.8633239002924711, 5.491715875156680582 ) ) ;
#26697=CARTESIAN_POINT ( 'NONE',  ( 194.9455394410084921, 292.9914163096879065, -15.01116663483170655 ) ) ;
#26698=CARTESIAN_POINT ( 'NONE',  ( 181.3660832969280250, 291.3269257893657596, 9.327634650582066200 ) ) ;
#26700=CARTESIAN_POINT ( 'NONE',  ( 164.4057847141585285, 245.8878231472837115, -5.819655715517686900 ) ) ;
#26701=CARTESIAN_POINT ( 'NONE',  ( 2.963002844326352747, 172.5177522451418781, -10.00000000000009592 ) ) ;
#26703=CARTESIAN_POINT ( 'NONE',  ( 155.8152618860606253, 260.7670451491295012, 0.000000000000000000 ) ) ;
#26706=CARTESIAN_POINT ( 'NONE',  ( 176.1555758231396567, 265.5273580598085914, -16.25916769215487889 ) ) ;
#26708=CARTESIAN_POINT ( 'NONE',  ( 77.38680066200176100, 224.6744531367911293, 4.594050593750047540 ) ) ;
#26709=CARTESIAN_POINT ( 'NONE',  ( 207.8570869662935365, 270.6279599915536664, -5.669188455878507504 ) ) ;
#26712=CARTESIAN_POINT ( 'NONE',  ( 163.3923068497962277, 257.9918827725503547, 15.63397831145243622 ) ) ;
#26721=CARTESIAN_POINT ( 'NONE',  ( 71.08131351252005459, 211.8458772461660544, 9.188101187500095079 ) ) ;
#26722=CARTESIAN_POINT ( 'NONE',  ( 171.5149613532572914, 288.8291111043322417, -1.065049549448901844 ) ) ;
#26724=CARTESIAN_POINT ( 'NONE',  ( 188.2744068810562510, 286.2937481655858960, -16.77334613339053249 ) ) ;
#26726=CARTESIAN_POINT ( 'NONE',  ( 191.7501012462608116, 287.4658672486679052, 16.07335574080813245 ) ) ;
#26727=CARTESIAN_POINT ( 'NONE',  ( -17.42236680055705023, 149.2012482093457777, 0.000000000000000000 ) ) ;
#26728=CARTESIAN_POINT ( 'NONE',  ( 129.2042476453684117, 238.7365022471901739, -10.00000000000009059 ) ) ;
#26732=CARTESIAN_POINT ( 'NONE',  ( 165.6980386070991926, 247.0211899460981044, -1.865356867150344655 ) ) ;
#26734=CARTESIAN_POINT ( 'NONE',  ( 162.9796882977680639, 248.3578945969637743, 9.683801903336119565 ) ) ;
#26736=FACE_OUTER_BOUND ( 'NONE', #85499, .T. ) ;
#26740=CARTESIAN_POINT ( 'NONE',  ( 189.4441960630004189, 289.9932173292452262, 14.44447376131311778 ) ) ;
#26741=CARTESIAN_POINT ( 'NONE',  ( 40.18174127881769664, 205.5530062829863027, -4.648177544792955347E-16 ) ) ;
#26744=ORIENTED_EDGE ( 'NONE', *, *, #9835, .F. ) ;
#26745=CARTESIAN_POINT ( 'NONE',  ( 110.1516887621107657, 227.7365022471902307, 10.00000000000009948 ) ) ;
#26749=ADVANCED_FACE ( 'NONE', ( #91883 ), #5253, .T. ) ;
#26752=CARTESIAN_POINT ( 'NONE',  ( 53.05822266071304938, 189.8932355074535678, -2.679491924311248496 ) ) ;
#26754=VERTEX_POINT ( 'NONE', #98466 ) ;
#26755=CARTESIAN_POINT ( 'NONE',  ( 186.3700259935355064, 298.5219211581387526, 1.062272678801966297 ) ) ;
#26756=CARTESIAN_POINT ( 'NONE',  ( 204.2457645315488719, 276.8829539310449945, 14.53406579917280261 ) ) ;
#26757=CARTESIAN_POINT ( 'NONE',  ( 147.7785919239399846, 274.6869658471848652, -7.924750738206837397 ) ) ;
#26760=CARTESIAN_POINT ( 'NONE',  ( 190.7685386727469279, 298.2261938635710976, -9.678376712886644029 ) ) ;
#26761=CARTESIAN_POINT ( 'NONE',  ( 187.5841530998652331, 291.2525622860537169, -13.74720276183634660 ) ) ;
#26762=EDGE_CURVE ( 'NONE', #13784, #52411, #62329, .T. ) ;
#26763=CARTESIAN_POINT ( 'NONE',  ( 164.1886994716367383, 246.2638258169049266, 4.302100816186628762 ) ) ;
#26767=CARTESIAN_POINT ( 'NONE',  ( 103.3950599391094443, 224.3768266524160140, -9.188101187500091527 ) ) ;
#26770=CARTESIAN_POINT ( 'NONE',  ( 166.2786698706664765, 279.3007919285489606, -14.16120680810289301 ) ) ;
#26772=ORIENTED_EDGE ( 'NONE', *, *, #2576, .F. ) ;
#26773=B_SPLINE_CURVE_WITH_KNOTS ( 'NONE', 3,
 ( #91545, #45882, #16501, #31195 ),
 .UNSPECIFIED., .F., .F.,
 ( 4, 4 ),
 ( 0.01063587648819574669, 0.01619468505063361569 ),
 .UNSPECIFIED. ) ;
#26776=CARTESIAN_POINT ( 'NONE',  ( 163.0358311274019343, 249.2395244830586307, 10.27721552788938908 ) ) ;
#26777=CARTESIAN_POINT ( 'NONE',  ( 206.6912923161529818, 272.6471755567893638, -9.325620632947922317 ) ) ;
#26778=CARTESIAN_POINT ( 'NONE',  ( 208.0941653616417852, 270.2173281654339689, 1.603026803260118704 ) ) ;
#26779=CARTESIAN_POINT ( 'NONE',  ( 94.00418374076319594, 215.8923013555410080, 4.594050593750050204 ) ) ;
#26780=ORIENTED_EDGE ( 'NONE', *, *, #5267, .T. ) ;
#26783=CARTESIAN_POINT ( 'NONE',  ( 162.7007457333762090, 248.8410372908842021, -10.94671474643812914 ) ) ;
#26787=CARTESIAN_POINT ( 'NONE',  ( 183.6498318386265396, 256.3252116762061519, 1.424693195823348635 ) ) ;
#26788=CARTESIAN_POINT ( 'NONE',  ( 165.5754880998921408, 285.4032371899495502, 0.7844207949055206353 ) ) ;
#26789=CARTESIAN_POINT ( 'NONE',  ( 137.4944631173567018, 256.3149278399160380, -9.188101187500095079 ) ) ;
#26791=CARTESIAN_POINT ( 'NONE',  ( -6.130263895410251962, 167.2677522451418781, 10.00000000000009592 ) ) ;
#26792=LINE ( 'NONE', #35378, #65799 ) ;
#26797=CARTESIAN_POINT ( 'NONE',  ( 114.8426596992763962, 247.1115022471903160, -5.000000000000047962 ) ) ;
#26800=DIRECTION ( 'NONE',  ( 0.4999999999999992784, -0.8660254037844390407, 0.000000000000000000 ) ) ;
#26802=( BOUNDED_CURVE ( )  B_SPLINE_CURVE ( 2, ( #61404, #58300, #19826, #81651, #88779, #73039, #87298, #72030, #72545 ),
 .UNSPECIFIED., .F., .T. ) 
 B_SPLINE_CURVE_WITH_KNOTS ( ( 3, 2, 2, 2, 3 ),
 ( 0.6169354838709677491, 0.6182795698924731242, 0.6209677419354838745, 0.6236559139784946248, 0.6250000000000000000 ),
 .UNSPECIFIED. ) 
 CURVE ( )  GEOMETRIC_REPRESENTATION_ITEM ( )  RATIONAL_B_SPLINE_CURVE ( ( 0.9330127018922194093, 0.9330127018922194093, 1.000000000000000000, 0.8660254037844387076, 1.000000000000000000, 0.8660254037844387076, 1.000000000000000000, 0.9330127018922194093, 0.9330127018922194093 ) ) 
 REPRESENTATION_ITEM ( '' )  );
#26805=CARTESIAN_POINT ( 'NONE',  ( 206.8851632406098702, 272.3113812655195716, -9.957011741946159233 ) ) ;
#26807=CARTESIAN_POINT ( 'NONE',  ( 207.5920568422024814, 271.0870056320159165, -1.586464549033245186 ) ) ;
#26808=CARTESIAN_POINT ( 'NONE',  ( 202.5283990184146035, 279.8575182549602118, -15.90040239656587140 ) ) ;
#26810=AXIS2_PLACEMENT_3D ( 'NONE', #72163, #79295, #9865 ) ;
#26813=CARTESIAN_POINT ( 'NONE',  ( 185.1232581413127036, 266.3925326034153613, 13.18423089168799933 ) ) ;
#26814=CARTESIAN_POINT ( 'NONE',  ( 170.1892289429057996, 282.6882086596259001, 13.36031953422248364 ) ) ;
#26815=EDGE_CURVE ( 'NONE', #52681, #23462, #84246, .T. ) ;
#26817=CARTESIAN_POINT ( 'NONE',  ( 90.89058176318043536, 234.8297689869269220, -2.679491924311252493 ) ) ;
#26820=CARTESIAN_POINT ( 'NONE',  ( 158.0014590649305717, 271.2370772881457697, -14.70865708044451736 ) ) ;
#26822=CARTESIAN_POINT ( 'NONE',  ( 161.1150691641480535, 251.5875096731584506, -13.48836942566120101 ) ) ;
#26823=CARTESIAN_POINT ( 'NONE',  ( 15.03297158952216961, 188.6744531367911293, 4.594050593750047540 ) ) ;
#26825=ORIENTED_EDGE ( 'NONE', *, *, #64750, .T. ) ;
#26826=EDGE_CURVE ( 'NONE', #26527, #34648, #52652, .T. ) ;
#26828=CARTESIAN_POINT ( 'NONE',  ( 195.6664450926536460, 278.3245960621525796, 17.18455885460583232 ) ) ;
#26830=CARTESIAN_POINT ( 'NONE',  ( 37.30632276492696064, 192.3458772461660544, 9.188101187500095079 ) ) ;
#26831=CARTESIAN_POINT ( 'NONE',  ( 161.6256441450323678, 250.7031678651938762, 14.48526717260977037 ) ) ;
#26833=CARTESIAN_POINT ( 'NONE',  ( 146.9709166616330549, 276.0859004375172390, 3.755270622130282732 ) ) ;
#26835=CARTESIAN_POINT ( 'NONE',  ( 178.0294974782117947, 292.4800352430163457, 5.617471776230186009 ) ) ;
#26839=CARTESIAN_POINT ( 'NONE',  ( 179.9555032624530497, 279.0079853041619913, -17.36825822513608486 ) ) ;
#26841=CARTESIAN_POINT ( 'NONE',  ( 164.5980941468485526, 256.8328644044750035, -14.91555327743531834 ) ) ;
#26842=EDGE_CURVE ( 'NONE', #68153, #40206, #65933, .T. ) ;
#26846=CARTESIAN_POINT ( 'NONE',  ( 83.66574516303664666, 219.1115022471902591, 10.00000000000009592 ) ) ;
#26849=CARTESIAN_POINT ( 'NONE',  ( 49.15987193134396449, 205.3149278399160949, -9.188101187500095079 ) ) ;
#26850=VERTEX_POINT ( 'NONE', #21936 ) ;
#26852=CARTESIAN_POINT ( 'NONE',  ( 150.7691137448031213, 269.5072301123068428, -15.63821625702598084 ) ) ;
#26855=CARTESIAN_POINT ( 'NONE',  ( 168.3183238356223228, 286.2632724110728759, 8.085195618967237152 ) ) ;
#26856=CARTESIAN_POINT ( 'NONE',  ( 207.1059763530604698, 271.9289217357780899, 6.370907250589925575 ) ) ;
#26857=CARTESIAN_POINT ( 'NONE',  ( 159.8440474668410332, 278.4957488270735553, -10.68596225390687415 ) ) ;
#26859=CARTESIAN_POINT ( 'NONE',  ( 185.7602392900914481, 263.0086591247442129, 11.24710565870787882 ) ) ;
#26861=FACE_OUTER_BOUND ( 'NONE', #9053, .T. ) ;
#26865=CARTESIAN_POINT ( 'NONE',  ( 174.6110402932947636, 255.0538503848414109, 8.239021665820192908 ) ) ;
#26869=CARTESIAN_POINT ( 'NONE',  ( 178.6471812665516552, 282.3158997316623982, 15.55331189247123547 ) ) ;
#26870=CARTESIAN_POINT ( 'NONE',  ( 190.8443993347725325, 300.0947993426467519, 8.522468760355437212 ) ) ;
#26871=CARTESIAN_POINT ( 'NONE',  ( 177.4279444979247273, 255.8030325494246711, -6.933745715773924623 ) ) ;
#26873=VERTEX_POINT ( 'NONE', #38111 ) ;
#26874=EDGE_LOOP ( 'NONE', ( #42200, #70648, #51099, #54822, #41274 ) ) ;
#26876=CARTESIAN_POINT ( 'NONE',  ( 207.8792014703394671, 270.5896565469619759, -5.780233892547864905 ) ) ;
#26878=CARTESIAN_POINT ( 'NONE',  ( 196.7491951525289835, 289.8673929779723721, -16.35352603081977207 ) ) ;
#26881=CARTESIAN_POINT ( 'NONE',  ( 198.2489255580726422, 287.2697837179150042, 18.53597557040773225 ) ) ;
#26884=CARTESIAN_POINT ( 'NONE',  ( 157.7733463334721478, 257.3755434007023268, -16.94489513499352995 ) ) ;
#26885=CARTESIAN_POINT ( 'NONE',  ( 109.0781781035623226, 233.7833772461660544, -9.188101187500095079 ) ) ;
#26887=CARTESIAN_POINT ( 'NONE',  ( 204.5621601773678719, 270.1235943821444607, 7.273613950894332270 ) ) ;
#26888=CARTESIAN_POINT ( 'NONE',  ( 35.43895548624285396, 181.2677522451417929, -5.000000000000041744 ) ) ;
#26891=CARTESIAN_POINT ( 'NONE',  ( 208.3135187673106543, 269.8373969220020285, 2.829653198597726682 ) ) ;
#26897=CARTESIAN_POINT ( 'NONE',  ( 77.73905735199544154, 209.5643266524159856, -9.188101187500093303 ) ) ;
#26899=CARTESIAN_POINT ( 'NONE',  ( 151.4361976351029000, 268.3518069213970421, 15.15218985681980612 ) ) ;
#26900=CARTESIAN_POINT ( 'NONE',  ( 199.3352131601118344, 270.6712675723642292, 12.00403451141520250 ) ) ;
#26901=CARTESIAN_POINT ( 'NONE',  ( 81.63706098559951840, 206.3932355074535963, -2.679491924311248496 ) ) ;
#26904=CARTESIAN_POINT ( 'NONE',  ( 155.6066474290145720, 261.1283759879266881, -18.16552045242181279 ) ) ;
#26906=CARTESIAN_POINT ( 'NONE',  ( 91.00660716696485508, 234.8967562850347122, -4.648177544792955347E-16 ) ) ;
#26908=CARTESIAN_POINT ( 'NONE',  ( 163.0918957739551445, 259.9684307908772212, -16.22645816865646040 ) ) ;
#26909=CARTESIAN_POINT ( 'NONE',  ( 206.6785509007829944, 270.7286264247209715, 2.448473520048410013 ) ) ;
#26910=CARTESIAN_POINT ( 'NONE',  ( 190.1190668544949460, 301.3511120508678118, 4.410340539513557090 ) ) ;
#26911=CARTESIAN_POINT ( 'NONE',  ( 164.2572333502590709, 246.1451216570909253, 2.155809084027023204 ) ) ;
#26912=CARTESIAN_POINT ( 'NONE',  ( 152.3820699219956225, 270.2311863471538800, -14.73681983046514254 ) ) ;
#26914=CARTESIAN_POINT ( 'NONE',  ( 166.4111547595541367, 255.8261474448014781, 13.77734897554943849 ) ) ;
#26915=CARTESIAN_POINT ( 'NONE',  ( 163.7423057141168385, 247.0370024851108610, -6.909410042141566066 ) ) ;
#26916=CARTESIAN_POINT ( 'NONE',  ( 122.2307653756559773, 247.5024278399160949, -9.188101187500093303 ) ) ;
#26917=ORIENTED_EDGE ( 'NONE', *, *, #19007, .T. ) ;
#26927=CARTESIAN_POINT ( 'NONE',  ( 179.4722142099873565, 269.7276464518548096, -17.35046799866735157 ) ) ;
#26928=CARTESIAN_POINT ( 'NONE',  ( 152.6809499003229860, 273.9044486092186048, 12.24870461040242553 ) ) ;
#26929=CARTESIAN_POINT ( 'NONE',  ( 147.7177902700356071, 275.4030622120182557, 3.691961389914627745 ) ) ;
#26931=CARTESIAN_POINT ( 'NONE',  ( 206.5431607373320730, 272.9037469775124691, -11.15649369879132102 ) ) ;
#26932=CARTESIAN_POINT ( 'NONE',  ( 143.7012754916490280, 257.3569598644533585, -9.188101187500093303 ) ) ;
#26933=CARTESIAN_POINT ( 'NONE',  ( 18.37649865285644779, 192.9637435831425023, 2.679491924311251605 ) ) ;
#26937=CARTESIAN_POINT ( 'NONE',  ( 190.2389970918280540, 301.1433867864428748, 4.601241515604689525 ) ) ;
#26939=CARTESIAN_POINT ( 'NONE',  ( 171.4999057815707033, 286.5447579310401238, -8.034712056625934906 ) ) ;
#26940=CARTESIAN_POINT ( 'NONE',  ( 205.0025969320384718, 269.2761223580778847, -4.589315089892217259 ) ) ;
#26941=CARTESIAN_POINT ( 'NONE',  ( 186.1630411436486554, 296.9614825196608194, -7.488375694256206749 ) ) ;
#26942=CARTESIAN_POINT ( 'NONE',  ( 137.9907970510500661, 257.1427522451419350, -10.00000000000009415 ) ) ;
#26944=ORIENTED_EDGE ( 'NONE', *, *, #88894, .T. ) ;
#26945=EDGE_CURVE ( 'NONE', #23996, #80478, #45298, .T. ) ;
#26946=CARTESIAN_POINT ( 'NONE',  ( 157.5520850189458884, 257.7587792392113215, 16.71892742266126319 ) ) ;
#26947=CARTESIAN_POINT ( 'NONE',  ( 148.3930300673291640, 273.6227277647267897, 8.375036249079425232 ) ) ;
#26948=CARTESIAN_POINT ( 'NONE',  ( 0.5816933075168655431, 161.9548013555410080, -4.594050593750042211 ) ) ;
#26950=CARTESIAN_POINT ( 'NONE',  ( 44.12627281972940807, 196.2833772461660828, -9.188101187500095079 ) ) ;
#26951=CARTESIAN_POINT ( 'NONE',  ( 178.6463706910270730, 259.1961072996702455, -10.35245457583735629 ) ) ;
#26954=CARTESIAN_POINT ( 'NONE',  ( 205.3704330671644414, 274.9349708856848338, -13.01557521325596944 ) ) ;
#26955=CARTESIAN_POINT ( 'NONE',  ( 192.2321494539393996, 293.0484659149655045, -14.31527305258243743 ) ) ;
#26957=CARTESIAN_POINT ( 'NONE',  ( 190.9498149295421570, 299.9122141765958531, -5.138500224925297566 ) ) ;
#26960=CARTESIAN_POINT ( 'NONE',  ( 71.30684095964828373, 218.6427522451419065, 10.00000000000009237 ) ) ;
#26965=CIRCLE ( 'NONE', #62510, 2.471954595299370006 ) ;
#26966=EDGE_CURVE ( 'NONE', #27863, #35723, #46544, .T. ) ;
#26967=CARTESIAN_POINT ( 'NONE',  ( 179.1629783499468260, 294.4842721394058458, 1.069721132174473288 ) ) ;
#26968=CARTESIAN_POINT ( 'NONE',  ( 40.86965645935567437, 187.7365022471901739, -10.00000000000009059 ) ) ;
#26969=PLANE ( 'NONE',  #73359 ) ;
#26970=CARTESIAN_POINT ( 'NONE',  ( 203.0337691736598629, 278.9821914694464340, 16.08167820133810011 ) ) ;
#26971=CARTESIAN_POINT ( 'NONE',  ( -5.399728507075681527, 173.8149278399160949, -9.188101187500095079 ) ) ;
#26973=CARTESIAN_POINT ( 'NONE',  ( 163.2659639011634169, 252.2459686854220422, 13.11545999390232353 ) ) ;
#26974=CARTESIAN_POINT ( 'NONE',  ( 153.3703256797887775, 265.0017988796566897, 16.44314709207578318 ) ) ;
#26976=CARTESIAN_POINT ( 'NONE',  ( 164.9103019330012216, 245.0139736909548560, 2.841678961959298810 ) ) ;
#26977=CARTESIAN_POINT ( 'NONE',  ( 183.3303171387637747, 279.0281335762378490, 17.06007825884248064 ) ) ;
#26979=CARTESIAN_POINT ( 'NONE',  ( 70.67536410627006660, 211.6115022471902591, 10.00000000000009592 ) ) ;
#26980=CARTESIAN_POINT ( 'NONE',  ( 146.4729408656479563, 243.8262482093457493, 3.021315404115420679E-15 ) ) ;
#26982=CARTESIAN_POINT ( 'NONE',  ( 165.6069501779841460, 285.3987855451247810, 0.3448102065264236904 ) ) ;
#26984=CARTESIAN_POINT ( 'NONE',  ( 181.8129518053731033, 270.5384970965435514, -17.23398818032472946 ) ) ;
#26986=CARTESIAN_POINT ( 'NONE',  ( 154.8679462054080318, 262.4078440388265676, 17.98338675682672871 ) ) ;
#26991=CARTESIAN_POINT ( 'NONE',  ( 153.4578721839791342, 264.8501638863745029, 16.85421393845643223 ) ) ;
#26992=CARTESIAN_POINT ( 'NONE',  ( 164.2600772519394923, 246.1401958748887182, -2.110785484364219311 ) ) ;
#26995=CARTESIAN_POINT ( 'NONE',  ( 125.8043565786058906, 231.8932355074535394, -2.679491924311248496 ) ) ;
#26996=ORIENTED_EDGE ( 'NONE', *, *, #88908, .F. ) ;
#26997=EDGE_LOOP ( 'NONE', ( #43941, #86854, #48698, #94936 ) ) ;
#27000=CARTESIAN_POINT ( 'NONE',  ( 164.2413944571582078, 246.1725554246774834, 7.304616466633322425 ) ) ;
#27002=ORIENTED_EDGE ( 'NONE', *, *, #39709, .T. ) ;
#27004=CARTESIAN_POINT ( 'NONE',  ( 177.1347673595945764, 262.9921672455169528, 15.53478677465993485 ) ) ;
#27010=B_SPLINE_CURVE_WITH_KNOTS ( 'NONE', 3,
 ( #94960, #89853, #66017, #96966, #13327, #82761, #27532, #89376, #59381, #37099, #36097, #29022, #19931, #90357, #66998, #58403, #27028, #20938, #74642, #52298, #13804, #50804 ),
 .UNSPECIFIED., .F., .F.,
 ( 4, 2, 2, 2, 2, 2, 2, 2, 2, 2, 4 ),
 ( 0.0003198756514526470991, 0.002147329819704916695, 0.002604193361768018626, 0.002661301304525904091, 0.002689855275904812562, 0.002718409247283721034, 0.002832625132799350583, 0.003061056903830601007, 0.003289488674861852299, 0.003517920445893102724, 0.003974783987955634798 ),
 .UNSPECIFIED. ) ;
#27013=CARTESIAN_POINT ( 'NONE',  ( 161.7910648966377209, 250.4166507187868831, 13.19274492748169436 ) ) ;
#27014=CARTESIAN_POINT ( 'NONE',  ( 166.1007185193450937, 274.1064974184767493, -15.20043799348013458 ) ) ;
#27017=EDGE_CURVE ( 'NONE', #71681, #441, #24844, .T. ) ;
#27018=CARTESIAN_POINT ( 'NONE',  ( 190.0340467409721441, 301.4983712071542641, 4.077645795029533282 ) ) ;
#27021=ORIENTED_EDGE ( 'NONE', *, *, #63629, .T. ) ;
#27022=CARTESIAN_POINT ( 'NONE',  ( 157.3910266414278851, 266.9754241737259122, -16.20060215746766374 ) ) ;
#27023=EDGE_LOOP ( 'NONE', ( #31100, #98959, #58026, #9315, #64638 ) ) ;
#27026=CARTESIAN_POINT ( 'NONE',  ( 159.1685125254583966, 259.5000883001122247, 16.69271994272259008 ) ) ;
#27027=CARTESIAN_POINT ( 'NONE',  ( 193.8257114866206905, 294.9310152224236390, 14.87231647135867796 ) ) ;
#27028=CARTESIAN_POINT ( 'NONE',  ( 188.5854780552674868, 298.6315526637507105, -4.814084629927046777 ) ) ;
#27030=CARTESIAN_POINT ( 'NONE',  ( 200.2629047362840424, 281.3048619616022279, -17.25979275631262055 ) ) ;
#27032=CARTESIAN_POINT ( 'NONE',  ( 158.4167541826878391, 256.2611283158722699, -16.34182606312789687 ) ) ;
#27033=VERTEX_POINT ( 'NONE', #6595 ) ;
#27037=CARTESIAN_POINT ( 'NONE',  ( 206.4537138826727301, 273.0586734743599209, 11.45643784582899016 ) ) ;
#27038=CARTESIAN_POINT ( 'NONE',  ( 164.3036517873781008, 252.3706336020835579, 13.60069832213670082 ) ) ;
#27039=CARTESIAN_POINT ( 'NONE',  ( 164.9103019330012216, 245.0139736909548560, 2.841678961959298810 ) ) ;
#27040=CARTESIAN_POINT ( 'NONE',  ( 198.5612432604688991, 286.7288335892616260, 18.30793681285053509 ) ) ;
#27043=ORIENTED_EDGE ( 'NONE', *, *, #17582, .T. ) ;
#27044=CARTESIAN_POINT ( 'NONE',  ( 187.3665724429023101, 277.0083082519628306, 16.89536893287339225 ) ) ;
#27048=CARTESIAN_POINT ( 'NONE',  ( 199.0022468604825292, 285.9649929477169508, -18.62203328612563169 ) ) ;
#27049=CARTESIAN_POINT ( 'NONE',  ( 148.4975630032294021, 273.4416714086831917, -10.35571102360928464 ) ) ;
#27051=CARTESIAN_POINT ( 'NONE',  ( 167.5508029243457599, 252.8355245762918173, -12.42550861741178991 ) ) ;
#27056=CARTESIAN_POINT ( 'NONE',  ( 35.43895548624285396, 181.2677522451417929, -5.000000000000041744 ) ) ;
#27057=CARTESIAN_POINT ( 'NONE',  ( 98.19890751640281223, 221.3768266524159856, -9.188101187500093303 ) ) ;
#27059=CARTESIAN_POINT ( 'NONE',  ( 167.4021843883327278, 282.9460231506713512, -10.86961029474059259 ) ) ;
#27061=CARTESIAN_POINT ( 'NONE',  ( 162.4279131726858623, 249.3135971479585464, 10.85034575916916921 ) ) ;
#27062=CARTESIAN_POINT ( 'NONE',  ( 17.65854496445001232, 174.8768266524159856, -9.188101187500091527 ) ) ;
#27064=ORIENTED_EDGE ( 'NONE', *, *, #19726, .T. ) ;
#27066=ORIENTED_EDGE ( 'NONE', *, *, #51502, .F. ) ;
#27067=CARTESIAN_POINT ( 'NONE',  ( 147.7840609055601817, 276.6774932931532476, -0.9735537997635442808 ) ) ;
#27069=CARTESIAN_POINT ( 'NONE',  ( 147.0670278774466908, 275.9194309285509235, 3.666898409139099257 ) ) ;
#27070=CARTESIAN_POINT ( 'NONE',  ( 193.6564271169084464, 262.6014873983580742, -4.146719891036213745 ) ) ;
#27075=CARTESIAN_POINT ( 'NONE',  ( 46.72434903108273119, 197.7833772461660828, -9.188101187500095079 ) ) ;
#27076=CARTESIAN_POINT ( 'NONE',  ( 86.02927282398376008, 227.1427522451419634, -10.00000000000009415 ) ) ;
#27079=B_SPLINE_CURVE_WITH_KNOTS ( 'NONE', 3,
 ( #8912, #61604, #69709, #86983 ),
 .UNSPECIFIED., .F., .F.,
 ( 4, 4 ),
 ( 0.03082140243953887179, 0.03988153003689407644 ),
 .UNSPECIFIED. ) ;
#27081=CARTESIAN_POINT ( 'NONE',  ( 181.2305897479128305, 260.5010089447542896, -10.41488471035008168 ) ) ;
#27082=CARTESIAN_POINT ( 'NONE',  ( -0.5554856785977280165, 179.6744531367911577, 4.594050593750047540 ) ) ;
#27084=CARTESIAN_POINT ( 'NONE',  ( 179.3484626673140383, 285.2557201243848795, -15.12459571388282420 ) ) ;
#27086=CARTESIAN_POINT ( 'NONE',  ( 146.8868584395697781, 276.2314935489248455, -3.891417269505058396 ) ) ;
#27088=CARTESIAN_POINT ( 'NONE',  ( 180.8890834033174713, 294.3766012452771861, 6.559837412958372305 ) ) ;
#27089=ADVANCED_FACE ( 'NONE', ( #53666 ), #10084, .F. ) ;
#27091=CARTESIAN_POINT ( 'NONE',  ( 164.9586510554008782, 244.9302305544571823, -1.717556444319656039 ) ) ;
#27094=ADVANCED_FACE ( 'NONE', ( #49088 ), #25431, .F. ) ;
#27095=CARTESIAN_POINT ( 'NONE',  ( -0.8439004895947717078, 156.9865022471901455, 1.119607411625061291E-15 ) ) ;
#27097=CARTESIAN_POINT ( 'NONE',  ( 126.2364799639240260, 237.5643266524160140, 9.188101187500095079 ) ) ;
#27100=CARTESIAN_POINT ( 'NONE',  ( -22.42236680055709641, 157.8615022471902591, 0.000000000000000000 ) ) ;
#27101=CARTESIAN_POINT ( 'NONE',  ( 196.4390255720217908, 290.4046224503736653, 16.34739044515864848 ) ) ;
#27102=CARTESIAN_POINT ( 'NONE',  ( 168.0462690533684338, 251.4142709888886884, 10.74789308012043954 ) ) ;
#27103=CARTESIAN_POINT ( 'NONE',  ( 150.3471325113991952, 270.2381230484028833, -13.97988400279308330 ) ) ;
#27104=ORIENTED_EDGE ( 'NONE', *, *, #80179, .T. ) ;
#27105=CARTESIAN_POINT ( 'NONE',  ( 190.7851751463332164, 300.1973786460605425, 8.237717828100052486 ) ) ;
#27106=CARTESIAN_POINT ( 'NONE',  ( 163.3471839416382352, 247.7213734702205841, 8.361547422486792058 ) ) ;
#27108=CARTESIAN_POINT ( 'NONE',  ( 159.6023402823087451, 258.6676503891110883, 17.43025742997651761 ) ) ;
#27109=CARTESIAN_POINT ( 'NONE',  ( 171.1200255626874593, 267.0209532845146896, -16.45006463731995083 ) ) ;
#27114=CARTESIAN_POINT ( 'NONE',  ( 165.5977178541590149, 269.2419187492577635, -16.64600468838175473 ) ) ;
#27115=B_SPLINE_SURFACE_WITH_KNOTS ( 'NONE', 3, 1, ( 
 ( #36954, #68846 ),
 ( #54130, #53641 ),
 ( #37441, #68351 ),
 ( #29859, #60729 ),
 ( #69354, #100273 ),
 ( #7052, #30358 ),
 ( #30858, #53156 ),
 ( #91691, #76472 ),
 ( #22254, #84112 ),
 ( #14664, #45540 ),
 ( #46031, #46536 ),
 ( #37933, #75475 ),
 ( #98787, #99767 ),
 ( #8067, #61243 ),
 ( #92209, #22764 ),
 ( #77473, #7548 ),
 ( #61743, #15134 ),
 ( #92692, #21756 ),
 ( #38942, #98283 ),
 ( #83598, #28871 ),
 ( #59747, #60235 ),
 ( #21273, #52150 ),
 ( #83099, #44542 ),
 ( #6060, #67865 ),
 ( #29369, #91196 ),
 ( #18164, #54634 ),
 ( #70349, #93185 ),
 ( #78474, #55631 ),
 ( #1964, #8563 ),
 ( #77968, #48563 ),
 ( #32849, #23740 ),
 ( #71877, #40930 ),
 ( #31837, #460 ),
 ( #71375, #16652 ) ),
 .UNSPECIFIED., .T., .F., .F.,
 ( 4, 2, 2, 2, 2, 2, 2, 2, 2, 2, 2, 2, 2, 2, 2, 2, 4 ),
 ( 2, 2 ),
 ( 0.000000000000000000, 0.06250000000000000000, 0.1250000000000000000, 0.1875000000000000000, 0.2500000000000000000, 0.3125000000000000000, 0.3750000000000000000, 0.4375000000000000000, 0.5000000000000000000, 0.5625000000000000000, 0.6250000000000000000, 0.6875000000000000000, 0.7500000000000000000, 0.8125000000000000000, 0.8750000000000000000, 0.9375000000000000000, 1.000000000000000000 ),
 ( 0.000000000000000000, 1.000000000000000000 ),
 .UNSPECIFIED. ) ;
#27118=CARTESIAN_POINT ( 'NONE',  ( 185.7140529529728497, 297.0115757928315361, 5.550365566574654963 ) ) ;
#27120=CARTESIAN_POINT ( 'NONE',  ( 149.6056361282314811, 276.8836032498194868, -0.0001402111935095534635 ) ) ;
#27122=( BOUNDED_CURVE ( )  B_SPLINE_CURVE ( 2, ( #86964, #49900, #3811, #96541, #94535, #55476, #86462, #16987, #71219 ),
 .UNSPECIFIED., .F., .T. ) 
 B_SPLINE_CURVE_WITH_KNOTS ( ( 3, 2, 2, 2, 3 ),
 ( 0.9153225806451612545, 0.9166666666666666297, 0.9193548387096773800, 0.9220430107526881303, 0.9233870967741935054 ),
 .UNSPECIFIED. ) 
 CURVE ( )  GEOMETRIC_REPRESENTATION_ITEM ( )  RATIONAL_B_SPLINE_CURVE ( ( 0.9330127018922194093, 0.9330127018922194093, 1.000000000000000000, 0.8660254037844387076, 1.000000000000000000, 0.8660254037844387076, 1.000000000000000000, 0.9330127018922194093, 0.9330127018922194093 ) ) 
 REPRESENTATION_ITEM ( '' )  );
#27124=CARTESIAN_POINT ( 'NONE',  ( 194.4430534426562076, 282.9522031543310732, 17.75811852729254881 ) ) ;
#27126=CARTESIAN_POINT ( 'NONE',  ( 173.8384530544828408, 272.7721218975195825, -16.35919102464103148 ) ) ;
#27127=VERTEX_POINT ( 'NONE', #27782 ) ;
#27128=CARTESIAN_POINT ( 'NONE',  ( 162.4683961769543146, 253.1913979656618778, 14.82777648277118310 ) ) ;
#27129=CARTESIAN_POINT ( 'NONE',  ( 194.2154056360670040, 294.2560451561701029, -15.66696967429384557 ) ) ;
#27132=DIRECTION ( 'NONE',  ( 0.4999999999999998890, -0.8660254037844385966, 0.000000000000000000 ) ) ;
#27133=CARTESIAN_POINT ( 'NONE',  ( -27.42236680055714260, 166.5217562850347406, 1.224646799147364892E-15 ) ) ;
#27135=ORIENTED_EDGE ( 'NONE', *, *, #49370, .F. ) ;
#27136=CARTESIAN_POINT ( 'NONE',  ( 84.66726058227095564, 213.5643266524159856, 9.188101187500095079 ) ) ;
#27138=CARTESIAN_POINT ( 'NONE',  ( 188.6826127332440421, 272.6057162039079458, 16.71479996418005243 ) ) ;
#27139=CARTESIAN_POINT ( 'NONE',  ( 182.2345731410963197, 257.9208214993698220, -5.932519869942172619 ) ) ;
#27143=ORIENTED_EDGE ( 'NONE', *, *, #38385, .T. ) ;
#27146=CARTESIAN_POINT ( 'NONE',  ( 206.8711744556208885, 269.6661967102621702, -5.660351959544826712E-12 ) ) ;
#27147=CARTESIAN_POINT ( 'NONE',  ( 154.9067123643522734, 262.3406990819208886, -18.18534662427576265 ) ) ;
#27148=ORIENTED_EDGE ( 'NONE', *, *, #51860, .F. ) ;
#27149=CARTESIAN_POINT ( 'NONE',  ( 164.3614934205162399, 245.9645379182051101, 2.163927203393636312 ) ) ;
#27151=CARTESIAN_POINT ( 'NONE',  ( 151.5945656433808324, 268.6161677518811075, 14.58547821675770351 ) ) ;
#27152=CARTESIAN_POINT ( 'NONE',  ( 162.0103126358019097, 277.3769015859130604, -12.92703519490087594 ) ) ;
#27153=CARTESIAN_POINT ( 'NONE',  ( 153.4542976351440302, 264.8563551865710224, -17.11782692037292009 ) ) ;
#27154=CARTESIAN_POINT ( 'NONE',  ( 182.4502886106904214, 259.6876753163259650, 10.69873880494191631 ) ) ;
#27156=CARTESIAN_POINT ( 'NONE',  ( 132.6770232609233062, 259.6589784336661637, -6.496448406907675876E-16 ) ) ;
#27159=EDGE_CURVE ( 'NONE', #82839, #51615, #35868, .T. ) ;
#27161=CARTESIAN_POINT ( 'NONE',  ( 199.9021804882490017, 270.2741479731562322, 9.563714619189552124 ) ) ;
#27163=CARTESIAN_POINT ( 'NONE',  ( -5.122212653107841795, 179.3967562850347406, 2.649461200531984646E-14 ) ) ;
#27166=CARTESIAN_POINT ( 'NONE',  ( 154.5051885171875483, 277.5048442334672245, 7.163368614392425116 ) ) ;
#27167=CARTESIAN_POINT ( 'NONE',  ( 165.3147752961083938, 246.7756614015693231, -1.872181691986823271 ) ) ;
#27168=CARTESIAN_POINT ( 'NONE',  ( 192.6435868206044972, 292.3535262516610373, -14.36478698284807365 ) ) ;
#27176=CARTESIAN_POINT ( 'NONE',  ( 164.0069374096083550, 277.9889559920678153, 13.17848772514222411 ) ) ;
#27177=CARTESIAN_POINT ( 'NONE',  ( 156.7704915376250767, 276.6929587230139873, 10.09098372363049201 ) ) ;
#27178=CARTESIAN_POINT ( 'NONE',  ( 203.7728381401813920, 277.7020864691337465, -14.30591445410113494 ) ) ;
#27179=CARTESIAN_POINT ( 'NONE',  ( 149.1903793729515257, 272.2416782560088677, 12.95958987445043675 ) ) ;
#27181=CARTESIAN_POINT ( 'NONE',  ( 163.5827852761539987, 273.8567145120941291, 14.80360896856500119 ) ) ;
#27184=CARTESIAN_POINT ( 'NONE',  ( 66.61587002248265321, 199.2677522451418213, -5.000000000000041744 ) ) ;
#27190=CARTESIAN_POINT ( 'NONE',  ( 192.2943420783192323, 297.5834248427583475, 12.53393473147773562 ) ) ;
#27193=LINE ( 'NONE', #65181, #62793 ) ;
#27194=CARTESIAN_POINT ( 'NONE',  ( 16.49491010205593255, 171.1423013555409796, -4.594050593750043987 ) ) ;
#27195=CARTESIAN_POINT ( 'NONE',  ( 97.06207562605321471, 226.8458772461660544, 9.188101187500095079 ) ) ;
#27196=CARTESIAN_POINT ( 'NONE',  ( 154.9903553346911735, 262.1958252075976361, -18.39016733948542637 ) ) ;
#27198=CARTESIAN_POINT ( 'NONE',  ( 186.2747105596910444, 296.7709437567457940, -7.332267729565418612 ) ) ;
#27202=DIRECTION ( 'NONE',  ( -0.8660254037844387076, -0.4999999999999998890, -0.000000000000000000 ) ) ;
#27203=CARTESIAN_POINT ( 'NONE',  ( 148.0826818691893152, 274.1602666119424043, -9.371267383421741926 ) ) ;
#27209=CARTESIAN_POINT ( 'NONE',  ( 88.77168660263453148, 215.3927522451417929, -10.00000000000009237 ) ) ;
#27212=CARTESIAN_POINT ( 'NONE',  ( 173.7468028372802564, 264.4725572781864003, -15.47520981000551465 ) ) ;
#27215=CARTESIAN_POINT ( 'NONE',  ( 87.26533679362427165, 215.0643266524160140, 9.188101187500095079 ) ) ;
#27216=CARTESIAN_POINT ( 'NONE',  ( 207.1007598919583472, 271.9379569114424271, -6.086525981869248092 ) ) ;
#27218=CYLINDRICAL_SURFACE ( 'NONE', #96744, 17.82106496071139645 ) ;
#27219=CARTESIAN_POINT ( 'NONE',  ( 195.7617614321055157, 291.5776783508526364, 16.33009124109666033 ) ) ;
#27220=CARTESIAN_POINT ( 'NONE',  ( 151.9006048953203276, 267.5474299512962943, 16.88304673825244251 ) ) ;
#27221=CARTESIAN_POINT ( 'NONE',  ( 199.1944722252943905, 285.6320488493591938, -18.17555833707144686 ) ) ;
#27222=CARTESIAN_POINT ( 'NONE',  ( 22.78591565582352985, 172.4155109091896065, 2.679491924311254714 ) ) ;
#27226=ORIENTED_EDGE ( 'NONE', *, *, #31318, .F. ) ;
#27230=CARTESIAN_POINT ( 'NONE',  ( 188.1715415252454875, 286.2139794281218315, -16.72207616993653545 ) ) ;
#27234=CARTESIAN_POINT ( 'NONE',  ( 120.0388121219830282, 250.1115022471903160, -5.000000000000047962 ) ) ;
#27235=CARTESIAN_POINT ( 'NONE',  ( 205.2937235227012707, 275.0678357141204629, -12.80017165135291535 ) ) ;
#27239=CARTESIAN_POINT ( 'NONE',  ( 168.5988957253557601, 248.5132396387117524, -1.885179999880600477 ) ) ;
#27240=ORIENTED_EDGE ( 'NONE', *, *, #62157, .F. ) ;
#27241=CARTESIAN_POINT ( 'NONE',  ( 163.3854574543125580, 247.6550818016845597, 10.82482370245618775 ) ) ;
#27247=CARTESIAN_POINT ( 'NONE',  ( 192.7167908629638760, 292.2639303239059814, 15.02160790781813660 ) ) ;
#27248=CARTESIAN_POINT ( 'NONE',  ( 158.3286757630593513, 256.4136846137193970, 16.79716696587219005 ) ) ;
#27256=CARTESIAN_POINT ( 'NONE',  ( 164.5789468726506470, 274.5585074141254722, 14.69886960705206569 ) ) ;
#27262=CARTESIAN_POINT ( 'NONE',  ( 147.6054094044680198, 274.9869267698931594, -8.596541856229405809 ) ) ;
#27264=CARTESIAN_POINT ( 'NONE',  ( 154.9910882912764123, 262.1945556895526579, 18.38052604520346023 ) ) ;
#27265=CARTESIAN_POINT ( 'NONE',  ( 147.4771028564622100, 275.6046161191591182, 9.141179566768406735E-14 ) ) ;
#27267=CARTESIAN_POINT ( 'NONE',  ( 208.0730008398676318, 270.2539861924646516, -3.911917750280078376 ) ) ;
#27271=CARTESIAN_POINT ( 'NONE',  ( 108.5912123618160763, 227.3768266524159856, -9.188101187500091527 ) ) ;
#27272=VERTEX_POINT ( 'NONE', #38851 ) ;
#27274=CARTESIAN_POINT ( 'NONE',  ( 166.5201100233303464, 278.0365861635631859, -13.36835105817650060 ) ) ;
#27279=CARTESIAN_POINT ( 'NONE',  ( 177.4333559188052050, 292.4950673467274669, -2.688042529096076994 ) ) ;
#27280=CARTESIAN_POINT ( 'NONE',  ( 157.0957870390718369, 258.5491105237443321, 17.69218919045495397 ) ) ;
#27282=CARTESIAN_POINT ( 'NONE',  ( 163.1968603775171118, 247.9817415208531202, 11.27455733958931994 ) ) ;
#27283=CARTESIAN_POINT ( 'NONE',  ( 92.46148921633090367, 218.0643266524160140, 9.188101187500095079 ) ) ;
#27284=ORIENTED_EDGE ( 'NONE', *, *, #60291, .F. ) ;
#27286=ORIENTED_EDGE ( 'NONE', *, *, #40095, .F. ) ;
#27290=CARTESIAN_POINT ( 'NONE',  ( 191.5793115159691524, 263.6492056449409347, -8.156572570947284717 ) ) ;
#27291=CARTESIAN_POINT ( 'NONE',  ( 154.2194984598485519, 265.5309884801890234, 17.12742652472672944 ) ) ;
#27293=CARTESIAN_POINT ( 'NONE',  ( 137.1700506867025808, 243.8768266524160140, -9.188101187500091527 ) ) ;
#27295=CARTESIAN_POINT ( 'NONE',  ( -10.09954699608895901, 171.6427522451419350, -10.00000000000009415 ) ) ;
#27296=CARTESIAN_POINT ( 'NONE',  ( 171.3840324641641359, 249.8316075428874683, -4.467467663849890691 ) ) ;
#27298=CARTESIAN_POINT ( 'NONE',  ( 204.5840280042472159, 276.2970644099866036, 14.65559382949596667 ) ) ;
#27300=CARTESIAN_POINT ( 'NONE',  ( 93.60468337831817109, 236.3967562850347122, -4.648177544792955347E-16 ) ) ;
#27301=CARTESIAN_POINT ( 'NONE',  ( 188.8377537886989899, 269.5936382258537378, 14.70355276031261660 ) ) ;
#27302=CARTESIAN_POINT ( 'NONE',  ( 178.4489778659152250, 285.3664758674125892, 13.08110770347619400 ) ) ;
#27304=CARTESIAN_POINT ( 'NONE',  ( 198.4446623809833170, 281.5023889509741934, -16.57120230699170094 ) ) ;
#27305=CARTESIAN_POINT ( 'NONE',  ( 122.1835217032046330, 252.8967562850346553, -4.648177544792955347E-16 ) ) ;
#27309=CARTESIAN_POINT ( 'NONE',  ( 167.8014687349847520, 250.0213847097312225, 6.957476650644477623 ) ) ;
#27311=CARTESIAN_POINT ( 'NONE',  ( 208.3682389855799499, 269.7426187237583690, -1.431169231381201890 ) ) ;
#27319=CARTESIAN_POINT ( 'NONE',  ( 180.0662822340164269, 262.4007578510376675, -14.24330825748563534 ) ) ;
#27323=( NAMED_UNIT ( * ) PLANE_ANGLE_UNIT ( ) SI_UNIT ( $, .RADIAN. ) );
#27324=CARTESIAN_POINT ( 'NONE',  ( 158.3644695203838069, 271.4464815599769167, -14.70628431356059451 ) ) ;
#27325=CARTESIAN_POINT ( 'NONE',  ( 205.7872507830675204, 272.2130214242461079, -9.506855900917111413 ) ) ;
#27326=CARTESIAN_POINT ( 'NONE',  ( 207.1432938686257046, 271.8642859028066141, -6.405155839440290322 ) ) ;
#27327=CARTESIAN_POINT ( 'NONE',  ( 10.89220085373657376, 189.3464784336661353, 1.353441290958777327E-15 ) ) ;
#27328=CARTESIAN_POINT ( 'NONE',  ( 207.0320938795157417, 270.2489720413080363, 3.395226072341499979 ) ) ;
#27329=EDGE_LOOP ( 'NONE', ( #29831, #49510, #86746, #90320 ) ) ;
#27332=CARTESIAN_POINT ( 'NONE',  ( -22.42236680055709641, 157.8615022471902591, 0.000000000000000000 ) ) ;
#27334=CARTESIAN_POINT ( 'NONE',  ( 41.20343708195693466, 194.5958772461660544, -9.188101187500095079 ) ) ;
#27336=CARTESIAN_POINT ( 'NONE',  ( 161.7910648966377209, 250.4166507187868831, 13.19274492748169436 ) ) ;
#27337=CARTESIAN_POINT ( 'NONE',  ( 146.9324727656309335, 276.1524872186338371, 3.813717745456558728 ) ) ;
#27340=CARTESIAN_POINT ( 'NONE',  ( 191.0702043019150835, 299.7036936669546776, -8.800021049343948576 ) ) ;
#27341=CARTESIAN_POINT ( 'NONE',  ( 177.1262862392189845, 269.6057104283654553, 17.56656865388298172 ) ) ;
#27345=CARTESIAN_POINT ( 'NONE',  ( 78.46959274033001464, 216.1115022471902591, 10.00000000000009592 ) ) ;
#27346=CARTESIAN_POINT ( 'NONE',  ( 50.34412104557527812, 188.3262482093458061, 3.021315404115420679E-15 ) ) ;
#27348=ORIENTED_EDGE ( 'NONE', *, *, #42979, .T. ) ;
#27349=CARTESIAN_POINT ( 'NONE',  ( 43.96371950863733247, 202.3149278399160949, -9.188101187500095079 ) ) ;
#27352=CARTESIAN_POINT ( 'NONE',  ( 151.1126408083691501, 268.9122237844355254, -15.82705194100464396 ) ) ;
#27354=ORIENTED_EDGE ( 'NONE', *, *, #91967, .F. ) ;
#27355=CARTESIAN_POINT ( 'NONE',  ( 171.3214800902178467, 286.5990332881968357, 8.223688229099183289 ) ) ;
#27356=CARTESIAN_POINT ( 'NONE',  ( 164.4858674010174298, 245.7491158648375347, -2.958464974013825355 ) ) ;
#27359=CARTESIAN_POINT ( 'NONE',  ( 189.4145974059905200, 265.0249961711397191, 10.45958848644401407 ) ) ;
#27361=CARTESIAN_POINT ( 'NONE',  ( 171.6881850446922613, 255.8132376700287125, 11.22435778083355196 ) ) ;
#27365=CARTESIAN_POINT ( 'NONE',  ( 174.8451195330017640, 255.1849038048701459, 8.216676969017473908 ) ) ;
#27366=DIRECTION ( 'NONE',  ( 0.8660254037844395958, 0.4999999999999985567, 0.000000000000000000 ) ) ;
#27369=CARTESIAN_POINT ( 'NONE',  ( 150.7226148805041817, 269.5877685077668957, 15.52819754351937576 ) ) ;
#27372=CARTESIAN_POINT ( 'NONE',  ( 161.7412967960748915, 250.5028515975580774, -14.36228887024421041 ) ) ;
#27374=ORIENTED_EDGE ( 'NONE', *, *, #81348, .F. ) ;
#27376=VECTOR ( 'NONE', #47333, 1000.000000000000000 ) ;
#27377=CARTESIAN_POINT ( 'NONE',  ( 198.3075590527773784, 287.1682275260610027, 16.94807365630277118 ) ) ;
#27380=CARTESIAN_POINT ( 'NONE',  ( 197.9813997048801184, 286.8186411885521920, 16.94230379787914131 ) ) ;
#27381=CARTESIAN_POINT ( 'NONE',  ( 116.3579438323015012, 247.1744531367911293, 4.594050593750047540 ) ) ;
#27383=CARTESIAN_POINT ( 'NONE',  ( 150.7530568467738590, 269.5350414755053521, 15.60317050893315916 ) ) ;
#27384=B_SPLINE_CURVE_WITH_KNOTS ( 'NONE', 3,
 ( #49496, #17607, #48516, #2425, #56600, #80452, #87586, #11024, #30927, #26706, #84668, #15211, #38517, #69428, #50003, #58579, #73803, #50487, #59573, #82459, #19131, #44381, #34786, #19628, #66690, #5894, #27212, #96644, #58096, #89552, #90036, #36287, #80959, #42870, #51491, #51996, #75313, #50985, #81935, #73315, #74327, #3906, #12513, #82937, #81442, #21119, #74824, #13022, #12013, #90548, #89079, #11524 ),
 .UNSPECIFIED., .F., .F.,
 ( 4, 2, 2, 2, 2, 2, 2, 2, 2, 2, 2, 2, 2, 2, 2, 2, 2, 2, 2, 2, 2, 2, 2, 2, 2, 4 ),
 ( 0.0008917468271082998289, 0.001373251144630191749, 0.001854755462152083562, 0.002095507620913045297, 0.002336259779674007466, 0.002456635859054485515, 0.002577011938434963564, 0.002697388017815441179, 0.002817764097195919228, 0.003058516255956880096, 0.003299268414717840964, 0.003780772732239826017, 0.004743781367283867248, 0.005706790002327906744, 0.006188294319849931696, 0.006669798637371957516, 0.006790174716752526637, 0.006850362756442810765, 0.006910550796133095759, 0.007030926875513786312, 0.007151302954894477731, 0.007392055113655964654, 0.007632807272417452445, 0.007873559431178938500, 0.008114311589940425423, 0.008595815907463411412 ),
 .UNSPECIFIED. ) ;
#27385=CARTESIAN_POINT ( 'NONE',  ( -22.42236680055709641, 157.8615022471902591, 0.000000000000000000 ) ) ;
#27389=AXIS2_PLACEMENT_3D ( 'NONE', #21924, #22425, #63789 ) ;
#27390=CARTESIAN_POINT ( 'NONE',  ( 163.7012083107868534, 247.1081852757374975, -6.544933039329257518 ) ) ;
#27391=EDGE_LOOP ( 'NONE', ( #39646, #18140, #78107, #42679 ) ) ;
#27393=CARTESIAN_POINT ( 'NONE',  ( 160.0072461633487535, 253.5063153963366744, 16.23938890643736244 ) ) ;
#27396=CARTESIAN_POINT ( 'NONE',  ( 76.87303194821102181, 209.0643266524160424, 9.188101187500095079 ) ) ;
#27397=ORIENTED_EDGE ( 'NONE', *, *, #82167, .T. ) ;
#27398=CARTESIAN_POINT ( 'NONE',  ( 170.7667195423792066, 283.6621974811555447, 12.84944695255637548 ) ) ;
#27399=CARTESIAN_POINT ( 'NONE',  ( 150.6571681785161445, 269.7011255207979730, 15.24894850018880454 ) ) ;
#27400=CARTESIAN_POINT ( 'NONE',  ( 193.8603219414924013, 294.8710681561126989, 15.36476279452078586 ) ) ;
#27401=CARTESIAN_POINT ( 'NONE',  ( 171.9660161825155171, 276.8101763654939305, 16.40752538293672202 ) ) ;
#27402=ORIENTED_EDGE ( 'NONE', *, *, #41723, .T. ) ;
#27408=ORIENTED_EDGE ( 'NONE', *, *, #15045, .T. ) ;
#27409=CARTESIAN_POINT ( 'NONE',  ( 147.9235661301700304, 274.4358631562076880, 9.736478568371106590 ) ) ;
#27412=CARTESIAN_POINT ( 'NONE',  ( 161.2133744761260061, 251.4172398781588811, -14.30368667312104058 ) ) ;
#27413=CARTESIAN_POINT ( 'NONE',  ( 206.4894746850401077, 270.6312975806551435, 2.443363978982824758 ) ) ;
#27414=CARTESIAN_POINT ( 'NONE',  ( 199.6930299107040412, 283.1861613635016397, -17.43055490872784574 ) ) ;
#27415=CARTESIAN_POINT ( 'NONE',  ( 176.9054780674279073, 269.9821856685988450, 16.79845386343675173 ) ) ;
#27417=CARTESIAN_POINT ( 'NONE',  ( 165.0297293518065658, 244.8071193337670195, 2.517333243890161665 ) ) ;
#27418=CARTESIAN_POINT ( 'NONE',  ( 132.9389821956409037, 240.8927522451417929, -10.00000000000009237 ) ) ;
#27419=CARTESIAN_POINT ( 'NONE',  ( 167.6768863921620039, 256.3367762910957026, 13.59289973228994342 ) ) ;
#27420=CARTESIAN_POINT ( 'NONE',  ( 8.231324050681719129, 168.8927522451417929, -10.00000000000009237 ) ) ;
#27421=B_SPLINE_CURVE_WITH_KNOTS ( 'NONE', 3,
 ( #3202, #2184, #41147, #63961, #49275, #34086, #81211, #87355, #17363, #64976, #80212, #55835, #72597, #94903, #26973, #88331, #57855, #2686 ),
 .UNSPECIFIED., .F., .F.,
 ( 4, 2, 2, 2, 2, 2, 2, 2, 4 ),
 ( 0.003270768999366409358, 0.003375574448574713074, 0.003480379897783016357, 0.003585185346991320073, 0.003689990796199623790, 0.003899601694616248136, 0.004109212593032872049, 0.004947656186699188156, 0.006624543374031750115 ),
 .UNSPECIFIED. ) ;
#27422=CARTESIAN_POINT ( 'NONE',  ( 133.4083396129551602, 238.6423013555409796, -4.594050593750043987 ) ) ;
#27426=CARTESIAN_POINT ( 'NONE',  ( 205.8278679583572739, 273.7726763696764465, -10.01757226791932176 ) ) ;
#27428=( BOUNDED_CURVE ( )  B_SPLINE_CURVE ( 2, ( #19815, #13213, #74013, #75505, #89265 ),
 .UNSPECIFIED., .F., .T. ) 
 B_SPLINE_CURVE_WITH_KNOTS ( ( 3, 2, 3 ),
 ( 0.000000000000000000, 0.002688172043010752903, 0.004032258064516129788 ),
 .UNSPECIFIED. ) 
 CURVE ( )  GEOMETRIC_REPRESENTATION_ITEM ( )  RATIONAL_B_SPLINE_CURVE ( ( 1.000000000000000000, 0.8660254037844387076, 1.000000000000000000, 0.9330127018922194093, 0.9330127018922194093 ) ) 
 REPRESENTATION_ITEM ( '' )  );
#27434=CARTESIAN_POINT ( 'NONE',  ( 166.2052710271649687, 248.2504166283805489, -5.515680059214410846 ) ) ;
#27435=CARTESIAN_POINT ( 'NONE',  ( 147.6576679470944384, 275.6425429203924296, 2.820251122944001487 ) ) ;
#27438=DIRECTION ( 'NONE',  ( -0.4999999999999987788, 0.8660254037844392627, 0.000000000000000000 ) ) ;
#27441=CARTESIAN_POINT ( 'NONE',  ( 204.8385597977314490, 275.8562024115307167, -12.64672659107585240 ) ) ;
#27442=CARTESIAN_POINT ( 'NONE',  ( 170.6631332514753581, 250.4690807168623508, 3.666193302703367962 ) ) ;
#27445=CARTESIAN_POINT ( 'NONE',  ( 149.6877696051026305, 271.3801731027346591, 11.89134584187677390 ) ) ;
#27447=CARTESIAN_POINT ( 'NONE',  ( 169.4870084614010750, 285.2172692466178319, -7.974559327038013734 ) ) ;
#27448=CARTESIAN_POINT ( 'NONE',  ( 198.2489255580726422, 287.2697837179150042, 18.53597557040773225 ) ) ;
#27449=CARTESIAN_POINT ( 'NONE',  ( 149.0244553356880886, 274.5290671187512999, 9.114935767028397251 ) ) ;
#27450=EDGE_CURVE ( 'NONE', #8803, #99288, #71203, .T. ) ;
#27451=CARTESIAN_POINT ( 'NONE',  ( 132.0007880082076781, 257.0177522451418781, 5.000000000000046185 ) ) ;
#27452=CARTESIAN_POINT ( 'NONE',  ( 172.2607799805669515, 283.9270791244886141, -12.74676459771014336 ) ) ;
#27454=B_SPLINE_CURVE_WITH_KNOTS ( 'NONE', 3,
 ( #55677, #2011, #17716, #32897 ),
 .UNSPECIFIED., .F., .F.,
 ( 4, 4 ),
 ( 0.003210172446339780092, 0.008633305421422422105 ),
 .UNSPECIFIED. ) ;
#27456=EDGE_CURVE ( 'NONE', #85402, #26873, #86454, .T. ) ;
#27457=CARTESIAN_POINT ( 'NONE',  ( 196.4982648257524147, 290.3020170531091821, 16.69353242256149628 ) ) ;
#27458=CARTESIAN_POINT ( 'NONE',  ( 148.3280470635002928, 273.7352816289870248, 9.058704604771318003 ) ) ;
#27459=CARTESIAN_POINT ( 'NONE',  ( -7.619092152155813480, 178.6589784336661637, -6.496448406907676862E-16 ) ) ;
#27460=CARTESIAN_POINT ( 'NONE',  ( 41.01373370305532973, 203.6744531367911293, 4.594050593750047540 ) ) ;
#27462=CARTESIAN_POINT ( 'NONE',  ( 178.6059155966152048, 259.3514611767804467, -10.88062025991058235 ) ) ;
#27465=CARTESIAN_POINT ( 'NONE',  ( 157.0887340267001946, 258.5613266995183039, -17.61824281915036394 ) ) ;
#27466=CARTESIAN_POINT ( 'NONE',  ( 192.5757274456924222, 292.4492253229388439, -14.29994009178870940 ) ) ;
#27471=CARTESIAN_POINT ( 'NONE',  ( 68.70876474829495351, 217.1427522451419065, 10.00000000000009415 ) ) ;
#27474=CARTESIAN_POINT ( 'NONE',  ( 163.3071340352992991, 277.0811303350653247, 14.49351327170118431 ) ) ;
#27476=CARTESIAN_POINT ( 'NONE',  ( 39.49844957003023893, 203.6115022471903160, -5.000000000000047962 ) ) ;
#27477=CARTESIAN_POINT ( 'NONE',  ( 181.7453103611686629, 291.7118052563983497, 9.176684814609201268 ) ) ;
#27478=CARTESIAN_POINT ( 'NONE',  ( 202.9689790241539242, 279.0944113002206564, 15.85114608332523289 ) ) ;
#27479=CARTESIAN_POINT ( 'NONE',  ( 1.717831006336420607, 180.9869531367911293, 4.594050593750046652 ) ) ;
#27480=CARTESIAN_POINT ( 'NONE',  ( 165.2814945196670919, 284.9282336261690034, 4.158235161442515704 ) ) ;
#27481=CARTESIAN_POINT ( 'NONE',  ( 153.3100492430090753, 265.1062007306585997, 16.32434963471121492 ) ) ;
#27483=CARTESIAN_POINT ( 'NONE',  ( 165.0538309624641613, 244.7653741195639157, 2.311334310144196547 ) ) ;
#27484=CARTESIAN_POINT ( 'NONE',  ( 164.5416088356626290, 245.6525688679454618, -1.463507744092769292 ) ) ;
#27486=DIRECTION ( 'NONE',  ( -0.8660254037844387076, -0.4999999999999998890, -0.000000000000000000 ) ) ;
#27489=CARTESIAN_POINT ( 'NONE',  ( 126.8249895137406043, 232.4824982072973683, 3.021315404115420679E-15 ) ) ;
#27493=CARTESIAN_POINT ( 'NONE',  ( 152.7050834466765536, 278.6643962355284998, -4.749106930788815184 ) ) ;
#27494=ORIENTED_EDGE ( 'NONE', *, *, #98548, .F. ) ;
#27496=CARTESIAN_POINT ( 'NONE',  ( 181.4735074999749145, 292.1586133693310785, 10.55809797880889001 ) ) ;
#27498=VERTEX_POINT ( 'NONE', #7976 ) ;
#27499=CARTESIAN_POINT ( 'NONE',  ( 192.8010417052266234, 296.7057953447782097, 12.10593424093686643 ) ) ;
#27505=CARTESIAN_POINT ( 'NONE',  ( 164.2709363216550855, 246.8183101628254406, -5.373927384795599949 ) ) ;
#27507=CARTESIAN_POINT ( 'NONE',  ( 192.8323852661406761, 296.6515067047851062, 11.86505947732313615 ) ) ;
#27510=CARTESIAN_POINT ( 'NONE',  ( 174.4445693293744455, 262.3909980173429517, 14.47875634103648856 ) ) ;
#27518=CARTESIAN_POINT ( 'NONE',  ( 159.5541294036357840, 254.7329949101089142, -15.49503750354262088 ) ) ;
#27519=CARTESIAN_POINT ( 'NONE',  ( 169.2920866366192456, 276.4291702812190579, -16.06723518864265188 ) ) ;
#27522=CARTESIAN_POINT ( 'NONE',  ( 174.4842243494688034, 276.9690305039630971, -15.77146616506232668 ) ) ;
#27523=CARTESIAN_POINT ( 'NONE',  ( 171.1204324191836292, 262.9359187872178154, -15.53146915371453929 ) ) ;
#27526=DIRECTION ( 'NONE',  ( 0.4999999999999998890, -0.8660254037844385966, 0.000000000000000000 ) ) ;
#27530=CARTESIAN_POINT ( 'NONE',  ( 169.0163292910675636, 272.4602990133035405, 17.15131738099888636 ) ) ;
#27531=CARTESIAN_POINT ( 'NONE',  ( 193.2864259971985916, 295.8650850898874296, 14.21409792694320551 ) ) ;
#27532=CARTESIAN_POINT ( 'NONE',  ( 188.6635337462180928, 298.6204119622300368, -4.269177026095916538 ) ) ;
#27534=CARTESIAN_POINT ( 'NONE',  ( 192.0523540417460993, 298.0025604169266558, 12.03387399082417275 ) ) ;
#27535=EDGE_CURVE ( 'NONE', #10970, #27272, #81576, .T. ) ;
#27537=CARTESIAN_POINT ( 'NONE',  ( 178.5255977161920669, 291.5666061038359089, 6.170387333470672253 ) ) ;
#27538=CARTESIAN_POINT ( 'NONE',  ( 196.9669828711821538, 289.4901735840007291, -17.16750406591627254 ) ) ;
#27541=CARTESIAN_POINT ( 'NONE',  ( 151.2546443255573934, 275.3395117651207897, -9.775857568146751220 ) ) ;
#27544=CARTESIAN_POINT ( 'NONE',  ( 159.4889735931715222, 254.4039898200529706, 16.88104032092801887 ) ) ;
#27546=B_SPLINE_CURVE_WITH_KNOTS ( 'NONE', 3,
 ( #1785, #2292, #62042, #55938 ),
 .UNSPECIFIED., .F., .F.,
 ( 4, 4 ),
 ( 0.009717938389684965469, 0.01571428049324324894 ),
 .UNSPECIFIED. ) ;
#27547=ORIENTED_EDGE ( 'NONE', *, *, #21783, .T. ) ;
#27548=CARTESIAN_POINT ( 'NONE',  ( 147.3572860122106647, 275.4166890918294825, -2.824341378914994038 ) ) ;
#27549=CARTESIAN_POINT ( 'NONE',  ( 199.0837164482014714, 266.3850903537827435, 6.043064621626092148 ) ) ;
#27550=CARTESIAN_POINT ( 'NONE',  ( 164.1954676172330210, 247.3737367566268972, 7.269074065105377791 ) ) ;
#27552=CARTESIAN_POINT ( 'NONE',  ( 125.1447535615809414, 236.3927522451417929, -10.00000000000009237 ) ) ;
#27553=EDGE_CURVE ( 'NONE', #12202, #13902, #29511, .T. ) ;
#27554=CARTESIAN_POINT ( 'NONE',  ( 198.6245008644510222, 286.6192682051993188, -17.88211844573111975 ) ) ;
#27555=CARTESIAN_POINT ( 'NONE',  ( 91.12263257074930323, 234.9637435831424739, 2.679491924311251605 ) ) ;
#27558=CARTESIAN_POINT ( 'NONE',  ( 167.2506521577460603, 252.9623063650430197, -12.17192564457983828 ) ) ;
#27560=CARTESIAN_POINT ( 'NONE',  ( 134.5031927440161326, 236.9155109091896065, 2.679491924311254714 ) ) ;
#27561=CARTESIAN_POINT ( 'NONE',  ( 207.0200405408487541, 272.0777669287182334, 6.494273599193515878 ) ) ;
#27562=CARTESIAN_POINT ( 'NONE',  ( 34.06774859691749668, 177.1427522451417360, 1.119607411625061291E-15 ) ) ;
#27563=CARTESIAN_POINT ( 'NONE',  ( 103.3950599391094443, 224.3768266524160140, -9.188101187500093303 ) ) ;
#27564=CARTESIAN_POINT ( 'NONE',  ( 180.8406542025288388, 294.1182405763964880, -2.664013851607027306 ) ) ;
#27565=CARTESIAN_POINT ( 'NONE',  ( 167.5023760217605400, 281.6905759989244871, -10.92128487528961678 ) ) ;
#27567=LINE ( 'NONE', #67031, #36908 ) ;
#27568=CARTESIAN_POINT ( 'NONE',  ( 20.95974617273066443, 195.1589784336661637, -6.496448406907675876E-16 ) ) ;
#27569=CARTESIAN_POINT ( 'NONE',  ( 200.7897860911934913, 282.8688841796032420, 18.17522996445731920 ) ) ;
#27570=ORIENTED_EDGE ( 'NONE', *, *, #13843, .T. ) ;
#27576=CARTESIAN_POINT ( 'NONE',  ( -22.42236680055709641, 157.8615022471902591, 0.000000000000000000 ) ) ;
#27577=DIRECTION ( 'NONE',  ( 0.5000000000000007772, -0.8660254037844381525, 0.000000000000000000 ) ) ;
#27578=CARTESIAN_POINT ( 'NONE',  ( 182.4011669864173086, 284.2493615651014238, 14.92779187816798547 ) ) ;
#27581=CARTESIAN_POINT ( 'NONE',  ( 47.75258065019424691, 204.5024278399160949, 9.188101187500095079 ) ) ;
#27582=CARTESIAN_POINT ( 'NONE',  ( 91.36976281398776223, 236.8927522451419350, 2.944929066748280225E-16 ) ) ;
#27584=CARTESIAN_POINT ( 'NONE',  ( 198.4497957874126257, 267.8821814322857904, -8.033238290564030493 ) ) ;
#27585=EDGE_CURVE ( 'NONE', #17408, #72864, #75456, .T. ) ;
#27586=EDGE_CURVE ( 'NONE', #2810, #70911, #1720, .T. ) ;
#27587=CARTESIAN_POINT ( 'NONE',  ( 2.692369909191673294, 162.3615022471902023, 5.000000000000051514 ) ) ;
#27588=CARTESIAN_POINT ( 'NONE',  ( -4.208943576872074210, 174.5024278399160949, 9.188101187500095079 ) ) ;
#27590=CARTESIAN_POINT ( 'NONE',  ( 150.7850480413316632, 269.4796311011364764, -14.43114374163211089 ) ) ;
#27592=CARTESIAN_POINT ( 'NONE',  ( 193.2053309019613891, 296.0055459150826778, -12.79465285318189061 ) ) ;
#27593=CARTESIAN_POINT ( 'NONE',  ( 164.3545367017254364, 245.9765873086048487, -5.942639963102972267 ) ) ;
#27594=CARTESIAN_POINT ( 'NONE',  ( 204.2143397907769611, 276.5280330293650195, 13.36303585211030054 ) ) ;
#27595=CARTESIAN_POINT ( 'NONE',  ( 186.8003541658358984, 299.2222177555264011, -0.6103433986344138917 ) ) ;
#27596=CARTESIAN_POINT ( 'NONE',  ( 207.4285356523023154, 271.3702326410368642, 7.833982582429932506 ) ) ;
#27598=CARTESIAN_POINT ( 'NONE',  ( -4.235833321083918079, 178.3615022471903160, 5.000000000000046185 ) ) ;
#27600=CARTESIAN_POINT ( 'NONE',  ( 128.8345561752773278, 239.0643266524160140, 9.188101187500095079 ) ) ;
#27602=CARTESIAN_POINT ( 'NONE',  ( 181.0193311394079103, 261.5502185760933003, 13.24438261311760812 ) ) ;
#27603=CARTESIAN_POINT ( 'NONE',  ( 150.9903069161591418, 270.0165872255406612, 13.76682917664489381 ) ) ;
#27606=CARTESIAN_POINT ( 'NONE',  ( 69.66731286396763778, 199.4824982072973967, 3.021315404115420679E-15 ) ) ;
#27608=CARTESIAN_POINT ( 'NONE',  ( 150.6571681785161445, 269.7011255207979730, 15.24894850018880454 ) ) ;
#27609=CARTESIAN_POINT ( 'NONE',  ( 163.4319133527347390, 247.5746178253062055, 7.647903095947664376 ) ) ;
#27610=CARTESIAN_POINT ( 'NONE',  ( 190.6522387254234729, 300.0187146158233986, 3.894424434267832247 ) ) ;
#27613=ORIENTED_EDGE ( 'NONE', *, *, #67126, .F. ) ;
#27616=B_SPLINE_CURVE_WITH_KNOTS ( 'NONE', 3,
 ( #83341, #53874, #84836, #84343, #52894, #13905, #15374, #44786, #60984, #6306, #37197, #45293, #60480, #83846, #76227, #14888, #71620, #64502, #9821, #17914, #16888, #63993, #39665, #95462, #79249, #17392, #40682, #70589 ),
 .UNSPECIFIED., .F., .F.,
 ( 4, 2, 2, 2, 2, 2, 2, 2, 2, 2, 2, 2, 2, 4 ),
 ( 0.0003625531286933231386, 0.002366764927985090181, 0.002867817877808072260, 0.002993081115263782760, 0.003024396924627741935, 0.003055712733991701111, 0.003087028543355660286, 0.003118344352719619461, 0.003243607590175527286, 0.003368870827631435111, 0.003619397302543357446, 0.003869923777455280215, 0.004120450252367202117, 0.004370976727279125319 ),
 .UNSPECIFIED. ) ;
#27618=CARTESIAN_POINT ( 'NONE',  ( 200.1686525782743331, 272.4625969671961343, 12.58813841635031849 ) ) ;
#27619=CARTESIAN_POINT ( 'NONE',  ( 177.7342311040593756, 255.2532439957012684, -8.367404576774948310 ) ) ;
#27622=CARTESIAN_POINT ( 'NONE',  ( 148.5349717444102566, 274.3968686471137630, -7.864641605647691769 ) ) ;
#27624=B_SPLINE_CURVE_WITH_KNOTS ( 'NONE', 3,
 ( #48929, #1833, #2337, #17518, #55990, #25631, #94061, #86988, #24614, #71240, #95069, #48424, #79373, #2849, #9936, #72243, #40799, #79867, #33738, #41301, #95583, #5321, #50905, #12941, #43800, #13430, #65611, #20528, #42303, #81854, #88485, #12430, #36695, #73235, #67103, #19047, #89951, #82859, #28108, #36198, #81367, #28603, #11449, #4832, #3827, #43298, #58015, #58982, #96068, #97064 ),
 .UNSPECIFIED., .F., .F.,
 ( 4, 2, 2, 2, 2, 2, 2, 2, 2, 2, 2, 2, 2, 2, 2, 2, 2, 2, 2, 2, 2, 2, 2, 2, 4 ),
 ( 0.0008219441068872318295, 0.001020485464105246216, 0.001119756142714287616, 0.001219026821323329016, 0.001417568178541411599, 0.001616109535759494183, 0.002013192250195829786, 0.002410274964632165388, 0.003204440393504899044, 0.003998605822377632700, 0.004792771251250365488, 0.005189853965686732316, 0.005388395322904916164, 0.005487666001513965587, 0.005586936680123015010, 0.005636572019427577886, 0.005686207358732140761, 0.005785478037341302074, 0.005984019394559623832, 0.006182560751777944723, 0.006381102108996266481, 0.006579643466214587372, 0.006778184823432909130, 0.006976726180651230021, 0.007175267537869550911 ),
 .UNSPECIFIED. ) ;
#27628=ORIENTED_EDGE ( 'NONE', *, *, #91884, .T. ) ;
#27629=CARTESIAN_POINT ( 'NONE',  ( 171.3751619920873281, 280.2398791927632828, 15.33202389549764888 ) ) ;
#27631=CARTESIAN_POINT ( 'NONE',  ( 194.5298665426430489, 293.7113828889860656, -16.13302716640051315 ) ) ;
#27632=CARTESIAN_POINT ( 'NONE',  ( 156.0746793001935657, 261.9946646095714300, -16.96186522563439780 ) ) ;
#27637=CYLINDRICAL_SURFACE ( 'NONE', #34966, 17.82106496071139645 ) ;
#27639=CARTESIAN_POINT ( 'NONE',  ( 89.24104401994878799, 213.1423013555409796, -4.594050593750043987 ) ) ;
#27642=CARTESIAN_POINT ( 'NONE',  ( 182.0114982784328959, 257.6695253748193863, -5.972343101773933682 ) ) ;
#27646=ORIENTED_EDGE ( 'NONE', *, *, #34322, .T. ) ;
#27650=CARTESIAN_POINT ( 'NONE',  ( 155.5066938333533528, 261.3015006940112244, -18.40036130547566273 ) ) ;
#27656=CARTESIAN_POINT ( 'NONE',  ( 157.4387554167717553, 281.9416217953914270, 2.906349061691626989 ) ) ;
#27657=CARTESIAN_POINT ( 'NONE',  ( 149.7817191771959244, 245.0327760586659451, 1.948934522072303157E-15 ) ) ;
#27658=CARTESIAN_POINT ( 'NONE',  ( -22.42236680055709641, 157.8615022471902591, 0.000000000000000000 ) ) ;
#27662=ORIENTED_EDGE ( 'NONE', *, *, #54652, .T. ) ;
#27663=CARTESIAN_POINT ( 'NONE',  ( 163.9449312135976129, 281.9653101204439736, 8.519335645788913780 ) ) ;
#27664=CARTESIAN_POINT ( 'NONE',  ( 203.6513521002680136, 271.6927919894359320, 9.604818643925334243 ) ) ;
#27667=CYLINDRICAL_SURFACE ( 'NONE', #98222, 10.00000000000010658 ) ;
#27669=CARTESIAN_POINT ( 'NONE',  ( 156.7777268389594667, 279.3827415317243776, 7.395700627148257489 ) ) ;
#27670=EDGE_CURVE ( 'NONE', #76355, #35626, #77712, .T. ) ;
#27672=DIRECTION ( 'NONE',  ( -0.8660254037844392627, -0.4999999999999987232, 0.000000000000000000 ) ) ;
#27673=ADVANCED_FACE ( 'NONE', ( #9868 ), #8837, .T. ) ;
#27677=CARTESIAN_POINT ( 'NONE',  ( 196.9526636073363477, 287.5149752765084941, -17.63101726665603053 ) ) ;
#27680=CARTESIAN_POINT ( 'NONE',  ( 160.5181951850485405, 275.9162642635258749, 12.68197119230242542 ) ) ;
#27685=CARTESIAN_POINT ( 'NONE',  ( 174.5885488454506174, 256.4458599265808516, 12.05082362884263425 ) ) ;
#27687=CARTESIAN_POINT ( 'NONE',  ( 203.6314934253803131, 269.6250664415474034, 5.533663177072089212 ) ) ;
#27688=ORIENTED_EDGE ( 'NONE', *, *, #37760, .T. ) ;
#27691=CARTESIAN_POINT ( 'NONE',  ( 116.9873692804980010, 249.8967562850347122, -4.648177544792955347E-16 ) ) ;
#27693=CARTESIAN_POINT ( 'NONE',  ( 175.2003707602579823, 290.7303100365182331, 2.563854479286836963 ) ) ;
#27694=CARTESIAN_POINT ( 'NONE',  ( 192.7259387352017939, 296.8358775046606297, 11.24705370801146209 ) ) ;
#27697=DIRECTION ( 'NONE',  ( -0.4999999999999987788, 0.8660254037844392627, 0.000000000000000000 ) ) ;
#27698=EDGE_CURVE ( 'NONE', #90703, #2331, #11735, .T. ) ;
#27699=CARTESIAN_POINT ( 'NONE',  ( 13.89683389070260944, 169.6423013555409796, -4.594050593750043987 ) ) ;
#27700=CARTESIAN_POINT ( 'NONE',  ( 94.81556191316359161, 234.7369531367911009, -4.594050593750048428 ) ) ;
#27701=CARTESIAN_POINT ( 'NONE',  ( 202.8874463667715133, 279.2356300052831557, -15.29930322226033468 ) ) ;
#27702=CARTESIAN_POINT ( 'NONE',  ( 36.44700672854521883, 203.3967562850347122, 1.101618078115930403E-13 ) ) ;
#27703=CARTESIAN_POINT ( 'NONE',  ( 186.4733072505212590, 296.4258963025324078, -7.261958780044511563 ) ) ;
#27706=CARTESIAN_POINT ( 'NONE',  ( 161.2168897513269314, 281.8122871204358262, 5.602797683376681270 ) ) ;
#27707=CARTESIAN_POINT ( 'NONE',  ( 147.6512387128590262, 274.9075480792844246, -8.209968531507987777 ) ) ;
#27710=CARTESIAN_POINT ( 'NONE',  ( 82.36670705735998865, 218.3615022471902591, -10.00000000000009592 ) ) ;
#27711=CARTESIAN_POINT ( 'NONE',  ( 138.9086373102437051, 262.5530062829863027, -4.648177544792955347E-16 ) ) ;
#27713=CARTESIAN_POINT ( 'NONE',  ( 82.55649720842890815, 206.2202760586659167, -5.415160957724236172E-17 ) ) ;
#27714=CARTESIAN_POINT ( 'NONE',  ( 161.1093323826042933, 251.5974460702646809, -13.93502574894237078 ) ) ;
#27715=CARTESIAN_POINT ( 'NONE',  ( 163.5420923545723326, 257.9286257799056443, 15.56078752504084761 ) ) ;
#27716=CARTESIAN_POINT ( 'NONE',  ( 157.7233946900069839, 257.4620621851055375, 16.86796251324260254 ) ) ;
#27719=CARTESIAN_POINT ( 'NONE',  ( 204.6250002032067528, 275.7806821083123623, -12.66782070737391130 ) ) ;
#27721=CARTESIAN_POINT ( 'NONE',  ( 192.5076277540105423, 297.2140032159341558, -13.10094381206144298 ) ) ;
#27728=CARTESIAN_POINT ( 'NONE',  ( 153.7955429123465763, 266.9533995729482285, 16.35447140258466092 ) ) ;
#27732=CARTESIAN_POINT ( 'NONE',  ( 126.6061714340150104, 257.2365022471903444, 2.944929066748280225E-16 ) ) ;
#27735=ORIENTED_EDGE ( 'NONE', *, *, #73652, .F. ) ;
#27736=CARTESIAN_POINT ( 'NONE',  ( 169.5597748164675522, 248.6071028964281027, -1.929381512893630912 ) ) ;
#27745=CARTESIAN_POINT ( 'NONE',  ( 205.7101366950456338, 274.3465869426791528, 12.22104789793548818 ) ) ;
#27751=CARTESIAN_POINT ( 'NONE',  ( 164.7832096898899579, 274.5337176909793584, 14.74445750113318532 ) ) ;
#27756=CARTESIAN_POINT ( 'NONE',  ( 182.9676386820643472, 296.0067668443529101, 0.4350290018456622887 ) ) ;
#27757=CARTESIAN_POINT ( 'NONE',  ( 163.8147431267737204, 246.9115372060205118, 7.125417796469586840 ) ) ;
#27758=CARTESIAN_POINT ( 'NONE',  ( 194.3177355571849318, 294.0788045336591381, -15.93712594727561616 ) ) ;
#27761=CARTESIAN_POINT ( 'NONE',  ( 188.7214848040405286, 296.7531490838067612, -10.06825767521683801 ) ) ;
#27762=CARTESIAN_POINT ( 'NONE',  ( 157.5487431480040925, 257.7645675294749594, -18.29554785922338311 ) ) ;
#27763=CARTESIAN_POINT ( 'NONE',  ( 170.3178023250738420, 289.0326318653803241, -4.561300590322002080 ) ) ;
#27765=CARTESIAN_POINT ( 'NONE',  ( 181.8155868826606536, 256.4333448833576767, 5.198317300223314064 ) ) ;
#27766=CARTESIAN_POINT ( 'NONE',  ( 92.21748570181026139, 233.2369531367911009, -4.594050593750048428 ) ) ;
#27767=ORIENTED_EDGE ( 'NONE', *, *, #99780, .T. ) ;
#27769=CARTESIAN_POINT ( 'NONE',  ( 110.7831656154889259, 244.7677522451419065, -5.000000000000047962 ) ) ;
#27771=VERTEX_POINT ( 'NONE', #63039 ) ;
#27774=FACE_OUTER_BOUND ( 'NONE', #79826, .T. ) ;
#27776=ADVANCED_FACE ( 'NONE', ( #93982 ), #86400, .T. ) ;
#27777=CARTESIAN_POINT ( 'NONE',  ( 163.2189713653645242, 247.9434441664957944, 10.97120828841990914 ) ) ;
#27781=CARTESIAN_POINT ( 'NONE',  ( 182.3700640764176342, 263.2847133751610045, -13.94439451147478337 ) ) ;
#27782=CARTESIAN_POINT ( 'NONE',  ( 179.9209375999747351, 276.5811748711908535, 17.74520275588677265 ) ) ;
#27785=ADVANCED_FACE ( 'NONE', ( #43219 ), #42716, .T. ) ;
#27786=CARTESIAN_POINT ( 'NONE',  ( 191.5054231872901767, 263.6613473635590594, -8.131552266941017848 ) ) ;
#27787=CARTESIAN_POINT ( 'NONE',  ( 153.4893010137675731, 265.2713640115015892, 16.29005549651170881 ) ) ;
#27789=CARTESIAN_POINT ( 'NONE',  ( 125.3701074643745841, 249.3149278399160949, 9.188101187500093303 ) ) ;
#27790=CYLINDRICAL_SURFACE ( 'NONE', #70625, 10.00000000000010658 ) ;
#27791=CARTESIAN_POINT ( 'NONE',  ( 168.2008345946905479, 248.1884056956802453, -5.064766917302788052 ) ) ;
#27792=EDGE_LOOP ( 'NONE', ( #67631, #22559, #6926, #43034 ) ) ;
#27793=CARTESIAN_POINT ( 'NONE',  ( 67.12105150802354103, 202.8927522451418213, 10.00000000000009948 ) ) ;
#27796=CARTESIAN_POINT ( 'NONE',  ( 189.6400116240601221, 270.3132688328793733, 14.33464930468576171 ) ) ;
#27797=CARTESIAN_POINT ( 'NONE',  ( 178.3967306507444164, 285.3765218324597868, 13.04961304002345734 ) ) ;
#27803=CARTESIAN_POINT ( 'NONE',  ( 206.7990506781679301, 271.8220439983479082, 6.357107087294847858 ) ) ;
#27806=CARTESIAN_POINT ( 'NONE',  ( 207.7837159184916231, 270.7550423741513441, -2.369602332675663448 ) ) ;
#27811=CYLINDRICAL_SURFACE ( 'NONE', #44956, 17.82106496071139645 ) ;
#27813=CARTESIAN_POINT ( 'NONE',  ( 157.7229324233670980, 270.7041103179763581, -15.79028221516555419 ) ) ;
#27815=CARTESIAN_POINT ( 'NONE',  ( 17.60459192459599365, 168.7202760586659736, -5.415160957724236172E-17 ) ) ;
#27820=CARTESIAN_POINT ( 'NONE',  ( 202.4677460062568173, 269.8620261455625950, 8.891765442197028690 ) ) ;
#27822=CARTESIAN_POINT ( 'NONE',  ( 45.37135788555205096, 190.8768266524160140, 9.188101187500096856 ) ) ;
#27823=EDGE_CURVE ( 'NONE', #55188, #69106, #22065, .T. ) ;
#27825=CARTESIAN_POINT ( 'NONE',  ( 170.8524479326273138, 287.4302738079429673, 7.076016408304939276 ) ) ;
#27826=CARTESIAN_POINT ( 'NONE',  ( 190.1858949294064871, 301.2353624297489887, -5.249932979468886707 ) ) ;
#27829=CARTESIAN_POINT ( 'NONE',  ( 146.5502055023624735, 276.8145935406849389, 0.3770461397900869427 ) ) ;
#27830=CARTESIAN_POINT ( 'NONE',  ( 176.4362609909801165, 275.0927880625443436, 17.39602988701090780 ) ) ;
#27833=CARTESIAN_POINT ( 'NONE',  ( 166.8557127037659882, 257.9341067576638125, -15.25166664705231589 ) ) ;
#27834=CARTESIAN_POINT ( 'NONE',  ( -22.42236680055709641, 157.8615022471902591, 0.000000000000000000 ) ) ;
#27835=CARTESIAN_POINT ( 'NONE',  ( 85.03695205236195420, 233.2365022471903160, 2.944929066748280225E-16 ) ) ;
#27837=CARTESIAN_POINT ( 'NONE',  ( 161.5877803775636039, 267.7196290107671075, -17.14067319960231472 ) ) ;
#27839=CARTESIAN_POINT ( 'NONE',  ( 62.15025298811053034, 212.8149278399160949, -9.188101187500095079 ) ) ;
#27840=ORIENTED_EDGE ( 'NONE', *, *, #22388, .F. ) ;
#27841=CARTESIAN_POINT ( 'NONE',  ( 162.7710398924988908, 263.3845876204081833, 17.15398367141938962 ) ) ;
#27842=CARTESIAN_POINT ( 'NONE',  ( 162.1795029284002112, 250.7317292623248477, 12.60364379007453550 ) ) ;
#27845=CARTESIAN_POINT ( 'NONE',  ( 171.0113606419460837, 287.1407938163278573, 8.604837063268337971 ) ) ;
#27846=CARTESIAN_POINT ( 'NONE',  ( 164.6460902696047128, 245.4716017159096566, -3.036414139157908476 ) ) ;
#27849=CARTESIAN_POINT ( 'NONE',  ( 189.7726967107949747, 264.4065126852114531, 11.24316165915873000 ) ) ;
#27850=CARTESIAN_POINT ( 'NONE',  ( 181.1477013271936016, 287.8971774238942203, -14.15342935774602218 ) ) ;
#27851=CARTESIAN_POINT ( 'NONE',  ( 171.3515257658276028, 255.7365519920522559, 11.37700587845633748 ) ) ;
#27856=CARTESIAN_POINT ( 'NONE',  ( 171.8160532838503514, 252.3804680471336610, 8.773019167658075546 ) ) ;
#27859=CARTESIAN_POINT ( 'NONE',  ( 181.9839621645596992, 283.9156450579300213, 14.95553656096354622 ) ) ;
#27860=CARTESIAN_POINT ( 'NONE',  ( 151.4281781455628675, 268.3656970847310390, 15.24742929158552585 ) ) ;
#27863=VERTEX_POINT ( 'NONE', #2770 ) ;
#27864=CARTESIAN_POINT ( 'NONE',  ( 207.6129110656513035, 271.0508850574501025, -5.265106572941297358 ) ) ;
#27865=CARTESIAN_POINT ( 'NONE',  ( 61.87308422990769685, 194.9824982072973967, 3.021315404115420679E-15 ) ) ;
#27866=CARTESIAN_POINT ( 'NONE',  ( 196.5806080813426888, 290.1593943507663766, -16.31912166233602690 ) ) ;
#27872=CARTESIAN_POINT ( 'NONE',  ( 114.4365367415960293, 243.0024278399160949, -9.188101187500093303 ) ) ;
#27873=CARTESIAN_POINT ( 'NONE',  ( 120.5439936075240155, 233.7365022471902307, 10.00000000000009948 ) ) ;
#27874=CARTESIAN_POINT ( 'NONE',  ( 199.5442653985851962, 283.0261893010793415, -17.63221794778640117 ) ) ;
#27876=CARTESIAN_POINT ( 'NONE',  ( 208.3132655666949233, 269.8378354783333180, 2.688523655043302707 ) ) ;
#27878=ORIENTED_EDGE ( 'NONE', *, *, #38592, .F. ) ;
#27881=CARTESIAN_POINT ( 'NONE',  ( 78.41572647264329987, 206.8923013555409796, 4.594050593750050204 ) ) ;
#27884=CARTESIAN_POINT ( 'NONE',  ( 198.7076130252130497, 286.4753137200327728, 17.36142183403824291 ) ) ;
#27885=EDGE_CURVE ( 'NONE', #68960, #96482, #42755, .T. ) ;
#27886=CARTESIAN_POINT ( 'NONE',  ( 175.5746833524315775, 278.5347786252573314, 16.94864957847115505 ) ) ;
#27887=ORIENTED_EDGE ( 'NONE', *, *, #9111, .T. ) ;
#27890=FACE_OUTER_BOUND ( 'NONE', #17340, .T. ) ;
#27892=ORIENTED_EDGE ( 'NONE', *, *, #61047, .F. ) ;
#27894=CARTESIAN_POINT ( 'NONE',  ( 207.4541616930702617, 271.3258470364304458, -6.834942797545373594 ) ) ;
#27895=EDGE_CURVE ( 'NONE', #312, #64387, #12325, .T. ) ;
#27896=CARTESIAN_POINT ( 'NONE',  ( 192.5076277540105423, 297.2140032159341558, -13.10094381206144298 ) ) ;
#27897=CARTESIAN_POINT ( 'NONE',  ( 172.6505904036989136, 280.8448313155626579, -15.39888677054324440 ) ) ;
#27901=CARTESIAN_POINT ( 'NONE',  ( 127.4269177983626236, 250.5024278399160949, -9.188101187500093303 ) ) ;
#27903=CARTESIAN_POINT ( 'NONE',  ( 146.5865263025993954, 276.7516840693029962, 0.4918294119671828835 ) ) ;
#27905=CARTESIAN_POINT ( 'NONE',  ( 198.8081898473356262, 282.3983615885804284, -17.60554210735202574 ) ) ;
#27908=CARTESIAN_POINT ( 'NONE',  ( 178.6317619811870259, 253.9327355832967612, -4.167451725846189170 ) ) ;
#27911=CARTESIAN_POINT ( 'NONE',  ( 120.6702889753612737, 247.1427522451419350, 10.00000000000009415 ) ) ;
#27912=CARTESIAN_POINT ( 'NONE',  ( 167.4764150005448755, 249.1180365860762720, -5.480813618351669803 ) ) ;
#27913=CARTESIAN_POINT ( 'NONE',  ( 205.9252530167937323, 273.9739945438741984, -10.37964514155334328 ) ) ;
#27914=CARTESIAN_POINT ( 'NONE',  ( 202.6109660208213086, 267.6076335798982200, 0.8660040287496835187 ) ) ;
#27915=CARTESIAN_POINT ( 'NONE',  ( 190.1752790837055045, 301.2537496138681945, -5.177773110520776711 ) ) ;
#27920=B_SPLINE_SURFACE_WITH_KNOTS ( 'NONE', 3, 1, ( 
 ( #41688, #72631 ),
 ( #24498, #1723 ),
 ( #75111, #98410 ),
 ( #28483, #89836 ),
 ( #88872, #74114 ),
 ( #20919, #4190 ),
 ( #34596, #42676 ),
 ( #73125, #5686 ),
 ( #90843, #66492 ),
 ( #29004, #58868 ),
 ( #49797, #42190 ),
 ( #20411, #11331 ),
 ( #3716, #6185 ),
 ( #37566, #60857 ),
 ( #91321, #68971 ),
 ( #52767, #14289 ),
 ( #46672, #91822 ),
 ( #77598, #45663 ),
 ( #99894, #84720 ),
 ( #15261, #46156 ),
 ( #77074, #7681 ),
 ( #90, #23366 ),
 ( #54250, #24875 ),
 ( #93825, #41058 ),
 ( #70472, #71502 ),
 ( #9705, #1087 ),
 ( #49192, #32972 ),
 ( #16772, #55749 ),
 ( #87757, #86741 ),
 ( #48179, #31965 ),
 ( #80128, #34005 ),
 ( #10689, #41568 ),
 ( #93312, #16274 ),
 ( #47169, #65866 ) ),
 .UNSPECIFIED., .T., .F., .F.,
 ( 4, 2, 2, 2, 2, 2, 2, 2, 2, 2, 2, 2, 2, 2, 2, 2, 4 ),
 ( 2, 2 ),
 ( 0.000000000000000000, 0.06250000000000000000, 0.1250000000000000000, 0.1875000000000000000, 0.2500000000000000000, 0.3125000000000000000, 0.3750000000000000000, 0.4375000000000000000, 0.5000000000000000000, 0.5625000000000000000, 0.6250000000000000000, 0.6875000000000000000, 0.7500000000000000000, 0.8125000000000000000, 0.8750000000000000000, 0.9375000000000000000, 1.000000000000000000 ),
 ( 0.000000000000000000, 1.000000000000000000 ),
 .UNSPECIFIED. ) ;
#27922=CARTESIAN_POINT ( 'NONE',  ( 190.6023073677431512, 300.5141149296460981, 3.174888932019753973 ) ) ;
#27925=CARTESIAN_POINT ( 'NONE',  ( 155.1601726304954809, 261.9016930232608615, -18.56587418422714464 ) ) ;
#27926=CARTESIAN_POINT ( 'NONE',  ( 149.0237174825091415, 274.5263358477994871, 9.114370506038131481 ) ) ;
#27927=CARTESIAN_POINT ( 'NONE',  ( 135.5370584069941913, 242.3927522451417929, -10.00000000000009059 ) ) ;
#27928=CARTESIAN_POINT ( 'NONE',  ( 172.4401916400875621, 283.6719894713717167, -12.41194507545851522 ) ) ;
#27931=CARTESIAN_POINT ( 'NONE',  ( 151.1126408083691501, 268.9122237844355254, -15.82705194100464396 ) ) ;
#27932=CARTESIAN_POINT ( 'NONE',  ( -5.021015940802495692, 180.1589784336661637, -6.496448406907676862E-16 ) ) ;
#27933=B_SPLINE_CURVE_WITH_KNOTS ( 'NONE', 3,
 ( #23413, #29538, #67530, #61911 ),
 .UNSPECIFIED., .F., .F.,
 ( 4, 4 ),
 ( 0.009408440947594234535, 0.01495930912883047283 ),
 .UNSPECIFIED. ) ;
#27935=CARTESIAN_POINT ( 'NONE',  ( 53.97765888354242492, 189.7202760586659736, -5.415160957724236172E-17 ) ) ;
#27939=CARTESIAN_POINT ( 'NONE',  ( 204.9184781223158609, 275.7177798128946620, -12.59106622113254126 ) ) ;
#27940=CARTESIAN_POINT ( 'NONE',  ( 192.4205004985176402, 292.7214258041265680, -14.22339032255528757 ) ) ;
#27942=CARTESIAN_POINT ( 'NONE',  ( 167.8546155174443015, 256.7248629110974889, 13.70153385259920142 ) ) ;
#27944=CARTESIAN_POINT ( 'NONE',  ( 198.0788209437629916, 287.5644135525011507, 18.31867165462247726 ) ) ;
#27945=ADVANCED_FACE ( 'NONE', ( #57935 ), #7570, .F. ) ;
#27946=CARTESIAN_POINT ( 'NONE',  ( 47.79785968963118137, 191.7365022471902307, 10.00000000000009592 ) ) ;
#27947=CYLINDRICAL_SURFACE ( 'NONE', #50617, 17.82106496071139645 ) ;
#27948=CARTESIAN_POINT ( 'NONE',  ( 189.8136646974935786, 301.8800841035353528, -0.6430783927310335102 ) ) ;
#27949=CARTESIAN_POINT ( 'NONE',  ( 20.25662117580333188, 176.3768266524159856, -9.188101187500091527 ) ) ;
#27951=EDGE_CURVE ( 'NONE', #73044, #40898, #74215, .T. ) ;
#27954=CARTESIAN_POINT ( 'NONE',  ( 157.0239713899953244, 269.7369771206523978, 16.31777668093047851 ) ) ;
#27955=CARTESIAN_POINT ( 'NONE',  ( 182.9121110983079745, 278.7409904731791244, 16.73155022942700398 ) ) ;
#27956=CARTESIAN_POINT ( 'NONE',  ( 193.8603219414924013, 294.8710681561126989, 15.36476279452078586 ) ) ;
#27957=CARTESIAN_POINT ( 'NONE',  ( 115.2756724011686202, 247.3615022471903160, 5.000000000000046185 ) ) ;
#27958=CARTESIAN_POINT ( 'NONE',  ( 176.8095048781594869, 260.7838774868672544, -13.17535878752048539 ) ) ;
#27965=CARTESIAN_POINT ( 'NONE',  ( 156.8525332442023341, 276.4918820038299714, 10.31694992604559324 ) ) ;
#27968=CARTESIAN_POINT ( 'NONE',  ( 166.5483893385236627, 250.3327489066329292, -10.49964665769386762 ) ) ;
#27970=CARTESIAN_POINT ( 'NONE',  ( 192.1883190596398094, 297.7670620978826150, 12.41391288785556668 ) ) ;
#27972=B_SPLINE_CURVE_WITH_KNOTS ( 'NONE', 3,
 ( #85323, #46777, #29586, #7272, #53374, #76684, #77700, #23970, #39149, #16378, #6785, #70062, #91417, #47269, #680, #31561 ),
 .UNSPECIFIED., .F., .F.,
 ( 4, 2, 2, 2, 2, 2, 2, 4 ),
 ( 3.103167691559091397E-17, 0.0005277448334066532805, 0.0007916172501099130255, 0.001055489666813172987, 0.001319362083516432624, 0.001583234500219692477, 0.001847106916922952331, 0.002110979333626212401 ),
 .UNSPECIFIED. ) ;
#27974=CARTESIAN_POINT ( 'NONE',  ( 155.5211745099813356, 261.2764194263634749, -17.18163098020766810 ) ) ;
#27975=ORIENTED_EDGE ( 'NONE', *, *, #85928, .F. ) ;
#27976=( BOUNDED_CURVE ( )  B_SPLINE_CURVE ( 2, ( #83754, #39082, #45687, #15796, #61889, #92840, #14315, #23391, #45202 ),
 .UNSPECIFIED., .F., .T. ) 
 B_SPLINE_CURVE_WITH_KNOTS ( ( 3, 2, 2, 2, 3 ),
 ( 0.6491935483870967527, 0.6505376344086021279, 0.6532258064516128782, 0.6559139784946236285, 0.6572580645161290036 ),
 .UNSPECIFIED. ) 
 CURVE ( )  GEOMETRIC_REPRESENTATION_ITEM ( )  RATIONAL_B_SPLINE_CURVE ( ( 0.9330127018922194093, 0.9330127018922194093, 1.000000000000000000, 0.8660254037844387076, 1.000000000000000000, 0.8660254037844387076, 1.000000000000000000, 0.9330127018922194093, 0.9330127018922194093 ) ) 
 REPRESENTATION_ITEM ( '' )  );
#27978=CARTESIAN_POINT ( 'NONE',  ( 159.1344352748853055, 279.7114264697810313, -10.00621538743078354 ) ) ;
#27979=CARTESIAN_POINT ( 'NONE',  ( 153.2712411579340426, 265.1734183057532732, 16.26687330118495467 ) ) ;
#27983=CARTESIAN_POINT ( 'NONE',  ( 178.2874402213737710, 264.0549037780814388, 14.92174102309952133 ) ) ;
#27984=ORIENTED_EDGE ( 'NONE', *, *, #95033, .F. ) ;
#27987=B_SPLINE_CURVE_WITH_KNOTS ( 'NONE', 3,
 ( #26787, #90630, #61158, #15547 ),
 .UNSPECIFIED., .F., .F.,
 ( 4, 4 ),
 ( 0.02131823508248953739, 0.02883180965995480252 ),
 .UNSPECIFIED. ) ;
#27991=CARTESIAN_POINT ( 'NONE',  ( 160.1969820541083607, 255.1776831935258372, -16.37528374203482073 ) ) ;
#27992=CARTESIAN_POINT ( 'NONE',  ( 164.3090168944849836, 246.0554299274959931, 2.641760039552302430 ) ) ;
#27996=CARTESIAN_POINT ( 'NONE',  ( 174.5846041374311710, 276.7874870096778182, -16.75558966740674549 ) ) ;
#27997=CARTESIAN_POINT ( 'NONE',  ( 172.3600888395878314, 263.7131837874231337, -15.46760836022099994 ) ) ;
#28001=ORIENTED_EDGE ( 'NONE', *, *, #15771, .T. ) ;
#28002=CARTESIAN_POINT ( 'NONE',  ( 149.7854447168632817, 277.1467554076948545, 4.663160563959508842 ) ) ;
#28003=ORIENTED_EDGE ( 'NONE', *, *, #36446, .T. ) ;
#28004=CARTESIAN_POINT ( 'NONE',  ( 156.4811347401371506, 266.4657705092222386, -16.23271684233645118 ) ) ;
#28009=CARTESIAN_POINT ( 'NONE',  ( 153.3127735718713609, 265.1014820546527631, 17.57722645152040641 ) ) ;
#28010=CARTESIAN_POINT ( 'NONE',  ( 178.1892993710524138, 292.1905823108662617, 7.166771068777840092 ) ) ;
#28012=CARTESIAN_POINT ( 'NONE',  ( 158.8791574486372440, 255.4602223656619628, -17.57574691297732272 ) ) ;
#28014=EDGE_LOOP ( 'NONE', ( #24268, #73733, #50798, #36932 ) ) ;
#28016=CARTESIAN_POINT ( 'NONE',  ( 165.0308887387863876, 244.8051112166122891, 1.948365933089477808 ) ) ;
#28017=CARTESIAN_POINT ( 'NONE',  ( 206.4695239676918845, 273.0312896038346366, 10.41704154450801667 ) ) ;
#28020=CARTESIAN_POINT ( 'NONE',  ( -17.42236680055705023, 149.2012482093457777, 0.000000000000000000 ) ) ;
#28021=CARTESIAN_POINT ( 'NONE',  ( 177.2307473631791765, 288.8998395665854559, -9.216979198774193804 ) ) ;
#28025=CARTESIAN_POINT ( 'NONE',  ( 126.9410149175250524, 232.5494855054051868, -2.679491924311248496 ) ) ;
#28026=CARTESIAN_POINT ( 'NONE',  ( 160.6612659640541381, 252.3735198723586848, -15.60644164121982591 ) ) ;
#28027=CARTESIAN_POINT ( 'NONE',  ( 190.3150247411125804, 301.0117030351020730, 0.1088388511812921067 ) ) ;
#28029=CARTESIAN_POINT ( 'NONE',  ( 170.5392822398632404, 255.6756181042317735, -11.78486988674311675 ) ) ;
#28030=CARTESIAN_POINT ( 'NONE',  ( 191.4420812244453600, 260.8157448279923187, -1.331758356259544085 ) ) ;
#28031=CARTESIAN_POINT ( 'NONE',  ( 52.48883062679681899, 211.1115022471903444, -5.000000000000047962 ) ) ;
#28032=CARTESIAN_POINT ( 'NONE',  ( 164.2600772519394923, 246.1401958748887182, -2.110785484364219311 ) ) ;
#28033=CARTESIAN_POINT ( 'NONE',  ( 27.13954536664190798, 193.1427522451419065, 10.00000000000009237 ) ) ;
#28034=CARTESIAN_POINT ( 'NONE',  ( 108.7534185771431510, 233.5958772461660260, -9.188101187500095079 ) ) ;
#28035=CARTESIAN_POINT ( 'NONE',  ( 183.5623937226978057, 296.1742073513109403, -2.708913905850958148 ) ) ;
#28036=CARTESIAN_POINT ( 'NONE',  ( 164.0485396284991850, 280.4819838086867776, -11.53262238567191211 ) ) ;
#28038=CARTESIAN_POINT ( 'NONE',  ( 208.2726345668874615, 269.9082104343620472, 2.818736869262927769 ) ) ;
#28039=CARTESIAN_POINT ( 'NONE',  ( 41.04123086662985997, 188.3768266524159856, -9.188101187500091527 ) ) ;
#28040=CARTESIAN_POINT ( 'NONE',  ( 173.3507806980417456, 251.4055554679256375, 5.750257727834116039 ) ) ;
#28043=CARTESIAN_POINT ( 'NONE',  ( 190.8089377949079903, 299.1047931790669736, 7.367255922332321738 ) ) ;
#28046=CARTESIAN_POINT ( 'NONE',  ( 190.2236813008869660, 301.1699145145108218, -5.401374690107298093 ) ) ;
#28047=CARTESIAN_POINT ( 'NONE',  ( 104.3601438707544133, 224.3927522451418213, -10.00000000000009237 ) ) ;
#28048=CARTESIAN_POINT ( 'NONE',  ( 161.8882824960653579, 250.2482648971885340, -13.83574485983625557 ) ) ;
#28049=CARTESIAN_POINT ( 'NONE',  ( 176.1923717941176619, 285.1500375202994064, -12.53270729091486402 ) ) ;
#28051=CARTESIAN_POINT ( 'NONE',  ( 86.17361039128113021, 233.8927522451419634, 2.944929066748280225E-16 ) ) ;
#28052=ORIENTED_EDGE ( 'NONE', *, *, #90672, .F. ) ;
#28055=CARTESIAN_POINT ( 'NONE',  ( 162.9466247808429102, 248.4151622881552441, 11.25765811906727443 ) ) ;
#28056=CARTESIAN_POINT ( 'NONE',  ( 207.5920568422024814, 271.0870056320159165, -1.586464549033245186 ) ) ;
#28058=ADVANCED_FACE ( 'NONE', ( #72426 ), #49101, .T. ) ;
#28059=CARTESIAN_POINT ( 'NONE',  ( 13.49027706508988267, 190.8464784336661637, 1.353441290958777327E-15 ) ) ;
#28060=CARTESIAN_POINT ( 'NONE',  ( 198.4782858197754649, 286.8725200914082620, -17.44895083299520522 ) ) ;
#28061=CARTESIAN_POINT ( 'NONE',  ( 173.8665542827094725, 250.6399523573830095, -0.9454928766311748722 ) ) ;
#28063=CARTESIAN_POINT ( 'NONE',  ( 53.49034604603116350, 195.5643266524160140, 9.188101187500095079 ) ) ;
#28065=CARTESIAN_POINT ( 'NONE',  ( 164.0179800784044915, 246.5595204798204065, -5.772998092557310557 ) ) ;
#28071=CARTESIAN_POINT ( 'NONE',  ( 12.14648056717180680, 164.4865022471901455, 1.119607411625061291E-15 ) ) ;
#28074=CARTESIAN_POINT ( 'NONE',  ( 124.8288415870092933, 249.0024278399161517, -9.188101187500093303 ) ) ;
#28076=CARTESIAN_POINT ( 'NONE',  ( 183.7975612849717777, 256.6346208101135176, -2.981236333899912161 ) ) ;
#28078=CARTESIAN_POINT ( 'NONE',  ( 188.3728390295439965, 260.6292366468635464, 6.857486809614422363 ) ) ;
#28079=CARTESIAN_POINT ( 'NONE',  ( 196.2225432063612232, 281.9592983342773778, 17.73143785322795196 ) ) ;
#28084=VERTEX_POINT ( 'NONE', #56690 ) ;
#28085=CARTESIAN_POINT ( 'NONE',  ( 160.7827666075975799, 284.1908911587130433, 0.8999949044102747431 ) ) ;
#28089=CARTESIAN_POINT ( 'NONE',  ( 193.9123665762526798, 270.9003325324202365, -13.75132347621049433 ) ) ;
#28090=ORIENTED_EDGE ( 'NONE', *, *, #18483, .F. ) ;
#28093=EDGE_CURVE ( 'NONE', #46269, #48318, #32396, .T. ) ;
#28094=EDGE_CURVE ( 'NONE', #5477, #469, #22326, .T. ) ;
#28096=CARTESIAN_POINT ( 'NONE',  ( 29.61132621015796218, 181.2365022471902307, 10.00000000000009948 ) ) ;
#28097=CARTESIAN_POINT ( 'NONE',  ( 185.8703600842969479, 296.7409536067417548, 5.193023113616601627 ) ) ;
#28099=CARTESIAN_POINT ( 'NONE',  ( 150.7294676703291998, 278.2523418184223942, -9.598868465181176928E-05 ) ) ;
#28101=CARTESIAN_POINT ( 'NONE',  ( 95.53204957371639239, 214.4155109091896065, 2.679491924311254714 ) ) ;
#28105=CARTESIAN_POINT ( 'NONE',  ( 156.3110802652713573, 261.4039762261047599, -17.34184811412823635 ) ) ;
#28107=CARTESIAN_POINT ( 'NONE',  ( 147.1259762202154207, 275.8173294038533641, -0.6716460511724978710 ) ) ;
#28108=CARTESIAN_POINT ( 'NONE',  ( 185.1915215135591666, 291.4364884111334391, 11.94946919150295983 ) ) ;
#28109=CARTESIAN_POINT ( 'NONE',  ( 204.9427641582406636, 275.6757151647582305, 14.40446820030680897 ) ) ;
#28111=ORIENTED_EDGE ( 'NONE', *, *, #2279, .T. ) ;
#28112=CARTESIAN_POINT ( 'NONE',  ( 87.75264963113552596, 209.2202760586659167, -5.415160957724236172E-17 ) ) ;
#28113=FACE_OUTER_BOUND ( 'NONE', #17386, .T. ) ;
#28115=CARTESIAN_POINT ( 'NONE',  ( 181.1066788586338703, 271.7431116842795973, -16.79793830016840772 ) ) ;
#28117=VERTEX_POINT ( 'NONE', #57680 ) ;
#28119=ORIENTED_EDGE ( 'NONE', *, *, #29347, .F. ) ;
#28122=DIRECTION ( 'NONE',  ( -0.4999999999999998890, 0.8660254037844387076, 0.000000000000000000 ) ) ;
#28125=DIRECTION ( 'NONE',  ( -0.4999999999999987788, 0.8660254037844392627, 0.000000000000000000 ) ) ;
#28126=EDGE_LOOP ( 'NONE', ( #74295, #48799, #14778 ) ) ;
#28128=CARTESIAN_POINT ( 'NONE',  ( 188.9164685758636608, 292.7259968989668550, -13.92583900068085612 ) ) ;
#28131=CARTESIAN_POINT ( 'NONE',  ( 194.5298665426430489, 293.7113828889860656, -16.13302716640051315 ) ) ;
#28132=B_SPLINE_CURVE_WITH_KNOTS ( 'NONE', 3,
 ( #41846, #78373, #34256, #97450, #58894, #89864, #32250, #63150, #24647, #55529, #98937, #92352, #13813, #44203 ),
 .UNSPECIFIED., .F., .F.,
 ( 4, 2, 2, 2, 2, 2, 4 ),
 ( 0.0005908581131731061812, 0.0008957186388731243169, 0.001200579164573142670, 0.001505439690273160805, 0.001810300215973178941, 0.002420021267373170543, 0.003029742318773161712 ),
 .UNSPECIFIED. ) ;
#28133=CARTESIAN_POINT ( 'NONE',  ( 11.25695247149110578, 165.7592609112379876, 2.679491924311254714 ) ) ;
#28135=CARTESIAN_POINT ( 'NONE',  ( 166.6488341214076740, 266.2507106308010520, -16.67339293460069882 ) ) ;
#28143=EDGE_CURVE ( 'NONE', #100197, #12032, #44019, .T. ) ;
#28145=CARTESIAN_POINT ( 'NONE',  ( 163.0309151244508712, 248.2691671304387739, 11.27270415168660200 ) ) ;
#28146=EDGE_CURVE ( 'NONE', #35245, #33613, #754, .T. ) ;
#28148=CARTESIAN_POINT ( 'NONE',  ( 149.0959959396991792, 276.3173998796609681, -5.502691077969892319 ) ) ;
#28149=CARTESIAN_POINT ( 'NONE',  ( 175.5923782935951465, 257.1381361707857991, -12.16266005493879021 ) ) ;
#28150=CARTESIAN_POINT ( 'NONE',  ( 157.5196022909033502, 258.1848738215194317, 16.72387774136761607 ) ) ;
#28158=CARTESIAN_POINT ( 'NONE',  ( 2.672015980952107572, 183.8967562850347122, -4.648177544792955347E-16 ) ) ;
#28160=CARTESIAN_POINT ( 'NONE',  ( 174.8100629882666226, 281.9492555863050711, -14.07939969178291051 ) ) ;
#28163=CARTESIAN_POINT ( 'NONE',  ( 161.2348838590686171, 272.7422516289890382, 15.21521688586838472 ) ) ;
#28164=CARTESIAN_POINT ( 'NONE',  ( 161.4314170165220332, 281.4313146435951580, -6.707529758775564233 ) ) ;
#28166=CARTESIAN_POINT ( 'NONE',  ( 201.3130515071547961, 268.8394849092184700, 6.031093409804897831 ) ) ;
#28167=ORIENTED_EDGE ( 'NONE', *, *, #55322, .F. ) ;
#28171=CARTESIAN_POINT ( 'NONE',  ( 189.8221425493700565, 274.2140629761119612, -15.64287807072788006 ) ) ;
#28173=CARTESIAN_POINT ( 'NONE',  ( 175.6300312749814054, 290.9929735238556532, 2.874909097761923160 ) ) ;
#28174=CARTESIAN_POINT ( 'NONE',  ( 152.7531861616124615, 266.0707158804971186, 17.45453282433162556 ) ) ;
#28175=CARTESIAN_POINT ( 'NONE',  ( 191.3077102587145646, 274.7514833773715850, 16.90660339326615969 ) ) ;
#28177=CARTESIAN_POINT ( 'NONE',  ( 7.212287079182728711, 162.7202760586659451, -5.415160957724236172E-17 ) ) ;
#28178=CARTESIAN_POINT ( 'NONE',  ( 104.5047417616495125, 221.9548013555409511, -4.594050593750042211 ) ) ;
#28180=CARTESIAN_POINT ( 'NONE',  ( 179.9432324357175617, 255.2313477386617819, -2.391771382723571371 ) ) ;
#28182=DIRECTION ( 'NONE',  ( -0.8660254037844387076, -0.4999999999999998890, -0.000000000000000000 ) ) ;
#28183=CARTESIAN_POINT ( 'NONE',  ( 193.7261517370125432, 295.1034577671335342, 14.97744313279139661 ) ) ;
#28185=CARTESIAN_POINT ( 'NONE',  ( 147.9791529310278122, 274.3395839928920168, -7.789432462804474433 ) ) ;
#28186=CARTESIAN_POINT ( 'NONE',  ( 196.5855195306807275, 266.6350943561007512, 8.187369356346602345 ) ) ;
#28188=CARTESIAN_POINT ( 'NONE',  ( 162.4519475857721886, 251.5162682124039577, -12.77131419988232786 ) ) ;
#28189=CARTESIAN_POINT ( 'NONE',  ( 43.66619682219493370, 206.0177522451419350, 5.000000000000046185 ) ) ;
#28191=CARTESIAN_POINT ( 'NONE',  ( 86.20995510670323370, 211.3923013555409796, 4.594050593750050204 ) ) ;
#28193=EDGE_CURVE ( 'NONE', #90499, #31470, #53125, .T. ) ;
#28195=CARTESIAN_POINT ( 'NONE',  ( 196.3341081413628899, 290.5863447708742342, 16.12390540996472410 ) ) ;
#28196=CARTESIAN_POINT ( 'NONE',  ( 151.9941942893360078, 267.3853283658117448, 16.97183802629870186 ) ) ;
#28197=CARTESIAN_POINT ( 'NONE',  ( 149.7588342556250041, 271.2570855174081430, 12.14104876789268062 ) ) ;
#28199=CARTESIAN_POINT ( 'NONE',  ( 204.6060263820569673, 275.8495439392309549, -12.70564820073907875 ) ) ;
#28201=CARTESIAN_POINT ( 'NONE',  ( 147.3379027498079381, 275.4502618871274535, -3.695260257281167249 ) ) ;
#28205=CARTESIAN_POINT ( 'NONE',  ( 60.73642589098854216, 194.3262482093457777, 3.021315404115420679E-15 ) ) ;
#28206=CARTESIAN_POINT ( 'NONE',  ( 147.5381343315788172, 275.1034506142203782, -4.056595942992749393 ) ) ;
#28207=CARTESIAN_POINT ( 'NONE',  ( 191.2640738146788806, 288.8540904607579591, -16.48495303880790530 ) ) ;
#28208=EDGE_CURVE ( 'NONE', #32720, #33264, #76703, .T. ) ;
#28216=CARTESIAN_POINT ( 'NONE',  ( 142.1946287021350201, 246.2365022471901739, -10.00000000000009059 ) ) ;
#28220=CARTESIAN_POINT ( 'NONE',  ( 190.9372308562805642, 299.3033410696684200, -6.605635028715870938 ) ) ;
#28222=CARTESIAN_POINT ( 'NONE',  ( 202.8787628851569593, 279.2506702366259788, 17.01435431865322556 ) ) ;
#28225=DIRECTION ( 'NONE',  ( -0.8660254037844387076, -0.4999999999999998890, -0.000000000000000000 ) ) ;
#28227=ORIENTED_EDGE ( 'NONE', *, *, #86723, .T. ) ;
#28229=CARTESIAN_POINT ( 'NONE',  ( 158.6888631046942919, 255.7898218377643218, 16.04723042051886495 ) ) ;
#28232=CARTESIAN_POINT ( 'NONE',  ( 192.3713340522295709, 271.8780416168410170, 15.57788208939756380 ) ) ;
#28235=CARTESIAN_POINT ( 'NONE',  ( 167.3724807468772156, 276.1273818265106570, 14.94019753784689364 ) ) ;
#28240=EDGE_CURVE ( 'NONE', #71770, #88756, #14956, .T. ) ;
#28241=CARTESIAN_POINT ( 'NONE',  ( 164.2851776226980860, 246.0967207574460929, 5.847738044744511754 ) ) ;
#28242=CARTESIAN_POINT ( 'NONE',  ( 165.6659538038370272, 273.9139261607198250, -15.19161387577927869 ) ) ;
#28246=CARTESIAN_POINT ( 'NONE',  ( 190.1063449786324213, 301.3731469862293011, 0.2163967485516588019 ) ) ;
#28248=CARTESIAN_POINT ( 'NONE',  ( 168.4629122334965530, 266.7134460659350452, 16.64887115331695355 ) ) ;
#28249=CARTESIAN_POINT ( 'NONE',  ( 182.0214274888115256, 256.7798808314274766, 5.137347305127032193 ) ) ;
#28251=CARTESIAN_POINT ( 'NONE',  ( 108.2124997955428967, 221.0327760586659451, 1.948934522072303157E-15 ) ) ;
#28255=CARTESIAN_POINT ( 'NONE',  ( 163.4018158682571595, 277.0544782939701918, -14.36443031031798512 ) ) ;
#28260=CARTESIAN_POINT ( 'NONE',  ( 176.8648875818473698, 292.4786256060604615, -2.731852314562509321 ) ) ;
#28261=CARTESIAN_POINT ( 'NONE',  ( 196.0395593785976018, 291.0965181932902510, 15.97855489120023087 ) ) ;
#28262=CARTESIAN_POINT ( 'NONE',  ( 206.6268150440956504, 272.7588534679261443, -10.76664753678610609 ) ) ;
#28263=CARTESIAN_POINT ( 'NONE',  ( 206.9821235601573051, 271.0354183991746595, -4.828536961709945174 ) ) ;
#28264=VERTEX_POINT ( 'NONE', #4311 ) ;
#28266=CARTESIAN_POINT ( 'NONE',  ( 163.0056347026689707, 248.3129541054019569, -11.27842346302751508 ) ) ;
#28267=ORIENTED_EDGE ( 'NONE', *, *, #9468, .F. ) ;
#28268=CARTESIAN_POINT ( 'NONE',  ( 168.9925526219222434, 247.8045925068635142, -0.5692285522127000785 ) ) ;
#28271=CARTESIAN_POINT ( 'NONE',  ( 137.3322569020296555, 250.0958772461660544, -9.188101187500095079 ) ) ;
#28273=CARTESIAN_POINT ( 'NONE',  ( 147.1270795744234476, 264.4111747905818675, -1.822351119449947324E-15 ) ) ;
#28274=ORIENTED_EDGE ( 'NONE', *, *, #27698, .T. ) ;
#28275=CARTESIAN_POINT ( 'NONE',  ( 204.9620549308181694, 275.6423025665365572, 14.49661402992083481 ) ) ;
#28276=CARTESIAN_POINT ( 'NONE',  ( -22.42236680055709641, 157.8615022471902591, 0.000000000000000000 ) ) ;
#28278=CARTESIAN_POINT ( 'NONE',  ( 170.1446682757344320, 248.6762405125142550, -0.2689902457364031774 ) ) ;
#28286=CARTESIAN_POINT ( 'NONE',  ( 59.22776434610305785, 198.8768266524159856, -9.188101187500091527 ) ) ;
#28287=CARTESIAN_POINT ( 'NONE',  ( 206.0870578475358172, 273.6937403561189512, -10.07771901274806581 ) ) ;
#28289=CARTESIAN_POINT ( 'NONE',  ( 185.7187107349099335, 289.5908206096054300, -14.74808349899648441 ) ) ;
#28290=ADVANCED_FACE ( 'NONE', ( #90962 ), #44300, .T. ) ;
#28292=CARTESIAN_POINT ( 'NONE',  ( 196.5206556047187405, 288.9772018564501650, -16.98128517232440515 ) ) ;
#28293=CARTESIAN_POINT ( 'NONE',  ( 196.1245817477023650, 288.9492551302209336, 17.30641872853625074 ) ) ;
#28295=CARTESIAN_POINT ( 'NONE',  ( 163.9961211234992788, 256.9275610305372766, 16.20495027727189807 ) ) ;
#28299=CARTESIAN_POINT ( 'NONE',  ( 187.9019955452718023, 260.0457317612239194, -6.306085470763082235 ) ) ;
#28300=CARTESIAN_POINT ( 'NONE',  ( 16.84647260051960060, 180.5333772461660544, 9.188101187500095079 ) ) ;
#28301=CARTESIAN_POINT ( 'NONE',  ( 50.34412104557527812, 188.3262482093458061, 3.021315404115420679E-15 ) ) ;
#28303=CARTESIAN_POINT ( 'NONE',  ( 180.2008674086625888, 256.3788900776044102, -7.862092545524210330 ) ) ;
#28308=CARTESIAN_POINT ( 'NONE',  ( 56.79189435007682363, 203.5958772461660544, -9.188101187500095079 ) ) ;
#28311=CARTESIAN_POINT ( 'NONE',  ( 151.2567985338353935, 268.6625352796243646, -15.71756535662528798 ) ) ;
#28312=CARTESIAN_POINT ( 'NONE',  ( 190.5653282632609091, 300.5781646174276602, -5.775635208185608604 ) ) ;
#28314=CARTESIAN_POINT ( 'NONE',  ( 197.6456421031980994, 287.3858497455466932, 17.15283754821559015 ) ) ;
#28315=CARTESIAN_POINT ( 'NONE',  ( 178.2069057043887597, 292.8217088069856686, 2.606728601885306418 ) ) ;
#28316=CARTESIAN_POINT ( 'NONE',  ( 176.1898462797690286, 274.9273359329014284, 17.22711636514044642 ) ) ;
#28319=CARTESIAN_POINT ( 'NONE',  ( 110.2779841299480239, 241.1427522451419350, 10.00000000000009415 ) ) ;
#28320=ADVANCED_FACE ( 'NONE', ( #83348 ), #27637, .T. ) ;
#28324=CARTESIAN_POINT ( 'NONE',  ( 95.42925689777524667, 239.2365022471903160, 2.944929066748280225E-16 ) ) ;
#28326=CARTESIAN_POINT ( 'NONE',  ( 164.9724657260474885, 270.3093585490532291, -16.49746900520251813 ) ) ;
#28327=ORIENTED_EDGE ( 'NONE', *, *, #81325, .F. ) ;
#28328=CARTESIAN_POINT ( 'NONE',  ( 63.55789136502527015, 201.3768266524160140, 9.188101187500098632 ) ) ;
#28329=VERTEX_POINT ( 'NONE', #21520 ) ;
#28330=CARTESIAN_POINT ( 'NONE',  ( 166.1585231282997199, 265.3369310901885001, 16.55309318940343388 ) ) ;
#28331=CARTESIAN_POINT ( 'NONE',  ( 161.5260038405503451, 251.2952618122203319, 12.95262340733779283 ) ) ;
#28334=CARTESIAN_POINT ( 'NONE',  ( 65.47921168356343458, 208.6115022471902307, 10.00000000000009592 ) ) ;
#28335=CARTESIAN_POINT ( 'NONE',  ( 165.0387478276132072, 244.7914988754632191, -2.473354058663827626 ) ) ;
#28338=CARTESIAN_POINT ( 'NONE',  ( 188.9788064033937758, 265.5261700445853421, 10.73023398055530642 ) ) ;
#28339=CARTESIAN_POINT ( 'NONE',  ( 196.2293283710122012, 290.7678286567270902, -17.07152402978540096 ) ) ;
#28340=CARTESIAN_POINT ( 'NONE',  ( 156.6823612109870396, 259.2651850631482375, 17.57884712310819708 ) ) ;
#28341=ORIENTED_EDGE ( 'NONE', *, *, #41819, .T. ) ;
#28344=CARTESIAN_POINT ( 'NONE',  ( 171.2037670605694473, 290.1117831344525939, -1.923673588436341841 ) ) ;
#28345=CARTESIAN_POINT ( 'NONE',  ( 168.1721027265311648, 255.0603569770035222, -13.93527711627501198 ) ) ;
#28347=FACE_OUTER_BOUND ( 'NONE', #38190, .T. ) ;
#28348=CARTESIAN_POINT ( 'NONE',  ( 167.5505310038667517, 261.6318463984700315, 17.07012949051403439 ) ) ;
#28349=CARTESIAN_POINT ( 'NONE',  ( 206.1798448551755598, 273.5330285446045195, -10.53862763475382813 ) ) ;
#28351=ORIENTED_EDGE ( 'NONE', *, *, #37580, .F. ) ;
#28352=ORIENTED_EDGE ( 'NONE', *, *, #47452, .T. ) ;
#28354=CARTESIAN_POINT ( 'NONE',  ( 207.1007598919583472, 271.9379569114424271, -6.086525981869248092 ) ) ;
#28357=ORIENTED_EDGE ( 'NONE', *, *, #62855, .F. ) ;
#28359=CARTESIAN_POINT ( 'NONE',  ( 198.2114954873088948, 287.3346145022089786, 18.52864136173620935 ) ) ;
#28360=FACE_OUTER_BOUND ( 'NONE', #17380, .T. ) ;
#28363=CARTESIAN_POINT ( 'NONE',  ( 132.2986577904151204, 241.0643266524160424, -9.188101187500093303 ) ) ;
#28364=DIRECTION ( 'NONE',  ( 0.4999999999999998890, -0.8660254037844385966, 0.000000000000000000 ) ) ;
#28366=CARTESIAN_POINT ( 'NONE',  ( 170.7338553607939957, 263.9049642311459252, 15.82425947459563353 ) ) ;
#28367=CARTESIAN_POINT ( 'NONE',  ( 115.3478411848173693, 230.7365022471902307, 10.00000000000009948 ) ) ;
#28370=VERTEX_POINT ( 'NONE', #44792 ) ;
#28372=CARTESIAN_POINT ( 'NONE',  ( 198.6755293322981117, 286.5308843062557571, 17.86676876308990103 ) ) ;
#28373=CARTESIAN_POINT ( 'NONE',  ( -27.42236680055714260, 166.5217562850347406, 1.224646799147364892E-15 ) ) ;
#28374=CARTESIAN_POINT ( 'NONE',  ( 72.54290492928882372, 206.5643266524159856, -9.188101187500093303 ) ) ;
#28376=CARTESIAN_POINT ( 'NONE',  ( 111.7394020023821781, 241.9865022471903160, 10.00000000000009415 ) ) ;
#28378=CARTESIAN_POINT ( 'NONE',  ( -17.65922707974272399, 170.6115022471903160, -5.000000000000047962 ) ) ;
#28380=ORIENTED_EDGE ( 'NONE', *, *, #54579, .F. ) ;
#28382=CARTESIAN_POINT ( 'NONE',  ( 153.4542976351440302, 264.8563551865710224, -17.11782692037292009 ) ) ;
#28383=CARTESIAN_POINT ( 'NONE',  ( 203.4682009197399566, 278.2297336128146412, -15.36039508894693206 ) ) ;
#28384=ORIENTED_EDGE ( 'NONE', *, *, #79534, .F. ) ;
#28387=CARTESIAN_POINT ( 'NONE',  ( 164.4320720012133847, 246.5467109461125119, 4.311465402957962212 ) ) ;
#28388=CARTESIAN_POINT ( 'NONE',  ( 199.5442653985851962, 283.0261893010793415, -17.63221794778640117 ) ) ;
#28392=CARTESIAN_POINT ( 'NONE',  ( 149.1004267900891307, 272.3974806997987343, -12.86882154300063341 ) ) ;
#28393=CARTESIAN_POINT ( 'NONE',  ( 36.56303213232966698, 203.4637435831424739, 2.679491924311303119 ) ) ;
#28395=CARTESIAN_POINT ( 'NONE',  ( 134.5444773117747275, 257.6744531367911577, 4.594050593750047540 ) ) ;
#28397=CARTESIAN_POINT ( 'NONE',  ( 182.1984841339006778, 258.0221543759674887, 6.508891290182809541 ) ) ;
#28405=CARTESIAN_POINT ( 'NONE',  ( 182.1470424277336804, 275.5479489297672444, -16.45731081755295477 ) ) ;
#28407=CARTESIAN_POINT ( 'NONE',  ( 206.1670584421323724, 273.5551752616418639, -11.23038754588519694 ) ) ;
#28408=CARTESIAN_POINT ( 'NONE',  ( 201.7502332754098120, 267.6057469551752206, 0.8447870975616070810 ) ) ;
#28409=CARTESIAN_POINT ( 'NONE',  ( 195.3076413944070566, 263.9809680824703833, 0.8396464432550897472 ) ) ;
#28413=CARTESIAN_POINT ( 'NONE',  ( 196.1609710299282767, 270.7725530739749047, 12.00615862555037161 ) ) ;
#28415=CARTESIAN_POINT ( 'NONE',  ( 190.7222376050763444, 300.3063896652212179, 3.365789908110941475 ) ) ;
#28419=B_SPLINE_CURVE_WITH_KNOTS ( 'NONE', 3,
 ( #90603, #75368, #22144, #61624 ),
 .UNSPECIFIED., .F., .F.,
 ( 4, 4 ),
 ( 0.008781669780308986456, 0.01506971286528496420 ),
 .UNSPECIFIED. ) ;
#28420=CARTESIAN_POINT ( 'NONE',  ( 197.9598023461055902, 287.7705598106892921, 18.23120408239484291 ) ) ;
#28421=CARTESIAN_POINT ( 'NONE',  ( 207.3536890771331116, 271.4998707120027461, 6.332947442802633553 ) ) ;
#28422=CARTESIAN_POINT ( 'NONE',  ( 138.9289912384832917, 241.0177522451417929, 5.000000000000051514 ) ) ;
#28423=CARTESIAN_POINT ( 'NONE',  ( 175.8485278518198527, 285.2463791769441173, -12.03390954887754383 ) ) ;
#28426=CARTESIAN_POINT ( 'NONE',  ( 198.9225589249066957, 286.1030165008847916, -17.03502353404871883 ) ) ;
#28427=CARTESIAN_POINT ( 'NONE',  ( 19.87790860953014160, 170.0327760586659451, 1.948934522072302763E-15 ) ) ;
#28428=B_SPLINE_CURVE_WITH_KNOTS ( 'NONE', 3,
 ( #37551, #35582, #13300, #91306 ),
 .UNSPECIFIED., .F., .F.,
 ( 4, 4 ),
 ( 0.04785166522048146798, 0.04887066958154937663 ),
 .UNSPECIFIED. ) ;
#28429=CARTESIAN_POINT ( 'NONE',  ( 177.5317288456356835, 258.4661256883071019, -10.34817642027781481 ) ) ;
#28432=CARTESIAN_POINT ( 'NONE',  ( 157.1850763439666139, 258.3944569110938687, -16.98181238659443437 ) ) ;
#28435=CARTESIAN_POINT ( 'NONE',  ( 167.4083242872330857, 256.8190524212876085, 14.60336118133068872 ) ) ;
#28436=CARTESIAN_POINT ( 'NONE',  ( 69.71912771937687126, 204.3927522451418497, 10.00000000000009592 ) ) ;
#28438=CARTESIAN_POINT ( 'NONE',  ( 150.5461004505574181, 269.8935004687035644, 13.73913105907748111 ) ) ;
#28439=EDGE_CURVE ( 'NONE', #70463, #37554, #63490, .T. ) ;
#28441=CARTESIAN_POINT ( 'NONE',  ( 56.45811372747557044, 196.7365022471902023, -10.00000000000009059 ) ) ;
#28442=CARTESIAN_POINT ( 'NONE',  ( 181.5699223927324795, 292.0049823800039803, 9.001579805457852856 ) ) ;
#28443=CARTESIAN_POINT ( 'NONE',  ( 147.7978300115112233, 274.6536445020713018, 7.902890709649431855 ) ) ;
#28445=CARTESIAN_POINT ( 'NONE',  ( 14.27519936121077926, 188.2369531367911293, -4.594050593750048428 ) ) ;
#28450=CARTESIAN_POINT ( 'NONE',  ( 201.8291755756830241, 280.5217801640038715, -16.04463949318729021 ) ) ;
#28451=CARTESIAN_POINT ( 'NONE',  ( 164.6649740431187183, 245.4388940607451843, -1.430729255012818557 ) ) ;
#28452=DIRECTION ( 'NONE',  ( -0.8660254037844387076, -0.4999999999999998890, -0.000000000000000000 ) ) ;
#28453=CARTESIAN_POINT ( 'NONE',  ( 153.5337505630658654, 266.4617915331671156, -16.61785508892420182 ) ) ;
#28457=CARTESIAN_POINT ( 'NONE',  ( 165.6111162920294362, 285.3959942432976504, 0.3651359175268718560 ) ) ;
#28461=LINE ( 'NONE', #20891, #51612 ) ;
#28464=CARTESIAN_POINT ( 'NONE',  ( 156.9140063554453377, 276.4170914181521539, 10.52199787263365494 ) ) ;
#28465=CARTESIAN_POINT ( 'NONE',  ( 206.2809287719926488, 273.3579460648492159, -10.70911012174624588 ) ) ;
#28466=ORIENTED_EDGE ( 'NONE', *, *, #45328, .F. ) ;
#28467=CARTESIAN_POINT ( 'NONE',  ( 195.5602278707908397, 290.3821284405168512, -16.61863160252172023 ) ) ;
#28470=CARTESIAN_POINT ( 'NONE',  ( 183.8754313647489198, 256.5225093191261294, -2.022205659181245174 ) ) ;
#28471=CARTESIAN_POINT ( 'NONE',  ( 154.9792334219179679, 262.2150889255981951, -17.21325849938693153 ) ) ;
#28474=CARTESIAN_POINT ( 'NONE',  ( 159.7144335965733433, 278.4664156918360050, -9.777473725360442458 ) ) ;
#28475=CARTESIAN_POINT ( 'NONE',  ( 204.8523313866422484, 275.8323493198358847, 14.65426965484541100 ) ) ;
#28476=CARTESIAN_POINT ( 'NONE',  ( 152.9262073036446168, 265.7710344717137900, 16.19159804214501008 ) ) ;
#28477=EDGE_LOOP ( 'NONE', ( #85325, #87017, #71483, #46219 ) ) ;
#28481=VERTEX_POINT ( 'NONE', #32603 ) ;
#28483=CARTESIAN_POINT ( 'NONE',  ( 196.6317700900902139, 290.0707791521982131, -17.91116578096951883 ) ) ;
#28485=CARTESIAN_POINT ( 'NONE',  ( 164.7462163020046262, 245.2981783406326599, 1.451255823150352064 ) ) ;
#28489=CARTESIAN_POINT ( 'NONE',  ( 174.4487371657580468, 277.2123390989709151, -15.64973371979014338 ) ) ;
#28490=CARTESIAN_POINT ( 'NONE',  ( 169.6261978958059728, 261.9618702208159675, -15.78807854465063798 ) ) ;
#28493=CARTESIAN_POINT ( 'NONE',  ( 147.2567621633200474, 275.5908015054806128, -3.647191014543873955 ) ) ;
#28496=CARTESIAN_POINT ( 'NONE',  ( 157.7366572918917882, 268.9116757437374758, 15.63315894949619178 ) ) ;
#28498=CARTESIAN_POINT ( 'NONE',  ( 156.2224770818481545, 267.4677849582849376, -16.91854127892884208 ) ) ;
#28499=CARTESIAN_POINT ( 'NONE',  ( 147.5848197185516142, 275.0225891520124151, 4.420251097676741736 ) ) ;
#28502=CARTESIAN_POINT ( 'NONE',  ( 153.3703256797887775, 265.0017988796566897, 16.44314709207578318 ) ) ;
#28503=CARTESIAN_POINT ( 'NONE',  ( 39.95181620016202118, 182.3262482093457209, 3.021315404115420679E-15 ) ) ;
#28504=CARTESIAN_POINT ( 'NONE',  ( 191.0478321355427624, 299.7424433957868928, -9.006798842970001218 ) ) ;
#28507=EDGE_CURVE ( 'NONE', #6045, #23996, #10132, .T. ) ;
#28509=CARTESIAN_POINT ( 'NONE',  ( 149.3801359649374092, 271.9130101976182914, -11.41245530317637424 ) ) ;
#28510=CARTESIAN_POINT ( 'NONE',  ( 165.0565241268390366, 244.7607094220335568, 2.191926263411719589 ) ) ;
#28513=CARTESIAN_POINT ( 'NONE',  ( 176.7429058980506227, 289.7743273258707291, -9.091347092446275369 ) ) ;
#28515=CARTESIAN_POINT ( 'NONE',  ( 149.4634369175186066, 271.7687287154290061, -11.52144114384952367 ) ) ;
#28518=CARTESIAN_POINT ( 'NONE',  ( 118.5773942495488882, 249.2677522451419065, -5.000000000000047962 ) ) ;
#28519=CARTESIAN_POINT ( 'NONE',  ( 159.8807525190996444, 253.7254088150106099, -15.62640036463813686 ) ) ;
#28520=CARTESIAN_POINT ( 'NONE',  ( 96.65612621980322672, 226.6115022471902307, 10.00000000000009592 ) ) ;
#28521=ORIENTED_EDGE ( 'NONE', *, *, #12641, .F. ) ;
#28522=CARTESIAN_POINT ( 'NONE',  ( 170.5265982536998592, 255.7106794591476557, -12.46252183393470858 ) ) ;
#28524=CARTESIAN_POINT ( 'NONE',  ( 207.1601050488701503, 271.8351680844880889, 6.320235450527015075 ) ) ;
#28525=EDGE_CURVE ( 'NONE', #11450, #76998, #4241, .T. ) ;
#28526=CARTESIAN_POINT ( 'NONE',  ( 40.63510790894947888, 184.2677522451417929, -5.000000000000041744 ) ) ;
#28527=CARTESIAN_POINT ( 'NONE',  ( 115.5194155920915620, 231.3768266524159856, 9.188101187500096856 ) ) ;
#28528=CARTESIAN_POINT ( 'NONE',  ( 181.1018697000030500, 294.2850109623373100, -2.647402609916298388 ) ) ;
#28529=CARTESIAN_POINT ( 'NONE',  ( 162.7502451860280530, 249.5826859877889490, -11.13675961672946713 ) ) ;
#28532=CARTESIAN_POINT ( 'NONE',  ( 25.77718602916411683, 191.8149278399160949, -9.188101187500095079 ) ) ;
#28536=ORIENTED_EDGE ( 'NONE', *, *, #77485, .F. ) ;
#28538=CARTESIAN_POINT ( 'NONE',  ( 181.1611384956651705, 267.7195240920720494, 14.99755381712351365 ) ) ;
#28542=B_SPLINE_CURVE_WITH_KNOTS ( 'NONE', 3,
 ( #33614, #86868, #64511, #87392, #42680, #32605, #55870, #95469, #26022, #56891, #17399, #48311, #87875, #18421, #79255, #49311, #26517, #80249, #3235, #57394, #88369, #18927, #9827, #43175, #45057, #7057, #68851, #15140, #69360, #37447, #35598, #85098, #53163, #35093, #74118, #61748, #89840, #37939, #22259, #76954, #45547, #23248, #4712, #22769, #58387, #53646, #84118, #99772, #100279, #75998 ),
 .UNSPECIFIED., .F., .F.,
 ( 4, 2, 2, 2, 2, 2, 2, 2, 2, 2, 2, 2, 2, 2, 2, 2, 2, 2, 2, 2, 2, 2, 2, 2, 4 ),
 ( 0.0001402968676236758798, 0.001130964830274715227, 0.001378631820937422162, 0.001626298811600129313, 0.001750132306931482997, 0.001873965802262836247, 0.001997799297594189932, 0.002121632792925543399, 0.002369299783588250767, 0.002616966774250957268, 0.003112300755576218915, 0.004102968718226588686, 0.005093636680876957590, 0.005588970662202106914, 0.005836637652864646447, 0.006084304643527185114, 0.006146221391192784218, 0.006208138138858384190, 0.006270054886523983295, 0.006331971634189583267, 0.006579638624852431582, 0.007074972606178260917, 0.007570306587504091987, 0.007817973578167001017, 0.008065640568829910914 ),
 .UNSPECIFIED. ) ;
#28543=CARTESIAN_POINT ( 'NONE',  ( 207.7296438747196134, 270.8486979012336633, -6.692930657757584001 ) ) ;
#28544=CARTESIAN_POINT ( 'NONE',  ( 178.1790154062099134, 287.6584321602529144, -13.04213889271035676 ) ) ;
#28545=CARTESIAN_POINT ( 'NONE',  ( 164.3713690399699772, 250.1140898715638627, 10.21268107768454492 ) ) ;
#28546=CARTESIAN_POINT ( 'NONE',  ( 93.89567024169240028, 225.0177522451418781, -10.00000000000009592 ) ) ;
#28547=ORIENTED_EDGE ( 'NONE', *, *, #16849, .T. ) ;
#28550=CARTESIAN_POINT ( 'NONE',  ( 157.6006514737650832, 281.0282930248237108, -1.590882658691914253 ) ) ;
#28551=CARTESIAN_POINT ( 'NONE',  ( 207.7625791259561652, 270.7916523727319031, -1.015623356719550063 ) ) ;
#28553=CARTESIAN_POINT ( 'NONE',  ( 18.14551070619625150, 181.2833772461660544, -9.188101187500095079 ) ) ;
#28557=CARTESIAN_POINT ( 'NONE',  ( 146.8574506849497538, 276.2824292740633041, -4.888313306692038118 ) ) ;
#28560=CARTESIAN_POINT ( 'NONE',  ( 60.66220569506229765, 196.6423013555410080, -4.594050593750043987 ) ) ;
#28561=CARTESIAN_POINT ( 'NONE',  ( 207.9622466093905189, 270.4458181468041289, 3.586592550214158681 ) ) ;
#28562=CARTESIAN_POINT ( 'NONE',  ( 203.6714976035736981, 276.2235336633698921, 13.32122003884233941 ) ) ;
#28567=( BOUNDED_CURVE ( )  B_SPLINE_CURVE ( 2, ( #57766, #89247, #73008, #20792, #80631, #82126, #13194, #3599, #19797 ),
 .UNSPECIFIED., .F., .T. ) 
 B_SPLINE_CURVE_WITH_KNOTS ( ( 3, 2, 2, 2, 3 ),
 ( 0.5120967741935483764, 0.5134408602150537515, 0.5161290322580645018, 0.5188172043010752521, 0.5201612903225806273 ),
 .UNSPECIFIED. ) 
 CURVE ( )  GEOMETRIC_REPRESENTATION_ITEM ( )  RATIONAL_B_SPLINE_CURVE ( ( 0.9330127018922194093, 0.9330127018922194093, 1.000000000000000000, 0.8660254037844387076, 1.000000000000000000, 0.8660254037844387076, 1.000000000000000000, 0.9330127018922194093, 0.9330127018922194093 ) ) 
 REPRESENTATION_ITEM ( '' )  );
#28568=CARTESIAN_POINT ( 'NONE',  ( 18.71383987920374992, 181.6115022471902591, 10.00000000000009592 ) ) ;
#28570=CARTESIAN_POINT ( 'NONE',  ( 137.4948102131217524, 244.0643266524159856, -9.188101187500093303 ) ) ;
#28572=CARTESIAN_POINT ( 'NONE',  ( 207.2266458903087312, 271.7199159663382488, -8.370253452505480141 ) ) ;
#28573=EDGE_CURVE ( 'NONE', #51377, #91972, #80412, .T. ) ;
#28576=CARTESIAN_POINT ( 'NONE',  ( 196.4677102463732012, 290.3549391369982686, 16.45225250689336249 ) ) ;
#28580=CARTESIAN_POINT ( 'NONE',  ( 151.4159295687746294, 268.3869122420484814, 14.78076517566594106 ) ) ;
#28581=CARTESIAN_POINT ( 'NONE',  ( 163.3647850011336971, 247.6908875409073403, 8.475775724498188168 ) ) ;
#28583=CARTESIAN_POINT ( 'NONE',  ( 169.7091093167843496, 266.1397787582689602, -16.87065449823908736 ) ) ;
#28584=CARTESIAN_POINT ( 'NONE',  ( 197.3149168070693520, 273.2883024837288417, -13.45903248082802506 ) ) ;
#28585=VERTEX_POINT ( 'NONE', #42678 ) ;
#28587=CARTESIAN_POINT ( 'NONE',  ( 168.4891346661264322, 282.2463884888330199, -10.92310856812336795 ) ) ;
#28590=CARTESIAN_POINT ( 'NONE',  ( 184.0101212780497235, 295.6693216559447706, 4.669920232876622279 ) ) ;
#28592=CARTESIAN_POINT ( 'NONE',  ( 148.1500140211902874, 275.9675759909871999, -0.0001745395379542502687 ) ) ;
#28593=CARTESIAN_POINT ( 'NONE',  ( 149.8363775701710381, 271.5102645707438000, -11.76379339081466568 ) ) ;
#28596=CARTESIAN_POINT ( 'NONE',  ( 166.7959447105422157, 276.3626885415273478, 15.91653206054683523 ) ) ;
#28598=CARTESIAN_POINT ( 'NONE',  ( -22.42236680055709641, 157.8615022471902591, 0.000000000000000000 ) ) ;
#28600=CARTESIAN_POINT ( 'NONE',  ( 156.0187427484829641, 261.9439754546441463, -16.96632779721737805 ) ) ;
#28602=CARTESIAN_POINT ( 'NONE',  ( 146.8859094598974480, 276.2331372299326517, -0.7994986043261681496 ) ) ;
#28603=CARTESIAN_POINT ( 'NONE',  ( 185.0260524818428678, 291.7194308270165948, 12.00076202787302826 ) ) ;
#28604=CARTESIAN_POINT ( 'NONE',  ( 164.2712161151136172, 246.1209027979328710, 7.276091357954241445 ) ) ;
#28609=CARTESIAN_POINT ( 'NONE',  ( 95.54687826519547400, 213.7202760586659167, -5.415160957724236172E-17 ) ) ;
#28610=CARTESIAN_POINT ( 'NONE',  ( 199.9134407114337364, 283.6250491837689651, 17.05367660732407842 ) ) ;
#28611=AXIS2_PLACEMENT_3D ( 'NONE', #17029, #63637, #84973 ) ;
#28612=CARTESIAN_POINT ( 'NONE',  ( 178.9462863553024761, 269.7444581634086376, -16.16615938913098205 ) ) ;
#28617=ORIENTED_EDGE ( 'NONE', *, *, #70776, .F. ) ;
#28619=B_SPLINE_CURVE_WITH_KNOTS ( 'NONE', 3,
 ( #29034, #98443, #21424, #52311 ),
 .UNSPECIFIED., .F., .F.,
 ( 4, 4 ),
 ( 0.003118693327000881740, 0.008537184786768493849 ),
 .UNSPECIFIED. ) ;
#28620=ORIENTED_EDGE ( 'NONE', *, *, #79413, .T. ) ;
#28622=CARTESIAN_POINT ( 'NONE',  ( 203.0026270830780675, 279.0361311525880978, -16.61345826058821373 ) ) ;
#28625=CARTESIAN_POINT ( 'NONE',  ( -22.42236680055709641, 157.8615022471902591, 0.000000000000000000 ) ) ;
#28626=CARTESIAN_POINT ( 'NONE',  ( 10.91961124514375925, 187.1115022471903160, -5.000000000000047962 ) ) ;
#28629=ORIENTED_EDGE ( 'NONE', *, *, #44370, .T. ) ;
#28633=EDGE_CURVE ( 'NONE', #51824, #59759, #82676, .T. ) ;
#28635=CARTESIAN_POINT ( 'NONE',  ( 167.4649754880705643, 284.0871937547507287, 9.157884509665418449 ) ) ;
#28636=CARTESIAN_POINT ( 'NONE',  ( 199.9084271263513983, 270.2648688396561738, 9.879193358459824381 ) ) ;
#28637=ORIENTED_EDGE ( 'NONE', *, *, #549, .T. ) ;
#28638=CARTESIAN_POINT ( 'NONE',  ( 203.0337691736598629, 278.9821914694464340, 16.08167820133810011 ) ) ;
#28640=CARTESIAN_POINT ( 'NONE',  ( 186.1788399154933416, 258.1552101551508827, 3.086633325358126623 ) ) ;
#28641=CARTESIAN_POINT ( 'NONE',  ( 161.3307343759124990, 281.5446215756635979, -6.416395075942769921 ) ) ;
#28642=DIRECTION ( 'NONE',  ( -0.8660254037844387076, -0.4999999999999998890, -0.000000000000000000 ) ) ;
#28646=EDGE_LOOP ( 'NONE', ( #72368, #72205, #67576, #58013 ) ) ;
#28647=CARTESIAN_POINT ( 'NONE',  ( 100.6254093204819497, 222.2365022471901739, -10.00000000000009237 ) ) ;
#28649=ORIENTED_EDGE ( 'NONE', *, *, #60897, .F. ) ;
#28650=CARTESIAN_POINT ( 'NONE',  ( 193.6136754191833234, 294.1685928848680760, -14.20288964755752126 ) ) ;
#28652=CARTESIAN_POINT ( 'NONE',  ( 171.6601131003222349, 279.7212932031995933, -14.57934018190033498 ) ) ;
#28653=CARTESIAN_POINT ( 'NONE',  ( 204.2488672143813346, 276.8775799267394291, -15.19253025301563831 ) ) ;
#28655=CARTESIAN_POINT ( 'NONE',  ( 164.7612133174728513, 274.2017939341284318, 14.96666266618639973 ) ) ;
#28656=CARTESIAN_POINT ( 'NONE',  ( -1.664820405372784862, 169.8458772461660544, 9.188101187500095079 ) ) ;
#28658=CARTESIAN_POINT ( 'NONE',  ( 185.1625343664165655, 295.6846680252337478, 8.558017805756747975 ) ) ;
#28661=ORIENTED_EDGE ( 'NONE', *, *, #71424, .F. ) ;
#28663=CARTESIAN_POINT ( 'NONE',  ( 190.1363311188550540, 273.6253742232181025, -15.77342137974315683 ) ) ;
#28664=B_SPLINE_CURVE_WITH_KNOTS ( 'NONE', 3,
 ( #79360, #87490, #41796, #40285 ),
 .UNSPECIFIED., .F., .F.,
 ( 4, 4 ),
 ( 0.01180092279712636506, 0.02028068562175033493 ),
 .UNSPECIFIED. ) ;
#28669=CARTESIAN_POINT ( 'NONE',  ( 153.1198285439165545, 279.2890930352092482, 3.903594709581249322 ) ) ;
#28671=CARTESIAN_POINT ( 'NONE',  ( -1.610867365518755978, 176.0024278399160949, 9.188101187500095079 ) ) ;
#28672=CARTESIAN_POINT ( 'NONE',  ( 124.1796696299359724, 236.3768266524159856, -9.188101187500091527 ) ) ;
#28674=CARTESIAN_POINT ( 'NONE',  ( 181.4013813872246317, 255.1929875330831123, -2.500114065624810866 ) ) ;
#28680=CARTESIAN_POINT ( 'NONE',  ( 193.7114073116034945, 295.1289958610702797, 14.86160832869823345 ) ) ;
#28681=CARTESIAN_POINT ( 'NONE',  ( 161.0965315767822972, 251.6196177163260188, -13.76772246540905442 ) ) ;
#28682=CARTESIAN_POINT ( 'NONE',  ( 194.4666154385731431, 293.8209370148700827, -14.56896502715340702 ) ) ;
#28684=EDGE_CURVE ( 'NONE', #20915, #14295, #90767, .T. ) ;
#28685=EDGE_CURVE ( 'NONE', #80346, #38805, #70404, .T. ) ;
#28688=CARTESIAN_POINT ( 'NONE',  ( 192.7212156920602411, 265.2891116966523555, 7.789557535538737199 ) ) ;
#28690=CARTESIAN_POINT ( 'NONE',  ( 162.3216050867536353, 251.8533766904920128, -12.94731468463284330 ) ) ;
#28691=DIRECTION ( 'NONE',  ( -0.8660254037844387076, -0.4999999999999998890, -0.000000000000000000 ) ) ;
#28692=EDGE_CURVE ( 'NONE', #37486, #2973, #98233, .T. ) ;
#28693=AXIS2_PLACEMENT_3D ( 'NONE', #17579, #40854, #38843 ) ;
#28695=B_SPLINE_CURVE_WITH_KNOTS ( 'NONE', 3,
 ( #57779, #80642, #12710, #65882, #43063, #5583, #27401, #42570, #81143, #4591, #51175, #88755, #34979, #59257, #98304, #11709, #81628, #20299, #19327, #35975, #82140, #43581, #11219, #74005, #90235, #50190, #73503, #44063, #20804, #4087, #58282, #89258, #73018, #12201, #34488, #57281, #42086, #51697, #82647, #19808, #66878, #50675, #96331, #97318, #74515, #3610, #13205, #65389, #35485, #27886 ),
 .UNSPECIFIED., .F., .F.,
 ( 4, 2, 2, 2, 2, 2, 2, 2, 2, 2, 2, 2, 2, 2, 2, 2, 2, 2, 2, 2, 2, 2, 2, 2, 4 ),
 ( 0.0001844887274763776805, 0.001204547440118925936, 0.001714576796440233199, 0.001842084135520550203, 0.001969591474600867424, 0.002097098813681184427, 0.002224606152761501865, 0.002479620830922128066, 0.002734635509082753834, 0.003244664865404003201, 0.004264723578046429944, 0.005284782290688856687, 0.005794811647010033630, 0.006049826325170582636, 0.006304841003331129907, 0.006368594672871270845, 0.006432348342411410916, 0.006496102011951550986, 0.006559855681491691057, 0.006814870359652014549, 0.007324899715972662401, 0.007579914394132985893, 0.007834929072293307650, 0.008089943750453632010, 0.008344958428613956369 ),
 .UNSPECIFIED. ) ;
#28696=CARTESIAN_POINT ( 'NONE',  ( 88.83448719433606300, 234.3464784336661353, 1.353441290958777327E-15 ) ) ;
#28699=CARTESIAN_POINT ( 'NONE',  ( 150.6571681785161445, 269.7011255207979730, 15.24894850018880454 ) ) ;
#28700=EDGE_CURVE ( 'NONE', #73728, #56872, #34965, .T. ) ;
#28702=CARTESIAN_POINT ( 'NONE',  ( 157.2168982216852555, 258.3393398020932636, 18.09635675623264106 ) ) ;
#28703=CARTESIAN_POINT ( 'NONE',  ( 199.8015111840774125, 284.5806265305737952, 18.33369416908775662 ) ) ;
#28705=CARTESIAN_POINT ( 'NONE',  ( 203.8348497297200765, 275.8166909402214628, -13.89836469095587823 ) ) ;
#28712=CARTESIAN_POINT ( 'NONE',  ( 172.4964346338612984, 290.8364761718990508, -0.5259165075563734248 ) ) ;
#28713=CARTESIAN_POINT ( 'NONE',  ( 147.5749551500760788, 275.0396750858066639, -4.254929048021584670 ) ) ;
#28714=CARTESIAN_POINT ( 'NONE',  ( 191.7192842763342071, 288.0556307037572310, -15.81806397776715301 ) ) ;
#28715=B_SPLINE_CURVE_WITH_KNOTS ( 'NONE', 3,
 ( #60736, #37448, #14173, #45548, #76481, #68358, #23249, #92218, #54642, #38949, #54137, #99773, #70355, #69361, #91698, #61749, #77479, #100280, #29865, #7555, #39436, #967, #15646, #62747, #45058, #92699, #93703, #76955, #8076, #22261, #69854, #53647, #23746, #467, #84603, #30366, #37940, #46038, #16163, #7058, #31356, #55143, #47061, #75999, #68852, #30866, #62239, #77974, #24266, #99283 ),
 .UNSPECIFIED., .F., .F.,
 ( 4, 2, 2, 2, 2, 2, 2, 2, 2, 2, 2, 2, 2, 2, 2, 2, 2, 2, 2, 2, 2, 2, 2, 2, 4 ),
 ( 0.0001446224335138595609, 0.0006466149904454740081, 0.001148607547377088591, 0.001399603825842918054, 0.001650600104308747517, 0.001776098243541699437, 0.001901596382774651574, 0.002027094522007603494, 0.002152592661240555413, 0.002403588939706498718, 0.002654585218172442456, 0.003156577775104445292, 0.004160562888968516448, 0.005164548002832586304, 0.005666540559764621232, 0.005917536838230639563, 0.006043034977463642224, 0.006168533116696644884, 0.006231282186313106750, 0.006294031255929570350, 0.006419529395162546989, 0.006670525673628498534, 0.007172518230560363459, 0.007674510787492226649, 0.008176503344424091574 ),
 .UNSPECIFIED. ) ;
#28716=EDGE_CURVE ( 'NONE', #39441, #55671, #22672, .T. ) ;
#28717=EDGE_CURVE ( 'NONE', #21425, #53525, #91942, .T. ) ;
#28720=CARTESIAN_POINT ( 'NONE',  ( 159.9014600375868440, 253.6895423408921886, 15.57825579621527368 ) ) ;
#28721=CARTESIAN_POINT ( 'NONE',  ( 157.7933305902885195, 268.4007073483575141, 16.64277213758561658 ) ) ;
#28722=CARTESIAN_POINT ( 'NONE',  ( 170.0991740787100923, 252.5905740194307327, -8.760565947542348297 ) ) ;
#28723=CARTESIAN_POINT ( 'NONE',  ( 137.7923328995641157, 240.3615022471902023, 5.000000000000051514 ) ) ;
#28724=CARTESIAN_POINT ( 'NONE',  ( 157.8043799545718286, 257.3217915922150496, -17.97575562758749257 ) ) ;
#28725=AXIS2_PLACEMENT_3D ( 'NONE', #82594, #13160, #29835 ) ;
#28726=ORIENTED_EDGE ( 'NONE', *, *, #22460, .F. ) ;
#28728=ORIENTED_EDGE ( 'NONE', *, *, #63552, .T. ) ;
#28730=CYLINDRICAL_SURFACE ( 'NONE', #20672, 17.82106496071139645 ) ;
#28734=CARTESIAN_POINT ( 'NONE',  ( 163.2942584940569191, 258.1478583562382028, 16.77787020301746779 ) ) ;
#28735=CARTESIAN_POINT ( 'NONE',  ( 158.4880851235930947, 256.1375795020725263, 17.48246009260925860 ) ) ;
#28737=CARTESIAN_POINT ( 'NONE',  ( 193.0920876067732195, 296.2016890559648914, -13.46848876679793072 ) ) ;
#28747=CARTESIAN_POINT ( 'NONE',  ( 174.2782839474101877, 256.8459632085913995, -12.31768510484773493 ) ) ;
#28748=CARTESIAN_POINT ( 'NONE',  ( 147.6264044922760377, 274.9505622111005323, -8.841872555777701592 ) ) ;
#28749=CARTESIAN_POINT ( 'NONE',  ( 204.1162911604698138, 275.2177209574938388, 13.42500254428782114 ) ) ;
#28754=CARTESIAN_POINT ( 'NONE',  ( 171.0032295034350511, 287.8336240595702407, -4.402522906269554781 ) ) ;
#28756=CARTESIAN_POINT ( 'NONE',  ( 195.1474640768281290, 265.6393084148356252, -8.887799905196541062 ) ) ;
#28757=CARTESIAN_POINT ( 'NONE',  ( 100.0117143358702236, 237.7369531367911009, -4.594050593750048428 ) ) ;
#28760=CARTESIAN_POINT ( 'NONE',  ( 165.6389704105113481, 271.1804200721081202, 16.38369493522007758 ) ) ;
#28761=CARTESIAN_POINT ( 'NONE',  ( 190.8551004859573084, 274.8686381574206621, 15.92302825397800703 ) ) ;
#28762=VERTEX_POINT ( 'NONE', #27874 ) ;
#28763=VERTEX_POINT ( 'NONE', #89726 ) ;
#28766=B_SPLINE_SURFACE_WITH_KNOTS ( 'NONE', 3, 1, ( 
 ( #31911, #79574 ),
 ( #2032, #95285 ),
 ( #59185, #51104 ),
 ( #81076, #82069 ),
 ( #18735, #43509 ),
 ( #74448, #50123 ),
 ( #88686, #35910 ),
 ( #97739, #51619 ),
 ( #11151, #42020 ),
 ( #72954, #11642 ),
 ( #42501, #34906 ),
 ( #96766, #92522 ),
 ( #36401, #70169 ),
 ( #62060, #16480 ),
 ( #53476, #30184 ),
 ( #78299, #15981 ),
 ( #92040, #39257 ),
 ( #15464, #7897 ),
 ( #70678, #69678 ),
 ( #31663, #32176 ),
 ( #63080, #13136 ),
 ( #11411, #63579 ),
 ( #3309, #9902 ),
 ( #88449, #56478 ),
 ( #55953, #86949 ),
 ( #26093, #34674 ),
 ( #19008, #65576 ),
 ( #17482, #96524 ),
 ( #86446, #40760 ),
 ( #78799, #18000 ),
 ( #9386, #43761 ),
 ( #59446, #50869 ),
 ( #43260, #90925 ),
 ( #50374, #51366 ) ),
 .UNSPECIFIED., .T., .F., .F.,
 ( 4, 2, 2, 2, 2, 2, 2, 2, 2, 2, 2, 2, 2, 2, 2, 2, 4 ),
 ( 2, 2 ),
 ( 0.000000000000000000, 0.06250000000000000000, 0.1250000000000000000, 0.1875000000000000000, 0.2500000000000000000, 0.3125000000000000000, 0.3750000000000000000, 0.4375000000000000000, 0.5000000000000000000, 0.5625000000000000000, 0.6250000000000000000, 0.6875000000000000000, 0.7500000000000000000, 0.8125000000000000000, 0.8750000000000000000, 0.9375000000000000000, 1.000000000000000000 ),
 ( 0.000000000000000000, 1.000000000000000000 ),
 .UNSPECIFIED. ) ;
#28767=CARTESIAN_POINT ( 'NONE',  ( 157.8849654228661166, 257.1822134667773980, 17.43614750057631468 ) ) ;
#28768=CARTESIAN_POINT ( 'NONE',  ( 159.2122473525774069, 254.8832937285494609, -16.22689353966294590 ) ) ;
#28771=ORIENTED_EDGE ( 'NONE', *, *, #33847, .T. ) ;
#28775=AXIS2_PLACEMENT_3D ( 'NONE', #76690, #62983, #84332 ) ;
#28777=CARTESIAN_POINT ( 'NONE',  ( 96.42157766939700991, 233.1427522451419065, -10.00000000000009592 ) ) ;
#28778=CARTESIAN_POINT ( 'NONE',  ( 192.2881909306969135, 261.2467072465593105, -0.09875216535559103170 ) ) ;
#28779=CARTESIAN_POINT ( 'NONE',  ( 186.7564666940997711, 290.4926955665019932, -13.42819013091626523 ) ) ;
#28782=ORIENTED_EDGE ( 'NONE', *, *, #84009, .F. ) ;
#28784=CARTESIAN_POINT ( 'NONE',  ( 204.8176812644112204, 275.8923650920285695, 14.65594551021579051 ) ) ;
#28785=B_SPLINE_SURFACE_WITH_KNOTS ( 'NONE', 3, 1, ( 
 ( #4644, #27931 ),
 ( #12762, #22328 ),
 ( #98356, #76062 ),
 ( #97365, #53228 ),
 ( #29434, #51222 ),
 ( #74056, #98858 ),
 ( #29928, #91762 ),
 ( #20857, #58815 ),
 ( #28945, #45124 ),
 ( #51749, #89777 ),
 ( #99349, #66440 ),
 ( #6131, #60803 ),
 ( #83675, #35537 ),
 ( #75546, #82691 ),
 ( #20353, #37515 ),
 ( #6641, #82191 ),
 ( #28426, #83169 ),
 ( #59822, #43627 ),
 ( #75054, #68422 ),
 ( #52716, #12254 ),
 ( #66925, #14238 ),
 ( #43111, #67936 ),
 ( #74566, #5144 ),
 ( #36025, #60309 ),
 ( #97856, #5630 ),
 ( #21831, #90788 ),
 ( #59308, #37028 ),
 ( #36524, #90288 ),
 ( #13257, #44117 ),
 ( #67424, #21339 ),
 ( #52224, #44610 ),
 ( #13732, #91266 ),
 ( #1547, #85690 ),
 ( #53710, #47119 ) ),
 .UNSPECIFIED., .T., .F., .F.,
 ( 4, 2, 2, 2, 2, 2, 2, 2, 2, 2, 2, 2, 2, 2, 2, 2, 4 ),
 ( 2, 2 ),
 ( 0.000000000000000000, 0.06250000000000000000, 0.1250000000000000000, 0.1875000000000000000, 0.2500000000000000000, 0.3125000000000000000, 0.3750000000000000000, 0.4375000000000000000, 0.5000000000000000000, 0.5625000000000000000, 0.6250000000000000000, 0.6875000000000000000, 0.7500000000000000000, 0.8125000000000000000, 0.8750000000000000000, 0.9375000000000000000, 1.000000000000000000 ),
 ( 0.000000000000000000, 1.000000000000000000 ),
 .UNSPECIFIED. ) ;
#28787=CARTESIAN_POINT ( 'NONE',  ( 190.3734512952871967, 263.7599240487260204, -9.676642372964348482 ) ) ;
#28788=CARTESIAN_POINT ( 'NONE',  ( 170.4175250103361066, 248.6523554852190330, -0.2712260920720951929 ) ) ;
#28791=EDGE_CURVE ( 'NONE', #14425, #26183, #28567, .T. ) ;
#28792=CARTESIAN_POINT ( 'NONE',  ( 199.0994567031226836, 281.8932881784735969, -16.60211735284051215 ) ) ;
#28796=CARTESIAN_POINT ( 'NONE',  ( 206.5441577893546992, 271.9902398542315609, 7.330342545849478419 ) ) ;
#28797=CARTESIAN_POINT ( 'NONE',  ( 62.52896555438372417, 219.1589784336661637, -6.496448406907675876E-16 ) ) ;
#28798=CARTESIAN_POINT ( 'NONE',  ( 159.3451320108506764, 254.6531307488737355, -16.72997986213134425 ) ) ;
#28800=CARTESIAN_POINT ( 'NONE',  ( 163.0424334805279045, 248.2492167524936804, -9.671494865076915914 ) ) ;
#28802=CARTESIAN_POINT ( 'NONE',  ( 161.2488013048736377, 251.3558788108169040, -13.10044423494716170 ) ) ;
#28806=CARTESIAN_POINT ( 'NONE',  ( 113.4714528099510744, 242.9865022471902876, -10.00000000000009592 ) ) ;
#28809=CARTESIAN_POINT ( 'NONE',  ( 157.6838031512220368, 270.7765766995603940, -14.92570125826960847 ) ) ;
#28812=CARTESIAN_POINT ( 'NONE',  ( 30.97368554763575688, 182.5643266524159856, -9.188101187500093303 ) ) ;
#28814=B_SPLINE_CURVE_WITH_KNOTS ( 'NONE', 3,
 ( #46218, #23934, #77667, #93890 ),
 .UNSPECIFIED., .F., .F.,
 ( 4, 4 ),
 ( 0.009363228237252623279, 0.01502890388146836675 ),
 .UNSPECIFIED. ) ;
#28815=EDGE_CURVE ( 'NONE', #73927, #75268, #12482, .T. ) ;
#28816=CARTESIAN_POINT ( 'NONE',  ( 157.4177733328310467, 257.9914139036126812, 18.29188238796808363 ) ) ;
#28817=CARTESIAN_POINT ( 'NONE',  ( 199.4570567059534767, 277.6076089953632504, 15.22630486869836908 ) ) ;
#28819=CARTESIAN_POINT ( 'NONE',  ( 197.6456421031980994, 287.3858497455466932, 17.15283754821559015 ) ) ;
#28821=CARTESIAN_POINT ( 'NONE',  ( 45.45211389745056607, 206.2369531367911293, -4.594050593750048428 ) ) ;
#28822=B_SPLINE_CURVE_WITH_KNOTS ( 'NONE', 3,
 ( #72654, #47800, #16911, #94456 ),
 .UNSPECIFIED., .F., .F.,
 ( 4, 4 ),
 ( 0.007537832009283896087, 0.01334040069055882592 ),
 .UNSPECIFIED. ) ;
#28825=CARTESIAN_POINT ( 'NONE',  ( 171.5036904379427654, 286.7056378984830758, 7.451739084606072261 ) ) ;
#28828=CARTESIAN_POINT ( 'NONE',  ( 202.9431422976768715, 270.0791902996022031, -6.592389727497273810 ) ) ;
#28829=CARTESIAN_POINT ( 'NONE',  ( 176.0175147867288672, 291.2181479268968474, 2.555819555636972940 ) ) ;
#28830=AXIS2_PLACEMENT_3D ( 'NONE', #3729, #87401, #58395 ) ;
#28831=ADVANCED_FACE ( 'NONE', ( #57269 ), #12188, .T. ) ;
#28832=CARTESIAN_POINT ( 'NONE',  ( 180.1023429053202847, 276.2675729333262780, 17.20643721484194799 ) ) ;
#28833=CARTESIAN_POINT ( 'NONE',  ( 182.2148741171517088, 280.9993675977776206, -17.23122524679219225 ) ) ;
#28835=CARTESIAN_POINT ( 'NONE',  ( 163.3019570347943841, 255.9604400728466373, -14.88202733670140887 ) ) ;
#28839=CARTESIAN_POINT ( 'NONE',  ( 100.4810717531844944, 235.4865022471902876, -10.00000000000009415 ) ) ;
#28840=CARTESIAN_POINT ( 'NONE',  ( 161.1027382213887336, 251.6088674925233022, 13.55451100897754557 ) ) ;
#28841=CARTESIAN_POINT ( 'NONE',  ( 164.8959392045564982, 270.4400157944439798, -16.73020286746915630 ) ) ;
#28842=ORIENTED_EDGE ( 'NONE', *, *, #54076, .T. ) ;
#28843=CARTESIAN_POINT ( 'NONE',  ( 55.76366273096530080, 196.8768266524160140, 9.188101187500098632 ) ) ;
#28845=CARTESIAN_POINT ( 'NONE',  ( 166.5588711558999364, 264.7233108584221100, 17.65853493413723641 ) ) ;
#28848=ORIENTED_EDGE ( 'NONE', *, *, #1251, .T. ) ;
#28850=CYLINDRICAL_SURFACE ( 'NONE', #2046, 17.82106496071139645 ) ;
#28852=CARTESIAN_POINT ( 'NONE',  ( 193.9796946036068164, 292.6643086402947915, -15.64068455845557537 ) ) ;
#28853=CARTESIAN_POINT ( 'NONE',  ( 176.9539730356219138, 274.6341514097922527, -16.77391188311105452 ) ) ;
#28855=CARTESIAN_POINT ( 'NONE',  ( 204.7088172315186512, 276.0809231281156144, 13.09496711537969027 ) ) ;
#28860=CARTESIAN_POINT ( 'NONE',  ( 167.3911405578172946, 287.7797177684797134, -2.777254742693934020 ) ) ;
#28864=CARTESIAN_POINT ( 'NONE',  ( 166.9564976376358061, 261.4857389862473269, 16.50069698162775467 ) ) ;
#28865=CARTESIAN_POINT ( 'NONE',  ( 159.2289198208967775, 254.8544161663325838, -15.88961297684315888 ) ) ;
#28866=EDGE_LOOP ( 'NONE', ( #1858, #47831 ) ) ;
#28867=VERTEX_POINT ( 'NONE', #99287 ) ;
#28870=CARTESIAN_POINT ( 'NONE',  ( 61.98910963369213789, 195.0494855054051584, -2.679491924311248496 ) ) ;
#28871=CARTESIAN_POINT ( 'NONE',  ( 162.6757594134126350, 248.8843148665554281, -10.86406770146305867 ) ) ;
#28873=CARTESIAN_POINT ( 'NONE',  ( 176.3865323452404823, 258.8737835494043225, 13.24306684835586623 ) ) ;
#28875=CARTESIAN_POINT ( 'NONE',  ( 161.0313979157349991, 262.9719707653000000, -17.46358780386706400 ) ) ;
#28876=EDGE_CURVE ( 'NONE', #33752, #34753, #44716, .T. ) ;
#28877=CARTESIAN_POINT ( 'NONE',  ( 120.4987145680870952, 246.5024278399160949, 9.188101187500095079 ) ) ;
#28879=VERTEX_POINT ( 'NONE', #98797 ) ;
#28880=CARTESIAN_POINT ( 'NONE',  ( 170.1749377657032198, 264.1434158296717101, 16.24854282405526718 ) ) ;
#28883=VERTEX_POINT ( 'NONE', #45063 ) ;
#28884=CARTESIAN_POINT ( 'NONE',  ( 201.0536821592508829, 281.7069444607843138, 16.57790100734148453 ) ) ;
#28885=EDGE_LOOP ( 'NONE', ( #22772, #90427, #71121, #54766, #28352 ) ) ;
#28889=CARTESIAN_POINT ( 'NONE',  ( 194.4891008911482118, 284.8786197582770114, 17.21347455856521691 ) ) ;
#28891=( BOUNDED_CURVE ( )  B_SPLINE_CURVE ( 2, ( #68839, #31344, #55129, #84590, #75986, #85608, #15632, #15128, #77962 ),
 .UNSPECIFIED., .F., .T. ) 
 B_SPLINE_CURVE_WITH_KNOTS ( ( 3, 2, 2, 2, 3 ),
 ( 0.9233870967741935054, 0.9247311827956988806, 0.9274193548387096309, 0.9301075268817203812, 0.9314516129032257563 ),
 .UNSPECIFIED. ) 
 CURVE ( )  GEOMETRIC_REPRESENTATION_ITEM ( )  RATIONAL_B_SPLINE_CURVE ( ( 0.9330127018922194093, 0.9330127018922194093, 1.000000000000000000, 0.8660254037844387076, 1.000000000000000000, 0.8660254037844387076, 1.000000000000000000, 0.9330127018922194093, 0.9330127018922194093 ) ) 
 REPRESENTATION_ITEM ( '' )  );
#28893=CARTESIAN_POINT ( 'NONE',  ( 155.1376601545389917, 261.9406857754215707, 18.55063430030667959 ) ) ;
#28898=CARTESIAN_POINT ( 'NONE',  ( 201.2535035105529744, 282.0657020489176716, -18.08976065250591958 ) ) ;
#28899=CARTESIAN_POINT ( 'NONE',  ( 155.6569868912636991, 261.0411854816857158, -17.75433477650897984 ) ) ;
#28904=CARTESIAN_POINT ( 'NONE',  ( 164.1492509520389831, 246.7605600116641540, 4.961886042938450814 ) ) ;
#28909=CARTESIAN_POINT ( 'NONE',  ( 164.7297297678022403, 245.3267338555121455, 3.020078936458732599 ) ) ;
#28910=CARTESIAN_POINT ( 'NONE',  ( 195.2792143904551949, 279.2177904473068679, 16.31973602825316405 ) ) ;
#28911=CARTESIAN_POINT ( 'NONE',  ( 164.1146561143383167, 246.3920726737087534, -7.362905700427413436 ) ) ;
#28913=CARTESIAN_POINT ( 'NONE',  ( 141.8249372320439647, 246.5643266524160140, 9.188101187500095079 ) ) ;
#28918=EDGE_CURVE ( 'NONE', #24285, #690, #63239, .T. ) ;
#28920=EDGE_CURVE ( 'NONE', #91209, #17524, #89835, .T. ) ;
#28921=CARTESIAN_POINT ( 'NONE',  ( 178.4631826488540867, 254.6961106986615562, 4.321611361837887522 ) ) ;
#28922=VERTEX_POINT ( 'NONE', #46549 ) ;
#28928=CARTESIAN_POINT ( 'NONE',  ( 182.3988913246011521, 262.5264951803217741, -13.38846801953669008 ) ) ;
#28929=CARTESIAN_POINT ( 'NONE',  ( 147.5848197185516142, 275.0225891520124151, 4.420251097676741736 ) ) ;
#28930=CARTESIAN_POINT ( 'NONE',  ( 182.8533132515951536, 280.6317719585726422, 16.86240594373356672 ) ) ;
#28931=CARTESIAN_POINT ( 'NONE',  ( 204.7764732025852084, 275.9637395487929439, -14.02287343454361412 ) ) ;
#28932=CARTESIAN_POINT ( 'NONE',  ( 192.8825254575952499, 268.5331795959783676, 12.33565966346110265 ) ) ;
#28936=DIRECTION ( 'NONE',  ( 0.4999999999999998890, -0.8660254037844385966, 0.000000000000000000 ) ) ;
#28937=CARTESIAN_POINT ( 'NONE',  ( 159.6610344727618269, 254.1059716346071866, 15.33388637456589620 ) ) ;
#28938=CARTESIAN_POINT ( 'NONE',  ( 207.2594843487139542, 271.6630380879379345, 5.140243983758119306 ) ) ;
#28940=CARTESIAN_POINT ( 'NONE',  ( -10.43332761869022640, 164.7833772461660544, -9.188101187500095079 ) ) ;
#28941=CARTESIAN_POINT ( 'NONE',  ( 175.3356445731998008, 284.9523473448756477, -12.04348899028328468 ) ) ;
#28942=ORIENTED_EDGE ( 'NONE', *, *, #65390, .T. ) ;
#28945=CARTESIAN_POINT ( 'NONE',  ( 199.2205425252482200, 285.5868937652708155, -18.05012564782189344 ) ) ;
#28946=CARTESIAN_POINT ( 'NONE',  ( 12.08367997547019002, 165.5327760586659451, 1.948934522072302763E-15 ) ) ;
#28947=CARTESIAN_POINT ( 'NONE',  ( 181.8637735408910316, 276.0006342513588606, -16.50086996363865666 ) ) ;
#28950=CARTESIAN_POINT ( 'NONE',  ( 71.81202244518927102, 202.2677522451417929, -5.000000000000041744 ) ) ;
#28953=CARTESIAN_POINT ( 'NONE',  ( 196.3825633952734790, 269.6078319146020021, -10.80602553522919251 ) ) ;
#28954=EDGE_CURVE ( 'NONE', #94086, #99632, #68073, .T. ) ;
#28956=CARTESIAN_POINT ( 'NONE',  ( 198.0167861310041530, 287.6718610000373246, 18.15276047493383160 ) ) ;
#28957=CARTESIAN_POINT ( 'NONE',  ( 180.3483110632917885, 294.3099715515549519, 1.024573422989016880 ) ) ;
#28958=CARTESIAN_POINT ( 'NONE',  ( 48.51954752611815991, 205.4865022471903444, -10.00000000000009415 ) ) ;
#28960=CARTESIAN_POINT ( 'NONE',  ( 190.5444288681022442, 300.6143634316900943, -1.000014190476072873 ) ) ;
#28962=CARTESIAN_POINT ( 'NONE',  ( 11.05475416482865114, 183.3149278399160664, 9.188101187500093303 ) ) ;
#28963=CARTESIAN_POINT ( 'NONE',  ( 164.2764444823383769, 284.8899537207625485, 4.278381809041608363 ) ) ;
#28966=CARTESIAN_POINT ( 'NONE',  ( 202.1632097545547424, 279.9122701607644785, -15.78860785990872451 ) ) ;
#28968=CARTESIAN_POINT ( 'NONE',  ( 164.6460902696047128, 245.4716017159096566, -3.036414139157908476 ) ) ;
#28969=DIRECTION ( 'NONE',  ( 0.5000000000000048850, -0.8660254037844358210, 0.000000000000000000 ) ) ;
#28971=CARTESIAN_POINT ( 'NONE',  ( 161.8743800460768796, 280.4803551579017267, 8.950406917861062794 ) ) ;
#28974=EDGE_CURVE ( 'NONE', #57520, #64780, #60740, .T. ) ;
#28979=CARTESIAN_POINT ( 'NONE',  ( 155.6518451030846961, 261.0500913200531841, 17.91778754207898317 ) ) ;
#28980=ORIENTED_EDGE ( 'NONE', *, *, #44182, .T. ) ;
#28985=ORIENTED_EDGE ( 'NONE', *, *, #29297, .F. ) ;
#28986=CARTESIAN_POINT ( 'NONE',  ( 196.2472167001637899, 289.0877869373891826, -17.11100897825607348 ) ) ;
#28989=CARTESIAN_POINT ( 'NONE',  ( 154.9528145190857344, 262.2608478075840708, -17.26679351315302213 ) ) ;
#28992=ORIENTED_EDGE ( 'NONE', *, *, #86110, .F. ) ;
#28996=CARTESIAN_POINT ( 'NONE',  ( 152.6757560589063303, 266.2048287524194166, 16.73757896668104195 ) ) ;
#29000=CARTESIAN_POINT ( 'NONE',  ( 16.79905537663784898, 192.0530062829863311, -4.648177544792955347E-16 ) ) ;
#29002=ORIENTED_EDGE ( 'NONE', *, *, #38710, .T. ) ;
#29004=CARTESIAN_POINT ( 'NONE',  ( 197.0226655822963551, 289.3937282992477549, -17.28982543158101493 ) ) ;
#29006=ORIENTED_EDGE ( 'NONE', *, *, #46394, .F. ) ;
#29007=CARTESIAN_POINT ( 'NONE',  ( 206.2456893945931142, 273.4189824569319285, 10.13882547285618152 ) ) ;
#29010=ORIENTED_EDGE ( 'NONE', *, *, #54181, .F. ) ;
#29011=CARTESIAN_POINT ( 'NONE',  ( 174.6285408418798966, 276.7099930269583865, -16.43498402137660364 ) ) ;
#29012=CARTESIAN_POINT ( 'NONE',  ( 172.2074374934617822, 264.1263164429906283, -15.87731566018440965 ) ) ;
#29013=ORIENTED_EDGE ( 'NONE', *, *, #99963, .F. ) ;
#29014=CARTESIAN_POINT ( 'NONE',  ( 158.6437384181921573, 274.8702825545737483, -13.55642847048332200 ) ) ;
#29017=ORIENTED_EDGE ( 'NONE', *, *, #5586, .T. ) ;
#29021=CARTESIAN_POINT ( 'NONE',  ( 147.1249913145849177, 275.8190353104462815, 3.637773609013635223 ) ) ;
#29022=CARTESIAN_POINT ( 'NONE',  ( 188.6203220463457626, 298.5727710222585074, -4.346736981754744100 ) ) ;
#29023=CARTESIAN_POINT ( 'NONE',  ( 148.9694607950094394, 272.6243204573405592, 11.81236034532910573 ) ) ;
#29024=CARTESIAN_POINT ( 'NONE',  ( 152.9920137376499838, 265.6570543845515431, 16.15798175643282164 ) ) ;
#29025=CARTESIAN_POINT ( 'NONE',  ( 191.4409630708763927, 299.0615206417621721, 9.874182956795676702 ) ) ;
#29026=CARTESIAN_POINT ( 'NONE',  ( 191.6723191112861855, 298.6608002251342100, -9.737039817265848995 ) ) ;
#29030=CARTESIAN_POINT ( 'NONE',  ( 149.7200635338602410, 271.3242383773507527, -12.12223662813266500 ) ) ;
#29033=CARTESIAN_POINT ( 'NONE',  ( 168.4907652997964931, 286.4387392943589816, 4.072501019507571485 ) ) ;
#29034=CARTESIAN_POINT ( 'NONE',  ( 163.8070446421170629, 255.0663642890118581, -15.42060242571707818 ) ) ;
#29035=ORIENTED_EDGE ( 'NONE', *, *, #54003, .F. ) ;
#29036=CARTESIAN_POINT ( 'NONE',  ( 205.7456069296021894, 269.2916946144356416, -2.908540672199198429 ) ) ;
#29038=CARTESIAN_POINT ( 'NONE',  ( 148.7862567239304781, 273.6578808824901898, 8.926082407994170964 ) ) ;
#29041=CARTESIAN_POINT ( 'NONE',  ( 180.3999454879367192, 283.0679475345629612, -15.21805286706472060 ) ) ;
#29042=ADVANCED_FACE ( 'NONE', ( #14674 ), #30870, .T. ) ;
#29045=CARTESIAN_POINT ( 'NONE',  ( 208.3764315856425640, 269.7284287242038658, -1.833640725398759441 ) ) ;
#29047=EDGE_CURVE ( 'NONE', #78500, #77084, #16042, .T. ) ;
#29048=CARTESIAN_POINT ( 'NONE',  ( 164.9836323268835940, 244.8869617230113249, -2.696511969808454534 ) ) ;
#29050=CARTESIAN_POINT ( 'NONE',  ( 57.45043449909734079, 190.6427522451417644, 1.119607411625061291E-15 ) ) ;
#29051=CARTESIAN_POINT ( 'NONE',  ( 118.9835172072293403, 233.3768266524159571, -9.188101187500093303 ) ) ;
#29055=CARTESIAN_POINT ( 'NONE',  ( 192.7874605187217014, 292.5376213369709149, 15.36506066506490598 ) ) ;
#29056=CARTESIAN_POINT ( 'NONE',  ( 35.84507844392322085, 185.3768266524159856, -9.188101187500091527 ) ) ;
#29057=CARTESIAN_POINT ( 'NONE',  ( 147.6207062567320918, 275.4717883725331831, -2.882099113126173950 ) ) ;
#29060=CARTESIAN_POINT ( 'NONE',  ( 9.025180670817464446, 166.0177522451418213, 5.000000000000051514 ) ) ;
#29061=CARTESIAN_POINT ( 'NONE',  ( 180.0656950739936519, 267.0717194386327833, 15.04285446902010293 ) ) ;
#29063=CARTESIAN_POINT ( 'NONE',  ( 167.6146168596400514, 252.8497314824998909, -12.44459218179994231 ) ) ;
#29065=CARTESIAN_POINT ( 'NONE',  ( 185.9240074134731060, 297.6458951198301861, -5.725235308961436509 ) ) ;
#29068=CARTESIAN_POINT ( 'NONE',  ( 181.8543694586977324, 262.7755081626895048, 12.52910138123640671 ) ) ;
#29069=CARTESIAN_POINT ( 'NONE',  ( 97.28760307318144385, 233.6427522451419065, 10.00000000000009237 ) ) ;
#29071=ORIENTED_EDGE ( 'NONE', *, *, #11354, .T. ) ;
#29073=CARTESIAN_POINT ( 'NONE',  ( 202.2773826701151165, 280.2922913237452462, 16.62862787739668846 ) ) ;
#29074=CARTESIAN_POINT ( 'NONE',  ( 162.7738416911812180, 248.7144313781379310, -11.09964294874192525 ) ) ;
#29076=CARTESIAN_POINT ( 'NONE',  ( 11.65032017781297036, 177.5333772461660544, 9.188101187500095079 ) ) ;
#29078=CARTESIAN_POINT ( 'NONE',  ( 192.1269172743776892, 272.3004713032796644, 14.80205975413855946 ) ) ;
#29081=CARTESIAN_POINT ( 'NONE',  ( 194.8372111074683914, 274.9995225832199708, -16.05741363709758573 ) ) ;
#29082=CARTESIAN_POINT ( 'NONE',  ( 62.82726920452340380, 197.8923013555409796, 4.594050593750050204 ) ) ;
#29083=CARTESIAN_POINT ( 'NONE',  ( 208.2555382576270233, 269.9378221106229034, 3.215405476967123199 ) ) ;
#29086=CARTESIAN_POINT ( 'NONE',  ( 207.6727254509676186, 270.9472835030587703, 7.315149605389819953 ) ) ;
#29088=CARTESIAN_POINT ( 'NONE',  ( 13.95070015838929400, 188.8615022471903160, 5.000000000000046185 ) ) ;
#29089=CARTESIAN_POINT ( 'NONE',  ( 207.5583741822599393, 271.1453457103705205, 3.140867606700001424 ) ) ;
#29090=CARTESIAN_POINT ( 'NONE',  ( 144.9103262809084924, 242.2202760586659167, -5.415160957724236172E-17 ) ) ;
#29100=CARTESIAN_POINT ( 'NONE',  ( 163.3607625274802899, 247.6978546696471710, 7.891137406151327305 ) ) ;
#29104=CARTESIAN_POINT ( 'NONE',  ( 196.5746262556701822, 272.7668379574431015, -13.37129446457116622 ) ) ;
#29109=CARTESIAN_POINT ( 'NONE',  ( 196.1715942132062764, 270.9921725689870868, 12.26687914476305608 ) ) ;
#29110=CARTESIAN_POINT ( 'NONE',  ( -22.42236680055709641, 157.8615022471902591, 0.000000000000000000 ) ) ;
#29115=CARTESIAN_POINT ( 'NONE',  ( 191.8610655169697452, 287.8363447181971537, -15.91263000500258507 ) ) ;
#29117=FACE_OUTER_BOUND ( 'NONE', #19293, .T. ) ;
#29121=ORIENTED_EDGE ( 'NONE', *, *, #93118, .T. ) ;
#29123=CARTESIAN_POINT ( 'NONE',  ( 191.5893301551938350, 298.8045413135534432, -8.323356515452589477 ) ) ;
#29125=CARTESIAN_POINT ( 'NONE',  ( 204.3574891606595827, 276.6894411969685166, 13.41627538812899978 ) ) ;
#29128=CARTESIAN_POINT ( 'NONE',  ( 82.93520977470207356, 212.5643266524159856, -9.188101187500093303 ) ) ;
#29129=CARTESIAN_POINT ( 'NONE',  ( 198.7134558283731280, 282.8386145195935910, 17.66748989068429054 ) ) ;
#29130=CARTESIAN_POINT ( 'NONE',  ( 178.5276804562001871, 269.4738238426553494, -16.27363614876470166 ) ) ;
#29134=CARTESIAN_POINT ( 'NONE',  ( -13.49147982757802389, 173.0177522451419350, 5.000000000000046185 ) ) ;
#29135=VERTEX_POINT ( 'NONE', #86133 ) ;
#29137=ORIENTED_EDGE ( 'NONE', *, *, #7239, .T. ) ;
#29140=ORIENTED_EDGE ( 'NONE', *, *, #41862, .F. ) ;
#29141=CARTESIAN_POINT ( 'NONE',  ( 207.1388427945310582, 271.8719953892863828, -6.773753280169677815 ) ) ;
#29142=DIRECTION ( 'NONE',  ( 0.4999999999999992784, -0.8660254037844390407, 0.000000000000000000 ) ) ;
#29143=CARTESIAN_POINT ( 'NONE',  ( 194.4032909867620447, 293.9306181827685123, -16.05392006271526384 ) ) ;
#29145=CARTESIAN_POINT ( 'NONE',  ( 166.9053537448537270, 266.3976873878679044, -16.70102891481623431 ) ) ;
#29149=ORIENTED_EDGE ( 'NONE', *, *, #3560, .T. ) ;
#29150=CARTESIAN_POINT ( 'NONE',  ( 165.0419687026099496, 282.1322928540902240, 8.848871264540955295 ) ) ;
#29152=ORIENTED_EDGE ( 'NONE', *, *, #34996, .T. ) ;
#29153=CARTESIAN_POINT ( 'NONE',  ( 163.2919429874875448, 247.8170536094679903, 9.876785378511263147 ) ) ;
#29154=CARTESIAN_POINT ( 'NONE',  ( 188.9334919176225753, 259.5804479054066292, 2.551952175883118734 ) ) ;
#29155=CARTESIAN_POINT ( 'NONE',  ( 152.6320618002989136, 277.3629613401518554, -5.218654699652803153 ) ) ;
#29157=CARTESIAN_POINT ( 'NONE',  ( 192.6848806138171142, 292.2684757097440524, -14.43291781176028010 ) ) ;
#29158=CARTESIAN_POINT ( 'NONE',  ( 168.2548547082295443, 252.8785486555144075, 11.97806002154297467 ) ) ;
#29159=CARTESIAN_POINT ( 'NONE',  ( 194.8138150604092402, 263.1618850616820282, -0.7962985949493808224 ) ) ;
#29161=CARTESIAN_POINT ( 'NONE',  ( 181.8990295830258219, 270.3834252994221288, -16.69949221592476007 ) ) ;
#29164=CARTESIAN_POINT ( 'NONE',  ( 160.9611857202788201, 281.7540198505617468, 8.630106242394084859 ) ) ;
#29166=CARTESIAN_POINT ( 'NONE',  ( -9.955209428791576443, 178.3927522451419350, 2.944929066748280225E-16 ) ) ;
#29167=CARTESIAN_POINT ( 'NONE',  ( 196.1419589699951871, 269.5805659641910097, -10.92749632951035821 ) ) ;
#29168=CARTESIAN_POINT ( 'NONE',  ( 174.8241034426651765, 281.2870359428685560, -14.17652806122567988 ) ) ;
#29169=CARTESIAN_POINT ( 'NONE',  ( 203.8706191249530093, 277.5327248354951735, -15.89555175277244992 ) ) ;
#29171=CARTESIAN_POINT ( 'NONE',  ( 164.2916406588784923, 274.2388883841279608, 14.76576668727659047 ) ) ;
#29172=CARTESIAN_POINT ( 'NONE',  ( -12.05712525078605069, 163.8458772461660544, 9.188101187500095079 ) ) ;
#29173=CARTESIAN_POINT ( 'NONE',  ( 2.169146224190643846, 165.3927522451418213, 10.00000000000009948 ) ) ;
#29174=CARTESIAN_POINT ( 'NONE',  ( 188.9577279717659621, 296.9832364615082838, 8.133352747287846185 ) ) ;
#29180=CARTESIAN_POINT ( 'NONE',  ( 173.1133627894660947, 289.7078603327026940, 2.584739366812427885 ) ) ;
#29181=DIRECTION ( 'NONE',  ( -0.8660254037844387076, -0.4999999999999998890, -0.000000000000000000 ) ) ;
#29182=DIRECTION ( 'NONE',  ( 0.4999999999999998890, -0.8660254037844385966, 0.000000000000000000 ) ) ;
#29185=CARTESIAN_POINT ( 'NONE',  ( 150.8203273413079728, 276.8881287278626928, 3.694477562601145681 ) ) ;
#29186=CARTESIAN_POINT ( 'NONE',  ( 27.50958393249801404, 180.5643266524160424, 9.188101187500095079 ) ) ;
#29187=CARTESIAN_POINT ( 'NONE',  ( 109.7816501962546454, 240.3149278399160949, 9.188101187500093303 ) ) ;
#29189=CARTESIAN_POINT ( 'NONE',  ( 182.7638336887914079, 257.5540677396648448, -2.311609576158096147 ) ) ;
#29192=CARTESIAN_POINT ( 'NONE',  ( 175.3541623712593491, 281.5767007636894164, -14.18713308759929248 ) ) ;
#29194=CARTESIAN_POINT ( 'NONE',  ( 193.8913555215501390, 294.8173164187117550, 15.40725395879721837 ) ) ;
#29195=CARTESIAN_POINT ( 'NONE',  ( 161.8926315922002743, 250.2407320417157166, -13.77020595223768495 ) ) ;
#29199=CARTESIAN_POINT ( 'NONE',  ( 196.3831153806621046, 266.1916474279236695, 8.338913457951525388 ) ) ;
#29200=CARTESIAN_POINT ( 'NONE',  ( 78.01622611019826081, 227.3967562850346837, -4.648177544792955347E-16 ) ) ;
#29204=CARTESIAN_POINT ( 'NONE',  ( 182.0490020842017600, 268.2371330760522028, 15.01509780616252421 ) ) ;
#29205=CARTESIAN_POINT ( 'NONE',  ( 99.63334886536203783, 219.1423013555409796, -4.594050593750043987 ) ) ;
#29208=CARTESIAN_POINT ( 'NONE',  ( 157.8360072705708603, 257.2670114739976839, 17.12122855844125269 ) ) ;
#29209=CARTESIAN_POINT ( 'NONE',  ( 200.3852774630119029, 283.5695136757138357, 18.18377108216431992 ) ) ;
#29210=CARTESIAN_POINT ( 'NONE',  ( 149.3915652274231149, 271.8932141343000239, 13.09942943774031221 ) ) ;
#29211=B_SPLINE_CURVE_WITH_KNOTS ( 'NONE', 3,
 ( #61070, #92039, #84426, #14972 ),
 .UNSPECIFIED., .F., .F.,
 ( 4, 4 ),
 ( 0.02816671503466520315, 0.03735342737572562577 ),
 .UNSPECIFIED. ) ;
#29212=CARTESIAN_POINT ( 'NONE',  ( 150.6626254231123880, 269.6916732958875969, -15.32062296289003811 ) ) ;
#29216=FACE_OUTER_BOUND ( 'NONE', #70375, .T. ) ;
#29221=CARTESIAN_POINT ( 'NONE',  ( 192.4663556654298588, 297.2854885702906245, -12.98646995774174684 ) ) ;
#29222=CARTESIAN_POINT ( 'NONE',  ( 149.5796913320911870, 271.5673701627850960, -12.80793412251569841 ) ) ;
#29225=CARTESIAN_POINT ( 'NONE',  ( 159.7953104873542145, 253.8733987550956783, 15.41928249285404107 ) ) ;
#29226=CARTESIAN_POINT ( 'NONE',  ( 157.6371076352215823, 268.6636118182534005, 15.72487649508922480 ) ) ;
#29229=CARTESIAN_POINT ( 'NONE',  ( 139.5965524907815904, 264.7365022471903444, 2.944929066748280225E-16 ) ) ;
#29233=CARTESIAN_POINT ( 'NONE',  ( 196.0106993659726413, 265.2146929077559889, -4.435233568084376188 ) ) ;
#29235=EDGE_CURVE ( 'NONE', #690, #94448, #35414, .T. ) ;
#29236=VERTEX_POINT ( 'NONE', #85623 ) ;
#29237=CARTESIAN_POINT ( 'NONE',  ( 181.6032198279386307, 290.8331366659457444, -10.99987666991614610 ) ) ;
#29239=CARTESIAN_POINT ( 'NONE',  ( -22.42236680055709641, 157.8615022471902591, 0.000000000000000000 ) ) ;
#29240=CARTESIAN_POINT ( 'NONE',  ( 206.1959456970884617, 273.5051410683664130, 10.96659245355821533 ) ) ;
#29241=CARTESIAN_POINT ( 'NONE',  ( 192.1389822274309722, 279.7169248230215430, -16.65130882895569187 ) ) ;
#29243=CARTESIAN_POINT ( 'NONE',  ( 201.0468719883840265, 282.4235983437597497, -16.59631526626950659 ) ) ;
#29248=CARTESIAN_POINT ( 'NONE',  ( 169.6623362669060668, 268.6156801215794303, -17.83028812261259333 ) ) ;
#29251=CARTESIAN_POINT ( 'NONE',  ( 157.6921299354026189, 257.5162143285667753, -18.18720974599499840 ) ) ;
#29254=CARTESIAN_POINT ( 'NONE',  ( 165.9193144349327724, 274.0694398605538140, -15.17841830940742476 ) ) ;
#29255=CARTESIAN_POINT ( 'NONE',  ( 204.0884846259506276, 275.1553707185394728, 13.46337290381501717 ) ) ;
#29257=CARTESIAN_POINT ( 'NONE',  ( 156.6084421796713002, 261.3932165810376205, -17.82046942966612590 ) ) ;
#29259=CARTESIAN_POINT ( 'NONE',  ( 167.3883760682938089, 286.9270113580703878, -4.952300633368714955 ) ) ;
#29261=CARTESIAN_POINT ( 'NONE',  ( 178.1219001827957698, 255.2992632418402650, 5.629378456750874449 ) ) ;
#29262=CARTESIAN_POINT ( 'NONE',  ( 111.5137010038235417, 241.3149278399161233, -9.188101187500095079 ) ) ;
#29264=CARTESIAN_POINT ( 'NONE',  ( 184.8686473015538922, 260.4039463730296120, -9.780166574822738212 ) ) ;
#29266=CARTESIAN_POINT ( 'NONE',  ( 190.0706732994661365, 292.5512512978990003, -14.47399639281167083 ) ) ;
#29267=ORIENTED_EDGE ( 'NONE', *, *, #2597, .F. ) ;
#29273=CARTESIAN_POINT ( 'NONE',  ( 196.4351339088274813, 290.4113630087520050, 17.20526457544535504 ) ) ;
#29274=CARTESIAN_POINT ( 'NONE',  ( 159.2394649670193303, 254.8361514374751664, -16.43133403737800791 ) ) ;
#29276=ORIENTED_EDGE ( 'NONE', *, *, #76496, .T. ) ;
#29277=CARTESIAN_POINT ( 'NONE',  ( 147.9431929457713011, 274.4018685143957441, 9.901114480726821654 ) ) ;
#29281=ORIENTED_EDGE ( 'NONE', *, *, #32022, .F. ) ;
#29282=B_SPLINE_CURVE_WITH_KNOTS ( 'NONE', 3,
 ( #45724, #15830, #29065, #76647 ),
 .UNSPECIFIED., .F., .F.,
 ( 4, 4 ),
 ( 0.03863331949670163745, 0.04715616731377302029 ),
 .UNSPECIFIED. ) ;
#29283=CARTESIAN_POINT ( 'NONE',  ( 164.9356397357043704, 244.9700873293209042, 2.799217332519396972 ) ) ;
#29284=EDGE_CURVE ( 'NONE', #75541, #18309, #22151, .T. ) ;
#29285=CARTESIAN_POINT ( 'NONE',  ( 167.4962802984076689, 246.9545338215429808, -0.8696054547567072524 ) ) ;
#29289=CARTESIAN_POINT ( 'NONE',  ( 158.1893771932294896, 280.3773502170195684, 5.704923391183662318 ) ) ;
#29292=CARTESIAN_POINT ( 'NONE',  ( 68.78093353194373094, 200.5177522451417929, 5.000000000000051514 ) ) ;
#29293=EDGE_CURVE ( 'NONE', #37700, #38232, #43365, .T. ) ;
#29295=B_SPLINE_CURVE_WITH_KNOTS ( 'NONE', 3,
 ( #49844, #56438, #17965, #47820 ),
 .UNSPECIFIED., .F., .F.,
 ( 4, 4 ),
 ( 0.03424363036717037456, 0.04307889571479175950 ),
 .UNSPECIFIED. ) ;
#29296=CARTESIAN_POINT ( 'NONE',  ( 189.6922020185305655, 263.1654225416511963, -9.791328709709494760 ) ) ;
#29297=EDGE_CURVE ( 'NONE', #14857, #53916, #71695, .T. ) ;
#29298=CARTESIAN_POINT ( 'NONE',  ( 192.6263115592815893, 271.4202054200192720, 14.08161611139827052 ) ) ;
#29299=CARTESIAN_POINT ( 'NONE',  ( 189.0338852884921721, 270.0244833716615176, -14.06004501950776842 ) ) ;
#29300=CARTESIAN_POINT ( 'NONE',  ( 152.3107445603601491, 271.8204453097907276, -13.76269077489604875 ) ) ;
#29303=CARTESIAN_POINT ( 'NONE',  ( 23.45662567177863167, 195.8967562850347122, -4.648177544792955347E-16 ) ) ;
#29305=CARTESIAN_POINT ( 'NONE',  ( 78.60473566001486745, 222.3149278399160664, 9.188101187500093303 ) ) ;
#29306=CARTESIAN_POINT ( 'NONE',  ( 159.9647205790309101, 253.5799718689968927, -16.48298384325780219 ) ) ;
#29308=CARTESIAN_POINT ( 'NONE',  ( 187.1789365411204926, 291.3781964708418286, -14.15416893886036220 ) ) ;
#29309=CARTESIAN_POINT ( 'NONE',  ( 161.1150691641480535, 251.5875096731584506, -13.48836942566120101 ) ) ;
#29310=CARTESIAN_POINT ( 'NONE',  ( 151.2671975087473015, 270.6445237267302559, 14.15418255155509542 ) ) ;
#29315=CARTESIAN_POINT ( 'NONE',  ( 195.9359860111818250, 291.2759125279654882, 17.49638312768267312 ) ) ;
#29317=CARTESIAN_POINT ( 'NONE',  ( 21.77181853666109745, 189.5024278399160949, 9.188101187500095079 ) ) ;
#29318=CARTESIAN_POINT ( 'NONE',  ( 169.9904317359561219, 275.5861877515991978, -16.87365932016444603 ) ) ;
#29322=CARTESIAN_POINT ( 'NONE',  ( 52.54321753458319932, 191.9548013555410080, -4.594050593750042211 ) ) ;
#29325=CARTESIAN_POINT ( 'NONE',  ( 165.5093369583051128, 275.0219039653110258, -16.16693748275729803 ) ) ;
#29326=CARTESIAN_POINT ( 'NONE',  ( -9.359816960141781550, 158.7365022471902023, 10.00000000000009948 ) ) ;
#29329=CARTESIAN_POINT ( 'NONE',  ( 159.5137144416034403, 255.6472557863606028, -16.29473761095158579 ) ) ;
#29331=CARTESIAN_POINT ( 'NONE',  ( 179.8145615969634434, 276.7378561409443591, 16.32957337418346100 ) ) ;
#29334=CARTESIAN_POINT ( 'NONE',  ( 192.3032628966054460, 266.2805749702787921, 11.62727084212969864 ) ) ;
#29335=EDGE_CURVE ( 'NONE', #78112, #13195, #25351, .T. ) ;
#29336=VECTOR ( 'NONE', #79757, 1000.000000000000000 ) ;
#29337=CARTESIAN_POINT ( 'NONE',  ( 21.99520779934447745, 195.0530062829863311, -4.648177544792955347E-16 ) ) ;
#29339=CARTESIAN_POINT ( 'NONE',  ( 101.4192659406176915, 219.3615022471902023, 5.000000000000051514 ) ) ;
#29340=CARTESIAN_POINT ( 'NONE',  ( 161.3193951073452581, 251.2336067582368742, 13.01220207292984377 ) ) ;
#29343=CARTESIAN_POINT ( 'NONE',  ( 57.82012596918833935, 210.3149278399160664, 9.188101187500093303 ) ) ;
#29345=CARTESIAN_POINT ( 'NONE',  ( 166.5857064600952526, 264.6722026030038251, 17.46362175718670429 ) ) ;
#29346=CARTESIAN_POINT ( 'NONE',  ( 190.2287563641723978, 301.1611242470490311, -4.521471513871881953 ) ) ;
#29347=EDGE_CURVE ( 'NONE', #8797, #59906, #40249, .T. ) ;
#29351=CARTESIAN_POINT ( 'NONE',  ( 165.0532575723395041, 244.7663672603923715, -2.144843157699870773 ) ) ;
#29355=CARTESIAN_POINT ( 'NONE',  ( 204.6487448717501252, 276.1849715073653897, 14.68262965895386607 ) ) ;
#29359=CARTESIAN_POINT ( 'NONE',  ( 172.6847352287274759, 251.7905635882845559, -7.423737323049481418 ) ) ;
#29360=EDGE_CURVE ( 'NONE', #31691, #89234, #86261, .T. ) ;
#29362=CARTESIAN_POINT ( 'NONE',  ( 182.3977840624999658, 284.1126370688600105, 14.97779424287036854 ) ) ;
#29363=ADVANCED_FACE ( 'NONE', ( #69740 ), #3735, .T. ) ;
#29364=CARTESIAN_POINT ( 'NONE',  ( 206.7923762329701276, 272.4720930770340033, -9.496103119940368487 ) ) ;
#29368=DIRECTION ( 'NONE',  ( -0.5000000000000006661, 0.8660254037844382635, -1.877843081442121204E-16 ) ) ;
#29369=CARTESIAN_POINT ( 'NONE',  ( 207.8446715390582540, 270.6494641423232679, -2.429516028743652800 ) ) ;
#29370=CARTESIAN_POINT ( 'NONE',  ( 164.3853877993040840, 245.9231516401292197, 5.995325337583643943 ) ) ;
#29371=CARTESIAN_POINT ( 'NONE',  ( 159.9014600375868440, 253.6895423408921886, 15.57825579621527368 ) ) ;
#29373=CARTESIAN_POINT ( 'NONE',  ( 204.3760460221041342, 271.7077994814860062, 9.919166744778580735 ) ) ;
#29374=CARTESIAN_POINT ( 'NONE',  ( 133.4083396129551602, 238.6423013555409796, -4.594050593750043987 ) ) ;
#29375=CARTESIAN_POINT ( 'NONE',  ( 82.23173768200972233, 206.0327760586659451, 1.948934522072303157E-15 ) ) ;
#29377=CARTESIAN_POINT ( 'NONE',  ( 171.1449649924396397, 264.1412602032671657, 15.82665639531467150 ) ) ;
#29380=ORIENTED_EDGE ( 'NONE', *, *, #33879, .T. ) ;
#29381=CARTESIAN_POINT ( 'NONE',  ( 160.7612047594922160, 254.0226279303306569, 15.66240655037786489 ) ) ;
#29382=VERTEX_POINT ( 'NONE', #42205 ) ;
#29387=CARTESIAN_POINT ( 'NONE',  ( 194.1866705654072689, 284.7458260699956440, 17.61685658156456213 ) ) ;
#29388=CARTESIAN_POINT ( 'NONE',  ( 191.7934382699952494, 298.4510156884799699, -8.680100145728863126 ) ) ;
#29390=CARTESIAN_POINT ( 'NONE',  ( 154.9683083969241011, 262.2340116239618055, 18.33261662430134109 ) ) ;
#29393=EDGE_CURVE ( 'NONE', #59906, #47888, #65562, .T. ) ;
#29394=CARTESIAN_POINT ( 'NONE',  ( 200.4628475472039213, 283.4351583487458583, -16.90921332594512450 ) ) ;
#29396=CARTESIAN_POINT ( 'NONE',  ( 163.7388909753429118, 261.0030389665530492, -17.17036421060282336 ) ) ;
#29397=CARTESIAN_POINT ( 'NONE',  ( 164.6597889008906463, 246.7339933633426483, 5.500642480278799873 ) ) ;
#29398=EDGE_CURVE ( 'NONE', #30511, #55652, #27010, .T. ) ;
#29399=CARTESIAN_POINT ( 'NONE',  ( 147.4427322147670907, 275.2686919276877120, -3.117028667211196868 ) ) ;
#29400=CARTESIAN_POINT ( 'NONE',  ( 164.9103019330012216, 245.0139736909548560, 2.841678961959298810 ) ) ;
#29401=CARTESIAN_POINT ( 'NONE',  ( 196.2878005184348353, 290.6665519265632724, -16.69183432842427806 ) ) ;
#29402=CARTESIAN_POINT ( 'NONE',  ( 201.6593076491624856, 268.7283862757352608, -7.798329487074514788 ) ) ;
#29403=CARTESIAN_POINT ( 'NONE',  ( 137.1425535231280151, 259.1744531367911009, 4.594050593750047540 ) ) ;
#29404=ORIENTED_EDGE ( 'NONE', *, *, #63416, .T. ) ;
#29407=CARTESIAN_POINT ( 'NONE',  ( 182.0290520670355647, 257.6954483311129707, 6.591660305417710752 ) ) ;
#29408=CARTESIAN_POINT ( 'NONE',  ( 155.9450630872215982, 261.9324000175035394, -16.96800591457008878 ) ) ;
#29412=CARTESIAN_POINT ( 'NONE',  ( 185.2961235551778714, 291.2460235572835927, 13.48139818756336616 ) ) ;
#29413=CARTESIAN_POINT ( 'NONE',  ( 182.1763566781647512, 275.7876014702704310, -16.43406825299696550 ) ) ;
#29417=CARTESIAN_POINT ( 'NONE',  ( 199.4759783357731351, 266.7372442807093762, 0.8265985939221809353 ) ) ;
#29418=CARTESIAN_POINT ( 'NONE',  ( 195.3555557534167519, 264.0388318245352934, 0.8383882831563513882 ) ) ;
#29419=CARTESIAN_POINT ( 'NONE',  ( 147.2443490232117256, 275.6123016948292275, 5.226063659459642352 ) ) ;
#29420=CARTESIAN_POINT ( 'NONE',  ( 183.8623045117518586, 281.0860684350564611, 16.35513551783298780 ) ) ;
#29421=CARTESIAN_POINT ( 'NONE',  ( 193.7028804065858480, 269.2481018004579596, 12.11718006226955602 ) ) ;
#29424=CARTESIAN_POINT ( 'NONE',  ( 205.2203921948319589, 274.5650203181114648, 11.44562195678287253 ) ) ;
#29426=CARTESIAN_POINT ( 'NONE',  ( 198.2040940955416488, 287.3474340887963763, 16.95806375232200480 ) ) ;
#29428=CARTESIAN_POINT ( 'NONE',  ( -3.180017766230537557, 156.7202760586659736, -5.415160957724236172E-17 ) ) ;
#29429=CARTESIAN_POINT ( 'NONE',  ( 172.1831654133907819, 283.7635488940352388, -12.63565973616138294 ) ) ;
#29430=ORIENTED_EDGE ( 'NONE', *, *, #46761, .F. ) ;
#29433=CARTESIAN_POINT ( 'NONE',  ( 202.4716377814179680, 274.0562387935223114, -13.02713981561660184 ) ) ;
#29434=CARTESIAN_POINT ( 'NONE',  ( 198.9832789858017463, 285.9978462703757600, -18.55676541969546278 ) ) ;
#29435=CARTESIAN_POINT ( 'NONE',  ( 2.232293911657190488, 172.0958772461660544, -9.188101187500095079 ) ) ;
#29441=DIRECTION ( 'NONE',  ( 0.4999999999999992784, -0.8660254037844390407, 0.000000000000000000 ) ) ;
#29442=CARTESIAN_POINT ( 'NONE',  ( 175.8941432106488492, 252.8195566316572922, -3.266688834427511789 ) ) ;
#29443=CARTESIAN_POINT ( 'NONE',  ( 150.6051381537932343, 269.7912441671369947, 13.72054362922755999 ) ) ;
#29444=CARTESIAN_POINT ( 'NONE',  ( 182.7446153974817946, 296.3825044924181498, 1.852756993870850133 ) ) ;
#29445=CARTESIAN_POINT ( 'NONE',  ( 57.17980156396254898, 210.4865022471903160, 10.00000000000009237 ) ) ;
#29447=CARTESIAN_POINT ( 'NONE',  ( 190.1730848958311810, 301.2575500587478814, 0.2415986433272204748 ) ) ;
#29449=CARTESIAN_POINT ( 'NONE',  ( 9.512059640396367755, 185.4869531367911293, 4.594050593750046652 ) ) ;
#29450=CARTESIAN_POINT ( 'NONE',  ( 164.5169933802496587, 285.4399748993757271, 4.369849052753852270 ) ) ;
#29451=CARTESIAN_POINT ( 'NONE',  ( 152.8134625983922490, 265.9663140294953791, 17.57333028169644251 ) ) ;
#29456=CARTESIAN_POINT ( 'NONE',  ( 206.9377610035629118, 272.2202792677204002, 7.440532334334675646 ) ) ;
#29457=CARTESIAN_POINT ( 'NONE',  ( 188.7267008190097499, 267.6263124316118933, 14.18876842644463920 ) ) ;
#29458=CARTESIAN_POINT ( 'NONE',  ( 116.9355544250887959, 244.9865022471903160, 10.00000000000009415 ) ) ;
#29461=CARTESIAN_POINT ( 'NONE',  ( 148.3997536239841679, 273.6110822229926498, 8.713694244701960301 ) ) ;
#29463=CARTESIAN_POINT ( 'NONE',  ( 198.5765922241581336, 267.0449333599083275, 7.976362536003974490 ) ) ;
#29471=( BOUNDED_CURVE ( )  B_SPLINE_CURVE ( 2, ( #21930, #20968, #6232, #52328, #36128, #75159, #74671, #36622, #12360 ),
 .UNSPECIFIED., .F., .T. ) 
 B_SPLINE_CURVE_WITH_KNOTS ( ( 3, 2, 2, 2, 3 ),
 ( 0.7056451612903226200, 0.7069892473118279952, 0.7096774193548387455, 0.7123655913978494958, 0.7137096774193548709 ),
 .UNSPECIFIED. ) 
 CURVE ( )  GEOMETRIC_REPRESENTATION_ITEM ( )  RATIONAL_B_SPLINE_CURVE ( ( 0.9330127018922194093, 0.9330127018922194093, 1.000000000000000000, 0.8660254037844387076, 1.000000000000000000, 0.8660254037844387076, 1.000000000000000000, 0.9330127018922194093, 0.9330127018922194093 ) ) 
 REPRESENTATION_ITEM ( '' )  );
#29472=CARTESIAN_POINT ( 'NONE',  ( 195.8779528940816874, 290.3143152550151740, -16.43829057065248023 ) ) ;
#29476=CARTESIAN_POINT ( 'NONE',  ( 155.4495868485232108, 261.4004128932040203, -18.48326470492642315 ) ) ;
#29477=VERTEX_POINT ( 'NONE', #59893 ) ;
#29479=CARTESIAN_POINT ( 'NONE',  ( 186.3138579965807935, 271.9636586987053306, -16.45016817854244096 ) ) ;
#29480=CARTESIAN_POINT ( 'NONE',  ( 204.9432097630379417, 275.6749433546094679, 13.74700047688257776 ) ) ;
#29482=CARTESIAN_POINT ( 'NONE',  ( 191.4044787581200069, 299.1247133251352466, 7.435199718141230818 ) ) ;
#29486=ORIENTED_EDGE ( 'NONE', *, *, #43944, .T. ) ;
#29489=CARTESIAN_POINT ( 'NONE',  ( 206.0627831668701901, 273.7357853363691902, 10.14454147593459687 ) ) ;
#29492=CARTESIAN_POINT ( 'NONE',  ( 149.7166446726674565, 271.3301600186404698, 12.26048591517335495 ) ) ;
#29493=CARTESIAN_POINT ( 'NONE',  ( 172.3444904895413856, 263.8722161183861203, -15.54433039079544088 ) ) ;
#29501=VERTEX_POINT ( 'NONE', #58884 ) ;
#29505=CARTESIAN_POINT ( 'NONE',  ( 189.9052851100924215, 301.7213928939034986, -1.077181946533001256 ) ) ;
#29506=CARTESIAN_POINT ( 'NONE',  ( 175.0305792595766263, 260.7322313912393952, -14.80875141956958707 ) ) ;
#29507=CARTESIAN_POINT ( 'NONE',  ( 192.4454213697443095, 297.3217478340386606, 12.58566886711101596 ) ) ;
#29508=CARTESIAN_POINT ( 'NONE',  ( 191.0739205222354258, 299.6972569845476073, 8.800115285385583519 ) ) ;
#29509=CARTESIAN_POINT ( 'NONE',  ( 146.5689048584090699, 276.7822053059436485, -0.4306668706573002492 ) ) ;
#29510=ADVANCED_FACE ( 'NONE', ( #30500 ), #86141, .F. ) ;
#29511=B_SPLINE_CURVE_WITH_KNOTS ( 'NONE', 3,
 ( #8962, #94105, #860, #55049, #16061, #56038, #48470, #87031, #94601, #18077, #33263, #40838, #79907, #1874, #86524, #47453, #16559, #24164, #78381, #24656 ),
 .UNSPECIFIED., .F., .F.,
 ( 4, 2, 2, 2, 2, 2, 2, 2, 2, 4 ),
 ( 0.003588130654998039452, 0.003719546847186400683, 0.003850963039374761913, 0.003982379231563123144, 0.004113795423751483507, 0.004376627808128081068, 0.004639460192504678629, 0.005690789730011110506, 0.006742119267517541516, 0.007793448805023973393 ),
 .UNSPECIFIED. ) ;
#29513=B_SPLINE_CURVE_WITH_KNOTS ( 'NONE', 3,
 ( #28303, #90157, #20731, #74933, #51616, #44495 ),
 .UNSPECIFIED., .F., .F.,
 ( 4, 2, 4 ),
 ( 0.01829576855254007664, 0.02279459486296724416, 0.02729342117339441168 ),
 .UNSPECIFIED. ) ;
#29516=CARTESIAN_POINT ( 'NONE',  ( 196.9319848161575806, 289.5507919934690335, -17.64330560362266453 ) ) ;
#29519=CARTESIAN_POINT ( 'NONE',  ( 168.3229878282932361, 286.3524262165808523, 4.038607488141395585 ) ) ;
#29522=CARTESIAN_POINT ( 'NONE',  ( 190.5470883969117892, 300.6097569926677693, -3.254269538324694455 ) ) ;
#29527=CARTESIAN_POINT ( 'NONE',  ( 191.4500230558827809, 297.4070410935535165, -10.84401322141531487 ) ) ;
#29528=CARTESIAN_POINT ( 'NONE',  ( 189.8160923722963389, 301.8758792474325787, -0.7767885082579778500 ) ) ;
#29530=ORIENTED_EDGE ( 'NONE', *, *, #17227, .F. ) ;
#29531=CARTESIAN_POINT ( 'NONE',  ( 208.2874212803407090, 269.8825990953837390, -1.143705256421198690 ) ) ;
#29534=CARTESIAN_POINT ( 'NONE',  ( 51.02741275436275004, 190.2677522451418213, -5.000000000000041744 ) ) ;
#29535=CARTESIAN_POINT ( 'NONE',  ( 107.1835739849013578, 238.8149278399160949, 9.188101187500093303 ) ) ;
#29536=CARTESIAN_POINT ( 'NONE',  ( 198.7829547491859330, 286.3448180261817129, -18.59838968157616179 ) ) ;
#29538=CARTESIAN_POINT ( 'NONE',  ( 167.4968739850875750, 271.4686504602936452, 17.49260192182149254 ) ) ;
#29539=CARTESIAN_POINT ( 'NONE',  ( 195.7291850945597957, 291.6341022226063160, 17.08310330964873813 ) ) ;
#29541=CARTESIAN_POINT ( 'NONE',  ( 34.97905304013878691, 184.8768266524159856, 9.188101187500098632 ) ) ;
#29542=CARTESIAN_POINT ( 'NONE',  ( 147.7362813631496863, 275.4859596630231522, -3.675214258173687298 ) ) ;
#29543=ORIENTED_EDGE ( 'NONE', *, *, #44983, .F. ) ;
#29544=CARTESIAN_POINT ( 'NONE',  ( 191.3220911622827600, 298.6397096588477780, 8.200542337010491067 ) ) ;
#29545=CARTESIAN_POINT ( 'NONE',  ( 181.6523902737856417, 267.3132069320698747, 14.96885079024440834 ) ) ;
#29547=CARTESIAN_POINT ( 'NONE',  ( 190.9441801652054096, 299.9219738747156043, -4.765040093794296716 ) ) ;
#29549=DIRECTION ( 'NONE',  ( 0.4999999999999992784, -0.8660254037844390407, 0.000000000000000000 ) ) ;
#29550=CARTESIAN_POINT ( 'NONE',  ( 179.0422977575919390, 287.4129436693755792, -12.34808154371113709 ) ) ;
#29551=CARTESIAN_POINT ( 'NONE',  ( 164.1116730098435426, 250.1177055282117863, 10.48172797642971155 ) ) ;
#29553=CARTESIAN_POINT ( 'NONE',  ( 117.2061873602236233, 225.1427522451417929, 1.119607411625061291E-15 ) ) ;
#29555=EDGE_CURVE ( 'NONE', #24507, #6222, #54794, .T. ) ;
#29556=CARTESIAN_POINT ( 'NONE',  ( 194.7741005058701660, 266.3470718410572999, -7.689080487137245790 ) ) ;
#29557=CARTESIAN_POINT ( 'NONE',  ( 158.0650824465715516, 281.3856441582040588, -1.598288696427632827 ) ) ;
#29558=CARTESIAN_POINT ( 'NONE',  ( 208.2912792141756029, 269.8759169579697641, -2.198672330625011995 ) ) ;
#29559=CARTESIAN_POINT ( 'NONE',  ( 20.20266813594930611, 170.2202760586659736, -5.415160957724236172E-17 ) ) ;
#29561=CARTESIAN_POINT ( 'NONE',  ( 192.1761047855001152, 272.2161798191603452, 14.46851533410970880 ) ) ;
#29564=CARTESIAN_POINT ( 'NONE',  ( 174.0659358162305068, 287.4380069074235280, 10.67600509024926581 ) ) ;
#29565=CARTESIAN_POINT ( 'NONE',  ( 54.68078388046974680, 208.5024278399160664, -9.188101187500093303 ) ) ;
#29566=CARTESIAN_POINT ( 'NONE',  ( 163.8947349411736525, 246.7729873192901664, -5.868803394723933309 ) ) ;
#29571=CARTESIAN_POINT ( 'NONE',  ( 17.34263298987836066, 187.4865022471903444, -10.00000000000009415 ) ) ;
#29572=CARTESIAN_POINT ( 'NONE',  ( 208.3117541397001844, 269.8404533466799080, 2.895672523916592578 ) ) ;
#29573=CARTESIAN_POINT ( 'NONE',  ( 128.9153121871758572, 254.4244531367911293, -4.594050593750046652 ) ) ;
#29575=CARTESIAN_POINT ( 'NONE',  ( 188.0428171265000117, 264.4088423580298581, 12.23537495986646029 ) ) ;
#29577=B_SPLINE_CURVE_WITH_KNOTS ( 'NONE', 3,
 ( #66607, #65129, #73245, #65622 ),
 .UNSPECIFIED., .F., .F.,
 ( 4, 4 ),
 ( 0.004660457163933351930, 0.01266542117972364531 ),
 .UNSPECIFIED. ) ;
#29580=CARTESIAN_POINT ( 'NONE',  ( 187.2510800322089324, 288.7440624129242224, 14.48677483733536420 ) ) ;
#29582=VERTEX_POINT ( 'NONE', #86760 ) ;
#29584=CARTESIAN_POINT ( 'NONE',  ( 180.6665526851674599, 287.6815954905284798, 14.11204521094005671 ) ) ;
#29585=CIRCLE ( 'NONE', #86263, 17.82106496071138224 ) ;
#29586=CARTESIAN_POINT ( 'NONE',  ( 196.3883463204838051, 288.9924089565074610, 17.07220126560286388 ) ) ;
#29587=CARTESIAN_POINT ( 'NONE',  ( 193.8905572877353052, 270.7343714464398658, -13.92882677973582872 ) ) ;
#29594=EDGE_CURVE ( 'NONE', #57617, #76220, #56065, .T. ) ;
#29597=CARTESIAN_POINT ( 'NONE',  ( 93.89567024169240028, 225.0177522451418781, -10.00000000000009592 ) ) ;
#29598=EDGE_CURVE ( 'NONE', #100032, #61618, #72884, .T. ) ;
#29600=CARTESIAN_POINT ( 'NONE',  ( 152.6740002182599767, 266.2078699576288159, -17.16212636348624088 ) ) ;
#29603=CARTESIAN_POINT ( 'NONE',  ( 175.1378461883211912, 279.3152656845848583, 16.63146252814350134 ) ) ;
#29605=CARTESIAN_POINT ( 'NONE',  ( 149.0359194785865498, 272.5092106407810206, 12.76357969772040590 ) ) ;
#29606=CARTESIAN_POINT ( 'NONE',  ( -22.42236680055709641, 157.8615022471902591, 0.000000000000000000 ) ) ;
#29609=CARTESIAN_POINT ( 'NONE',  ( 147.2784190576484491, 275.5532906641692534, 0.2793038414862047958 ) ) ;
#29612=CARTESIAN_POINT ( 'NONE',  ( 163.8147431267737204, 246.9115372060205118, 7.125417796469586840 ) ) ;
#29615=CARTESIAN_POINT ( 'NONE',  ( 97.11602866590727956, 233.0024278399160664, 9.188101187500095079 ) ) ;
#29616=CARTESIAN_POINT ( 'NONE',  ( 202.9830217136424437, 279.0700886485516889, 15.21791590704638075 ) ) ;
#29617=CARTESIAN_POINT ( 'NONE',  ( 178.3900700529107439, 269.3831628842910959, -16.31511681271764047 ) ) ;
#29627=CARTESIAN_POINT ( 'NONE',  ( 208.2175703429120688, 270.0035844679667889, 2.257951022351344150 ) ) ;
#29638=CARTESIAN_POINT ( 'NONE',  ( 167.4154476021087135, 283.9804021233929348, 9.114543589697493786 ) ) ;
#29640=CARTESIAN_POINT ( 'NONE',  ( 124.3429387061717364, 231.0494855054051300, -2.679491924311248496 ) ) ;
#29641=EDGE_LOOP ( 'NONE', ( #91910, #14586, #11933, #91062 ) ) ;
#29642=CARTESIAN_POINT ( 'NONE',  ( 202.9216520459657147, 279.1763840310111391, 15.75371595331685803 ) ) ;
#29643=CARTESIAN_POINT ( 'NONE',  ( 188.2136819673668242, 260.7815903057019682, 2.765234107804726005 ) ) ;
#29644=CARTESIAN_POINT ( 'NONE',  ( 160.9550112742611248, 282.2102974542603420, -6.127038402763485436 ) ) ;
#29645=LINE ( 'NONE', #31119, #32782 ) ;
#29646=CARTESIAN_POINT ( 'NONE',  ( 158.0940639500165901, 257.7445122115800586, 16.87026726729103387 ) ) ;
#29647=CARTESIAN_POINT ( 'NONE',  ( 174.5970010251735687, 290.1372909713314243, 7.765872408461218512 ) ) ;
#29648=CARTESIAN_POINT ( 'NONE',  ( 194.6410797438239229, 263.4546428906130018, -0.7807572112392382468 ) ) ;
#29650=CARTESIAN_POINT ( 'NONE',  ( 94.05805000844988228, 235.1115022471902876, -5.000000000000047962 ) ) ;
#29651=CARTESIAN_POINT ( 'NONE',  ( 194.1568482115562517, 293.9028091603209987, -14.13911859744283461 ) ) ;
#29652=CARTESIAN_POINT ( 'NONE',  ( 2.169146224190643846, 165.3927522451418213, 10.00000000000009592 ) ) ;
#29655=CARTESIAN_POINT ( 'NONE',  ( 164.0834751870549439, 246.4460796239905562, -8.551802143958536107 ) ) ;
#29658=CARTESIAN_POINT ( 'NONE',  ( 161.5845086034577776, 251.1610536727440603, -12.80556992964895713 ) ) ;
#29659=CARTESIAN_POINT ( 'NONE',  ( -3.478321416370212305, 177.9869531367911293, 4.594050593750046652 ) ) ;
#29661=CARTESIAN_POINT ( 'NONE',  ( 185.0981174815935617, 295.5755628286759134, 8.523774916173438854 ) ) ;
#29663=ORIENTED_EDGE ( 'NONE', *, *, #65791, .T. ) ;
#29666=CARTESIAN_POINT ( 'NONE',  ( 175.5383291916544408, 291.1589915617879001, 3.239589670356908258 ) ) ;
#29668=CARTESIAN_POINT ( 'NONE',  ( 201.9466639498089648, 280.8651129503298876, -16.50130735264049164 ) ) ;
#29670=CARTESIAN_POINT ( 'NONE',  ( 150.0383903883423500, 276.7166470372682738, 3.302347238614709912 ) ) ;
#29671=B_SPLINE_CURVE_WITH_KNOTS ( 'NONE', 3,
 ( #27067, #95522, #26567, #96497, #64565, #43234, #57948, #19966, #97004, #19493 ),
 .UNSPECIFIED., .F., .F.,
 ( 4, 2, 2, 2, 4 ),
 ( 2.941174414789049541E-15, 0.0004007808608854804104, 0.0008015617217680197056, 0.001202342582650559001, 0.001603123443533098188 ),
 .UNSPECIFIED. ) ;
#29672=CARTESIAN_POINT ( 'NONE',  ( 20.74358691754956396, 182.7833772461660544, -9.188101187500095079 ) ) ;
#29674=CARTESIAN_POINT ( 'NONE',  ( 128.9971094863694532, 233.0327760586659451, 1.948934522072303157E-15 ) ) ;
#29675=CARTESIAN_POINT ( 'NONE',  ( 178.7059724048094154, 292.0117454520415095, -7.090766484047969165 ) ) ;
#29676=CARTESIAN_POINT ( 'NONE',  ( 183.0630607540572043, 257.7369719463336537, -2.333968474862014642 ) ) ;
#29677=CARTESIAN_POINT ( 'NONE',  ( 206.3344875830494516, 271.9951829204101159, -7.959596699499296157 ) ) ;
#29680=CARTESIAN_POINT ( 'NONE',  ( 178.1741645575075381, 283.4573702867252791, -14.54551446833769290 ) ) ;
#29682=CARTESIAN_POINT ( 'NONE',  ( 155.3738696901333469, 261.5315588585399951, 17.02116401938635804 ) ) ;
#29683=CARTESIAN_POINT ( 'NONE',  ( 161.2977680094314223, 251.2710659906439616, -13.03191437619249982 ) ) ;
#29684=CARTESIAN_POINT ( 'NONE',  ( 189.6666044902458168, 284.7049877867155487, 17.41007887138588117 ) ) ;
#29686=CARTESIAN_POINT ( 'NONE',  ( 170.7208444631169755, 279.4758202746681377, 13.90914101253246393 ) ) ;
#29687=CARTESIAN_POINT ( 'NONE',  ( 192.6195712009543399, 265.2424128860524206, 7.804296869474439013 ) ) ;
#29688=CARTESIAN_POINT ( 'NONE',  ( 174.4665098196985298, 288.5002641398569949, -10.08633113632384237 ) ) ;
#29689=CARTESIAN_POINT ( 'NONE',  ( 61.41971759977597145, 206.2677522451418781, 10.00000000000009592 ) ) ;
#29691=CARTESIAN_POINT ( 'NONE',  ( 185.0331805397589733, 269.4951233173647438, 15.91801816997161545 ) ) ;
#29692=CARTESIAN_POINT ( 'NONE',  ( 86.72372382049398709, 227.0024278399160949, 9.188101187500095079 ) ) ;
#29694=CARTESIAN_POINT ( 'NONE',  ( 150.8757650385446993, 269.3225046528533539, 14.31332712971473953 ) ) ;
#29698=FACE_OUTER_BOUND ( 'NONE', #48413, .T. ) ;
#29700=CARTESIAN_POINT ( 'NONE',  ( 173.5309596338303493, 267.4569899417176657, -16.80614428785976955 ) ) ;
#29702=CARTESIAN_POINT ( 'NONE',  ( 147.1125781744767949, 275.8405354997948962, -5.216646253929903665 ) ) ;
#29703=CARTESIAN_POINT ( 'NONE',  ( -22.42236680055709641, 157.8615022471902591, 0.000000000000000000 ) ) ;
#29704=ORIENTED_EDGE ( 'NONE', *, *, #50811, .F. ) ;
#29707=CARTESIAN_POINT ( 'NONE',  ( 193.1649355862271591, 296.0755126543221536, -12.21556774862162698 ) ) ;
#29709=ORIENTED_EDGE ( 'NONE', *, *, #8899, .F. ) ;
#29712=CARTESIAN_POINT ( 'NONE',  ( 159.5764336135613632, 254.2525046211064819, 15.32981087583629076 ) ) ;
#29713=CARTESIAN_POINT ( 'NONE',  ( 180.7071999899477532, 263.3223274914530521, -12.85640988611793745 ) ) ;
#29715=CARTESIAN_POINT ( 'NONE',  ( 169.3416567082309712, 252.0478821765268549, -8.660523848214891629 ) ) ;
#29717=CARTESIAN_POINT ( 'NONE',  ( 140.8234218128096700, 242.1115022471902023, -5.000000000000041744 ) ) ;
#29718=VERTEX_POINT ( 'NONE', #95851 ) ;
#29720=EDGE_CURVE ( 'NONE', #31958, #29236, #74017, .T. ) ;
#29723=EDGE_CURVE ( 'NONE', #39441, #59283, #51704, .T. ) ;
#29724=CARTESIAN_POINT ( 'NONE',  ( 185.2584469233223388, 292.7362939515155631, -10.54904948314711177 ) ) ;
#29725=ORIENTED_EDGE ( 'NONE', *, *, #32427, .F. ) ;
#29726=CARTESIAN_POINT ( 'NONE',  ( 199.4720805209845196, 266.1420231043892954, 4.760232788326643316 ) ) ;
#29727=CARTESIAN_POINT ( 'NONE',  ( 159.1834766195183022, 255.6368035042336260, 16.04288454290252375 ) ) ;
#29728=CARTESIAN_POINT ( 'NONE',  ( 190.9576542968843569, 279.0470868181286619, -16.53509681315556890 ) ) ;
#29729=CARTESIAN_POINT ( 'NONE',  ( 192.9443876183610769, 296.4575129401721370, -13.55710008152484569 ) ) ;
#29730=CARTESIAN_POINT ( 'NONE',  ( 153.0790963368640689, 265.5062228982576471, -17.74594954892339160 ) ) ;
#29739=CARTESIAN_POINT ( 'NONE',  ( 205.0994677818405023, 275.4042965269534307, -14.14519517703424789 ) ) ;
#29740=CARTESIAN_POINT ( 'NONE',  ( 161.9775247817796924, 252.0936927241524472, 14.33142805341373283 ) ) ;
#29743=CARTESIAN_POINT ( 'NONE',  ( 164.3330377059402849, 246.0138246616164110, 7.208046019122525294 ) ) ;
#29744=CARTESIAN_POINT ( 'NONE',  ( 165.1530561822516461, 246.1540134663977426, 3.111834517001636602 ) ) ;
#29746=CARTESIAN_POINT ( 'NONE',  ( 149.0807665407234026, 276.4376266709116408, -5.539133476438467873 ) ) ;
#29749=CARTESIAN_POINT ( 'NONE',  ( 170.7538221939619518, 287.5752100735740555, -4.616036123583530326 ) ) ;
#29752=CARTESIAN_POINT ( 'NONE',  ( 178.0362721790638716, 255.4572819550275256, 5.227042922011960968 ) ) ;
#29753=CARTESIAN_POINT ( 'NONE',  ( 112.3797264076079756, 241.8149278399160949, 9.188101187500093303 ) ) ;
#29755=CARTESIAN_POINT ( 'NONE',  ( 183.3817364967617607, 260.1897163651752294, -9.412515908218015426 ) ) ;
#29757=CARTESIAN_POINT ( 'NONE',  ( 188.3087688221885685, 273.5212203147432319, 15.65619296925988380 ) ) ;
#29758=EDGE_LOOP ( 'NONE', ( #57441, #29767, #95896, #84712 ) ) ;
#29762=CARTESIAN_POINT ( 'NONE',  ( 192.8192650027745572, 296.6742316675438929, 11.53388506931248969 ) ) ;
#29764=ORIENTED_EDGE ( 'NONE', *, *, #59224, .T. ) ;
#29765=CARTESIAN_POINT ( 'NONE',  ( 147.9745743502305118, 274.3475143274592938, 10.02752110366533778 ) ) ;
#29766=( BOUNDED_CURVE ( )  B_SPLINE_CURVE ( 2, ( #92410, #17366, #34088, #95435, #41149, #18887, #56358, #9793, #3684 ),
 .UNSPECIFIED., .F., .T. ) 
 B_SPLINE_CURVE_WITH_KNOTS ( ( 3, 2, 2, 2, 3 ),
 ( 0.2459677419354838745, 0.2473118279569892497, 0.2500000000000000000, 0.2526881720430107503, 0.2540322580645161255 ),
 .UNSPECIFIED. ) 
 CURVE ( )  GEOMETRIC_REPRESENTATION_ITEM ( )  RATIONAL_B_SPLINE_CURVE ( ( 0.9330127018922194093, 0.9330127018922194093, 1.000000000000000000, 0.8660254037844387076, 1.000000000000000000, 0.8660254037844387076, 1.000000000000000000, 0.9330127018922194093, 0.9330127018922194093 ) ) 
 REPRESENTATION_ITEM ( '' )  );
#29767=ORIENTED_EDGE ( 'NONE', *, *, #98949, .F. ) ;
#29768=CARTESIAN_POINT ( 'NONE',  ( 45.83126033165611091, 187.2677522451417929, -5.000000000000041744 ) ) ;
#29770=CARTESIAN_POINT ( 'NONE',  ( 151.3542526322075901, 269.2885850756041464, -14.28695254860580199 ) ) ;
#29777=CARTESIAN_POINT ( 'NONE',  ( 153.4495116231415750, 264.8646448025247082, -16.73555355292144498 ) ) ;
#29779=CARTESIAN_POINT ( 'NONE',  ( 204.7705395286511703, 275.9740169735222821, 14.67688412961845579 ) ) ;
#29780=B_SPLINE_CURVE_WITH_KNOTS ( 'NONE', 3,
 ( #77111, #6726, #37604, #46712, #22420, #53311, #84266, #76624, #22908, #5724, #38608, #36612, #75634, #14813, #53795, #46195, #69512, #29041, #126, #6220, #31010, #61900, #92850, #59911, #90882, #21430, #37116, #68020, #48732, #77640, #39093, #8720, #31502, #79164, #32524, #72033, #2637, #24912, #47210, #32002, #47699, #64420, #25935, #33014 ),
 .UNSPECIFIED., .F., .F.,
 ( 4, 2, 2, 2, 2, 2, 2, 2, 2, 2, 2, 2, 2, 2, 2, 2, 2, 2, 2, 2, 2, 4 ),
 ( 0.001220187808576486330, 0.001695729215737192637, 0.002171270622897898944, 0.002409041326478252205, 0.002646812030058605034, 0.002765697381848733743, 0.002884582733638858115, 0.003122353437219106426, 0.003597894844379531491, 0.004073436251539956122, 0.005024519065860657933, 0.005975601880181360612, 0.006451143287341669884, 0.006926684694501980023, 0.007045570046292093554, 0.007105012722187119961, 0.007164455398082144634, 0.007283340749872173163, 0.007402226101662200825, 0.007877767508822457188, 0.008353308915982713551, 0.008828850323142968179 ),
 .UNSPECIFIED. ) ;
#29782=CARTESIAN_POINT ( 'NONE',  ( 190.6381889276718482, 264.1129242778857815, -9.562837835864641534 ) ) ;
#29783=CARTESIAN_POINT ( 'NONE',  ( 170.1122289929976432, 248.6907458515703411, -0.2685048055858946237 ) ) ;
#29784=CARTESIAN_POINT ( 'NONE',  ( 189.1301257125411723, 269.7442529300492424, -13.96337808587025719 ) ) ;
#29789=CARTESIAN_POINT ( 'NONE',  ( 189.6102000772831104, 298.8605291158151545, 7.657631583920184504 ) ) ;
#29791=CARTESIAN_POINT ( 'NONE',  ( 80.68904315757745849, 208.2048013555409796, 4.594050593750051981 ) ) ;
#29792=CARTESIAN_POINT ( 'NONE',  ( 159.3237119419271437, 254.6902313965507858, -15.56765445935501191 ) ) ;
#29793=CARTESIAN_POINT ( 'NONE',  ( -17.42236680055705023, 149.2012482093457777, 0.000000000000000000 ) ) ;
#29796=CARTESIAN_POINT ( 'NONE',  ( 197.3670252091396549, 288.0924216084537761, -16.92913523793449571 ) ) ;
#29797=CARTESIAN_POINT ( 'NONE',  ( 161.5757715694810770, 250.7895496999525449, -14.51803553215175135 ) ) ;
#29801=CARTESIAN_POINT ( 'NONE',  ( 112.2445834879230944, 245.6115022471903160, -5.000000000000047962 ) ) ;
#29807=CARTESIAN_POINT ( 'NONE',  ( 26.88721494746919660, 177.1423013555409796, -4.594050593750043987 ) ) ;
#29808=CARTESIAN_POINT ( 'NONE',  ( 52.43496435911014686, 191.8923013555410080, 4.594050593750050204 ) ) ;
#29809=CARTESIAN_POINT ( 'NONE',  ( 196.4982648257524147, 290.3020170531091821, 16.69353242256149628 ) ) ;
#29810=AXIS2_PLACEMENT_3D ( 'NONE', #95595, #86495, #48943 ) ;
#29813=CARTESIAN_POINT ( 'NONE',  ( 143.8274474304129171, 253.8458772461660260, 9.188101187500095079 ) ) ;
#29814=CARTESIAN_POINT ( 'NONE',  ( 50.56751030825868298, 193.8768266524160140, 9.188101187500096856 ) ) ;
#29816=CARTESIAN_POINT ( 'NONE',  ( 199.2383506163646132, 285.5560492466715345, -17.78808061564097898 ) ) ;
#29817=CARTESIAN_POINT ( 'NONE',  ( -15.56633235393031178, 168.4865022471903160, 10.00000000000009415 ) ) ;
#29822=CARTESIAN_POINT ( 'NONE',  ( 179.9582481332349460, 276.5203812193133217, 17.70049429017921128 ) ) ;
#29824=CARTESIAN_POINT ( 'NONE',  ( 153.5342532903791550, 264.7178679293513710, 18.03047267014487431 ) ) ;
#29828=CARTESIAN_POINT ( 'NONE',  ( 99.75938391669748739, 221.7365022471902023, 10.00000000000009592 ) ) ;
#29829=CARTESIAN_POINT ( 'NONE',  ( 161.3644539559160478, 251.1555625431813894, 12.97746593258196413 ) ) ;
#29830=CARTESIAN_POINT ( 'NONE',  ( 164.8599319342901310, 270.5031674125197583, -17.06886410118275776 ) ) ;
#29831=ORIENTED_EDGE ( 'NONE', *, *, #48309, .F. ) ;
#29832=CARTESIAN_POINT ( 'NONE',  ( 53.24634253151052832, 210.7369531367911293, -4.594050593750048428 ) ) ;
#29835=DIRECTION ( 'NONE',  ( 0.4999999999999998890, -0.8660254037844385966, 0.000000000000000000 ) ) ;
#29836=CARTESIAN_POINT ( 'NONE',  ( 190.5541309856500050, 300.5975588711562523, -4.167177996129430184 ) ) ;
#29837=CARTESIAN_POINT ( 'NONE',  ( 204.8008807586744524, 272.7600038595665524, -10.89009281376315741 ) ) ;
#29838=ADVANCED_FACE ( 'NONE', ( #89262 ), #38288, .F. ) ;
#29842=CARTESIAN_POINT ( 'NONE',  ( 148.0346525705264469, 274.2434557974783615, -9.381294579651672905 ) ) ;
#29845=CARTESIAN_POINT ( 'NONE',  ( 157.3370492947211119, 258.1312320390110244, 17.02065074437983228 ) ) ;
#29850=CARTESIAN_POINT ( 'NONE',  ( 170.8843335314017509, 274.4719442773359219, 17.28596511953734449 ) ) ;
#29852=CARTESIAN_POINT ( 'NONE',  ( 174.1122061744133021, 261.2364706500421789, -15.53837272058243890 ) ) ;
#29857=CARTESIAN_POINT ( 'NONE',  ( 159.4259928985412103, 282.8382026192845160, -3.335402803703788166 ) ) ;
#29859=CARTESIAN_POINT ( 'NONE',  ( 208.3790849386676598, 269.7238329819538762, -1.525282248498321946 ) ) ;
#29860=CARTESIAN_POINT ( 'NONE',  ( 204.2129321040862919, 276.9398213635460024, 14.41515352680879758 ) ) ;
#29861=CARTESIAN_POINT ( 'NONE',  ( 198.6587626159274294, 286.5599251108861267, 17.99840276545888784 ) ) ;
#29863=CARTESIAN_POINT ( 'NONE',  ( 128.9153121871758572, 254.4244531367911293, -4.594050593750046652 ) ) ;
#29864=CARTESIAN_POINT ( 'NONE',  ( 159.6568082460325115, 254.5034209454928202, -15.34944651258716242 ) ) ;
#29865=CARTESIAN_POINT ( 'NONE',  ( 178.8631597503538728, 258.1335624377610429, 9.789943529626453866 ) ) ;
#29866=CARTESIAN_POINT ( 'NONE',  ( 69.78227540684341079, 211.0958772461660544, -9.188101187500095079 ) ) ;
#29868=CARTESIAN_POINT ( 'NONE',  ( 174.0353712165220088, 265.6378307261092004, 16.31703135812460914 ) ) ;
#29869=CARTESIAN_POINT ( 'NONE',  ( 184.3288588942493504, 256.6513847527468215, 0.3136419966290590056 ) ) ;
#29870=ORIENTED_EDGE ( 'NONE', *, *, #30959, .F. ) ;
#29874=CARTESIAN_POINT ( 'NONE',  ( 80.03926378114135787, 227.0177522451419350, 5.000000000000046185 ) ) ;
#29876=CARTESIAN_POINT ( 'NONE',  ( 184.3226795282388650, 274.5458599865910969, 17.66928848808302988 ) ) ;
#29877=CARTESIAN_POINT ( 'NONE',  ( 191.1747001918821525, 299.5227014763493116, -9.654804683100723040 ) ) ;
#29879=CARTESIAN_POINT ( 'NONE',  ( 194.4165969972361552, 293.9075714965812267, 14.23342188338008718 ) ) ;
#29883=CARTESIAN_POINT ( 'NONE',  ( 201.0110605751355877, 282.4856255309966286, -16.99872517744415035 ) ) ;
#29890=CARTESIAN_POINT ( 'NONE',  ( 197.0145049354283913, 280.1669261707720580, 16.47791621818247165 ) ) ;
#29891=CARTESIAN_POINT ( 'NONE',  ( 198.2505066714982149, 285.2670451491296149, 0.000000000000000000 ) ) ;
#29892=CARTESIAN_POINT ( 'NONE',  ( 140.7695555451228984, 242.8923013555409796, 4.594050593750050204 ) ) ;
#29894=CARTESIAN_POINT ( 'NONE',  ( 1.096698433646719151, 159.8932355074535678, -2.679491924311248496 ) ) ;
#29895=CARTESIAN_POINT ( 'NONE',  ( 182.5394281695505185, 257.5236203636924301, 6.760540572999865994 ) ) ;
#29898=CARTESIAN_POINT ( 'NONE',  ( 153.2906404175950854, 265.1398178023911782, -17.60231834963988007 ) ) ;
#29902=CARTESIAN_POINT ( 'NONE',  ( 195.7060787468133185, 265.4134732632927580, 4.554624283109690808 ) ) ;
#29903=DIRECTION ( 'NONE',  ( -0.8660254037844387076, -0.4999999999999998890, -0.000000000000000000 ) ) ;
#29905=CARTESIAN_POINT ( 'NONE',  ( 184.7951035468651355, 263.5683215496842990, -12.50918047892673890 ) ) ;
#29907=EDGE_CURVE ( 'NONE', #22014, #42521, #31769, .T. ) ;
#29908=CARTESIAN_POINT ( 'NONE',  ( 198.7483143037687796, 265.7987759441807043, 0.1112591014730011513 ) ) ;
#29913=B_SPLINE_CURVE_WITH_KNOTS ( 'NONE', 3,
 ( #64373, #65367, #41050, #87747, #32963, #41559, #11195, #96309, #64881, #25893, #11688, #57756, #71986, #96816 ),
 .UNSPECIFIED., .F., .F.,
 ( 4, 2, 2, 2, 2, 2, 4 ),
 ( 0.0008768251031193197457, 0.001145890065292074367, 0.001414955027464828881, 0.001684019989637583394, 0.001953084951810337908, 0.002491214876155846934, 0.003029344800501355961 ),
 .UNSPECIFIED. ) ;
#29915=CARTESIAN_POINT ( 'NONE',  ( 177.3366806090162697, 264.4717330485077014, -15.58596816512555883 ) ) ;
#29916=CARTESIAN_POINT ( 'NONE',  ( 196.2319806131264954, 270.7896828814228911, 11.99002728859442257 ) ) ;
#29919=CARTESIAN_POINT ( 'NONE',  ( 151.2546443255573934, 275.3395117651207897, -9.775857568146751220 ) ) ;
#29922=CARTESIAN_POINT ( 'NONE',  ( 159.5764336135613632, 254.2525046211064819, 15.32981087583629076 ) ) ;
#29923=CARTESIAN_POINT ( 'NONE',  ( -16.57695564860984661, 170.4244531367911293, -4.594050593750046652 ) ) ;
#29926=CARTESIAN_POINT ( 'NONE',  ( 178.7469694055837692, 256.4911572975941567, 8.720117528295025622 ) ) ;
#29928=CARTESIAN_POINT ( 'NONE',  ( 199.1216527653377000, 285.7581758537840528, -18.37739894744384728 ) ) ;
#29929=CARTESIAN_POINT ( 'NONE',  ( 13.57207436428344316, 169.4548013555409796, -4.594050593750042211 ) ) ;
#29932=CARTESIAN_POINT ( 'NONE',  ( 157.7847820078105201, 257.3557362317297361, -18.02899742403477035 ) ) ;
#29934=CARTESIAN_POINT ( 'NONE',  ( 149.8257819617332700, 277.0756371120140784, 4.657797871342554963 ) ) ;
#29936=CARTESIAN_POINT ( 'NONE',  ( 175.5126768985223009, 253.5007195332992183, -3.702306847772006915 ) ) ;
#29937=CARTESIAN_POINT ( 'NONE',  ( 197.9988809731023025, 287.7028736432410483, 18.08661327024293897 ) ) ;
#29938=VECTOR ( 'NONE', #46069, 1000.000000000000000 ) ;
#29940=CARTESIAN_POINT ( 'NONE',  ( 181.9363424492615309, 295.0529423534600255, 1.015868974045746720 ) ) ;
#29941=CARTESIAN_POINT ( 'NONE',  ( 52.99401211233780629, 194.7365022471902023, 10.00000000000009592 ) ) ;
#29942=DIRECTION ( 'NONE',  ( 0.4999999999999998890, -0.8660254037844385966, 0.000000000000000000 ) ) ;
#29943=CARTESIAN_POINT ( 'NONE',  ( 8.456677953475336906, 181.8149278399161233, 9.188101187500093303 ) ) ;
#29947=CARTESIAN_POINT ( 'NONE',  ( 158.4546827590755811, 270.8972676159339699, 16.19068674916076844 ) ) ;
#29949=EDGE_CURVE ( 'NONE', #53789, #87662, #5213, .T. ) ;
#29950=CARTESIAN_POINT ( 'NONE',  ( 185.2016103895410595, 266.7518736163806352, 14.11053221384207212 ) ) ;
#29951=CARTESIAN_POINT ( 'NONE',  ( 153.7186906689185832, 265.0943440466812149, -16.48577743300708320 ) ) ;
#29952=CARTESIAN_POINT ( 'NONE',  ( 160.5614375844315305, 280.0629237280704160, 9.137926588329262856 ) ) ;
#29955=CARTESIAN_POINT ( 'NONE',  ( 147.7978300115112233, 274.6536445020713018, 7.902890709649431855 ) ) ;
#29957=CARTESIAN_POINT ( 'NONE',  ( 194.4459411895494725, 293.8567458645873103, 14.31012567920753042 ) ) ;
#29959=CARTESIAN_POINT ( 'NONE',  ( 184.7666555901016636, 290.6098824792631490, 12.15622735957478540 ) ) ;
#29961=EDGE_CURVE ( 'NONE', #48040, #35225, #18098, .T. ) ;
#29964=VERTEX_POINT ( 'NONE', #12002 ) ;
#29968=CARTESIAN_POINT ( 'NONE',  ( 155.5322964227545413, 261.2571557083629159, -18.35853982030605280 ) ) ;
#29970=ORIENTED_EDGE ( 'NONE', *, *, #32439, .T. ) ;
#29971=CARTESIAN_POINT ( 'NONE',  ( 186.2372707961799563, 272.0007479897874987, -16.24101813976637487 ) ) ;
#29972=CARTESIAN_POINT ( 'NONE',  ( 204.2556901454867955, 276.8657622634082713, 13.61111001399713949 ) ) ;
#29974=CARTESIAN_POINT ( 'NONE',  ( 201.3715986869907510, 281.8611552031986776, -17.89433714524984964 ) ) ;
#29976=FACE_OUTER_BOUND ( 'NONE', #44081, .T. ) ;
#29979=CARTESIAN_POINT ( 'NONE',  ( 148.1672759425158290, 274.0137453789218398, 7.847779094015780110 ) ) ;
#29981=ORIENTED_EDGE ( 'NONE', *, *, #96544, .F. ) ;
#29982=CARTESIAN_POINT ( 'NONE',  ( 206.3907062969896060, 273.1678058140250300, 11.56942460516550675 ) ) ;
#29984=ORIENTED_EDGE ( 'NONE', *, *, #48746, .T. ) ;
#29985=CARTESIAN_POINT ( 'NONE',  ( 190.2318383114841254, 301.1557861577188078, 3.177919994438449525 ) ) ;
#29991=CARTESIAN_POINT ( 'NONE',  ( 103.3262782077763120, 218.9155109091896065, 2.679491924311254714 ) ) ;
#29993=VERTEX_POINT ( 'NONE', #50478 ) ;
#29995=CARTESIAN_POINT ( 'NONE',  ( 147.5498377207569263, 275.0831797495432056, 4.097967709737811326 ) ) ;
#29996=CARTESIAN_POINT ( 'NONE',  ( 147.6430623265936219, 274.9217099957185155, 8.258152514891218487 ) ) ;
#29997=CARTESIAN_POINT ( 'NONE',  ( 149.1903793729515257, 272.2416782560088677, 12.95958987445043675 ) ) ;
#29998=CARTESIAN_POINT ( 'NONE',  ( 192.6224552386041182, 297.0151161785129261, 12.49354144254605181 ) ) ;
#29999=CARTESIAN_POINT ( 'NONE',  ( 147.1749864263339020, 275.7324412367667605, 0.5903044561608349339 ) ) ;
#30000=CARTESIAN_POINT ( 'NONE',  ( 191.8456210280128005, 298.3606325003146367, -9.135603544929113085 ) ) ;
#30001=CARTESIAN_POINT ( 'NONE',  ( 159.9040744856012850, 255.4269131533854420, 16.38690128260775936 ) ) ;
#30003=CARTESIAN_POINT ( 'NONE',  ( 149.4965729687386045, 271.7113353911534546, -11.48413836595348059 ) ) ;
#30006=CARTESIAN_POINT ( 'NONE',  ( 168.1440244810862055, 286.5563420518730027, 3.650993266842447849 ) ) ;
#30010=CARTESIAN_POINT ( 'NONE',  ( 190.3243315981879107, 300.9955830857887236, -4.786543493425554630 ) ) ;
#30012=CARTESIAN_POINT ( 'NONE',  ( 202.9053066868392818, 278.8211341806578503, 15.06259384972848636 ) ) ;
#30015=CARTESIAN_POINT ( 'NONE',  ( 190.8763451968731886, 298.2172932904716731, -9.609917527147246119 ) ) ;
#30017=CARTESIAN_POINT ( 'NONE',  ( 169.1095075563655143, 285.5585736834383965, -7.565734909916525197 ) ) ;
#30020=CARTESIAN_POINT ( 'NONE',  ( 206.8851632406098702, 272.3113812655195716, -9.957011741946159233 ) ) ;
#30022=CARTESIAN_POINT ( 'NONE',  ( 42.80017141841058503, 185.5177522451417929, 5.000000000000051514 ) ) ;
#30023=CARTESIAN_POINT ( 'NONE',  ( 112.9213393807382886, 229.8768266524160140, 9.188101187500096856 ) ) ;
#30025=CARTESIAN_POINT ( 'NONE',  ( 199.1944722252943905, 285.6320488493591938, -18.17555833707144686 ) ) ;
#30027=CARTESIAN_POINT ( 'NONE',  ( 157.3412122618683497, 258.1240215684019290, 16.75554199904894048 ) ) ;
#30028=CARTESIAN_POINT ( 'NONE',  ( 172.2604035111071994, 250.9201653963260696, -4.030415234405903213 ) ) ;
#30029=CARTESIAN_POINT ( 'NONE',  ( 30.29666933122289407, 197.4869531367911293, 4.594050593750046652 ) ) ;
#30031=VERTEX_POINT ( 'NONE', #95651 ) ;
#30032=CARTESIAN_POINT ( 'NONE',  ( 176.7754569686200625, 262.2288517614920238, -15.26617267356994567 ) ) ;
#30033=CARTESIAN_POINT ( 'NONE',  ( 177.9063225670694521, 265.5284957633090244, 15.62507714768716305 ) ) ;
#30034=EDGE_CURVE ( 'NONE', #71782, #85768, #64310, .T. ) ;
#30041=CARTESIAN_POINT ( 'NONE',  ( 104.3601438707544133, 224.3927522451418213, -10.00000000000009059 ) ) ;
#30043=ORIENTED_EDGE ( 'NONE', *, *, #21952, .T. ) ;
#30045=CARTESIAN_POINT ( 'NONE',  ( 155.4838159167009906, 279.7196639355038883, -1.614956184126561611 ) ) ;
#30046=CARTESIAN_POINT ( 'NONE',  ( -27.42236680055714260, 166.5217562850347406, 1.224646799147364892E-15 ) ) ;
#30048=CARTESIAN_POINT ( 'NONE',  ( 12.00188267627663308, 186.9244531367911293, -4.594050593750046652 ) ) ;
#30050=CARTESIAN_POINT ( 'NONE',  ( 192.2734905965078553, 272.0667696282540646, 14.25396137523372886 ) ) ;
#30051=CARTESIAN_POINT ( 'NONE',  ( 192.4867975473904949, 297.2500821921321972, -13.04960750009181325 ) ) ;
#30053=CARTESIAN_POINT ( 'NONE',  ( 174.4584291273796453, 286.7546150749506637, 10.19462971651400807 ) ) ;
#30054=CARTESIAN_POINT ( 'NONE',  ( 57.27886009182306282, 210.0024278399160949, -9.188101187500093303 ) ) ;
#30055=CARTESIAN_POINT ( 'NONE',  ( 200.3414094930810165, 283.6454952284590263, 16.87912319229835489 ) ) ;
#30059=( BOUNDED_CURVE ( )  B_SPLINE_CURVE ( 2, ( #73093, #35054, #11788, #81704, #4669, #10783, #2690, #96407, #88838 ),
 .UNSPECIFIED., .F., .T. ) 
 B_SPLINE_CURVE_WITH_KNOTS ( ( 3, 2, 2, 2, 3 ),
 ( 0.5766129032258064946, 0.5779569892473118697, 0.5806451612903226200, 0.5833333333333333703, 0.5846774193548387455 ),
 .UNSPECIFIED. ) 
 CURVE ( )  GEOMETRIC_REPRESENTATION_ITEM ( )  RATIONAL_B_SPLINE_CURVE ( ( 0.9330127018922194093, 0.9330127018922194093, 1.000000000000000000, 0.8660254037844387076, 1.000000000000000000, 0.8660254037844387076, 1.000000000000000000, 0.9330127018922194093, 0.9330127018922194093 ) ) 
 REPRESENTATION_ITEM ( '' )  );
#30060=ORIENTED_EDGE ( 'NONE', *, *, #96231, .T. ) ;
#30063=CARTESIAN_POINT ( 'NONE',  ( 165.4943819508360434, 269.3512166473536809, 17.11647148302431631 ) ) ;
#30064=CARTESIAN_POINT ( 'NONE',  ( 10.91961124514380366, 177.1115022471902307, 10.00000000000009592 ) ) ;
#30065=CARTESIAN_POINT ( 'NONE',  ( 163.9354095869165633, 246.7025367662834014, -7.289870401565430313 ) ) ;
#30066=CARTESIAN_POINT ( 'NONE',  ( 134.1114646098825176, 257.4244531367911577, -4.594050593750046652 ) ) ;
#30068=B_SPLINE_CURVE_WITH_KNOTS ( 'NONE', 3,
 ( #9141, #30934, #61817, #7129, #68926, #8143, #62826, #77555, #53718, #1556, #31424, #53237, #61324, #78553, #7634, #54718, #39017, #93782, #62314, #93269, #77028, #39506, #38013, #70433, #85700, #16236, #47626, #92769, #31922, #30435, #84189, #47127, #24341, #70954, #78050, #50, #32440, #92286, #55216, #91774, #22339, #14738, #45621, #99851, #84678, #22833 ),
 .UNSPECIFIED., .F., .F.,
 ( 4, 2, 2, 2, 2, 2, 2, 2, 2, 2, 2, 2, 2, 2, 2, 2, 2, 2, 2, 2, 2, 2, 4 ),
 ( 0.0005579239295771397551, 0.001560669089151106408, 0.002062041668938070435, 0.002187384813884852858, 0.002312727958831635282, 0.002438071103778417272, 0.002563414248725199695, 0.002814100538618904621, 0.003064786828512609980, 0.003566159408300144298, 0.004568904567875151784, 0.005571649727450158837, 0.006073022307237618128, 0.006323708597131346906, 0.006574394887025075684, 0.006699738031971940941, 0.006762409604445303313, 0.006825081176918663950, 0.007075767466812139458, 0.007577140046599087006, 0.008078512626386038023, 0.008329198916279562104, 0.008579885206173084450 ),
 .UNSPECIFIED. ) ;
#30070=ADVANCED_FACE ( 'NONE', ( #2410 ), #57579, .T. ) ;
#30077=B_SPLINE_CURVE_WITH_KNOTS ( 'NONE', 3,
 ( #95484, #73141, #10830, #41710 ),
 .UNSPECIFIED., .F., .F.,
 ( 4, 4 ),
 ( 0.01048155653827781073, 0.01885456469717847194 ),
 .UNSPECIFIED. ) ;
#30079=CARTESIAN_POINT ( 'NONE',  ( 151.8246416459486738, 268.5104669391655534, -14.87942003997596352 ) ) ;
#30082=ORIENTED_EDGE ( 'NONE', *, *, #42120, .T. ) ;
#30083=FACE_OUTER_BOUND ( 'NONE', #77605, .T. ) ;
#30089=DIRECTION ( 'NONE',  ( -0.8660254037844387076, -0.4999999999999998890, -0.000000000000000000 ) ) ;
#30090=CARTESIAN_POINT ( 'NONE',  ( 204.2441997346916480, 270.1807567755661807, -7.723805382780020601 ) ) ;
#30092=DIRECTION ( 'NONE',  ( 0.4999999999999992784, -0.8660254037844390407, 0.000000000000000000 ) ) ;
#30094=CARTESIAN_POINT ( 'NONE',  ( 152.8651171364917900, 265.8768457450651113, -16.25664868183201861 ) ) ;
#30095=ORIENTED_EDGE ( 'NONE', *, *, #85133, .T. ) ;
#30096=CARTESIAN_POINT ( 'NONE',  ( 190.7801068464975742, 281.0515339637562420, 16.66579443870669053 ) ) ;
#30100=CARTESIAN_POINT ( 'NONE',  ( 149.7162292714551199, 271.3308795146458010, 12.12826134257344357 ) ) ;
#30101=CARTESIAN_POINT ( 'NONE',  ( 200.3293654959697392, 273.7156512906800572, 13.98704503334941229 ) ) ;
#30104=CARTESIAN_POINT ( 'NONE',  ( 191.5521510896938935, 298.8689373439769952, -9.847378829740700112 ) ) ;
#30106=CARTESIAN_POINT ( 'NONE',  ( 204.5133713884061706, 276.4194452585140311, 14.87364779308245843 ) ) ;
#30108=ORIENTED_EDGE ( 'NONE', *, *, #28815, .T. ) ;
#30109=CARTESIAN_POINT ( 'NONE',  ( 96.08779704679574252, 226.2833772461660260, -9.188101187500095079 ) ) ;
#30110=CARTESIAN_POINT ( 'NONE',  ( 203.1594176127779861, 278.7645619890024591, 16.51125172500342231 ) ) ;
#30111=CARTESIAN_POINT ( 'NONE',  ( 178.0116618716515973, 269.0027435595893053, -16.91056692113554760 ) ) ;
#30115=ORIENTED_EDGE ( 'NONE', *, *, #53722, .F. ) ;
#30120=CARTESIAN_POINT ( 'NONE',  ( 207.5570596878370679, 271.1476224814971374, 2.444960520848353358 ) ) ;
#30121=CARTESIAN_POINT ( 'NONE',  ( -22.42236680055709641, 157.8615022471902591, 0.000000000000000000 ) ) ;
#30127=AXIS2_PLACEMENT_3D ( 'NONE', #97464, #49843, #11378 ) ;
#30128=FACE_OUTER_BOUND ( 'NONE', #59722, .T. ) ;
#30130=CARTESIAN_POINT ( 'NONE',  ( -22.42236680055709641, 157.8615022471902591, 0.000000000000000000 ) ) ;
#30131=ORIENTED_EDGE ( 'NONE', *, *, #35562, .F. ) ;
#30132=CARTESIAN_POINT ( 'NONE',  ( 202.2603678735342214, 280.3217618159037556, 16.49712126737133744 ) ) ;
#30133=CARTESIAN_POINT ( 'NONE',  ( 185.5178088754986732, 257.9886162347545451, 3.053422304497617645 ) ) ;
#30134=CARTESIAN_POINT ( 'NONE',  ( 165.7096765433480243, 246.6079469402106668, -2.628825658309415836 ) ) ;
#30137=CARTESIAN_POINT ( 'NONE',  ( 168.4964275335260879, 253.5783752955648822, 11.53270701355078742 ) ) ;
#30138=CARTESIAN_POINT ( 'NONE',  ( 192.8389457671851801, 263.0020653644326103, -0.7569367516056485501 ) ) ;
#30140=CARTESIAN_POINT ( 'NONE',  ( 181.6867268255581678, 270.7552855298207533, -16.03927706080179760 ) ) ;
#30143=CARTESIAN_POINT ( 'NONE',  ( 0.4370954166216904357, 184.3927522451419350, 2.944929066748280225E-16 ) ) ;
#30145=CARTESIAN_POINT ( 'NONE',  ( 193.1774878905343371, 266.9097302922900781, -11.44520343211384983 ) ) ;
#30147=CARTESIAN_POINT ( 'NONE',  ( 203.5750579584898219, 278.0446517925538501, -15.66676355934540332 ) ) ;
#30150=CARTESIAN_POINT ( 'NONE',  ( -9.729855525997876953, 171.3149278399160664, 9.188101187500093303 ) ) ;
#30151=CARTESIAN_POINT ( 'NONE',  ( 4.599382176350318652, 161.9155109091896350, 2.679491924311254714 ) ) ;
#30152=CARTESIAN_POINT ( 'NONE',  ( 188.9734557794317595, 297.2153733544514012, 9.139690452204975557 ) ) ;
#30156=CARTESIAN_POINT ( 'NONE',  ( 161.5266078408477597, 251.3399204103630211, 13.01505764280997468 ) ) ;
#30157=EDGE_CURVE ( 'NONE', #46058, #60977, #90909, .T. ) ;
#30158=CARTESIAN_POINT ( 'NONE',  ( 200.1233510698300222, 282.0231834965481994, 17.42297826929840809 ) ) ;
#30159=AXIS2_PLACEMENT_3D ( 'NONE', #84607, #15146, #46043 ) ;
#30162=CARTESIAN_POINT ( 'NONE',  ( 162.7471009177916130, 248.7607477562823703, -10.22904224531126438 ) ) ;
#30164=CARTESIAN_POINT ( 'NONE',  ( 152.5937463967839847, 278.0176957858930678, 3.715656952871561280 ) ) ;
#30165=CARTESIAN_POINT ( 'NONE',  ( 13.97758990260114231, 185.0024278399160949, 9.188101187500095079 ) ) ;
#30166=CARTESIAN_POINT ( 'NONE',  ( 125.2893514524760548, 233.9548013555409796, -4.594050593750042211 ) ) ;
#30171=CARTESIAN_POINT ( 'NONE',  ( 190.5526305594705434, 299.9695577504274979, -4.324655322867677398 ) ) ;
#30172=CARTESIAN_POINT ( 'NONE',  ( 157.2333142128019858, 258.3109064714224132, 16.87956768598436597 ) ) ;
#30173=CARTESIAN_POINT ( 'NONE',  ( 193.7118145980225279, 295.1282904202991517, 14.61271143546694162 ) ) ;
#30174=CARTESIAN_POINT ( 'NONE',  ( 161.6755750489535046, 250.6166850027345276, -13.01404233079112061 ) ) ;
#30175=CARTESIAN_POINT ( 'NONE',  ( 189.8944967759784390, 284.6695464243575771, 16.74947250714170011 ) ) ;
#30176=CARTESIAN_POINT ( 'NONE',  ( 167.7287949414774744, 278.2917028285691003, 14.65232981943655588 ) ) ;
#30177=CARTESIAN_POINT ( 'NONE',  ( 189.8280524984248530, 300.0247317190094236, -0.5815489268893287989 ) ) ;
#30180=CARTESIAN_POINT ( 'NONE',  ( 184.4418290349794347, 268.6877477094485585, -15.38013229235870583 ) ) ;
#30184=CARTESIAN_POINT ( 'NONE',  ( 163.7012083107868534, 247.1081852757374975, -6.544933039329257518 ) ) ;
#30185=CARTESIAN_POINT ( 'NONE',  ( 185.1206366404793471, 269.5993361517367362, 15.81333004430259948 ) ) ;
#30186=CARTESIAN_POINT ( 'NONE',  ( 99.98491136382573075, 228.5333772461660828, 9.188101187500095079 ) ) ;
#30188=CARTESIAN_POINT ( 'NONE',  ( 191.4044787581200069, 299.1247133251352466, 7.435199718141230818 ) ) ;
#30189=CARTESIAN_POINT ( 'NONE',  ( 177.1347673595945764, 262.9921672455169528, 15.53478677465993485 ) ) ;
#30191=CARTESIAN_POINT ( 'NONE',  ( 103.4219496833212162, 240.5177522451419350, 5.000000000000046185 ) ) ;
#30192=B_SPLINE_CURVE_WITH_KNOTS ( 'NONE', 3,
 ( #80162, #19350, #11730, #34432 ),
 .UNSPECIFIED., .F., .F.,
 ( 4, 4 ),
 ( 0.009240307309658310833, 0.01507866790100597862 ),
 .UNSPECIFIED. ) ;
#30193=CARTESIAN_POINT ( 'NONE',  ( 201.7550856928311589, 271.1410374022044607, -9.839847481188424894 ) ) ;
#30194=CARTESIAN_POINT ( 'NONE',  ( 198.5970767652345899, 286.6667681383942181, -17.17073100918929640 ) ) ;
#30195=DIRECTION ( 'NONE',  ( -0.8660254037844387076, -0.4999999999999998890, -0.000000000000000000 ) ) ;
#30198=CARTESIAN_POINT ( 'NONE',  ( 4.767222435543962078, 166.8927522451418213, 10.00000000000009948 ) ) ;
#30201=CARTESIAN_POINT ( 'NONE',  ( 178.5316424161641748, 280.3506190370360400, 15.79244575417478735 ) ) ;
#30203=CARTESIAN_POINT ( 'NONE',  ( 147.5749398328735822, 275.0397016159798227, -4.620786157167191099 ) ) ;
#30204=CARTESIAN_POINT ( 'NONE',  ( 149.1486417047969155, 272.3139700178423368, -11.47583619705022606 ) ) ;
#30205=EDGE_CURVE ( 'NONE', #45578, #34461, #53703, .T. ) ;
#30211=CARTESIAN_POINT ( 'NONE',  ( 182.9169972424188586, 263.6770152411878598, -13.86124712002487236 ) ) ;
#30212=CARTESIAN_POINT ( 'NONE',  ( 169.9766547505107894, 252.5201543592683322, -8.760183188246276842 ) ) ;
#30213=CARTESIAN_POINT ( 'NONE',  ( 171.0458462729697260, 282.1216204770890386, -14.11865471209823930 ) ) ;
#30214=EDGE_LOOP ( 'NONE', ( #80498, #37205, #85482 ) ) ;
#30217=VERTEX_POINT ( 'NONE', #8374 ) ;
#30218=CARTESIAN_POINT ( 'NONE',  ( 168.1909178643507232, 248.9330331115285162, 6.596560970029747395 ) ) ;
#30219=CARTESIAN_POINT ( 'NONE',  ( 182.3561040761404968, 291.0252386590130413, -10.82420555737414247 ) ) ;
#30223=CARTESIAN_POINT ( 'NONE',  ( 190.8872452503548232, 277.9998427814335855, -17.37787329346898346 ) ) ;
#30224=CARTESIAN_POINT ( 'NONE',  ( 192.7446300355631479, 296.8035032227751913, -13.50572488576995411 ) ) ;
#30225=CARTESIAN_POINT ( 'NONE',  ( 152.7691010214056462, 266.0431505347400503, -16.40662330462167162 ) ) ;
#30234=CARTESIAN_POINT ( 'NONE',  ( 175.3460070743044810, 258.5034201212096718, 13.02170940230438667 ) ) ;
#30236=VERTEX_POINT ( 'NONE', #1275 ) ;
#30240=CARTESIAN_POINT ( 'NONE',  ( 174.4482263059820468, 257.3207558651999989, -11.99955440495903858 ) ) ;
#30241=CARTESIAN_POINT ( 'NONE',  ( 190.6324986747941068, 299.9733286590040962, -4.183702684017944762 ) ) ;
#30242=CARTESIAN_POINT ( 'NONE',  ( 165.0424088038023456, 244.7851578786982145, -1.332161216135762105 ) ) ;
#30243=CARTESIAN_POINT ( 'NONE',  ( 197.5277397434883255, 272.9434654477590243, -13.23775816460648080 ) ) ;
#30245=CARTESIAN_POINT ( 'NONE',  ( 147.9748066657072627, 274.3471119452502762, 9.387104374042873900 ) ) ;
#30246=CARTESIAN_POINT ( 'NONE',  ( 171.6332223966747392, 250.6993909615997609, -5.719266321659834063 ) ) ;
#30247=CARTESIAN_POINT ( 'NONE',  ( 165.8055607888911709, 266.0341751366186713, 17.30635120499955804 ) ) ;
#30248=CARTESIAN_POINT ( 'NONE',  ( 185.1069551167274199, 285.7384112475837696, -15.13345330922732401 ) ) ;
#30249=CARTESIAN_POINT ( 'NONE',  ( 113.4086522182495145, 224.0327760586659451, 1.948934522072303157E-15 ) ) ;
#30252=CARTESIAN_POINT ( 'NONE',  ( 160.9978133751494624, 283.8066770274658666, 2.192527523246561749 ) ) ;
#30253=CARTESIAN_POINT ( 'NONE',  ( 187.9688059934449313, 273.8547072571687409, 16.05218478527549308 ) ) ;
#30256=CARTESIAN_POINT ( 'NONE',  ( 180.1453383632374994, 295.1715722599841456, -2.140036363759055149 ) ) ;
#30257=CARTESIAN_POINT ( 'NONE',  ( 196.0727848089514964, 291.0389700598140621, 17.56388901715066808 ) ) ;
#30258=CARTESIAN_POINT ( 'NONE',  ( 159.3995226465659982, 254.5589234043588078, -16.81133486613867234 ) ) ;
#30261=CARTESIAN_POINT ( 'NONE',  ( 194.7222134385861807, 293.3782282925342884, 16.03497216414424997 ) ) ;
#30264=ORIENTED_EDGE ( 'NONE', *, *, #79664, .T. ) ;
#30265=CARTESIAN_POINT ( 'NONE',  ( 191.7763301340909265, 267.4862631225445853, -12.60863414139059735 ) ) ;
#30266=B_SPLINE_CURVE_WITH_KNOTS ( 'NONE', 3,
 ( #44091, #74034, #98331, #50217, #21319, #81171, #27434, #89763, #43092, #36003, #75035, #11736, #27912, #58308, #5612, #42600, #13714, #4624, #20837, #4115, #51729, #75524, #89285, #36504, #81658, #59798, #82168, #67407, #66908, #44589 ),
 .UNSPECIFIED., .F., .F.,
 ( 4, 2, 2, 2, 2, 2, 2, 2, 2, 2, 2, 2, 2, 2, 4 ),
 ( 0.001616355120345336219, 0.002274024124150745597, 0.002931693127956154325, 0.004247031135566920607, 0.004904700139372303314, 0.005233534641275029362, 0.005397951892226427080, 0.005439056204964282798, 0.005480160517702137649, 0.005521264830439992499, 0.005562369143177847350, 0.005726786394129246803, 0.005891203645080646256, 0.006220038146983454704, 0.006877707150789046445 ),
 .UNSPECIFIED. ) ;
#30267=CARTESIAN_POINT ( 'NONE',  ( 193.6139411566157378, 262.7946681891672256, 4.750614067181518685 ) ) ;
#30268=CARTESIAN_POINT ( 'NONE',  ( -11.32641631811692662, 174.2677522451419350, -5.000000000000047962 ) ) ;
#30269=CARTESIAN_POINT ( 'NONE',  ( 202.8211298556536804, 279.3504935719197988, 17.07914446815911447 ) ) ;
#30270=CARTESIAN_POINT ( 'NONE',  ( 184.3160629641438106, 288.6786004691003882, -13.34280541894466765 ) ) ;
#30273=ORIENTED_EDGE ( 'NONE', *, *, #99722, .F. ) ;
#30275=CARTESIAN_POINT ( 'NONE',  ( 147.5813496936708020, 275.0285994114094592, 4.516581957185684004 ) ) ;
#30277=CARTESIAN_POINT ( 'NONE',  ( 189.7845653727764272, 264.2201878795776224, -9.220148691588715195 ) ) ;
#30278=CARTESIAN_POINT ( 'NONE',  ( 192.9083073729183582, 270.9347064964478022, 14.76982790152045055 ) ) ;
#30279=CARTESIAN_POINT ( 'NONE',  ( 192.3260883533780259, 271.6660879014408465, -14.49459676434517164 ) ) ;
#30286=CARTESIAN_POINT ( 'NONE',  ( 155.6435836392643637, 261.0644005951349982, 17.58841156286628049 ) ) ;
#30287=CARTESIAN_POINT ( 'NONE',  ( 32.20940242151128530, 182.7365022471902876, 10.00000000000009948 ) ) ;
#30289=ADVANCED_FACE ( 'NONE', ( #47845 ), #38245, .T. ) ;
#30290=CARTESIAN_POINT ( 'NONE',  ( 77.41429782557628414, 209.3768266524159571, -9.188101187500091527 ) ) ;
#30291=CARTESIAN_POINT ( 'NONE',  ( 206.1798448551755598, 273.5330285446045195, -10.53862763475382813 ) ) ;
#30292=CARTESIAN_POINT ( 'NONE',  ( 192.5284579606305613, 297.1779242397361713, -13.15228012403107272 ) ) ;
#30293=CARTESIAN_POINT ( 'NONE',  ( 207.8446715390582540, 270.6494641423232679, -2.429516028743652800 ) ) ;
#30294=EDGE_CURVE ( 'NONE', #90439, #57797, #14780, .T. ) ;
#30295=CARTESIAN_POINT ( 'NONE',  ( 196.2506489124965299, 288.9087261997057112, -17.23880585552221234 ) ) ;
#30296=CARTESIAN_POINT ( 'NONE',  ( 161.3773209892555371, 251.1332761876949746, -14.50043705923759241 ) ) ;
#30299=B_SPLINE_CURVE_WITH_KNOTS ( 'NONE', 3,
 ( #54125, #47048, #8557, #85087 ),
 .UNSPECIFIED., .F., .F.,
 ( 4, 4 ),
 ( 0.04103871331059693456, 0.04887120950165270428 ),
 .UNSPECIFIED. ) ;
#30303=CARTESIAN_POINT ( 'NONE',  ( 205.4651907542742890, 274.7708457572024940, -12.42986464854210027 ) ) ;
#30304=B_SPLINE_CURVE_WITH_KNOTS ( 'NONE', 3,
 ( #60462, #84326, #93419, #21980, #37665, #52874, #91927, #83825, #45275, #68575, #38154, #69072, #30582, #92418, #22968, #53855, #46252, #77176, #78697, #39649, #9284, #16873, #10789, #32064, #33587, #26489, #72096, #80221, #63479, #56370, #17897, #1699, #2696, #18897, #71600, #40159, #71100, #86841, #57366, #86336, #17376, #88340, #55358, #32582, #24477, #34095, #94416, #24969 ),
 .UNSPECIFIED., .F., .F.,
 ( 4, 2, 2, 2, 2, 2, 2, 2, 2, 2, 2, 2, 2, 2, 2, 2, 2, 2, 2, 2, 2, 2, 2, 4 ),
 ( 0.002501527887315633213, 0.002918846236623728971, 0.003127505411277738470, 0.003231834998604704405, 0.003336164585931669906, 0.003440494173258635408, 0.003544823760585601342, 0.003753482935239675460, 0.004170801284547748233, 0.005005437983164006538, 0.005840074681780264843, 0.006674711380396523147, 0.007092029729704573369, 0.007509348079012624459, 0.007613677666339734376, 0.007665842460003294105, 0.007718007253666853834, 0.007770172047330414430, 0.007822336840993975027, 0.007926666428321096219, 0.008135325602975338605, 0.008343984777629584459, 0.008761303126938145558, 0.009178621476246706656 ),
 .UNSPECIFIED. ) ;
#30305=CARTESIAN_POINT ( 'NONE',  ( 195.6974783896144174, 291.6890198465123945, 16.70600479393688431 ) ) ;
#30307=CARTESIAN_POINT ( 'NONE',  ( 27.59033994439653270, 195.9244531367911293, -4.594050593750046652 ) ) ;
#30308=VECTOR ( 'NONE', #47384, 1000.000000000000000 ) ;
#30309=CARTESIAN_POINT ( 'NONE',  ( 60.22919299317007358, 196.3923013555409796, 4.594050593750050204 ) ) ;
#30311=CARTESIAN_POINT ( 'NONE',  ( 199.4509464742678801, 277.6162209133078704, 15.23248329428225389 ) ) ;
#30313=CARTESIAN_POINT ( 'NONE',  ( -13.68994397906405602, 176.2365022471903444, 2.944929066748280225E-16 ) ) ;
#30314=CARTESIAN_POINT ( 'NONE',  ( 50.64826632015721231, 209.2369531367911293, -4.594050593750048428 ) ) ;
#30317=CARTESIAN_POINT ( 'NONE',  ( -14.62813816649718213, 172.3615022471903160, 5.000000000000046185 ) ) ;
#30318=CARTESIAN_POINT ( 'NONE',  ( -7.699934936221591641, 156.3615022471902023, 5.000000000000051514 ) ) ;
#30320=CARTESIAN_POINT ( 'NONE',  ( 205.2391015854675516, 275.1624436846170738, -14.01434138479280911 ) ) ;
#30321=CARTESIAN_POINT ( 'NONE',  ( 158.9583395483327308, 256.9617481484739869, -16.95571191692422275 ) ) ;
#30322=CARTESIAN_POINT ( 'NONE',  ( 175.6268470825654049, 291.0373744556468409, 2.379281674685343351 ) ) ;
#30323=CARTESIAN_POINT ( 'NONE',  ( 159.6898930778639283, 254.0559870643349143, 16.90891900388599822 ) ) ;
#30325=CARTESIAN_POINT ( 'NONE',  ( 201.3244920114063063, 281.9427463586865201, 17.21113171619803595 ) ) ;
#30327=CARTESIAN_POINT ( 'NONE',  ( 114.8426596992764388, 237.1115022471902307, 10.00000000000009592 ) ) ;
#30333=CARTESIAN_POINT ( 'NONE',  ( 206.3423291502491566, 273.2515974901050413, -10.76717883871977577 ) ) ;
#30334=CARTESIAN_POINT ( 'NONE',  ( 190.0974356945988575, 279.3567963776670240, -17.44568797921136039 ) ) ;
#30335=CARTESIAN_POINT ( 'NONE',  ( 189.5255948787495015, 270.7606473226053367, 15.83079519377715627 ) ) ;
#30337=DIRECTION ( 'NONE',  ( -0.8660254037844387076, -0.4999999999999998890, -0.000000000000000000 ) ) ;
#30338=CARTESIAN_POINT ( 'NONE',  ( 164.9779129355220562, 244.8968679994381148, -1.771286574179712803 ) ) ;
#30339=CARTESIAN_POINT ( 'NONE',  ( 147.6264044922760377, 274.9505622111005323, -8.841872555777701592 ) ) ;
#30341=CYLINDRICAL_SURFACE ( 'NONE', #76458, 17.82106496071139645 ) ;
#30344=EDGE_LOOP ( 'NONE', ( #73433, #57511, #89949 ) ) ;
#30349=CARTESIAN_POINT ( 'NONE',  ( -22.42236680055709641, 157.8615022471902591, 0.000000000000000000 ) ) ;
#30352=CARTESIAN_POINT ( 'NONE',  ( -6.130263895410251962, 167.2677522451418781, 10.00000000000009592 ) ) ;
#30354=CARTESIAN_POINT ( 'NONE',  ( 174.8261646120922421, 286.1039399097584806, 11.04222616188278749 ) ) ;
#30356=CARTESIAN_POINT ( 'NONE',  ( 160.1224120645151174, 282.3532393352595591, -3.187131287737694052 ) ) ;
#30358=CARTESIAN_POINT ( 'NONE',  ( 163.2742264920156572, 247.8477394797576778, -9.850275379362519956 ) ) ;
#30359=CARTESIAN_POINT ( 'NONE',  ( 204.2457645315488719, 276.8829539310449945, 14.53406579917280261 ) ) ;
#30360=CARTESIAN_POINT ( 'NONE',  ( 188.7060284211345618, 295.2753450948700902, -11.24849810963761776 ) ) ;
#30361=CARTESIAN_POINT ( 'NONE',  ( 204.0604753336787667, 271.4817813032398703, 9.862283393711939183 ) ) ;
#30363=CARTESIAN_POINT ( 'NONE',  ( 137.1160976468485728, 237.7202760586660020, -5.415160957724236172E-17 ) ) ;
#30364=CARTESIAN_POINT ( 'NONE',  ( 160.1889510292459704, 254.1022327335691955, -15.33409651099172777 ) ) ;
#30366=CARTESIAN_POINT ( 'NONE',  ( 181.9407744531946491, 260.3728692333327785, 9.471612455673151132 ) ) ;
#30367=CARTESIAN_POINT ( 'NONE',  ( 71.43287601098374751, 221.2369531367911293, -4.594050593750048428 ) ) ;
#30368=ORIENTED_EDGE ( 'NONE', *, *, #98725, .T. ) ;
#30372=CARTESIAN_POINT ( 'NONE',  ( 167.2515702596184042, 262.0622343731731689, -17.21809106051008342 ) ) ;
#30378=CARTESIAN_POINT ( 'NONE',  ( 146.9456733906991417, 276.1296230653242105, -0.7988785540157754550 ) ) ;
#30380=CARTESIAN_POINT ( 'NONE',  ( 155.4216552449402684, 261.4487918497463284, 18.51722274565528892 ) ) ;
#30381=CARTESIAN_POINT ( 'NONE',  ( 79.84079962965540744, 210.2365022471901739, -10.00000000000009237 ) ) ;
#30383=AXIS2_PLACEMENT_3D ( 'NONE', #45983, #76430, #76899 ) ;
#30384=CARTESIAN_POINT ( 'NONE',  ( 161.9818314276490128, 250.0862333946917602, -13.01265917937909045 ) ) ;
#30385=VERTEX_POINT ( 'NONE', #52844 ) ;
#30388=CARTESIAN_POINT ( 'NONE',  ( 164.4261001824251878, 245.8526357240660900, 1.583002802772015549 ) ) ;
#30389=CARTESIAN_POINT ( 'NONE',  ( 161.7518432240285620, 284.4801498230883112, 0.5359932121324623155 ) ) ;
#30390=CARTESIAN_POINT ( 'NONE',  ( 198.9721957120447655, 281.0613474150461570, 17.36564602955951386 ) ) ;
#30394=CARTESIAN_POINT ( 'NONE',  ( 156.8463053224485009, 274.3823876006896398, 13.73651536856081989 ) ) ;
#30396=CARTESIAN_POINT ( 'NONE',  ( 153.2283961777204695, 265.2476279883323400, -17.66880461074566000 ) ) ;
#30400=CARTESIAN_POINT ( 'NONE',  ( 197.5221644013859645, 266.2761734353669567, 4.458159567591970962 ) ) ;
#30401=CARTESIAN_POINT ( 'NONE',  ( 148.3745023213073750, 276.3025496145838815, -3.856079141225808637 ) ) ;
#30403=CIRCLE ( 'NONE', #25573, 17.82106496071138224 ) ;
#30404=CARTESIAN_POINT ( 'NONE',  ( 184.5990297707867001, 263.7127329470384325, -12.27809941363454271 ) ) ;
#30406=CARTESIAN_POINT ( 'NONE',  ( 198.3987358442466586, 266.1842203803777238, 0.8103656318469341091 ) ) ;
#30408=ORIENTED_EDGE ( 'NONE', *, *, #69967, .F. ) ;
#30409=CARTESIAN_POINT ( 'NONE',  ( 190.8907028847385448, 300.0145992415348815, -5.421341690443150618 ) ) ;
#30410=CARTESIAN_POINT ( 'NONE',  ( 186.4922146040686357, 282.5459359838986302, 16.18330935361411349 ) ) ;
#30412=AXIS2_PLACEMENT_3D ( 'NONE', #59502, #98546, #22015 ) ;
#30413=CARTESIAN_POINT ( 'NONE',  ( 164.2723164851102808, 246.1189969011916503, -1.993789335506892302 ) ) ;
#30414=CARTESIAN_POINT ( 'NONE',  ( 193.9844289374573520, 294.6561085335266625, 15.49818881749970245 ) ) ;
#30415=CARTESIAN_POINT ( 'NONE',  ( 192.8080529993486039, 268.3314956550081547, 12.47957376853008959 ) ) ;
#30417=CARTESIAN_POINT ( 'NONE',  ( 21.07736754015083491, 189.6427522451419350, -10.00000000000009592 ) ) ;
#30418=CARTESIAN_POINT ( 'NONE',  ( 165.4384176284148964, 285.1150933481030165, -3.137621857651547330 ) ) ;
#30420=CARTESIAN_POINT ( 'NONE',  ( 198.6742831389107096, 286.5330427765190393, 17.60232614297041565 ) ) ;
#30422=CARTESIAN_POINT ( 'NONE',  ( -10.27112140336314994, 171.0024278399161233, -9.188101187500093303 ) ) ;
#30423=CARTESIAN_POINT ( 'NONE',  ( 78.30721297357251842, 216.0177522451418497, -10.00000000000009592 ) ) ;
#30427=CARTESIAN_POINT ( 'NONE',  ( -22.42236680055709641, 157.8615022471902591, 0.000000000000000000 ) ) ;
#30428=CARTESIAN_POINT ( 'NONE',  ( 6.913983429043053519, 183.9869531367911009, 4.594050593750046652 ) ) ;
#30431=CARTESIAN_POINT ( 'NONE',  ( 204.9463377925012253, 275.6695254486514841, -14.15865086131798378 ) ) ;
#30433=B_SPLINE_SURFACE_WITH_KNOTS ( 'NONE', 3, 1, ( 
 ( #95485, #81264 ),
 ( #35109, #66019 ),
 ( #41202, #2745 ),
 ( #18439, #96968 ),
 ( #27534, #89378 ),
 ( #33634, #48327 ),
 ( #40707, #17940 ),
 ( #26038, #79273 ),
 ( #56908, #87894 ),
 ( #51296, #68005 ),
 ( #98929, #29024 ),
 ( #82268, #37100 ),
 ( #52300, #83238 ),
 ( #75131, #67000 ),
 ( #97927, #81756 ),
 ( #59895, #28502 ),
 ( #19933, #68497 ),
 ( #12841, #90863 ),
 ( #6205, #74138 ),
 ( #35614, #20430 ),
 ( #75617, #90359 ),
 ( #89855, #21415 ),
 ( #43701, #60880 ),
 ( #20940, #99421 ),
 ( #58886, #28009 ),
 ( #83746, #13806 ),
 ( #29998, #36099 ),
 ( #74644, #4731 ),
 ( #29507, #60384 ),
 ( #5219, #14309 ),
 ( #91340, #21900 ),
 ( #45195, #44685 ),
 ( #5706, #98433 ),
 ( #51821, #36597 ) ),
 .UNSPECIFIED., .T., .F., .F.,
 ( 4, 2, 2, 2, 2, 2, 2, 2, 2, 2, 2, 2, 2, 2, 2, 2, 4 ),
 ( 2, 2 ),
 ( 0.000000000000000000, 0.06250000000000000000, 0.1250000000000000000, 0.1875000000000000000, 0.2500000000000000000, 0.3125000000000000000, 0.3750000000000000000, 0.4375000000000000000, 0.5000000000000000000, 0.5625000000000000000, 0.6250000000000000000, 0.6875000000000000000, 0.7500000000000000000, 0.8125000000000000000, 0.8750000000000000000, 0.9375000000000000000, 1.000000000000000000 ),
 ( 0.000000000000000000, 1.000000000000000000 ),
 .UNSPECIFIED. ) ;
#30434=CARTESIAN_POINT ( 'NONE',  ( 175.8155514549374914, 252.9580239610218371, -3.267414397889120359 ) ) ;
#30435=CARTESIAN_POINT ( 'NONE',  ( 190.6298455067565101, 261.9054759779421602, -0.7664710513680175197 ) ) ;
#30436=CARTESIAN_POINT ( 'NONE',  ( 183.0585217367469681, 295.7022925660351689, 1.036231964973731490 ) ) ;
#30437=CARTESIAN_POINT ( 'NONE',  ( 72.04657099559547362, 205.7365022471902023, -10.00000000000009059 ) ) ;
#30440=CARTESIAN_POINT ( 'NONE',  ( 147.6618183892331331, 274.8892235422768522, 8.990680574201936892 ) ) ;
#30441=CARTESIAN_POINT ( 'NONE',  ( 36.52174756457106497, 182.7048013555409796, 4.594050593750051981 ) ) ;
#30446=CARTESIAN_POINT ( 'NONE',  ( 151.1811967613751335, 268.7934813906678642, -15.79361349403328418 ) ) ;
#30447=CARTESIAN_POINT ( 'NONE',  ( 207.6918009085542849, 270.9142438413412037, 7.009114282139513818 ) ) ;
#30448=CARTESIAN_POINT ( 'NONE',  ( 188.8867764286892452, 268.2031459771304753, 13.62204560104310502 ) ) ;
#30449=CARTESIAN_POINT ( 'NONE',  ( 159.9437897750486570, 278.5723957854588662, -9.797752282130973711 ) ) ;
#30450=CARTESIAN_POINT ( 'NONE',  ( 179.9845513519039741, 262.5466105634188239, -14.24360566215998958 ) ) ;
#30453=CARTESIAN_POINT ( 'NONE',  ( 190.6084209867335915, 300.5035258309363826, -0.5505750481748228342 ) ) ;
#30456=CARTESIAN_POINT ( 'NONE',  ( 155.1376601545389917, 261.9406857754215707, 18.55063430030667959 ) ) ;
#30458=FACE_OUTER_BOUND ( 'NONE', #34610, .T. ) ;
#30460=CARTESIAN_POINT ( 'NONE',  ( 148.5405002604136939, 273.7531191599721865, -8.243767320729981307 ) ) ;
#30462=ORIENTED_EDGE ( 'NONE', *, *, #82998, .F. ) ;
#30466=CARTESIAN_POINT ( 'NONE',  ( 180.6905943096166993, 256.8005298396895455, -7.802981789431568060 ) ) ;
#30467=VERTEX_POINT ( 'NONE', #98480 ) ;
#30468=VERTEX_POINT ( 'NONE', #35159 ) ;
#30469=CARTESIAN_POINT ( 'NONE',  ( 202.4652556304803852, 279.1494446843323658, 15.55728013657999398 ) ) ;
#30471=ORIENTED_EDGE ( 'NONE', *, *, #23587, .F. ) ;
#30472=CARTESIAN_POINT ( 'NONE',  ( 150.8359915840788688, 269.3913942967808453, 15.73449616766854575 ) ) ;
#30478=EDGE_CURVE ( 'NONE', #82087, #16991, #41326, .T. ) ;
#30479=CARTESIAN_POINT ( 'NONE',  ( 147.7870527676176948, 274.6723112360602386, 9.257357958194809555 ) ) ;
#30480=VECTOR ( 'NONE', #60708, 1000.000000000000000 ) ;
#30482=ORIENTED_EDGE ( 'NONE', *, *, #99485, .T. ) ;
#30483=CARTESIAN_POINT ( 'NONE',  ( 195.9713281756800427, 291.2146981034049418, 17.52210387885178022 ) ) ;
#30485=CARTESIAN_POINT ( 'NONE',  ( 158.1038083475960718, 265.1254946056319000, 17.35475346825555931 ) ) ;
#30487=CARTESIAN_POINT ( 'NONE',  ( 148.9232972370683399, 272.7042780851529642, 12.27045554427055940 ) ) ;
#30492=CARTESIAN_POINT ( 'NONE',  ( 190.8264243556038195, 300.1259329198319961, 8.466983560044813117 ) ) ;
#30497=AXIS2_PLACEMENT_3D ( 'NONE', #32501, #40574, #63392 ) ;
#30499=CARTESIAN_POINT ( 'NONE',  ( 147.1199024702499969, 275.8278494473859723, 5.224467159276165340 ) ) ;
#30500=FACE_OUTER_BOUND ( 'NONE', #36710, .T. ) ;
#30501=CARTESIAN_POINT ( 'NONE',  ( 190.1519139143167081, 301.2942192743771557, 4.481136594690903863 ) ) ;
#30503=CARTESIAN_POINT ( 'NONE',  ( 146.6045776406848802, 276.7204182345944901, 0.5293868638167662510 ) ) ;
#30504=CARTESIAN_POINT ( 'NONE',  ( 146.9235493515124062, 276.1679430252639804, 0.7994986043261682607 ) ) ;
#30505=CARTESIAN_POINT ( 'NONE',  ( 162.5659316022686482, 257.3233763081025813, 15.61851065589861243 ) ) ;
#30509=CARTESIAN_POINT ( 'NONE',  ( 170.0120225124279330, 288.8437964431653313, 4.419511376178223649 ) ) ;
#30511=VERTEX_POINT ( 'NONE', #48116 ) ;
#30512=CARTESIAN_POINT ( 'NONE',  ( 190.7355618834574500, 300.2833113380910959, -3.494153871398564259 ) ) ;
#30515=EDGE_CURVE ( 'NONE', #93599, #81863, #86079, .T. ) ;
#30516=LINE ( 'NONE', #61405, #14013 ) ;
#30518=CARTESIAN_POINT ( 'NONE',  ( 40.72531889205820477, 200.9865022471903160, -10.00000000000009592 ) ) ;
#30521=VERTEX_POINT ( 'NONE', #79568 ) ;
#30522=CARTESIAN_POINT ( 'NONE',  ( 163.4218292706009095, 247.5920839679097014, -10.44611490715852042 ) ) ;
#30523=EDGE_CURVE ( 'NONE', #28922, #58170, #37732, .T. ) ;
#30524=CARTESIAN_POINT ( 'NONE',  ( 206.2041691044954348, 273.4908977089264113, -9.455375957961031474 ) ) ;
#30526=CARTESIAN_POINT ( 'NONE',  ( 45.83126033165607538, 197.2677522451418781, 10.00000000000009592 ) ) ;
#30527=CARTESIAN_POINT ( 'NONE',  ( 127.8874276638293850, 235.4548013555409796, -4.594050593750042211 ) ) ;
#30528=B_SPLINE_CURVE_WITH_KNOTS ( 'NONE', 3,
 ( #73171, #80292, #11864, #74669, #26560, #89405, #97468, #73658, #43224, #34158, #34642, #65541, #96488, #88922, #4236, #19482, #28035, #51329, #74166, #96994, #4757, #35136, #82296, #18972, #66541, #28528, #66047, #49847, #12866, #67028, #36125, #27564, #43726, #5246, #97955, #18464, #10863, #41737, #80806, #135, #53320, #68526, #52817, #84277, #61416, #98458, #6230, #46203, #52326, #77120, #38103, #90890 ),
 .UNSPECIFIED., .F., .F.,
 ( 4, 2, 2, 2, 2, 2, 2, 2, 2, 2, 2, 2, 2, 2, 2, 2, 2, 2, 2, 2, 2, 2, 2, 2, 2, 4 ),
 ( 0.0006745074493109526727, 0.0008837329331894130339, 0.001092958417067873503, 0.001197571159007103630, 0.001302183900946333756, 0.001406796642885563883, 0.001511409384824794009, 0.001929860352581865435, 0.002348311320338936862, 0.003185213255853080582, 0.004022115191367223869, 0.004859017126881367589, 0.005277468094638439015, 0.005486693578516984270, 0.005591306320456222202, 0.005643612691425760504, 0.005695919062395299673, 0.005748225433364837975, 0.005800531804334376276, 0.005905144546273446808, 0.006114370030151567922, 0.006323595514029689904, 0.006532820997907811018, 0.006742046481785933000, 0.006951271965664054114, 0.007369722933420295476 ),
 .UNSPECIFIED. ) ;
#30529=CARTESIAN_POINT ( 'NONE',  ( 199.2299651681423143, 285.5705732690366858, -17.65328173313980642 ) ) ;
#30532=CARTESIAN_POINT ( 'NONE',  ( 157.7529601300917363, 257.4108533407307959, 16.91445305439664892 ) ) ;
#30533=CARTESIAN_POINT ( 'NONE',  ( 175.4516086236820342, 253.5594085358976884, -4.077166357663031704 ) ) ;
#30534=CARTESIAN_POINT ( 'NONE',  ( 41.74435586355720318, 207.1589784336661637, -6.496448406907675876E-16 ) ) ;
#30535=CARTESIAN_POINT ( 'NONE',  ( 27.19136022205111658, 198.0530062829863311, -4.648177544792955347E-16 ) ) ;
#30543=CARTESIAN_POINT ( 'NONE',  ( 15.66239703771868719, 191.3967562850346837, -4.648177544792955347E-16 ) ) ;
#30544=CARTESIAN_POINT ( 'NONE',  ( 190.9498149295421570, 299.9122141765958531, -5.138500224925297566 ) ) ;
#30545=PLANE ( 'NONE',  #59572 ) ;
#30547=CARTESIAN_POINT ( 'NONE',  ( 164.8398358111874415, 250.3986661409049361, 10.19718004758793484 ) ) ;
#30548=B_SPLINE_CURVE_WITH_KNOTS ( 'NONE', 3,
 ( #50937, #74771, #90985, #44820, #98058, #98566, #51438, #82405, #5349, #81886, #36230, #4865, #67136, #66641, #28635, #29638, #97571, #91467, #59518, #51946, #82886, #44326, #75258, #36727, #67633, #29150, #60021, #52927, #83879, #75755, #21546, #52428, #41456, #83375, #4347, #97095, #13940, #6341, #35243, #66149, #27663, #24021, #8331, #38715, #69621, #38203, #54399, #91982 ),
 .UNSPECIFIED., .F., .F.,
 ( 4, 2, 2, 2, 2, 2, 2, 2, 2, 2, 2, 2, 2, 2, 2, 2, 2, 2, 2, 2, 2, 2, 2, 4 ),
 ( 0.0006698723108304612634, 0.001653363054844869239, 0.001899235740848491481, 0.002145108426852113722, 0.002268044769853887546, 0.002390981112855661370, 0.002513917455857435628, 0.002636853798859209452, 0.002882726484862757534, 0.003128599170866305616, 0.003620344542873517139, 0.004603835286888004370, 0.005587326030902491601, 0.006079071402909690981, 0.006570816774916890361, 0.006693753117918673293, 0.006755221289419565192, 0.006816689460920456224, 0.006939625803922164562, 0.007062562146923872033, 0.007308434832927166412, 0.007554307518930460791, 0.008046052890937049548, 0.008537798262943638306 ),
 .UNSPECIFIED. ) ;
#30549=CARTESIAN_POINT ( 'NONE',  ( 118.5773942495489592, 229.2677522451417929, -5.000000000000041744 ) ) ;
#30551=CARTESIAN_POINT ( 'NONE',  ( 194.6550018378799507, 292.9242970792882943, -14.88548128926688463 ) ) ;
#30554=CARTESIAN_POINT ( 'NONE',  ( 203.0507839702407580, 278.9527209772879814, 16.21318481136342626 ) ) ;
#30557=CARTESIAN_POINT ( 'NONE',  ( 26.48065812185646806, 198.3464784336661637, 1.353441290958777327E-15 ) ) ;
#30561=CARTESIAN_POINT ( 'NONE',  ( 179.4408063581041688, 277.4340371255875652, 17.62723233342114071 ) ) ;
#30562=CARTESIAN_POINT ( 'NONE',  ( 194.9775624055715468, 275.3010545703284038, -15.63051501613322003 ) ) ;
#30563=CARTESIAN_POINT ( 'NONE',  ( 71.05451054047556170, 202.6423013555409796, -4.594050593750043987 ) ) ;
#30567=ORIENTED_EDGE ( 'NONE', *, *, #86359, .F. ) ;
#30570=CARTESIAN_POINT ( 'NONE',  ( 13.51768745649711789, 178.6115022471902591, 10.00000000000009592 ) ) ;
#30571=CARTESIAN_POINT ( 'NONE',  ( 208.1415148974628266, 270.1353163636768500, 3.453641150550738725 ) ) ;
#30572=CARTESIAN_POINT ( 'NONE',  ( 135.5998589986957086, 261.3464784336661637, 1.353441290958777327E-15 ) ) ;
#30576=CARTESIAN_POINT ( 'NONE',  ( 189.4731981977795101, 299.9930995634677515, 4.873517838202077179 ) ) ;
#30580=CARTESIAN_POINT ( 'NONE',  ( 183.2347291344400730, 286.2791671247540535, 15.72992646725049326 ) ) ;
#30582=CARTESIAN_POINT ( 'NONE',  ( 156.6575251390178209, 280.1398687009162245, -5.349388280191599954 ) ) ;
#30585=ORIENTED_EDGE ( 'NONE', *, *, #60881, .F. ) ;
#30586=CARTESIAN_POINT ( 'NONE',  ( 206.5536402976238151, 272.8855958466460265, 8.283930970375774194 ) ) ;
#30587=ADVANCED_FACE ( 'NONE', ( #6755 ), #53659, .F. ) ;
#30593=CARTESIAN_POINT ( 'NONE',  ( 149.8172510487983402, 272.9568577616375364, 11.41474127177868425 ) ) ;
#30594=CARTESIAN_POINT ( 'NONE',  ( 163.4055107321044318, 247.6203485056908846, -10.24153090796238530 ) ) ;
#30595=CARTESIAN_POINT ( 'NONE',  ( 201.3053499423511425, 281.9759013948520874, -16.75960365258566398 ) ) ;
#30597=CARTESIAN_POINT ( 'NONE',  ( 191.8019569549158518, 281.4351414054034990, 16.70232326611636964 ) ) ;
#30600=CARTESIAN_POINT ( 'NONE',  ( 148.9694607950094394, 272.6243204573405592, 11.81236034532910573 ) ) ;
#30606=CARTESIAN_POINT ( 'NONE',  ( 167.4011299790239775, 281.5488363183706042, 12.98604958840868662 ) ) ;
#30611=CARTESIAN_POINT ( 'NONE',  ( 103.7198194655286017, 224.5643266524159856, -9.188101187500093303 ) ) ;
#30612=FACE_OUTER_BOUND ( 'NONE', #66835, .T. ) ;
#30614=CARTESIAN_POINT ( 'NONE',  ( 151.0778907302193943, 268.9724126853576536, 15.84769371787143832 ) ) ;
#30615=CARTESIAN_POINT ( 'NONE',  ( 136.7639277290221571, 249.7677522451418497, 10.00000000000009592 ) ) ;
#30616=ORIENTED_EDGE ( 'NONE', *, *, #50036, .T. ) ;
#30618=VERTEX_POINT ( 'NONE', #23683 ) ;
#30620=ORIENTED_EDGE ( 'NONE', *, *, #72159, .T. ) ;
#30626=CARTESIAN_POINT ( 'NONE',  ( 163.7587049410067266, 247.0085981909329576, -6.137518685179130351 ) ) ;
#30627=CARTESIAN_POINT ( 'NONE',  ( 195.7944228926560868, 283.4259135625417798, 17.81926924524233868 ) ) ;
#30628=CARTESIAN_POINT ( 'NONE',  ( 170.9271208801252158, 283.6173671677598236, 12.30198536427989353 ) ) ;
#30629=CARTESIAN_POINT ( 'NONE',  ( 147.8163551302855296, 274.6215580551378821, -9.286329195885331345 ) ) ;
#30632=CARTESIAN_POINT ( 'NONE',  ( 166.6760794757555288, 247.0815379807098964, 1.916300026573462878 ) ) ;
#30634=DIRECTION ( 'NONE',  ( 0.4999999999999998890, -0.8660254037844385966, 0.000000000000000000 ) ) ;
#30638=ORIENTED_EDGE ( 'NONE', *, *, #40866, .T. ) ;
#30639=EDGE_CURVE ( 'NONE', #76828, #39058, #78866, .T. ) ;
#30640=CARTESIAN_POINT ( 'NONE',  ( -27.42236680055714260, 166.5217562850347406, 1.224646799147364892E-15 ) ) ;
#30641=CARTESIAN_POINT ( 'NONE',  ( 186.9301476837522671, 260.0195029309103916, 2.866143204992003479 ) ) ;
#30644=CARTESIAN_POINT ( 'NONE',  ( 200.5810378487751393, 283.2304467414622877, 18.38516374632547112 ) ) ;
#30645=CARTESIAN_POINT ( 'NONE',  ( 157.9878497072205050, 281.0327258848784595, 1.976071138188537635 ) ) ;
#30647=( BOUNDED_CURVE ( )  B_SPLINE_CURVE ( 2, ( #46572, #70385, #40473, #9610, #79021, #93221, #94228, #71405, #32881 ),
 .UNSPECIFIED., .F., .F. ) 
 B_SPLINE_CURVE_WITH_KNOTS ( ( 3, 2, 2, 2, 3 ),
 ( 0.7298387096774193727, 0.7311827956989247479, 0.7338709677419354982, 0.7365591397849462485, 0.7379032258064516236 ),
 .UNSPECIFIED. ) 
 CURVE ( )  GEOMETRIC_REPRESENTATION_ITEM ( )  RATIONAL_B_SPLINE_CURVE ( ( 0.9330127018922194093, 0.9330127018922194093, 1.000000000000000000, 0.8660254037844387076, 1.000000000000000000, 0.8660254037844387076, 1.000000000000000000, 0.9330127018922194093, 0.9330127018922194093 ) ) 
 REPRESENTATION_ITEM ( '' )  );
#30649=CARTESIAN_POINT ( 'NONE',  ( 155.3605053979525223, 261.5547064916044064, -18.59460972482254704 ) ) ;
#30650=EDGE_CURVE ( 'NONE', #69000, #74125, #87542, .T. ) ;
#30653=CARTESIAN_POINT ( 'NONE',  ( 6.860117161356328097, 174.7677522451418781, 10.00000000000009592 ) ) ;
#30654=CARTESIAN_POINT ( 'NONE',  ( 192.8656348049960059, 266.9067490818276269, -11.31435781342206504 ) ) ;
#30657=CARTESIAN_POINT ( 'NONE',  ( 169.0081789574249456, 280.3483017457910478, -14.43549772046353574 ) ) ;
#30659=CARTESIAN_POINT ( 'NONE',  ( -12.81524457486244550, 175.6589784336661353, -6.496448406907675876E-16 ) ) ;
#30662=CARTESIAN_POINT ( 'NONE',  ( 187.2498241109438197, 296.0094539997018046, 8.138855039951142345 ) ) ;
#30664=EDGE_CURVE ( 'NONE', #81112, #18408, #23817, .T. ) ;
#30669=CARTESIAN_POINT ( 'NONE',  ( -17.42236680055705023, 149.2012482093457777, 0.000000000000000000 ) ) ;
#30670=FACE_OUTER_BOUND ( 'NONE', #51180, .T. ) ;
#30672=CARTESIAN_POINT ( 'NONE',  ( 167.1443788062580609, 247.6230354218334924, 5.209738392609174262 ) ) ;
#30673=CARTESIAN_POINT ( 'NONE',  ( 21.28450569914983248, 195.3464784336661637, 1.353441290958777525E-15 ) ) ;
#30674=CARTESIAN_POINT ( 'NONE',  ( 117.5758788303146076, 244.8149278399160664, 9.188101187500093303 ) ) ;
#30675=CARTESIAN_POINT ( 'NONE',  ( 180.0968189326222557, 292.5754757235382613, -6.169244772567886947 ) ) ;
#30676=CARTESIAN_POINT ( 'NONE',  ( 183.0802513414319606, 257.7480130289799831, -2.340672193140110657 ) ) ;
#30677=CARTESIAN_POINT ( 'NONE',  ( 153.3843775842402124, 274.2552327709109932, -12.20347941078255616 ) ) ;
#30678=CARTESIAN_POINT ( 'NONE',  ( 178.2729695640300349, 283.8809743909798158, -15.09020537081628888 ) ) ;
#30679=CARTESIAN_POINT ( 'NONE',  ( 189.7838259857693686, 299.9317662682615833, -5.554424272425116271 ) ) ;
#30680=CARTESIAN_POINT ( 'NONE',  ( 195.8627871995700502, 291.4026965887302936, 17.41145040657729481 ) ) ;
#30681=CARTESIAN_POINT ( 'NONE',  ( 194.2321518193436987, 294.2270399159019121, 13.98132384850917020 ) ) ;
#30682=CARTESIAN_POINT ( 'NONE',  ( 207.8570869662935365, 270.6279599915536664, -5.669188455878507504 ) ) ;
#30684=CARTESIAN_POINT ( 'NONE',  ( 193.0673599610802569, 264.3079050832715211, 7.416874666535670180 ) ) ;
#30685=CARTESIAN_POINT ( 'NONE',  ( 171.4993218643381852, 279.8819833531975974, 13.90609482443614908 ) ) ;
#30689=CARTESIAN_POINT ( 'NONE',  ( 180.8455629192530125, 266.6468860283634967, -14.68397486445532252 ) ) ;
#30692=CARTESIAN_POINT ( 'NONE',  ( 185.1323751026578464, 269.6436051631800979, 15.74023217557582477 ) ) ;
#30693=CARTESIAN_POINT ( 'NONE',  ( 90.89164462408909628, 223.2833772461660260, -9.188101187500095079 ) ) ;
#30698=FACE_OUTER_BOUND ( 'NONE', #27391, .T. ) ;
#30699=CARTESIAN_POINT ( 'NONE',  ( 192.0737711319585230, 277.0892155713485181, 17.32299324414631414 ) ) ;
#30700=CARTESIAN_POINT ( 'NONE',  ( 201.2026048815914692, 270.3487196048755550, -10.12796269912754710 ) ) ;
#30701=CARTESIAN_POINT ( 'NONE',  ( 190.6420043223797620, 261.1713590208896107, -4.660055732604916123 ) ) ;
#30703=CARTESIAN_POINT ( 'NONE',  ( 52.48883062679684741, 201.1115022471902591, 10.00000000000009592 ) ) ;
#30704=CARTESIAN_POINT ( 'NONE',  ( 192.4335622838504207, 297.3422883733380786, -12.83044365323471325 ) ) ;
#30709=CARTESIAN_POINT ( 'NONE',  ( 199.8990292968633469, 270.1221403762914406, 9.242915985417027969 ) ) ;
#30710=CARTESIAN_POINT ( 'NONE',  ( 196.5475899070771675, 290.2165835061676944, -17.89382743182097002 ) ) ;
#30711=EDGE_LOOP ( 'NONE', ( #54037, #2720, #79310, #55627 ) ) ;
#30713=CARTESIAN_POINT ( 'NONE',  ( 175.1271263694729328, 272.4273639404348728, 17.81557788710851042 ) ) ;
#30714=CARTESIAN_POINT ( 'NONE',  ( 180.0421887822893439, 262.9451233745447780, -12.84000619916867159 ) ) ;
#30715=CARTESIAN_POINT ( 'NONE',  ( 173.0587134762232324, 253.8503347386293854, -9.001391358779716967 ) ) ;
#30717=CARTESIAN_POINT ( 'NONE',  ( 152.6992418905140028, 266.1641500988167763, 17.27767170937316621 ) ) ;
#30718=ORIENTED_EDGE ( 'NONE', *, *, #75807, .T. ) ;
#30719=CARTESIAN_POINT ( 'NONE',  ( 187.1956594725295417, 278.7701613363302044, 17.25881440492993590 ) ) ;
#30724=B_SPLINE_CURVE_WITH_KNOTS ( 'NONE', 3,
 ( #99289, #97800, #15149, #60743 ),
 .UNSPECIFIED., .F., .F.,
 ( 4, 4 ),
 ( 0.006074498585399344674, 0.01174373323087292767 ),
 .UNSPECIFIED. ) ;
#30726=ADVANCED_FACE ( 'NONE', ( #51489 ), #60070, .T. ) ;
#30728=CARTESIAN_POINT ( 'NONE',  ( 159.0141149511101446, 255.2264691145165330, 17.40381185983830292 ) ) ;
#30729=CARTESIAN_POINT ( 'NONE',  ( 190.6321288753560736, 278.4426617264936112, -16.55712034464263027 ) ) ;
#30730=CARTESIAN_POINT ( 'NONE',  ( 192.6535100158423290, 296.9613277265186184, -13.39826475700667174 ) ) ;
#30733=CARTESIAN_POINT ( 'NONE',  ( 115.9793180381956148, 237.7677522451418497, 10.00000000000009592 ) ) ;
#30738=FACE_OUTER_BOUND ( 'NONE', #92338, .T. ) ;
#30742=CARTESIAN_POINT ( 'NONE',  ( 172.7634016531041539, 271.0112792648602635, 16.42974606472167665 ) ) ;
#30744=ORIENTED_EDGE ( 'NONE', *, *, #29335, .F. ) ;
#30745=CARTESIAN_POINT ( 'NONE',  ( 154.9032082715209810, 280.6326124547101699, -2.389722542998433230 ) ) ;
#30747=CARTESIAN_POINT ( 'NONE',  ( 206.6093111437328957, 272.7891711126852101, -9.934261249647553527 ) ) ;
#30748=CARTESIAN_POINT ( 'NONE',  ( 148.1846401255833996, 275.9836697316168284, -5.368268268079755323 ) ) ;
#30751=CARTESIAN_POINT ( 'NONE',  ( 178.6782777294722848, 260.6412425082613709, 13.57969907341511551 ) ) ;
#30753=CARTESIAN_POINT ( 'NONE',  ( 186.7621306400879462, 287.1057732871925623, -15.90520287716750225 ) ) ;
#30754=CARTESIAN_POINT ( 'NONE',  ( 103.0428032491157779, 239.4869531367911293, 4.594050593750046652 ) ) ;
#30756=CARTESIAN_POINT ( 'NONE',  ( 186.7511758073848682, 262.6631644945539392, -10.04217688415225496 ) ) ;
#30758=CARTESIAN_POINT ( 'NONE',  ( 188.0217479200190382, 273.7640949189246840, 16.90097692181329236 ) ) ;
#30763=CARTESIAN_POINT ( 'NONE',  ( 192.7699314614395689, 296.7596798676532899, 11.34673828722139177 ) ) ;
#30766=CARTESIAN_POINT ( 'NONE',  ( 88.86189758574322184, 232.1115022471902876, -5.000000000000047962 ) ) ;
#30768=CARTESIAN_POINT ( 'NONE',  ( 148.0737445431542767, 274.1757465147189237, 10.26368672933362980 ) ) ;
#30770=CARTESIAN_POINT ( 'NONE',  ( 194.9757425430702824, 292.9391030023704161, -15.21392314336593365 ) ) ;
#30772=ORIENTED_EDGE ( 'NONE', *, *, #61047, .T. ) ;
#30773=CARTESIAN_POINT ( 'NONE',  ( 188.1032490429140580, 266.2180392766005639, -11.82133915774577559 ) ) ;
#30775=CARTESIAN_POINT ( 'NONE',  ( 190.7104275908211264, 284.0216516728820011, -16.91638317915403533 ) ) ;
#30776=CARTESIAN_POINT ( 'NONE',  ( 193.0146740725342056, 262.6358330379304107, 4.705848471798295130 ) ) ;
#30777=CARTESIAN_POINT ( 'NONE',  ( 158.4506253844079708, 263.4166843688063295, 17.67374169831186848 ) ) ;
#30778=CARTESIAN_POINT ( 'NONE',  ( 204.6053525328498779, 273.0989532408518130, -10.15815190134183332 ) ) ;
#30779=CARTESIAN_POINT ( 'NONE',  ( 184.3757908040668099, 288.5642296694110769, -13.61842078453970295 ) ) ;
#30780=CARTESIAN_POINT ( 'NONE',  ( 160.8008004585890376, 281.5710333326640580, 5.628202240593611627 ) ) ;
#30781=CARTESIAN_POINT ( 'NONE',  ( 153.2583947049096764, 265.1956690150883560, -17.64103123457563882 ) ) ;
#30782=ORIENTED_EDGE ( 'NONE', *, *, #94225, .T. ) ;
#30783=CARTESIAN_POINT ( 'NONE',  ( 204.7259617510281942, 272.8945987308273970, -9.650000825374167590 ) ) ;
#30785=CARTESIAN_POINT ( 'NONE',  ( 163.7898901466472523, 247.5855377128527834, -7.511645082746166047 ) ) ;
#30786=EDGE_CURVE ( 'NONE', #69106, #40327, #64084, .T. ) ;
#30787=CARTESIAN_POINT ( 'NONE',  ( 141.9699493749754140, 259.7505386000626686, -7.968025677899344572 ) ) ;
#30788=CARTESIAN_POINT ( 'NONE',  ( 189.0756608774803453, 270.0634534580582908, -14.06871611248690890 ) ) ;
#30789=CARTESIAN_POINT ( 'NONE',  ( 185.1141009223508149, 296.8708822037961568, -4.333820615423671363 ) ) ;
#30791=CARTESIAN_POINT ( 'NONE',  ( 28.07773955407504118, 197.0177522451419350, 5.000000000000046185 ) ) ;
#30793=CARTESIAN_POINT ( 'NONE',  ( 191.4411680433141214, 282.7668619920169135, -17.27576285388926536 ) ) ;
#30795=CARTESIAN_POINT ( 'NONE',  ( 76.27746593522670082, 214.8458772461660544, 9.188101187500095079 ) ) ;
#30797=CARTESIAN_POINT ( 'NONE',  ( 147.4271219180435253, 275.2957297547342819, -3.800519706258907782 ) ) ;
#30798=CARTESIAN_POINT ( 'NONE',  ( 207.9743173328493526, 270.4249110404894054, -2.481515874287090639 ) ) ;
#30800=CARTESIAN_POINT ( 'NONE',  ( 207.8431546909062320, 270.6520914003897360, -6.441273666418043220 ) ) ;
#30802=CARTESIAN_POINT ( 'NONE',  ( 48.88270317314112390, 187.4824982072973967, 3.021315404115420679E-15 ) ) ;
#30805=CARTESIAN_POINT ( 'NONE',  ( 165.9714824136468394, 249.3895961940136488, -9.198834327378280662 ) ) ;
#30806=CARTESIAN_POINT ( 'NONE',  ( 163.9665205130568495, 246.6486510615381178, -4.977134839185944237 ) ) ;
#30807=CARTESIAN_POINT ( 'NONE',  ( 157.8562613713738472, 257.2319303423452652, 17.81420683562559404 ) ) ;
#30808=DIRECTION ( 'NONE',  ( -0.8660254037844387076, -0.4999999999999998890, -0.000000000000000000 ) ) ;
#30811=CARTESIAN_POINT ( 'NONE',  ( 50.62146334811270521, 200.0333772461660544, 9.188101187500095079 ) ) ;
#30812=CARTESIAN_POINT ( 'NONE',  ( 164.3815567799200039, 246.8702290586211632, -5.719362487965026887 ) ) ;
#30815=CARTESIAN_POINT ( 'NONE',  ( -14.62813816649718213, 172.3615022471903160, 5.000000000000046185 ) ) ;
#30817=CARTESIAN_POINT ( 'NONE',  ( 196.6129024267879402, 268.7927177136375576, -10.56481122998096289 ) ) ;
#30819=CARTESIAN_POINT ( 'NONE',  ( 150.7691137448031213, 269.5072301123068428, -15.63821625702598084 ) ) ;
#30820=CARTESIAN_POINT ( 'NONE',  ( 196.5475899070771675, 290.2165835061676944, -17.89382743182097002 ) ) ;
#30822=CARTESIAN_POINT ( 'NONE',  ( 60.95981515367195414, 199.8768266524160140, 9.188101187500096856 ) ) ;
#30825=CARTESIAN_POINT ( 'NONE',  ( 198.2819808855875863, 287.2125302111982705, 18.53535247371401695 ) ) ;
#30826=FACE_OUTER_BOUND ( 'NONE', #2107, .T. ) ;
#30828=CARTESIAN_POINT ( 'NONE',  ( 99.68721513304873838, 238.3615022471903160, 5.000000000000046185 ) ) ;
#30829=CARTESIAN_POINT ( 'NONE',  ( 161.5875797534026219, 250.7690973254556468, 12.95526170413129030 ) ) ;
#30830=CARTESIAN_POINT ( 'NONE',  ( 165.0509870607838252, 244.7702999017660375, -2.356357909806504392 ) ) ;
#30831=VERTEX_POINT ( 'NONE', #22086 ) ;
#30833=CARTESIAN_POINT ( 'NONE',  ( 202.8371121491529152, 271.7102578477088173, 10.98807562330369869 ) ) ;
#30835=CARTESIAN_POINT ( 'NONE',  ( 159.9531724557437826, 253.5999738052623229, -15.71074128491364874 ) ) ;
#30836=CARTESIAN_POINT ( 'NONE',  ( 187.5118225138183163, 276.9259439731086445, -17.64892817816586756 ) ) ;
#30841=CARTESIAN_POINT ( 'NONE',  ( 207.6900289502458179, 270.9173129631602706, 7.178327969100043227 ) ) ;
#30842=CARTESIAN_POINT ( 'NONE',  ( 147.7112127936102866, 274.8036699242858276, -9.124700685424272706 ) ) ;
#30855=CARTESIAN_POINT ( 'NONE',  ( 174.3506819931331506, 286.9267872025895940, 11.76311152586403885 ) ) ;
#30858=CARTESIAN_POINT ( 'NONE',  ( 208.2874212803407090, 269.8825990953837390, -1.143705256421198690 ) ) ;
#30859=CARTESIAN_POINT ( 'NONE',  ( 163.7010375032499212, 247.1084811230698506, 6.649922295230481950 ) ) ;
#30861=CARTESIAN_POINT ( 'NONE',  ( 188.4191156127841964, 294.8423196679893294, -11.05441416046296510 ) ) ;
#30862=CARTESIAN_POINT ( 'NONE',  ( 157.0978663001774862, 258.5455091378672137, -17.31223197570816552 ) ) ;
#30863=EDGE_CURVE ( 'NONE', #99756, #17862, #29211, .T. ) ;
#30864=CARTESIAN_POINT ( 'NONE',  ( 143.3676317564762144, 244.3923013555409511, 4.594050593750050204 ) ) ;
#30865=CARTESIAN_POINT ( 'NONE',  ( 159.5827168731687209, 254.9346697425724528, -15.70473076143803759 ) ) ;
#30866=CARTESIAN_POINT ( 'NONE',  ( 182.5138934050887940, 259.5598872865875251, 9.236875158659382024 ) ) ;
#30867=CARTESIAN_POINT ( 'NONE',  ( 65.12704176573704729, 220.6589784336661637, -6.496448406907675876E-16 ) ) ;
#30869=CARTESIAN_POINT ( 'NONE',  ( 151.3560786774222322, 268.4905770267490652, 15.54402364351346932 ) ) ;
#30870=CYLINDRICAL_SURFACE ( 'NONE', #73891, 17.82106496071139645 ) ;
#30871=ORIENTED_EDGE ( 'NONE', *, *, #60254, .F. ) ;
#30872=CARTESIAN_POINT ( 'NONE',  ( 196.1154025625812380, 290.9651539452228235, -16.59765440650598478 ) ) ;
#30873=ORIENTED_EDGE ( 'NONE', *, *, #93523, .F. ) ;
#30875=CARTESIAN_POINT ( 'NONE',  ( 197.6872697694112162, 287.3145487930856916, 17.07396129458168232 ) ) ;
#30876=CARTESIAN_POINT ( 'NONE',  ( 191.6723191112861855, 298.6608002251342100, -9.737039817265848995 ) ) ;
#30878=CARTESIAN_POINT ( 'NONE',  ( 193.7901930790854976, 294.9925349088783264, 14.24765323155741115 ) ) ;
#30880=CARTESIAN_POINT ( 'NONE',  ( 85.15457341978220995, 207.7202760586659167, -5.415160957724236172E-17 ) ) ;
#30881=VERTEX_POINT ( 'NONE', #90034 ) ;
#30885=CARTESIAN_POINT ( 'NONE',  ( 162.0148977879440508, 250.0289607786390604, -13.13131188671606786 ) ) ;
#30886=ORIENTED_EDGE ( 'NONE', *, *, #26525, .F. ) ;
#30888=CARTESIAN_POINT ( 'NONE',  ( 183.7401645296863819, 275.5702118650854686, 17.68276783697519505 ) ) ;
#30890=CARTESIAN_POINT ( 'NONE',  ( 185.1790142135946837, 260.5378326486920741, -9.806357480331048038 ) ) ;
#30894=CARTESIAN_POINT ( 'NONE',  ( 186.0348036264326481, 259.0250182415348945, 6.435743254585703177 ) ) ;
#30896=CARTESIAN_POINT ( 'NONE',  ( 200.6680263064462792, 283.0797783131037022, -17.21821073473145347 ) ) ;
#30900=CARTESIAN_POINT ( 'NONE',  ( 198.9991959707468538, 266.7910966233320664, 4.538875652460267140 ) ) ;
#30902=CARTESIAN_POINT ( 'NONE',  ( 199.0746189151364831, 265.2438329385483939, 1.559867394473611002 ) ) ;
#30905=CARTESIAN_POINT ( 'NONE',  ( 152.9518609051173996, 270.9304444175188564, 13.97502339724686138 ) ) ;
#30909=EDGE_CURVE ( 'NONE', #45951, #39202, #2663, .T. ) ;
#30910=CARTESIAN_POINT ( 'NONE',  ( 205.2391015854675516, 275.1624436846170738, -14.01434138479280911 ) ) ;
#30914=CARTESIAN_POINT ( 'NONE',  ( 171.1711017573581159, 274.6214328870215695, 17.23018440474811186 ) ) ;
#30915=CARTESIAN_POINT ( 'NONE',  ( 165.9702209435083944, 286.5350195535361877, -3.323153172973990266 ) ) ;
#30917=DIRECTION ( 'NONE',  ( -0.8660254037844387076, -0.4999999999999998890, -0.000000000000000000 ) ) ;
#30919=CARTESIAN_POINT ( 'NONE',  ( -7.997457622663985966, 160.0643266524160140, -9.188101187500093303 ) ) ;
#30920=B_SPLINE_CURVE_WITH_KNOTS ( 'NONE', 3,
 ( #49604, #95270, #3532, #65309 ),
 .UNSPECIFIED., .F., .F.,
 ( 4, 4 ),
 ( 0.008171099580468714138, 0.01417519103088871364 ),
 .UNSPECIFIED. ) ;
#30921=CARTESIAN_POINT ( 'NONE',  ( 188.4688990864094080, 295.3997683978527675, -11.43812978727723717 ) ) ;
#30922=ORIENTED_EDGE ( 'NONE', *, *, #59504, .T. ) ;
#30926=CARTESIAN_POINT ( 'NONE',  ( 18.84898279888859918, 187.8149278399161233, 9.188101187500093303 ) ) ;
#30927=CARTESIAN_POINT ( 'NONE',  ( 176.0882202740374964, 265.4570366886316037, -16.33249936588881823 ) ) ;
#30928=CARTESIAN_POINT ( 'NONE',  ( 178.4436848606596300, 273.6446589788789083, -17.07804873076608843 ) ) ;
#30932=FACE_OUTER_BOUND ( 'NONE', #70022, .T. ) ;
#30934=CARTESIAN_POINT ( 'NONE',  ( 188.9729628992022867, 259.4128536004376997, -0.8123650975293817966 ) ) ;
#30935=CARTESIAN_POINT ( 'NONE',  ( 65.98439316910437924, 202.2365022471902023, 10.00000000000009592 ) ) ;
#30936=( BOUNDED_CURVE ( )  B_SPLINE_CURVE ( 2, ( #71567, #2163, #79695, #10257, #2662, #4645, #43112, #11272, #19378, #41632, #87821, #19860, #3664, #88309, #57335, #18360, #5145, #4137, #49253, #88812, #57832, #34065, #64956, #18862, #49745, #95409, #80190, #74567, #74057, #42624, #50237, #73066, #80697, #3181, #35031, #95901, #10757, #72574, #81192, #26459, #82192, #65935, #42135, #34542, #65440, #96385, #26948, #11760, #58816, #73553, #96889, #27459, #43628, #64450, #58330, #89305, #25966, #56836, #50726, #81682, #12255, #35538, #66441, #27932, #97367, #89778, #20354, #51223, #12763, #59309, #75055, #52225, #29435, #60310, #13733, #44611, #90789, #68423, #5631, #21340, #44118, #75547, #67425, #91267, #6132, #76063, #83170, #91763, #6642, #99350, #37029, #36525, #67937, #28946, #37516, #98859, #21832, #97857, #14239, #52717, #14731, #68919, #83676, #45125, #99844, #7122, #29929, #98357, #60804, #76543, #59824, #22329, #30428, #53229, #84181, #45612, #77020, #61317, #38006, #92280, #22827, #53711, #13258, #84667, #15210, #46106, #36026, #66926, #90289, #28427, #20858, #51750, #82692, #78041, #79068, #38516, #16230, #17741, #70426, #78545, #39010, #1035, #94760, #41, #25324, #2034, #40511, #70944, #71446, #31913, #77547, #94266, #62818, #9133, #61811, #93774, #69916, #40004, #47618, #48123, #48641, #30926, #85691, #1548, #92761, #32921, #47120, #63825, #8137, #55209, #24332, #54709, #56210, #8632, #86190, #16726, #32431, #63326, #24822, #39499, #531, #69427, #55696, #62306, #86685, #9653, #17217, #87207, #7624, #23316, #54203, #85171, #15714, #46616, #31418, #93262, #23816, #2547, #20233, #19258, #33430, #42994, #18240, #49135, #80069, #72456, #64836, #10135, #64327, #89673, #89194, #57709, #72956, #88188, #95783, #10640, #50125, #41514, #95287, #87706, #34426, #79576, #42022, #81078, #3062, #25847, #65326, #81562, #11644, #41002, #18737, #11153, #71944, #49621, #26830, #3548, #56724, #33949, #26335, #57212, #19743, #96768, #88688, #80574, #96263, #42503, #73440, #4024, #34908, #12131, #65808, #35417, #27334, #58216, #50607, #73931, #4517, #66324, #97256, #27822, #58698, #92168, #67820, #21715, #75946, #22212, #43995, #6523, #99728, #82575, #68304, #37399, #14620, #35912, #99227, #53110, #74937, #44499, #74450, #90163, #67309, #66811, #45499, #29814, #83054, #5030, #29322, #51106, #60687, #91645, #28821, #13138, #6014, #21228, #91150, #5520, #84066, #52598, #83555, #59705, #20735, #14120, #45000, #52107, #51621, #76432, #7005, #90671, #59187, #13627, #37892, #75430, #36907, #68800, #30314, #98743, #36403, #61200, #82071, #98236, #60189, #97741, #12639, #43511, #28308, #77932, #47017, #55102, #53603, #15100, #9538, #30822, #8032, #24710, #54095, #38905, #39889, #7506, #62196, #61702, #92654, #85051, #76908, #23204, #8523, #69316, #71336, #84561, #39392, #15598, #70309, #40399, #45991, #1928, #48006, #86576, #16613, #17109, #922, #46498, #70824, #77434, #69809, #38403, #94157, #16119, #1433, #62700, #419, #100238, #31308, #93147, #93657, #23698, #78950, #54593, #32814, #85575, #31798, #24222, #86089, #47509, #78436, #63719, #94657, #32314, #9017, #63215, #55593, #41914, #26721, #95167, #72849, #42398, #64216, #3441, #34318, #88583, #79466, #11037, #57603, #10528, #2439, #87089, #18125, #10030, #40892, #19145, #65216, #72347, #17625, #26225, #25212, #96158, #50019, #79960, #25735, #64729, #41403, #71841, #80973, #11538, #73332, #3919, #56096, #18633, #48529, #33317, #56615, #57101, #87599, #49026, #2952, #33841, #95678, #88083, #49512, #80466, #86909, #8349, #8840, #7851, #62521, #62020, #31127, #9871, #63539, #47335, #38734, #93987, #15423, #71168, #1764, #93483, #46842, #70639, #85913, #55418, #70126, #32644, #86403, #24537, #16935, #63042, #47822, #78761, #16440, #85392, #9348, #71674, #24038, #23526, #78260, #48352, #39711, #54937, #79302, #17446, #1253, #54416, #40224, #32134, #39219, #739, #69638, #56441, #94481, #246, #25036, #55916, #40728, #46320, #77246, #2264, #92971, #31623, #33146, #15938, #64046, #94991, #77765, #25553, #26059, #27057, #18463, #10361, #95513, #42231, #2773, #4756, #87435, #11381, #56935, #80805, #74164, #79795, #35638, #81781, #19955, #50338, #50832, #34641, #73170, #41227, #10862, #87920, #17968, #27563, #49846, #4235, #96487, #49351, #72168, #33662, #65049, #57938, #64552, #12357, #95999, #43223, #80290, #26559, #57433, #41736, #48863, #58428, #3760, #35135, #88921, #72680, #3274, #34157, #88412, #19481, #18970, #66540, #65539, #97467, #81290, #11863, #42719, #73656, #66046, #96992, #28034, #89404, #45222, #99944, #75643, #29535, #83773, #30023, #51847, #14334, #7218, #90390, #76160, #6737, #22428, #43725, #37613, #21438, #59920, #28527, #51328, #5731, #5244, #74667, #53319, #68525, #90889, #82295, #37123, #58910, #99447, #60908, #36619, #20964, #13832, #29051, #98952, #67528, #76633, #98457, #68031, #60408, #6229, #91363, #21927, #52324, #59410, #52816, #14821, #83266, #67027, #44710, #91873, #84276, #45709, #38102, #69014, #36124, #12865, #89880, #20454, #82788, #13352, #97954, #44218, #75155, #84767, #85793, #23917, #32011, #30527, #92368, #86787, #7724, #85269, #1649, #31017, #8727, #16325, #39100, #46719, #69520, #70519, #61908, #53802, #134, #47218, #46202, #48226, #61415, #78140, #92857, #39599, #17321, #22916, #79173, #24920, #93360, #15303, #629, #1134, #62921, #77119, #54301, #77647, #93871, #23411, #15815, #86284, #70013, #8233, #31509, #24428, #71546, #55304, #16820, #47707, #78645, #9228, #40107, #71047, #32533, #63427, #94366, #40612, #55794, #80678, #95880, #10738, #18343, #41106, #42116, #33533, #25420, #10237, #57317, #17842, #64936, #73050, #64430, #48743, #88288, #4117, #3643, #63921, #41612, #34046, #94860, #72557, #49721, #26438, #56313, #25944, #72041, #2140, #42602, #18841, #34524, #73536, #12235, #96869, #56819, #35012, #87309, #11253, #3161, #65423, #96366, #2645, #26932, #89288 ),
 .UNSPECIFIED., .F., .T. ) 
 B_SPLINE_CURVE_WITH_KNOTS ( ( 3, 2, 2, 2, 2, 2, 2, 2, 2, 2, 2, 2, 2, 2, 2, 2, 2, 2, 2, 2, 2, 2, 2, 2, 2, 2, 2, 2, 2, 2, 2, 2, 2, 2, 2, 2, 2, 2, 2, 2, 2, 2, 2, 2, 2, 2, 2, 2, 2, 2, 2, 2, 2, 2, 2, 2, 2, 2, 2, 2, 2, 2, 2, 2, 2, 2, 2, 2, 2, 2, 2, 2, 2, 2, 2, 2, 2, 2, 2, 2, 2, 2, 2, 2, 2, 2, 2, 2, 2, 2, 2, 2, 2, 2, 2, 2, 2, 2, 2, 2, 2, 2, 2, 2, 2, 2, 2, 2, 2, 2, 2, 2, 2, 2, 2, 2, 2, 2, 2, 2, 2, 2, 2, 2, 2, 2, 2, 2, 2, 2, 2, 2, 2, 2, 2, 2, 2, 2, 2, 2, 2, 2, 2, 2, 2, 2, 2, 2, 2, 2, 2, 2, 2, 2, 2, 2, 2, 2, 2, 2, 2, 2, 2, 2, 2, 2, 2, 2, 2, 2, 2, 2, 2, 2, 2, 2, 2, 2, 2, 2, 2, 2, 2, 2, 2, 2, 2, 2, 2, 2, 2, 2, 2, 2, 2, 2, 2, 2, 2, 2, 2, 2, 2, 2, 2, 2, 2, 2, 2, 2, 2, 2, 2, 2, 2, 2, 2, 2, 2, 2, 2, 2, 2, 2, 2, 2, 2, 2, 2, 2, 2, 2, 2, 2, 2, 2, 2, 2, 2, 2, 2, 2, 2, 2, 2, 2, 2, 2, 2, 2, 2, 2, 2, 2, 2, 2, 2, 2, 2, 2, 2, 2, 2, 2, 2, 2, 2, 2, 2, 2, 2, 2, 2, 2, 2, 2, 2, 2, 2, 2, 2, 2, 2, 2, 2, 2, 2, 2, 2, 2, 2, 2, 2, 2, 2, 2, 2, 2, 2, 2, 2, 2, 2, 2, 2, 2, 2, 2, 2, 2, 2, 2, 2, 2, 2, 2, 2, 2, 2, 2, 2, 2, 2, 2, 2, 2, 2, 2, 2, 2, 2, 2, 2, 2, 2, 2, 2, 2, 2, 2, 2, 2, 2, 2, 2, 2, 2, 2, 2, 2, 2, 2, 2, 2, 2, 2, 2, 2, 2, 2, 2, 2, 2, 2, 2, 2, 2, 3 ),
 ( 0.000000000000000000, 0.002688172043010752903, 0.005376344086021505805, 0.008064516129032257841, 0.01075268817204301161, 0.01344086021505376365, 0.01612903225806451568, 0.01881720430107526945, 0.02150537634408602322, 0.02419354838709677352, 0.02688172043010752729, 0.02956989247311828106, 0.03225806451612903136, 0.03494623655913978166, 0.03763440860215053890, 0.04032258064516128920, 0.04301075268817204644, 0.04569892473118279674, 0.04838709677419354704, 0.05107526881720430428, 0.05376344086021505458, 0.05645161290322580488, 0.05913978494623656212, 0.06182795698924731242, 0.06451612903225806273, 0.06720430107526881303, 0.06989247311827956333, 0.07258064516129032751, 0.07526881720430107781, 0.07795698924731182811, 0.08064516129032257841, 0.08333333333333332871, 0.08602150537634409289, 0.08870967741935484319, 0.09139784946236559349, 0.09408602150537634379, 0.09677419354838709409, 0.09946236559139784439, 0.1021505376344086086, 0.1048387096774193589, 0.1075268817204301092, 0.1102150537634408595, 0.1129032258064516098, 0.1155913978494623601, 0.1182795698924731242, 0.1209677419354838745, 0.1236559139784946248, 0.1263440860215053752, 0.1290322580645161255, 0.1317204301075268758, 0.1344086021505376261, 0.1370967741935483764, 0.1397849462365591267, 0.1424731182795699047, 0.1451612903225806550, 0.1478494623655914053, 0.1505376344086021556, 0.1532258064516129059, 0.1559139784946236562, 0.1586021505376344065, 0.1612903225806451568, 0.1639784946236559071, 0.1666666666666666574, 0.1693548387096774077, 0.1720430107526881858, 0.1747311827956989361, 0.1774193548387096864, 0.1801075268817204367, 0.1827956989247311870, 0.1854838709677419373, 0.1881720430107526876, 0.1908602150537634379, 0.1935483870967741882, 0.1962365591397849385, 0.1989247311827956888, 0.2016129032258064391, 0.2043010752688172171, 0.2069892473118279674, 0.2096774193548387177, 0.2123655913978494680, 0.2150537634408602183, 0.2177419354838709686, 0.2204301075268817189, 0.2231182795698924692, 0.2258064516129032195, 0.2284946236559139698, 0.2311827956989247201, 0.2338709677419354704, 0.2365591397849462485, 0.2392473118279569988, 0.2419354838709677491, 0.2446236559139784994, 0.2473118279569892497, 0.2500000000000000000, 0.2526881720430107503, 0.2553763440860215006, 0.2580645161290322509, 0.2607526881720430012, 0.2634408602150537515, 0.2661290322580645018, 0.2688172043010752521, 0.2715053763440860024, 0.2741935483870967527, 0.2768817204301075030, 0.2795698924731182533, 0.2822580645161290591, 0.2849462365591398094, 0.2876344086021505597, 0.2903225806451613100, 0.2930107526881720603, 0.2956989247311828106, 0.2983870967741935609, 0.3010752688172043112, 0.3037634408602150615, 0.3064516129032258118, 0.3091397849462365621, 0.3118279569892473124, 0.3145161290322580627, 0.3172043010752688130, 0.3198924731182795633, 0.3225806451612903136, 0.3252688172043010639, 0.3279569892473118142, 0.3306451612903225645, 0.3333333333333333148, 0.3360215053763440651, 0.3387096774193548154, 0.3413978494623655657, 0.3440860215053763715, 0.3467741935483871218, 0.3494623655913978721, 0.3521505376344086224, 0.3548387096774193727, 0.3575268817204301230, 0.3602150537634408733, 0.3629032258064516236, 0.3655913978494623739, 0.3682795698924731242, 0.3709677419354838745, 0.3736559139784946248, 0.3763440860215053752, 0.3790322580645161255, 0.3817204301075268758, 0.3844086021505376261, 0.3870967741935483764, 0.3897849462365591267, 0.3924731182795698770, 0.3951612903225806273, 0.3978494623655913776, 0.4005376344086021279, 0.4032258064516128782, 0.4059139784946236285, 0.4086021505376344343, 0.4112903225806451846, 0.4139784946236559349, 0.4166666666666666852, 0.4193548387096774355, 0.4220430107526881858, 0.4247311827956989361, 0.4274193548387096864, 0.4301075268817204367, 0.4327956989247311870, 0.4354838709677419373, 0.4381720430107526876, 0.4408602150537634379, 0.4435483870967741882, 0.4462365591397849385, 0.4489247311827956888, 0.4516129032258064391, 0.4543010752688171894, 0.4569892473118279397, 0.4596774193548386900, 0.4623655913978494403, 0.4650537634408601906, 0.4677419354838709409, 0.4704301075268817467, 0.4731182795698924970, 0.4758064516129032473, 0.4784946236559139976, 0.4811827956989247479, 0.4838709677419354982, 0.4865591397849462485, 0.4892473118279569988, 0.4919354838709677491, 0.4946236559139784994, 0.4973118279569892497, 0.5000000000000000000, 0.5026881720430107503, 0.5053763440860215006, 0.5080645161290322509, 0.5107526881720430012, 0.5134408602150537515, 0.5161290322580645018, 0.5188172043010752521, 0.5215053763440860024, 0.5241935483870967527, 0.5268817204301075030, 0.5295698924731182533, 0.5322580645161290036, 0.5349462365591397539, 0.5376344086021505042, 0.5403225806451612545, 0.5430107526881720048, 0.5456989247311827551, 0.5483870967741935054, 0.5510752688172042557, 0.5537634408602150060, 0.5564516129032257563, 0.5591397849462365066, 0.5618279569892472569, 0.5645161290322581182, 0.5672043010752688685, 0.5698924731182796188, 0.5725806451612903691, 0.5752688172043011194, 0.5779569892473118697, 0.5806451612903226200, 0.5833333333333333703, 0.5860215053763441206, 0.5887096774193548709, 0.5913978494623656212, 0.5940860215053763715, 0.5967741935483871218, 0.5994623655913978721, 0.6021505376344086224, 0.6048387096774193727, 0.6075268817204301230, 0.6102150537634408733, 0.6129032258064516236, 0.6155913978494623739, 0.6182795698924731242, 0.6209677419354838745, 0.6236559139784946248, 0.6263440860215053752, 0.6290322580645161255, 0.6317204301075268758, 0.6344086021505376261, 0.6370967741935483764, 0.6397849462365591267, 0.6424731182795698770, 0.6451612903225806273, 0.6478494623655913776, 0.6505376344086021279, 0.6532258064516128782, 0.6559139784946236285, 0.6586021505376343788, 0.6612903225806451291, 0.6639784946236558794, 0.6666666666666666297, 0.6693548387096773800, 0.6720430107526881303, 0.6747311827956988806, 0.6774193548387096309, 0.6801075268817203812, 0.6827956989247311315, 0.6854838709677418818, 0.6881720430107527431, 0.6908602150537634934, 0.6935483870967742437, 0.6962365591397849940, 0.6989247311827957443, 0.7016129032258064946, 0.7043010752688172449, 0.7069892473118279952, 0.7096774193548387455, 0.7123655913978494958, 0.7150537634408602461, 0.7177419354838709964, 0.7204301075268817467, 0.7231182795698924970, 0.7258064516129032473, 0.7284946236559139976, 0.7311827956989247479, 0.7338709677419354982, 0.7365591397849462485, 0.7392473118279569988, 0.7419354838709677491, 0.7446236559139784994, 0.7473118279569892497, 0.7500000000000000000, 0.7526881720430107503, 0.7553763440860215006, 0.7580645161290322509, 0.7607526881720430012, 0.7634408602150537515, 0.7661290322580645018, 0.7688172043010752521, 0.7715053763440860024, 0.7741935483870967527, 0.7768817204301075030, 0.7795698924731182533, 0.7822580645161290036, 0.7849462365591397539, 0.7876344086021505042, 0.7903225806451612545, 0.7930107526881720048, 0.7956989247311827551, 0.7983870967741935054, 0.8010752688172042557, 0.8037634408602150060, 0.8064516129032257563, 0.8091397849462365066, 0.8118279569892472569, 0.8145161290322581182, 0.8172043010752688685, 0.8198924731182796188, 0.8225806451612903691, 0.8252688172043011194, 0.8279569892473118697, 0.8306451612903226200, 0.8333333333333333703, 0.8360215053763441206, 0.8387096774193548709, 0.8413978494623656212, 0.8440860215053763715, 0.8467741935483871218, 0.8494623655913978721, 0.8521505376344086224, 0.8548387096774193727, 0.8575268817204301230, 0.8602150537634408733, 0.8629032258064516236, 0.8655913978494623739, 0.8682795698924731242, 0.8709677419354838745, 0.8736559139784946248, 0.8763440860215053752, 0.8790322580645161255, 0.8817204301075268758, 0.8844086021505376261, 0.8870967741935483764, 0.8897849462365591267, 0.8924731182795698770, 0.8951612903225806273, 0.8978494623655913776, 0.9005376344086021279, 0.9032258064516128782, 0.9059139784946236285, 0.9086021505376343788, 0.9112903225806451291, 0.9139784946236558794, 0.9166666666666666297, 0.9193548387096773800, 0.9220430107526881303, 0.9247311827956988806, 0.9274193548387096309, 0.9301075268817203812, 0.9327956989247311315, 0.9354838709677418818, 0.9381720430107527431, 0.9408602150537634934, 0.9435483870967742437, 0.9462365591397849940, 0.9489247311827957443, 0.9516129032258064946, 0.9543010752688172449, 0.9569892473118279952, 0.9596774193548387455, 0.9623655913978494958, 0.9650537634408602461, 0.9677419354838709964, 0.9704301075268817467, 0.9731182795698924970, 0.9758064516129032473, 0.9784946236559139976, 0.9811827956989247479, 0.9838709677419354982, 0.9855363728105643872 ),
 .UNSPECIFIED. ) 
 CURVE ( )  GEOMETRIC_REPRESENTATION_ITEM ( )  RATIONAL_B_SPLINE_CURVE ( ( 1.000000000000000000, 0.8660254037844387076, 1.000000000000000000, 0.8660254037844387076, 1.000000000000000000, 0.8660254037844387076, 1.000000000000000000, 0.8660254037844387076, 1.000000000000000000, 0.8660254037844387076, 1.000000000000000000, 0.8660254037844387076, 1.000000000000000000, 0.8660254037844387076, 1.000000000000000000, 0.8660254037844387076, 1.000000000000000000, 0.8660254037844387076, 1.000000000000000000, 0.8660254037844387076, 1.000000000000000000, 0.8660254037844387076, 1.000000000000000000, 0.8660254037844387076, 1.000000000000000000, 0.8660254037844387076, 1.000000000000000000, 0.8660254037844387076, 1.000000000000000000, 0.8660254037844387076, 1.000000000000000000, 0.8660254037844387076, 1.000000000000000000, 0.8660254037844387076, 1.000000000000000000, 0.8660254037844387076, 1.000000000000000000, 0.8660254037844387076, 1.000000000000000000, 0.8660254037844387076, 1.000000000000000000, 0.8660254037844387076, 1.000000000000000000, 0.8660254037844387076, 1.000000000000000000, 0.8660254037844387076, 1.000000000000000000, 0.8660254037844387076, 1.000000000000000000, 0.8660254037844387076, 1.000000000000000000, 0.8660254037844387076, 1.000000000000000000, 0.8660254037844387076, 1.000000000000000000, 0.8660254037844387076, 1.000000000000000000, 0.8660254037844387076, 1.000000000000000000, 0.8660254037844387076, 1.000000000000000000, 0.8660254037844387076, 1.000000000000000000, 0.8660254037844387076, 1.000000000000000000, 0.8660254037844387076, 1.000000000000000000, 0.8660254037844387076, 1.000000000000000000, 0.8660254037844387076, 1.000000000000000000, 0.8660254037844387076, 1.000000000000000000, 0.8660254037844387076, 1.000000000000000000, 0.8660254037844387076, 1.000000000000000000, 0.8660254037844387076, 1.000000000000000000, 0.8660254037844387076, 1.000000000000000000, 0.8660254037844387076, 1.000000000000000000, 0.8660254037844387076, 1.000000000000000000, 0.8660254037844387076, 1.000000000000000000, 0.8660254037844387076, 1.000000000000000000, 0.8660254037844387076, 1.000000000000000000, 0.8660254037844387076, 1.000000000000000000, 0.8660254037844387076, 1.000000000000000000, 0.8660254037844387076, 1.000000000000000000, 0.8660254037844387076, 1.000000000000000000, 0.8660254037844387076, 1.000000000000000000, 0.8660254037844387076, 1.000000000000000000, 0.8660254037844387076, 1.000000000000000000, 0.8660254037844387076, 1.000000000000000000, 0.8660254037844387076, 1.000000000000000000, 0.8660254037844387076, 1.000000000000000000, 0.8660254037844387076, 1.000000000000000000, 0.8660254037844387076, 1.000000000000000000, 0.8660254037844387076, 1.000000000000000000, 0.8660254037844387076, 1.000000000000000000, 0.8660254037844387076, 1.000000000000000000, 0.8660254037844387076, 1.000000000000000000, 0.8660254037844387076, 1.000000000000000000, 0.8660254037844387076, 1.000000000000000000, 0.8660254037844387076, 1.000000000000000000, 0.8660254037844387076, 1.000000000000000000, 0.8660254037844387076, 1.000000000000000000, 0.8660254037844387076, 1.000000000000000000, 0.8660254037844387076, 1.000000000000000000, 0.8660254037844387076, 1.000000000000000000, 0.8660254037844387076, 1.000000000000000000, 0.8660254037844387076, 1.000000000000000000, 0.8660254037844387076, 1.000000000000000000, 0.8660254037844387076, 1.000000000000000000, 0.8660254037844387076, 1.000000000000000000, 0.8660254037844387076, 1.000000000000000000, 0.8660254037844387076, 1.000000000000000000, 0.8660254037844387076, 1.000000000000000000, 0.8660254037844387076, 1.000000000000000000, 0.8660254037844387076, 1.000000000000000000, 0.8660254037844387076, 1.000000000000000000, 0.8660254037844387076, 1.000000000000000000, 0.8660254037844387076, 1.000000000000000000, 0.8660254037844387076, 1.000000000000000000, 0.8660254037844387076, 1.000000000000000000, 0.8660254037844387076, 1.000000000000000000, 0.8660254037844387076, 1.000000000000000000, 0.8660254037844387076, 1.000000000000000000, 0.8660254037844387076, 1.000000000000000000, 0.8660254037844387076, 1.000000000000000000, 0.8660254037844387076, 1.000000000000000000, 0.8660254037844387076, 1.000000000000000000, 0.8660254037844387076, 1.000000000000000000, 0.8660254037844387076, 1.000000000000000000, 0.8660254037844387076, 1.000000000000000000, 0.8660254037844387076, 1.000000000000000000, 0.8660254037844387076, 1.000000000000000000, 0.8660254037844387076, 1.000000000000000000, 0.8660254037844387076, 1.000000000000000000, 0.8660254037844387076, 1.000000000000000000, 0.8660254037844387076, 1.000000000000000000, 0.8660254037844387076, 1.000000000000000000, 0.8660254037844387076, 1.000000000000000000, 0.8660254037844387076, 1.000000000000000000, 0.8660254037844387076, 1.000000000000000000, 0.8660254037844387076, 1.000000000000000000, 0.8660254037844387076, 1.000000000000000000, 0.8660254037844387076, 1.000000000000000000, 0.8660254037844387076, 1.000000000000000000, 0.8660254037844387076, 1.000000000000000000, 0.8660254037844387076, 1.000000000000000000, 0.8660254037844387076, 1.000000000000000000, 0.8660254037844387076, 1.000000000000000000, 0.8660254037844387076, 1.000000000000000000, 0.8660254037844387076, 1.000000000000000000, 0.8660254037844387076, 1.000000000000000000, 0.8660254037844387076, 1.000000000000000000, 0.8660254037844387076, 1.000000000000000000, 0.8660254037844387076, 1.000000000000000000, 0.8660254037844387076, 1.000000000000000000, 0.8660254037844387076, 1.000000000000000000, 0.8660254037844387076, 1.000000000000000000, 0.8660254037844387076, 1.000000000000000000, 0.8660254037844387076, 1.000000000000000000, 0.8660254037844387076, 1.000000000000000000, 0.8660254037844387076, 1.000000000000000000, 0.8660254037844387076, 1.000000000000000000, 0.8660254037844387076, 1.000000000000000000, 0.8660254037844387076, 1.000000000000000000, 0.8660254037844387076, 1.000000000000000000, 0.8660254037844387076, 1.000000000000000000, 0.8660254037844387076, 1.000000000000000000, 0.8660254037844387076, 1.000000000000000000, 0.8660254037844387076, 1.000000000000000000, 0.8660254037844387076, 1.000000000000000000, 0.8660254037844387076, 1.000000000000000000, 0.8660254037844387076, 1.000000000000000000, 0.8660254037844387076, 1.000000000000000000, 0.8660254037844387076, 1.000000000000000000, 0.8660254037844387076, 1.000000000000000000, 0.8660254037844387076, 1.000000000000000000, 0.8660254037844387076, 1.000000000000000000, 0.8660254037844387076, 1.000000000000000000, 0.8660254037844387076, 1.000000000000000000, 0.8660254037844387076, 1.000000000000000000, 0.8660254037844387076, 1.000000000000000000, 0.8660254037844387076, 1.000000000000000000, 0.8660254037844387076, 1.000000000000000000, 0.8660254037844387076, 1.000000000000000000, 0.8660254037844387076, 1.000000000000000000, 0.8660254037844387076, 1.000000000000000000, 0.8660254037844387076, 1.000000000000000000, 0.8660254037844387076, 1.000000000000000000, 0.8660254037844387076, 1.000000000000000000, 0.8660254037844387076, 1.000000000000000000, 0.8660254037844387076, 1.000000000000000000, 0.8660254037844387076, 1.000000000000000000, 0.8660254037844387076, 1.000000000000000000, 0.8660254037844387076, 1.000000000000000000, 0.8660254037844387076, 1.000000000000000000, 0.8660254037844387076, 1.000000000000000000, 0.8660254037844387076, 1.000000000000000000, 0.8660254037844387076, 1.000000000000000000, 0.8660254037844387076, 1.000000000000000000, 0.8660254037844387076, 1.000000000000000000, 0.8660254037844387076, 1.000000000000000000, 0.8660254037844387076, 1.000000000000000000, 0.8660254037844387076, 1.000000000000000000, 0.8660254037844387076, 1.000000000000000000, 0.8660254037844387076, 1.000000000000000000, 0.8660254037844387076, 1.000000000000000000, 0.8660254037844387076, 1.000000000000000000, 0.8660254037844387076, 1.000000000000000000, 0.8660254037844387076, 1.000000000000000000, 0.8660254037844387076, 1.000000000000000000, 0.8660254037844387076, 1.000000000000000000, 0.8660254037844387076, 1.000000000000000000, 0.8660254037844387076, 1.000000000000000000, 0.8660254037844387076, 1.000000000000000000, 0.8660254037844387076, 1.000000000000000000, 0.8660254037844387076, 1.000000000000000000, 0.8660254037844387076, 1.000000000000000000, 0.8660254037844387076, 1.000000000000000000, 0.8660254037844387076, 1.000000000000000000, 0.8660254037844387076, 1.000000000000000000, 0.8660254037844387076, 1.000000000000000000, 0.8660254037844387076, 1.000000000000000000, 0.8660254037844387076, 1.000000000000000000, 0.8660254037844387076, 1.000000000000000000, 0.8660254037844387076, 1.000000000000000000, 0.8660254037844387076, 1.000000000000000000, 0.8660254037844387076, 1.000000000000000000, 0.8660254037844387076, 1.000000000000000000, 0.8660254037844387076, 1.000000000000000000, 0.8660254037844387076, 1.000000000000000000, 0.8660254037844387076, 1.000000000000000000, 0.8660254037844387076, 1.000000000000000000, 0.8660254037844387076, 1.000000000000000000, 0.8660254037844387076, 1.000000000000000000, 0.8660254037844387076, 1.000000000000000000, 0.8660254037844387076, 1.000000000000000000, 0.8660254037844387076, 1.000000000000000000, 0.8660254037844387076, 1.000000000000000000, 0.8660254037844387076, 1.000000000000000000, 0.8660254037844387076, 1.000000000000000000, 0.8660254037844387076, 1.000000000000000000, 0.8660254037844387076, 1.000000000000000000, 0.8660254037844387076, 1.000000000000000000, 0.8660254037844387076, 1.000000000000000000, 0.8660254037844387076, 1.000000000000000000, 0.8660254037844387076, 1.000000000000000000, 0.8660254037844387076, 1.000000000000000000, 0.8660254037844387076, 1.000000000000000000, 0.8660254037844387076, 1.000000000000000000, 0.8660254037844387076, 1.000000000000000000, 0.8660254037844387076, 1.000000000000000000, 0.8660254037844387076, 1.000000000000000000, 0.8660254037844387076, 1.000000000000000000, 0.8660254037844387076, 1.000000000000000000, 0.8660254037844387076, 1.000000000000000000, 0.8660254037844387076, 1.000000000000000000, 0.8660254037844387076, 1.000000000000000000, 0.8660254037844387076, 1.000000000000000000, 0.8660254037844387076, 1.000000000000000000, 0.8660254037844387076, 1.000000000000000000, 0.8660254037844387076, 1.000000000000000000, 0.8660254037844387076, 1.000000000000000000, 0.8660254037844387076, 1.000000000000000000, 0.8660254037844387076, 1.000000000000000000, 0.8660254037844387076, 1.000000000000000000, 0.8660254037844387076, 1.000000000000000000, 0.8660254037844387076, 1.000000000000000000, 0.8660254037844387076, 1.000000000000000000, 0.8660254037844387076, 1.000000000000000000, 0.8660254037844387076, 1.000000000000000000, 0.8660254037844387076, 1.000000000000000000, 0.8660254037844387076, 1.000000000000000000, 0.8660254037844387076, 1.000000000000000000, 0.8660254037844387076, 1.000000000000000000, 0.8660254037844387076, 1.000000000000000000, 0.8660254037844387076, 1.000000000000000000, 0.8660254037844387076, 1.000000000000000000, 0.8660254037844387076, 1.000000000000000000, 0.8660254037844387076, 1.000000000000000000, 0.8660254037844387076, 1.000000000000000000, 0.8660254037844387076, 1.000000000000000000, 0.8660254037844387076, 1.000000000000000000, 0.8660254037844387076, 1.000000000000000000, 0.8660254037844387076, 1.000000000000000000, 0.8660254037844387076, 1.000000000000000000, 0.8660254037844387076, 1.000000000000000000, 0.8660254037844387076, 1.000000000000000000, 0.8660254037844387076, 1.000000000000000000, 0.8660254037844387076, 1.000000000000000000, 0.8660254037844387076, 1.000000000000000000, 0.8660254037844387076, 1.000000000000000000, 0.8660254037844387076, 1.000000000000000000, 0.8660254037844387076, 1.000000000000000000, 0.8660254037844387076, 1.000000000000000000, 0.8660254037844387076, 1.000000000000000000, 0.8660254037844387076, 1.000000000000000000, 0.8660254037844387076, 1.000000000000000000, 0.8660254037844387076, 1.000000000000000000, 0.8660254037844387076, 1.000000000000000000, 0.8660254037844387076, 1.000000000000000000, 0.8660254037844387076, 1.000000000000000000, 0.8660254037844387076, 1.000000000000000000, 0.8660254037844387076, 1.000000000000000000, 0.8660254037844387076, 1.000000000000000000, 0.8660254037844387076, 1.000000000000000000, 0.8660254037844387076, 1.000000000000000000, 0.8660254037844387076, 1.000000000000000000, 0.8660254037844387076, 1.000000000000000000, 0.8660254037844387076, 1.000000000000000000, 0.8660254037844387076, 1.000000000000000000, 0.8660254037844387076, 1.000000000000000000, 0.8660254037844387076, 1.000000000000000000, 0.8660254037844387076, 1.000000000000000000, 0.8660254037844387076, 1.000000000000000000, 0.8660254037844387076, 1.000000000000000000, 0.8660254037844387076, 1.000000000000000000, 0.8660254037844387076, 1.000000000000000000, 0.8660254037844387076, 1.000000000000000000, 0.8660254037844387076, 1.000000000000000000, 0.8660254037844387076, 1.000000000000000000, 0.8660254037844387076, 1.000000000000000000, 0.8660254037844387076, 1.000000000000000000, 0.8660254037844387076, 1.000000000000000000, 0.8660254037844387076, 1.000000000000000000, 0.8660254037844387076, 1.000000000000000000, 0.8660254037844387076, 1.000000000000000000, 0.8660254037844387076, 1.000000000000000000, 0.8660254037844387076, 1.000000000000000000, 0.8660254037844387076, 1.000000000000000000, 0.8660254037844387076, 1.000000000000000000, 0.8660254037844387076, 1.000000000000000000, 0.8660254037844387076, 1.000000000000000000, 0.8660254037844387076, 1.000000000000000000, 0.8660254037844387076, 1.000000000000000000, 0.8660254037844387076, 1.000000000000000000, 0.8660254037844387076, 1.000000000000000000, 0.8660254037844387076, 1.000000000000000000, 0.8660254037844387076, 1.000000000000000000, 0.8660254037844387076, 1.000000000000000000, 0.8660254037844387076, 1.000000000000000000, 0.8660254037844387076, 1.000000000000000000, 0.8660254037844387076, 1.000000000000000000, 0.8660254037844387076, 1.000000000000000000, 0.8660254037844387076, 1.000000000000000000, 0.8660254037844387076, 1.000000000000000000, 0.8660254037844387076, 1.000000000000000000, 0.8660254037844387076, 1.000000000000000000, 0.8660254037844387076, 1.000000000000000000, 0.8660254037844387076, 1.000000000000000000, 0.8660254037844387076, 1.000000000000000000, 0.8660254037844387076, 1.000000000000000000, 0.8660254037844387076, 1.000000000000000000, 0.8660254037844387076, 1.000000000000000000, 0.8660254037844387076, 1.000000000000000000, 0.8660254037844387076, 1.000000000000000000, 0.8660254037844387076, 1.000000000000000000, 0.8660254037844387076, 1.000000000000000000, 0.8660254037844387076, 1.000000000000000000, 0.8660254037844387076, 1.000000000000000000, 0.8660254037844387076, 1.000000000000000000, 0.8660254037844387076, 1.000000000000000000, 0.8660254037844387076, 1.000000000000000000, 0.8660254037844387076, 1.000000000000000000, 0.8660254037844387076, 1.000000000000000000, 0.8660254037844387076, 1.000000000000000000, 0.8660254037844387076, 1.000000000000000000, 0.8660254037844387076, 1.000000000000000000, 0.8660254037844387076, 1.000000000000000000, 0.8660254037844387076, 1.000000000000000000, 0.8660254037844387076, 1.000000000000000000, 0.8660254037844387076, 1.000000000000000000, 0.8660254037844387076, 1.000000000000000000, 0.8660254037844387076, 1.000000000000000000, 0.8660254037844387076, 1.000000000000000000, 0.8660254037844387076, 1.000000000000000000, 0.8660254037844387076, 1.000000000000000000, 0.8660254037844387076, 1.000000000000000000, 0.8660254037844387076, 1.000000000000000000, 0.8660254037844387076, 1.000000000000000000, 0.8660254037844387076, 1.000000000000000000, 0.8660254037844387076, 1.000000000000000000, 0.8660254037844387076, 1.000000000000000000, 0.8660254037844387076, 1.000000000000000000, 0.8660254037844387076, 1.000000000000000000, 0.8660254037844387076, 1.000000000000000000, 0.8660254037844387076, 1.000000000000000000, 0.8660254037844387076, 1.000000000000000000, 0.8660254037844387076, 1.000000000000000000, 0.8660254037844387076, 1.000000000000000000, 0.8660254037844387076, 1.000000000000000000, 0.8660254037844387076, 1.000000000000000000, 0.8660254037844387076, 1.000000000000000000, 0.8660254037844387076, 1.000000000000000000, 0.8660254037844387076, 1.000000000000000000, 0.8660254037844387076, 1.000000000000000000, 0.8660254037844387076, 1.000000000000000000, 0.8660254037844387076, 1.000000000000000000, 0.8660254037844387076, 1.000000000000000000, 0.8660254037844387076, 1.000000000000000000, 0.8660254037844387076, 1.000000000000000000, 0.8660254037844387076, 1.000000000000000000, 0.8660254037844387076, 1.000000000000000000, 0.9169986265629754829, 0.9368410486966849415 ) ) 
 REPRESENTATION_ITEM ( '' )  );
#30937=CARTESIAN_POINT ( 'NONE',  ( 167.9496373820661290, 248.6204696539478789, -6.517719931589019744 ) ) ;
#30939=CARTESIAN_POINT ( 'NONE',  ( 33.57141466322406131, 196.3149278399160949, -9.188101187500095079 ) ) ;
#30942=CARTESIAN_POINT ( 'NONE',  ( 203.3114313796560282, 269.4513687231070662, -5.937407854999036338 ) ) ;
#30946=CARTESIAN_POINT ( 'NONE',  ( 159.8715144876434238, 278.4871566375445582, -9.860745765539576269 ) ) ;
#30951=CARTESIAN_POINT ( 'NONE',  ( 188.8167911736601354, 269.9502213024455841, -14.08247674505766867 ) ) ;
#30952=ORIENTED_EDGE ( 'NONE', *, *, #22000, .F. ) ;
#30957=CARTESIAN_POINT ( 'NONE',  ( 207.8575108622103755, 270.6272257822888037, -6.381720258959569847 ) ) ;
#30958=CARTESIAN_POINT ( 'NONE',  ( 174.6066048939933921, 262.0940252294753918, 15.79829227059981278 ) ) ;
#30959=EDGE_CURVE ( 'NONE', #95124, #25119, #46041, .T. ) ;
#30961=CARTESIAN_POINT ( 'NONE',  ( 181.2335612792182076, 257.5653981390558442, -7.611125781952750025 ) ) ;
#30967=CARTESIAN_POINT ( 'NONE',  ( 153.3544108199959908, 265.0293642254135307, -17.49105661178601423 ) ) ;
#30969=CARTESIAN_POINT ( 'NONE',  ( 201.1945576647943312, 267.4339689888946054, -5.629323321537795799 ) ) ;
#30972=CARTESIAN_POINT ( 'NONE',  ( 147.6121581866023007, 274.9752375363476631, 8.700660424766859080 ) ) ;
#30974=ORIENTED_EDGE ( 'NONE', *, *, #30909, .F. ) ;
#30975=CARTESIAN_POINT ( 'NONE',  ( 157.2168982216852555, 258.3393398020932636, 18.09635675623264106 ) ) ;
#30976=B_SPLINE_CURVE_WITH_KNOTS ( 'NONE', 3,
 ( #8440, #60616, #46935, #23120, #37823, #15515, #55023, #86004, #47427, #39309, #38822, #99655, #30241, #38323 ),
 .UNSPECIFIED., .F., .F.,
 ( 4, 2, 2, 2, 2, 2, 4 ),
 ( 2.792110050598545343E-17, 0.0004826660903813697365, 0.0007239991355720011264, 0.0009653321807626326790, 0.001206665225953264123, 0.001447998271143895567, 0.001930664361525126363 ),
 .UNSPECIFIED. ) ;
#30977=CARTESIAN_POINT ( 'NONE',  ( 158.2129804214947058, 265.2348010298870236, 17.61986633405762603 ) ) ;
#30980=CARTESIAN_POINT ( 'NONE',  ( 149.4539134692060145, 271.7852238117696402, 12.95627816374690688 ) ) ;
#30983=B_SPLINE_CURVE_WITH_KNOTS ( 'NONE', 3,
 ( #18861, #64449, #95408, #26458, #56835, #87820, #88308 ),
 .UNSPECIFIED., .F., .F.,
 ( 4, 3, 4 ),
 ( 0.000000000000000000, 0.001498044985889790620, 0.001795433657425995512 ),
 .UNSPECIFIED. ) ;
#30985=CARTESIAN_POINT ( 'NONE',  ( 143.0969038086192597, 260.4263049900483225, -7.951529393128359935 ) ) ;
#30990=ORIENTED_EDGE ( 'NONE', *, *, #43523, .T. ) ;
#30991=CARTESIAN_POINT ( 'NONE',  ( 190.6384534477846557, 299.7466497614934156, 5.268453997566757252 ) ) ;
#30994=CARTESIAN_POINT ( 'NONE',  ( 148.9275518150011806, 272.6969089400084272, 12.34519124974546500 ) ) ;
#30995=CARTESIAN_POINT ( 'NONE',  ( 173.8450891585409011, 276.9012038130899214, -15.64775106871585031 ) ) ;
#30996=FACE_OUTER_BOUND ( 'NONE', #44569, .T. ) ;
#30997=CARTESIAN_POINT ( 'NONE',  ( 146.9370072200009645, 276.1446333132804511, -3.799807221059707363 ) ) ;
#30998=DIRECTION ( 'NONE',  ( -0.8660254037844387076, -0.4999999999999998890, -0.000000000000000000 ) ) ;
#31002=CARTESIAN_POINT ( 'NONE',  ( 154.7926630903251350, 264.2811358641517927, -17.33176059627759358 ) ) ;
#31004=CARTESIAN_POINT ( 'NONE',  ( 106.3178956768819319, 226.0643266524159856, -9.188101187500093303 ) ) ;
#31006=CARTESIAN_POINT ( 'NONE',  ( 191.7187529716733820, 298.5803744197520473, -8.487597704798396592 ) ) ;
#31009=CARTESIAN_POINT ( 'NONE',  ( 203.5555343017997529, 278.0784677578903370, -15.71723084798551362 ) ) ;
#31010=CARTESIAN_POINT ( 'NONE',  ( 181.2388288815258477, 283.4805243373127723, -15.08248537652952059 ) ) ;
#31011=CARTESIAN_POINT ( 'NONE',  ( 147.9595119098395060, 274.3736032395026427, -9.979693660141967015 ) ) ;
#31012=CARTESIAN_POINT ( 'NONE',  ( 165.4948777162425131, 284.0002391267994994, -8.475767388502914557 ) ) ;
#31014=CARTESIAN_POINT ( 'NONE',  ( 207.6837091943624785, 270.9282591014416539, -1.156610046911421552 ) ) ;
#31016=CARTESIAN_POINT ( 'NONE',  ( 54.13067045125697518, 195.3927522451418213, 10.00000000000009592 ) ) ;
#31017=CARTESIAN_POINT ( 'NONE',  ( 121.2293367285889616, 249.9869531367911293, 4.594050593750046652 ) ) ;
#31019=DIRECTION ( 'NONE',  ( 0.4999999999999998890, -0.8660254037844385966, 0.000000000000000000 ) ) ;
#31020=CARTESIAN_POINT ( 'NONE',  ( 157.3988263959001870, 258.0242309610243865, 16.72376558639979294 ) ) ;
#31022=CARTESIAN_POINT ( 'NONE',  ( 49.51212862133765213, 190.2048013555409796, 4.594050593750051981 ) ) ;
#31025=B_SPLINE_CURVE_WITH_KNOTS ( 'NONE', 3,
 ( #82894, #5852, #97580, #29158, #89993, #75266, #11971, #58057, #4357, #20569, #43841, #74780, #3865, #80918, #22041, #30137, #37239, #31121, #84378, #6352, #7332, #68137, #14925, #15930, #52936, #54409, #7843, #46313, #14451, #92964, #91476, #52437, #83889, #45332, #76265, #92474, #62012, #61021, #99554, #31616, #91991, #239, #6837, #77237, #99065, #46835, #23516, #37723, #22543, #90993 ),
 .UNSPECIFIED., .F., .F.,
 ( 4, 2, 2, 2, 2, 2, 2, 2, 2, 2, 2, 2, 2, 2, 2, 2, 2, 2, 2, 2, 2, 2, 2, 2, 4 ),
 ( 0.0007513920313679374680, 0.0009574642477403361596, 0.001060500355926582722, 0.001163536464112829068, 0.001266572572299075414, 0.001369608680485322194, 0.001575680896857799057, 0.001987825329602752999, 0.002399969762347706724, 0.003224258627837614175, 0.004048547493327522492, 0.004872836358817429943, 0.005284980791562383234, 0.005491053007934861181, 0.005594089116121140487, 0.005645607170214243277, 0.005697125224307346067, 0.005800161332493488330, 0.005903197440679630592, 0.006109269657051875219, 0.006521414089796225694, 0.006727486306168400064, 0.006933558522540574434, 0.007139630738912749672, 0.007345702955284924042 ),
 .UNSPECIFIED. ) ;
#31026=ORIENTED_EDGE ( 'NONE', *, *, #4992, .T. ) ;
#31029=B_SPLINE_SURFACE_WITH_KNOTS ( 'NONE', 3, 1, ( 
 ( #22166, #29765 ),
 ( #30261, #14575 ),
 ( #65888, #29277 ),
 ( #58288, #27409 ),
 ( #89264, #35491 ),
 ( #34985, #6959 ),
 ( #45451, #73509 ),
 ( #53551, #88761 ),
 ( #65397, #50196 ),
 ( #75896, #19814 ),
 ( #81148, #11715 ),
 ( #98696, #99678 ),
 ( #53058, #4093 ),
 ( #74012, #14069 ),
 ( #37846, #61147 ),
 ( #92119, #96842 ),
 ( #22671, #84016 ),
 ( #11225, #6474 ),
 ( #60145, #50682 ),
 ( #42576, #81637 ),
 ( #43069, #83507 ),
 ( #37353, #44955 ),
 ( #4598, #73024 ),
 ( #91107, #21673 ),
 ( #94595, #39334 ),
 ( #15047, #45938 ),
 ( #92598, #76856 ),
 ( #78883, #93083 ),
 ( #100183, #32254 ),
 ( #85511, #54038 ),
 ( #31249, #30768 ),
 ( #62136, #23639 ),
 ( #16553, #84993 ),
 ( #54530, #61649 ) ),
 .UNSPECIFIED., .T., .F., .F.,
 ( 4, 2, 2, 2, 2, 2, 2, 2, 2, 2, 2, 2, 2, 2, 2, 2, 4 ),
 ( 2, 2 ),
 ( 0.000000000000000000, 0.06250000000000000000, 0.1250000000000000000, 0.1875000000000000000, 0.2500000000000000000, 0.3125000000000000000, 0.3750000000000000000, 0.4375000000000000000, 0.5000000000000000000, 0.5625000000000000000, 0.6250000000000000000, 0.6875000000000000000, 0.7500000000000000000, 0.8125000000000000000, 0.8750000000000000000, 0.9375000000000000000, 1.000000000000000000 ),
 ( 0.000000000000000000, 1.000000000000000000 ),
 .UNSPECIFIED. ) ;
#31031=CARTESIAN_POINT ( 'NONE',  ( 147.5813496936708020, 275.0285994114094592, 4.516581957185684004 ) ) ;
#31033=EDGE_CURVE ( 'NONE', #34720, #3513, #77482, .T. ) ;
#31034=CARTESIAN_POINT ( 'NONE',  ( 198.2505066714982149, 285.2670451491296149, 0.000000000000000000 ) ) ;
#31035=CARTESIAN_POINT ( 'NONE',  ( 157.3948608031964511, 270.9082508132711382, -14.72219542052569885 ) ) ;
#31036=CARTESIAN_POINT ( 'NONE',  ( 114.6081111488702931, 223.6427522451417644, 1.119607411625061291E-15 ) ) ;
#31038=ORIENTED_EDGE ( 'NONE', *, *, #97788, .F. ) ;
#31040=CARTESIAN_POINT ( 'NONE',  ( 202.8787628851569593, 279.2506702366259788, 17.01435431865322556 ) ) ;
#31042=CARTESIAN_POINT ( 'NONE',  ( 32.43492986863949312, 189.5333772461660544, 9.188101187500095079 ) ) ;
#31045=CARTESIAN_POINT ( 'NONE',  ( 39.49844957003031709, 183.6115022471902023, -5.000000000000041744 ) ) ;
#31047=CARTESIAN_POINT ( 'NONE',  ( 177.3741080081426844, 288.0714115368494959, 10.68489811804565726 ) ) ;
#31048=CARTESIAN_POINT ( 'NONE',  ( 56.16917826928300883, 212.4244531367911577, -4.594050593750046652 ) ) ;
#31049=CARTESIAN_POINT ( 'NONE',  ( 161.2799361541916028, 251.3019516699124836, 14.40628917569557110 ) ) ;
#31053=CARTESIAN_POINT ( 'NONE',  ( 33.86928444543146810, 180.3615022471902023, 5.000000000000051514 ) ) ;
#31054=CARTESIAN_POINT ( 'NONE',  ( 163.7183543885751078, 247.0784873978576854, -6.786164904910574336 ) ) ;
#31055=CARTESIAN_POINT ( 'NONE',  ( 0.1486806056246424423, 161.7048013555410080, 4.594050593750051981 ) ) ;
#31057=CARTESIAN_POINT ( 'NONE',  ( 167.6362108137774669, 262.4817980704067395, -16.57735221840392725 ) ) ;
#31058=CARTESIAN_POINT ( 'NONE',  ( 185.3427542040608387, 260.2457244105148675, 7.085506836970698608 ) ) ;
#31059=CARTESIAN_POINT ( 'NONE',  ( 164.9103019330012216, 245.0139736909548560, 2.841678961959298810 ) ) ;
#31063=CARTESIAN_POINT ( 'NONE',  ( 187.4171132689631634, 261.5282790321019206, -9.397869408254909018 ) ) ;
#31068=CARTESIAN_POINT ( 'NONE',  ( 159.8912210074807945, 253.7072768612558775, 15.17831030338107112 ) ) ;
#31069=CARTESIAN_POINT ( 'NONE',  ( 205.2121761402296443, 275.2090799237855094, -14.05269615702442465 ) ) ;
#31070=EDGE_CURVE ( 'NONE', #52312, #54608, #66697, .T. ) ;
#31072=CARTESIAN_POINT ( 'NONE',  ( 153.2712411579340426, 265.1734183057532732, 16.26687330118495467 ) ) ;
#31075=CARTESIAN_POINT ( 'NONE',  ( 207.6067494229581314, 271.0615573356529353, -1.924113146155245868 ) ) ;
#31079=CARTESIAN_POINT ( 'NONE',  ( 169.3716973832724761, 248.0780012208689982, 1.470315277928950781 ) ) ;
#31082=ADVANCED_FACE ( 'NONE', ( #1291 ), #98940, .T. ) ;
#31084=ORIENTED_EDGE ( 'NONE', *, *, #44110, .F. ) ;
#31088=CARTESIAN_POINT ( 'NONE',  ( 184.2795938587219382, 282.7716313920612379, -17.16491284908262216 ) ) ;
#31091=ORIENTED_EDGE ( 'NONE', *, *, #73514, .T. ) ;
#31092=CARTESIAN_POINT ( 'NONE',  ( 200.1103929410127762, 284.0456276340304953, 17.67835211026828901 ) ) ;
#31093=B_SPLINE_CURVE_WITH_KNOTS ( 'NONE', 3,
 ( #38995, #83661, #45111, #61797 ),
 .UNSPECIFIED., .F., .F.,
 ( 4, 4 ),
 ( 2.098622547487930532E-15, 0.004943534199230881221 ),
 .UNSPECIFIED. ) ;
#31095=CARTESIAN_POINT ( 'NONE',  ( 141.5270674498366077, 242.5177522451417929, 5.000000000000051514 ) ) ;
#31096=ORIENTED_EDGE ( 'NONE', *, *, #66550, .F. ) ;
#31097=ORIENTED_EDGE ( 'NONE', *, *, #13650, .F. ) ;
#31100=ORIENTED_EDGE ( 'NONE', *, *, #97454, .F. ) ;
#31103=CARTESIAN_POINT ( 'NONE',  ( 164.3545367017254364, 245.9765873086048487, -5.942639963102972267 ) ) ;
#31105=CARTESIAN_POINT ( 'NONE',  ( 165.6431331270639760, 271.4262817979627584, 17.22401055456362684 ) ) ;
#31106=CARTESIAN_POINT ( 'NONE',  ( 167.0646487823995585, 282.1497282158676398, 11.94391941918240185 ) ) ;
#31107=CARTESIAN_POINT ( 'NONE',  ( 194.8067605455144076, 293.2317884077015151, -16.00245909155922774 ) ) ;
#31109=CARTESIAN_POINT ( 'NONE',  ( 198.2505066714982149, 285.2670451491296149, 0.000000000000000000 ) ) ;
#31111=CARTESIAN_POINT ( 'NONE',  ( 167.0648401017704430, 247.0325385398216440, 1.942792713102396762 ) ) ;
#31113=CARTESIAN_POINT ( 'NONE',  ( -22.42236680055709641, 157.8615022471902591, 0.000000000000000000 ) ) ;
#31116=ORIENTED_EDGE ( 'NONE', *, *, #50862, .F. ) ;
#31117=CARTESIAN_POINT ( 'NONE',  ( 168.3105211781452795, 256.9082286493703009, -14.73656021653829384 ) ) ;
#31118=CARTESIAN_POINT ( 'NONE',  ( 159.2102594322688844, 254.8867369075254885, -16.13039487917589199 ) ) ;
#31119=CARTESIAN_POINT ( 'NONE',  ( -17.42236680055705023, 149.2012482093457777, 0.000000000000000000 ) ) ;
#31121=CARTESIAN_POINT ( 'NONE',  ( 168.9042932422607919, 253.9312568212353085, 11.43877001047246189 ) ) ;
#31122=CARTESIAN_POINT ( 'NONE',  ( 161.0249958932952552, 283.1118547020287224, 2.115121692784775576 ) ) ;
#31123=CARTESIAN_POINT ( 'NONE',  ( 193.9307011644069973, 294.7491677662272878, -14.33994679320232990 ) ) ;
#31124=DIRECTION ( 'NONE',  ( 0.4999999999999992784, -0.8660254037844390407, 0.000000000000000000 ) ) ;
#31126=CARTESIAN_POINT ( 'NONE',  ( 8.159155267032986103, 175.5177522451418781, -10.00000000000009592 ) ) ;
#31127=CARTESIAN_POINT ( 'NONE',  ( 82.77265646360999085, 218.5958772461660544, -9.188101187500095079 ) ) ;
#31128=CARTESIAN_POINT ( 'NONE',  ( 196.0257901730189474, 269.4247523037524275, -10.81113306140426999 ) ) ;
#31130=CARTESIAN_POINT ( 'NONE',  ( 163.8240215689833690, 246.8954664726980184, -8.949281535847481095 ) ) ;
#31132=CARTESIAN_POINT ( 'NONE',  ( -1.313257906909115480, 179.2369531367911293, -4.594050593750048428 ) ) ;
#31133=CARTESIAN_POINT ( 'NONE',  ( -22.42236680055709641, 157.8615022471902591, 0.000000000000000000 ) ) ;
#31134=ADVANCED_FACE ( 'NONE', ( #13341 ), #56155, .F. ) ;
#31135=CARTESIAN_POINT ( 'NONE',  ( 200.1782072557437857, 283.9281697954355650, 18.05177561285849208 ) ) ;
#31139=ADVANCED_FACE ( 'NONE', ( #86271 ), #84450, .F. ) ;
#31141=CARTESIAN_POINT ( 'NONE',  ( 157.6036818288543486, 257.6694109429415107, -16.73826488331764395 ) ) ;
#31142=CARTESIAN_POINT ( 'NONE',  ( 162.8917261183091227, 248.5102495609312143, -11.80346065365840680 ) ) ;
#31143=CARTESIAN_POINT ( 'NONE',  ( 106.8138825148102740, 239.1427522451419065, -10.00000000000009592 ) ) ;
#31144=CARTESIAN_POINT ( 'NONE',  ( 176.8408657501080654, 282.3818803302173137, -15.82416175011198689 ) ) ;
#31145=CARTESIAN_POINT ( 'NONE',  ( 18.65997361151702449, 172.3923013555409796, 4.594050593750050204 ) ) ;
#31146=CARTESIAN_POINT ( 'NONE',  ( 130.4855038751826726, 236.9548013555409796, -4.594050593750042211 ) ) ;
#31147=CARTESIAN_POINT ( 'NONE',  ( 183.5021136046642596, 257.1513431580297038, -3.213728371295248465 ) ) ;
#31155=CARTESIAN_POINT ( 'NONE',  ( 195.9713281756800427, 291.2146981034049418, 17.52210387885178022 ) ) ;
#31156=CARTESIAN_POINT ( 'NONE',  ( 194.4165969972361552, 293.9075714965812267, 14.23342188338008718 ) ) ;
#31157=CARTESIAN_POINT ( 'NONE',  ( 207.2167723318516153, 271.7370174712370954, -6.606038862010207957 ) ) ;
#31159=CARTESIAN_POINT ( 'NONE',  ( 148.1829914015846157, 273.9865254053503349, -9.304102644963160529 ) ) ;
#31162=CARTESIAN_POINT ( 'NONE',  ( 187.1736806720859647, 299.3961564376974138, 1.305121339064515551 ) ) ;
#31163=CARTESIAN_POINT ( 'NONE',  ( 168.4104533980780900, 278.9328176548356168, 14.99313165221212252 ) ) ;
#31164=CARTESIAN_POINT ( 'NONE',  ( 192.5170171266991304, 265.2796291261559531, 8.180105463325700654 ) ) ;
#31166=CARTESIAN_POINT ( 'NONE',  ( 189.8314329296643450, 301.8493086226544619, -0.8085564604676659384 ) ) ;
#31167=CARTESIAN_POINT ( 'NONE',  ( 180.8012419246406353, 266.7401795635341273, -14.70472759341407709 ) ) ;
#31169=ORIENTED_EDGE ( 'NONE', *, *, #99358, .F. ) ;
#31170=CARTESIAN_POINT ( 'NONE',  ( 151.9556655013304862, 274.5278385319554104, -11.22762646749768756 ) ) ;
#31171=CARTESIAN_POINT ( 'NONE',  ( 185.2582332437331445, 272.4808076714297727, 17.23139995252659773 ) ) ;
#31172=CARTESIAN_POINT ( 'NONE',  ( 111.8384605302426991, 241.5024278399160664, -9.188101187500093303 ) ) ;
#31174=CARTESIAN_POINT ( 'NONE',  ( 151.0778907302193943, 268.9724126853576536, 15.84769371787143832 ) ) ;
#31178=CARTESIAN_POINT ( 'NONE',  ( 191.6230175057792451, 276.9742630895800630, 16.77582784212352252 ) ) ;
#31179=CARTESIAN_POINT ( 'NONE',  ( 196.7941661740290158, 289.7895008838662534, 17.93043241841150959 ) ) ;
#31180=DIRECTION ( 'NONE',  ( 0.4999999999999992784, -0.8660254037844390407, 0.000000000000000000 ) ) ;
#31182=CARTESIAN_POINT ( 'NONE',  ( 123.3201800421238090, 253.5530062829863311, -4.648177544792955347E-16 ) ) ;
#31185=CARTESIAN_POINT ( 'NONE',  ( 163.7565952011062507, 255.1539107282341092, -15.17543724475343048 ) ) ;
#31188=CARTESIAN_POINT ( 'NONE',  ( 200.1795251174064560, 269.7820628003561296, 8.922369943785961155 ) ) ;
#31189=CARTESIAN_POINT ( 'NONE',  ( 149.4908848037268001, 271.7211875819559737, -12.92288068979413573 ) ) ;
#31195=CARTESIAN_POINT ( 'NONE',  ( 181.9559929377375056, 291.6402902057536721, -11.43735378946719372 ) ) ;
#31198=CARTESIAN_POINT ( 'NONE',  ( 153.1745822862813498, 265.3408363824576668, 16.18092354043443493 ) ) ;
#31200=VERTEX_POINT ( 'NONE', #14204 ) ;
#31204=CARTESIAN_POINT ( 'NONE',  ( 164.3996301846870267, 247.3020492865104529, 7.248807534621905191 ) ) ;
#31205=B_SPLINE_CURVE_WITH_KNOTS ( 'NONE', 3,
 ( #32267, #56048, #55550, #86534, #41358, #17064, #48480, #2907, #9483, #40354, #79422, #62150, #71291, #9988, #81416, #20582, #81910, #51463, #73287, #58556, #58072, #28166, #34275, #89054, #73781, #43854, #4370, #80934, #3879, #35268, #19604, #82430, #12489, #65171, #43356, #27687, #50464, #11987, #57561, #34763 ),
 .UNSPECIFIED., .F., .F.,
 ( 4, 2, 2, 2, 2, 2, 2, 2, 2, 2, 2, 2, 2, 2, 2, 2, 2, 2, 2, 4 ),
 ( 0.002905659672395857849, 0.003105746374355510941, 0.003305833076315163599, 0.003405876427294977568, 0.003505919778274790670, 0.003605963129254604639, 0.003706006480234417741, 0.003906093182194044378, 0.004106179884153671016, 0.004506353288073101232, 0.005306700095912135137, 0.006107046903751169042, 0.007707740519429236853, 0.007907827221389052141, 0.007957848896878968667, 0.008007870572368885193, 0.008107913923348666202, 0.008508087327267866568, 0.008908260731187066933, 0.009308434135106267299 ),
 .UNSPECIFIED. ) ;
#31208=VERTEX_POINT ( 'NONE', #97827 ) ;
#31210=EDGE_CURVE ( 'NONE', #45557, #29501, #74464, .T. ) ;
#31211=CARTESIAN_POINT ( 'NONE',  ( 205.9755752649865315, 273.8868338532529378, 12.31646113325132674 ) ) ;
#31214=CARTESIAN_POINT ( 'NONE',  ( 111.2161783173811500, 245.0177522451419065, 5.000000000000046185 ) ) ;
#31217=EDGE_CURVE ( 'NONE', #86029, #20189, #4993, .T. ) ;
#31219=CARTESIAN_POINT ( 'NONE',  ( 195.8729049011480470, 290.8691304563884614, 15.97541058376903855 ) ) ;
#31220=VERTEX_POINT ( 'NONE', #24782 ) ;
#31223=CARTESIAN_POINT ( 'NONE',  ( 170.1342846507165518, 269.5121279834121992, 16.76028639438306911 ) ) ;
#31224=( BOUNDED_CURVE ( )  B_SPLINE_CURVE ( 2, ( #21547, #22029, #15409, #83376, #84372, #44327, #52929, #90986, #76732 ),
 .UNSPECIFIED., .F., .T. ) 
 B_SPLINE_CURVE_WITH_KNOTS ( ( 3, 2, 2, 2, 3 ),
 ( 0.1653225806451612823, 0.1666666666666666574, 0.1693548387096774077, 0.1720430107526881858, 0.1733870967741935609 ),
 .UNSPECIFIED. ) 
 CURVE ( )  GEOMETRIC_REPRESENTATION_ITEM ( )  RATIONAL_B_SPLINE_CURVE ( ( 0.9330127018922194093, 0.9330127018922194093, 1.000000000000000000, 0.8660254037844387076, 1.000000000000000000, 0.8660254037844387076, 1.000000000000000000, 0.9330127018922194093, 0.9330127018922194093 ) ) 
 REPRESENTATION_ITEM ( '' )  );
#31225=EDGE_LOOP ( 'NONE', ( #62721, #49320, #8926, #4875, #9836 ) ) ;
#31226=CARTESIAN_POINT ( 'NONE',  ( 164.5519675908388422, 246.2604196026755687, 2.628616105114974122 ) ) ;
#31227=CARTESIAN_POINT ( 'NONE',  ( 206.7182525013508041, 272.6004791462452204, -10.42767927275168205 ) ) ;
#31229=CARTESIAN_POINT ( 'NONE',  ( 197.7385643933960750, 285.3845219642180382, -17.06910720252511027 ) ) ;
#31231=CARTESIAN_POINT ( 'NONE',  ( 167.7191586515327231, 249.2659981153678359, -5.464437866973313795 ) ) ;
#31233=CARTESIAN_POINT ( 'NONE',  ( 186.1263547150109900, 286.8862237501084564, -16.18252752151998308 ) ) ;
#31234=CARTESIAN_POINT ( 'NONE',  ( 137.8467198073504107, 241.2048013555409796, 4.594050593750051981 ) ) ;
#31235=CARTESIAN_POINT ( 'NONE',  ( 186.7214803242468122, 262.7147121518711401, -9.981163800224575056 ) ) ;
#31237=CARTESIAN_POINT ( 'NONE',  ( 179.9513890298225078, 291.5425348745724818, -10.01420112412196772 ) ) ;
#31238=ORIENTED_EDGE ( 'NONE', *, *, #95684, .T. ) ;
#31239=AXIS2_PLACEMENT_3D ( 'NONE', #25171, #63676, #17578 ) ;
#31241=CARTESIAN_POINT ( 'NONE',  ( 178.5998364833490939, 254.7693240753903297, 1.328249545842869139 ) ) ;
#31243=CARTESIAN_POINT ( 'NONE',  ( 171.1538413615039360, 287.7943309346417209, -4.649139628941194147 ) ) ;
#31244=CARTESIAN_POINT ( 'NONE',  ( 146.6671492545637534, 276.6120410202449307, 3.340372238077111255 ) ) ;
#31245=FACE_OUTER_BOUND ( 'NONE', #44907, .T. ) ;
#31246=CARTESIAN_POINT ( 'NONE',  ( 201.0844796915553161, 282.3584598911111812, -16.59562674965125950 ) ) ;
#31247=CARTESIAN_POINT ( 'NONE',  ( 177.2389597949545248, 288.8581041804060874, -9.261545317147978906 ) ) ;
#31248=EDGE_LOOP ( 'NONE', ( #38566, #23735, #34834, #39617, #89275 ) ) ;
#31249=CARTESIAN_POINT ( 'NONE',  ( 194.7900099568305166, 293.2608012783592812, 16.38313017464638932 ) ) ;
#31250=CARTESIAN_POINT ( 'NONE',  ( 164.8624568345837531, 246.3845970976477417, 4.092954484416948979 ) ) ;
#31252=CARTESIAN_POINT ( 'NONE',  ( 194.2223991963907963, 294.2439319543634610, -14.97294938100067441 ) ) ;
#31253=CARTESIAN_POINT ( 'NONE',  ( 167.9496373820661290, 248.6204696539478789, -6.517719931589019744 ) ) ;
#31255=CARTESIAN_POINT ( 'NONE',  ( 188.1709242600894925, 266.2605123816134665, -11.82625739451866131 ) ) ;
#31256=CIRCLE ( 'NONE', #37688, 17.82106496071138935 ) ;
#31257=CARTESIAN_POINT ( 'NONE',  ( 156.9511562921923939, 276.6036013291395079, 10.24360920285362653 ) ) ;
#31258=CARTESIAN_POINT ( 'NONE',  ( 193.1664498718385232, 262.6697469753432870, 4.718537006446267945 ) ) ;
#31259=CARTESIAN_POINT ( 'NONE',  ( 190.6893905452545823, 300.3632824417117604, 3.294993852933539191 ) ) ;
#31261=CARTESIAN_POINT ( 'NONE',  ( 163.3456309634439663, 283.9452505866142928, -7.113541931128232854 ) ) ;
#31262=CARTESIAN_POINT ( 'NONE',  ( 156.8144410367226840, 280.3425935702447305, 5.941698292227072464 ) ) ;
#31263=CARTESIAN_POINT ( 'NONE',  ( 160.4258337542706272, 283.3657075219940680, -4.450354451773817388 ) ) ;
#31264=ORIENTED_EDGE ( 'NONE', *, *, #18828, .F. ) ;
#31265=CARTESIAN_POINT ( 'NONE',  ( 190.5541309856500050, 300.5975588711562523, -4.167177996129430184 ) ) ;
#31266=B_SPLINE_SURFACE_WITH_KNOTS ( 'NONE', 3, 1, ( 
 ( #22710, #15579 ),
 ( #62682, #39374 ),
 ( #53588, #70807 ),
 ( #47001, #54572 ),
 ( #402, #86069 ),
 ( #30303, #7491 ),
 ( #61686, #23680 ),
 ( #61189, #100221 ),
 ( #84543, #15086 ),
 ( #92638, #85556 ),
 ( #31780, #16595 ),
 ( #14611, #46482 ),
 ( #68790, #70289 ),
 ( #93635, #8016 ),
 ( #38384, #45974 ),
 ( #76891, #24202 ),
 ( #47491, #31291 ),
 ( #78416, #23187 ),
 ( #69297, #30806 ),
 ( #8998, #85033 ),
 ( #54080, #91635 ),
 ( #22203, #93131 ),
 ( #38889, #69792 ),
 ( #16097, #49007 ),
 ( #25714, #88560 ),
 ( #96141, #17600 ),
 ( #3424, #26700 ),
 ( #32791, #72327 ),
 ( #19125, #42379 ),
 ( #71317, #34299 ),
 ( #11021, #2417 ),
 ( #57584, #33819 ),
 ( #3903, #11521 ),
 ( #1910, #17091 ) ),
 .UNSPECIFIED., .T., .F., .F.,
 ( 4, 2, 2, 2, 2, 2, 2, 2, 2, 2, 2, 2, 2, 2, 2, 2, 4 ),
 ( 2, 2 ),
 ( 0.000000000000000000, 0.06250000000000000000, 0.1250000000000000000, 0.1875000000000000000, 0.2500000000000000000, 0.3125000000000000000, 0.3750000000000000000, 0.4375000000000000000, 0.5000000000000000000, 0.5625000000000000000, 0.6250000000000000000, 0.6875000000000000000, 0.7500000000000000000, 0.8125000000000000000, 0.8750000000000000000, 0.9375000000000000000, 1.000000000000000000 ),
 ( 0.000000000000000000, 1.000000000000000000 ),
 .UNSPECIFIED. ) ;
#31268=CARTESIAN_POINT ( 'NONE',  ( 186.7629878510455512, 262.7841317527147567, -8.999996197527845965 ) ) ;
#31271=CARTESIAN_POINT ( 'NONE',  ( 184.7908904391260592, 296.8361954622408234, -4.367935385452441643 ) ) ;
#31272=CARTESIAN_POINT ( 'NONE',  ( 204.3073682595353091, 276.3816438339565593, 13.21529881594027422 ) ) ;
#31273=CARTESIAN_POINT ( 'NONE',  ( 27.19136022205111658, 198.0530062829863311, -4.648177544792955347E-16 ) ) ;
#31274=CARTESIAN_POINT ( 'NONE',  ( 155.0197698005585494, 262.1448778582381465, 18.42918111182112284 ) ) ;
#31275=CARTESIAN_POINT ( 'NONE',  ( 191.2333131753503892, 283.1309561651182776, -16.66095403317861923 ) ) ;
#31277=CARTESIAN_POINT ( 'NONE',  ( 82.61045024828291616, 212.3768266524159856, -9.188101187500091527 ) ) ;
#31279=CARTESIAN_POINT ( 'NONE',  ( 147.1603453755519695, 275.7578002805973370, -5.230822882238410187 ) ) ;
#31281=EDGE_CURVE ( 'NONE', #34720, #97734, #6234, .T. ) ;
#31282=CARTESIAN_POINT ( 'NONE',  ( 203.0026270830780675, 279.0361311525880978, -16.61345826058821373 ) ) ;
#31288=CARTESIAN_POINT ( 'NONE',  ( 207.6777884554021512, 270.9385141221390541, 6.417167147861016829 ) ) ;
#31290=CARTESIAN_POINT ( 'NONE',  ( 166.0155133103885703, 249.5026163374074599, -9.152316162654148712 ) ) ;
#31291=CARTESIAN_POINT ( 'NONE',  ( 163.9864329842212953, 246.6141616497770030, -4.773827767272011080 ) ) ;
#31292=CARTESIAN_POINT ( 'NONE',  ( 196.1573359623355088, 290.8925231663144473, 17.55680092534192482 ) ) ;
#31294=ADVANCED_FACE ( 'NONE', ( #95243 ), #85281, .F. ) ;
#31296=CARTESIAN_POINT ( 'NONE',  ( 39.95835201613431309, 200.0024278399160949, 9.188101187500095079 ) ) ;
#31297=CARTESIAN_POINT ( 'NONE',  ( 55.05949644674294774, 214.8464784336661637, 1.353441290958777327E-15 ) ) ;
#31298=CARTESIAN_POINT ( 'NONE',  ( 57.11559101558731300, 215.3297689869269220, -2.679491924311252493 ) ) ;
#31300=CARTESIAN_POINT ( 'NONE',  ( 163.6320872669321602, 257.9766140902174243, 15.55573320749642896 ) ) ;
#31301=CARTESIAN_POINT ( 'NONE',  ( -7.699934936221591641, 156.3615022471902023, 5.000000000000051514 ) ) ;
#31303=CARTESIAN_POINT ( 'NONE',  ( 196.4096156673327869, 269.1445197880362343, -10.54851971483136630 ) ) ;
#31308=CARTESIAN_POINT ( 'NONE',  ( 70.72975101405640430, 202.4548013555409796, -4.594050593750042211 ) ) ;
#31310=CARTESIAN_POINT ( 'NONE',  ( 154.8579861482817535, 262.4250953638155011, -17.69813260923097786 ) ) ;
#31311=CARTESIAN_POINT ( 'NONE',  ( 198.3449891235413531, 287.1033967417670283, 16.95540786497457120 ) ) ;
#31313=CARTESIAN_POINT ( 'NONE',  ( 153.6005803596509054, 264.6029860754553056, 18.07864614867099462 ) ) ;
#31316=CARTESIAN_POINT ( 'NONE',  ( 103.9451733683222443, 237.4865022471903160, 10.00000000000009237 ) ) ;
#31317=CARTESIAN_POINT ( 'NONE',  ( 18.62362889609498851, 174.8927522451418213, -10.00000000000009237 ) ) ;
#31318=EDGE_CURVE ( 'NONE', #57035, #42320, #85346, .T. ) ;
#31319=CARTESIAN_POINT ( 'NONE',  ( 164.2723164851102808, 246.1189969011916503, -1.993789335506892302 ) ) ;
#31325=CARTESIAN_POINT ( 'NONE',  ( 206.8775514429320026, 272.3245652858344670, -9.838455694836268250 ) ) ;
#31326=CARTESIAN_POINT ( 'NONE',  ( 186.8361490887116645, 276.6032954149434886, -17.09107860825236713 ) ) ;
#31329=CARTESIAN_POINT ( 'NONE',  ( 173.4028078701637696, 251.4564948467337047, 0.3090336303432728027 ) ) ;
#31334=CARTESIAN_POINT ( 'NONE',  ( 148.1632261683078013, 274.0207597936089883, -7.853210555358286271 ) ) ;
#31335=B_SPLINE_CURVE_WITH_KNOTS ( 'NONE', 3,
 ( #80917, #3863, #11488, #19083 ),
 .UNSPECIFIED., .F., .F.,
 ( 4, 4 ),
 ( 0.007733555512259023858, 0.01590650797624234419 ),
 .UNSPECIFIED. ) ;
#31337=ORIENTED_EDGE ( 'NONE', *, *, #48446, .T. ) ;
#31340=DIRECTION ( 'NONE',  ( -0.8660254037844387076, -0.4999999999999998890, -0.000000000000000000 ) ) ;
#31342=EDGE_CURVE ( 'NONE', #71334, #8428, #35674, .T. ) ;
#31344=CARTESIAN_POINT ( 'NONE',  ( 130.0937757410490576, 257.4637435831425023, 2.679491924311251605 ) ) ;
#31345=CARTESIAN_POINT ( 'NONE',  ( -9.233521592304517966, 172.1427522451419065, 10.00000000000009415 ) ) ;
#31347=CARTESIAN_POINT ( 'NONE',  ( 170.8837800509748490, 284.6422579550419982, 10.91543698957328701 ) ) ;
#31351=CARTESIAN_POINT ( 'NONE',  ( 204.2799274532736433, 276.8237820148827950, 13.55359442435934803 ) ) ;
#31352=CARTESIAN_POINT ( 'NONE',  ( 185.4129985849131401, 292.6123411851212381, -10.72120707279806417 ) ) ;
#31353=CARTESIAN_POINT ( 'NONE',  ( 204.7519188734507622, 276.0062688943993408, -12.76027478560537531 ) ) ;
#31354=CARTESIAN_POINT ( 'NONE',  ( 131.5133883985292016, 255.9244531367911293, -4.594050593750046652 ) ) ;
#31355=CARTESIAN_POINT ( 'NONE',  ( 203.2786752506974040, 268.5145164534344531, 2.480206815910183771 ) ) ;
#31356=CARTESIAN_POINT ( 'NONE',  ( 182.0609731580854316, 260.3214751816357193, 9.357376519101284984 ) ) ;
#31357=CARTESIAN_POINT ( 'NONE',  ( 77.03558525930309031, 203.0327760586659451, 1.948934522072303157E-15 ) ) ;
#31358=ORIENTED_EDGE ( 'NONE', *, *, #10713, .F. ) ;
#31359=CARTESIAN_POINT ( 'NONE',  ( 150.8359915840788688, 269.3913942967808453, 15.73449616766854575 ) ) ;
#31361=ORIENTED_EDGE ( 'NONE', *, *, #21352, .F. ) ;
#31362=CARTESIAN_POINT ( 'NONE',  ( 157.4853229503657133, 257.8744145340106684, -17.61474390190301165 ) ) ;
#31367=CARTESIAN_POINT ( 'NONE',  ( 147.3047606266276546, 275.5076657283461827, -0.02269072295920609994 ) ) ;
#31369=DIRECTION ( 'NONE',  ( -0.8660254037844387076, -0.4999999999999998890, -0.000000000000000000 ) ) ;
#31370=CARTESIAN_POINT ( 'NONE',  ( 162.4263297320084121, 249.3163397476629086, 11.18012070315788087 ) ) ;
#31371=CARTESIAN_POINT ( 'NONE',  ( 85.53328598605538957, 214.0643266524159856, -9.188101187500093303 ) ) ;
#31372=ORIENTED_EDGE ( 'NONE', *, *, #63416, .F. ) ;
#31373=EDGE_LOOP ( 'NONE', ( #27613, #15634, #36070, #36755 ) ) ;
#31374=CARTESIAN_POINT ( 'NONE',  ( 200.3152516538017380, 283.6908019351069470, -17.43933074397117977 ) ) ;
#31376=ADVANCED_FACE ( 'NONE', ( #12606 ), #60921, .F. ) ;
#31377=B_SPLINE_CURVE_WITH_KNOTS ( 'NONE', 3,
 ( #61428, #92381, #22930, #29063 ),
 .UNSPECIFIED., .F., .F.,
 ( 4, 4 ),
 ( 0.0001207921824033371633, 0.005340818303214702259 ),
 .UNSPECIFIED. ) ;
#31379=CARTESIAN_POINT ( 'NONE',  ( 165.0308887387863876, 244.8051112166122891, 1.948365933089477808 ) ) ;
#31380=CARTESIAN_POINT ( 'NONE',  ( 161.5731931013706628, 284.2088213097117091, 0.5314451569754123916 ) ) ;
#31381=CARTESIAN_POINT ( 'NONE',  ( 207.3988330342936877, 270.8564699888902396, -1.301389719878858875 ) ) ;
#31382=CARTESIAN_POINT ( 'NONE',  ( 200.0394048839106347, 267.9517317495682960, -8.074306449384252460 ) ) ;
#31383=ORIENTED_EDGE ( 'NONE', *, *, #14166, .T. ) ;
#31385=CARTESIAN_POINT ( 'NONE',  ( -27.42236680055714260, 166.5217562850347406, 1.224646799147364892E-15 ) ) ;
#31386=CARTESIAN_POINT ( 'NONE',  ( 157.2948870673828026, 280.9759411348209142, 6.053012778684776940 ) ) ;
#31387=CARTESIAN_POINT ( 'NONE',  ( 152.6740002182599767, 266.2078699576288159, -17.16212636348624088 ) ) ;
#31392=CARTESIAN_POINT ( 'NONE',  ( 196.3606441383045649, 265.7307755575039323, 4.429610383328119738 ) ) ;
#31395=CARTESIAN_POINT ( 'NONE',  ( 187.8316118507717079, 266.3710757443984107, -12.34398216243838320 ) ) ;
#31399=EDGE_CURVE ( 'NONE', #41212, #73983, #13431, .T. ) ;
#31400=CARTESIAN_POINT ( 'NONE',  ( 162.6476498368881494, 248.9330020812748785, 10.75824100428386743 ) ) ;
#31405=CARTESIAN_POINT ( 'NONE',  ( 176.1389927384235534, 285.2568696065857239, -12.19707684924138036 ) ) ;
#31410=CARTESIAN_POINT ( 'NONE',  ( 192.2417256132786179, 262.2162190891563682, 3.002089893086772765 ) ) ;
#31412=CARTESIAN_POINT ( 'NONE',  ( 5.317335864756744357, 180.0024278399160949, -9.188101187500093303 ) ) ;
#31415=DIRECTION ( 'NONE',  ( -0.8660254037844387076, -0.4999999999999998890, -0.000000000000000000 ) ) ;
#31416=CARTESIAN_POINT ( 'NONE',  ( 198.0816276881963915, 264.5915495180347534, -1.723934393811154182E-14 ) ) ;
#31418=CARTESIAN_POINT ( 'NONE',  ( 24.66750420662404508, 194.2369531367911293, -4.594050593750048428 ) ) ;
#31421=CARTESIAN_POINT ( 'NONE',  ( 147.1259762202154207, 275.8173294038533641, -0.6716460511724978710 ) ) ;
#31422=CARTESIAN_POINT ( 'NONE',  ( 140.7332108297008517, 245.3927522451417929, -10.00000000000009237 ) ) ;
#31424=CARTESIAN_POINT ( 'NONE',  ( 187.5207547097004692, 259.2518634157261204, -0.7857520814055728442 ) ) ;
#31425=CARTESIAN_POINT ( 'NONE',  ( 71.18054559181101126, 205.2365022471902023, 10.00000000000009592 ) ) ;
#31427=EDGE_CURVE ( 'NONE', #99896, #88304, #32783, .T. ) ;
#31428=CARTESIAN_POINT ( 'NONE',  ( 204.7788459716290390, 270.7538572138115569, 6.060631932661717514 ) ) ;
#31429=CARTESIAN_POINT ( 'NONE',  ( 26.91401791951368949, 186.3458772461660544, 9.188101187500095079 ) ) ;
#31431=CARTESIAN_POINT ( 'NONE',  ( 73.84283235153957037, 201.8932355074535963, -2.679491924311248496 ) ) ;
#31436=CARTESIAN_POINT ( 'NONE',  ( 159.9092487632085238, 278.3844945790232828, -10.24712064432635472 ) ) ;
#31442=CARTESIAN_POINT ( 'NONE',  ( 188.8930654812573380, 270.1357654272443938, -15.31858714226914486 ) ) ;
#31450=CARTESIAN_POINT ( 'NONE',  ( -27.42236680055714260, 166.5217562850347406, 1.224646799147364892E-15 ) ) ;
#31452=CARTESIAN_POINT ( 'NONE',  ( 151.0715479399129606, 268.9833987204304435, 14.24612252017116987 ) ) ;
#31455=ORIENTED_EDGE ( 'NONE', *, *, #78752, .F. ) ;
#31456=ORIENTED_EDGE ( 'NONE', *, *, #90945, .T. ) ;
#31460=CARTESIAN_POINT ( 'NONE',  ( 190.8623743139412454, 300.0636657654615647, 8.577953960666059530 ) ) ;
#31464=CARTESIAN_POINT ( 'NONE',  ( 148.1634546024981205, 274.0203641339852538, 9.324875965062235039 ) ) ;
#31466=EDGE_CURVE ( 'NONE', #33264, #91209, #34066, .T. ) ;
#31469=CARTESIAN_POINT ( 'NONE',  ( 161.8330907632800404, 267.0924558059494416, 16.50031884935262028 ) ) ;
#31470=VERTEX_POINT ( 'NONE', #54303 ) ;
#31472=CARTESIAN_POINT ( 'NONE',  ( 190.7862358025146534, 300.1955415356651429, 3.573119809004446257 ) ) ;
#31474=ORIENTED_EDGE ( 'NONE', *, *, #28507, .F. ) ;
#31476=CARTESIAN_POINT ( 'NONE',  ( 159.6430037033188114, 255.2459832026828224, 16.03379434140432735 ) ) ;
#31477=CARTESIAN_POINT ( 'NONE',  ( 150.6051381537932343, 269.7912441671369947, 13.72054362922755999 ) ) ;
#31479=VERTEX_POINT ( 'NONE', #22918 ) ;
#31482=B_SPLINE_CURVE_WITH_KNOTS ( 'NONE', 3,
 ( #26828, #4515, #57707, #35415 ),
 .UNSPECIFIED., .F., .F.,
 ( 4, 4 ),
 ( 0.005796625092869264924, 0.01143961042366389153 ),
 .UNSPECIFIED. ) ;
#31483=CARTESIAN_POINT ( 'NONE',  ( 190.1635032421960148, 301.2741459696644029, -5.047660290019184259 ) ) ;
#31484=CARTESIAN_POINT ( 'NONE',  ( 189.8147415777049218, 301.8782188922952514, -0.5019643756309712934 ) ) ;
#31486=CARTESIAN_POINT ( 'NONE',  ( 190.6094661480870798, 300.5017155583701083, 4.598210453186021951 ) ) ;
#31487=CARTESIAN_POINT ( 'NONE',  ( 157.1378598138013558, 259.5494816622388612, -17.27281705625119912 ) ) ;
#31488=CARTESIAN_POINT ( 'NONE',  ( 191.0626252760453383, 299.7168209248331436, 8.862249628642642207 ) ) ;
#31489=CARTESIAN_POINT ( 'NONE',  ( 147.5749398328735822, 275.0397016159798227, -4.620786157167191099 ) ) ;
#31490=CARTESIAN_POINT ( 'NONE',  ( 163.6900654399419466, 257.4571500704111600, 15.51179371342129620 ) ) ;
#31492=CARTESIAN_POINT ( 'NONE',  ( 205.7639495959071212, 274.2533802642843170, 10.79039487422292432 ) ) ;
#31496=CARTESIAN_POINT ( 'NONE',  ( 105.1810637865323628, 231.5333772461660828, 9.188101187500095079 ) ) ;
#31498=CARTESIAN_POINT ( 'NONE',  ( 146.6647111637776106, 276.6162639173599587, -0.6373001129109082674 ) ) ;
#31500=CARTESIAN_POINT ( 'NONE',  ( 192.9064638172013417, 270.9369261147751331, 14.92505667092759758 ) ) ;
#31502=CARTESIAN_POINT ( 'NONE',  ( 183.2940791498508872, 284.7098848858684619, -14.97307289601423186 ) ) ;
#31504=CARTESIAN_POINT ( 'NONE',  ( 165.6569603496038496, 284.1908122977653761, -8.522347108096667512 ) ) ;
#31508=CARTESIAN_POINT ( 'NONE',  ( 206.3117289818846700, 272.0185653065639713, 8.038418397519199843 ) ) ;
#31509=CARTESIAN_POINT ( 'NONE',  ( 127.4808708382166316, 256.6589784336661637, -6.496448406907676862E-16 ) ) ;
#31511=CARTESIAN_POINT ( 'NONE',  ( 188.5613127796079880, 298.7266913302852345, 4.776745480473671535 ) ) ;
#31512=CARTESIAN_POINT ( 'NONE',  ( 196.3519702320103590, 290.5554067223432639, 17.39042812051341969 ) ) ;
#31515=CARTESIAN_POINT ( 'NONE',  ( 41.36564329728401646, 200.8149278399160664, -9.188101187500095079 ) ) ;
#31522=CARTESIAN_POINT ( 'NONE',  ( 174.5201653990494322, 262.1690094913359985, 14.32490148041052258 ) ) ;
#31525=CARTESIAN_POINT ( 'NONE',  ( 202.8874463667715133, 279.2356300052831557, -15.29930322226033468 ) ) ;
#31527=CARTESIAN_POINT ( 'NONE',  ( 10.68506269473756909, 183.6427522451419350, -10.00000000000009592 ) ) ;
#31529=CARTESIAN_POINT ( 'NONE',  ( 100.8238734719678860, 239.0177522451419350, 5.000000000000046185 ) ) ;
#31530=B_SPLINE_SURFACE_WITH_KNOTS ( 'NONE', 3, 1, ( 
 ( #56374, #2202 ),
 ( #1702, #86340 ),
 ( #79235, #95934 ),
 ( #87372, #64990 ),
 ( #72614, #63483 ),
 ( #32068, #64488 ),
 ( #10292, #41164 ),
 ( #94420, #2704 ),
 ( #9288, #18396 ),
 ( #57371, #72101 ),
 ( #70574, #56871 ),
 ( #40163, #62979 ),
 ( #16876, #3216 ),
 ( #34100, #71604 ),
 ( #33592, #39653 ),
 ( #88346, #71104 ),
 ( #95449, #9807 ),
 ( #26000, #40667 ),
 ( #18905, #49781 ),
 ( #55360, #93926 ),
 ( #1191, #80740 ),
 ( #24481, #47762 ),
 ( #32585, #24974 ),
 ( #55851, #86846 ),
 ( #82227, #59345 ),
 ( #28465, #4172 ),
 ( #34578, #50274 ),
 ( #19416, #42171 ),
 ( #19894, #65976 ),
 ( #81226, #65478 ),
 ( #97891, #42658 ),
 ( #81718, #51262 ),
 ( #66962, #12800 ),
 ( #50766, #11802 ) ),
 .UNSPECIFIED., .T., .F., .F.,
 ( 4, 2, 2, 2, 2, 2, 2, 2, 2, 2, 2, 2, 2, 2, 2, 2, 4 ),
 ( 2, 2 ),
 ( 0.000000000000000000, 0.06250000000000000000, 0.1250000000000000000, 0.1875000000000000000, 0.2500000000000000000, 0.3125000000000000000, 0.3750000000000000000, 0.4375000000000000000, 0.5000000000000000000, 0.5625000000000000000, 0.6250000000000000000, 0.6875000000000000000, 0.7500000000000000000, 0.8125000000000000000, 0.8750000000000000000, 0.9375000000000000000, 1.000000000000000000 ),
 ( 0.000000000000000000, 1.000000000000000000 ),
 .UNSPECIFIED. ) ;
#31533=VERTEX_POINT ( 'NONE', #52327 ) ;
#31535=CARTESIAN_POINT ( 'NONE',  ( 203.0398866899141126, 278.9715956204779559, 16.57839218037009132 ) ) ;
#31537=CARTESIAN_POINT ( 'NONE',  ( 27.59033994439653270, 195.9244531367911293, -4.594050593750046652 ) ) ;
#31542=CARTESIAN_POINT ( 'NONE',  ( 185.9406580756425171, 265.4572926502605128, 14.02042132963198817 ) ) ;
#31543=CARTESIAN_POINT ( 'NONE',  ( 62.85372508080289577, 219.3464784336661637, 1.353441290958777327E-15 ) ) ;
#31544=CARTESIAN_POINT ( 'NONE',  ( 200.5438717407500917, 283.2948203288816558, 18.39667691545567152 ) ) ;
#31549=CARTESIAN_POINT ( 'NONE',  ( 31.19903945042937821, 195.4865022471903160, 10.00000000000009237 ) ) ;
#31551=CARTESIAN_POINT ( 'NONE',  ( -11.27255005043015856, 173.4869531367911293, 4.594050593750046652 ) ) ;
#31553=CARTESIAN_POINT ( 'NONE',  ( 200.4119102014255134, 282.6799346856502098, 16.91998934435313728 ) ) ;
#31554=CARTESIAN_POINT ( 'NONE',  ( 185.3347439640575658, 260.3534090642163505, 6.375270193058597989 ) ) ;
#31555=CARTESIAN_POINT ( 'NONE',  ( 205.8918578537579833, 274.0318366629789466, 11.52627491423194250 ) ) ;
#31556=CARTESIAN_POINT ( 'NONE',  ( 186.9626043371740707, 259.3098172291293508, -2.387369219704509327 ) ) ;
#31558=ORIENTED_EDGE ( 'NONE', *, *, #2518, .T. ) ;
#31559=DIRECTION ( 'NONE',  ( -0.8660254037844387076, -0.4999999999999998890, -0.000000000000000000 ) ) ;
#31560=CARTESIAN_POINT ( 'NONE',  ( 179.1598829120495964, 285.8685653680148562, 13.04984300519404528 ) ) ;
#31561=CARTESIAN_POINT ( 'NONE',  ( 196.1370092075112268, 290.1209220278959720, 16.40156295354631411 ) ) ;
#31563=ORIENTED_EDGE ( 'NONE', *, *, #60680, .T. ) ;
#31565=AXIS2_PLACEMENT_3D ( 'NONE', #817, #93556, #83468 ) ;
#31566=CARTESIAN_POINT ( 'NONE',  ( 157.7593757092099906, 257.3997412317380054, -18.08445832352326121 ) ) ;
#31567=CARTESIAN_POINT ( 'NONE',  ( 192.1149248854976861, 297.8941845364767005, 12.26771790733441314 ) ) ;
#31570=CARTESIAN_POINT ( 'NONE',  ( 207.6875671281972870, 270.9215769640275653, -2.211577121115235300 ) ) ;
#31571=CARTESIAN_POINT ( 'NONE',  ( 200.9445292274600092, 282.6008612054670266, -16.62830946367346741 ) ) ;
#31573=VERTEX_POINT ( 'NONE', #13836 ) ;
#31574=CARTESIAN_POINT ( 'NONE',  ( 190.5573062922015026, 281.4271296422851947, 16.94287472538490391 ) ) ;
#31578=CARTESIAN_POINT ( 'NONE',  ( -17.42236680055705023, 149.2012482093457777, 0.000000000000000000 ) ) ;
#31580=CARTESIAN_POINT ( 'NONE',  ( 146.5157004908022031, 276.8743579738231233, -0.1877253132609108255 ) ) ;
#31582=CARTESIAN_POINT ( 'NONE',  ( 149.6564118588553924, 271.4344863124460971, -11.76165597393390172 ) ) ;
#31585=ORIENTED_EDGE ( 'NONE', *, *, #40095, .T. ) ;
#31586=CARTESIAN_POINT ( 'NONE',  ( 161.4025183475459073, 251.0896330829197041, 14.50747140106038735 ) ) ;
#31587=FACE_OUTER_BOUND ( 'NONE', #87883, .T. ) ;
#31591=ORIENTED_EDGE ( 'NONE', *, *, #37146, .T. ) ;
#31594=ORIENTED_EDGE ( 'NONE', *, *, #6093, .T. ) ;
#31597=CARTESIAN_POINT ( 'NONE',  ( 163.8398374448017591, 246.8680725722146008, -5.948785025486735378 ) ) ;
#31599=CARTESIAN_POINT ( 'NONE',  ( 167.1501680486316559, 282.0009818228157314, 11.65768677921798790 ) ) ;
#31601=CARTESIAN_POINT ( 'NONE',  ( 194.7900911235093133, 293.2606606935473792, -14.66228443412922999 ) ) ;
#31608=CYLINDRICAL_SURFACE ( 'NONE', #929, 17.82106496071139645 ) ;
#31609=DIRECTION ( 'NONE',  ( 0.4999999999999992784, -0.8660254037844390407, 0.000000000000000000 ) ) ;
#31610=CARTESIAN_POINT ( 'NONE',  ( 198.2819808855875863, 287.2125302111982705, 18.53535247371401695 ) ) ;
#31613=CARTESIAN_POINT ( 'NONE',  ( 159.2713554375903300, 254.7809155221686410, -15.70062444474382168 ) ) ;
#31616=CARTESIAN_POINT ( 'NONE',  ( 171.6554683614685075, 255.1804135649609577, 10.96344727419213072 ) ) ;
#31617=CARTESIAN_POINT ( 'NONE',  ( 190.8112310826165867, 262.0020291435678246, -0.6932856109839961034 ) ) ;
#31619=CARTESIAN_POINT ( 'NONE',  ( 154.9949866785712231, 262.1878034846902779, -17.93766467320931213 ) ) ;
#31620=CARTESIAN_POINT ( 'NONE',  ( 128.5163324648304410, 256.5530062829863027, -4.648177544792955347E-16 ) ) ;
#31622=CARTESIAN_POINT ( 'NONE',  ( 23.74761253515288217, 184.5177522451418497, -10.00000000000009592 ) ) ;
#31623=CARTESIAN_POINT ( 'NONE',  ( 88.50972766791687718, 234.1589784336661353, -6.496448406907676862E-16 ) ) ;
#31625=CARTESIAN_POINT ( 'NONE',  ( -22.42236680055709641, 157.8615022471902591, 0.000000000000000000 ) ) ;
#31626=CARTESIAN_POINT ( 'NONE',  ( 167.0149686599001200, 278.0521133782755214, -13.60968902122515090 ) ) ;
#31628=CARTESIAN_POINT ( 'NONE',  ( 7.969365115964081703, 187.6589784336661637, -6.496448406907675876E-16 ) ) ;
#31630=CARTESIAN_POINT ( 'NONE',  ( 161.1884843536000744, 251.4603508349806873, 13.21272898143761942 ) ) ;
#31631=VERTEX_POINT ( 'NONE', #77121 ) ;
#31634=CARTESIAN_POINT ( 'NONE',  ( 197.8141251302497778, 265.6821229749213558, -2.897974208861140433 ) ) ;
#31635=EDGE_CURVE ( 'NONE', #12301, #41077, #27933, .T. ) ;
#31638=CARTESIAN_POINT ( 'NONE',  ( 201.9906765889849112, 280.7888808231018061, -16.23360557870388732 ) ) ;
#31639=CARTESIAN_POINT ( 'NONE',  ( 105.0176211588661772, 242.9860189848785126, -2.679491924311252493 ) ) ;
#31641=CARTESIAN_POINT ( 'NONE',  ( 29.07873433320978052, 199.8464784336661637, 1.353441290958777525E-15 ) ) ;
#31642=CARTESIAN_POINT ( 'NONE',  ( 199.0369196554013627, 277.3085947641471876, 15.18055274685867673 ) ) ;
#31644=CARTESIAN_POINT ( 'NONE',  ( 153.3257670986663470, 273.8331553043774989, -11.88532112633179594 ) ) ;
#31645=ADVANCED_FACE ( 'NONE', ( #68527 ), #90891, .T. ) ;
#31647=CARTESIAN_POINT ( 'NONE',  ( 182.5436984794861814, 260.5467356096382900, -10.91178052607559046 ) ) ;
#31650=CARTESIAN_POINT ( 'NONE',  ( 194.2669918475045279, 294.1666952169902629, 14.00965265288584050 ) ) ;
#31651=CARTESIAN_POINT ( 'NONE',  ( 207.1019571622349815, 271.9358831784929293, -5.989975140547304733 ) ) ;
#31654=CARTESIAN_POINT ( 'NONE',  ( 147.7467138384290308, 274.7421803109381813, -9.190172068879620682 ) ) ;
#31655=CARTESIAN_POINT ( 'NONE',  ( 189.2703867623931728, 262.7700255369126694, 8.020027416226151118 ) ) ;
#31656=CARTESIAN_POINT ( 'NONE',  ( 167.9135783974399772, 278.5162520875397831, 14.81510772495481554 ) ) ;
#31657=CARTESIAN_POINT ( 'NONE',  ( 192.5295226464411371, 265.2521209099669477, 8.400182565873334894 ) ) ;
#31658=CARTESIAN_POINT ( 'NONE',  ( 146.7818291168261453, 276.4134096722012828, -0.7617065417431535534 ) ) ;
#31659=CARTESIAN_POINT ( 'NONE',  ( -17.42236680055705023, 149.2012482093457777, 0.000000000000000000 ) ) ;
#31660=CARTESIAN_POINT ( 'NONE',  ( 180.7783084174795079, 266.7965790172731886, -14.72117180798574232 ) ) ;
#31662=CARTESIAN_POINT ( 'NONE',  ( 186.3032856786115303, 294.1815019053933611, 11.41626773807880468 ) ) ;
#31663=CARTESIAN_POINT ( 'NONE',  ( 207.5570596878370679, 271.1476224814971374, 2.444960520848353358 ) ) ;
#31664=CARTESIAN_POINT ( 'NONE',  ( 189.0720805967732758, 299.7343203868808246, 4.955419684386629164 ) ) ;
#31665=CARTESIAN_POINT ( 'NONE',  ( 108.1307024963493149, 242.4244531367911293, -4.594050593750046652 ) ) ;
#31667=CARTESIAN_POINT ( 'NONE',  ( 191.4941427383744781, 298.9694107557253346, 8.584406880462095657 ) ) ;
#31669=CARTESIAN_POINT ( 'NONE',  ( 136.3105610988903607, 261.0530062829863027, -4.648177544792955347E-16 ) ) ;
#31670=CARTESIAN_POINT ( 'NONE',  ( 195.2304193712978986, 279.0657389023923542, 16.29610427727775246 ) ) ;
#31671=CARTESIAN_POINT ( 'NONE',  ( 150.4957438262301253, 269.9807207005363807, -15.25519111672087114 ) ) ;
#31672=CARTESIAN_POINT ( 'NONE',  ( 192.1929114410880288, 263.4101189793182698, -4.344445731632683660 ) ) ;
#31673=CARTESIAN_POINT ( 'NONE',  ( 149.9475948592590839, 271.6738979692356111, -11.66626220284549298 ) ) ;
#31674=CARTESIAN_POINT ( 'NONE',  ( 58.02232427585079222, 192.7592609112379876, 2.679491924311254714 ) ) ;
#31675=DIRECTION ( 'NONE',  ( -0.8660254037844387076, -0.4999999999999998890, -0.000000000000000000 ) ) ;
#31678=FACE_OUTER_BOUND ( 'NONE', #21510, .T. ) ;
#31679=CARTESIAN_POINT ( 'NONE',  ( 199.9984457123739503, 270.0849612724584290, 9.145354784334640996 ) ) ;
#31681=CARTESIAN_POINT ( 'NONE',  ( 180.1105033416455967, 262.3445359189764190, -12.66037080800385084 ) ) ;
#31688=CARTESIAN_POINT ( 'NONE',  ( 181.4735074999749145, 292.1586133693310785, 10.55809797880889001 ) ) ;
#31689=CARTESIAN_POINT ( 'NONE',  ( 194.4032909867620447, 293.9306181827685123, -16.05392006271526384 ) ) ;
#31690=CARTESIAN_POINT ( 'NONE',  ( 156.6941734481478079, 259.2447256682348211, 17.84224415335075520 ) ) ;
#31691=VERTEX_POINT ( 'NONE', #99947 ) ;
#31693=CARTESIAN_POINT ( 'NONE',  ( 159.1215725138524704, 256.7057375585948193, 16.87965583163218142 ) ) ;
#31694=CARTESIAN_POINT ( 'NONE',  ( 193.0105523955311355, 296.3429121844422980, -12.00165843972855839 ) ) ;
#31699=CARTESIAN_POINT ( 'NONE',  ( 155.1865148098964937, 261.8560670301561686, -16.99758927948949605 ) ) ;
#31700=VERTEX_POINT ( 'NONE', #45712 ) ;
#31702=ORIENTED_EDGE ( 'NONE', *, *, #61148, .F. ) ;
#31705=VERTEX_POINT ( 'NONE', #6231 ) ;
#31709=CARTESIAN_POINT ( 'NONE',  ( 155.5066938333533528, 261.3015006940112244, -18.40036130547566273 ) ) ;
#31711=CARTESIAN_POINT ( 'NONE',  ( 207.3988330342936877, 270.8564699888902396, -1.301389719878858875 ) ) ;
#31712=CARTESIAN_POINT ( 'NONE',  ( 164.4575000359379828, 245.7982495824318505, -1.032884424947213997 ) ) ;
#31713=CARTESIAN_POINT ( 'NONE',  ( 190.3440926964027540, 300.9613558596673784, 1.920019422129680464 ) ) ;
#31718=CARTESIAN_POINT ( 'NONE',  ( 49.89075441544353851, 199.6115022471902591, 10.00000000000009592 ) ) ;
#31720=CARTESIAN_POINT ( 'NONE',  ( 122.7720312530212396, 247.8149278399160949, 9.188101187500093303 ) ) ;
#31727=CARTESIAN_POINT ( 'NONE',  ( 203.6388180714938301, 276.2575050999084283, 13.35755797172022952 ) ) ;
#31729=CARTESIAN_POINT ( 'NONE',  ( 173.7521259494088781, 289.6425462570808236, -4.709990374833325610 ) ) ;
#31730=CARTESIAN_POINT ( 'NONE',  ( 157.4656258344471098, 257.9085309395441641, 18.30485740784190796 ) ) ;
#31733=CARTESIAN_POINT ( 'NONE',  ( 173.3670856503965183, 287.2530419906886436, -9.722124389285141888 ) ) ;
#31739=CARTESIAN_POINT ( 'NONE',  ( 148.4083960970861256, 273.5961130204771052, -8.574185186226726429 ) ) ;
#31742=CARTESIAN_POINT ( 'NONE',  ( 188.3092780937153350, 266.3409406274001299, -11.83214085844302943 ) ) ;
#31743=CARTESIAN_POINT ( 'NONE',  ( 160.2261283380418035, 278.9007923701936420, 10.53197256397347203 ) ) ;
#31744=CARTESIAN_POINT ( 'NONE',  ( 192.1948126989040873, 297.7558147847510099, -10.38004547301857272 ) ) ;
#31745=CARTESIAN_POINT ( 'NONE',  ( 149.4491471355718772, 271.7934793437897270, 11.43912701239353780 ) ) ;
#31746=CARTESIAN_POINT ( 'NONE',  ( 204.6742660055938643, 272.9835131625996496, -9.777367022634962268 ) ) ;
#31747=CARTESIAN_POINT ( 'NONE',  ( 164.4368094649636305, 283.5685030574936150, -6.732700809822128818 ) ) ;
#31748=CARTESIAN_POINT ( 'NONE',  ( 154.9259971922039938, 277.6026755967128565, -8.943939257718048097 ) ) ;
#31749=CARTESIAN_POINT ( 'NONE',  ( 200.8147387322574957, 282.8256649374973790, -18.02438097732020239 ) ) ;
#31751=CARTESIAN_POINT ( 'NONE',  ( 190.8683709797118411, 300.0532792356709706, -4.461919767133968762 ) ) ;
#31752=CARTESIAN_POINT ( 'NONE',  ( 193.8848781386269309, 267.1185884883711879, -11.59377028749509364 ) ) ;
#31754=CARTESIAN_POINT ( 'NONE',  ( 163.5128695541682191, 247.8493887573044105, -7.994499776565081817 ) ) ;
#31756=DIRECTION ( 'NONE',  ( -0.8660254037844387076, -0.4999999999999998890, -0.000000000000000000 ) ) ;
#31757=EDGE_CURVE ( 'NONE', #37198, #21557, #38881, .T. ) ;
#31758=CARTESIAN_POINT ( 'NONE',  ( 184.5615956163028955, 297.0763260467899158, -4.452223854632125999 ) ) ;
#31759=CARTESIAN_POINT ( 'NONE',  ( 192.5254593562406171, 297.1831179748913314, 11.00703791256144015 ) ) ;
#31761=ADVANCED_FACE ( 'NONE', ( #47709 ), #48229, .T. ) ;
#31764=CARTESIAN_POINT ( 'NONE',  ( 0.4734401320438119676, 161.8923013555410080, 4.594050593750050204 ) ) ;
#31765=CARTESIAN_POINT ( 'NONE',  ( 97.82019495012963262, 215.0327760586659451, 1.948934522072303157E-15 ) ) ;
#31766=CARTESIAN_POINT ( 'NONE',  ( 37.35373998880870516, 180.8262482093457493, 3.021315404115420679E-15 ) ) ;
#31767=CARTESIAN_POINT ( 'NONE',  ( 192.9633865298379476, 296.4246058602058156, -11.85717392250713864 ) ) ;
#31769=LINE ( 'NONE', #62673, #4310 ) ;
#31772=CARTESIAN_POINT ( 'NONE',  ( -22.42236680055709641, 157.8615022471902591, 0.000000000000000000 ) ) ;
#31773=CARTESIAN_POINT ( 'NONE',  ( 163.1008115941903895, 248.1481028935802442, 11.25332017433677834 ) ) ;
#31774=CARTESIAN_POINT ( 'NONE',  ( 163.3718935141138786, 265.0702796956427392, 17.82925771866536735 ) ) ;
#31776=EDGE_CURVE ( 'NONE', #90496, #47930, #75161, .T. ) ;
#31777=CARTESIAN_POINT ( 'NONE',  ( 177.8610022267205863, 290.0596117902207425, 9.769913558664320874 ) ) ;
#31780=CARTESIAN_POINT ( 'NONE',  ( 205.0423986797212592, 275.5031431113662279, -12.28496450925721462 ) ) ;
#31781=CARTESIAN_POINT ( 'NONE',  ( 196.4351339088274813, 290.4113630087520050, 17.20526457544535504 ) ) ;
#31785=CARTESIAN_POINT ( 'NONE',  ( 40.49996498926459765, 188.0643266524160140, 9.188101187500095079 ) ) ;
#31786=CARTESIAN_POINT ( 'NONE',  ( 77.73905735199544154, 209.5643266524159571, -9.188101187500093303 ) ) ;
#31790=CARTESIAN_POINT ( 'NONE',  ( 147.7245617474428911, 256.0958772461660828, -9.188101187500095079 ) ) ;
#31793=CARTESIAN_POINT ( 'NONE',  ( 196.6461856324828830, 268.7375099474577951, -10.58772324698134604 ) ) ;
#31798=CARTESIAN_POINT ( 'NONE',  ( 68.48323730116675279, 210.3458772461660544, 9.188101187500095079 ) ) ;
#31799=CARTESIAN_POINT ( 'NONE',  ( 173.1933364606677799, 257.0593323752887045, -13.27564283692902691 ) ) ;
#31800=CARTESIAN_POINT ( 'NONE',  ( 203.1526193585190470, 278.7763369107815379, -16.67658907091021447 ) ) ;
#31801=AXIS2_PLACEMENT_3D ( 'NONE', #77752, #93473, #62506 ) ;
#31802=CARTESIAN_POINT ( 'NONE',  ( 159.2554912534056939, 254.8083930951974878, 16.49944922174842432 ) ) ;
#31804=CARTESIAN_POINT ( 'NONE',  ( 153.2249512918476455, 276.7798453101777341, 7.180601189652168870 ) ) ;
#31806=CARTESIAN_POINT ( 'NONE',  ( 105.8215617431884539, 245.2365022471903444, 2.944929066748280225E-16 ) ) ;
#31807=( BOUNDED_CURVE ( )  B_SPLINE_CURVE ( 2, ( #9888, #40746, #2288, #78277, #25574, #39728, #54782, #29991, #91332 ),
 .UNSPECIFIED., .F., .T. ) 
 B_SPLINE_CURVE_WITH_KNOTS ( ( 3, 2, 2, 2, 3 ),
 ( 0.6814516129032257563, 0.6827956989247311315, 0.6854838709677418818, 0.6881720430107527431, 0.6895161290322581182 ),
 .UNSPECIFIED. ) 
 CURVE ( )  GEOMETRIC_REPRESENTATION_ITEM ( )  RATIONAL_B_SPLINE_CURVE ( ( 0.9330127018922194093, 0.9330127018922194093, 1.000000000000000000, 0.8660254037844387076, 1.000000000000000000, 0.8660254037844387076, 1.000000000000000000, 0.9330127018922194093, 0.9330127018922194093 ) ) 
 REPRESENTATION_ITEM ( '' )  );
#31808=CARTESIAN_POINT ( 'NONE',  ( 200.8551880497955437, 282.7556046643899776, 18.00894873733387058 ) ) ;
#31809=CARTESIAN_POINT ( 'NONE',  ( 164.3524132573224392, 245.9802652221976587, -2.749586949851067441 ) ) ;
#31810=ORIENTED_EDGE ( 'NONE', *, *, #65744, .F. ) ;
#31812=CARTESIAN_POINT ( 'NONE',  ( 184.7850555545515192, 271.2875256772542230, 16.11813442280277542 ) ) ;
#31814=CARTESIAN_POINT ( 'NONE',  ( 159.3586121662929713, 254.6297824347537642, -15.50090345830412630 ) ) ;
#31815=CARTESIAN_POINT ( 'NONE',  ( 190.1758200331204876, 279.2204749713225169, -17.78067544974210890 ) ) ;
#31817=ORIENTED_EDGE ( 'NONE', *, *, #41427, .F. ) ;
#31818=CARTESIAN_POINT ( 'NONE',  ( 173.2954469512942239, 251.6588534220469739, -0.1071739093455414404 ) ) ;
#31819=ORIENTED_EDGE ( 'NONE', *, *, #59647, .F. ) ;
#31820=DIRECTION ( 'NONE',  ( -0.4999999999999987788, 0.8660254037844392627, 0.000000000000000000 ) ) ;
#31821=CARTESIAN_POINT ( 'NONE',  ( 147.6095889327917803, 274.9796876144846465, -8.460961150142429332 ) ) ;
#31822=B_SPLINE_CURVE_WITH_KNOTS ( 'NONE', 3,
 ( #17610, #47994, #30812, #78937, #63708, #94644, #7495, #23192, #100226, #69799, #61691, #92644, #85039, #85562, #25723, #64717 ),
 .UNSPECIFIED., .F., .F.,
 ( 4, 2, 2, 2, 2, 2, 2, 4 ),
 ( 0.0005957069887743393069, 0.0008992575955524882789, 0.001202808202330637143, 0.001506358809108786223, 0.001809909415886935304, 0.002113460022665083950, 0.002417010629443233465, 0.003024111842999524253 ),
 .UNSPECIFIED. ) ;
#31823=CARTESIAN_POINT ( 'NONE',  ( 206.7951683401124399, 270.7576251107032590, -5.378181275766958258 ) ) ;
#31824=VERTEX_POINT ( 'NONE', #33534 ) ;
#31825=ADVANCED_FACE ( 'NONE', ( #64433 ), #8236, .T. ) ;
#31827=CARTESIAN_POINT ( 'NONE',  ( 21.99520779934447745, 195.0530062829863311, -4.648177544792955347E-16 ) ) ;
#31829=EDGE_CURVE ( 'NONE', #58437, #27033, #18844, .T. ) ;
#31832=CARTESIAN_POINT ( 'NONE',  ( 159.8597520197352537, 253.7617827468940277, -16.74905990210778839 ) ) ;
#31833=ORIENTED_EDGE ( 'NONE', *, *, #5156, .T. ) ;
#31834=CARTESIAN_POINT ( 'NONE',  ( 174.5161929735236583, 286.6389660134419159, 11.76074990303198220 ) ) ;
#31837=CARTESIAN_POINT ( 'NONE',  ( 208.3699316049496133, 269.7396870210121733, -1.898463622294385811 ) ) ;
#31838=CARTESIAN_POINT ( 'NONE',  ( 154.9344967692067598, 262.2925750810547356, 17.30210568643136781 ) ) ;
#31840=CARTESIAN_POINT ( 'NONE',  ( 204.6475128369918082, 276.1871054541632020, -13.72068618491070779 ) ) ;
#31841=CARTESIAN_POINT ( 'NONE',  ( 208.0730008398676318, 270.2539861924646516, -3.911917750280078376 ) ) ;
#31843=CARTESIAN_POINT ( 'NONE',  ( 206.5911069559201110, 270.4023401184283557, 3.160577138512981055 ) ) ;
#31844=CARTESIAN_POINT ( 'NONE',  ( 195.6460486738788518, 290.5633724012552079, -16.40341345355467695 ) ) ;
#31845=CARTESIAN_POINT ( 'NONE',  ( 90.02596631606967037, 210.5327760586659451, 1.948934522072303157E-15 ) ) ;
#31846=EDGE_LOOP ( 'NONE', ( #10549, #40939, #60000, #23418 ) ) ;
#31847=CARTESIAN_POINT ( 'NONE',  ( 150.6487462746963502, 269.7157126861102370, 15.18501655901553704 ) ) ;
#31848=CARTESIAN_POINT ( 'NONE',  ( 195.2347945672775325, 277.4660317214627980, -17.03751719888963123 ) ) ;
#31852=CARTESIAN_POINT ( 'NONE',  ( 196.1005589118404373, 290.9908639024753825, -16.71343850857806501 ) ) ;
#31856=DIRECTION ( 'NONE',  ( -0.4999999999999987788, 0.8660254037844392627, 0.000000000000000000 ) ) ;
#31857=EDGE_CURVE ( 'NONE', #30831, #93932, #95203, .T. ) ;
#31860=CARTESIAN_POINT ( 'NONE',  ( -22.42236680055709641, 157.8615022471902591, 0.000000000000000000 ) ) ;
#31862=CARTESIAN_POINT ( 'NONE',  ( 157.4883523481626639, 280.5151220735496622, 7.290131461700886106 ) ) ;
#31864=CARTESIAN_POINT ( 'NONE',  ( 89.24104401994878799, 213.1423013555409796, -4.594050593750043987 ) ) ;
#31867=ORIENTED_EDGE ( 'NONE', *, *, #30294, .T. ) ;
#31868=CARTESIAN_POINT ( 'NONE',  ( 163.4178923001155681, 247.5989030008181260, -10.38047187240561442 ) ) ;
#31871=CARTESIAN_POINT ( 'NONE',  ( 184.0702669486040008, 275.1941235734948918, 16.36998289429038067 ) ) ;
#31873=CARTESIAN_POINT ( 'NONE',  ( 206.1823507212516802, 271.5286882572439140, -8.119960357998227352 ) ) ;
#31877=CARTESIAN_POINT ( 'NONE',  ( 189.2891873318943396, 295.0123130764713437, 11.41301585810447783 ) ) ;
#31878=CARTESIAN_POINT ( 'NONE',  ( 185.8275728834229596, 259.3864893694817511, 5.920843924932031932 ) ) ;
#31881=CARTESIAN_POINT ( 'NONE',  ( 111.3525576494051563, 223.5494855054051584, -2.679491924311248496 ) ) ;
#31882=DIRECTION ( 'NONE',  ( 0.4999999999999998890, -0.8660254037844385966, 0.000000000000000000 ) ) ;
#31884=CARTESIAN_POINT ( 'NONE',  ( 188.2145160130152419, 294.1882611685968527, -12.46123440450256936 ) ) ;
#31886=CARTESIAN_POINT ( 'NONE',  ( 200.1782072557437857, 283.9281697954355650, 18.05177561285849208 ) ) ;
#31888=CARTESIAN_POINT ( 'NONE',  ( 187.7420758953736595, 266.0326380175162058, -11.83518821542502586 ) ) ;
#31890=CARTESIAN_POINT ( 'NONE',  ( 153.2338012341922990, 270.4421391452444254, 13.91873268832451416 ) ) ;
#31893=CARTESIAN_POINT ( 'NONE',  ( 170.5373622343556690, 269.7751423367952270, 17.81562764448176850 ) ) ;
#31894=EDGE_CURVE ( 'NONE', #19653, #62639, #36260, .T. ) ;
#31897=CARTESIAN_POINT ( 'NONE',  ( 207.5686001603237116, 271.1276337968068333, 7.659944433763431704 ) ) ;
#31898=CARTESIAN_POINT ( 'NONE',  ( 194.4459411895494725, 293.8567458645873103, 14.31012567920753042 ) ) ;
#31900=CARTESIAN_POINT ( 'NONE',  ( 199.1671527971112141, 281.9112550430394322, -16.60146190726549165 ) ) ;
#31902=CARTESIAN_POINT ( 'NONE',  ( 165.1772004350705458, 286.3187765620995151, -3.363692932437915228 ) ) ;
#31904=CARTESIAN_POINT ( 'NONE',  ( 188.2316138847417051, 260.8329576480458059, 3.008261098653536525 ) ) ;
#31906=CARTESIAN_POINT ( 'NONE',  ( -7.294332625736644538, 178.8464784336661637, 1.353441290958777327E-15 ) ) ;
#31909=CARTESIAN_POINT ( 'NONE',  ( 160.1902186677070574, 253.5786389215288068, -14.79079237559988691 ) ) ;
#31911=CARTESIAN_POINT ( 'NONE',  ( 208.3135187673106543, 269.8373969220020285, 2.829653198597726682 ) ) ;
#31912=CARTESIAN_POINT ( 'NONE',  ( 176.5752601597114335, 288.5842064133888130, 11.38490813771325350 ) ) ;
#31913=CARTESIAN_POINT ( 'NONE',  ( 16.25090658753528317, 186.3149278399161233, 9.188101187500093303 ) ) ;
#31915=CARTESIAN_POINT ( 'NONE',  ( 64.10800479423804177, 214.4865022471902876, -10.00000000000009592 ) ) ;
#31918=CARTESIAN_POINT ( 'NONE',  ( 191.1192699377806719, 299.6187094927299199, -9.526914969203620132 ) ) ;
#31921=CARTESIAN_POINT ( 'NONE',  ( 186.8377166567931909, 295.8024518766285382, -7.974395351236546858 ) ) ;
#31922=CARTESIAN_POINT ( 'NONE',  ( 190.5217488035042379, 261.8431898049273059, -0.7587358768599492542 ) ) ;
#31924=CARTESIAN_POINT ( 'NONE',  ( 68.58246938045769525, 203.7365022471902023, 10.00000000000009592 ) ) ;
#31927=CARTESIAN_POINT ( 'NONE',  ( 40.66251830035667325, 182.0327760586659451, 1.948934522072303157E-15 ) ) ;
#31929=ADVANCED_FACE ( 'NONE', ( #66421 ), #77132, .F. ) ;
#31932=CARTESIAN_POINT ( 'NONE',  ( 173.6088960567799120, 251.7861549345625178, -6.312679096147793878 ) ) ;
#31934=CARTESIAN_POINT ( 'NONE',  ( -5.122212653107841795, 179.3967562850347406, 2.649461200531984646E-14 ) ) ;
#31935=CARTESIAN_POINT ( 'NONE',  ( 162.9249713293285424, 280.6004508475537023, -9.976534934921010844 ) ) ;
#31936=CARTESIAN_POINT ( 'NONE',  ( 205.6544395269333165, 269.2573939850345255, -1.340776332317544339 ) ) ;
#31938=CARTESIAN_POINT ( 'NONE',  ( 162.9796882977680639, 248.3578945969637743, 9.683801903336119565 ) ) ;
#31939=CARTESIAN_POINT ( 'NONE',  ( 108.6902708896766114, 226.8927522451418213, 10.00000000000009948 ) ) ;
#31940=CARTESIAN_POINT ( 'NONE',  ( 188.5189969585072731, 269.7688609434800924, -14.07648933449623208 ) ) ;
#31942=AXIS2_PLACEMENT_3D ( 'NONE', #83230, #57527, #88503 ) ;
#31946=CARTESIAN_POINT ( 'NONE',  ( 161.5029716424245407, 251.3413373469583973, -13.00020995489466458 ) ) ;
#31952=CARTESIAN_POINT ( 'NONE',  ( 191.2645787786270262, 299.3670271975948367, 7.309947121636420242 ) ) ;
#31953=CARTESIAN_POINT ( 'NONE',  ( 180.9038145878475916, 257.6994971499530607, -7.472903516740896812 ) ) ;
#31958=VERTEX_POINT ( 'NONE', #98335 ) ;
#31963=CARTESIAN_POINT ( 'NONE',  ( 147.8465295590381743, 274.5692944114487091, 9.322947948439978205 ) ) ;
#31965=CARTESIAN_POINT ( 'NONE',  ( 149.1004267900891307, 272.3974806997987343, -12.86882154300063341 ) ) ;
#31966=CARTESIAN_POINT ( 'NONE',  ( 83.50336539627915045, 219.0177522451418497, -10.00000000000009592 ) ) ;
#31972=FACE_OUTER_BOUND ( 'NONE', #61989, .T. ) ;
#31974=CARTESIAN_POINT ( 'NONE',  ( 54.68078388046973970, 208.5024278399160949, -9.188101187500093303 ) ) ;
#31975=ORIENTED_EDGE ( 'NONE', *, *, #37993, .F. ) ;
#31978=CARTESIAN_POINT ( 'NONE',  ( 190.8094645593471341, 300.1553081486349015, 8.399847186519689757 ) ) ;
#31980=CARTESIAN_POINT ( 'NONE',  ( 172.8855825645377990, 271.3786399235225417, 16.45412496818341097 ) ) ;
#31982=ORIENTED_EDGE ( 'NONE', *, *, #99902, .T. ) ;
#31985=CARTESIAN_POINT ( 'NONE',  ( 165.6039301651514961, 278.9421411211367285, 14.15335429374977139 ) ) ;
#31987=CARTESIAN_POINT ( 'NONE',  ( 175.3038007714868058, 260.9809825493145468, -14.68767903443118605 ) ) ;
#31988=CARTESIAN_POINT ( 'NONE',  ( 171.4076116757450450, 275.9429945178056869, -16.88996634460038848 ) ) ;
#31989=FACE_OUTER_BOUND ( 'NONE', #86228, .T. ) ;
#31990=CARTESIAN_POINT ( 'NONE',  ( 192.4212750754384160, 297.3635704425909125, -12.73704185013552248 ) ) ;
#31991=CARTESIAN_POINT ( 'NONE',  ( 160.1876870865671947, 255.7147813180542073, 16.12179979881591407 ) ) ;
#31992=DIRECTION ( 'NONE',  ( -0.4999999999999987788, 0.8660254037844392627, 0.000000000000000000 ) ) ;
#31995=CARTESIAN_POINT ( 'NONE',  ( 207.7655736232174206, 270.7864657513322300, 3.530742899761726949 ) ) ;
#31997=CARTESIAN_POINT ( 'NONE',  ( 111.5140480995885497, 229.0643266524159856, -9.188101187500093303 ) ) ;
#32001=CARTESIAN_POINT ( 'NONE',  ( 203.4696564630250464, 278.2272125378923988, -16.38980782817167636 ) ) ;
#32002=CARTESIAN_POINT ( 'NONE',  ( 182.8969736784899567, 285.4463084877070287, -15.16533932269233986 ) ) ;
#32004=CARTESIAN_POINT ( 'NONE',  ( 178.0214568497756886, 255.3923698286970705, 4.825899244335746019 ) ) ;
#32009=CARTESIAN_POINT ( 'NONE',  ( 182.1624531057215393, 260.1812964409709252, 10.65669563999669833 ) ) ;
#32010=CARTESIAN_POINT ( 'NONE',  ( 205.9474858145129019, 272.6472302773099159, 9.310014741362042656 ) ) ;
#32011=CARTESIAN_POINT ( 'NONE',  ( 128.9971094863694532, 233.0327760586659451, 1.948934522072302763E-15 ) ) ;
#32012=CARTESIAN_POINT ( 'NONE',  ( 189.7310370775148840, 294.7812428202356614, -12.66668878006862364 ) ) ;
#32014=CARTESIAN_POINT ( 'NONE',  ( 189.1692022066353331, 299.6200726245371015, 4.912915616140450581 ) ) ;
#32015=CARTESIAN_POINT ( 'NONE',  ( 195.9920715006079490, 291.1787696107118677, 15.99608784761372071 ) ) ;
#32017=CARTESIAN_POINT ( 'NONE',  ( 53.16558651961199899, 195.3768266524160140, 9.188101187500098632 ) ) ;
#32019=ORIENTED_EDGE ( 'NONE', *, *, #69849, .T. ) ;
#32022=EDGE_CURVE ( 'NONE', #87147, #91470, #57970, .T. ) ;
#32023=CARTESIAN_POINT ( 'NONE',  ( 175.0915097197001558, 261.2351211855327051, 15.18232397002616629 ) ) ;
#32026=CARTESIAN_POINT ( 'NONE',  ( 178.3743760340321387, 261.1640921747737139, 13.34356303130173949 ) ) ;
#32027=AXIS2_PLACEMENT_3D ( 'NONE', #39417, #16636, #8545 ) ;
#32028=CARTESIAN_POINT ( 'NONE',  ( 124.2787281577965075, 235.8927522451418213, 10.00000000000009592 ) ) ;
#32029=CARTESIAN_POINT ( 'NONE',  ( 194.5514039441539751, 292.7602831052016086, -15.13274470691405149 ) ) ;
#32030=ORIENTED_EDGE ( 'NONE', *, *, #16354, .F. ) ;
#32031=CARTESIAN_POINT ( 'NONE',  ( 189.9462859318020946, 301.6503773875500087, -1.164147598593831656 ) ) ;
#32033=CARTESIAN_POINT ( 'NONE',  ( 34.68144358152915174, 181.6423013555409796, -4.594050593750043987 ) ) ;
#32038=CARTESIAN_POINT ( 'NONE',  ( 168.9285091408607684, 266.8905904589466900, 17.77692745299157195 ) ) ;
#32039=CARTESIAN_POINT ( 'NONE',  ( 62.79092448910136426, 200.3927522451417929, -10.00000000000009059 ) ) ;
#32041=CARTESIAN_POINT ( 'NONE',  ( 184.7966971888043020, 257.5870176390811821, 1.382809315717336229 ) ) ;
#32042=CARTESIAN_POINT ( 'NONE',  ( 204.7519188734507622, 276.0062688943993408, -12.76027478560537531 ) ) ;
#32044=ORIENTED_EDGE ( 'NONE', *, *, #86860, .T. ) ;
#32046=CARTESIAN_POINT ( 'NONE',  ( 27.73493783529162116, 193.4865022471903444, -10.00000000000009415 ) ) ;
#32047=CARTESIAN_POINT ( 'NONE',  ( 32.84087927488944558, 199.7677522451419350, -5.000000000000047962 ) ) ;
#32048=CARTESIAN_POINT ( 'NONE',  ( 162.6264071486809542, 248.9697954965390920, 10.36322805486644683 ) ) ;
#32050=CARTESIAN_POINT ( 'NONE',  ( -3.504777292649704279, 156.5327760586659451, 1.948934522072303157E-15 ) ) ;
#32052=CARTESIAN_POINT ( 'NONE',  ( 164.1204250983133477, 260.5664103406105028, -16.15875528054763421 ) ) ;
#32053=CARTESIAN_POINT ( 'NONE',  ( 170.9051221141708083, 262.8660520292235674, 16.32175538396744230 ) ) ;
#32054=EDGE_CURVE ( 'NONE', #54506, #4704, #44668, .T. ) ;
#32055=CARTESIAN_POINT ( 'NONE',  ( 185.8626946602280441, 259.3471889805154547, 7.308832903665572367 ) ) ;
#32056=DIRECTION ( 'NONE',  ( 0.5000000000000048850, -0.8660254037844358210, 0.000000000000000000 ) ) ;
#32063=CARTESIAN_POINT ( 'NONE',  ( 181.8249261631527531, 287.9314247020339508, 13.64167460269014320 ) ) ;
#32064=CARTESIAN_POINT ( 'NONE',  ( 154.0709734344990522, 278.1335148570522620, -5.205178880588171353 ) ) ;
#32066=CARTESIAN_POINT ( 'NONE',  ( 159.0552039522962957, 259.4077134839495216, 16.69544169553007151 ) ) ;
#32068=CARTESIAN_POINT ( 'NONE',  ( 206.8851632406098702, 272.3113812655195716, -9.957011741946159233 ) ) ;
#32069=CARTESIAN_POINT ( 'NONE',  ( 56.31377616017810084, 209.9865022471902876, -10.00000000000009592 ) ) ;
#32070=CARTESIAN_POINT ( 'NONE',  ( 152.6757560589063303, 266.2048287524194166, 16.73757896668104195 ) ) ;
#32071=CARTESIAN_POINT ( 'NONE',  ( 188.5410240070633563, 293.7196559869043426, 13.01390607220156248 ) ) ;
#32072=CARTESIAN_POINT ( 'NONE',  ( 191.5235241413101903, 298.4719041358723075, 8.455706032256406601 ) ) ;
#32073=CARTESIAN_POINT ( 'NONE',  ( 208.3699316049496133, 269.7396870210121733, -1.898463622294385811 ) ) ;
#32074=CARTESIAN_POINT ( 'NONE',  ( 154.8679462054080318, 262.4078440388265676, 17.98338675682672871 ) ) ;
#32077=ORIENTED_EDGE ( 'NONE', *, *, #37270, .T. ) ;
#32079=CARTESIAN_POINT ( 'NONE',  ( 164.4506649252758734, 248.7574976766044585, 10.04808630291115357 ) ) ;
#32082=CARTESIAN_POINT ( 'NONE',  ( 155.3659625055495326, 262.0475265963984839, -17.02029351793501988 ) ) ;
#32084=CARTESIAN_POINT ( 'NONE',  ( 162.8384627734353387, 250.8402808221231624, -13.07578932517241732 ) ) ;
#32087=CARTESIAN_POINT ( 'NONE',  ( 204.9004517216375518, 275.7490024547470853, 14.55104398969427670 ) ) ;
#32089=ORIENTED_EDGE ( 'NONE', *, *, #42263, .T. ) ;
#32090=CARTESIAN_POINT ( 'NONE',  ( 161.4396252346964218, 251.0253620690641299, 14.51972485405798885 ) ) ;
#32092=CARTESIAN_POINT ( 'NONE',  ( 148.7588072053147243, 273.7711778218048835, -8.803803025135483296 ) ) ;
#32093=B_SPLINE_SURFACE_WITH_KNOTS ( 'NONE', 3, 1, ( 
 ( #40443, #87136 ),
 ( #1967, #9579 ),
 ( #55140, #32852 ),
 ( #39433, #85096 ),
 ( #77971, #55634 ),
 ( #54637, #94199 ),
 ( #17668, #24753 ),
 ( #86619, #46539 ),
 ( #69357, #17153 ),
 ( #85616, #38945 ),
 ( #8566, #94693 ),
 ( #8070, #71378 ),
 ( #92695, #63761 ),
 ( #62236, #24262 ),
 ( #69851, #38443 ),
 ( #70352, #47550 ),
 ( #100276, #48051 ),
 ( #31353, #86125 ),
 ( #23246, #1476 ),
 ( #78993, #30862 ),
 ( #25255, #56138 ),
 ( #48566, #16159 ),
 ( #93188, #23743 ),
 ( #47057, #964 ),
 ( #31840, #32357 ),
 ( #63258, #62743 ),
 ( #93699, #16655 ),
 ( #78477, #9064 ),
 ( #57143, #27762 ),
 ( #79507, #18167 ),
 ( #95719, #19188 ),
 ( #66260, #11578 ),
 ( #18672, #2995 ),
 ( #57644, #42436 ) ),
 .UNSPECIFIED., .T., .F., .F.,
 ( 4, 2, 2, 2, 2, 2, 2, 2, 2, 2, 2, 2, 2, 2, 2, 2, 4 ),
 ( 2, 2 ),
 ( 0.000000000000000000, 0.06250000000000000000, 0.1250000000000000000, 0.1875000000000000000, 0.2500000000000000000, 0.3125000000000000000, 0.3750000000000000000, 0.4375000000000000000, 0.5000000000000000000, 0.5625000000000000000, 0.6250000000000000000, 0.6875000000000000000, 0.7500000000000000000, 0.8125000000000000000, 0.8750000000000000000, 0.9375000000000000000, 1.000000000000000000 ),
 ( 0.000000000000000000, 1.000000000000000000 ),
 .UNSPECIFIED. ) ;
#32094=VERTEX_POINT ( 'NONE', #40494 ) ;
#32097=ORIENTED_EDGE ( 'NONE', *, *, #53103, .T. ) ;
#32099=ORIENTED_EDGE ( 'NONE', *, *, #55322, .T. ) ;
#32101=FACE_OUTER_BOUND ( 'NONE', #34222, .T. ) ;
#32102=ORIENTED_EDGE ( 'NONE', *, *, #31342, .T. ) ;
#32103=CARTESIAN_POINT ( 'NONE',  ( 164.4915767550571957, 245.7392269735623529, -6.407198159945809657 ) ) ;
#32104=AXIS2_PLACEMENT_3D ( 'NONE', #43103, #97847, #97357 ) ;
#32106=ADVANCED_FACE ( 'NONE', ( #85670 ), #47101, .T. ) ;
#32109=CARTESIAN_POINT ( 'NONE',  ( 194.3541845315608612, 294.0156730581561533, -14.67567721756631016 ) ) ;
#32111=DIRECTION ( 'NONE',  ( -0.8660254037844359321, -0.5000000000000051070, -0.000000000000000000 ) ) ;
#32114=CIRCLE ( 'NONE', #19213, 5.000000000000023981 ) ;
#32115=CARTESIAN_POINT ( 'NONE',  ( 198.6517795750437472, 276.7950782437291082, -15.35400847641894195 ) ) ;
#32116=CARTESIAN_POINT ( 'NONE',  ( 164.3090168944849836, 246.0554299274959931, 2.641760039552302430 ) ) ;
#32117=CARTESIAN_POINT ( 'NONE',  ( 197.8809552785519656, 287.9071269377202498, 17.61728046362068412 ) ) ;
#32119=FACE_OUTER_BOUND ( 'NONE', #85077, .T. ) ;
#32120=CARTESIAN_POINT ( 'NONE',  ( 168.2393331516044839, 256.9261763197810069, -14.65768061478250139 ) ) ;
#32121=CARTESIAN_POINT ( 'NONE',  ( 159.9470087484377814, 253.6106496594791508, -16.54933891566789939 ) ) ;
#32123=( BOUNDED_CURVE ( )  B_SPLINE_CURVE ( 2, ( #11330, #66491, #96443, #97419, #88870, #58384, #4189, #11818, #12311 ),
 .UNSPECIFIED., .F., .T. ) 
 B_SPLINE_CURVE_WITH_KNOTS ( ( 3, 2, 2, 2, 3 ),
 ( 0.5766129032258064946, 0.5779569892473118697, 0.5806451612903226200, 0.5833333333333333703, 0.5846774193548387455 ),
 .UNSPECIFIED. ) 
 CURVE ( )  GEOMETRIC_REPRESENTATION_ITEM ( )  RATIONAL_B_SPLINE_CURVE ( ( 0.9330127018922194093, 0.9330127018922194093, 1.000000000000000000, 0.8660254037844387076, 1.000000000000000000, 0.8660254037844387076, 1.000000000000000000, 0.9330127018922194093, 0.9330127018922194093 ) ) 
 REPRESENTATION_ITEM ( '' )  );
#32125=CARTESIAN_POINT ( 'NONE',  ( 200.6800100461949228, 283.0590218669948399, 18.32402613046234308 ) ) ;
#32126=CARTESIAN_POINT ( 'NONE',  ( 115.2960263294082068, 225.8262482093458061, 3.021315404115420679E-15 ) ) ;
#32128=CYLINDRICAL_SURFACE ( 'NONE', #68801, 17.82106496071139645 ) ;
#32133=CARTESIAN_POINT ( 'NONE',  ( 18.62362889609498851, 174.8927522451417929, -10.00000000000009059 ) ) ;
#32134=CARTESIAN_POINT ( 'NONE',  ( 88.13101510164368335, 227.8149278399160949, -9.188101187500095079 ) ) ;
#32137=CARTESIAN_POINT ( 'NONE',  ( 174.5189524011659614, 282.4582611793903197, -14.74069674323029666 ) ) ;
#32138=CARTESIAN_POINT ( 'NONE',  ( 166.9710150895549816, 278.2521958780282603, -13.38400322088418015 ) ) ;
#32140=CARTESIAN_POINT ( 'NONE',  ( 5.344833028331274605, 164.7048013555410080, 4.594050593750051981 ) ) ;
#32142=CARTESIAN_POINT ( 'NONE',  ( 161.4726291907278721, 250.9681975403669867, 14.52346149734912117 ) ) ;
#32143=ORIENTED_EDGE ( 'NONE', *, *, #60859, .T. ) ;
#32145=UNCERTAINTY_MEASURE_WITH_UNIT (LENGTH_MEASURE( 1.000000000000000082E-05 ), #88338, 'distance_accuracy_value', 'NONE');
#32148=CARTESIAN_POINT ( 'NONE',  ( 189.0883302520865641, 261.4014440129419086, -6.086672140557672250 ) ) ;
#32149=CARTESIAN_POINT ( 'NONE',  ( 148.3005007218871754, 275.7829932922234093, 6.053100225771809839 ) ) ;
#32151=CARTESIAN_POINT ( 'NONE',  ( 207.5462191418491500, 271.1663988579299485, -5.239401497773396699 ) ) ;
#32153=CARTESIAN_POINT ( 'NONE',  ( 185.0684497205900527, 286.3477220876792444, 16.15350733335134237 ) ) ;
#32155=CARTESIAN_POINT ( 'NONE',  ( 35.79112540406920573, 179.2202760586659736, -5.415160957724236172E-17 ) ) ;
#32156=CARTESIAN_POINT ( 'NONE',  ( 84.29722201641486379, 226.1427522451419065, 10.00000000000009237 ) ) ;
#32157=CARTESIAN_POINT ( 'NONE',  ( 199.6370389866197570, 277.2768894341252235, 15.10745654191603826 ) ) ;
#32160=CARTESIAN_POINT ( 'NONE',  ( 182.1677925300641618, 260.8189200811837622, -10.57058814963136939 ) ) ;
#32161=EDGE_CURVE ( 'NONE', #28264, #42536, #26, .T. ) ;
#32166=CARTESIAN_POINT ( 'NONE',  ( -13.55913805958770624, 162.9786897466781852, -9.594050593750095501 ) ) ;
#32167=CARTESIAN_POINT ( 'NONE',  ( 176.2580550267919932, 278.7780497695933946, -16.99066290002705060 ) ) ;
#32168=CARTESIAN_POINT ( 'NONE',  ( 148.3253847707240141, 273.7398928553401447, -9.074433450356286457 ) ) ;
#32169=CARTESIAN_POINT ( 'NONE',  ( 190.0365785169351227, 262.5605203951380417, 8.321803530341849608 ) ) ;
#32170=CARTESIAN_POINT ( 'NONE',  ( 204.1953342137782954, 276.9703018036655067, 13.84727111424505885 ) ) ;
#32171=CARTESIAN_POINT ( 'NONE',  ( 26.50806851326374414, 176.1115022471901739, -5.000000000000041744 ) ) ;
#32172=CARTESIAN_POINT ( 'NONE',  ( 146.6647111637776106, 276.6162639173599587, -0.6373001129109082674 ) ) ;
#32173=CARTESIAN_POINT ( 'NONE',  ( 189.8147415777049218, 301.8782188922952514, -0.5019643756309712934 ) ) ;
#32175=CARTESIAN_POINT ( 'NONE',  ( 152.3114242215494869, 267.6756387370063521, -15.40863746480569851 ) ) ;
#32176=CARTESIAN_POINT ( 'NONE',  ( 163.8111161534324935, 246.9178193081252743, -7.110480325054721717 ) ) ;
#32178=CARTESIAN_POINT ( 'NONE',  ( 162.1227137712282342, 251.8422180177273901, -14.11218862277787345 ) ) ;
#32179=CARTESIAN_POINT ( 'NONE',  ( 108.9159718882352479, 227.5643266524159856, -9.188101187500093303 ) ) ;
#32183=DIRECTION ( 'NONE',  ( -0.8660254037844387076, -0.4999999999999998890, -0.000000000000000000 ) ) ;
#32184=CARTESIAN_POINT ( 'NONE',  ( 191.5665563241051359, 276.8936798736086757, 16.95695192525134587 ) ) ;
#32185=CARTESIAN_POINT ( 'NONE',  ( 191.3376789240739697, 299.2404140316400003, -7.572576518662374134 ) ) ;
#32186=CARTESIAN_POINT ( 'NONE',  ( 192.0543497034057054, 263.3254378250766763, -4.345169357874051563 ) ) ;
#32187=CARTESIAN_POINT ( 'NONE',  ( 149.1004267900891307, 272.3974806997987343, -12.86882154300063341 ) ) ;
#32188=CARTESIAN_POINT ( 'NONE',  ( 49.38557292990258674, 205.9865022471902876, 10.00000000000009415 ) ) ;
#32189=LINE ( 'NONE', #94037, #74205 ) ;
#32192=CARTESIAN_POINT ( 'NONE',  ( 189.7324944835817178, 265.9585424814845851, 10.76132878117026159 ) ) ;
#32194=CARTESIAN_POINT ( 'NONE',  ( 196.5613103808260860, 267.5413228629882383, 9.637417835835831781 ) ) ;
#32195=EDGE_LOOP ( 'NONE', ( #41557, #22108, #73738, #28119 ) ) ;
#32197=CARTESIAN_POINT ( 'NONE',  ( -22.42236680055709641, 157.8615022471902591, 0.000000000000000000 ) ) ;
#32200=CARTESIAN_POINT ( 'NONE',  ( 172.9438399295877957, 262.8668947608421718, -16.49499919880818766 ) ) ;
#32201=CARTESIAN_POINT ( 'NONE',  ( 192.6224552386041182, 297.0151161785129261, 12.49354144254605181 ) ) ;
#32202=CARTESIAN_POINT ( 'NONE',  ( 190.9225659192872229, 280.7668985173125975, 16.65464037187561175 ) ) ;
#32207=CARTESIAN_POINT ( 'NONE',  ( 164.3996301846870267, 247.3020492865104529, 7.248807534621905191 ) ) ;
#32210=ORIENTED_EDGE ( 'NONE', *, *, #86399, .F. ) ;
#32214=CARTESIAN_POINT ( 'NONE',  ( 204.2133777088835700, 276.9390495533970693, 13.75768580338462144 ) ) ;
#32215=B_SPLINE_CURVE_WITH_KNOTS ( 'NONE', 3,
 ( #94545, #25099, #65958, #21848, #29450, #98375, #67446, #89324, #5650, #52244, #36540, #28963, #35557, #60326, #82210, #98871, #83188, #37044, #91282, #13275, #27480, #58348, #51766, #81210, #35051, #89797, #43134, #11782, #74584, #12781, #20876, #75562, #42642, #6150, #97873, #43646, #44137, #13748, #96909, #75071, #73572, #4154, #19878, #90804, #82708, #36042, #50748, #81701, #12274, #59841, #21359, #74076 ),
 .UNSPECIFIED., .F., .F.,
 ( 4, 2, 2, 2, 2, 2, 2, 2, 2, 2, 2, 2, 2, 2, 2, 2, 2, 2, 2, 2, 2, 2, 2, 2, 2, 4 ),
 ( 0.0001369149182890826025, 0.001149345445623905365, 0.001402453077457536598, 0.001655560709291167831, 0.001782114525207983882, 0.001908668341124799498, 0.002035222157041615115, 0.002161775972958430731, 0.002414883604792085817, 0.002667991236625740469, 0.003174206500293014210, 0.004186637027627614603, 0.005199067554962213261, 0.005705282818629513891, 0.005958390450463124308, 0.006084944266379932985, 0.006211498082296740796, 0.006274774990255143833, 0.006338051898213546871, 0.006464605714130344273, 0.006717713345963950353, 0.007223928609631210217, 0.007477036241464778132, 0.007730143873298345181, 0.007983251505131912229, 0.008236359136965481012 ),
 .UNSPECIFIED. ) ;
#32223=CARTESIAN_POINT ( 'NONE',  ( 175.0525616523904091, 258.5361325477437049, 12.82765623556165835 ) ) ;
#32224=EDGE_LOOP ( 'NONE', ( #99626, #97027, #35624, #45310 ) ) ;
#32227=CARTESIAN_POINT ( 'NONE',  ( 173.2978849248910365, 270.6387814481042255, 17.71865970584200767 ) ) ;
#32231=CARTESIAN_POINT ( 'NONE',  ( 185.1874674929625542, 281.7807588590592331, -16.37341951865305489 ) ) ;
#32232=CARTESIAN_POINT ( 'NONE',  ( 164.7349053118283564, 245.3177695503021027, -2.492200678360605437 ) ) ;
#32233=CARTESIAN_POINT ( 'NONE',  ( 147.9420216129083769, 274.4038973224264168, -6.684832208247039276 ) ) ;
#32234=CARTESIAN_POINT ( 'NONE',  ( 196.0610340319988154, 284.4280829583078685, -17.56065396538383894 ) ) ;
#32236=CARTESIAN_POINT ( 'NONE',  ( 186.4022004759940501, 277.8269278096638004, -17.81691120636144277 ) ) ;
#32237=ADVANCED_FACE ( 'NONE', ( #12622 ), #41494, .T. ) ;
#32239=CARTESIAN_POINT ( 'NONE',  ( 157.9319255052028836, 280.9761857261652267, 2.111273384039783707 ) ) ;
#32240=CARTESIAN_POINT ( 'NONE',  ( 130.8370663736463655, 246.3458772461660544, 9.188101187500095079 ) ) ;
#32241=CARTESIAN_POINT ( 'NONE',  ( 186.9363924785116922, 262.3438794472209565, -10.23320327271459362 ) ) ;
#32244=B_SPLINE_CURVE_WITH_KNOTS ( 'NONE', 3,
 ( #17213, #32918, #9649, #1031, #63822, #85687, #93771, #47117, #9130, #87204, #64324, #31909, #78038, #17736, #54199, #8629, #70941, #1544 ),
 .UNSPECIFIED., .F., .F.,
 ( 4, 2, 2, 2, 2, 2, 2, 2, 4 ),
 ( 1.040834085586084257E-17, 0.0002877161428173316722, 0.0005754322856346529361, 0.0008631484284519741999, 0.001150864571269295464, 0.001438580714086616728, 0.001726296856903937992, 0.002014012999721259255, 0.002301729142538580519 ),
 .UNSPECIFIED. ) ;
#32247=CARTESIAN_POINT ( 'NONE',  ( 111.7912168577913974, 246.8967562850347122, -4.648177544792955347E-16 ) ) ;
#32248=CARTESIAN_POINT ( 'NONE',  ( 180.7877033413244021, 256.2435947011284725, 1.191093872994401393 ) ) ;
#32250=CARTESIAN_POINT ( 'NONE',  ( 190.5440129798993212, 300.2296708901008628, 2.619235206888629541 ) ) ;
#32253=CARTESIAN_POINT ( 'NONE',  ( 169.3277966998927866, 263.8928266120187800, -17.36417683515335142 ) ) ;
#32254=CARTESIAN_POINT ( 'NONE',  ( 148.2098452982477568, 273.9400130919484582, 10.40469228891075026 ) ) ;
#32257=CARTESIAN_POINT ( 'NONE',  ( 148.3629184514745987, 273.6748826132846375, -8.219814532462343948 ) ) ;
#32261=CARTESIAN_POINT ( 'NONE',  ( 157.2721445379966951, 276.7763377113812453, 10.24542939855939849 ) ) ;
#32262=CARTESIAN_POINT ( 'NONE',  ( 151.7267614974901733, 267.8485355488985533, -16.42520090999607874 ) ) ;
#32263=CARTESIAN_POINT ( 'NONE',  ( 190.8072577185990610, 300.1591305089344814, 3.698484652594827171 ) ) ;
#32264=CARTESIAN_POINT ( 'NONE',  ( 14.65434579541631521, 169.2677522451417929, -5.000000000000041744 ) ) ;
#32265=CARTESIAN_POINT ( 'NONE',  ( 161.4920976794100795, 281.5001473778777381, -6.616262511153973236 ) ) ;
#32266=CARTESIAN_POINT ( 'NONE',  ( 153.4834637178363153, 276.1882586661345726, -8.644278876002948309 ) ) ;
#32267=CARTESIAN_POINT ( 'NONE',  ( 200.5039526449628795, 267.3497397166782434, 6.370409075474873006 ) ) ;
#32269=CARTESIAN_POINT ( 'NONE',  ( 147.0538900202505488, 275.9421863647172017, 5.192507380313251986 ) ) ;
#32271=CARTESIAN_POINT ( 'NONE',  ( 157.2948870673828026, 280.9759411348209142, 6.053012778684776940 ) ) ;
#32272=CARTESIAN_POINT ( 'NONE',  ( -22.42236680055709641, 157.8615022471902591, 0.000000000000000000 ) ) ;
#32273=CARTESIAN_POINT ( 'NONE',  ( 187.5025819648600134, 297.9165075386694639, -4.258172756825077343 ) ) ;
#32274=CARTESIAN_POINT ( 'NONE',  ( 204.2143397907769611, 276.5280330293650195, 13.36303585211030054 ) ) ;
#32279=CARTESIAN_POINT ( 'NONE',  ( 86.66977078063996487, 220.8458772461660544, 9.188101187500095079 ) ) ;
#32281=CARTESIAN_POINT ( 'NONE',  ( 192.4212750754384160, 297.3635704425909125, -12.73704185013552248 ) ) ;
#32283=B_SPLINE_CURVE_WITH_KNOTS ( 'NONE', 3,
 ( #99092, #37756, #92025, #76294 ),
 .UNSPECIFIED., .F., .F.,
 ( 4, 4 ),
 ( 0.01312060649816892619, 0.01948601111665982516 ),
 .UNSPECIFIED. ) ;
#32284=CIRCLE ( 'NONE', #1567, 14.82106496071144619 ) ;
#32291=CARTESIAN_POINT ( 'NONE',  ( 189.3775153017087973, 300.6355170167246911, -1.634152055493470757 ) ) ;
#32293=CARTESIAN_POINT ( 'NONE',  ( 161.9230673771116358, 250.1880157158810505, 12.87702452034784883 ) ) ;
#32294=CARTESIAN_POINT ( 'NONE',  ( 169.2311904526189323, 252.2068874694283238, -9.079601461500399040 ) ) ;
#32295=CARTESIAN_POINT ( 'NONE',  ( 161.4297399252889136, 251.4380930145043180, 13.08186051037274922 ) ) ;
#32296=CARTESIAN_POINT ( 'NONE',  ( 157.1837449796689725, 258.3967629017010381, 16.97243084443542216 ) ) ;
#32297=CARTESIAN_POINT ( 'NONE',  ( -5.676897265278508797, 155.9824982072973683, -6.972266317189433020E-16 ) ) ;
#32298=EDGE_CURVE ( 'NONE', #66637, #25284, #96778, .T. ) ;
#32300=CARTESIAN_POINT ( 'NONE',  ( 37.27951979288245354, 183.1423013555409796, -4.594050593750043987 ) ) ;
#32302=CARTESIAN_POINT ( 'NONE',  ( 77.36034478572226192, 203.2202760586659736, -5.415160957724236172E-17 ) ) ;
#32308=CARTESIAN_POINT ( 'NONE',  ( 196.2417448688663626, 269.4613107492011181, -10.73862409626361369 ) ) ;
#32314=CARTESIAN_POINT ( 'NONE',  ( 67.34640541081718368, 215.8149278399160664, -9.188101187500095079 ) ) ;
#32315=CARTESIAN_POINT ( 'NONE',  ( 99.59154365750384841, 216.7592609112380444, 2.679491924311254714 ) ) ;
#32316=CARTESIAN_POINT ( 'NONE',  ( 155.4495868485232108, 261.4004128932040203, -18.48326470492642315 ) ) ;
#32317=CARTESIAN_POINT ( 'NONE',  ( 159.2111180226792726, 254.8852497853115722, 16.01057445397460910 ) ) ;
#32318=CARTESIAN_POINT ( 'NONE',  ( 187.6582181093866382, 259.5698042993466288, -5.491801991258111748 ) ) ;
#32319=CARTESIAN_POINT ( 'NONE',  ( 202.0830002332459117, 280.6289715805018545, 17.37494336322426136 ) ) ;
#32323=CARTESIAN_POINT ( 'NONE',  ( 117.4407359106297974, 228.6115022471901739, -5.000000000000041744 ) ) ;
#32324=CARTESIAN_POINT ( 'NONE',  ( 161.4726291907278721, 250.9681975403669867, 14.52346149734912117 ) ) ;
#32325=CARTESIAN_POINT ( 'NONE',  ( 164.3138894970802824, 246.0469903322357368, -2.642126690130961020 ) ) ;
#32328=CARTESIAN_POINT ( 'NONE',  ( 185.4693431800836549, 271.4295055675165713, 16.77522542003663020 ) ) ;
#32329=ORIENTED_EDGE ( 'NONE', *, *, #29393, .T. ) ;
#32330=CARTESIAN_POINT ( 'NONE',  ( 206.2041691044954348, 273.4908977089264113, -9.455375957961031474 ) ) ;
#32331=FACE_OUTER_BOUND ( 'NONE', #58158, .T. ) ;
#32332=DIRECTION ( 'NONE',  ( -0.8660254037844387076, -0.4999999999999998890, -0.000000000000000000 ) ) ;
#32334=CARTESIAN_POINT ( 'NONE',  ( 177.1640644942122265, 252.7834580030144878, -0.2671950879854613770 ) ) ;
#32336=CARTESIAN_POINT ( 'NONE',  ( 156.6812872898450735, 261.2670451491295012, 0.000000000000000000 ) ) ;
#32338=CARTESIAN_POINT ( 'NONE',  ( 48.93451802855033606, 192.3927522451418213, 10.00000000000009948 ) ) ;
#32339=CARTESIAN_POINT ( 'NONE',  ( 206.9658671503163134, 271.7722489768942182, -5.682263345440972557 ) ) ;
#32349=CARTESIAN_POINT ( 'NONE',  ( 206.5237403681858552, 272.9373840435757188, -10.81420335655575116 ) ) ;
#32350=ORIENTED_EDGE ( 'NONE', *, *, #49738, .F. ) ;
#32351=CARTESIAN_POINT ( 'NONE',  ( 171.5552605186996686, 284.7348010384742452, 10.70351548841014555 ) ) ;
#32355=CARTESIAN_POINT ( 'NONE',  ( 155.3017250444513024, 261.6565170503553190, 18.58368563027307374 ) ) ;
#32356=CARTESIAN_POINT ( 'NONE',  ( 185.4281315057809252, 292.4669413526785888, -10.95545331475209672 ) ) ;
#32357=CARTESIAN_POINT ( 'NONE',  ( 157.1965120183049578, 258.3746497421212780, -18.06591467563559306 ) ) ;
#32358=CARTESIAN_POINT ( 'NONE',  ( 150.1064787036151245, 245.2202760586659167, -5.415160957724236172E-17 ) ) ;
#32361=CARTESIAN_POINT ( 'NONE',  ( 206.4640599017556895, 270.6242529349663073, 2.487210561828315125 ) ) ;
#32363=CARTESIAN_POINT ( 'NONE',  ( 93.00275509369619442, 218.3768266524159856, -9.188101187500091527 ) ) ;
#32365=CARTESIAN_POINT ( 'NONE',  ( 191.4941427383744781, 298.9694107557253346, 8.584406880462095657 ) ) ;
#32373=CARTESIAN_POINT ( 'NONE',  ( 146.5095091551180815, 276.8850816817948726, 0.1418322875769769398 ) ) ;
#32376=CARTESIAN_POINT ( 'NONE',  ( 162.4198556707359842, 249.3275531507180460, 11.06129461055015106 ) ) ;
#32377=CARTESIAN_POINT ( 'NONE',  ( 71.75763553740291911, 221.4244531367911293, -4.594050593750046652 ) ) ;
#32378=VERTEX_POINT ( 'NONE', #10582 ) ;
#32381=B_SPLINE_CURVE_WITH_KNOTS ( 'NONE', 3,
 ( #19528, #50388, #81340, #11914 ),
 .UNSPECIFIED., .F., .F.,
 ( 4, 4 ),
 ( 0.02696644195202606634, 0.03618975469407011841 ),
 .UNSPECIFIED. ) ;
#32382=CARTESIAN_POINT ( 'NONE',  ( 115.4741365526546417, 244.1427522451419350, 10.00000000000009415 ) ) ;
#32383=B_SPLINE_SURFACE_WITH_KNOTS ( 'NONE', 3, 1, ( 
 ( #15567, #53088 ),
 ( #30292, #91624 ),
 ( #46470, #77906 ),
 ( #61180, #84042 ),
 ( #38373, #31279 ),
 ( #93623, #69286 ),
 ( #92147, #77400 ),
 ( #45479, #92626 ),
 ( #22194, #14600 ),
 ( #68781, #62167 ),
 ( #100211, #7478 ),
 ( #8493, #93116 ),
 ( #22700, #76413 ),
 ( #6986, #37871 ),
 ( #39363, #23668 ),
 ( #54560, #53577 ),
 ( #16085, #30797 ),
 ( #85544, #61676 ),
 ( #15076, #46991 ),
 ( #70277, #888 ),
 ( #31767, #45965 ),
 ( #76882, #62671 ),
 ( #24190, #55073 ),
 ( #86059, #16585 ),
 ( #47481, #78405 ),
 ( #8986, #39857 ),
 ( #70792, #1402 ),
 ( #73302, #72313 ),
 ( #56581, #25702 ),
 ( #32281, #94128 ),
 ( #9502, #87055 ),
 ( #41884, #10492 ),
 ( #40864, #48496 ),
 ( #2919, #63688 ) ),
 .UNSPECIFIED., .T., .F., .F.,
 ( 4, 2, 2, 2, 2, 2, 2, 2, 2, 2, 2, 2, 2, 2, 2, 2, 4 ),
 ( 2, 2 ),
 ( 0.000000000000000000, 0.06250000000000000000, 0.1250000000000000000, 0.1875000000000000000, 0.2500000000000000000, 0.3125000000000000000, 0.3750000000000000000, 0.4375000000000000000, 0.5000000000000000000, 0.5625000000000000000, 0.6250000000000000000, 0.6875000000000000000, 0.7500000000000000000, 0.8125000000000000000, 0.8750000000000000000, 0.9375000000000000000, 1.000000000000000000 ),
 ( 0.000000000000000000, 1.000000000000000000 ),
 .UNSPECIFIED. ) ;
#32384=CARTESIAN_POINT ( 'NONE',  ( 163.0424334805279045, 248.2492167524936804, -9.671494865076915914 ) ) ;
#32385=ORIENTED_EDGE ( 'NONE', *, *, #57742, .T. ) ;
#32387=CARTESIAN_POINT ( 'NONE',  ( 183.8301289239822722, 272.2411597453489662, -17.34995410509954183 ) ) ;
#32388=CARTESIAN_POINT ( 'NONE',  ( 187.4250779816339900, 264.0915145022557908, -12.27137290262548852 ) ) ;
#32390=B_SPLINE_CURVE_WITH_KNOTS ( 'NONE', 3,
 ( #77661, #15829, #1149, #46734, #62933, #86299, #16833, #47720, #71058, #32543, #94377, #17333, #69033, #80181, #48754, #71558, #25955, #25434, #81182, #50227, #11749, #33545, #11262, #79686, #2155, #96372, #65431, #10247, #42612, #56827, #26450, #64944, #87813, #96879, #18351, #57325, #88297, #18853, #49734, #80687, #10747, #49244, #40621, #42125, #64441, #57823, #34054, #41623 ),
 .UNSPECIFIED., .F., .F.,
 ( 4, 2, 2, 2, 2, 2, 2, 2, 2, 2, 2, 2, 2, 2, 2, 2, 2, 2, 2, 2, 2, 2, 2, 4 ),
 ( 0.0008566085972837732439, 0.001056739686836194372, 0.001156805231612405152, 0.001256870776388615716, 0.001457001865941131603, 0.001657132955493647707, 0.002057395134598692492, 0.002457657313703737710, 0.003258181671913780008, 0.004058706030123822306, 0.004859230388333865905, 0.005259492567438886837, 0.005459623656991471896, 0.005559689201767801722, 0.005609721974155967503, 0.005659754746544131548, 0.005709787518932297329, 0.005759820291320463109, 0.005859885836096787731, 0.006060016925649376260, 0.006460279104754438825, 0.006860541283859499656, 0.007060672373412010122, 0.007260803462964518853 ),
 .UNSPECIFIED. ) ;
#32391=ORIENTED_EDGE ( 'NONE', *, *, #28791, .T. ) ;
#32394=CARTESIAN_POINT ( 'NONE',  ( 206.1405152101578437, 273.6011494880188479, -9.618815605734603480 ) ) ;
#32395=LINE ( 'NONE', #94234, #20608 ) ;
#32396=LINE ( 'NONE', #86161, #62498 ) ;
#32397=CARTESIAN_POINT ( 'NONE',  ( 109.5562962934610738, 227.3927522451417929, -10.00000000000009237 ) ) ;
#32398=CYLINDRICAL_SURFACE ( 'NONE', #37283, 17.82106496071139645 ) ;
#32400=CARTESIAN_POINT ( 'NONE',  ( 202.8239709173147389, 277.7017072501616894, -15.26945558628286470 ) ) ;
#32401=CARTESIAN_POINT ( 'NONE',  ( 161.5875797534026219, 250.7690973254556468, 12.95526170413129030 ) ) ;
#32403=CARTESIAN_POINT ( 'NONE',  ( 185.0420741367827020, 264.2165883964872251, -12.05581981974006744 ) ) ;
#32405=CARTESIAN_POINT ( 'NONE',  ( 110.8733765985977300, 241.4865022471902876, -10.00000000000009592 ) ) ;
#32406=CARTESIAN_POINT ( 'NONE',  ( 155.3654218642418527, 271.4162630973418686, 14.04413973620215828 ) ) ;
#32408=CARTESIAN_POINT ( 'NONE',  ( 184.2948240331882914, 264.1576318679792053, 13.78297524835661925 ) ) ;
#32409=CARTESIAN_POINT ( 'NONE',  ( 163.1008115941903895, 248.1481028935802442, 11.25332017433677834 ) ) ;
#32410=B_SPLINE_CURVE_WITH_KNOTS ( 'NONE', 3,
 ( #46393, #60594, #16506, #24106 ),
 .UNSPECIFIED., .F., .F.,
 ( 4, 4 ),
 ( 0.001717231910942013280, 0.007031907792270792809 ),
 .UNSPECIFIED. ) ;
#32412=CARTESIAN_POINT ( 'NONE',  ( 164.3138894970802824, 246.0469903322357368, -2.642126690130961020 ) ) ;
#32413=CARTESIAN_POINT ( 'NONE',  ( 180.4856426815808845, 267.2495753203921254, -15.61375793168770620 ) ) ;
#32415=CARTESIAN_POINT ( 'NONE',  ( 199.1239910296074243, 281.8565664318417703, -16.59351424064629654 ) ) ;
#32416=EDGE_CURVE ( 'NONE', #66772, #53637, #45929, .T. ) ;
#32418=CARTESIAN_POINT ( 'NONE',  ( 172.1882770616424239, 274.9807513487110668, 16.44417690625383344 ) ) ;
#32419=CARTESIAN_POINT ( 'NONE',  ( 166.5511016027801361, 286.2022811075372033, -3.211568022117319288 ) ) ;
#32422=CARTESIAN_POINT ( 'NONE',  ( 194.8728601672216598, 266.1307473366540535, -7.448611987400203915 ) ) ;
#32424=CARTESIAN_POINT ( 'NONE',  ( -4.208943576872074210, 174.5024278399160949, 9.188101187500095079 ) ) ;
#32427=EDGE_CURVE ( 'NONE', #42896, #15150, #88373, .T. ) ;
#32431=CARTESIAN_POINT ( 'NONE',  ( 28.72751893051112049, 178.2048013555409796, 4.594050593750051981 ) ) ;
#32432=CARTESIAN_POINT ( 'NONE',  ( 171.4603946439460458, 289.8468835499439251, 4.041829335023700231 ) ) ;
#32435=CARTESIAN_POINT ( 'NONE',  ( 147.2999496562918296, 275.5159985734018164, -0.1418322875769767455 ) ) ;
#32438=CARTESIAN_POINT ( 'NONE',  ( 186.8364736135580699, 295.8946893679862455, -7.705750633037059316 ) ) ;
#32439=EDGE_CURVE ( 'NONE', #20045, #44171, #68904, .T. ) ;
#32440=CARTESIAN_POINT ( 'NONE',  ( 190.7840340658656544, 261.9460261807228676, -1.050979231100866773 ) ) ;
#32441=ADVANCED_FACE ( 'NONE', ( #86630 ), #52061, .T. ) ;
#32443=CARTESIAN_POINT ( 'NONE',  ( 71.90223342829808928, 198.9865022471901739, 1.119607411625061291E-15 ) ) ;
#32444=CARTESIAN_POINT ( 'NONE',  ( 164.4528277499967714, 246.1922880518520458, 1.577904702918717650 ) ) ;
#32446=CARTESIAN_POINT ( 'NONE',  ( 172.8673893914040036, 290.0046394668156040, 5.992580976346847166 ) ) ;
#32447=CARTESIAN_POINT ( 'NONE',  ( 23.55782238408397689, 196.6589784336661637, -6.496448406907675876E-16 ) ) ;
#32450=CARTESIAN_POINT ( 'NONE',  ( 199.0756812798354645, 285.8378008023734083, -18.45377816087746936 ) ) ;
#32454=CARTESIAN_POINT ( 'NONE',  ( 29.55951135474875358, 176.3262482093457777, 3.021315404115420679E-15 ) ) ;
#32455=CARTESIAN_POINT ( 'NONE',  ( 202.6802583809553369, 277.9056299575880757, -15.43640205419024269 ) ) ;
#32456=CARTESIAN_POINT ( 'NONE',  ( 207.0300480714610671, 270.6212163841511256, -1.302876346950213149 ) ) ;
#32458=CARTESIAN_POINT ( 'NONE',  ( 162.8789161433191452, 248.5324370884573568, 9.731756914259689140 ) ) ;
#32459=CARTESIAN_POINT ( 'NONE',  ( 196.8104339078508076, 289.7613243423628546, -16.40335862274955403 ) ) ;
#32460=CARTESIAN_POINT ( 'NONE',  ( 185.5175662163113088, 267.6491969837045986, -14.61920004980039955 ) ) ;
#32468=CARTESIAN_POINT ( 'NONE',  ( 25.04665064082957926, 175.2677522451417929, -5.000000000000041744 ) ) ;
#32469=CARTESIAN_POINT ( 'NONE',  ( 178.7933174507511467, 282.3263610565340969, 15.41595973002548803 ) ) ;
#32470=CARTESIAN_POINT ( 'NONE',  ( 151.3589047706063582, 268.4856820897672378, 14.56544807350869419 ) ) ;
#32471=CARTESIAN_POINT ( 'NONE',  ( 180.5860009740894156, 257.6394960767527778, -7.420540326864959901 ) ) ;
#32472=CARTESIAN_POINT ( 'NONE',  ( 149.4491471355718772, 271.7934793437897270, 11.43912701239353780 ) ) ;
#32476=CARTESIAN_POINT ( 'NONE',  ( 161.8882824960653579, 250.2482648971885340, -13.83574485983625557 ) ) ;
#32479=CARTESIAN_POINT ( 'NONE',  ( 153.0790963368640689, 265.5062228982576471, -17.74594954892339160 ) ) ;
#32481=DIRECTION ( 'NONE',  ( 0.8660254037844395958, 0.4999999999999985567, 0.000000000000000000 ) ) ;
#32483=B_SPLINE_CURVE_WITH_KNOTS ( 'NONE', 3,
 ( #68269, #61662, #31263, #14081 ),
 .UNSPECIFIED., .F., .F.,
 ( 4, 4 ),
 ( 0.009073585509988487535, 0.01733964532496718933 ),
 .UNSPECIFIED. ) ;
#32484=CARTESIAN_POINT ( 'NONE',  ( 157.1002372043759010, 258.5414026113353430, -17.73553732786789539 ) ) ;
#32485=CARTESIAN_POINT ( 'NONE',  ( 98.68587325814904432, 227.7833772461660544, -9.188101187500095079 ) ) ;
#32486=EDGE_CURVE ( 'NONE', #35100, #99896, #99080, .T. ) ;
#32487=CARTESIAN_POINT ( 'NONE',  ( 180.5853021615070872, 287.4186537074930925, -13.97997887675522399 ) ) ;
#32490=CARTESIAN_POINT ( 'NONE',  ( 208.3057440179679531, 269.8508631828800617, 2.969924427282375046 ) ) ;
#32491=B_SPLINE_CURVE_WITH_KNOTS ( 'NONE', 3,
 ( #69140, #30657, #5862, #92483, #23030, #84886, #15426, #46323, #36747, #250, #62023, #54419, #85395, #93990, #41232, #55421, #25557, #17971, #47339, #17449, #47825, #70129, #85917, #39222, #78764, #63046, #39714, #48866, #71677, #8353, #16443, #32138, #24541, #93486, #742, #46846, #78263, #8844, #31626, #55919, #86408, #62525, #79798, #70642, #16939, #24042, #87438, #40228 ),
 .UNSPECIFIED., .F., .F.,
 ( 4, 2, 2, 2, 2, 2, 2, 2, 2, 2, 2, 2, 2, 2, 2, 2, 2, 2, 2, 2, 2, 2, 2, 4 ),
 ( 0.0005932163644935171086, 0.001587166566766770115, 0.001835654117335065207, 0.002084141667903359647, 0.002208385443187456994, 0.002332629218471554342, 0.002456872993755651255, 0.002581116769039748168, 0.002829604319607905566, 0.003078091870176063397, 0.003575066971312377325, 0.004569017173584972655, 0.005562967375857569285, 0.006059942476993858060, 0.006556917578130146834, 0.006681161353414236809, 0.006743283241056252306, 0.006805405128698267803, 0.006929648903982187774, 0.007053892679266107746, 0.007302380229833928607, 0.007550867780401747734, 0.008047842881537415477, 0.008544817982673081486 ),
 .UNSPECIFIED. ) ;
#32495=CARTESIAN_POINT ( 'NONE',  ( 159.4230536986738400, 254.5181664265525683, 16.83068086755798376 ) ) ;
#32498=CARTESIAN_POINT ( 'NONE',  ( 54.51857766514267212, 202.2833772461660828, -9.188101187500095079 ) ) ;
#32501=CARTESIAN_POINT ( 'NONE',  ( -22.42236680055709641, 157.8615022471902591, 0.000000000000000000 ) ) ;
#32502=CARTESIAN_POINT ( 'NONE',  ( 175.4753921014799403, 272.5933248971207945, 16.60100264507961043 ) ) ;
#32504=CARTESIAN_POINT ( 'NONE',  ( 187.8824611759788183, 271.4673514592827246, -16.49468309722856674 ) ) ;
#32506=CARTESIAN_POINT ( 'NONE',  ( 146.8195026170398023, 276.3481572557323034, 4.765869558735466249 ) ) ;
#32509=CARTESIAN_POINT ( 'NONE',  ( 172.9131096068250599, 260.2067844819827087, -13.87985791031445260 ) ) ;
#32510=CARTESIAN_POINT ( 'NONE',  ( 170.7736899422801571, 275.3227619045933920, -16.19396132888206452 ) ) ;
#32512=CARTESIAN_POINT ( 'NONE',  ( 193.2140586456748679, 295.9904290195353269, -12.67640480829088823 ) ) ;
#32513=CARTESIAN_POINT ( 'NONE',  ( 190.4163244163388242, 300.8362468508201459, 4.691083071570470331 ) ) ;
#32514=CARTESIAN_POINT ( 'NONE',  ( 31.36687970962302785, 200.4637435831424739, 2.679491924311251605 ) ) ;
#32515=CARTESIAN_POINT ( 'NONE',  ( 205.8379285891498682, 274.1252448892948905, 10.44730901608240181 ) ) ;
#32518=DIRECTION ( 'NONE',  ( 0.4999999999999998890, -0.8660254037844385966, 0.000000000000000000 ) ) ;
#32519=CARTESIAN_POINT ( 'NONE',  ( 110.7287787077026451, 243.9244531367911293, -4.594050593750046652 ) ) ;
#32521=CARTESIAN_POINT ( 'NONE',  ( 191.8210230231139803, 298.4032374945642232, -8.800268167321144475 ) ) ;
#32523=CARTESIAN_POINT ( 'NONE',  ( 203.4357368910538355, 278.2859629599173559, -16.45855118664066197 ) ) ;
#32524=CARTESIAN_POINT ( 'NONE',  ( 183.2596571801339280, 284.8004292275762168, -14.94647318252461687 ) ) ;
#32527=CARTESIAN_POINT ( 'NONE',  ( 177.9929206047679031, 255.3858926944306234, 4.850379692699073431 ) ) ;
#32528=ORIENTED_EDGE ( 'NONE', *, *, #79413, .F. ) ;
#32530=CARTESIAN_POINT ( 'NONE',  ( 154.6560229494072871, 273.6100238714292914, -13.40105020477086839 ) ) ;
#32531=CARTESIAN_POINT ( 'NONE',  ( 185.9207523352618523, 262.0077436853858330, 9.914687552586279651 ) ) ;
#32532=CARTESIAN_POINT ( 'NONE',  ( 164.9402323277223275, 244.9621327266073081, -1.073314903116530106 ) ) ;
#32533=CARTESIAN_POINT ( 'NONE',  ( 132.2983106946500982, 253.3149278399160949, -9.188101187500095079 ) ) ;
#32534=CARTESIAN_POINT ( 'NONE',  ( 189.6995965464004712, 294.6853058160613159, -12.59856403867662955 ) ) ;
#32535=CARTESIAN_POINT ( 'NONE',  ( 185.7715223625128260, 296.9187202208149756, 4.298953271262141662 ) ) ;
#32536=B_SPLINE_CURVE_WITH_KNOTS ( 'NONE', 3,
 ( #67585, #68084, #59972, #12414, #59467, #35697, #67083, #43281, #74226, #82841, #21984, #99006, #66597, #97521, #14396, #52880, #83830, #89934, #45279, #20513, #12921, #43780, #5303, #28587, #90449, #44281, #22972, #55719, #71966, #95314, #46256, #14876, #9675, #25871, #91933, #18266, #41029, #9153, #49160, #24843, #84330, #15361, #71470, #40029 ),
 .UNSPECIFIED., .F., .F.,
 ( 4, 2, 2, 2, 2, 2, 2, 2, 2, 2, 2, 2, 2, 2, 2, 2, 2, 2, 2, 2, 2, 4 ),
 ( 0.0003194575834195127750, 0.001336248915430739625, 0.001844644581436353159, 0.002098842414439147999, 0.002225941330940528831, 0.002353040247441909663, 0.002607238080444787987, 0.002861435913447666311, 0.003369831579453307167, 0.004386622911464483493, 0.005403414243475661120, 0.005911809909481204398, 0.006166007742483933969, 0.006420205575486663541, 0.006483755033737345283, 0.006547304491988027025, 0.006610853950238708768, 0.006674403408489390510, 0.006928601241492172991, 0.007436996907497737952, 0.007945392573503302913, 0.008453788239508869609 ),
 .UNSPECIFIED. ) ;
#32537=CARTESIAN_POINT ( 'NONE',  ( 188.4211857319924945, 281.8444091920245569, -16.71250961025338810 ) ) ;
#32539=CARTESIAN_POINT ( 'NONE',  ( 40.68897417663616523, 203.4869531367911293, 4.594050593750046652 ) ) ;
#32542=CARTESIAN_POINT ( 'NONE',  ( 171.0832173816872626, 259.7879900724919935, 15.08573027344413653 ) ) ;
#32543=CARTESIAN_POINT ( 'NONE',  ( 151.5918080220145896, 278.2509154019998050, -1.647039589299454043 ) ) ;
#32546=CARTESIAN_POINT ( 'NONE',  ( 156.6119464822673990, 270.4807277697740346, -14.77393801743134105 ) ) ;
#32547=CARTESIAN_POINT ( 'NONE',  ( 122.4745085665788906, 241.5177522451418497, -10.00000000000009592 ) ) ;
#32549=VERTEX_POINT ( 'NONE', #32247 ) ;
#32551=CARTESIAN_POINT ( 'NONE',  ( 163.3706531435203146, 247.6807236201477735, 10.06957846017757241 ) ) ;
#32552=CYLINDRICAL_SURFACE ( 'NONE', #44735, 10.00000000000010658 ) ;
#32553=CARTESIAN_POINT ( 'NONE',  ( 28.37560933628243731, 181.0643266524159856, -9.188101187500093303 ) ) ;
#32556=CARTESIAN_POINT ( 'NONE',  ( 146.8516045228164160, 276.2925551239072774, 3.995954059407343273 ) ) ;
#32559=CARTESIAN_POINT ( 'NONE',  ( 51.46042545625488174, 210.5177522451419065, 5.000000000000046185 ) ) ;
#32560=CARTESIAN_POINT ( 'NONE',  ( 172.1508111218572026, 287.0958522653913860, 7.470856674359275473 ) ) ;
#32561=CARTESIAN_POINT ( 'NONE',  ( 184.6893784852484828, 257.7963074246405313, 1.363638931471332638 ) ) ;
#32562=EDGE_CURVE ( 'NONE', #26502, #35860, #95539, .T. ) ;
#32563=CARTESIAN_POINT ( 'NONE',  ( 205.2660270307054304, 275.1158074454486382, -13.97598661256119179 ) ) ;
#32564=CARTESIAN_POINT ( 'NONE',  ( 162.2294822266495089, 251.8890613771950200, -13.02408023403573978 ) ) ;
#32566=EDGE_CURVE ( 'NONE', #64025, #14234, #54355, .T. ) ;
#32567=CARTESIAN_POINT ( 'NONE',  ( 27.73493783529170997, 173.4865022471901739, 1.119607411625061291E-15 ) ) ;
#32570=CARTESIAN_POINT ( 'NONE',  ( 162.8037981520209314, 248.6625452659484381, 9.809699077002424161 ) ) ;
#32571=CARTESIAN_POINT ( 'NONE',  ( 146.7502831681854332, 255.5333772461660260, 9.188101187500095079 ) ) ;
#32573=CARTESIAN_POINT ( 'NONE',  ( 163.8921714668630045, 247.1588185633375758, 6.247182185919442077 ) ) ;
#32574=CARTESIAN_POINT ( 'NONE',  ( 200.1233510698300222, 282.0231834965481994, 17.42297826929840809 ) ) ;
#32577=CARTESIAN_POINT ( 'NONE',  ( 183.1886578041060716, 257.7166335271973594, -2.049690715180576106 ) ) ;
#32579=ORIENTED_EDGE ( 'NONE', *, *, #56548, .F. ) ;
#32580=CARTESIAN_POINT ( 'NONE',  ( 179.5196496019146650, 266.1175816663657656, 16.29367087753972498 ) ) ;
#32581=CARTESIAN_POINT ( 'NONE',  ( 148.5274394637608282, 249.8927522451417929, -10.00000000000009237 ) ) ;
#32582=CARTESIAN_POINT ( 'NONE',  ( 153.1991487056075130, 277.8144349384043608, -5.978376906038552541 ) ) ;
#32585=CARTESIAN_POINT ( 'NONE',  ( 206.0946696452135427, 273.6805563358039421, -10.19627505985792837 ) ) ;
#32589=CARTESIAN_POINT ( 'NONE',  ( 162.6425574510925003, 248.9418223522047526, -10.70838742014210077 ) ) ;
#32594=DIRECTION ( 'NONE',  ( 0.5000000000000048850, -0.8660254037844358210, 0.000000000000000000 ) ) ;
#32597=CARTESIAN_POINT ( 'NONE',  ( 165.3929592122126451, 286.2279243276498732, 4.432946431554212197 ) ) ;
#32602=EDGE_CURVE ( 'NONE', #44538, #53287, #46000, .T. ) ;
#32603=CARTESIAN_POINT ( 'NONE',  ( 2.117331368781439682, 160.4824982072973683, 3.021315404115420679E-15 ) ) ;
#32604=VERTEX_POINT ( 'NONE', #97098 ) ;
#32605=CARTESIAN_POINT ( 'NONE',  ( 173.9797063438981013, 267.3139811165434594, 17.17281660156877621 ) ) ;
#32607=CARTESIAN_POINT ( 'NONE',  ( 151.0036289208911171, 269.1010379121764799, 14.24595189915657478 ) ) ;
#32612=CARTESIAN_POINT ( 'NONE',  ( 202.6551236945213361, 279.6380246773706517, 15.55476940527561425 ) ) ;
#32613=VERTEX_POINT ( 'NONE', #42825 ) ;
#32617=CARTESIAN_POINT ( 'NONE',  ( 160.8275201602635036, 271.0864152119986556, 16.51521213740326743 ) ) ;
#32618=ORIENTED_EDGE ( 'NONE', *, *, #90867, .F. ) ;
#32625=CARTESIAN_POINT ( 'NONE',  ( 188.9516232634142909, 259.5449388965931234, 2.625812016075142807 ) ) ;
#32627=CARTESIAN_POINT ( 'NONE',  ( 164.5348324038273518, 245.6643059921780718, 1.473102934610569958 ) ) ;
#32628=CARTESIAN_POINT ( 'NONE',  ( 205.7668501412109663, 274.2483563724483133, 11.09689540819876896 ) ) ;
#32629=CARTESIAN_POINT ( 'NONE',  ( 198.1679321590325458, 277.6257778925182720, -16.56331389466651061 ) ) ;
#32631=CARTESIAN_POINT ( 'NONE',  ( 147.3775965199690461, 275.3815102604642675, -3.878554353302192226 ) ) ;
#32633=CARTESIAN_POINT ( 'NONE',  ( 159.8188415394622268, 253.8326417772889840, -15.43862849427313222 ) ) ;
#32636=CARTESIAN_POINT ( 'NONE',  ( 200.8551880497955437, 282.7556046643899776, 18.00894873733387058 ) ) ;
#32637=CARTESIAN_POINT ( 'NONE',  ( -27.42236680055714260, 166.5217562850347406, 1.224646799147364892E-15 ) ) ;
#32638=ORIENTED_EDGE ( 'NONE', *, *, #76713, .F. ) ;
#32639=CARTESIAN_POINT ( 'NONE',  ( 155.0112353102835243, 262.1596600290110359, -17.54170487059483818 ) ) ;
#32640=CARTESIAN_POINT ( 'NONE',  ( 138.9289912384832917, 241.0177522451417929, 5.000000000000051514 ) ) ;
#32641=CARTESIAN_POINT ( 'NONE',  ( -3.297639133650708043, 162.2365022471902023, -10.00000000000009237 ) ) ;
#32643=CARTESIAN_POINT ( 'NONE',  ( 22.44857442947627035, 173.7677522451417929, -5.000000000000041744 ) ) ;
#32644=CARTESIAN_POINT ( 'NONE',  ( 80.71549903385694336, 229.6589784336661353, -6.496448406907676862E-16 ) ) ;
#32647=CARTESIAN_POINT ( 'NONE',  ( 163.1177074157340030, 248.1188384722309195, 11.53923137679231026 ) ) ;
#32648=CARTESIAN_POINT ( 'NONE',  ( 13.13906166239122619, 169.2048013555410080, 4.594050593750051981 ) ) ;
#32650=CARTESIAN_POINT ( 'NONE',  ( 161.3227470381586102, 251.2278010437646856, 14.45097375514160731 ) ) ;
#32653=CARTESIAN_POINT ( 'NONE',  ( 165.9091197491159164, 246.2627970730538323, -2.747640711776688338 ) ) ;
#32654=CARTESIAN_POINT ( 'NONE',  ( 200.9106067213441520, 267.7885642596323805, -3.100825223188956148 ) ) ;
#32658=CARTESIAN_POINT ( 'NONE',  ( 112.1543725048143898, 228.8927522451417929, -10.00000000000009237 ) ) ;
#32660=CARTESIAN_POINT ( 'NONE',  ( 35.81758128034870481, 200.6744531367911293, 4.594050593750047540 ) ) ;
#32661=CARTESIAN_POINT ( 'NONE',  ( 79.60625107924917643, 216.7677522451418497, 10.00000000000009592 ) ) ;
#32662=CARTESIAN_POINT ( 'NONE',  ( 195.9148236425762661, 275.2641294645287076, 15.61648565824300050 ) ) ;
#32668=CARTESIAN_POINT ( 'NONE',  ( -12.00317221093202136, 170.0024278399160949, 9.188101187500095079 ) ) ;
#32669=CARTESIAN_POINT ( 'NONE',  ( 194.3252252352508265, 294.0658320307167628, 14.07225870721148731 ) ) ;
#32670=CARTESIAN_POINT ( 'NONE',  ( 151.1811967613751335, 268.7934813906678642, -15.79361349403328418 ) ) ;
#32672=CARTESIAN_POINT ( 'NONE',  ( 194.9636675848471441, 292.9600174435121289, -15.57898232594655319 ) ) ;
#32673=CARTESIAN_POINT ( 'NONE',  ( 190.6479877716197393, 262.7614712451651826, 8.392489763586285179 ) ) ;
#32674=CARTESIAN_POINT ( 'NONE',  ( 204.6780326111993986, 276.1342436545999703, 14.85609018352459287 ) ) ;
#32676=CARTESIAN_POINT ( 'NONE',  ( 191.8453338867844877, 298.3611298435110371, -9.039024722281077118 ) ) ;
#32677=CARTESIAN_POINT ( 'NONE',  ( 148.3190727836317535, 273.7508255376806119, 8.080277324579027365 ) ) ;
#32678=ORIENTED_EDGE ( 'NONE', *, *, #33382, .T. ) ;
#32680=CARTESIAN_POINT ( 'NONE',  ( 161.6725611998193983, 251.8560077465454299, -13.81138343693815251 ) ) ;
#32681=CARTESIAN_POINT ( 'NONE',  ( 115.2218061334819623, 228.1423013555409796, -4.594050593750043987 ) ) ;
#32684=FACE_OUTER_BOUND ( 'NONE', #54532, .T. ) ;
#32685=CARTESIAN_POINT ( 'NONE',  ( 195.7291534503633272, 291.6341570319625021, 16.44925029361851543 ) ) ;
#32686=CARTESIAN_POINT ( 'NONE',  ( 143.0969038086192597, 260.4263049900483225, -7.951529393128359935 ) ) ;
#32687=CARTESIAN_POINT ( 'NONE',  ( 149.9821146867828929, 276.3814977895287370, -6.888571825090875400 ) ) ;
#32689=CARTESIAN_POINT ( 'NONE',  ( 196.9976074755333286, 289.4371302133026802, -16.79549473444794216 ) ) ;
#32691=CARTESIAN_POINT ( 'NONE',  ( 172.8847284319935795, 290.1773784869942006, -1.864525648362560295 ) ) ;
#32692=CARTESIAN_POINT ( 'NONE',  ( 155.7716105177659927, 262.8426515368366267, -17.72795275872529430 ) ) ;
#32694=CARTESIAN_POINT ( 'NONE',  ( 189.4381674897702794, 265.0040801212285828, 12.03645615491573828 ) ) ;
#32696=CARTESIAN_POINT ( 'NONE',  ( 175.6497225671480749, 278.5846401578337463, 15.45330369560194050 ) ) ;
#32697=CARTESIAN_POINT ( 'NONE',  ( 198.8044191836357584, 269.5069306727704088, 9.250748962204042414 ) ) ;
#32703=CARTESIAN_POINT ( 'NONE',  ( 192.7507137768506880, 296.7929658737652971, 11.30364540927242345 ) ) ;
#32704=ORIENTED_EDGE ( 'NONE', *, *, #19726, .F. ) ;
#32705=ADVANCED_FACE ( 'NONE', ( #56427 ), #10347, .T. ) ;
#32706=CARTESIAN_POINT ( 'NONE',  ( 159.9635946688021022, 268.7707599091479551, -17.14635356962945778 ) ) ;
#32708=CARTESIAN_POINT ( 'NONE',  ( 190.0370014622527322, 286.8089957100377205, 16.96978714573610247 ) ) ;
#32709=ORIENTED_EDGE ( 'NONE', *, *, #39279, .T. ) ;
#32710=CARTESIAN_POINT ( 'NONE',  ( 164.7173348071851819, 279.5549278273611549, 11.88884794519514365 ) ) ;
#32711=CARTESIAN_POINT ( 'NONE',  ( 194.4826705584825390, 293.7931287314651740, -16.11258321617245315 ) ) ;
#32712=CARTESIAN_POINT ( 'NONE',  ( 10.46624461501205872, 188.3967562850346837, -4.648177544792955347E-16 ) ) ;
#32713=ORIENTED_EDGE ( 'NONE', *, *, #84708, .F. ) ;
#32715=CARTESIAN_POINT ( 'NONE',  ( 146.4729408656479563, 243.8262482093457493, 3.021315404115420679E-15 ) ) ;
#32716=CARTESIAN_POINT ( 'NONE',  ( 69.71912771937687126, 204.3927522451418213, 10.00000000000009948 ) ) ;
#32719=CARTESIAN_POINT ( 'NONE',  ( 155.1398527401465230, 261.9368881057492899, -17.02245700497956449 ) ) ;
#32720=VERTEX_POINT ( 'NONE', #1752 ) ;
#32721=( BOUNDED_CURVE ( )  B_SPLINE_CURVE ( 2, ( #76206, #60964, #6782, #68572, #91923, #70568, #78189, #55844, #40661 ),
 .UNSPECIFIED., .F., .T. ) 
 B_SPLINE_CURVE_WITH_KNOTS ( ( 3, 2, 2, 2, 3 ),
 ( 0.4475806451612903136, 0.4489247311827956888, 0.4516129032258064391, 0.4543010752688171894, 0.4556451612903225645 ),
 .UNSPECIFIED. ) 
 CURVE ( )  GEOMETRIC_REPRESENTATION_ITEM ( )  RATIONAL_B_SPLINE_CURVE ( ( 0.9330127018922194093, 0.9330127018922194093, 1.000000000000000000, 0.8660254037844387076, 1.000000000000000000, 0.8660254037844387076, 1.000000000000000000, 0.9330127018922194093, 0.9330127018922194093 ) ) 
 REPRESENTATION_ITEM ( '' )  );
#32723=CARTESIAN_POINT ( 'NONE',  ( 178.4103510133881230, 261.0373811071510772, 12.15853430941466762 ) ) ;
#32726=ORIENTED_EDGE ( 'NONE', *, *, #96221, .F. ) ;
#32727=CARTESIAN_POINT ( 'NONE',  ( 173.0071317692371053, 271.0804120453940413, 16.43005499174315887 ) ) ;
#32729=ORIENTED_EDGE ( 'NONE', *, *, #2265, .F. ) ;
#32730=CARTESIAN_POINT ( 'NONE',  ( 185.3138185638633217, 281.8611869091093354, -16.40392399104547039 ) ) ;
#32732=CARTESIAN_POINT ( 'NONE',  ( 147.9288777062709528, 274.4266632365326473, -6.420914853544658740 ) ) ;
#32733=CARTESIAN_POINT ( 'NONE',  ( 196.3804621193912112, 284.6068645810997850, -17.33595723632800656 ) ) ;
#32735=CARTESIAN_POINT ( 'NONE',  ( 201.1060504099706350, 282.3210983108598384, -18.18000168485860257 ) ) ;
#32737=CARTESIAN_POINT ( 'NONE',  ( 157.9598681688460715, 280.9884947929961072, 2.154129884594043531 ) ) ;
#32738=CARTESIAN_POINT ( 'NONE',  ( 125.9924764494033980, 252.7369531367911293, -4.594050593750048428 ) ) ;
#32741=ADVANCED_FACE ( 'NONE', ( #32119 ), #61763, .F. ) ;
#32742=ORIENTED_EDGE ( 'NONE', *, *, #10635, .T. ) ;
#32745=CARTESIAN_POINT ( 'NONE',  ( 203.6424794855465450, 276.2395053873065649, 13.34248587893602433 ) ) ;
#32746=CARTESIAN_POINT ( 'NONE',  ( 177.7978932797991263, 254.0055511546904654, 1.349567550766762825 ) ) ;
#32747=CARTESIAN_POINT ( 'NONE',  ( 171.8805646714124862, 288.2467586487748576, -4.631873833586762856 ) ) ;
#32748=CARTESIAN_POINT ( 'NONE',  ( 146.7209719250423632, 276.5188174203767062, 3.774014941632788389 ) ) ;
#32750=CARTESIAN_POINT ( 'NONE',  ( 200.9521687275011175, 282.5876292032514243, -18.16013154125647944 ) ) ;
#32751=CARTESIAN_POINT ( 'NONE',  ( 175.0853012839055509, 287.6725234473790351, -9.381267066206161687 ) ) ;
#32752=CARTESIAN_POINT ( 'NONE',  ( 174.9264754436019302, 282.2672310181519606, 14.40274484580208814 ) ) ;
#32753=CARTESIAN_POINT ( 'NONE',  ( 177.2275806558985778, 256.0915070734015444, -7.361266378673213318 ) ) ;
#32755=CARTESIAN_POINT ( 'NONE',  ( 148.3874010092782498, 273.6324775792697892, -8.328854486678444857 ) ) ;
#32756=CARTESIAN_POINT ( 'NONE',  ( 12.05626958406300098, 167.7677522451417929, -5.000000000000041744 ) ) ;
#32759=CARTESIAN_POINT ( 'NONE',  ( 190.6688270659779221, 284.0946164064107506, -17.60360843008351495 ) ) ;
#32760=CARTESIAN_POINT ( 'NONE',  ( 151.9683803660127808, 267.4300393925500998, -16.94882632825642332 ) ) ;
#32761=CARTESIAN_POINT ( 'NONE',  ( 190.6023073677431512, 300.5141149296460981, 3.174888932019753973 ) ) ;
#32762=CARTESIAN_POINT ( 'NONE',  ( 203.0337691736598629, 278.9821914694464340, 16.08167820133810011 ) ) ;
#32763=CARTESIAN_POINT ( 'NONE',  ( 153.5124280503948171, 269.9541434048999804, 14.88175143766969377 ) ) ;
#32764=CARTESIAN_POINT ( 'NONE',  ( 154.9134057170828100, 277.4270410806878999, -8.857178202958200686 ) ) ;
#32766=FACE_OUTER_BOUND ( 'NONE', #87514, .T. ) ;
#32768=CARTESIAN_POINT ( 'NONE',  ( 165.8366156597141696, 280.8532225693821260, -11.02208513961526926 ) ) ;
#32769=CARTESIAN_POINT ( 'NONE',  ( 187.1558864241382594, 261.9731673870204531, -8.720117667986704291 ) ) ;
#32771=CARTESIAN_POINT ( 'NONE',  ( 85.13974472830308571, 208.4155109091896350, 2.679491924311254714 ) ) ;
#32772=CARTESIAN_POINT ( 'NONE',  ( 6.354935675815381657, 181.1427522451419350, 10.00000000000009415 ) ) ;
#32777=CARTESIAN_POINT ( 'NONE',  ( 90.02596631606967037, 210.5327760586659451, 1.948934522072303157E-15 ) ) ;
#32778=CARTESIAN_POINT ( 'NONE',  ( 203.5258219653775313, 278.1299310341851765, -16.21052911601769608 ) ) ;
#32780=CARTESIAN_POINT ( 'NONE',  ( 147.9466025080311624, 275.4568191937016195, 4.863263704339665594 ) ) ;
#32781=CARTESIAN_POINT ( 'NONE',  ( 202.7754741559590173, 279.4295715634463022, -15.65855077192107636 ) ) ;
#32782=VECTOR ( 'NONE', #76736, 1000.000000000000000 ) ;
#32783=B_SPLINE_CURVE_WITH_KNOTS ( 'NONE', 3,
 ( #66542, #81784, #50340, #12868, #97470, #12359, #57941, #28529, #96996, #5247, #19957, #17575, #50834, #20967 ),
 .UNSPECIFIED., .F., .F.,
 ( 4, 2, 2, 2, 2, 2, 4 ),
 ( 0.001073766153608202850, 0.001318213484469830509, 0.001562660815331458168, 0.002051555477054679659, 0.002296002807916289971, 0.002540450138777900716, 0.003029344800501188560 ),
 .UNSPECIFIED. ) ;
#32787=FACE_OUTER_BOUND ( 'NONE', #56307, .T. ) ;
#32788=CARTESIAN_POINT ( 'NONE',  ( 208.1912724900461740, 270.0491336852600170, -0.9856800448607289100 ) ) ;
#32789=CARTESIAN_POINT ( 'NONE',  ( 207.9308153155450611, 270.5002587446924167, 5.985796430201889784 ) ) ;
#32790=CARTESIAN_POINT ( 'NONE',  ( 169.2274513788552497, 252.2158712044186757, -9.272252751866769671 ) ) ;
#32791=CARTESIAN_POINT ( 'NONE',  ( 205.4591571362178968, 274.7812962902297613, -13.63513100400704658 ) ) ;
#32792=CARTESIAN_POINT ( 'NONE',  ( 168.2913993615551078, 273.7323137512423159, 16.83521432247344407 ) ) ;
#32793=EDGE_CURVE ( 'NONE', #86134, #21873, #91934, .T. ) ;
#32799=CARTESIAN_POINT ( 'NONE',  ( 48.78150646083578579, 186.7202760586659736, -5.415160957724236172E-17 ) ) ;
#32803=CARTESIAN_POINT ( 'NONE',  ( 61.79834339388186493, 215.6744531367911293, 4.594050593750047540 ) ) ;
#32806=CARTESIAN_POINT ( 'NONE',  ( 175.5746833524315775, 278.5347786252573314, 16.94864957847115505 ) ) ;
#32810=CARTESIAN_POINT ( 'NONE',  ( 164.2257943664163804, 246.1995755744450776, 2.121218676196017287E-15 ) ) ;
#32811=CARTESIAN_POINT ( 'NONE',  ( 149.1486417047969155, 272.3139700178423368, -11.47583619705022606 ) ) ;
#32812=VERTEX_POINT ( 'NONE', #47576 ) ;
#32814=CARTESIAN_POINT ( 'NONE',  ( 64.07166007881600933, 216.9869531367911293, 4.594050593750046652 ) ) ;
#32816=CARTESIAN_POINT ( 'NONE',  ( -22.42236680055709641, 157.8615022471902591, 0.000000000000000000 ) ) ;
#32817=CARTESIAN_POINT ( 'NONE',  ( 172.8067276174556355, 290.3015201877066147, -0.3301680610896204904 ) ) ;
#32819=CARTESIAN_POINT ( 'NONE',  ( 202.1076200406028818, 280.5863288232868058, 16.88052457987451760 ) ) ;
#32820=CARTESIAN_POINT ( 'NONE',  ( 114.8426596992763962, 247.1115022471903160, -5.000000000000047962 ) ) ;
#32821=CARTESIAN_POINT ( 'NONE',  ( 200.6449165581618956, 283.1198055712825976, 18.35107460171532523 ) ) ;
#32822=CARTESIAN_POINT ( 'NONE',  ( 206.8986117509267899, 272.2880877623646825, 6.975890063856878598 ) ) ;
#32824=CARTESIAN_POINT ( 'NONE',  ( 149.1198674273730660, 273.3870518558833851, -9.828147701528390456 ) ) ;
#32825=CARTESIAN_POINT ( 'NONE',  ( 185.3272745120582101, 271.3634168311705253, 16.73381828275187999 ) ) ;
#32827=CARTESIAN_POINT ( 'NONE',  ( 202.2576150004249200, 280.3265299319959354, 16.24828394350762295 ) ) ;
#32833=CARTESIAN_POINT ( 'NONE',  ( 170.4750202401941408, 250.3351638306627365, 3.406270645389806173 ) ) ;
#32834=CARTESIAN_POINT ( 'NONE',  ( 148.6206126714731397, 275.0791264792570132, 7.693551923222978317 ) ) ;
#32842=CARTESIAN_POINT ( 'NONE',  ( 167.9894996763587756, 276.8290543759245566, 15.53392256876827204 ) ) ;
#32845=VERTEX_POINT ( 'NONE', #88147 ) ;
#32846=CARTESIAN_POINT ( 'NONE',  ( 185.9403311553370770, 296.8630701276886157, 7.448205859860947520 ) ) ;
#32848=CARTESIAN_POINT ( 'NONE',  ( 148.2670916631250861, 273.8408594794321971, -7.980554973576580835 ) ) ;
#32849=CARTESIAN_POINT ( 'NONE',  ( 208.3194307158603067, 269.8271571267425770, -2.120200867047394855 ) ) ;
#32850=CARTESIAN_POINT ( 'NONE',  ( 154.8989000222956349, 262.3542304552891551, 17.41779271305265908 ) ) ;
#32851=CARTESIAN_POINT ( 'NONE',  ( 185.2939906634090619, 292.6913508051172812, -11.83370942357023026 ) ) ;
#32852=CARTESIAN_POINT ( 'NONE',  ( 157.8429099974857195, 257.2550556002704525, -17.85752049034686095 ) ) ;
#32853=CARTESIAN_POINT ( 'NONE',  ( 137.1425535231280151, 259.1744531367911009, 4.594050593750047540 ) ) ;
#32856=VECTOR ( 'NONE', #45765, 1000.000000000000000 ) ;
#32858=CARTESIAN_POINT ( 'NONE',  ( 78.11742282250361313, 228.1589784336661353, -6.496448406907675876E-16 ) ) ;
#32859=ORIENTED_EDGE ( 'NONE', *, *, #66106, .F. ) ;
#32860=CARTESIAN_POINT ( 'NONE',  ( 150.6431064791187850, 269.7254810985950257, 15.11064854015152470 ) ) ;
#32864=CARTESIAN_POINT ( 'NONE',  ( 195.3376996304517945, 292.3121749368662563, -16.73230682301962702 ) ) ;
#32867=CARTESIAN_POINT ( 'NONE',  ( 83.23273246114447943, 208.8615022471902023, 5.000000000000051514 ) ) ;
#32869=CARTESIAN_POINT ( 'NONE',  ( 162.8386403195304410, 249.0994062285972461, 10.29435687412694911 ) ) ;
#32871=CARTESIAN_POINT ( 'NONE',  ( 207.6964130646365163, 270.9062553526738384, 2.975933372805272814 ) ) ;
#32872=CARTESIAN_POINT ( 'NONE',  ( 89.32180003184730310, 228.5024278399160949, 9.188101187500095079 ) ) ;
#32873=ORIENTED_EDGE ( 'NONE', *, *, #14466, .F. ) ;
#32876=CARTESIAN_POINT ( 'NONE',  ( 208.1912724900461740, 270.0491336852600170, -0.9856800448607289100 ) ) ;
#32878=ADVANCED_FACE ( 'NONE', ( #64287 ), #48078, .T. ) ;
#32880=CARTESIAN_POINT ( 'NONE',  ( 165.1988661533298739, 286.0649040768676628, 1.324426972201139918 ) ) ;
#32881=CARTESIAN_POINT ( 'NONE',  ( 110.0998739067015606, 222.8262482093458061, 3.021315404115420679E-15 ) ) ;
#32883=ORIENTED_EDGE ( 'NONE', *, *, #33652, .F. ) ;
#32884=CARTESIAN_POINT ( 'NONE',  ( 188.7025032568610641, 295.1526436589835498, 11.77953644933642430 ) ) ;
#32885=CARTESIAN_POINT ( 'NONE',  ( 158.1484577441942747, 274.4577636394142246, 13.02392648995051161 ) ) ;
#32886=CARTESIAN_POINT ( 'NONE',  ( 159.2713554375903300, 254.7809155221686410, -15.70062444474382168 ) ) ;
#32887=CARTESIAN_POINT ( 'NONE',  ( 155.8082389063325195, 262.2725718350632178, -17.02355505207763287 ) ) ;
#32888=CARTESIAN_POINT ( 'NONE',  ( 177.5742234820266106, 284.9350511118382769, 13.03802085023674628 ) ) ;
#32889=CYLINDRICAL_SURFACE ( 'NONE', #95346, 17.82106496071139645 ) ;
#32890=CARTESIAN_POINT ( 'NONE',  ( 139.7950166422676261, 261.5177522451418781, 5.000000000000046185 ) ) ;
#32891=VERTEX_POINT ( 'NONE', #79536 ) ;
#32892=CARTESIAN_POINT ( 'NONE',  ( 203.6032271198143633, 277.1556831885280303, -14.25317073278892011 ) ) ;
#32893=CARTESIAN_POINT ( 'NONE',  ( 200.7897860911934913, 282.8688841796032420, 18.17522996445731920 ) ) ;
#32895=CARTESIAN_POINT ( 'NONE',  ( 187.8608301704034886, 266.3119843265345708, -12.10641229248959405 ) ) ;
#32897=CARTESIAN_POINT ( 'NONE',  ( 199.4720805209845196, 266.1420231043892954, 4.760232788326643316 ) ) ;
#32898=CARTESIAN_POINT ( 'NONE',  ( 153.1398868314278729, 270.6072410628295302, 13.89127424760058283 ) ) ;
#32900=CARTESIAN_POINT ( 'NONE',  ( 206.8968397926183229, 272.2911568841838061, 7.145103750817420440 ) ) ;
#32901=CARTESIAN_POINT ( 'NONE',  ( 179.4063595725527875, 266.1022058418245706, -14.81063788915213308 ) ) ;
#32902=CARTESIAN_POINT ( 'NONE',  ( 185.6113847613186465, 266.0283385180310347, 13.02359781958079488 ) ) ;
#32903=CARTESIAN_POINT ( 'NONE',  ( 199.2216792767152640, 281.9425204638906166, -16.60457197858584522 ) ) ;
#32907=CARTESIAN_POINT ( 'NONE',  ( 168.7545650535763002, 272.9722043789810186, 15.95301077176753601 ) ) ;
#32908=CARTESIAN_POINT ( 'NONE',  ( 181.5493510114948492, 273.6912172031477439, 16.52691019570659847 ) ) ;
#32910=CARTESIAN_POINT ( 'NONE',  ( 192.0613752418878448, 262.3092312885352158, 2.971550368156713251 ) ) ;
#32911=CARTESIAN_POINT ( 'NONE',  ( 207.7836085030675690, 270.7552284231231852, -5.468305433308493058 ) ) ;
#32912=CARTESIAN_POINT ( 'NONE',  ( -0.5554856785977280165, 179.6744531367911577, 4.594050593750047540 ) ) ;
#32915=EDGE_CURVE ( 'NONE', #63230, #983, #49542, .T. ) ;
#32916=EDGE_CURVE ( 'NONE', #99556, #34648, #4888, .T. ) ;
#32917=AXIS2_PLACEMENT_3D ( 'NONE', #97418, #13313, #52766 ) ;
#32918=CARTESIAN_POINT ( 'NONE',  ( 161.3295519522830830, 253.0809256290032465, -15.05235766421041532 ) ) ;
#32921=CARTESIAN_POINT ( 'NONE',  ( 27.67213724359008964, 174.5327760586659736, 1.948934522072302763E-15 ) ) ;
#32924=CARTESIAN_POINT ( 'NONE',  ( 180.9647783388077755, 293.3161038431775296, 6.181325619054465648 ) ) ;
#32925=CARTESIAN_POINT ( 'NONE',  ( 146.6363376198206652, 276.6654083370839885, -0.5879280619134327202 ) ) ;
#32926=CARTESIAN_POINT ( 'NONE',  ( 196.2967275982209117, 290.6510897708104721, 17.16888829023426055 ) ) ;
#32927=CARTESIAN_POINT ( 'NONE',  ( 6.950328144465094837, 181.4865022471903160, -10.00000000000009592 ) ) ;
#32930=CARTESIAN_POINT ( 'NONE',  ( 186.5128128464827455, 296.3652354721813822, -8.829210103799347564 ) ) ;
#32931=CARTESIAN_POINT ( 'NONE',  ( -27.42236680055714260, 166.5217562850347406, 1.224646799147364892E-15 ) ) ;
#32932=CARTESIAN_POINT ( 'NONE',  ( 90.08876690777130136, 209.4865022471901455, 1.119607411625061291E-15 ) ) ;
#32935=CARTESIAN_POINT ( 'NONE',  ( 203.4000736791844872, 270.0313898409100375, 6.690177824349802904 ) ) ;
#32936=CARTESIAN_POINT ( 'NONE',  ( 48.83545950068980090, 192.8768266524159856, -9.188101187500091527 ) ) ;
#32937=CARTESIAN_POINT ( 'NONE',  ( 190.5217943342473745, 281.4870030958396683, 17.81127109971334121 ) ) ;
#32938=CARTESIAN_POINT ( 'NONE',  ( 204.9345165894207526, 270.9732339236668963, -6.503218611638661883 ) ) ;
#32939=CARTESIAN_POINT ( 'NONE',  ( 151.0801312611820890, 268.9685319718947198, -15.83903210480701240 ) ) ;
#32940=CARTESIAN_POINT ( 'NONE',  ( 144.9863040978925142, 263.1751974929321705, -1.822351119449946140E-15 ) ) ;
#32947=CARTESIAN_POINT ( 'NONE',  ( 162.9148248802443106, 248.4702413316674381, 9.709394404200100581 ) ) ;
#32948=CARTESIAN_POINT ( 'NONE',  ( 196.4783028304046013, 290.3365922432724346, -16.37291435488387492 ) ) ;
#32949=CARTESIAN_POINT ( 'NONE',  ( 189.0300115529333311, 269.8965634406930576, -15.48922461594477795 ) ) ;
#32950=VERTEX_POINT ( 'NONE', #97217 ) ;
#32956=DIRECTION ( 'NONE',  ( -0.8660254037844387076, -0.4999999999999998890, -0.000000000000000000 ) ) ;
#32959=CARTESIAN_POINT ( 'NONE',  ( 149.6071296322179194, 271.5198456328920997, 12.75640156477042453 ) ) ;
#32960=ORIENTED_EDGE ( 'NONE', *, *, #24673, .T. ) ;
#32962=CARTESIAN_POINT ( 'NONE',  ( 189.6192806120793364, 274.1937585566731741, -15.66399881635599201 ) ) ;
#32963=CARTESIAN_POINT ( 'NONE',  ( 151.0960476679098008, 269.3483702054729747, -13.92775656254562300 ) ) ;
#32965=CARTESIAN_POINT ( 'NONE',  ( 152.7729059155601021, 266.0365602647466972, -17.50667083025758686 ) ) ;
#32969=CARTESIAN_POINT ( 'NONE',  ( 157.0877926458200307, 258.5629572190321710, -17.40668770468195703 ) ) ;
#32970=B_SPLINE_CURVE_WITH_KNOTS ( 'NONE', 3,
 ( #26419, #18819, #42586, #64412, #34994, #3145, #34030, #17824, #96347, #73519, #88772, #49703, #95862, #18325, #56801, #48725, #42100, #79657, #80657, #26914, #11236, #73033, #95376, #57794, #3626, #34504, #65406, #25928, #50205, #80155, #94844, #81156, #87293, #11724, #65896, #27419, #25405, #10221, #41089, #72025, #2627, #33516, #87786, #47528 ),
 .UNSPECIFIED., .F., .F.,
 ( 4, 2, 2, 2, 2, 2, 2, 2, 2, 2, 2, 2, 2, 2, 2, 2, 2, 2, 2, 2, 2, 4 ),
 ( 0.0008953238127824564166, 0.0009931015673485474055, 0.001090879321914638286, 0.001188657076480728950, 0.001286434831046820047, 0.001481990340179001591, 0.001677545849311183569, 0.002068656867575712974, 0.002459767885840242162, 0.004024211958898229677, 0.004806433995427187439, 0.005197545013691587390, 0.005393100522823786498, 0.005490878277389886486, 0.005588656031955986474, 0.005637544909239055116, 0.005686433786522122891, 0.005784211541088147418, 0.005979767050220238973, 0.006370878068484379583, 0.006761989086748520193, 0.007153100105012659936 ),
 .UNSPECIFIED. ) ;
#32971=CARTESIAN_POINT ( 'NONE',  ( 102.9345500736427113, 239.4244531367911293, -4.594050593750046652 ) ) ;
#32972=CARTESIAN_POINT ( 'NONE',  ( 148.9322735291567597, 272.6887306911919495, -12.40988026045598858 ) ) ;
#32973=CARTESIAN_POINT ( 'NONE',  ( 183.7864977633626324, 289.5743890241738541, -13.10971297814887215 ) ) ;
#32978=ORIENTED_EDGE ( 'NONE', *, *, #19445, .T. ) ;
#32980=CARTESIAN_POINT ( 'NONE',  ( 159.2554912534056939, 254.8083930951974878, 16.49944922174842432 ) ) ;
#32983=CARTESIAN_POINT ( 'NONE',  ( 66.96803994030899787, 197.2202760586659736, -5.415160957724236172E-17 ) ) ;
#32985=CARTESIAN_POINT ( 'NONE',  ( 191.5694344253287511, 298.8390017285333897, 8.250976118904059575 ) ) ;
#32987=CARTESIAN_POINT ( 'NONE',  ( 176.5111396222833946, 273.2017208239215620, 16.97504237463097709 ) ) ;
#32992=CARTESIAN_POINT ( 'NONE',  ( 177.8586651343115363, 288.9770943732676756, 11.13517240723511392 ) ) ;
#32993=CARTESIAN_POINT ( 'NONE',  ( 170.9811431790156462, 280.9458665424763240, 14.82329785628973440 ) ) ;
#32994=EDGE_LOOP ( 'NONE', ( #69897, #36022, #1988, #42822 ) ) ;
#32995=CARTESIAN_POINT ( 'NONE',  ( 171.7034968969801980, 259.3927777497087277, -13.81093080074480461 ) ) ;
#32996=CARTESIAN_POINT ( 'NONE',  ( 173.8399428679245773, 278.0649905663252639, -16.28034435741132668 ) ) ;
#32998=CYLINDRICAL_SURFACE ( 'NONE', #1426, 17.82106496071139645 ) ;
#32999=CARTESIAN_POINT ( 'NONE',  ( 193.1569697810063531, 296.0893098336876506, -13.02398914535779539 ) ) ;
#33001=CARTESIAN_POINT ( 'NONE',  ( 148.9275518150011806, 272.6969089400084272, 12.34519124974546500 ) ) ;
#33002=CARTESIAN_POINT ( 'NONE',  ( 178.8499588115995209, 270.3591463898502525, 16.16603941770465624 ) ) ;
#33007=CARTESIAN_POINT ( 'NONE',  ( 109.0781781035623226, 233.7833772461660544, -9.188101187500095079 ) ) ;
#33008=ORIENTED_EDGE ( 'NONE', *, *, #8161, .T. ) ;
#33009=CARTESIAN_POINT ( 'NONE',  ( 191.1192699377806719, 299.6187094927299199, -9.526914969203620132 ) ) ;
#33011=CARTESIAN_POINT ( 'NONE',  ( 155.1398527401465230, 261.9368881057492899, -17.02245700497956449 ) ) ;
#33012=EDGE_CURVE ( 'NONE', #58450, #35, #42358, .T. ) ;
#33013=B_SPLINE_CURVE_WITH_KNOTS ( 'NONE', 3,
 ( #56945, #95003, #33157, #41748, #10872, #87931 ),
 .UNSPECIFIED., .F., .F.,
 ( 4, 2, 4 ),
 ( 0.02072061098569386028, 0.02529064359198138212, 0.02986067619826890049 ),
 .UNSPECIFIED. ) ;
#33014=CARTESIAN_POINT ( 'NONE',  ( 182.8075329105516289, 285.5996758505444291, -15.91971760981349071 ) ) ;
#33016=CARTESIAN_POINT ( 'NONE',  ( 174.8677899224096564, 252.9159942513826707, 5.064243870650649626 ) ) ;
#33019=( BOUNDED_CURVE ( )  B_SPLINE_CURVE ( 2, ( #80272, #41714, #11357, #34619, #55895, #57412, #42211, #65031, #88393 ),
 .UNSPECIFIED., .F., .T. ) 
 B_SPLINE_CURVE_WITH_KNOTS ( ( 3, 2, 2, 2, 3 ),
 ( 0.6733870967741935054, 0.6747311827956988806, 0.6774193548387096309, 0.6801075268817203812, 0.6814516129032257563 ),
 .UNSPECIFIED. ) 
 CURVE ( )  GEOMETRIC_REPRESENTATION_ITEM ( )  RATIONAL_B_SPLINE_CURVE ( ( 0.9330127018922194093, 0.9330127018922194093, 1.000000000000000000, 0.8660254037844387076, 1.000000000000000000, 0.8660254037844387076, 1.000000000000000000, 0.9330127018922194093, 0.9330127018922194093 ) ) 
 REPRESENTATION_ITEM ( '' )  );
#33020=CARTESIAN_POINT ( 'NONE',  ( 154.5768095353619174, 273.4844840904814305, -13.32170113451727111 ) ) ;
#33021=CARTESIAN_POINT ( 'NONE',  ( 182.7382853101230182, 260.8451441236999244, 9.502958598710858240 ) ) ;
#33022=CARTESIAN_POINT ( 'NONE',  ( 164.6359882590319899, 245.4890989114802551, -0.8957991669032092652 ) ) ;
#33024=CARTESIAN_POINT ( 'NONE',  ( 150.6386650955079176, 269.7331738006648720, -15.06054658539322766 ) ) ;
#33025=CARTESIAN_POINT ( 'NONE',  ( 188.7422573179599397, 298.9020585943546280, 4.794932212363814727 ) ) ;
#33027=CARTESIAN_POINT ( 'NONE',  ( 61.04057116557046925, 215.2369531367911009, -4.594050593750048428 ) ) ;
#33029=CARTESIAN_POINT ( 'NONE',  ( 205.0716081116550527, 275.4525508911965517, -12.57761053684872188 ) ) ;
#33031=EDGE_CURVE ( 'NONE', #61735, #30468, #60467, .T. ) ;
#33033=CARTESIAN_POINT ( 'NONE',  ( 174.2107174956932454, 262.0554560900756087, 14.36206619626495140 ) ) ;
#33035=CARTESIAN_POINT ( 'NONE',  ( 178.6412003039374383, 292.1250764344173945, -7.162751075077554930 ) ) ;
#33036=CARTESIAN_POINT ( 'NONE',  ( 155.6328838216860220, 261.0829332228125850, -17.51014940606912518 ) ) ;
#33037=CARTESIAN_POINT ( 'NONE',  ( 180.0228151894829978, 262.0024909477526194, 12.25612893952419924 ) ) ;
#33039=CARTESIAN_POINT ( 'NONE',  ( 125.0725847779322351, 243.0177522451418497, -10.00000000000009592 ) ) ;
#33042=ADVANCED_FACE ( 'NONE', ( #91601 ), #54477, .F. ) ;
#33043=CARTESIAN_POINT ( 'NONE',  ( 189.8238368927809745, 301.8624653444729802, -0.3620111495846872751 ) ) ;
#33045=CARTESIAN_POINT ( 'NONE',  ( 30.62142885764206568, 197.6744531367911293, 4.594050593750047540 ) ) ;
#33049=CARTESIAN_POINT ( 'NONE',  ( 190.9559560067148425, 299.9015775189195665, -4.895152914295826108 ) ) ;
#33053=CARTESIAN_POINT ( 'NONE',  ( 66.61587002248265321, 199.2677522451418213, -5.000000000000041744 ) ) ;
#33055=CARTESIAN_POINT ( 'NONE',  ( 121.2656814440110367, 247.4865022471902876, -10.00000000000009592 ) ) ;
#33056=CARTESIAN_POINT ( 'NONE',  ( 181.5287480975334802, 256.6865332137753626, 1.316448668424534452 ) ) ;
#33057=CARTESIAN_POINT ( 'NONE',  ( 204.7237927799493775, 276.0549847173622879, -12.81020997223575364 ) ) ;
#33061=CARTESIAN_POINT ( 'NONE',  ( 36.90037335867700818, 182.1115022471902023, -5.000000000000041744 ) ) ;
#33063=DIRECTION ( 'NONE',  ( 0.8660254037844387076, 0.4999999999999998890, 0.000000000000000000 ) ) ;
#33064=CARTESIAN_POINT ( 'NONE',  ( 162.7561251957091031, 248.7451172484279027, 11.07313294959361194 ) ) ;
#33065=CARTESIAN_POINT ( 'NONE',  ( -12.32793173735119652, 169.8149278399160664, 9.188101187500093303 ) ) ;
#33068=CARTESIAN_POINT ( 'NONE',  ( 169.7667591601442041, 263.3286932583389444, 15.85558928611421159 ) ) ;
#33069=CARTESIAN_POINT ( 'NONE',  ( 192.1640094933931096, 297.8091675017319062, 12.36911124822534447 ) ) ;
#33073=CARTESIAN_POINT ( 'NONE',  ( 186.7082609234106485, 259.3128397857586265, -2.368698930973139216 ) ) ;
#33079=CARTESIAN_POINT ( 'NONE',  ( 166.0359548300953350, 285.6250091532941724, 0.4950489585154529970 ) ) ;
#33081=CARTESIAN_POINT ( 'NONE',  ( 206.9483995484939101, 272.2018527673814106, 9.530154192725417417 ) ) ;
#33086=CARTESIAN_POINT ( 'NONE',  ( 207.6508796976096107, 270.9851214578045528, 6.713685698622268383 ) ) ;
#33089=CARTESIAN_POINT ( 'NONE',  ( 116.9873692804980010, 249.8967562850347122, -4.648177544792955347E-16 ) ) ;
#33090=CARTESIAN_POINT ( 'NONE',  ( 193.8365934467825298, 294.9121671145370556, 14.14845633038902584 ) ) ;
#33093=CARTESIAN_POINT ( 'NONE',  ( 156.2856527893789007, 276.9858201599269591, -10.11406258096672950 ) ) ;
#33095=VERTEX_POINT ( 'NONE', #35763 ) ;
#33097=CARTESIAN_POINT ( 'NONE',  ( 155.4968470730201204, 262.5308716345893458, -17.34543517382400424 ) ) ;
#33104=CARTESIAN_POINT ( 'NONE',  ( 161.8811854682448939, 250.2605573099562264, 13.51112293479948789 ) ) ;
#33105=CARTESIAN_POINT ( 'NONE',  ( 166.1269882802908171, 273.9879501969531930, -15.27021006158703287 ) ) ;
#33108=ORIENTED_EDGE ( 'NONE', *, *, #47274, .T. ) ;
#33109=CARTESIAN_POINT ( 'NONE',  ( 171.1037398668862579, 254.7221107261599684, -11.48652484307285881 ) ) ;
#33110=CARTESIAN_POINT ( 'NONE',  ( 202.9972156839127990, 279.0455039708822937, 16.77197898838388213 ) ) ;
#33113=CARTESIAN_POINT ( 'NONE',  ( 156.7891510251116927, 266.6197213971674955, -16.22205799199115361 ) ) ;
#33122=CARTESIAN_POINT ( 'NONE',  ( 174.5758580735184182, 290.0543502012598651, 6.328980342067771936 ) ) ;
#33127=CARTESIAN_POINT ( 'NONE',  ( 206.0691053506789387, 273.7248349927971844, 11.70564474658248422 ) ) ;
#33128=CARTESIAN_POINT ( 'NONE',  ( 190.9810003742392439, 298.2187262335144737, -9.520436992407670829 ) ) ;
#33129=CARTESIAN_POINT ( 'NONE',  ( 207.0261077644705097, 271.6721741260535623, 5.334318399223184848 ) ) ;
#33130=VERTEX_POINT ( 'NONE', #97114 ) ;
#33132=CARTESIAN_POINT ( 'NONE',  ( 169.0033239945426260, 257.7505650133988411, -14.14853767920301131 ) ) ;
#33138=CARTESIAN_POINT ( 'NONE',  ( 200.1385401540174769, 283.9968752310148830, 17.30012534137638625 ) ) ;
#33139=CARTESIAN_POINT ( 'NONE',  ( 109.6465072765698210, 234.1115022471902307, 10.00000000000009592 ) ) ;
#33141=CARTESIAN_POINT ( 'NONE',  ( 152.5864982446449005, 269.4261691430817791, 15.31489403458886400 ) ) ;
#33144=CARTESIAN_POINT ( 'NONE',  ( 164.3706594650489023, 245.9486618633701482, -1.665857659249071698 ) ) ;
#33145=CARTESIAN_POINT ( 'NONE',  ( 13.35530768973961457, 178.5177522451418497, -10.00000000000009592 ) ) ;
#33146=CARTESIAN_POINT ( 'NONE',  ( 90.05242219234915524, 231.9869531367911293, 4.594050593750046652 ) ) ;
#33150=CARTESIAN_POINT ( 'NONE',  ( 162.9529104326093716, 248.4042752199367214, 11.77079043123004176 ) ) ;
#33151=CARTESIAN_POINT ( 'NONE',  ( 2.773212693257451900, 184.6589784336661637, -6.496448406907675876E-16 ) ) ;
#33152=CARTESIAN_POINT ( 'NONE',  ( 184.1438436585225134, 256.9788754071735184, 3.690260418413948251 ) ) ;
#33155=ORIENTED_EDGE ( 'NONE', *, *, #27698, .F. ) ;
#33156=CARTESIAN_POINT ( 'NONE',  ( 199.0331857822236543, 266.6627783094973552, -2.856755361176172681 ) ) ;
#33157=CARTESIAN_POINT ( 'NONE',  ( 184.6303280917163363, 262.2872244324082089, 12.09539929678677517 ) ) ;
#33158=CARTESIAN_POINT ( 'NONE',  ( 164.4568492923521887, 247.7993767033852919, 8.703614106482779889 ) ) ;
#33159=CARTESIAN_POINT ( 'NONE',  ( 161.6755750489535046, 250.6166850027345276, -13.01404233079112061 ) ) ;
#33163=CARTESIAN_POINT ( 'NONE',  ( 33.89617418964321871, 196.5024278399160949, -9.188101187500093303 ) ) ;
#33164=CARTESIAN_POINT ( 'NONE',  ( 75.63696797857046761, 221.1427522451418781, -10.00000000000009415 ) ) ;
#33165=CARTESIAN_POINT ( 'NONE',  ( 196.3340813134408052, 275.6274763521643649, 15.39790310608117174 ) ) ;
#33170=CARTESIAN_POINT ( 'NONE',  ( 175.2303977473730470, 281.2452381793661402, -14.37900534504002081 ) ) ;
#33173=EDGE_CURVE ( 'NONE', #97169, #73589, #14365, .T. ) ;
#33175=CARTESIAN_POINT ( 'NONE',  ( 207.1432938686257046, 271.8642859028066141, -6.405155839440290322 ) ) ;
#33177=CARTESIAN_POINT ( 'NONE',  ( 194.3011251241114508, 294.1075746476782342, -14.76047579547631905 ) ) ;
#33179=ADVANCED_FACE ( 'NONE', ( #57555 ), #91714, .F. ) ;
#33181=CARTESIAN_POINT ( 'NONE',  ( 204.8189571845487080, 275.8901551335242175, 13.43702398685204358 ) ) ;
#33182=CARTESIAN_POINT ( 'NONE',  ( 146.8637854207107409, 276.2714571898724216, 0.7988785540157756770 ) ) ;
#33183=CARTESIAN_POINT ( 'NONE',  ( 207.4826643481121664, 271.2764789897469768, 7.783310782367018454 ) ) ;
#33184=VERTEX_POINT ( 'NONE', #92004 ) ;
#33185=CARTESIAN_POINT ( 'NONE',  ( 181.1381746692000831, 268.2224384537198034, 15.93641414596886463 ) ) ;
#33186=CARTESIAN_POINT ( 'NONE',  ( 108.5637151982415389, 242.6744531367911293, 4.594050593750047540 ) ) ;
#33190=CARTESIAN_POINT ( 'NONE',  ( 195.7578697689113199, 291.5844189092309193, 17.18796537138345215 ) ) ;
#33192=CARTESIAN_POINT ( 'NONE',  ( 204.4580234391050624, 272.8508129992514455, -9.749047436841882686 ) ) ;
#33193=CARTESIAN_POINT ( 'NONE',  ( 190.1696732520942135, 261.0657627445133357, -4.620374468803995605 ) ) ;
#33194=CARTESIAN_POINT ( 'NONE',  ( 148.9285945872975390, 272.6951028054104427, -12.01265727652413240 ) ) ;
#33195=CARTESIAN_POINT ( 'NONE',  ( 190.2514126175606464, 263.1309047876983414, 9.365642484728958550 ) ) ;
#33196=CARTESIAN_POINT ( 'NONE',  ( 175.7360147442049083, 291.5370265259801386, -1.082392496102676738 ) ) ;
#33197=CARTESIAN_POINT ( 'NONE',  ( 194.6820509838467785, 270.8910309865917156, -14.27696746312268239 ) ) ;
#33198=EDGE_LOOP ( 'NONE', ( #25733, #77587, #22775, #79739, #56495, #36582, #55111, #36069, #7694, #31337, #45527, #82540, #98652, #67839, #27397, #30273, #79920, #95360, #59899, #8301 ) ) ;
#33199=CARTESIAN_POINT ( 'NONE',  ( 189.2480760824234096, 265.7019095893114127, 10.75718835852465283 ) ) ;
#33200=CARTESIAN_POINT ( 'NONE',  ( 176.0605106315991293, 278.7961450278489224, 15.46843456374776338 ) ) ;
#33201=CARTESIAN_POINT ( 'NONE',  ( 165.5220966049394349, 269.3702310919443335, -16.46924383601979258 ) ) ;
#33203=CARTESIAN_POINT ( 'NONE',  ( 200.1971017585360926, 272.2107728627942720, 12.83095891089018536 ) ) ;
#33207=CARTESIAN_POINT ( 'NONE',  ( 148.1271767189874424, 275.1914202840015378, 5.919243137104419183 ) ) ;
#33208=ORIENTED_EDGE ( 'NONE', *, *, #44744, .F. ) ;
#33209=CARTESIAN_POINT ( 'NONE',  ( 190.8416422453866232, 280.8388896373550097, 16.64352526479659744 ) ) ;
#33210=B_SPLINE_SURFACE_WITH_KNOTS ( 'NONE', 3, 1, ( 
 ( #84070, #100236 ),
 ( #52110, #45004 ),
 ( #30820, #21718 ),
 ( #23202, #60691 ),
 ( #45502, #38401 ),
 ( #83559, #90675 ),
 ( #76435, #21231 ),
 ( #37402, #91649 ),
 ( #92172, #74940 ),
 ( #61700, #22216 ),
 ( #14123, #61205 ),
 ( #54093, #75950 ),
 ( #6526, #68308 ),
 ( #99231, #53113 ),
 ( #5524, #7010 ),
 ( #37895, #99731 ),
 ( #22722, #53601 ),
 ( #78947, #79463 ),
 ( #71838, #1925 ),
 ( #54591, #15596 ),
 ( #78434, #32811 ),
 ( #25732, #10027 ),
 ( #56093, #8030 ),
 ( #16611, #39887 ),
 ( #87086, #64213 ),
 ( #63716, #17107 ),
 ( #95164, #17622 ),
 ( #9015, #38903 ),
 ( #920, #23696 ),
 ( #63213, #24220 ),
 ( #48003, #85573 ),
 ( #71333, #93655 ),
 ( #62698, #94155 ),
 ( #55100, #33314 ) ),
 .UNSPECIFIED., .T., .F., .F.,
 ( 4, 2, 2, 2, 2, 2, 2, 2, 2, 2, 2, 2, 2, 2, 2, 2, 4 ),
 ( 2, 2 ),
 ( 0.000000000000000000, 0.06250000000000000000, 0.1250000000000000000, 0.1875000000000000000, 0.2500000000000000000, 0.3125000000000000000, 0.3750000000000000000, 0.4375000000000000000, 0.5000000000000000000, 0.5625000000000000000, 0.6250000000000000000, 0.6875000000000000000, 0.7500000000000000000, 0.8125000000000000000, 0.8750000000000000000, 0.9375000000000000000, 1.000000000000000000 ),
 ( 0.000000000000000000, 1.000000000000000000 ),
 .UNSPECIFIED. ) ;
#33212=CARTESIAN_POINT ( 'NONE',  ( 195.3690366949981296, 290.3742493059416461, -16.73554728058864427 ) ) ;
#33214=CARTESIAN_POINT ( 'NONE',  ( 164.8655127169167827, 279.6105928571379309, 11.86288285680936383 ) ) ;
#33216=CARTESIAN_POINT ( 'NONE',  ( 147.8163551302855296, 274.6215580551378821, -9.286329195885331345 ) ) ;
#33217=CARTESIAN_POINT ( 'NONE',  ( 108.1850894041355957, 243.2677522451419065, -5.000000000000047962 ) ) ;
#33223=CARTESIAN_POINT ( 'NONE',  ( 154.8833801513861772, 262.3811116602312268, -17.49275566389638215 ) ) ;
#33224=ORIENTED_EDGE ( 'NONE', *, *, #30034, .F. ) ;
#33225=VERTEX_POINT ( 'NONE', #45825 ) ;
#33227=ORIENTED_EDGE ( 'NONE', *, *, #79064, .F. ) ;
#33233=CARTESIAN_POINT ( 'NONE',  ( 164.8012313184158018, 245.2028895370295913, -2.462952685407667097 ) ) ;
#33234=CARTESIAN_POINT ( 'NONE',  ( 147.6842102149426239, 274.8504397624737408, -5.874512262071210245 ) ) ;
#33236=CARTESIAN_POINT ( 'NONE',  ( 192.4663556654298588, 297.2854885702906245, -12.98646995774174684 ) ) ;
#33237=CARTESIAN_POINT ( 'NONE',  ( 152.8328714238065515, 265.9326969577624027, -16.29536156676786263 ) ) ;
#33240=EDGE_CURVE ( 'NONE', #14896, #38420, #32491, .T. ) ;
#33241=CARTESIAN_POINT ( 'NONE',  ( 154.0522741418830606, 280.1392850030782711, 2.230978122590827617 ) ) ;
#33242=CARTESIAN_POINT ( 'NONE',  ( 128.2389901622930495, 244.8458772461660544, 9.188101187500095079 ) ) ;
#33246=ORIENTED_EDGE ( 'NONE', *, *, #88434, .T. ) ;
#33249=ORIENTED_EDGE ( 'NONE', *, *, #74474, .F. ) ;
#33250=CARTESIAN_POINT ( 'NONE',  ( 203.5065352982886111, 276.4905705151080042, 13.85652113363879323 ) ) ;
#33251=CARTESIAN_POINT ( 'NONE',  ( 177.6229113889583573, 253.4088548334622146, 1.384122540242602950 ) ) ;
#33252=CARTESIAN_POINT ( 'NONE',  ( 172.9134852821738093, 290.3302075368507076, -5.008290383854661521 ) ) ;
#33253=CARTESIAN_POINT ( 'NONE',  ( 146.8702612584350220, 276.2602407099124662, 4.074116067346697179 ) ) ;
#33254=CARTESIAN_POINT ( 'NONE',  ( 156.0507216674837707, 279.5060275253360373, 7.618106348741741307 ) ) ;
#33256=CARTESIAN_POINT ( 'NONE',  ( 164.0241303531365702, 249.6968001490059237, 11.40766388789279517 ) ) ;
#33258=CARTESIAN_POINT ( 'NONE',  ( 171.8643346617544125, 280.1325139634143966, 13.88504993119007125 ) ) ;
#33259=ADVANCED_FACE ( 'NONE', ( #2268 ), #70699, .F. ) ;
#33260=CARTESIAN_POINT ( 'NONE',  ( 177.1425110050965088, 256.0051583568908313, -7.288962701963175306 ) ) ;
#33262=CARTESIAN_POINT ( 'NONE',  ( 194.3177355571849318, 294.0788045336591381, -15.93712594727561616 ) ) ;
#33263=CARTESIAN_POINT ( 'NONE',  ( 152.6922851986468572, 273.5033374046732888, 11.91467210813521582 ) ) ;
#33264=VERTEX_POINT ( 'NONE', #58433 ) ;
#33265=CARTESIAN_POINT ( 'NONE',  ( 163.9394958709336549, 277.9080926337546771, 13.13436882728932886 ) ) ;
#33266=CARTESIAN_POINT ( 'NONE',  ( 205.1070472173078940, 268.9988147858434786, -3.031129214391079518 ) ) ;
#33267=CARTESIAN_POINT ( 'NONE',  ( 192.1051365471491579, 297.9111384358179180, -10.71776918011019220 ) ) ;
#33269=CARTESIAN_POINT ( 'NONE',  ( 162.8789161433191452, 248.5324370884573568, 9.731756914259689140 ) ) ;
#33270=CARTESIAN_POINT ( 'NONE',  ( 153.5196858120735044, 269.9415063994401294, 14.50335029241602491 ) ) ;
#33271=CARTESIAN_POINT ( 'NONE',  ( 151.6355143709362494, 275.0870865548936877, -8.630920780667789671 ) ) ;
#33272=CARTESIAN_POINT ( 'NONE',  ( 201.0356089830534643, 282.4431064412383989, -18.18835788025466371 ) ) ;
#33274=VECTOR ( 'NONE', #57743, 1000.000000000000114 ) ;
#33275=CARTESIAN_POINT ( 'NONE',  ( 12.39361081041026580, 166.4155109091896065, 2.679491924311254714 ) ) ;
#33279=CARTESIAN_POINT ( 'NONE',  ( 192.0963028965829551, 297.9264387674147656, 11.34530024772836754 ) ) ;
#33281=CARTESIAN_POINT ( 'NONE',  ( 155.6126298223767890, 261.1180141786725244, 18.15400560664037855 ) ) ;
#33282=EDGE_CURVE ( 'NONE', #68650, #83827, #50594, .T. ) ;
#33283=CARTESIAN_POINT ( 'NONE',  ( -10.94779052401099051, 173.6744531367911293, 4.594050593750047540 ) ) ;
#33284=CARTESIAN_POINT ( 'NONE',  ( 94.73480590126506229, 219.3768266524160140, 9.188101187500098632 ) ) ;
#33285=CARTESIAN_POINT ( 'NONE',  ( 155.2922060645262263, 261.6730044072216401, -16.98884022075611355 ) ) ;
#33290=CARTESIAN_POINT ( 'NONE',  ( 162.1709154337574716, 282.3874689244844376, 5.612144347381637033 ) ) ;
#33293=CARTESIAN_POINT ( 'NONE',  ( 161.9199371792244619, 250.1934373776594214, 14.05412690039883827 ) ) ;
#33296=CARTESIAN_POINT ( 'NONE',  ( 167.0271109968743417, 287.8086958075197686, 0.5416428030073258126 ) ) ;
#33297=CARTESIAN_POINT ( 'NONE',  ( 187.3225869936034371, 268.9281182169409590, 15.57271238421296289 ) ) ;
#33299=CARTESIAN_POINT ( 'NONE',  ( 207.8431546909062320, 270.6520914003897360, -6.441273666418043220 ) ) ;
#33301=CARTESIAN_POINT ( 'NONE',  ( 50.26990084964904071, 190.6423013555410080, -4.594050593750043987 ) ) ;
#33303=CARTESIAN_POINT ( 'NONE',  ( 66.20992061623260838, 209.0333772461660544, 9.188101187500095079 ) ) ;
#33304=CARTESIAN_POINT ( 'NONE',  ( 161.2133744761260061, 251.4172398781588811, -14.30368667312104058 ) ) ;
#33306=CARTESIAN_POINT ( 'NONE',  ( 106.6154183633243377, 222.3615022471902023, 5.000000000000051514 ) ) ;
#33308=CARTESIAN_POINT ( 'NONE',  ( 200.2812248566589801, 283.7497380765769890, 17.06302258474581990 ) ) ;
#33309=EDGE_CURVE ( 'NONE', #29501, #90465, #27567, .T. ) ;
#33314=CARTESIAN_POINT ( 'NONE',  ( 149.2923684163597784, 272.0650280510108701, -12.99082738998495756 ) ) ;
#33315=VERTEX_POINT ( 'NONE', #12361 ) ;
#33317=CARTESIAN_POINT ( 'NONE',  ( 81.74442484449845381, 211.8768266524160140, 9.188101187500096856 ) ) ;
#33319=CARTESIAN_POINT ( 'NONE',  ( 170.0999411130123633, 288.2716680735795194, -1.080197458295449442 ) ) ;
#33321=CARTESIAN_POINT ( 'NONE',  ( 153.6322440704845178, 264.5481429195353371, 18.09763679434087180 ) ) ;
#33326=CARTESIAN_POINT ( 'NONE',  ( 190.1285921677634008, 286.6309046793794550, 16.34626960247791772 ) ) ;
#33327=CARTESIAN_POINT ( 'NONE',  ( 121.4100190113083784, 254.2365022471903728, 2.944929066748280225E-16 ) ) ;
#33328=CARTESIAN_POINT ( 'NONE',  ( 12.05626958406292104, 187.7677522451419065, -5.000000000000047962 ) ) ;
#33329=B_SPLINE_CURVE_WITH_KNOTS ( 'NONE', 3,
 ( #52736, #6661, #29951, #4673, #37539, #5169, #35564, #59848, #36048, #66951, #66464, #97880, #28453, #91289 ),
 .UNSPECIFIED., .F., .F.,
 ( 4, 2, 2, 2, 2, 2, 4 ),
 ( 0.0008442750654606336752, 0.001116754662652982583, 0.001389234259845331275, 0.001661713857037679966, 0.001934193454230028874, 0.002479152648614570999, 0.003024111842999113123 ),
 .UNSPECIFIED. ) ;
#33332=CARTESIAN_POINT ( 'NONE',  ( 187.4913029195216438, 273.0290542173935933, 15.64619952351353760 ) ) ;
#33334=CARTESIAN_POINT ( 'NONE',  ( 163.4216610345155800, 247.5923753613567442, 10.58669027323842826 ) ) ;
#33336=CARTESIAN_POINT ( 'NONE',  ( 201.4066285247549786, 281.8004817444100354, -17.79749223817309201 ) ) ;
#33339=ORIENTED_EDGE ( 'NONE', *, *, #36803, .F. ) ;
#33341=CARTESIAN_POINT ( 'NONE',  ( 171.1596004093629517, 249.5938752278392485, 2.804888548739752352 ) ) ;
#33348=CARTESIAN_POINT ( 'NONE',  ( 168.1217531603526538, 276.7950771177830234, 15.34514958204382573 ) ) ;
#33353=CARTESIAN_POINT ( 'NONE',  ( 183.0914503401605202, 295.7967818983725010, 0.7459396247526526302 ) ) ;
#33355=CARTESIAN_POINT ( 'NONE',  ( 194.9819925439454664, 292.9282776833073285, -15.33279721168237586 ) ) ;
#33357=CARTESIAN_POINT ( 'NONE',  ( 194.5047661587782386, 293.7548580291293092, 14.86680123054176583 ) ) ;
#33358=CARTESIAN_POINT ( 'NONE',  ( 159.6209877835443081, 264.4662034727394371, 17.77637312803328129 ) ) ;
#33360=CARTESIAN_POINT ( 'NONE',  ( 207.4651458030734830, 271.3068219998286850, -3.821411492560412793 ) ) ;
#33361=CARTESIAN_POINT ( 'NONE',  ( 204.0632701483897620, 269.1718737286272471, 2.454364474035033883 ) ) ;
#33363=CARTESIAN_POINT ( 'NONE',  ( 84.07169456928664886, 219.3458772461660544, 9.188101187500095079 ) ) ;
#33365=CARTESIAN_POINT ( 'NONE',  ( 150.0459203272414470, 271.3762512067029320, 12.15191700100081640 ) ) ;
#33367=VERTEX_POINT ( 'NONE', #29055 ) ;
#33368=CYLINDRICAL_SURFACE ( 'NONE', #81841, 17.82106496071139645 ) ;
#33372=CARTESIAN_POINT ( 'NONE',  ( 191.0724301404414689, 299.6998384015373063, -9.342134220577969828 ) ) ;
#33376=CARTESIAN_POINT ( 'NONE',  ( 207.6821401748263156, 270.9309767229963768, 1.759036204183980878 ) ) ;
#33377=CARTESIAN_POINT ( 'NONE',  ( 95.05956542768421969, 219.5643266524160140, 9.188101187500095079 ) ) ;
#33378=EDGE_LOOP ( 'NONE', ( #58879, #48936, #32102, #39905 ) ) ;
#33381=CARTESIAN_POINT ( 'NONE',  ( 200.4117560436087047, 283.5236514288079093, -18.06783071421079612 ) ) ;
#33382=EDGE_CURVE ( 'NONE', #59249, #59130, #68722, .T. ) ;
#33388=CARTESIAN_POINT ( 'NONE',  ( -3.532187684056935062, 168.7677522451418781, 10.00000000000009592 ) ) ;
#33393=CARTESIAN_POINT ( 'NONE',  ( 160.5038987594522837, 275.6177743208444326, 12.83085644997012409 ) ) ;
#33394=FACE_OUTER_BOUND ( 'NONE', #64131, .T. ) ;
#33395=CARTESIAN_POINT ( 'NONE',  ( 190.0534303668326288, 269.9073674132432643, 15.26070177760127322 ) ) ;
#33396=CARTESIAN_POINT ( 'NONE',  ( 153.2283961777204695, 265.2476279883323400, -17.66880461074566000 ) ) ;
#33398=CARTESIAN_POINT ( 'NONE',  ( 104.2158063034569579, 237.6427522451419065, -10.00000000000009592 ) ) ;
#33400=EDGE_LOOP ( 'NONE', ( #92809, #78985, #16815, #33208 ) ) ;
#33401=CARTESIAN_POINT ( 'NONE',  ( 6.228640307978117185, 167.7365022471902307, 10.00000000000009948 ) ) ;
#33402=CARTESIAN_POINT ( 'NONE',  ( 161.4726291907278721, 250.9681975403669867, 14.52346149734912117 ) ) ;
#33406=CARTESIAN_POINT ( 'NONE',  ( 116.2138665886018458, 231.2365022471901739, -10.00000000000009237 ) ) ;
#33407=CARTESIAN_POINT ( 'NONE',  ( 163.1811051052586663, 248.0090304528921195, -11.35285691990875456 ) ) ;
#33408=VERTEX_POINT ( 'NONE', #8238 ) ;
#33411=CARTESIAN_POINT ( 'NONE',  ( 164.4440639631384045, 245.8215215431751233, -2.910115319305802029 ) ) ;
#33412=CARTESIAN_POINT ( 'NONE',  ( 178.2835513063369888, 265.3754860723226443, -14.94893715224946540 ) ) ;
#33413=CARTESIAN_POINT ( 'NONE',  ( 184.4647054688699370, 266.0064431806318908, 13.20040557144585414 ) ) ;
#33414=CARTESIAN_POINT ( 'NONE',  ( 199.1948953252038734, 281.7345316833016113, -16.58223543088974949 ) ) ;
#33417=CARTESIAN_POINT ( 'NONE',  ( 171.9427383041699215, 274.8029616261534329, 16.32014694790107256 ) ) ;
#33418=CARTESIAN_POINT ( 'NONE',  ( 180.7206978303440508, 273.1106064130323148, 17.40382843373642530 ) ) ;
#33419=CARTESIAN_POINT ( 'NONE',  ( 161.0071479579559082, 273.4094594936241833, -15.40207120388050832 ) ) ;
#33421=CARTESIAN_POINT ( 'NONE',  ( 191.7224207879665983, 261.3713821052344883, 3.085656737073688483 ) ) ;
#33423=CARTESIAN_POINT ( 'NONE',  ( 4.992923434102598534, 167.5643266524160140, -9.188101187500093303 ) ) ;
#33427=CARTESIAN_POINT ( 'NONE',  ( 175.2159268917944530, 255.4244057975548685, 8.238669877113455442 ) ) ;
#33430=CARTESIAN_POINT ( 'NONE',  ( 33.92367135321775606, 181.2048013555409796, 4.594050593750051981 ) ) ;
#33432=CARTESIAN_POINT ( 'NONE',  ( 164.4678285797544106, 245.7803600197737524, -6.875991496205872799 ) ) ;
#33435=CARTESIAN_POINT ( 'NONE',  ( 179.0573227211665426, 291.9330542595874363, 6.082073241091874749 ) ) ;
#33436=CARTESIAN_POINT ( 'NONE',  ( 98.68481039724036918, 239.3297689869269220, -2.679491924311252493 ) ) ;
#33441=CARTESIAN_POINT ( 'NONE',  ( 93.62503730655774348, 214.8615022471902023, 5.000000000000051514 ) ) ;
#33443=B_SPLINE_CURVE_WITH_KNOTS ( 'NONE', 3,
 ( #60961, #84320, #99494, #37658 ),
 .UNSPECIFIED., .F., .F.,
 ( 4, 4 ),
 ( 0.02269224187031961687, 0.02872765270316010588 ),
 .UNSPECIFIED. ) ;
#33444=CARTESIAN_POINT ( 'NONE',  ( 161.8799941797769293, 267.8308235043324430, -16.86646120607376531 ) ) ;
#33445=CARTESIAN_POINT ( 'NONE',  ( 47.42782112377506820, 204.3149278399160664, 9.188101187500093303 ) ) ;
#33446=CARTESIAN_POINT ( 'NONE',  ( 159.2511875226268216, 254.8158473755685520, 15.75855490706745599 ) ) ;
#33454=DIRECTION ( 'NONE',  ( 0.8660254037844395958, 0.4999999999999985567, 0.000000000000000000 ) ) ;
#33456=CARTESIAN_POINT ( 'NONE',  ( 95.76410038128526026, 214.5494855054052152, -2.679491924311248496 ) ) ;
#33458=CARTESIAN_POINT ( 'NONE',  ( 202.4900219881211854, 279.9239892212719383, 15.63116161057562259 ) ) ;
#33459=CARTESIAN_POINT ( 'NONE',  ( 149.3253462891332219, 272.0079086998416074, -12.99539319630191336 ) ) ;
#33469=CARTESIAN_POINT ( 'NONE',  ( 178.7520316380132499, 282.5168896195049228, 15.81395202663239274 ) ) ;
#33471=CARTESIAN_POINT ( 'NONE',  ( 151.0036289208911171, 269.1010379121764799, 14.24595189915657478 ) ) ;
#33472=CARTESIAN_POINT ( 'NONE',  ( 177.3441421416205799, 256.1034110073948113, -7.247860626662943062 ) ) ;
#33477=CARTESIAN_POINT ( 'NONE',  ( 174.6568604941508340, 274.7935765301870674, 17.62145267448687846 ) ) ;
#33479=CARTESIAN_POINT ( 'NONE',  ( 200.6985908945154335, 283.0268388936558495, -17.74173253065502820 ) ) ;
#33483=CARTESIAN_POINT ( 'NONE',  ( 157.3198323354746435, 258.1610526871778006, -16.77630483474704093 ) ) ;
#33484=CARTESIAN_POINT ( 'NONE',  ( 112.9752924205922824, 236.0333772461660544, 9.188101187500095079 ) ) ;
#33485=B_SPLINE_CURVE_WITH_KNOTS ( 'NONE', 3,
 ( #95508, #25547, #56929, #73649 ),
 .UNSPECIFIED., .F., .F.,
 ( 4, 4 ),
 ( 0.04392709020753635812, 0.04887066958154935581 ),
 .UNSPECIFIED. ) ;
#33486=B_SPLINE_CURVE_WITH_KNOTS ( 'NONE', 3,
 ( #46361, #70170, #31171, #60071 ),
 .UNSPECIFIED., .F., .F.,
 ( 4, 4 ),
 ( 0.02479711570197204798, 0.03404299025597421618 ),
 .UNSPECIFIED. ) ;
#33487=CARTESIAN_POINT ( 'NONE',  ( 182.7250377612010936, 287.9595840865778769, -13.19241888926224071 ) ) ;
#33491=CARTESIAN_POINT ( 'NONE',  ( 207.5290616128274337, 271.1961165699281651, 2.604679844609484984 ) ) ;
#33494=CARTESIAN_POINT ( 'NONE',  ( -22.42236680055709641, 157.8615022471902591, 0.000000000000000000 ) ) ;
#33496=CARTESIAN_POINT ( 'NONE',  ( 68.45643432912224569, 201.1423013555409796, -4.594050593750043987 ) ) ;
#33498=CARTESIAN_POINT ( 'NONE',  ( 150.7530568467738590, 269.5350414755053521, 15.60317050893315916 ) ) ;
#33499=CARTESIAN_POINT ( 'NONE',  ( 150.7108765041139691, 269.6080999720726936, 13.72660302980452407 ) ) ;
#33509=CARTESIAN_POINT ( 'NONE',  ( 173.8979489505312586, 277.9637680410879170, -15.96371148716977117 ) ) ;
#33510=CARTESIAN_POINT ( 'NONE',  ( 162.2240457438445560, 259.4344955095195360, -16.32888341801637111 ) ) ;
#33513=CARTESIAN_POINT ( 'NONE',  ( 148.9230895364621574, 272.7046378331555161, 12.20434325797056019 ) ) ;
#33514=CARTESIAN_POINT ( 'NONE',  ( 180.8902496232956310, 271.3945185957094282, 16.78426242912689403 ) ) ;
#33515=CARTESIAN_POINT ( 'NONE',  ( 164.3939401533646958, 245.9083385283718712, 2.844462461176849200 ) ) ;
#33516=CARTESIAN_POINT ( 'NONE',  ( 168.1332551043281285, 255.5560320396268423, 13.96088319188761950 ) ) ;
#33519=CARTESIAN_POINT ( 'NONE',  ( 118.1714448432989144, 239.0333772461660544, 9.188101187500095079 ) ) ;
#33524=CARTESIAN_POINT ( 'NONE',  ( 204.7235752877335244, 276.0553614249301972, 14.82397698933823271 ) ) ;
#33527=ORIENTED_EDGE ( 'NONE', *, *, #54999, .F. ) ;
#33529=CARTESIAN_POINT ( 'NONE',  ( 157.9584063519955635, 274.6739674095948658, -12.56162459328316316 ) ) ;
#33530=CARTESIAN_POINT ( 'NONE',  ( 147.7269416596823248, 275.9539214970327521, 2.717771182133930541 ) ) ;
#33531=CARTESIAN_POINT ( 'NONE',  ( 182.0644918927315814, 260.4883331680307492, 9.524347663358822658 ) ) ;
#33533=CARTESIAN_POINT ( 'NONE',  ( 137.3322569020296555, 250.0958772461660544, -9.188101187500095079 ) ) ;
#33534=CARTESIAN_POINT ( 'NONE',  ( 57.23161641937174693, 215.3967562850347122, -4.648177544792955347E-16 ) ) ;
#33536=CARTESIAN_POINT ( 'NONE',  ( 59.38997056143013964, 205.0958772461660828, -9.188101187500095079 ) ) ;
#33538=AXIS2_PLACEMENT_3D ( 'NONE', #26258, #25770, #10059 ) ;
#33539=CARTESIAN_POINT ( 'NONE',  ( 207.6628070930962906, 270.9644626028195376, 7.378217122120054761 ) ) ;
#33540=CARTESIAN_POINT ( 'NONE',  ( 157.8820657059571033, 257.1872359237914338, -17.60412210594719440 ) ) ;
#33541=CARTESIAN_POINT ( 'NONE',  ( 174.4320096083763190, 251.4713395514856416, 3.621238935830661365 ) ) ;
#33543=CARTESIAN_POINT ( 'NONE',  ( 165.6871908161093643, 250.8440145507587715, 11.60328334000779726 ) ) ;
#33544=CARTESIAN_POINT ( 'NONE',  ( 171.3957680990430390, 259.8009312154816257, 15.34336344307106792 ) ) ;
#33545=CARTESIAN_POINT ( 'NONE',  ( 154.8275264459192613, 279.3822692668657623, -1.584013062148165396 ) ) ;
#33546=CARTESIAN_POINT ( 'NONE',  ( 154.4470374439381146, 277.6591429590598068, -9.115886381272481742 ) ) ;
#33547=CARTESIAN_POINT ( 'NONE',  ( 155.1398527401465230, 261.9368881057492899, -17.02245700497956449 ) ) ;
#33550=CARTESIAN_POINT ( 'NONE',  ( 127.7428297729342717, 237.8927522451417929, -10.00000000000009059 ) ) ;
#33552=ORIENTED_EDGE ( 'NONE', *, *, #67444, .F. ) ;
#33556=CARTESIAN_POINT ( 'NONE',  ( 48.78150646083578579, 186.7202760586659736, -5.415160957724236172E-17 ) ) ;
#33560=DIRECTION ( 'NONE',  ( -0.8660254037844387076, -0.4999999999999998890, -0.000000000000000000 ) ) ;
#33561=CARTESIAN_POINT ( 'NONE',  ( 190.8683709797118411, 300.0532792356709706, -4.461919767133968762 ) ) ;
#33563=B_SPLINE_CURVE_WITH_KNOTS ( 'NONE', 3,
 ( #64007, #25513, #40188, #71128 ),
 .UNSPECIFIED., .F., .F.,
 ( 4, 4 ),
 ( 0.007140653581439226905, 0.01527480993219123249 ),
 .UNSPECIFIED. ) ;
#33565=CARTESIAN_POINT ( 'NONE',  ( 52.39861964368801495, 214.3927522451419634, 2.944929066748280225E-16 ) ) ;
#33566=CARTESIAN_POINT ( 'NONE',  ( 173.9238158565421770, 289.3171369187040227, 8.002423422717384938 ) ) ;
#33567=CARTESIAN_POINT ( 'NONE',  ( 184.7990890438850329, 257.6713462901447542, 1.377030906181146097 ) ) ;
#33568=CARTESIAN_POINT ( 'NONE',  ( 157.6036818288543486, 257.6694109429415107, -16.73826488331764395 ) ) ;
#33571=CARTESIAN_POINT ( 'NONE',  ( 45.99364009841357159, 197.3615022471902591, -10.00000000000009592 ) ) ;
#33572=CARTESIAN_POINT ( 'NONE',  ( 185.0682636646367314, 294.3875985914592661, 9.867065237507818054 ) ) ;
#33575=CARTESIAN_POINT ( 'NONE',  ( 8.375921941576814689, 166.4548013555410080, -4.594050593750042211 ) ) ;
#33577=CARTESIAN_POINT ( 'NONE',  ( 164.3996301846870267, 247.3020492865104529, 7.248807534621905191 ) ) ;
#33583=CARTESIAN_POINT ( 'NONE',  ( 186.9451997612131038, 258.7018344183949807, -2.460581910096537150 ) ) ;
#33584=CARTESIAN_POINT ( 'NONE',  ( 149.2923684163597784, 272.0650280510108701, -12.99082738998495756 ) ) ;
#33587=CARTESIAN_POINT ( 'NONE',  ( 153.9505496568006322, 278.0639657297674034, -5.205343530163337284 ) ) ;
#33589=CARTESIAN_POINT ( 'NONE',  ( 160.3910089434251347, 252.8416187631903824, 14.67024385955689780 ) ) ;
#33590=CARTESIAN_POINT ( 'NONE',  ( 153.2359015056687781, 277.7311577273633247, -5.083231879104856965 ) ) ;
#33592=CARTESIAN_POINT ( 'NONE',  ( 206.3018347371251195, 273.3217358710584790, -9.309724106897926177 ) ) ;
#33593=CARTESIAN_POINT ( 'NONE',  ( 54.51751480423398988, 213.8297689869269220, -2.679491924311252493 ) ) ;
#33595=CARTESIAN_POINT ( 'NONE',  ( 192.8323852661406761, 296.6515067047851062, 11.86505947732313615 ) ) ;
#33596=CARTESIAN_POINT ( 'NONE',  ( 164.9335952247126045, 244.9736285262353306, -1.661461410667423255 ) ) ;
#33599=CARTESIAN_POINT ( 'NONE',  ( 154.9226727788713731, 262.3130548330639726, 18.22497199616848818 ) ) ;
#33600=VERTEX_POINT ( 'NONE', #48230 ) ;
#33602=CARTESIAN_POINT ( 'NONE',  ( 158.5416719719927130, 277.8521597524036792, -9.836060501838524317 ) ) ;
#33611=AXIS2_PLACEMENT_3D ( 'NONE', #71049, #9230, #79677 ) ;
#33613=VERTEX_POINT ( 'NONE', #61913 ) ;
#33614=CARTESIAN_POINT ( 'NONE',  ( 175.1183745746886871, 267.9007702990796247, 17.47926410801357022 ) ) ;
#33615=CARTESIAN_POINT ( 'NONE',  ( 206.4768661561222984, 273.0185725604343361, 11.39716120335626925 ) ) ;
#33617=CARTESIAN_POINT ( 'NONE',  ( 151.4268868568842379, 274.9972536827360159, -8.604776644755594006 ) ) ;
#33620=CARTESIAN_POINT ( 'NONE',  ( 172.0721957670934898, 256.4003672175040833, -11.61734053971215452 ) ) ;
#33621=ORIENTED_EDGE ( 'NONE', *, *, #73853, .T. ) ;
#33623=CARTESIAN_POINT ( 'NONE',  ( 158.5402111638430824, 267.6492219652220683, -16.22994191499176608 ) ) ;
#33627=ADVANCED_FACE ( 'NONE', ( #23921 ), #71051, .T. ) ;
#33629=( BOUNDED_CURVE ( )  B_SPLINE_CURVE ( 2, ( #43998, #6017, #15098, #29817, #75433, #29326, #30318, #98240, #52602 ),
 .UNSPECIFIED., .F., .T. ) 
 B_SPLINE_CURVE_WITH_KNOTS ( ( 3, 2, 2, 2, 3 ),
 ( 0.004032258064516129788, 0.005376344086021505805, 0.008064516129032257841, 0.01075268817204301161, 0.01209677419354838676 ),
 .UNSPECIFIED. ) 
 CURVE ( )  GEOMETRIC_REPRESENTATION_ITEM ( )  RATIONAL_B_SPLINE_CURVE ( ( 0.9330127018922194093, 0.9330127018922194093, 1.000000000000000000, 0.8660254037844387076, 1.000000000000000000, 0.8660254037844387076, 1.000000000000000000, 0.9330127018922192983, 0.9330127018922194093 ) ) 
 REPRESENTATION_ITEM ( '' )  );
#33630=CARTESIAN_POINT ( 'NONE',  ( 159.0888396382809447, 259.5703526363064384, 16.71962710754473491 ) ) ;
#33631=CARTESIAN_POINT ( 'NONE',  ( 193.4506777133003368, 295.5805927723682203, 14.77919976000363000 ) ) ;
#33632=CARTESIAN_POINT ( 'NONE',  ( 188.1412547211656943, 273.5593357346770063, 17.08033167198486879 ) ) ;
#33634=CARTESIAN_POINT ( 'NONE',  ( 192.0331311261993790, 298.0358554833232461, 11.82583305898340953 ) ) ;
#33635=CARTESIAN_POINT ( 'NONE',  ( -17.42236680055705023, 149.2012482093457777, 0.000000000000000000 ) ) ;
#33637=CARTESIAN_POINT ( 'NONE',  ( 196.9412859255907620, 289.5346819993642953, -17.37273023188612342 ) ) ;
#33642=CARTESIAN_POINT ( 'NONE',  ( 205.7639495959071212, 274.2533802642843170, 10.79039487422292432 ) ) ;
#33643=CARTESIAN_POINT ( 'NONE',  ( 149.3629284598386278, 271.9428144707212027, -12.99253781774931049 ) ) ;
#33644=CARTESIAN_POINT ( 'NONE',  ( 164.6241018286200699, 245.5096868128744632, 3.031483545445131433 ) ) ;
#33645=CARTESIAN_POINT ( 'NONE',  ( 206.8251824619401873, 271.5843563996517673, 6.058312812321095642 ) ) ;
#33648=VERTEX_POINT ( 'NONE', #79678 ) ;
#33650=CARTESIAN_POINT ( 'NONE',  ( 146.8463403758815389, 276.3016728938570736, -2.700094491758966875 ) ) ;
#33651=CARTESIAN_POINT ( 'NONE',  ( 171.5219099648802796, 259.6759708972976455, -14.96685982020008332 ) ) ;
#33652=EDGE_CURVE ( 'NONE', #8187, #70225, #92006, .T. ) ;
#33653=CARTESIAN_POINT ( 'NONE',  ( 163.7831042501927072, 247.9065475540300554, 8.386170005195905830 ) ) ;
#33655=CARTESIAN_POINT ( 'NONE',  ( 200.7897860911934913, 282.8688841796032420, 18.17522996445731920 ) ) ;
#33656=CARTESIAN_POINT ( 'NONE',  ( 191.0099562606770860, 262.1165538832237303, -0.7421737651540062375 ) ) ;
#33657=ORIENTED_EDGE ( 'NONE', *, *, #62596, .F. ) ;
#33659=CIRCLE ( 'NONE', #36885, 14.82106496071144619 ) ;
#33661=CARTESIAN_POINT ( 'NONE',  ( 19.34531673258195639, 188.6427522451419350, 10.00000000000009237 ) ) ;
#33662=CARTESIAN_POINT ( 'NONE',  ( 99.38934535084139554, 234.3149278399160949, 9.188101187500093303 ) ) ;
#33665=CARTESIAN_POINT ( 'NONE',  ( 207.5772549350081988, 271.1126432873252838, 2.658056670308439617 ) ) ;
#33666=CARTESIAN_POINT ( 'NONE',  ( 18.36166996137734841, 193.6589784336661637, -6.496448406907675876E-16 ) ) ;
#33669=B_SPLINE_CURVE_WITH_KNOTS ( 'NONE', 3,
 ( #80822, #79808, #74179, #75658 ),
 .UNSPECIFIED., .F., .F.,
 ( 4, 4 ),
 ( 0.0009145195436546301338, 0.001503970514818383109 ),
 .UNSPECIFIED. ) ;
#33670=ORIENTED_EDGE ( 'NONE', *, *, #2265, .T. ) ;
#33671=CARTESIAN_POINT ( 'NONE',  ( 185.8137939302156099, 260.3527139192792106, -5.808480177743201800 ) ) ;
#33674=CARTESIAN_POINT ( 'NONE',  ( 195.1546726974473245, 264.9111313380191177, -4.390412657300894139 ) ) ;
#33677=CARTESIAN_POINT ( 'NONE',  ( 33.57176175898906934, 184.0643266524159856, -9.188101187500093303 ) ) ;
#33678=CARTESIAN_POINT ( 'NONE',  ( 79.60625107924913380, 226.7677522451419350, -5.000000000000047962 ) ) ;
#33679=AXIS2_PLACEMENT_3D ( 'NONE', #46633, #77558, #39020 ) ;
#33681=B_SPLINE_CURVE_WITH_KNOTS ( 'NONE', 3,
 ( #23324, #15725, #54211, #85179 ),
 .UNSPECIFIED., .F., .F.,
 ( 4, 4 ),
 ( 0.01724406098665899612, 0.02362940485487354664 ),
 .UNSPECIFIED. ) ;
#33683=B_SPLINE_CURVE_WITH_KNOTS ( 'NONE', 3,
 ( #78113, #8703, #98928, #29506, #60383, #31987, #1109, #40582, #10213, #2620, #63897, #9205, #40078, #9728, #70494, #1623, #47683, #39571, #94835, #71023, #24402, #64908, #64404, #10711, #32509, #95367, #49694, #2113, #25398, #80146, #3138, #55277, #25920, #41588, #63401, #32995, #62893, #78618, #55769, #56286, #87284, #87778, #71523, #93848, #17815, #86257, #48716, #18810, #79647, #18314 ),
 .UNSPECIFIED., .F., .F.,
 ( 4, 2, 2, 2, 2, 2, 2, 2, 2, 2, 2, 2, 2, 2, 2, 2, 2, 2, 2, 2, 2, 2, 2, 2, 4 ),
 ( 0.001348966706550652024, 0.001814384599846849324, 0.002279802493143046407, 0.002512511439791146033, 0.002628865913115252008, 0.002745220386439358416, 0.002861574859763464391, 0.002977929333087570365, 0.003210638279735712926, 0.003676056173031953811, 0.004141474066328193829, 0.005072309852920743253, 0.006003145639513294413, 0.006468563532809569125, 0.006933981426105842970, 0.007050335899429947643, 0.007108513136091999113, 0.007166690372754051450, 0.007283044846078170001, 0.007399399319402288552, 0.007632108266050384275, 0.007864817212698478263, 0.008097526159346574853, 0.008330235105994669709, 0.008795652999290947890 ),
 .UNSPECIFIED. ) ;
#33684=CARTESIAN_POINT ( 'NONE',  ( 178.7559403991110969, 259.1783237468100083, -10.26446977356301815 ) ) ;
#33687=CARTESIAN_POINT ( 'NONE',  ( -2.124636079309504488, 160.3923013555410080, 4.594050593750050204 ) ) ;
#33690=CARTESIAN_POINT ( 'NONE',  ( 199.1216527653377000, 285.7581758537840528, -18.37739894744384728 ) ) ;
#33691=CARTESIAN_POINT ( 'NONE',  ( 186.8532369007405691, 282.7788865962135105, 16.19183947954036285 ) ) ;
#33692=CARTESIAN_POINT ( 'NONE',  ( 147.4563929227680603, 275.2450308873625886, -3.847749617713808412 ) ) ;
#33695=CARTESIAN_POINT ( 'NONE',  ( 204.5133713884061706, 276.4194452585140311, 14.87364779308245843 ) ) ;
#33696=CARTESIAN_POINT ( 'NONE',  ( 146.5095091551180815, 276.8850816817948726, 0.1418322875769769398 ) ) ;
#33697=CARTESIAN_POINT ( 'NONE',  ( 164.4781197247689306, 245.7625352337404649, -1.511762618280499515 ) ) ;
#33698=VERTEX_POINT ( 'NONE', #17324 ) ;
#33699=CIRCLE ( 'NONE', #59551, 17.82106496071138224 ) ;
#33700=CARTESIAN_POINT ( 'NONE',  ( -9.864998445682774175, 175.1115022471903160, -5.000000000000047962 ) ) ;
#33701=CARTESIAN_POINT ( 'NONE',  ( 161.3862585056135686, 251.5213894571381559, -13.16453305755435288 ) ) ;
#33702=CARTESIAN_POINT ( 'NONE',  ( 123.0160347675418677, 232.6423013555409796, -4.594050593750043987 ) ) ;
#33708=CARTESIAN_POINT ( 'NONE',  ( 196.1241105319816143, 290.9500712997905794, 15.97146679939154268 ) ) ;
#33709=CARTESIAN_POINT ( 'NONE',  ( 190.6266536543345467, 300.4719459242942321, -7.634394059267482824 ) ) ;
#33711=CARTESIAN_POINT ( 'NONE',  ( 189.6469694556133163, 261.3224043400873029, -4.488274779931007430 ) ) ;
#33714=CARTESIAN_POINT ( 'NONE',  ( 176.2137180456981582, 292.6001369887544001, -1.126497586118241578 ) ) ;
#33717=CARTESIAN_POINT ( 'NONE',  ( 189.2133311240501428, 265.6839626369376788, 10.75809594643768818 ) ) ;
#33718=B_SPLINE_CURVE_WITH_KNOTS ( 'NONE', 3,
 ( #66329, #97261, #66818, #51111 ),
 .UNSPECIFIED., .F., .F.,
 ( 4, 4 ),
 ( 0.02587343813425229538, 0.03511505140344501480 ),
 .UNSPECIFIED. ) ;
#33719=CARTESIAN_POINT ( 'NONE',  ( 175.7664583004113581, 278.6328268015002436, 15.45987238875895642 ) ) ;
#33720=CARTESIAN_POINT ( 'NONE',  ( 168.0773408278945737, 271.5331236227465297, -17.46290692964277369 ) ) ;
#33726=CARTESIAN_POINT ( 'NONE',  ( 150.5916768389222682, 278.2969151622902473, -4.257825285333056330E-05 ) ) ;
#33727=AXIS2_PLACEMENT_3D ( 'NONE', #27576, #57446, #19969 ) ;
#33729=CARTESIAN_POINT ( 'NONE',  ( 191.0828858044439187, 280.5038866170701226, 16.76379900847850735 ) ) ;
#33734=CARTESIAN_POINT ( 'NONE',  ( 194.6356465353167948, 293.5281665672507643, -16.13180903283129197 ) ) ;
#33738=CARTESIAN_POINT ( 'NONE',  ( 187.0283284352577482, 292.0378153221775506, 12.26537691906332661 ) ) ;
#33739=CARTESIAN_POINT ( 'NONE',  ( 150.6931560952953646, 269.6387926204777727, 14.65021044537114037 ) ) ;
#33743=CARTESIAN_POINT ( 'NONE',  ( 189.4317935910015933, 300.3290466316845482, 3.295136749739974835 ) ) ;
#33744=CARTESIAN_POINT ( 'NONE',  ( 35.77629671259011701, 179.9155109091896065, 2.679491924311254714 ) ) ;
#33749=CARTESIAN_POINT ( 'NONE',  ( 178.4554328054981056, 260.9870558088289272, 12.11472630447901544 ) ) ;
#33752=VERTEX_POINT ( 'NONE', #82173 ) ;
#33753=CARTESIAN_POINT ( 'NONE',  ( 173.0740556585676870, 271.0053932585017265, 16.44676307064808185 ) ) ;
#33754=CARTESIAN_POINT ( 'NONE',  ( 155.6328838216860220, 261.0829332228125850, -17.51014940606912518 ) ) ;
#33759=CARTESIAN_POINT ( 'NONE',  ( 161.9362388422072740, 277.2664551573698759, -12.85986196030900075 ) ) ;
#33760=CARTESIAN_POINT ( 'NONE',  ( 193.1977289678065404, 296.0187128512746995, -12.37159405312863925 ) ) ;
#33762=CARTESIAN_POINT ( 'NONE',  ( 201.4617167010348737, 281.7050662241970826, -17.43131506460443703 ) ) ;
#33766=CARTESIAN_POINT ( 'NONE',  ( 154.4124318019600821, 279.5684750503268106, 2.145998202272423327 ) ) ;
#33768=CARTESIAN_POINT ( 'NONE',  ( 136.0332187963529975, 249.3458772461660544, 9.188101187500095079 ) ) ;
#33769=ORIENTED_EDGE ( 'NONE', *, *, #6687, .F. ) ;
#33774=EDGE_CURVE ( 'NONE', #49648, #77284, #65150, .T. ) ;
#33777=B_SPLINE_CURVE_WITH_KNOTS ( 'NONE', 3,
 ( #3224, #2211, #87381, #55861, #78205, #85863, #16390, #25492, #71111, #8792, #1712, #79245, #95458, #49301, #48300, #39661, #33093, #47281, #70585, #40678, #86352, #71616, #63989, #33602, #94931, #56385, #17910, #41174, #2715, #11322, #59355, #18915, #28474, #73116, #34586, #50283, #4697, #35082, #81726, #20401, #88862, #65986, #11810, #36071, #42181, #75100, #95943, #12812, #44164, #82236, #3707, #97409, #65486, #27978 ),
 .UNSPECIFIED., .F., .F.,
 ( 4, 2, 2, 2, 2, 2, 2, 2, 2, 2, 2, 2, 2, 2, 2, 2, 2, 2, 2, 2, 2, 2, 2, 2, 2, 2, 4 ),
 ( 0.0006796803024578544411, 0.0008900614930580021296, 0.001100442683658149710, 0.001205633278958223500, 0.001310823874258297290, 0.001416014469558371080, 0.001521205064858445087, 0.001731586255458504413, 0.001941967446058563956, 0.002362729827258603678, 0.003204254589658812793, 0.004045779352059021908, 0.004887304114459229722, 0.005308066495659372226, 0.005518447686259440009, 0.005623638281559479105, 0.005676233579209463524, 0.005728828876859447077, 0.005781424174509430629, 0.005834019472159414181, 0.005939210067459516594, 0.006149591258059718818, 0.006570353639260159695, 0.006780734829860449522, 0.006991116020460741085, 0.007201497211061031779, 0.007411878401661323341 ),
 .UNSPECIFIED. ) ;
#33778=CARTESIAN_POINT ( 'NONE',  ( 174.4636408308574005, 253.7873770250515406, -9.029445656122202735 ) ) ;
#33782=CARTESIAN_POINT ( 'NONE',  ( 153.7897413227238701, 277.0882903415827627, 7.164246204486259373 ) ) ;
#33783=CARTESIAN_POINT ( 'NONE',  ( 200.7694952279801157, 282.9040289856181403, -17.94628235092568502 ) ) ;
#33785=CARTESIAN_POINT ( 'NONE',  ( 171.4518979572709441, 280.1349275936351546, 13.78886128221634522 ) ) ;
#33787=CARTESIAN_POINT ( 'NONE',  ( 177.6627089506813775, 255.3829110640776321, -8.402693274504045462 ) ) ;
#33790=CARTESIAN_POINT ( 'NONE',  ( 183.8332630652478201, 272.5615133970043757, -16.17603297288676600 ) ) ;
#33793=CARTESIAN_POINT ( 'NONE',  ( 163.2061145480615210, 278.0382269583403172, 13.71808048336174224 ) ) ;
#33795=CARTESIAN_POINT ( 'NONE',  ( 191.9061344778403679, 298.2558201306721912, -9.413471345614182084 ) ) ;
#33796=CARTESIAN_POINT ( 'NONE',  ( 148.9275518150011806, 272.6969089400084272, 12.34519124974546500 ) ) ;
#33797=CARTESIAN_POINT ( 'NONE',  ( 162.8042930031641049, 248.6616881586264469, 11.14389129512055554 ) ) ;
#33799=CARTESIAN_POINT ( 'NONE',  ( 151.8965004642948600, 275.2307284912582759, -8.622094983838675120 ) ) ;
#33801=ORIENTED_EDGE ( 'NONE', *, *, #85707, .F. ) ;
#33804=CARTESIAN_POINT ( 'NONE',  ( 193.4149181402707995, 276.1162583725824788, -16.31078380200698064 ) ) ;
#33806=CARTESIAN_POINT ( 'NONE',  ( 192.6224552386041182, 297.0151161785129261, 12.49354144254605181 ) ) ;
#33809=CARTESIAN_POINT ( 'NONE',  ( -6.887775800123916881, 157.6423013555410080, -4.594050593750043987 ) ) ;
#33810=CARTESIAN_POINT ( 'NONE',  ( 155.1865148098964937, 261.8560670301561686, -16.99758927948949605 ) ) ;
#33813=CARTESIAN_POINT ( 'NONE',  ( 178.6034478761426101, 280.7652058965896344, -16.81717848226262291 ) ) ;
#33815=CARTESIAN_POINT ( 'NONE',  ( 162.4375581431960427, 282.5611924947268108, 5.618517507943365352 ) ) ;
#33816=CARTESIAN_POINT ( 'NONE',  ( 190.4202270817170017, 300.3952711937946560, -0.8604814952887831492 ) ) ;
#33817=CARTESIAN_POINT ( 'NONE',  ( 162.6396274730868186, 248.9468972229755082, -10.26162218571527518 ) ) ;
#33818=CARTESIAN_POINT ( 'NONE',  ( 207.3608985824721174, 271.4873834824583128, 4.969352111496849744 ) ) ;
#33819=CARTESIAN_POINT ( 'NONE',  ( 164.7307586990986863, 245.3249516942294122, -5.338649886695495894 ) ) ;
#33822=CARTESIAN_POINT ( 'NONE',  ( 180.9235756063633858, 293.2599282431580718, -8.659743166530571301 ) ) ;
#33824=CARTESIAN_POINT ( 'NONE',  ( 54.35637144981559743, 196.0643266524159856, -9.188101187500093303 ) ) ;
#33827=CARTESIAN_POINT ( 'NONE',  ( 71.13526655237410523, 218.0024278399160664, 9.188101187500095079 ) ) ;
#33828=CARTESIAN_POINT ( 'NONE',  ( 161.1750406344237661, 251.4836360396366501, -14.21198410781773802 ) ) ;
#33830=AXIS2_PLACEMENT_3D ( 'NONE', #76887, #38380, #69293 ) ;
#33831=DIRECTION ( 'NONE',  ( 0.4999999999999998890, -0.8660254037844385966, 0.000000000000000000 ) ) ;
#33832=CARTESIAN_POINT ( 'NONE',  ( 197.4842693130445923, 286.5942071846287149, -17.75505217046438489 ) ) ;
#33835=CARTESIAN_POINT ( 'NONE',  ( 176.6803982052660160, 270.1099931746196035, -17.20834088444772902 ) ) ;
#33837=CARTESIAN_POINT ( 'NONE',  ( 128.4003070610459929, 256.4860189848785694, -2.679491924311252493 ) ) ;
#33841=CARTESIAN_POINT ( 'NONE',  ( 77.73871025623044773, 221.8149278399160664, -9.188101187500095079 ) ) ;
#33844=CARTESIAN_POINT ( 'NONE',  ( 169.6038083371201992, 288.1641641989402842, -1.090344386142415578 ) ) ;
#33845=CARTESIAN_POINT ( 'NONE',  ( 192.5284579606305613, 297.1779242397361713, -13.15228012403107272 ) ) ;
#33847=EDGE_CURVE ( 'NONE', #93728, #55151, #40897, .T. ) ;
#33851=CARTESIAN_POINT ( 'NONE',  ( 193.8458974004921060, 288.0417099115973656, 16.67148095953266917 ) ) ;
#33853=AXIS2_PLACEMENT_3D ( 'NONE', #86143, #31369, #25271 ) ;
#33855=CARTESIAN_POINT ( 'NONE',  ( 117.8737486125219505, 248.8615022471903160, 5.000000000000046185 ) ) ;
#33856=CARTESIAN_POINT ( 'NONE',  ( 12.94829542258092658, 189.8297689869269504, -2.679491924311252493 ) ) ;
#33858=ORIENTED_EDGE ( 'NONE', *, *, #33173, .T. ) ;
#33859=CARTESIAN_POINT ( 'NONE',  ( 165.5488484770429523, 246.8969043953118785, -1.737601649715255991 ) ) ;
#33861=CARTESIAN_POINT ( 'NONE',  ( 202.4017613376760494, 280.0768611521521620, 15.73960524502980540 ) ) ;
#33862=CYLINDRICAL_SURFACE ( 'NONE', #22311, 10.00000000000010658 ) ;
#33865=CARTESIAN_POINT ( 'NONE',  ( 31.25085430583858681, 200.3967562850347122, -4.648177544792955347E-16 ) ) ;
#33868=CARTESIAN_POINT ( 'NONE',  ( 41.06812061084161769, 204.5177522451419350, 5.000000000000046185 ) ) ;
#33869=CARTESIAN_POINT ( 'NONE',  ( 153.4613150239306094, 264.8442007126561748, -16.86932470306368259 ) ) ;
#33871=EDGE_LOOP ( 'NONE', ( #13711, #87253, #94076, #28090 ) ) ;
#33875=CARTESIAN_POINT ( 'NONE',  ( 52.48883062679690426, 191.1115022471902023, -5.000000000000041744 ) ) ;
#33879=EDGE_CURVE ( 'NONE', #94756, #21068, #71270, .T. ) ;
#33881=CARTESIAN_POINT ( 'NONE',  ( 194.3708539535661259, 293.9868007723104029, -16.01585187499628304 ) ) ;
#33883=CARTESIAN_POINT ( 'NONE',  ( 155.5770330754656072, 261.1796695529068302, 18.26969263326161297 ) ) ;
#33885=CARTESIAN_POINT ( 'NONE',  ( 187.2429337685844359, 291.3981873160698228, -14.13502898539333508 ) ) ;
#33886=CARTESIAN_POINT ( 'NONE',  ( 208.0844008978733086, 270.2342407127895285, -4.836932903224296254 ) ) ;
#33887=CARTESIAN_POINT ( 'NONE',  ( 166.1759841011777610, 265.4597452293433548, 16.55821447247043920 ) ) ;
#33890=CARTESIAN_POINT ( 'NONE',  ( 87.02133327910362937, 230.2369531367911009, -4.594050593750048428 ) ) ;
#33892=CARTESIAN_POINT ( 'NONE',  ( 150.6790040019602088, 269.6633047651677089, 15.38315204620803378 ) ) ;
#33894=CARTESIAN_POINT ( 'NONE',  ( 166.3356402791620781, 279.2072638237854676, -13.54689619094178177 ) ) ;
#33901=CARTESIAN_POINT ( 'NONE',  ( 159.2536436069973718, 254.8115933126508992, -15.76697951715411250 ) ) ;
#33903=CARTESIAN_POINT ( 'NONE',  ( 85.18102929606172324, 229.1744531367911293, 4.594050593750047540 ) ) ;
#33905=CARTESIAN_POINT ( 'NONE',  ( 207.6555576926778883, 270.9770189326688410, -1.235081510489080436 ) ) ;
#33910=CARTESIAN_POINT ( 'NONE',  ( -17.74943806285152448, 173.8927522451419634, 2.944929066748280225E-16 ) ) ;
#33912=VECTOR ( 'NONE', #56205, 1000.000000000000000 ) ;
#33915=CARTESIAN_POINT ( 'NONE',  ( 160.6448124520779288, 275.6763703598426787, 14.01705192569017022 ) ) ;
#33919=DIRECTION ( 'NONE',  ( 0.4999999999999998890, -0.8660254037844385966, 0.000000000000000000 ) ) ;
#33920=ADVANCED_FACE ( 'NONE', ( #1528 ), #46382, .F. ) ;
#33921=CYLINDRICAL_SURFACE ( 'NONE', #58255, 17.82106496071139645 ) ;
#33922=CARTESIAN_POINT ( 'NONE',  ( 202.7282074973916792, 277.5114398175890642, -15.40750263959311184 ) ) ;
#33925=CARTESIAN_POINT ( 'NONE',  ( 161.7910648966377209, 250.4166507187868831, 13.19274492748169436 ) ) ;
#33929=CARTESIAN_POINT ( 'NONE',  ( 109.1931406464380530, 245.3967562850346837, -4.648177544792955347E-16 ) ) ;
#33931=CARTESIAN_POINT ( 'NONE',  ( 202.3349865675690182, 280.1925184466412020, -15.80981137687728655 ) ) ;
#33933=CARTESIAN_POINT ( 'NONE',  ( 182.1361237887369668, 264.3643447715849106, 13.55130394885500067 ) ) ;
#33934=CARTESIAN_POINT ( 'NONE',  ( 199.2404585781709443, 281.6525708895557614, -16.58724268975067062 ) ) ;
#33937=( BOUNDED_CURVE ( )  B_SPLINE_CURVE ( 2, ( #66991, #90350, #60373, #45186, #60870, #98422, #68484, #20930, #97430 ),
 .UNSPECIFIED., .F., .T. ) 
 B_SPLINE_CURVE_WITH_KNOTS ( ( 3, 2, 2, 2, 3 ),
 ( 0.6330645161290322509, 0.6344086021505376261, 0.6370967741935483764, 0.6397849462365591267, 0.6411290322580645018 ),
 .UNSPECIFIED. ) 
 CURVE ( )  GEOMETRIC_REPRESENTATION_ITEM ( )  RATIONAL_B_SPLINE_CURVE ( ( 0.9330127018922194093, 0.9330127018922194093, 1.000000000000000000, 0.8660254037844387076, 1.000000000000000000, 0.8660254037844387076, 1.000000000000000000, 0.9330127018922194093, 0.9330127018922194093 ) ) 
 REPRESENTATION_ITEM ( '' )  );
#33938=CARTESIAN_POINT ( 'NONE',  ( 155.5066938333533528, 261.3015006940112244, -18.40036130547566273 ) ) ;
#33940=CARTESIAN_POINT ( 'NONE',  ( 158.7260864440790726, 271.6582352343255025, -14.71012893904847729 ) ) ;
#33941=CARTESIAN_POINT ( 'NONE',  ( 206.0345876666409026, 273.1343529140784767, -9.309084676637942479 ) ) ;
#33942=CARTESIAN_POINT ( 'NONE',  ( 207.1572261440131797, 271.8401544939704877, -5.633070628900782140 ) ) ;
#33943=CARTESIAN_POINT ( 'NONE',  ( 17.11727908708474288, 174.5643266524160424, 9.188101187500095079 ) ) ;
#33945=ORIENTED_EDGE ( 'NONE', *, *, #10578, .T. ) ;
#33949=CARTESIAN_POINT ( 'NONE',  ( 43.26059451170998926, 183.5327760586659451, 1.948934522072302763E-15 ) ) ;
#33951=CARTESIAN_POINT ( 'NONE',  ( 146.9376205018946848, 276.1435710778808925, 5.066564108429441937 ) ) ;
#33953=CARTESIAN_POINT ( 'NONE',  ( 178.4805636753592353, 291.7095812787227374, 5.876746774786301586 ) ) ;
#33954=CARTESIAN_POINT ( 'NONE',  ( 178.4024347723586459, 293.9091254782996430, 2.739406101672524851 ) ) ;
#33955=CARTESIAN_POINT ( 'NONE',  ( 149.5479608754428114, 271.6223289258474551, 11.58749366327964303 ) ) ;
#33956=CARTESIAN_POINT ( 'NONE',  ( 182.5885846253425768, 280.2995767727080079, -16.09058154987042855 ) ) ;
#33962=CARTESIAN_POINT ( 'NONE',  ( 182.5686778644665083, 296.6873302901632314, 1.787712280751329708 ) ) ;
#33963=CARTESIAN_POINT ( 'NONE',  ( 88.86189758574333553, 212.1115022471902023, -5.000000000000041744 ) ) ;
#33966=EDGE_CURVE ( 'NONE', #67335, #30385, #100150, .T. ) ;
#33967=CARTESIAN_POINT ( 'NONE',  ( 46.23738328933649200, 191.3768266524159856, -9.188101187500091527 ) ) ;
#33968=CARTESIAN_POINT ( 'NONE',  ( 159.3528137482544196, 254.6398255893999476, 16.73628156321660398 ) ) ;
#33970=CARTESIAN_POINT ( 'NONE',  ( 162.8271773159503937, 263.3686283302618563, 17.75290566180205687 ) ) ;
#33971=CARTESIAN_POINT ( 'NONE',  ( 147.5693121967435957, 275.0494489676833041, 4.210973343677100189 ) ) ;
#33975=CARTESIAN_POINT ( 'NONE',  ( 167.5658046615882597, 285.5733867727782354, 7.972160045818313279 ) ) ;
#33976=CARTESIAN_POINT ( 'NONE',  ( 164.3706594650489023, 245.9486618633701482, -1.665857659249071698 ) ) ;
#33977=CARTESIAN_POINT ( 'NONE',  ( 147.1495358447521369, 275.7765229371483997, 6.477374713577704668 ) ) ;
#33978=CARTESIAN_POINT ( 'NONE',  ( 190.7608863809561797, 298.9511920904263320, -7.863160954977485240 ) ) ;
#33980=CARTESIAN_POINT ( 'NONE',  ( 202.2773826701151165, 280.2922913237452462, 16.62862787739668846 ) ) ;
#33981=CARTESIAN_POINT ( 'NONE',  ( 196.2878005184348353, 290.6665519265632724, -16.69183432842427806 ) ) ;
#33982=CARTESIAN_POINT ( 'NONE',  ( 204.4735667670548764, 276.4883888850707763, 14.55282211540290227 ) ) ;
#33983=ORIENTED_EDGE ( 'NONE', *, *, #2, .T. ) ;
#33988=CARTESIAN_POINT ( 'NONE',  ( 179.4777768328064269, 283.0882700270193482, 16.09770196021716515 ) ) ;
#33989=CARTESIAN_POINT ( 'NONE',  ( 191.1489696025915919, 299.5672681643093256, 8.892130899335590755 ) ) ;
#33990=CARTESIAN_POINT ( 'NONE',  ( 177.7013443376605437, 255.3287069125248365, -6.832982159536398648 ) ) ;
#33995=ADVANCED_FACE ( 'NONE', ( #72128 ), #97915, .T. ) ;
#33996=CARTESIAN_POINT ( 'NONE',  ( 207.1770866921659717, 271.8057550155037347, -5.569195235244989384 ) ) ;
#33997=CARTESIAN_POINT ( 'NONE',  ( 196.8435556370661459, 289.7039558245273838, -16.43899056939217118 ) ) ;
#33999=CARTESIAN_POINT ( 'NONE',  ( 153.0308080659177392, 265.5898606369461277, -17.74682723936668438 ) ) ;
#34000=CARTESIAN_POINT ( 'NONE',  ( 159.6978881494930249, 254.0421391940632532, 15.34888828951022610 ) ) ;
#34003=CARTESIAN_POINT ( 'NONE',  ( 157.3661765229227285, 258.0807821998820373, -18.27254492731150748 ) ) ;
#34004=CARTESIAN_POINT ( 'NONE',  ( 105.5326262849960131, 240.9244531367911293, -4.594050593750046652 ) ) ;
#34005=CARTESIAN_POINT ( 'NONE',  ( 149.1429535397850827, 272.3238222086447990, -12.91457852089092384 ) ) ;
#34006=CARTESIAN_POINT ( 'NONE',  ( 184.1161166760942649, 288.9931618037095973, -13.06163573803795686 ) ) ;
#34008=CARTESIAN_POINT ( 'NONE',  ( 207.8060684685902686, 270.7163266217015689, 2.015725026008670540 ) ) ;
#34011=CARTESIAN_POINT ( 'NONE',  ( 157.6466783816650832, 259.5949387289228412, 17.71616314254395519 ) ) ;
#34013=CARTESIAN_POINT ( 'NONE',  ( 63.34103791831415009, 213.5024278399160949, 9.188101187500095079 ) ) ;
#34015=CARTESIAN_POINT ( 'NONE',  ( 191.5766842709549280, 298.8264446275616137, 8.039910086100929831 ) ) ;
#34016=CARTESIAN_POINT ( 'NONE',  ( 150.9195128607351251, 269.2467312020988857, 13.93698123781031484 ) ) ;
#34017=CARTESIAN_POINT ( 'NONE',  ( 176.5965672854825925, 273.2588103071500427, 17.23532591839911277 ) ) ;
#34023=CARTESIAN_POINT ( 'NONE',  ( 207.7296438747196134, 270.8486979012336633, -6.692930657757584001 ) ) ;
#34025=CARTESIAN_POINT ( 'NONE',  ( 190.6094661480870798, 300.5017155583701083, 4.598210453186021951 ) ) ;
#34026=EDGE_CURVE ( 'NONE', #21258, #78457, #36060, .T. ) ;
#34027=CARTESIAN_POINT ( 'NONE',  ( 180.3226476666923190, 271.1461042115498685, 16.43934610314749634 ) ) ;
#34028=CARTESIAN_POINT ( 'NONE',  ( 164.8616299252405213, 245.0982760813026857, 1.544363874765093625 ) ) ;
#34029=FACE_OUTER_BOUND ( 'NONE', #43685, .T. ) ;
#34030=CARTESIAN_POINT ( 'NONE',  ( 164.1196843314846774, 253.9561035179159205, 14.46087810102053517 ) ) ;
#34031=CARTESIAN_POINT ( 'NONE',  ( 208.0287371622045782, 270.3306531311065442, 3.558879245883286746 ) ) ;
#34032=CARTESIAN_POINT ( 'NONE',  ( 120.4987145680870952, 246.5024278399160949, 9.188101187500095079 ) ) ;
#34034=CARTESIAN_POINT ( 'NONE',  ( 146.5913834600193582, 276.7432712258716947, -0.4909717733184599253 ) ) ;
#34036=CARTESIAN_POINT ( 'NONE',  ( 203.0026270830780675, 279.0361311525880978, -16.61345826058821373 ) ) ;
#34042=CARTESIAN_POINT ( 'NONE',  ( 158.1111710560796837, 275.7850098430334924, -12.43649661082534053 ) ) ;
#34043=CARTESIAN_POINT ( 'NONE',  ( 147.7887599827787994, 276.1980330845831304, 2.700269039940759619 ) ) ;
#34044=CARTESIAN_POINT ( 'NONE',  ( 182.0304806200197163, 260.4090999588434556, 10.44904933884112452 ) ) ;
#34045=CARTESIAN_POINT ( 'NONE',  ( 156.1927096727130788, 279.9932537871562204, -6.834036338872565786 ) ) ;
#34046=CARTESIAN_POINT ( 'NONE',  ( 136.3847812948166336, 258.7369531367911009, -4.594050593750048428 ) ) ;
#34048=CARTESIAN_POINT ( 'NONE',  ( 19.14685258109593136, 191.8615022471903160, 5.000000000000046185 ) ) ;
#34050=CARTESIAN_POINT ( 'NONE',  ( 68.48323730116675279, 210.3458772461660544, 9.188101187500095079 ) ) ;
#34051=CARTESIAN_POINT ( 'NONE',  ( 170.9866585576324383, 249.8975409664863037, 4.362717337680877883 ) ) ;
#34053=CARTESIAN_POINT ( 'NONE',  ( 170.3178023250738420, 289.0326318653803241, -4.561300590322002080 ) ) ;
#34054=CARTESIAN_POINT ( 'NONE',  ( 154.8605589353703351, 280.6980785630116770, -0.9605439388476536555 ) ) ;
#34055=CARTESIAN_POINT ( 'NONE',  ( 172.4250300583619264, 287.9095745046552679, -8.433196622960897670 ) ) ;
#34056=CARTESIAN_POINT ( 'NONE',  ( 202.8151641853381477, 279.3608264160075692, -16.28741359973609448 ) ) ;
#34058=CARTESIAN_POINT ( 'NONE',  ( 195.5324022567268685, 289.7225984500359459, 16.26972560970180481 ) ) ;
#34059=CARTESIAN_POINT ( 'NONE',  ( 121.6084831627943998, 251.0177522451418781, 5.000000000000046185 ) ) ;
#34061=ORIENTED_EDGE ( 'NONE', *, *, #99531, .F. ) ;
#34062=B_SPLINE_CURVE_WITH_KNOTS ( 'NONE', 3,
 ( #55169, #61777, #8594, #32387 ),
 .UNSPECIFIED., .F., .F.,
 ( 4, 4 ),
 ( 0.008234140320758805837, 0.01447576861028371242 ),
 .UNSPECIFIED. ) ;
#34064=CARTESIAN_POINT ( 'NONE',  ( 147.6618183892331331, 274.8892235422768522, 8.990680574201936892 ) ) ;
#34065=CARTESIAN_POINT ( 'NONE',  ( -3.504777292649705167, 156.5327760586659451, 1.948934522072302763E-15 ) ) ;
#34066=B_SPLINE_CURVE_WITH_KNOTS ( 'NONE', 3,
 ( #25167, #89882, #13356, #74670, #1886, #48482, #42721, #65542, #58431, #28036, #71294, #88924, #79424, #58912, #82790, #51849, #35137, #9990, #40851, #20456, #51330, #82297, #32768, #63673, #2394, #56050, #74167, #27565, #67029, #97956, #73659, #94612, #81292, #87043, #90392, #43727, #34643, #36127, #71796, #89406, #4759, #96489, #27059, #11865, #4237, #66048 ),
 .UNSPECIFIED., .F., .F.,
 ( 4, 2, 2, 2, 2, 2, 2, 2, 2, 2, 2, 2, 2, 2, 2, 2, 2, 2, 2, 2, 2, 2, 4 ),
 ( 0.0001777723017766823428, 0.0006668324149998756251, 0.001155892528223068962, 0.001400422584834609034, 0.001644952641446149541, 0.001767217669751986906, 0.001889482698057824706, 0.002011747726363662288, 0.002134012754669499870, 0.002623072867893023671, 0.003112132981116547473, 0.004090253207563457165, 0.005068373434010366857, 0.005557433547233746676, 0.005801963603845436586, 0.006046493660457125628, 0.006107626174610013628, 0.006168758688762901628, 0.006291023717068675893, 0.006535553773680317230, 0.007024613886903500158, 0.007513674000126683086, 0.008002734113349866882 ),
 .UNSPECIFIED. ) ;
#34067=CARTESIAN_POINT ( 'NONE',  ( 175.7270353543445935, 256.4821516345319310, -11.00345789725119872 ) ) ;
#34069=CARTESIAN_POINT ( 'NONE',  ( 33.27389197678166965, 200.0177522451419350, 5.000000000000046185 ) ) ;
#34072=CARTESIAN_POINT ( 'NONE',  ( 147.5634954182374372, 275.0595239235922236, 4.682022975662822439 ) ) ;
#34074=CARTESIAN_POINT ( 'NONE',  ( 167.5661991301409444, 256.5966495963957072, 13.73677599192672716 ) ) ;
#34075=CARTESIAN_POINT ( 'NONE',  ( 61.92489908531693033, 199.8927522451418213, 10.00000000000009592 ) ) ;
#34076=CARTESIAN_POINT ( 'NONE',  ( 163.0264227101321808, 256.4156498409448659, -15.66890022965337970 ) ) ;
#34077=CARTESIAN_POINT ( 'NONE',  ( 157.8719920515997046, 257.2046840049564480, -17.69857783492101433 ) ) ;
#34079=EDGE_CURVE ( 'NONE', #34648, #29382, #7176, .T. ) ;
#34080=EDGE_CURVE ( 'NONE', #21251, #23755, #66408, .T. ) ;
#34081=CARTESIAN_POINT ( 'NONE',  ( 42.09652578138355494, 205.1115022471903160, -5.000000000000047962 ) ) ;
#34082=CARTESIAN_POINT ( 'NONE',  ( 185.0916526433780689, 294.1912918594279063, 9.743016488043720003 ) ) ;
#34083=CARTESIAN_POINT ( 'NONE',  ( 149.7444450951932993, 271.6994330048118513, -11.56253598978762831 ) ) ;
#34084=CARTESIAN_POINT ( 'NONE',  ( 10.02652254571713719, 176.5958772461660544, -9.188101187500095079 ) ) ;
#34086=CARTESIAN_POINT ( 'NONE',  ( 164.3127595687991231, 252.5384005146300694, 13.43484586212805354 ) ) ;
#34088=CARTESIAN_POINT ( 'NONE',  ( 22.88158713136840561, 194.0177522451419350, 5.000000000000046185 ) ) ;
#34090=CARTESIAN_POINT ( 'NONE',  ( 165.0297293518065658, 244.8071193337670195, 2.517333243890161665 ) ) ;
#34091=FACE_OUTER_BOUND ( 'NONE', #74172, .T. ) ;
#34092=CARTESIAN_POINT ( 'NONE',  ( 65.91222438545561602, 218.8615022471903160, 5.000000000000046185 ) ) ;
#34093=CARTESIAN_POINT ( 'NONE',  ( 178.9979651084586578, 262.3326641942140327, -12.86811127174943614 ) ) ;
#34095=CARTESIAN_POINT ( 'NONE',  ( 153.0281328741066886, 278.1111380155435882, -6.210770828869143223 ) ) ;
#34097=CARTESIAN_POINT ( 'NONE',  ( 67.62392126478502519, 221.3967562850346837, -4.648177544792955347E-16 ) ) ;
#34098=FACE_OUTER_BOUND ( 'NONE', #26029, .T. ) ;
#34099=CARTESIAN_POINT ( 'NONE',  ( 156.8945693171665425, 276.4456326148838912, 10.43105563263390856 ) ) ;
#34100=CARTESIAN_POINT ( 'NONE',  ( 206.3454060440500086, 273.2462681537123785, -9.268083217908118954 ) ) ;
#34101=ORIENTED_EDGE ( 'NONE', *, *, #4156, .F. ) ;
#34102=CARTESIAN_POINT ( 'NONE',  ( 153.3127735718713609, 265.1014820546527631, 17.57722645152040641 ) ) ;
#34103=CARTESIAN_POINT ( 'NONE',  ( 164.3274319858398087, 246.0235340536434592, -1.770631424362269168 ) ) ;
#34104=B_SPLINE_CURVE_WITH_KNOTS ( 'NONE', 3,
 ( #38169, #31079, #23474, #76695 ),
 .UNSPECIFIED., .F., .F.,
 ( 4, 4 ),
 ( 0.001830914869364597564, 0.009761397888737791476 ),
 .UNSPECIFIED. ) ;
#34112=CARTESIAN_POINT ( 'NONE',  ( 196.1749740761792111, 288.8619730569873809, -17.33086882175758703 ) ) ;
#34113=CARTESIAN_POINT ( 'NONE',  ( 177.8721144827672731, 263.9665094508621905, 14.68891706277765330 ) ) ;
#34119=CARTESIAN_POINT ( 'NONE',  ( 161.5504728662519369, 250.8333683393111926, 12.94300825113363373 ) ) ;
#34120=CARTESIAN_POINT ( 'NONE',  ( 169.5095520540864982, 276.3819341640797802, -15.71460239395836744 ) ) ;
#34122=EDGE_LOOP ( 'NONE', ( #58368, #89599 ) ) ;
#34123=CARTESIAN_POINT ( 'NONE',  ( 148.3010860587701814, 276.5068540982774721, -3.904121881399305050 ) ) ;
#34124=ORIENTED_EDGE ( 'NONE', *, *, #16678, .T. ) ;
#34125=CARTESIAN_POINT ( 'NONE',  ( 160.3638665304753488, 268.9007647980437241, -16.83629063676312398 ) ) ;
#34127=CARTESIAN_POINT ( 'NONE',  ( 177.9669066697758524, 253.3125553430435275, -3.218270011446984213 ) ) ;
#34130=CARTESIAN_POINT ( 'NONE',  ( 147.7331950265948137, 274.7655955798928744, 7.332100195727512038 ) ) ;
#34131=CARTESIAN_POINT ( 'NONE',  ( 178.3794556815479098, 289.5192613054423987, -9.351548050966405512 ) ) ;
#34133=CARTESIAN_POINT ( 'NONE',  ( 193.7596376655525887, 294.6616349329243576, 13.47874803057572279 ) ) ;
#34135=CARTESIAN_POINT ( 'NONE',  ( 158.6468336853046139, 255.8626189275596801, -16.06042259295567476 ) ) ;
#34136=ORIENTED_EDGE ( 'NONE', *, *, #8315, .F. ) ;
#34140=CARTESIAN_POINT ( 'NONE',  ( 190.8261335000477743, 298.8222043136631783, -8.159106789104095370 ) ) ;
#34142=ORIENTED_EDGE ( 'NONE', *, *, #30157, .T. ) ;
#34144=CARTESIAN_POINT ( 'NONE',  ( 187.1933455069532215, 276.8274618490077046, 17.59017769528927744 ) ) ;
#34149=CARTESIAN_POINT ( 'NONE',  ( 47.29267820409027934, 188.1115022471902023, -5.000000000000041744 ) ) ;
#34150=CARTESIAN_POINT ( 'NONE',  ( 190.5793395442805149, 300.5538963668226415, -0.3437584566168827571 ) ) ;
#34156=CARTESIAN_POINT ( 'NONE',  ( 21.22170510744821570, 196.3927522451419634, 2.944929066748280225E-16 ) ) ;
#34157=CARTESIAN_POINT ( 'NONE',  ( 108.5912123618160905, 227.3768266524159856, -9.188101187500093303 ) ) ;
#34158=CARTESIAN_POINT ( 'NONE',  ( 184.0238465689049292, 296.8912303140136828, -2.771834375495716873 ) ) ;
#34160=CARTESIAN_POINT ( 'NONE',  ( 163.0311878320900121, 248.2686947869521532, 10.33250033289960435 ) ) ;
#34161=CARTESIAN_POINT ( 'NONE',  ( 29.16053163240333745, 178.4548013555409796, -4.594050593750042211 ) ) ;
#34162=CARTESIAN_POINT ( 'NONE',  ( 180.3268137483904354, 258.1330830615356149, 10.30874540274224849 ) ) ;
#34164=VERTEX_POINT ( 'NONE', #14787 ) ;
#34165=CARTESIAN_POINT ( 'NONE',  ( 185.2070000183807394, 260.0088792301957028, -5.784610090025596563 ) ) ;
#34168=CARTESIAN_POINT ( 'NONE',  ( 192.9721262430356887, 263.8139873464725724, -4.229629090758195709 ) ) ;
#34170=CARTESIAN_POINT ( 'NONE',  ( 182.3765091510860827, 284.2746805155291554, 14.91661155942450634 ) ) ;
#34171=CARTESIAN_POINT ( 'NONE',  ( 168.0994545464640737, 251.8035359048624855, 10.51302091382670056 ) ) ;
#34172=CARTESIAN_POINT ( 'NONE',  ( 44.28847903505648986, 202.5024278399160949, -9.188101187500093303 ) ) ;
#34173=CARTESIAN_POINT ( 'NONE',  ( 89.56554322277027325, 212.5177522451417929, 5.000000000000051514 ) ) ;
#34177=CARTESIAN_POINT ( 'NONE',  ( 7.590999645455913658, 169.0643266524160140, -9.188101187500093303 ) ) ;
#34179=CARTESIAN_POINT ( 'NONE',  ( 199.2299651681423143, 285.5705732690366858, -17.65328173313980642 ) ) ;
#34181=CARTESIAN_POINT ( 'NONE',  ( 193.1977289678065404, 296.0187128512746995, -12.37159405312863925 ) ) ;
#34184=CARTESIAN_POINT ( 'NONE',  ( 164.2851776226980860, 246.0967207574460929, 5.847738044744511754 ) ) ;
#34185=DIRECTION ( 'NONE',  ( -0.4999999999999987788, 0.8660254037844392627, 0.000000000000000000 ) ) ;
#34186=CARTESIAN_POINT ( 'NONE',  ( 164.3274319858398087, 246.0235340536434592, -1.770631424362269168 ) ) ;
#34189=CARTESIAN_POINT ( 'NONE',  ( 6.950328144465177438, 161.4865022471901455, 1.119607411625061291E-15 ) ) ;
#34191=CARTESIAN_POINT ( 'NONE',  ( 128.2121871902485566, 235.6423013555409796, -4.594050593750043987 ) ) ;
#34196=CARTESIAN_POINT ( 'NONE',  ( 151.0217401543597475, 269.4701321406242869, 13.82207127286603843 ) ) ;
#34197=CARTESIAN_POINT ( 'NONE',  ( 196.3341081413628899, 290.5863447708742342, 16.12390540996472410 ) ) ;
#34199=CARTESIAN_POINT ( 'NONE',  ( 150.4061938829137830, 270.1358257521749238, -15.15106128367595062 ) ) ;
#34201=CARTESIAN_POINT ( 'NONE',  ( 191.0170959869219303, 299.7956799668270946, 7.353346939903929069 ) ) ;
#34202=CARTESIAN_POINT ( 'NONE',  ( 148.9831146496684084, 272.6006712873522133, -12.63706091291043343 ) ) ;
#34207=CARTESIAN_POINT ( 'NONE',  ( 189.0039683861011497, 265.7567017869877759, 11.47791173151251165 ) ) ;
#34208=CARTESIAN_POINT ( 'NONE',  ( 175.3277058627924987, 278.9854953265928543, 15.46303258205545461 ) ) ;
#34209=CARTESIAN_POINT ( 'NONE',  ( 168.8411136774919044, 271.8979524934410961, -17.10145977970367426 ) ) ;
#34210=CARTESIAN_POINT ( 'NONE',  ( 196.3306825188763014, 270.8885471599495531, 12.02977562913896037 ) ) ;
#34213=CARTESIAN_POINT ( 'NONE',  ( 192.3401793061076717, 297.5040324353506094, 12.56432540404525611 ) ) ;
#34215=DIRECTION ( 'NONE',  ( -0.8660254037844359321, -0.5000000000000051070, -0.000000000000000000 ) ) ;
#34217=CARTESIAN_POINT ( 'NONE',  ( 195.3624787578944222, 290.3824063481519602, -16.76522224015156226 ) ) ;
#34219=CARTESIAN_POINT ( 'NONE',  ( 167.3220989969731818, 280.7870397072532569, 11.65856738288337269 ) ) ;
#34220=CARTESIAN_POINT ( 'NONE',  ( 147.6512387128590262, 274.9075480792844246, -8.209968531507987777 ) ) ;
#34221=CARTESIAN_POINT ( 'NONE',  ( 158.0832193973161566, 263.1600005068700057, -16.98150214051203477 ) ) ;
#34222=EDGE_LOOP ( 'NONE', ( #81515, #41493, #4243, #2592 ) ) ;
#34226=VERTEX_POINT ( 'NONE', #47177 ) ;
#34232=CARTESIAN_POINT ( 'NONE',  ( 94.74134171723733289, 237.0530062829862743, -4.648177544792955347E-16 ) ) ;
#34234=FACE_OUTER_BOUND ( 'NONE', #75254, .T. ) ;
#34238=ORIENTED_EDGE ( 'NONE', *, *, #53447, .T. ) ;
#34239=CARTESIAN_POINT ( 'NONE',  ( 185.8652519749559247, 282.2268457654508325, -16.59405335779809221 ) ) ;
#34242=CARTESIAN_POINT ( 'NONE',  ( 158.7111944379298336, 274.7584504872774005, -13.07079675756365233 ) ) ;
#34243=CARTESIAN_POINT ( 'NONE',  ( 193.1649355862271591, 296.0755126543221536, -12.21556774862162698 ) ) ;
#34244=CARTESIAN_POINT ( 'NONE',  ( 152.6873874250818517, 266.1846826352417565, -16.66598363829485763 ) ) ;
#34246=CARTESIAN_POINT ( 'NONE',  ( 2.620201125542898080, 178.9865022471903160, 10.00000000000009415 ) ) ;
#34247=CARTESIAN_POINT ( 'NONE',  ( 137.8731756836298814, 262.6589784336661069, -6.496448406907675876E-16 ) ) ;
#34249=ORIENTED_EDGE ( 'NONE', *, *, #65679, .T. ) ;
#34252=EDGE_LOOP ( 'NONE', ( #16180, #1329, #52009, #71621 ) ) ;
#34253=CARTESIAN_POINT ( 'NONE',  ( 1.230952036757517520, 161.5177522451418213, 5.000000000000051514 ) ) ;
#34256=CARTESIAN_POINT ( 'NONE',  ( 190.2409037545352817, 300.2489383464547927, 3.136352422388450911 ) ) ;
#34257=CARTESIAN_POINT ( 'NONE',  ( 157.7405083909982295, 280.7048132376855847, -7.110344775676333384 ) ) ;
#34259=CARTESIAN_POINT ( 'NONE',  ( 171.7908256294744831, 280.0902348243839128, 13.88385109847706644 ) ) ;
#34264=CARTESIAN_POINT ( 'NONE',  ( 185.0512884836414855, 273.0606714723194841, -16.92976292810380556 ) ) ;
#34266=ORIENTED_EDGE ( 'NONE', *, *, #90029, .F. ) ;
#34267=CARTESIAN_POINT ( 'NONE',  ( 164.0851047064185479, 278.1576806158360569, 13.30924083603244945 ) ) ;
#34269=CARTESIAN_POINT ( 'NONE',  ( 156.3862274318223626, 277.3475818783230693, 10.00078872878025571 ) ) ;
#34272=CARTESIAN_POINT ( 'NONE',  ( 202.3139361598622372, 280.2289788223093865, 15.93832709035092421 ) ) ;
#34275=CARTESIAN_POINT ( 'NONE',  ( 201.5343969995564635, 268.9872460397318719, 6.024498516268275594 ) ) ;
#34276=EDGE_LOOP ( 'NONE', ( #65229, #10330, #41820, #28111 ) ) ;
#34277=CARTESIAN_POINT ( 'NONE',  ( 12.50963621419470329, 166.4824982072973967, 3.021315404115420679E-15 ) ) ;
#34279=EDGE_CURVE ( 'NONE', #53306, #66866, #19243, .T. ) ;
#34282=CARTESIAN_POINT ( 'NONE',  ( 192.6773196027083372, 296.9200883123592689, 11.15745042875121484 ) ) ;
#34285=CARTESIAN_POINT ( 'NONE',  ( 163.0309151244508712, 248.2691671304387739, 11.27270415168660200 ) ) ;
#34286=CARTESIAN_POINT ( 'NONE',  ( 6.183361268541194278, 180.5024278399160664, 9.188101187500095079 ) ) ;
#34287=CARTESIAN_POINT ( 'NONE',  ( 105.6144235841895664, 219.5327760586659451, 1.948934522072303157E-15 ) ) ;
#34288=CARTESIAN_POINT ( 'NONE',  ( 203.5629025532486196, 278.0657055720176913, -15.85226727704602823 ) ) ;
#34290=CARTESIAN_POINT ( 'NONE',  ( 180.0469694969276588, 255.4107081643116715, -2.376983049801016712 ) ) ;
#34292=AXIS2_PLACEMENT_3D ( 'NONE', #87241, #72494, #41040 ) ;
#34294=CARTESIAN_POINT ( 'NONE',  ( 161.0074043740847856, 281.6987162223563814, 5.593313803799454753 ) ) ;
#34296=CARTESIAN_POINT ( 'NONE',  ( 181.0995730718790071, 291.1750261779234279, 9.327186099670552011 ) ) ;
#34299=CARTESIAN_POINT ( 'NONE',  ( 164.6595190653735870, 245.4483423593538305, -5.562352988119640962 ) ) ;
#34301=CARTESIAN_POINT ( 'NONE',  ( 166.2257170601846497, 253.6475096207515492, -13.42941508109017690 ) ) ;
#34304=CARTESIAN_POINT ( 'NONE',  ( 79.98487687335507701, 226.1744531367911293, 4.594050593750047540 ) ) ;
#34305=CARTESIAN_POINT ( 'NONE',  ( 207.7320178805681508, 270.8445860024863237, -5.379955943374661764 ) ) ;
#34310=DIRECTION ( 'NONE',  ( 0.4999999999999998890, -0.8660254037844385966, 0.000000000000000000 ) ) ;
#34311=CARTESIAN_POINT ( 'NONE',  ( 176.2999854890552172, 269.8567107842857240, -17.42186202513282112 ) ) ;
#34312=EDGE_CURVE ( 'NONE', #4372, #91593, #20293, .T. ) ;
#34318=CARTESIAN_POINT ( 'NONE',  ( 72.38035161819672680, 212.5958772461660544, -9.188101187500095079 ) ) ;
#34319=CARTESIAN_POINT ( 'NONE',  ( 170.8968330173543109, 288.5550931528428009, -1.069972840386552049 ) ) ;
#34321=CARTESIAN_POINT ( 'NONE',  ( 188.9765056315804088, 286.3781189046455893, -15.97876018633670725 ) ) ;
#34322=EDGE_CURVE ( 'NONE', #78871, #80478, #11871, .T. ) ;
#34325=CARTESIAN_POINT ( 'NONE',  ( 190.0153548218945048, 286.5829638478824677, 16.39362643471642755 ) ) ;
#34326=CARTESIAN_POINT ( 'NONE',  ( 191.2622316156482043, 288.8574828335728171, -16.55244734589887656 ) ) ;
#34327=CARTESIAN_POINT ( 'NONE',  ( 121.2656814440110367, 247.4865022471903444, -10.00000000000009415 ) ) ;
#34328=CARTESIAN_POINT ( 'NONE',  ( 205.2391015854675516, 275.1624436846170738, -14.01434138479280911 ) ) ;
#34331=ORIENTED_EDGE ( 'NONE', *, *, #18872, .T. ) ;
#34332=CARTESIAN_POINT ( 'NONE',  ( 169.5338548541099897, 248.2712795993637371, -1.960221964079814860 ) ) ;
#34334=CARTESIAN_POINT ( 'NONE',  ( 162.9148248802443106, 248.4702413316674381, 9.709394404200100581 ) ) ;
#34335=CARTESIAN_POINT ( 'NONE',  ( 207.3718082758823869, 270.6308103407627073, -0.3710573916699856922 ) ) ;
#34336=CARTESIAN_POINT ( 'NONE',  ( 153.3859906278383676, 264.9746663937372091, -17.41799046551451013 ) ) ;
#34337=VERTEX_POINT ( 'NONE', #67883 ) ;
#34340=CARTESIAN_POINT ( 'NONE',  ( 189.3827389365466445, 289.9845130480852049, 14.42905932677018122 ) ) ;
#34341=CARTESIAN_POINT ( 'NONE',  ( 168.5042146316756373, 248.9333234090209430, 3.460101701789785711 ) ) ;
#34342=CARTESIAN_POINT ( 'NONE',  ( 193.8652130780152731, 280.5836658925297229, -17.72338988841175933 ) ) ;
#34343=CARTESIAN_POINT ( 'NONE',  ( 193.6888222081633444, 273.0013374295587028, 15.75238434690954747 ) ) ;
#34344=EDGE_LOOP ( 'NONE', ( #56347, #41757, #66703, #62752 ) ) ;
#34345=CARTESIAN_POINT ( 'NONE',  ( 103.9451733683222301, 237.4865022471903160, 10.00000000000009415 ) ) ;
#34349=CARTESIAN_POINT ( 'NONE',  ( 44.24123536260515976, 207.8967562850346837, -4.648177544792955347E-16 ) ) ;
#34352=CARTESIAN_POINT ( 'NONE',  ( 186.3255980153079747, 298.7107439718217279, 1.073797455116038746 ) ) ;
#34353=CARTESIAN_POINT ( 'NONE',  ( 163.9942050550062049, 246.6007000282974673, 5.791111691696777974 ) ) ;
#34354=CARTESIAN_POINT ( 'NONE',  ( 194.6943296385021824, 293.4265244509877562, -16.10917128197217352 ) ) ;
#34357=CARTESIAN_POINT ( 'NONE',  ( 132.0211419364472363, 235.4824982072973683, 3.021315404115420679E-15 ) ) ;
#34358=CARTESIAN_POINT ( 'NONE',  ( 187.6043408702985005, 291.4350663380896549, -13.94014698167784161 ) ) ;
#34359=CARTESIAN_POINT ( 'NONE',  ( 164.0673170565375187, 246.4740663270022765, 4.489294478468116800 ) ) ;
#34360=CARTESIAN_POINT ( 'NONE',  ( 165.9079365288987162, 265.8636615913461014, 16.81383221254800375 ) ) ;
#34362=CARTESIAN_POINT ( 'NONE',  ( 106.1553423657898492, 232.0958772461660260, -9.188101187500095079 ) ) ;
#34363=B_SPLINE_CURVE_WITH_KNOTS ( 'NONE', 3,
 ( #89388, #3746, #35622, #19939 ),
 .UNSPECIFIED., .F., .F.,
 ( 4, 4 ),
 ( 0.01639396528500873529, 0.02525301955254147593 ),
 .UNSPECIFIED. ) ;
#34366=CARTESIAN_POINT ( 'NONE',  ( 163.0250628725154058, 276.5629096397734088, -14.03379528916789809 ) ) ;
#34368=AXIS2_PLACEMENT_3D ( 'NONE', #98516, #59971, #58961 ) ;
#34371=CARTESIAN_POINT ( 'NONE',  ( 197.4842693130445923, 286.5942071846287149, -17.75505217046438489 ) ) ;
#34375=CARTESIAN_POINT ( 'NONE',  ( 208.3408670980087152, 269.7900282237308147, 2.175586895783760077 ) ) ;
#34376=CARTESIAN_POINT ( 'NONE',  ( 101.1217432541752856, 223.0643266524159571, -9.188101187500093303 ) ) ;
#34384=CARTESIAN_POINT ( 'NONE',  ( 94.74134171723733289, 237.0530062829862743, -4.648177544792955347E-16 ) ) ;
#34385=CYLINDRICAL_SURFACE ( 'NONE', #95349, 10.00000000000010658 ) ;
#34386=CARTESIAN_POINT ( 'NONE',  ( 133.0835800865360170, 238.4548013555409796, -4.594050593750042211 ) ) ;
#34390=ORIENTED_EDGE ( 'NONE', *, *, #59673, .T. ) ;
#34391=CARTESIAN_POINT ( 'NONE',  ( 204.8467418195402843, 275.8420307340491036, 13.15258587511997135 ) ) ;
#34392=CARTESIAN_POINT ( 'NONE',  ( 160.5681497667090980, 275.6440229244402644, 12.83602361646179801 ) ) ;
#34393=CARTESIAN_POINT ( 'NONE',  ( 159.8597520197352537, 253.7617827468940277, -16.74905990210778839 ) ) ;
#34394=CARTESIAN_POINT ( 'NONE',  ( 192.3665687060960465, 271.8525640515161967, 14.11498752457012351 ) ) ;
#34395=CARTESIAN_POINT ( 'NONE',  ( 178.3938943706652651, 285.5145968506380996, 14.34020567925480982 ) ) ;
#34401=CARTESIAN_POINT ( 'NONE',  ( 200.6800100461949228, 283.0590218669948399, 18.32402613046234308 ) ) ;
#34403=CARTESIAN_POINT ( 'NONE',  ( 206.8791291248445532, 272.3218326606039454, -10.16823074922856840 ) ) ;
#34404=CARTESIAN_POINT ( 'NONE',  ( 178.5319624062738058, 291.5826149054348093, -6.133725113071555768 ) ) ;
#34405=CARTESIAN_POINT ( 'NONE',  ( -27.42236680055714260, 166.5217562850347406, 1.224646799147364892E-15 ) ) ;
#34408=CARTESIAN_POINT ( 'NONE',  ( 180.7138497164156661, 266.8527603518880937, -16.19060323297924242 ) ) ;
#34410=CARTESIAN_POINT ( 'NONE',  ( 168.7933227874096929, 282.1232148736041268, 13.17276477419401459 ) ) ;
#34413=CARTESIAN_POINT ( 'NONE',  ( 155.3716771045260714, 261.5353565282119348, -18.54934131471355840 ) ) ;
#34417=EDGE_CURVE ( 'NONE', #47161, #82896, #98887, .T. ) ;
#34418=CARTESIAN_POINT ( 'NONE',  ( 7.915412076110063033, 181.5024278399160664, -9.188101187500093303 ) ) ;
#34420=EDGE_LOOP ( 'NONE', ( #53556, #82239, #63753, #53201 ) ) ;
#34421=EDGE_CURVE ( 'NONE', #56117, #5319, #28715, .T. ) ;
#34424=CARTESIAN_POINT ( 'NONE',  ( 184.5121120432382611, 270.3687502014600454, 16.77398936818960351 ) ) ;
#34426=CARTESIAN_POINT ( 'NONE',  ( 30.29666933122289407, 197.4869531367911293, 4.594050593750046652 ) ) ;
#34427=CARTESIAN_POINT ( 'NONE',  ( 161.7587802986029999, 250.4725692828850754, 14.33336164792646450 ) ) ;
#34428=CARTESIAN_POINT ( 'NONE',  ( 190.7569505155522904, 300.2462651405980978, -5.670926626284815697 ) ) ;
#34430=CARTESIAN_POINT ( 'NONE',  ( 178.4427175726033568, 291.7705066098333759, 5.794587143940031382 ) ) ;
#34431=CARTESIAN_POINT ( 'NONE',  ( 191.0604813119340690, 299.7205343796033503, -9.270812881586136811 ) ) ;
#34432=CARTESIAN_POINT ( 'NONE',  ( 160.0166746459236435, 283.6086068001695253, 2.232576205374148248 ) ) ;
#34435=CARTESIAN_POINT ( 'NONE',  ( 165.0676804254514138, 257.0913205595731483, -14.93706007131700098 ) ) ;
#34437=EDGE_CURVE ( 'NONE', #47944, #37486, #96393, .T. ) ;
#34439=CARTESIAN_POINT ( 'NONE',  ( 78.46959274032997200, 226.1115022471903160, -5.000000000000047962 ) ) ;
#34441=CARTESIAN_POINT ( 'NONE',  ( 162.1170296077141018, 267.9449120310337662, -16.75957877514680661 ) ) ;
#34442=CARTESIAN_POINT ( 'NONE',  ( 54.03161192339643293, 195.8768266524159856, -9.188101187500091527 ) ) ;
#34445=CARTESIAN_POINT ( 'NONE',  ( 146.9709166616330549, 276.0859004375172390, 3.755270622130282732 ) ) ;
#34449=CARTESIAN_POINT ( 'NONE',  ( 167.8870021103015233, 285.0517102558676470, 7.659404562680429684 ) ) ;
#34450=CARTESIAN_POINT ( 'NONE',  ( 164.9404048476745004, 244.9618339132846074, -2.801285734921658666 ) ) ;
#34454=CARTESIAN_POINT ( 'NONE',  ( 196.2630260332681189, 290.7094625936034049, -17.43112004684450866 ) ) ;
#34455=CARTESIAN_POINT ( 'NONE',  ( 171.3320430264542154, 255.7635525530785401, 11.44407331594274524 ) ) ;
#34459=CARTESIAN_POINT ( 'NONE',  ( 174.3675516979637905, 254.9025437404973218, 8.247627981828351551 ) ) ;
#34461=VERTEX_POINT ( 'NONE', #80509 ) ;
#34463=CARTESIAN_POINT ( 'NONE',  ( 151.4159295687746294, 268.3869122420484814, 14.78076517566594106 ) ) ;
#34464=CARTESIAN_POINT ( 'NONE',  ( 177.3812267363185242, 255.8896424273514469, -7.004123935190221140 ) ) ;
#34468=CARTESIAN_POINT ( 'NONE',  ( 161.8839333999304415, 250.2557977526613229, -13.90128376743482441 ) ) ;
#34469=CARTESIAN_POINT ( 'NONE',  ( 196.2379679265050925, 290.7528645076583871, -16.93678934971137906 ) ) ;
#34473=CARTESIAN_POINT ( 'NONE',  ( 189.0689802957956260, 269.8288687927027354, -15.50864081522695415 ) ) ;
#34476=CARTESIAN_POINT ( 'NONE',  ( 157.2777284163744582, 258.2339788142568864, -16.82360006463426316 ) ) ;
#34477=CARTESIAN_POINT ( 'NONE',  ( 118.9295641673753181, 227.2202760586659736, -5.415160957724236172E-17 ) ) ;
#34480=CARTESIAN_POINT ( 'NONE',  ( 164.4817765375028102, 245.7562014482918755, -6.334578229142199035 ) ) ;
#34483=CARTESIAN_POINT ( 'NONE',  ( 198.4264492142971221, 286.9623037257889564, 17.00126466006521397 ) ) ;
#34484=CARTESIAN_POINT ( 'NONE',  ( 71.67687952550437558, 206.0643266524160424, 9.188101187500095079 ) ) ;
#34487=CARTESIAN_POINT ( 'NONE',  ( 204.1541407990405332, 272.6956988606675623, 11.22829397770025395 ) ) ;
#34488=CARTESIAN_POINT ( 'NONE',  ( 175.6230877040034102, 278.4164368346121137, 15.50752949055044638 ) ) ;
#34489=B_SPLINE_CURVE_WITH_KNOTS ( 'NONE', 3,
 ( #56709, #17204, #2018, #86177 ),
 .UNSPECIFIED., .F., .F.,
 ( 4, 4 ),
 ( 0.01333939463499779488, 0.01972261937988741692 ),
 .UNSPECIFIED. ) ;
#34491=( BOUNDED_CURVE ( )  B_SPLINE_CURVE ( 2, ( #54082, #64199, #41386, #80957, #2932, #65686, #4393, #66200, #27711 ),
 .UNSPECIFIED., .F., .T. ) 
 B_SPLINE_CURVE_WITH_KNOTS ( ( 3, 2, 2, 2, 3 ),
 ( 0.9637096774193548709, 0.9650537634408602461, 0.9677419354838709964, 0.9704301075268817467, 0.9717741935483871218 ),
 .UNSPECIFIED. ) 
 CURVE ( )  GEOMETRIC_REPRESENTATION_ITEM ( )  RATIONAL_B_SPLINE_CURVE ( ( 0.9330127018922194093, 0.9330127018922194093, 1.000000000000000000, 0.8660254037844387076, 1.000000000000000000, 0.8660254037844387076, 1.000000000000000000, 0.9330127018922194093, 0.9330127018922194093 ) ) 
 REPRESENTATION_ITEM ( '' )  );
#34492=CARTESIAN_POINT ( 'NONE',  ( 181.4632975752175525, 255.1188003790442167, 1.936479460681336695 ) ) ;
#34493=CARTESIAN_POINT ( 'NONE',  ( 155.5322964227545413, 261.2571557083629159, -18.35853982030605280 ) ) ;
#34496=CARTESIAN_POINT ( 'NONE',  ( 173.9756991879395116, 277.8259260648333679, -15.76639585222196516 ) ) ;
#34497=CARTESIAN_POINT ( 'NONE',  ( 162.8741883755088509, 259.8356047474810566, -16.24831708344704850 ) ) ;
#34501=CARTESIAN_POINT ( 'NONE',  ( 164.2545401858843945, 246.1497863546213978, 2.275217130759496609 ) ) ;
#34502=CARTESIAN_POINT ( 'NONE',  ( 164.9617201910520237, 244.9249146555742414, 2.745022583679548767 ) ) ;
#34504=CARTESIAN_POINT ( 'NONE',  ( 167.3715206515632872, 256.4254025383586963, 13.71134816071423757 ) ) ;
#34506=CARTESIAN_POINT ( 'NONE',  ( 1.094572704733512092, 182.9860189848785410, -2.679491924311240503 ) ) ;
#34507=CARTESIAN_POINT ( 'NONE',  ( 129.7005815790617760, 239.5643266524159856, -9.188101187500093303 ) ) ;
#34508=ORIENTED_EDGE ( 'NONE', *, *, #84930, .F. ) ;
#34509=CARTESIAN_POINT ( 'NONE',  ( 146.6138605399200117, 276.7043397814778132, -0.5394499176159462950 ) ) ;
#34512=CARTESIAN_POINT ( 'NONE',  ( 199.0532324483041009, 282.6079911291746498, -17.61480581509741583 ) ) ;
#34513=EDGE_CURVE ( 'NONE', #11813, #7544, #5739, .T. ) ;
#34514=CARTESIAN_POINT ( 'NONE',  ( 164.4864504671816690, 245.7481059646165704, 6.337356894698421783 ) ) ;
#34523=CARTESIAN_POINT ( 'NONE',  ( 206.7127649687076314, 272.6099838315917623, -10.35326570309970506 ) ) ;
#34524=CARTESIAN_POINT ( 'NONE',  ( 140.0925393287100178, 257.8149278399160949, -9.188101187500095079 ) ) ;
#34526=CARTESIAN_POINT ( 'NONE',  ( 190.0370014622527322, 286.8089957100377205, 16.96978714573610247 ) ) ;
#34528=CARTESIAN_POINT ( 'NONE',  ( 170.6852122113414225, 250.4783651670598488, 3.454835134718858392 ) ) ;
#34530=CARTESIAN_POINT ( 'NONE',  ( 190.4163244163388242, 300.8362468508201459, 4.691083071570470331 ) ) ;
#34532=CARTESIAN_POINT ( 'NONE',  ( 172.4392911513491242, 287.3831240604444588, -8.176537520936799197 ) ) ;
#34535=CARTESIAN_POINT ( 'NONE',  ( 193.5083605049795210, 288.6373469989542855, 16.03391007790886391 ) ) ;
#34537=CARTESIAN_POINT ( 'NONE',  ( 136.3309150271299757, 239.5177522451417929, 5.000000000000051514 ) ) ;
#34538=CARTESIAN_POINT ( 'NONE',  ( 173.4505375608857491, 284.9503170016366198, -13.05978560202663452 ) ) ;
#34539=ORIENTED_EDGE ( 'NONE', *, *, #91745, .F. ) ;
#34540=CARTESIAN_POINT ( 'NONE',  ( 196.4677102463732012, 290.3549391369982686, 16.45225250689336249 ) ) ;
#34541=CARTESIAN_POINT ( 'NONE',  ( 190.5444288681022442, 300.6143634316900943, -1.000014190476072873 ) ) ;
#34542=CARTESIAN_POINT ( 'NONE',  ( -1.394013918807642360, 163.8768266524159856, 9.188101187500096856 ) ) ;
#34543=CARTESIAN_POINT ( 'NONE',  ( 35.81758128034870481, 200.6744531367911293, 4.594050593750047540 ) ) ;
#34544=CARTESIAN_POINT ( 'NONE',  ( 178.4336282224923309, 273.6370629074921226, -17.24514701715171228 ) ) ;
#34546=CARTESIAN_POINT ( 'NONE',  ( 188.0775634319173832, 267.1413101313072502, 14.31780989748781252 ) ) ;
#34549=CARTESIAN_POINT ( 'NONE',  ( 146.7845206192450007, 276.4087478532630939, 4.443586170796542945 ) ) ;
#34551=CARTESIAN_POINT ( 'NONE',  ( 163.2942584940569191, 258.1478583562382028, 16.77787020301746779 ) ) ;
#34552=CARTESIAN_POINT ( 'NONE',  ( 73.03889176721723686, 199.6427522451417644, 1.119607411625061291E-15 ) ) ;
#34556=CARTESIAN_POINT ( 'NONE',  ( 181.1541159318895211, 294.6564104570541645, 1.018405793603249565 ) ) ;
#34557=CARTESIAN_POINT ( 'NONE',  ( 51.26196130476894552, 193.7365022471901739, -10.00000000000009059 ) ) ;
#34559=CARTESIAN_POINT ( 'NONE',  ( 149.7701467413202749, 271.6257199327137073, -11.62364177631229190 ) ) ;
#34560=CARTESIAN_POINT ( 'NONE',  ( -4.533703103291247594, 174.3149278399161233, 9.188101187500093303 ) ) ;
#34562=DIRECTION ( 'NONE',  ( -0.8660254037844387076, -0.4999999999999998890, -0.000000000000000000 ) ) ;
#34563=CARTESIAN_POINT ( 'NONE',  ( 192.0712386031329686, 297.9698513971258649, 12.12276320360788873 ) ) ;
#34566=CARTESIAN_POINT ( 'NONE',  ( 180.0205270375271880, 277.0212420910811488, 16.30529632528782358 ) ) ;
#34567=CARTESIAN_POINT ( 'NONE',  ( 193.7706395672514645, 295.0264025848412075, 15.16938698680137065 ) ) ;
#34568=CARTESIAN_POINT ( 'NONE',  ( 76.20885775532401851, 203.2592609112379876, 2.679491924311254714 ) ) ;
#34569=CARTESIAN_POINT ( 'NONE',  ( 179.7261617362159427, 262.7909812490211152, -12.86163648858739172 ) ) ;
#34575=CARTESIAN_POINT ( 'NONE',  ( 153.1318494048608159, 277.9249485213736079, -4.812811992226706082 ) ) ;
#34577=CARTESIAN_POINT ( 'NONE',  ( 156.9230943565391669, 276.4044123300005822, 10.58617205435853315 ) ) ;
#34578=CARTESIAN_POINT ( 'NONE',  ( 206.3423291502491566, 273.2515974901050413, -10.76717883871977577 ) ) ;
#34581=CARTESIAN_POINT ( 'NONE',  ( 207.0200405408487541, 272.0777669287182334, 6.494273599193515878 ) ) ;
#34584=EDGE_LOOP ( 'NONE', ( #46690, #51284, #42789, #71907, #55603 ) ) ;
#34585=EDGE_LOOP ( 'NONE', ( #93818, #4464, #75491, #82315, #15870 ) ) ;
#34586=CARTESIAN_POINT ( 'NONE',  ( 159.7567037358847699, 278.4970363524427626, -9.767935059668046094 ) ) ;
#34587=FACE_OUTER_BOUND ( 'NONE', #64214, .T. ) ;
#34589=CARTESIAN_POINT ( 'NONE',  ( 192.1640094933931096, 297.8091675017319062, 12.36911124822534447 ) ) ;
#34592=CARTESIAN_POINT ( 'NONE',  ( 178.2850679595637473, 263.9267319943502912, 15.11778687281824141 ) ) ;
#34596=CARTESIAN_POINT ( 'NONE',  ( 196.8363552541316324, 289.7164272536036265, -17.80258609350122967 ) ) ;
#34597=CARTESIAN_POINT ( 'NONE',  ( 36.66582480827072743, 198.6427522451419350, -10.00000000000009592 ) ) ;
#34599=CARTESIAN_POINT ( 'NONE',  ( 200.8828793852583203, 282.7076418644388696, 17.90302398138411633 ) ) ;
#34600=CARTESIAN_POINT ( 'NONE',  ( 166.1395527380942667, 274.1522324139922944, -15.18991220291641575 ) ) ;
#34601=DIRECTION ( 'NONE',  ( -0.8660254037844387076, -0.4999999999999998890, -0.000000000000000000 ) ) ;
#34602=B_SPLINE_SURFACE_WITH_KNOTS ( 'NONE', 3, 1, ( 
 ( #46787, #77707 ),
 ( #8292, #70071 ),
 ( #686, #33596 ),
 ( #65481, #26497 ),
 ( #94925, #55854 ),
 ( #88349, #18908 ),
 ( #11317, #10295 ),
 ( #11805, #49784 ),
 ( #88856, #35074 ),
 ( #19422, #95452 ),
 ( #71608, #34103 ),
 ( #41168, #4175 ),
 ( #42661, #26992 ),
 ( #65980, #80745 ),
 ( #42175, #73595 ),
 ( #87375, #72105 ),
 ( #73110, #96933 ),
 ( #95938, #50277 ),
 ( #81230, #72617 ),
 ( #3703, #57878 ),
 ( #34581, #57376 ),
 ( #96428, #56874 ),
 ( #86849, #2708 ),
 ( #10800, #64491 ),
 ( #17382, #48293 ),
 ( #17904, #79239 ),
 ( #9811, #40671 ),
 ( #2205, #49293 ),
 ( #33086, #64995 ),
 ( #63982, #25486 ),
 ( #80232, #56377 ),
 ( #48801, #79734 ),
 ( #26004, #87858 ),
 ( #18401, #41673 ) ),
 .UNSPECIFIED., .T., .F., .F.,
 ( 4, 2, 2, 2, 2, 2, 2, 2, 2, 2, 2, 2, 2, 2, 2, 2, 4 ),
 ( 2, 2 ),
 ( 0.000000000000000000, 0.06250000000000000000, 0.1250000000000000000, 0.1875000000000000000, 0.2500000000000000000, 0.3125000000000000000, 0.3750000000000000000, 0.4375000000000000000, 0.5000000000000000000, 0.5625000000000000000, 0.6250000000000000000, 0.6875000000000000000, 0.7500000000000000000, 0.8125000000000000000, 0.8750000000000000000, 0.9375000000000000000, 1.000000000000000000 ),
 ( 0.000000000000000000, 1.000000000000000000 ),
 .UNSPECIFIED. ) ;
#34603=ORIENTED_EDGE ( 'NONE', *, *, #38874, .T. ) ;
#34604=CARTESIAN_POINT ( 'NONE',  ( 174.4470096775725096, 277.0272586029935269, -17.07083632119895356 ) ) ;
#34607=CARTESIAN_POINT ( 'NONE',  ( 156.7672756052014620, 266.5620104575966138, -16.23688817329552236 ) ) ;
#34609=CARTESIAN_POINT ( 'NONE',  ( -22.42236680055709641, 157.8615022471902591, 0.000000000000000000 ) ) ;
#34610=EDGE_LOOP ( 'NONE', ( #21302, #56113, #46689 ) ) ;
#34611=CARTESIAN_POINT ( 'NONE',  ( 159.2149555070472786, 259.5139964546949614, 16.68861687308905317 ) ) ;
#34612=CARTESIAN_POINT ( 'NONE',  ( 147.8749077915786643, 274.5201418708599022, 7.075400916280408126 ) ) ;
#34613=CARTESIAN_POINT ( 'NONE',  ( 180.2491029045606012, 291.6074392935250899, -9.950551294970233940 ) ) ;
#34616=CARTESIAN_POINT ( 'NONE',  ( 176.9554221106268130, 290.7336789374555792, 6.091561936831863200 ) ) ;
#34617=CARTESIAN_POINT ( 'NONE',  ( 197.1275133052921262, 289.2121267159609488, -18.14557307217323867 ) ) ;
#34618=VERTEX_POINT ( 'NONE', #78997 ) ;
#34619=CARTESIAN_POINT ( 'NONE',  ( 99.16399144804778132, 221.3927522451417929, -10.00000000000009237 ) ) ;
#34621=CARTESIAN_POINT ( 'NONE',  ( 164.9103019330012216, 245.0139736909548560, 2.841678961959298810 ) ) ;
#34622=CARTESIAN_POINT ( 'NONE',  ( 205.7639495959071212, 274.2533802642843170, 10.79039487422292432 ) ) ;
#34623=CARTESIAN_POINT ( 'NONE',  ( 160.0072461633487535, 253.5063153963366744, 16.23938890643736244 ) ) ;
#34625=ORIENTED_EDGE ( 'NONE', *, *, #72061, .F. ) ;
#34626=CARTESIAN_POINT ( 'NONE',  ( 187.6615196811425221, 277.1468961788498859, 17.16910232051792917 ) ) ;
#34628=CARTESIAN_POINT ( 'NONE',  ( 164.2507602871578740, 247.8507055370842806, 8.654211643685846056 ) ) ;
#34631=CARTESIAN_POINT ( 'NONE',  ( 198.6786699363856314, 286.5254446204100418, -18.23156697103042845 ) ) ;
#34633=CARTESIAN_POINT ( 'NONE',  ( 189.9718059322956094, 301.6061754500863117, -1.293200095882213185 ) ) ;
#34638=DIRECTION ( 'NONE',  ( 0.4999999999999992784, -0.8660254037844390407, 0.000000000000000000 ) ) ;
#34640=CARTESIAN_POINT ( 'NONE',  ( 28.87159617421078295, 194.1427522451419350, -10.00000000000009415 ) ) ;
#34641=CARTESIAN_POINT ( 'NONE',  ( 96.79126913948809374, 232.8149278399160949, 9.188101187500093303 ) ) ;
#34642=CARTESIAN_POINT ( 'NONE',  ( 184.0204834781850423, 296.8556583875038086, -2.767185464358945524 ) ) ;
#34643=CARTESIAN_POINT ( 'NONE',  ( 167.9076177050584704, 282.0442412872837394, -10.81069426134948763 ) ) ;
#34646=CARTESIAN_POINT ( 'NONE',  ( 21.36630299834339652, 173.9548013555409796, -4.594050593750042211 ) ) ;
#34648=VERTEX_POINT ( 'NONE', #28756 ) ;
#34649=ORIENTED_EDGE ( 'NONE', *, *, #53380, .F. ) ;
#34650=CARTESIAN_POINT ( 'NONE',  ( 185.6371458920492614, 259.0387137507489115, -5.368070696299057865 ) ) ;
#34652=CARTESIAN_POINT ( 'NONE',  ( 193.1296824374275047, 263.5099161404405095, -3.843190626297300572 ) ) ;
#34653=B_SPLINE_CURVE_WITH_KNOTS ( 'NONE', 3,
 ( #96464, #57408, #80779, #73627, #80268, #27030, #87411 ),
 .UNSPECIFIED., .F., .F.,
 ( 4, 3, 4 ),
 ( 0.001258777641685644277, 0.001498048468333237297, 0.002225082062310303373 ),
 .UNSPECIFIED. ) ;
#34655=CARTESIAN_POINT ( 'NONE',  ( 161.8153478334749877, 250.3745914384277285, -14.21120979595050215 ) ) ;
#34658=CARTESIAN_POINT ( 'NONE',  ( 40.58072100116311276, 203.4244531367911293, -4.594050593750046652 ) ) ;
#34659=CARTESIAN_POINT ( 'NONE',  ( 93.02964483790795214, 234.5177522451419350, 5.000000000000046185 ) ) ;
#34663=FACE_OUTER_BOUND ( 'NONE', #34344, .T. ) ;
#34664=CARTESIAN_POINT ( 'NONE',  ( 4.614210867829412699, 161.2202760586659451, -5.415160957724236172E-17 ) ) ;
#34666=CARTESIAN_POINT ( 'NONE',  ( 198.7829547491859330, 286.3448180261817129, -18.59838968157616179 ) ) ;
#34668=CARTESIAN_POINT ( 'NONE',  ( 147.4323331177958494, 275.2867036919951147, -5.064030047414062707 ) ) ;
#34670=CARTESIAN_POINT ( 'NONE',  ( 164.3330377059402849, 246.0138246616164110, 7.208046019122525294 ) ) ;
#34671=CARTESIAN_POINT ( 'NONE',  ( 78.92295937046175425, 204.8262482093457777, 3.021315404115420679E-15 ) ) ;
#34672=CARTESIAN_POINT ( 'NONE',  ( 147.6121581866023007, 274.9752375363476631, 8.700660424766859080 ) ) ;
#34674=CARTESIAN_POINT ( 'NONE',  ( 164.3053959849042087, 246.0617015268593661, -7.251939739328854273 ) ) ;
#34675=CARTESIAN_POINT ( 'NONE',  ( 9.548404355818492562, 162.9865022471901455, 1.119607411625061291E-15 ) ) ;
#34677=CARTESIAN_POINT ( 'NONE',  ( 116.3579438323015012, 247.1744531367911293, 4.594050593750047540 ) ) ;
#34681=CARTESIAN_POINT ( 'NONE',  ( 170.3290958195750022, 289.6815776661216546, -1.151831906498994140 ) ) ;
#34682=CARTESIAN_POINT ( 'NONE',  ( 190.1893769843902362, 293.1304489240072257, 14.15308602958251250 ) ) ;
#34685=CARTESIAN_POINT ( 'NONE',  ( 151.2057546125658973, 268.7509459446807227, 15.78031848731319187 ) ) ;
#34686=CARTESIAN_POINT ( 'NONE',  ( 207.7656302052884598, 270.7863677483104539, -0.3981791975740528455 ) ) ;
#34687=EDGE_CURVE ( 'NONE', #57805, #73019, #80731, .T. ) ;
#34688=CARTESIAN_POINT ( 'NONE',  ( 190.1578907173511084, 300.2574240630518148, 3.242419245672157224 ) ) ;
#34689=CARTESIAN_POINT ( 'NONE',  ( 175.6461609673314115, 292.5563777142869526, -1.142818921673324439 ) ) ;
#34693=CARTESIAN_POINT ( 'NONE',  ( 167.6360249118671106, 271.0525740842397795, -16.39345155401522192 ) ) ;
#34696=CARTESIAN_POINT ( 'NONE',  ( 29.90546183718886653, 199.6199935810940929, 2.679491924311251605 ) ) ;
#34698=CARTESIAN_POINT ( 'NONE',  ( 148.5199441514828891, 273.7928082822475062, -8.166875775410368021 ) ) ;
#34700=CARTESIAN_POINT ( 'NONE',  ( 194.0821437630113451, 282.7473781295547610, 17.16106363911004351 ) ) ;
#34703=ORIENTED_EDGE ( 'NONE', *, *, #24044, .T. ) ;
#34705=EDGE_CURVE ( 'NONE', #62607, #98890, #57770, .T. ) ;
#34706=CARTESIAN_POINT ( 'NONE',  ( 147.9311236323648870, 274.4227731784279172, -7.799459659034405412 ) ) ;
#34708=ORIENTED_EDGE ( 'NONE', *, *, #28573, .F. ) ;
#34710=CARTESIAN_POINT ( 'NONE',  ( 205.6855624989150044, 273.4764227299817207, -9.799032349006141729 ) ) ;
#34712=B_SPLINE_CURVE_WITH_KNOTS ( 'NONE', 3,
 ( #4264, #27084, #19981, #50858 ),
 .UNSPECIFIED., .F., .F.,
 ( 4, 4 ),
 ( 0.02920254411432028976, 0.03834810336565397382 ),
 .UNSPECIFIED. ) ;
#34714=CARTESIAN_POINT ( 'NONE',  ( 95.92559083146868204, 220.0643266524159856, -9.188101187500093303 ) ) ;
#34718=CARTESIAN_POINT ( 'NONE',  ( 181.8377039732492904, 257.3392381919999821, -6.047806239234591708 ) ) ;
#34719=ORIENTED_EDGE ( 'NONE', *, *, #33173, .F. ) ;
#34720=VERTEX_POINT ( 'NONE', #84487 ) ;
#34721=CARTESIAN_POINT ( 'NONE',  ( 178.3028575937270261, 261.0369606096485882, 12.20229237870471195 ) ) ;
#34725=VERTEX_POINT ( 'NONE', #60623 ) ;
#34727=CARTESIAN_POINT ( 'NONE',  ( 202.8151641853381477, 279.3608264160075692, -16.28741359973609448 ) ) ;
#34729=CARTESIAN_POINT ( 'NONE',  ( 165.0278996183383811, 244.8102885250982865, 2.103256185480505636 ) ) ;
#34730=CARTESIAN_POINT ( 'NONE',  ( 190.0146931831988013, 301.5318925525250506, 2.191471318341308372 ) ) ;
#34731=CARTESIAN_POINT ( 'NONE',  ( 161.5320111222139019, 277.4805626463597719, -13.30372288155974836 ) ) ;
#34732=CARTESIAN_POINT ( 'NONE',  ( 152.8651171364917900, 265.8768457450651113, -16.25664868183201861 ) ) ;
#34735=CARTESIAN_POINT ( 'NONE',  ( 139.7681268980558968, 245.3768266524160140, -9.188101187500091527 ) ) ;
#34737=B_SPLINE_CURVE_WITH_KNOTS ( 'NONE', 3,
 ( #24475, #93417, #1185, #32580 ),
 .UNSPECIFIED., .F., .F.,
 ( 4, 4 ),
 ( 0.01376870305819338433, 0.02013848192403042137 ),
 .UNSPECIFIED. ) ;
#34740=CARTESIAN_POINT ( 'NONE',  ( 204.0604753336787667, 271.4817813032398703, 9.862283393711939183 ) ) ;
#34741=ORIENTED_EDGE ( 'NONE', *, *, #47664, .F. ) ;
#34742=EDGE_CURVE ( 'NONE', #2437, #85768, #55235, .T. ) ;
#34743=CARTESIAN_POINT ( 'NONE',  ( 2.001305964997000864, 160.4155109091896065, 2.679491924311254714 ) ) ;
#34745=CARTESIAN_POINT ( 'NONE',  ( 156.5891564345135691, 279.5636921043310394, 7.514476345455489259 ) ) ;
#34746=CARTESIAN_POINT ( 'NONE',  ( 164.4854433269806577, 246.2060377238486808, -1.879056492287135116 ) ) ;
#34747=CARTESIAN_POINT ( 'NONE',  ( 174.8813198920379648, 282.2092175607240279, 14.35867413939171122 ) ) ;
#34750=VERTEX_POINT ( 'NONE', #8943 ) ;
#34751=CARTESIAN_POINT ( 'NONE',  ( -27.42236680055714260, 166.5217562850347406, 1.224646799147364892E-15 ) ) ;
#34753=VERTEX_POINT ( 'NONE', #25134 ) ;
#34755=EDGE_CURVE ( 'NONE', #32378, #62928, #85653, .T. ) ;
#34756=CARTESIAN_POINT ( 'NONE',  ( 204.9919120605564444, 269.2057140325208593, -2.990236076290825107 ) ) ;
#34757=CARTESIAN_POINT ( 'NONE',  ( 164.1222658720982963, 246.3788921866353405, -8.359706015582100136 ) ) ;
#34759=CARTESIAN_POINT ( 'NONE',  ( 163.1008115941903895, 248.1481028935802442, 11.25332017433677834 ) ) ;
#34760=FACE_OUTER_BOUND ( 'NONE', #67782, .T. ) ;
#34763=CARTESIAN_POINT ( 'NONE',  ( 203.9648368022151601, 269.0477214045654364, 5.644613064108824574 ) ) ;
#34764=ORIENTED_EDGE ( 'NONE', *, *, #65731, .F. ) ;
#34767=CARTESIAN_POINT ( 'NONE',  ( 189.8468993113617955, 274.1474532089198419, -15.62931057064303708 ) ) ;
#34769=CARTESIAN_POINT ( 'NONE',  ( 153.4242699508872647, 264.9083646613370320, 16.62000820703435267 ) ) ;
#34772=CARTESIAN_POINT ( 'NONE',  ( 1.258015332399702757, 171.5333772461660828, 9.188101187500095079 ) ) ;
#34773=CARTESIAN_POINT ( 'NONE',  ( 105.2078667585768557, 240.7369531367911009, -4.594050593750048428 ) ) ;
#34774=CARTESIAN_POINT ( 'NONE',  ( 154.9067123643522734, 262.3406990819208886, -18.18534662427576265 ) ) ;
#34776=CARTESIAN_POINT ( 'NONE',  ( 179.9589285649147996, 254.9571903017543946, -2.426322644417845620 ) ) ;
#34779=CARTESIAN_POINT ( 'NONE',  ( -22.42236680055709641, 157.8615022471902591, 0.000000000000000000 ) ) ;
#34780=CARTESIAN_POINT ( 'NONE',  ( 194.2154056360670040, 294.2560451561701029, -15.66696967429384557 ) ) ;
#34782=B_SPLINE_CURVE_WITH_KNOTS ( 'NONE', 3,
 ( #51256, #43658, #59338, #90318 ),
 .UNSPECIFIED., .F., .F.,
 ( 4, 4 ),
 ( 0.01272487254098708317, 0.01903269051692836264 ),
 .UNSPECIFIED. ) ;
#34786=CARTESIAN_POINT ( 'NONE',  ( 175.3120318915934490, 265.2928129103611923, -15.67177354101544395 ) ) ;
#34787=B_SPLINE_CURVE_WITH_KNOTS ( 'NONE', 3,
 ( #38229, #90520, #28658, #29661, #98591, #83904, #75284, #100074, #5867, #91492, #45348, #15431, #76279, #52453, #6370, #6853, #22054, #46328, #30662, #36753, #5373, #21092, #29174, #44846, #36256, #98081, #91007, #51969, #83399, #37253, #68152, #37740, #53443, #30152, #63051, #55923 ),
 .UNSPECIFIED., .F., .F.,
 ( 4, 2, 2, 2, 2, 2, 2, 2, 2, 2, 2, 2, 2, 2, 2, 2, 2, 4 ),
 ( 0.003089973116247706104, 0.003286963708836297335, 0.003483954301424888132, 0.003582449597719183747, 0.003680944894013478928, 0.003877935486602134777, 0.004271916671779446908, 0.004665897856956759474, 0.005453860227311384604, 0.006241822597666009734, 0.007817747338375338056, 0.008014737930963938828, 0.008063985579110994478, 0.008113233227258048394, 0.008211728523552230818, 0.008605709708728910209, 0.008999690893905589600, 0.009393672079082267257 ),
 .UNSPECIFIED. ) ;
#34788=CARTESIAN_POINT ( 'NONE',  ( 76.95378796010953693, 224.4244531367911293, -4.594050593750046652 ) ) ;
#34789=CARTESIAN_POINT ( 'NONE',  ( 161.4143265314674522, 251.0691807084224365, -12.94469757303959234 ) ) ;
#34792=CARTESIAN_POINT ( 'NONE',  ( 196.2609093297512857, 290.7131288316392670, 16.03897268885959448 ) ) ;
#34793=CARTESIAN_POINT ( 'NONE',  ( 199.6932924450039764, 284.7680668849795325, 17.37765808470670237 ) ) ;
#34795=CARTESIAN_POINT ( 'NONE',  ( 173.1680667592106317, 268.1563685006378819, -16.28935171270416404 ) ) ;
#34804=CARTESIAN_POINT ( 'NONE',  ( 54.63354020801843092, 213.8967562850347122, -4.648177544792955347E-16 ) ) ;
#34805=EDGE_CURVE ( 'NONE', #53225, #1108, #8262, .T. ) ;
#34807=CARTESIAN_POINT ( 'NONE',  ( 193.5618293018212910, 288.4941101508381394, 16.06832059134343282 ) ) ;
#34810=CARTESIAN_POINT ( 'NONE',  ( 113.6157903772484303, 249.7365022471903444, 2.944929066748280225E-16 ) ) ;
#34811=CARTESIAN_POINT ( 'NONE',  ( 157.8429099974857195, 257.2550556002704525, -17.85752049034686095 ) ) ;
#34815=ORIENTED_EDGE ( 'NONE', *, *, #25118, .F. ) ;
#34816=CARTESIAN_POINT ( 'NONE',  ( 202.8167949821795446, 279.3580017930215149, 15.61966256214195070 ) ) ;
#34817=CARTESIAN_POINT ( 'NONE',  ( 179.0122920114791327, 284.0021645867860798, 15.65938388908703871 ) ) ;
#34822=CARTESIAN_POINT ( 'NONE',  ( 189.8548326329087104, 290.2376382689330967, 14.46855031197147312 ) ) ;
#34825=CARTESIAN_POINT ( 'NONE',  ( 193.2460171754006808, 295.9350752223151062, -13.17791578539254083 ) ) ;
#34826=CARTESIAN_POINT ( 'NONE',  ( 203.7690284654797210, 275.7086850192775955, -13.99192714286714612 ) ) ;
#34827=AXIS2_PLACEMENT_3D ( 'NONE', #23792, #93232, #54676 ) ;
#34832=CARTESIAN_POINT ( 'NONE',  ( 81.06766895168334486, 217.6115022471902591, 10.00000000000009592 ) ) ;
#34834=ORIENTED_EDGE ( 'NONE', *, *, #86399, .T. ) ;
#34835=CARTESIAN_POINT ( 'NONE',  ( 186.3625697200866114, 298.6552741896666703, 1.069755126919976096 ) ) ;
#34837=CARTESIAN_POINT ( 'NONE',  ( 176.9569807898301974, 265.3464266694197136, -16.55715408367980501 ) ) ;
#34839=CARTESIAN_POINT ( 'NONE',  ( 201.3559594018653911, 274.8723170797262583, -14.12745182062582394 ) ) ;
#34842=CARTESIAN_POINT ( 'NONE',  ( 163.9705683675892942, 246.6416399718259527, 5.157764633724318593 ) ) ;
#34843=CARTESIAN_POINT ( 'NONE',  ( 166.6337920219200441, 265.6691252616788006, 16.54534502771603499 ) ) ;
#34844=CARTESIAN_POINT ( 'NONE',  ( 180.2352183475922800, 256.5785695326966902, 4.914414593082182314 ) ) ;
#34845=CARTESIAN_POINT ( 'NONE',  ( 107.7251869580316281, 226.8768266524160140, 9.188101187500098632 ) ) ;
#34848=CARTESIAN_POINT ( 'NONE',  ( 163.0197392065574604, 276.6372685320687310, -14.12728359470665751 ) ) ;
#34849=ORIENTED_EDGE ( 'NONE', *, *, #24624, .F. ) ;
#34853=CARTESIAN_POINT ( 'NONE',  ( 176.9594653488500455, 293.0447406222712061, -2.803451863092930374 ) ) ;
#34854=CARTESIAN_POINT ( 'NONE',  ( 196.1241105319816143, 290.9500712997905794, 15.97146679939154268 ) ) ;
#34855=CARTESIAN_POINT ( 'NONE',  ( 206.5081929095101998, 272.9643130319303737, -9.215516226794479238 ) ) ;
#34857=CARTESIAN_POINT ( 'NONE',  ( 91.43256340568937901, 235.8464784336661353, 1.353441290958777327E-15 ) ) ;
#34859=AXIS2_PLACEMENT_3D ( 'NONE', #93361, #16326, #27438 ) ;
#34861=EDGE_LOOP ( 'NONE', ( #55789, #97363, #73390, #92979 ) ) ;
#34866=EDGE_CURVE ( 'NONE', #12230, #62531, #77092, .T. ) ;
#34867=CARTESIAN_POINT ( 'NONE',  ( 191.4086613504252341, 263.7107970214009924, -8.083176656581560593 ) ) ;
#34870=CARTESIAN_POINT ( 'NONE',  ( 133.1643360984345179, 253.8149278399160949, 9.188101187500093303 ) ) ;
#34872=FACE_OUTER_BOUND ( 'NONE', #10526, .T. ) ;
#34875=CARTESIAN_POINT ( 'NONE',  ( 157.3370492947211119, 258.1312320390110244, 17.02065074437983228 ) ) ;
#34881=CARTESIAN_POINT ( 'NONE',  ( 178.3194779259755194, 285.3457979227533770, 13.03892382964784069 ) ) ;
#34885=CARTESIAN_POINT ( 'NONE',  ( 200.6449165581618956, 283.1198055712825976, 18.35107460171532523 ) ) ;
#34888=CARTESIAN_POINT ( 'NONE',  ( 167.8874878883961230, 249.4612090931145474, 8.049769325627208261 ) ) ;
#34890=CARTESIAN_POINT ( 'NONE',  ( 162.7459776558209228, 248.7626933030860812, -9.895605163646791880 ) ) ;
#34891=CARTESIAN_POINT ( 'NONE',  ( 163.2143008875826240, 247.9515336713096474, -10.88636441666107579 ) ) ;
#34893=CARTESIAN_POINT ( 'NONE',  ( 181.9334155871473513, 264.0643945792503473, 13.76495337570946376 ) ) ;
#34894=CARTESIAN_POINT ( 'NONE',  ( 80.05961770938091604, 205.4824982072973967, 3.021315404115420679E-15 ) ) ;
#34896=CARTESIAN_POINT ( 'NONE',  ( 152.7153488183568300, 266.1362520814392951, 17.33540622643059237 ) ) ;
#34900=CARTESIAN_POINT ( 'NONE',  ( 205.9981425428302373, 272.8521996776938749, -9.276084512156598905 ) ) ;
#34901=CARTESIAN_POINT ( 'NONE',  ( 12.94935828348961593, 178.2833772461660544, -9.188101187500095079 ) ) ;
#34902=DIRECTION ( 'NONE',  ( 0.4999999999999998890, -0.8660254037844385966, 0.000000000000000000 ) ) ;
#34903=ORIENTED_EDGE ( 'NONE', *, *, #5954, .T. ) ;
#34905=CARTESIAN_POINT ( 'NONE',  ( 36.90037335867700818, 182.1115022471902023, -5.000000000000041744 ) ) ;
#34906=CARTESIAN_POINT ( 'NONE',  ( 163.8398374448017591, 246.8680725722146008, -5.948785025486735378 ) ) ;
#34908=CARTESIAN_POINT ( 'NONE',  ( 44.31597619863101301, 187.2048013555409796, 4.594050593750051981 ) ) ;
#34910=EDGE_CURVE ( 'NONE', #91683, #14425, #70615, .T. ) ;
#34912=CARTESIAN_POINT ( 'NONE',  ( 190.8957779480239765, 300.0058089740729770, -4.541438514207768229 ) ) ;
#34914=CARTESIAN_POINT ( 'NONE',  ( 181.7846118114498495, 294.3892353584903390, 6.386930120770952790 ) ) ;
#34915=CARTESIAN_POINT ( 'NONE',  ( 146.5095091551180815, 276.8850816817948726, 0.1418322875769769398 ) ) ;
#34918=CARTESIAN_POINT ( 'NONE',  ( 179.4052326654324929, 278.4640086126446477, -16.45363309275438013 ) ) ;
#34920=CARTESIAN_POINT ( 'NONE',  ( 93.16602416993194424, 213.0494855054051584, -2.679491924311248496 ) ) ;
#34924=CARTESIAN_POINT ( 'NONE',  ( 79.76863084600667264, 216.8615022471902591, -10.00000000000009592 ) ) ;
#34928=CARTESIAN_POINT ( 'NONE',  ( 42.50247518763358556, 195.3458772461660544, 9.188101187500095079 ) ) ;
#34931=CARTESIAN_POINT ( 'NONE',  ( 190.4976253092930278, 300.6954295735222900, -5.764807383508308902 ) ) ;
#34935=CARTESIAN_POINT ( 'NONE',  ( 171.3240658019900025, 286.5505184989698932, 7.546585824849171509 ) ) ;
#34939=CARTESIAN_POINT ( 'NONE',  ( 185.7387126045402681, 263.0356376848994842, 11.21768123893770941 ) ) ;
#34940=CARTESIAN_POINT ( 'NONE',  ( 178.9433923089253256, 286.0771944333194483, -14.51609702535374424 ) ) ;
#34941=CARTESIAN_POINT ( 'NONE',  ( 171.2953940480069264, 255.8198119141705149, 11.80824276626711899 ) ) ;
#34942=VERTEX_POINT ( 'NONE', #71649 ) ;
#34950=EDGE_CURVE ( 'NONE', #11091, #20729, #61350, .T. ) ;
#34954=CARTESIAN_POINT ( 'NONE',  ( 207.2337123599961899, 271.7076764818092443, -5.443417788256701861 ) ) ;
#34955=DIRECTION ( 'NONE',  ( 0.4999999999999998890, -0.8660254037844385966, 0.000000000000000000 ) ) ;
#34956=CARTESIAN_POINT ( 'NONE',  ( 149.2593905435863348, 272.1221474021800759, -12.98626158366800176 ) ) ;
#34960=CARTESIAN_POINT ( 'NONE',  ( 184.3563745939584919, 257.8924429673292025, 6.070039865595379780 ) ) ;
#34963=CARTESIAN_POINT ( 'NONE',  ( 113.3268549190559753, 245.4244531367911293, -4.594050593750046652 ) ) ;
#34964=FACE_OUTER_BOUND ( 'NONE', #1774, .T. ) ;
#34965=LINE ( 'NONE', #51684, #15570 ) ;
#34966=AXIS2_PLACEMENT_3D ( 'NONE', #58985, #96567, #20034 ) ;
#34968=CARTESIAN_POINT ( 'NONE',  ( 164.4963285489318991, 245.7309966251440301, -6.672251175510283794 ) ) ;
#34972=CARTESIAN_POINT ( 'NONE',  ( 198.3449891235413531, 287.1033967417670283, 16.95540786497457120 ) ) ;
#34974=CARTESIAN_POINT ( 'NONE',  ( 81.44681538588882574, 208.6423013555409796, -4.594050593750043987 ) ) ;
#34975=CARTESIAN_POINT ( 'NONE',  ( 174.9992441152388096, 285.3729034877181903, 13.43039555807443719 ) ) ;
#34976=CARTESIAN_POINT ( 'NONE',  ( 191.5694459269389824, 298.8389818071599962, 7.944420692511652504 ) ) ;
#34977=CARTESIAN_POINT ( 'NONE',  ( 151.0171360864231644, 269.0776428152087760, 14.21401713093731267 ) ) ;
#34979=CARTESIAN_POINT ( 'NONE',  ( 171.8853837999505743, 276.6425513415854880, 16.11255734744161217 ) ) ;
#34980=ORIENTED_EDGE ( 'NONE', *, *, #93239, .T. ) ;
#34981=EDGE_CURVE ( 'NONE', #58917, #87772, #97835, .T. ) ;
#34985=CARTESIAN_POINT ( 'NONE',  ( 194.7759874552263852, 293.2850889635864178, 15.50361547754712532 ) ) ;
#34987=CARTESIAN_POINT ( 'NONE',  ( 163.6930646551726909, 260.3320553973381379, -16.18243281979474446 ) ) ;
#34990=CARTESIAN_POINT ( 'NONE',  ( 160.5893190321802138, 270.9897182155185078, 16.60663562724527864 ) ) ;
#34991=CARTESIAN_POINT ( 'NONE',  ( 206.2520115784021471, 273.4080321133600933, 11.69992874350409018 ) ) ;
#34993=CARTESIAN_POINT ( 'NONE',  ( 127.5984922056368163, 251.1427522451419065, -10.00000000000009592 ) ) ;
#34994=CARTESIAN_POINT ( 'NONE',  ( 164.1646814417103144, 253.9179673720841208, 14.54048895392611485 ) ) ;
#34996=EDGE_CURVE ( 'NONE', #18309, #4228, #23845, .T. ) ;
#34997=CARTESIAN_POINT ( 'NONE',  ( 134.5180214354952284, 236.2202760586659736, -5.415160957724236172E-17 ) ) ;
#35000=CARTESIAN_POINT ( 'NONE',  ( 191.0702043019150835, 299.7036936669546776, -8.800021049343948576 ) ) ;
#35003=VECTOR ( 'NONE', #59346, 1000.000000000000000 ) ;
#35011=CARTESIAN_POINT ( 'NONE',  ( 206.6347703933553532, 272.7450743988160866, -10.98802705318387574 ) ) ;
#35012=CARTESIAN_POINT ( 'NONE',  ( 143.8274474304129171, 253.8458772461660260, 9.188101187500095079 ) ) ;
#35013=CARTESIAN_POINT ( 'NONE',  ( 189.5059428776464756, 300.4130739301078279, -3.423561384717671796 ) ) ;
#35014=CARTESIAN_POINT ( 'NONE',  ( 146.9709166616330549, 276.0859004375172390, 3.755270622130282732 ) ) ;
#35016=CARTESIAN_POINT ( 'NONE',  ( 204.8057697639265768, 275.9129964160624695, -12.68356524114230766 ) ) ;
#35017=CARTESIAN_POINT ( 'NONE',  ( 171.4502795663483994, 250.9255985275387104, 3.410053715956228970 ) ) ;
#35019=CARTESIAN_POINT ( 'NONE',  ( 149.6896757981861583, 271.3768714794653647, 12.49809796062302603 ) ) ;
#35021=CARTESIAN_POINT ( 'NONE',  ( 169.4056225884307310, 285.0682111663155638, -8.437954092449052368 ) ) ;
#35022=CARTESIAN_POINT ( 'NONE',  ( 202.9490938173916561, 279.1288534886517709, -16.56031645010252973 ) ) ;
#35023=CARTESIAN_POINT ( 'NONE',  ( 157.5068167110588035, 270.9949351285441708, -14.70592521109709416 ) ) ;
#35024=CARTESIAN_POINT ( 'NONE',  ( 129.4027117968543621, 255.5177522451419350, 5.000000000000046185 ) ) ;
#35025=CARTESIAN_POINT ( 'NONE',  ( 175.9979136080305011, 285.3618921757466182, -12.01256837341941086 ) ) ;
#35028=CARTESIAN_POINT ( 'NONE',  ( 157.2744851780909414, 258.2395962677452985, 18.17792129701959070 ) ) ;
#35029=B_SPLINE_CURVE_WITH_KNOTS ( 'NONE', 3,
 ( #90567, #13528, #44396, #75331, #53979, #78317, #38285, #84937, #32194, #77823, #39767, #70697, #40279, #92540, #47393, #69196, #8405, #14990, #39276, #63597, #100124, #62579, #32697, #7394, #85452, #24096, #47880, #794, #55478, #30709, #1311, #8898, #1812, #61589, #31679, #22606, #62079, #70186, #31188, #53493, #23087, #93540, #93026, #86464, #94042, #7915 ),
 .UNSPECIFIED., .F., .F.,
 ( 4, 2, 2, 2, 2, 2, 2, 2, 2, 2, 2, 2, 2, 2, 2, 2, 2, 2, 2, 2, 2, 2, 4 ),
 ( 0.002409292539555501350, 0.002836404853134061061, 0.003049961009923312077, 0.003156739088317942355, 0.003263517166712573067, 0.003370295245107203345, 0.003477073323501833624, 0.003690629480291128875, 0.004117741793869665601, 0.004971966421026801503, 0.005826191048183937404, 0.006680415675341073306, 0.007107527988919563194, 0.007534640302498051348, 0.007641418380892598360, 0.007694807420089909596, 0.007748196459287221699, 0.007854974537681806007, 0.007961752616076388581, 0.008388864929654481217, 0.008815977243232575589, 0.009029533400021706041, 0.009243089556810838228 ),
 .UNSPECIFIED. ) ;
#35030=CARTESIAN_POINT ( 'NONE',  ( 147.6207754342248961, 274.9603120256437592, 8.795690793376332195 ) ) ;
#35031=CARTESIAN_POINT ( 'NONE',  ( -2.016382903836450691, 160.4548013555409796, -4.594050593750042211 ) ) ;
#35033=CARTESIAN_POINT ( 'NONE',  ( 42.82723471405275717, 195.5333772461660544, 9.188101187500095079 ) ) ;
#35034=CARTESIAN_POINT ( 'NONE',  ( 178.7635222630899534, 259.0797437575516824, -11.44071160735324710 ) ) ;
#35037=CARTESIAN_POINT ( 'NONE',  ( 204.6713671561005299, 276.1457885614869951, -12.94307097876490431 ) ) ;
#35038=CARTESIAN_POINT ( 'NONE',  ( 188.7855976875974306, 290.4470481293840862, -14.77264779262060301 ) ) ;
#35039=CARTESIAN_POINT ( 'NONE',  ( 190.3286155001717930, 300.9881631498979004, -5.624828231725103045 ) ) ;
#35041=CARTESIAN_POINT ( 'NONE',  ( 171.2418428706442342, 258.0450685527933388, 14.49083553076813402 ) ) ;
#35042=CARTESIAN_POINT ( 'NONE',  ( 70.51298433951257039, 211.5177522451418497, -10.00000000000009592 ) ) ;
#35044=CARTESIAN_POINT ( 'NONE',  ( 157.7847820078105201, 257.3557362317297361, -18.02899742403477035 ) ) ;
#35045=FACE_OUTER_BOUND ( 'NONE', #53473, .T. ) ;
#35047=CARTESIAN_POINT ( 'NONE',  ( 48.51954752611824517, 185.4865022471901739, 1.119607411625061291E-15 ) ) ;
#35048=CARTESIAN_POINT ( 'NONE',  ( 184.6473554711987504, 293.6427102601792853, 9.570857982651210349 ) ) ;
#35049=CARTESIAN_POINT ( 'NONE',  ( 163.3854574543125580, 247.6550818016845597, 10.82482370245618775 ) ) ;
#35050=CARTESIAN_POINT ( 'NONE',  ( 3.802138503898990329, 166.8768266524160140, 9.188101187500098632 ) ) ;
#35051=CARTESIAN_POINT ( 'NONE',  ( 166.9877576141370810, 285.6245928529402249, 4.094825844093839429 ) ) ;
#35052=CARTESIAN_POINT ( 'NONE',  ( 153.4289928607825573, 264.9001843414388873, 17.27358709529985958 ) ) ;
#35054=CARTESIAN_POINT ( 'NONE',  ( 84.23513719695283442, 207.8932355074535678, -2.679491924311248496 ) ) ;
#35056=CARTESIAN_POINT ( 'NONE',  ( 180.5543891548928741, 277.3255815685567995, 16.32703862730248900 ) ) ;
#35057=CARTESIAN_POINT ( 'NONE',  ( 193.8913555215501390, 294.8173164187117550, 15.40725395879721837 ) ) ;
#35058=CARTESIAN_POINT ( 'NONE',  ( 148.9504735598738137, 272.6572073132907690, -11.88406006066344744 ) ) ;
#35059=CARTESIAN_POINT ( 'NONE',  ( 177.3592972006726427, 260.4793513326881111, -13.85185052211657109 ) ) ;
#35062=CARTESIAN_POINT ( 'NONE',  ( 115.5259514080638468, 249.0530062829863311, -4.648177544792955347E-16 ) ) ;
#35066=CARTESIAN_POINT ( 'NONE',  ( 153.0818245731483103, 277.5927342487316878, -5.205759267561572479 ) ) ;
#35072=EDGE_LOOP ( 'NONE', ( #36352, #12435, #5422, #25491 ) ) ;
#35073=CARTESIAN_POINT ( 'NONE',  ( 152.4703890395534813, 267.8466532369516813, 15.62370772889803128 ) ) ;
#35074=CARTESIAN_POINT ( 'NONE',  ( 164.4781197247689306, 245.7625352337404649, -1.511762618280499515 ) ) ;
#35081=ORIENTED_EDGE ( 'NONE', *, *, #46625, .F. ) ;
#35082=CARTESIAN_POINT ( 'NONE',  ( 159.7776096774677228, 278.5608043355848622, -9.713761887137795981 ) ) ;
#35083=CARTESIAN_POINT ( 'NONE',  ( 164.2712161151136172, 246.1209027979328710, 7.276091357954241445 ) ) ;
#35084=CARTESIAN_POINT ( 'NONE',  ( 152.6656396574222754, 266.2223508737794759, 17.04346597795114349 ) ) ;
#35086=CARTESIAN_POINT ( 'NONE',  ( 17.70578863690133886, 169.4824982072973967, 3.021315404115420679E-15 ) ) ;
#35087=CARTESIAN_POINT ( 'NONE',  ( 178.3153863976500588, 263.9796422997153513, 15.06320836021970067 ) ) ;
#35088=ORIENTED_EDGE ( 'NONE', *, *, #42792, .T. ) ;
#35089=CARTESIAN_POINT ( 'NONE',  ( -22.42236680055709641, 157.8615022471902591, 0.000000000000000000 ) ) ;
#35093=CARTESIAN_POINT ( 'NONE',  ( 177.1727833070994791, 269.3651756797060557, 16.08978429131461141 ) ) ;
#35094=CARTESIAN_POINT ( 'NONE',  ( 166.2726692463831171, 274.2434846602475318, -15.18227389483641510 ) ) ;
#35097=CARTESIAN_POINT ( 'NONE',  ( 176.5585609647920364, 278.9355578903217747, -16.94606152164766755 ) ) ;
#35099=CARTESIAN_POINT ( 'NONE',  ( 156.8295168708270069, 266.6489491931308180, -16.21854842269177510 ) ) ;
#35100=VERTEX_POINT ( 'NONE', #46178 ) ;
#35101=CARTESIAN_POINT ( 'NONE',  ( 157.5614123822272745, 268.8543676321601765, 15.62611732898177053 ) ) ;
#35103=ADVANCED_FACE ( 'NONE', ( #83748 ), #98962, .F. ) ;
#35105=CARTESIAN_POINT ( 'NONE',  ( 169.0307616625812557, 272.4356441479760633, 16.34146891005438818 ) ) ;
#35106=CARTESIAN_POINT ( 'NONE',  ( 194.0554856868662057, 294.5330346333298053, 14.40212516007646038 ) ) ;
#35108=CARTESIAN_POINT ( 'NONE',  ( 142.9884853222707477, 243.3615022471901739, 5.000000000000051514 ) ) ;
#35109=CARTESIAN_POINT ( 'NONE',  ( 192.1396999271463812, 297.8512729055811974, 12.32430960859512403 ) ) ;
#35111=CARTESIAN_POINT ( 'NONE',  ( 159.1219488725454028, 255.0396952838110849, -16.66430026305668122 ) ) ;
#35114=AXIS2_PLACEMENT_3D ( 'NONE', #55275, #2111, #24892 ) ;
#35115=CARTESIAN_POINT ( 'NONE',  ( 206.5479446040613141, 272.8954610772809133, 10.74757481123993230 ) ) ;
#35117=CARTESIAN_POINT ( 'NONE',  ( 206.5571822944673670, 272.8794609281530938, 10.95833005210827515 ) ) ;
#35121=CARTESIAN_POINT ( 'NONE',  ( 187.6284309019235366, 277.1362090929395663, 17.09713795014519988 ) ) ;
#35124=DIRECTION ( 'NONE',  ( 0.4999999999999992784, -0.8660254037844390407, 0.000000000000000000 ) ) ;
#35126=CARTESIAN_POINT ( 'NONE',  ( 160.4256652780435672, 252.7815922308273002, -16.16855709575365552 ) ) ;
#35127=CARTESIAN_POINT ( 'NONE',  ( 190.3940121281077893, 300.8748928676694163, 0.04809511090732299099 ) ) ;
#35132=CARTESIAN_POINT ( 'NONE',  ( 123.3201800421238090, 253.5530062829863311, -4.648177544792955347E-16 ) ) ;
#35133=CARTESIAN_POINT ( 'NONE',  ( 207.6508796976096107, 270.9851214578045528, 6.713685698622268383 ) ) ;
#35134=CARTESIAN_POINT ( 'NONE',  ( 29.01593374150816729, 200.8927522451419634, 2.944929066748280225E-16 ) ) ;
#35135=CARTESIAN_POINT ( 'NONE',  ( 107.7251869580316281, 226.8768266524160140, 9.188101187500096856 ) ) ;
#35136=CARTESIAN_POINT ( 'NONE',  ( 181.9644534062184107, 294.8608557540333663, -2.655205150443219697 ) ) ;
#35137=CARTESIAN_POINT ( 'NONE',  ( 164.2913008600799287, 280.3343451829814512, -11.31047592362255827 ) ) ;
#35139=CARTESIAN_POINT ( 'NONE',  ( 163.1611253217825492, 248.0436364529968216, 11.42797785440508029 ) ) ;
#35140=CARTESIAN_POINT ( 'NONE',  ( 24.31594170816038059, 184.8458772461660544, 9.188101187500095079 ) ) ;
#35141=LINE ( 'NONE', #87927, #88371 ) ;
#35144=B_SPLINE_CURVE_WITH_KNOTS ( 'NONE', 3,
 ( #74866, #21643, #12560, #66250, #89598, #52042 ),
 .UNSPECIFIED., .F., .F.,
 ( 4, 2, 4 ),
 ( 8.689474584194192324E-15, 0.0005080340594498560436, 0.001016068118891022640 ),
 .UNSPECIFIED. ) ;
#35147=CARTESIAN_POINT ( 'NONE',  ( 185.2951076684100258, 260.0657642104216052, -5.799074855275172524 ) ) ;
#35149=CARTESIAN_POINT ( 'NONE',  ( 193.5052912260503888, 264.1446421622504204, -4.343934653911574628 ) ) ;
#35150=ADVANCED_FACE ( 'NONE', ( #30996 ), #32998, .T. ) ;
#35151=CARTESIAN_POINT ( 'NONE',  ( 207.8232941427535536, 270.6864908788566026, -6.505149060073906142 ) ) ;
#35155=CARTESIAN_POINT ( 'NONE',  ( 51.75829523846230273, 194.5643266524159856, -9.188101187500093303 ) ) ;
#35156=CARTESIAN_POINT ( 'NONE',  ( 95.69988983291003137, 219.3927522451418213, 10.00000000000009592 ) ) ;
#35157=VERTEX_POINT ( 'NONE', #54792 ) ;
#35159=CARTESIAN_POINT ( 'NONE',  ( 180.4572463832561482, 261.7460625851787199, -13.63662180976220384 ) ) ;
#35160=CARTESIAN_POINT ( 'NONE',  ( 178.8233793429807008, 259.2497683303841995, -10.29503125857851131 ) ) ;
#35161=CARTESIAN_POINT ( 'NONE',  ( -9.892408837089961438, 177.3464784336661637, 1.353441290958777327E-15 ) ) ;
#35163=CARTESIAN_POINT ( 'NONE',  ( 151.2646864780760723, 268.6488729594320830, -14.38346604407754548 ) ) ;
#35165=CARTESIAN_POINT ( 'NONE',  ( 192.5143468344189728, 297.2023654272867361, -12.06830393602581530 ) ) ;
#35166=CARTESIAN_POINT ( 'NONE',  ( 194.9499559406243918, 279.5747724307917679, 17.51673600049429780 ) ) ;
#35167=CARTESIAN_POINT ( 'NONE',  ( 164.4936379324916516, 245.7356569095223051, 6.719479797016231437 ) ) ;
#35169=CARTESIAN_POINT ( 'NONE',  ( 164.6649740431187183, 245.4388940607451843, -1.430729255012818557 ) ) ;
#35171=CARTESIAN_POINT ( 'NONE',  ( 165.1672732435949342, 269.2213042464348405, 17.45144253968057413 ) ) ;
#35172=CARTESIAN_POINT ( 'NONE',  ( -3.369807917299440181, 168.8615022471902591, -10.00000000000009592 ) ) ;
#35174=CARTESIAN_POINT ( 'NONE',  ( 130.3772506997096343, 236.8923013555409796, 4.594050593750050204 ) ) ;
#35176=B_SPLINE_CURVE_WITH_KNOTS ( 'NONE', 3,
 ( #70360, #31848, #79514, #69858 ),
 .UNSPECIFIED., .F., .F.,
 ( 4, 4 ),
 ( 0.03943544382253093283, 0.04790621245170952752 ),
 .UNSPECIFIED. ) ;
#35179=CARTESIAN_POINT ( 'NONE',  ( 196.1573359623355088, 290.8925231663144473, 17.55680092534192482 ) ) ;
#35182=ORIENTED_EDGE ( 'NONE', *, *, #5954, .F. ) ;
#35183=CARTESIAN_POINT ( 'NONE',  ( 151.4384131719918685, 268.3479694989391078, 14.98299707687648841 ) ) ;
#35184=CARTESIAN_POINT ( 'NONE',  ( 208.2268492240826561, 269.9875129743418256, -0.3614433915064274583 ) ) ;
#35187=CARTESIAN_POINT ( 'NONE',  ( 172.6634619271783038, 267.9388633272891980, -16.30849192416249238 ) ) ;
#35189=VERTEX_POINT ( 'NONE', #63403 ) ;
#35191=CARTESIAN_POINT ( 'NONE',  ( 166.0350694293928768, 270.1027909330327930, -16.28260794856732119 ) ) ;
#35193=B_SPLINE_SURFACE_WITH_KNOTS ( 'NONE', 3, 1, ( 
 ( #1260, #32142 ),
 ( #47343, #25560 ),
 ( #62529, #746 ),
 ( #254, #32650 ),
 ( #93994, #17452 ),
 ( #46851, #92978 ),
 ( #48360, #78767 ),
 ( #31135, #24544 ),
 ( #8358, #39226 ),
 ( #2272, #94996 ),
 ( #94488, #16942 ),
 ( #55424, #31630 ),
 ( #56447, #16446 ),
 ( #93490, #86413 ),
 ( #70134, #54944 ),
 ( #17973, #24048 ),
 ( #9354, #85920 ),
 ( #40232, #71175 ),
 ( #47830, #79309 ),
 ( #78267, #87441 ),
 ( #8848, #70645 ),
 ( #40735, #23532 ),
 ( #69646, #1771 ),
 ( #62028, #25047 ),
 ( #71680, #77253 ),
 ( #7860, #54423 ),
 ( #85400, #38741 ),
 ( #97474, #57440 ),
 ( #64560, #89410 ),
 ( #27569, #18977 ),
 ( #58916, #96004 ),
 ( #48868, #89886 ),
 ( #95519, #42237 ),
 ( #10867, #88418 ) ),
 .UNSPECIFIED., .T., .F., .F.,
 ( 4, 2, 2, 2, 2, 2, 2, 2, 2, 2, 2, 2, 2, 2, 2, 2, 4 ),
 ( 2, 2 ),
 ( 0.000000000000000000, 0.06250000000000000000, 0.1250000000000000000, 0.1875000000000000000, 0.2500000000000000000, 0.3125000000000000000, 0.3750000000000000000, 0.4375000000000000000, 0.5000000000000000000, 0.5625000000000000000, 0.6250000000000000000, 0.6875000000000000000, 0.7500000000000000000, 0.8125000000000000000, 0.8750000000000000000, 0.9375000000000000000, 1.000000000000000000 ),
 ( 0.000000000000000000, 1.000000000000000000 ),
 .UNSPECIFIED. ) ;
#35194=ADVANCED_FACE ( 'NONE', ( #31989 ), #69028, .F. ) ;
#35196=CARTESIAN_POINT ( 'NONE',  ( 199.6745771582872351, 272.3907837538676517, 12.39460699429984203 ) ) ;
#35197=CARTESIAN_POINT ( 'NONE',  ( 185.8859980584196023, 296.7027117258024873, 4.750670030249517950 ) ) ;
#35200=CARTESIAN_POINT ( 'NONE',  ( 148.6183282077989816, 273.6856180928681397, -8.486299949745918170 ) ) ;
#35202=CARTESIAN_POINT ( 'NONE',  ( 157.5670606312586415, 279.0380996213595495, -9.710625198711769102 ) ) ;
#35205=CARTESIAN_POINT ( 'NONE',  ( 89.99855592466245469, 222.7677522451418781, 10.00000000000009592 ) ) ;
#35208=EDGE_CURVE ( 'NONE', #79294, #49558, #74675, .T. ) ;
#35209=CARTESIAN_POINT ( 'NONE',  ( 194.3177355571849318, 294.0788045336591381, -15.93712594727561616 ) ) ;
#35214=AXIS2_PLACEMENT_3D ( 'NONE', #65732, #81488, #68222 ) ;
#35215=CARTESIAN_POINT ( 'NONE',  ( 58.25437508341968851, 192.8932355074535678, -2.679491924311248496 ) ) ;
#35217=CARTESIAN_POINT ( 'NONE',  ( 78.44218234892279895, 228.3464784336661637, 1.353441290958777525E-15 ) ) ;
#35221=DIRECTION ( 'NONE',  ( 0.4999999999999998890, -0.8660254037844385966, 0.000000000000000000 ) ) ;
#35222=ORIENTED_EDGE ( 'NONE', *, *, #20105, .T. ) ;
#35223=ORIENTED_EDGE ( 'NONE', *, *, #39155, .T. ) ;
#35224=CARTESIAN_POINT ( 'NONE',  ( -3.194846457709630272, 157.4155109091896350, 2.679491924311251605 ) ) ;
#35225=VERTEX_POINT ( 'NONE', #84623 ) ;
#35229=CARTESIAN_POINT ( 'NONE',  ( 202.7754741559590173, 279.4295715634463022, -15.65855077192107636 ) ) ;
#35231=CARTESIAN_POINT ( 'NONE',  ( 182.9704806738767786, 279.7017868584060238, -16.88939609177110412 ) ) ;
#35234=CARTESIAN_POINT ( 'NONE',  ( 151.8835309833198153, 268.6765239516433894, 14.96763668012306248 ) ) ;
#35238=CARTESIAN_POINT ( 'NONE',  ( 137.3322569020296555, 250.0958772461660544, -9.188101187500095079 ) ) ;
#35239=CARTESIAN_POINT ( 'NONE',  ( 168.0351016175754637, 267.0074190867483708, -17.62211840267826091 ) ) ;
#35243=CARTESIAN_POINT ( 'NONE',  ( 164.0398389372132044, 281.8052652109336691, 8.614039144221564470 ) ) ;
#35245=VERTEX_POINT ( 'NONE', #51707 ) ;
#35249=CARTESIAN_POINT ( 'NONE',  ( 156.4050736080099000, 278.8659540353394846, 7.272296007666364304 ) ) ;
#35250=LINE ( 'NONE', #35751, #65852 ) ;
#35255=CARTESIAN_POINT ( 'NONE',  ( 185.1243922746118074, 273.1384459838623116, -16.79753314444298695 ) ) ;
#35259=CARTESIAN_POINT ( 'NONE',  ( 194.3452430042056847, 293.4673175397701357, -14.50972866970454866 ) ) ;
#35260=CARTESIAN_POINT ( 'NONE',  ( 201.2772264434572946, 267.1716386788893942, -2.196353493170192905 ) ) ;
#35263=AXIS2_PLACEMENT_3D ( 'NONE', #89653, #51086, #20715 ) ;
#35266=CARTESIAN_POINT ( 'NONE',  ( 161.4322953877310738, 281.4157690633189759, -6.765754283059072449 ) ) ;
#35268=CARTESIAN_POINT ( 'NONE',  ( 203.3726069110276740, 270.0503998713792839, 5.990016924711733637 ) ) ;
#35271=ORIENTED_EDGE ( 'NONE', *, *, #39279, .F. ) ;
#35276=CARTESIAN_POINT ( 'NONE',  ( 152.7153488183568300, 266.1362520814392951, 17.33540622643059237 ) ) ;
#35279=CARTESIAN_POINT ( 'NONE',  ( 52.94219725692860834, 189.8262482093458061, 3.021315404115420679E-15 ) ) ;
#35280=CARTESIAN_POINT ( 'NONE',  ( -0.9884983804899494242, 179.4244531367911577, -4.594050593750046652 ) ) ;
#35281=CARTESIAN_POINT ( 'NONE',  ( 93.70588009062352342, 237.1589784336661637, -6.496448406907675876E-16 ) ) ;
#35283=CARTESIAN_POINT ( 'NONE',  ( 186.3805910356028619, 295.6218943418388108, -7.683998803325324367 ) ) ;
#35286=CARTESIAN_POINT ( 'NONE',  ( 170.4623819437503016, 288.8056674672355939, -5.476885062779371260 ) ) ;
#35287=CARTESIAN_POINT ( 'NONE',  ( 160.7713118735465230, 281.8391587724178748, 5.260302810648785687 ) ) ;
#35288=CARTESIAN_POINT ( 'NONE',  ( 148.3253847707240141, 273.7398928553401447, -9.074433450356286457 ) ) ;
#35291=DIRECTION ( 'NONE',  ( 0.4999999999999992784, -0.8660254037844390407, 0.000000000000000000 ) ) ;
#35295=CARTESIAN_POINT ( 'NONE',  ( 84.04489159724214176, 210.1423013555409796, -4.594050593750043987 ) ) ;
#35296=CARTESIAN_POINT ( 'NONE',  ( 207.4218731373931632, 271.3817724553659332, -5.249531240730909154 ) ) ;
#35299=CARTESIAN_POINT ( 'NONE',  ( 195.8947060313465443, 291.3474115503753410, 16.07878593000791767 ) ) ;
#35300=CARTESIAN_POINT ( 'NONE',  ( 200.0565326084237938, 284.1389164665869771, 16.92133041920757108 ) ) ;
#35301=CARTESIAN_POINT ( 'NONE',  ( 150.9003228897357189, 269.2799692068659283, -14.30003212299500781 ) ) ;
#35302=CARTESIAN_POINT ( 'NONE',  ( 173.5129947698212334, 267.4886862244790109, -17.45415247818019111 ) ) ;
#35304=CARTESIAN_POINT ( 'NONE',  ( 147.1603453755519695, 275.7578002805973370, -5.230822882238410187 ) ) ;
#35310=CARTESIAN_POINT ( 'NONE',  ( 189.7011281277219439, 286.7593913854856282, -15.88714824190844155 ) ) ;
#35315=CARTESIAN_POINT ( 'NONE',  ( 205.8099205723994203, 269.1131406545866298, -1.356034389334280776 ) ) ;
#35316=CARTESIAN_POINT ( 'NONE',  ( 139.5243837071329267, 251.3615022471902307, -10.00000000000009592 ) ) ;
#35317=CARTESIAN_POINT ( 'NONE',  ( 205.3943609285979051, 274.8935266139653777, -13.14270440534009943 ) ) ;
#35319=VERTEX_POINT ( 'NONE', #64671 ) ;
#35323=CARTESIAN_POINT ( 'NONE',  ( 197.0063477221338815, 265.1879394709707753, -4.577846407058970613 ) ) ;
#35329=AXIS2_PLACEMENT_3D ( 'NONE', #45146, #6659, #37536 ) ;
#35330=CARTESIAN_POINT ( 'NONE',  ( 189.2647483391328933, 290.1520017563908596, 14.35190764732333690 ) ) ;
#35331=CARTESIAN_POINT ( 'NONE',  ( -22.42236680055709641, 157.8615022471902591, 0.000000000000000000 ) ) ;
#35332=CARTESIAN_POINT ( 'NONE',  ( 157.5052804517226264, 258.3460506454662777, -16.81904061521691673 ) ) ;
#35340=B_SPLINE_CURVE_WITH_KNOTS ( 'NONE', 3,
 ( #98735, #89660, #42982, #83546, #36898, #43985, #90663, #82564 ),
 .UNSPECIFIED., .F., .F.,
 ( 4, 2, 2, 4 ),
 ( 0.002053660639095798539, 0.002297581679447361584, 0.002541502719798924628, 0.003029344800502051585 ),
 .UNSPECIFIED. ) ;
#35342=ORIENTED_EDGE ( 'NONE', *, *, #98217, .T. ) ;
#35347=CARTESIAN_POINT ( 'NONE',  ( 164.6886454784808222, 273.3769192494668232, -15.25705676796773780 ) ) ;
#35348=CARTESIAN_POINT ( 'NONE',  ( 165.3552783545318050, 246.2432519206945472, 4.078954813822171843 ) ) ;
#35349=CARTESIAN_POINT ( 'NONE',  ( 193.9204722154232741, 294.7668848255750049, 15.43855698596013859 ) ) ;
#35350=CARTESIAN_POINT ( 'NONE',  ( 126.3716228836088646, 243.7677522451418497, 10.00000000000009592 ) ) ;
#35352=CARTESIAN_POINT ( 'NONE',  ( 164.3666959528347320, 245.9555268679014830, 4.217718140385406933 ) ) ;
#35354=CARTESIAN_POINT ( 'NONE',  ( 181.1216305184527471, 255.7546495805296161, 5.273460715939602750 ) ) ;
#35355=CARTESIAN_POINT ( 'NONE',  ( 99.38934535084139554, 234.3149278399160949, 9.188101187500093303 ) ) ;
#35359=CARTESIAN_POINT ( 'NONE',  ( 166.6551839283834227, 278.1147546280273559, -13.36279048790327728 ) ) ;
#35361=ORIENTED_EDGE ( 'NONE', *, *, #56548, .T. ) ;
#35363=CARTESIAN_POINT ( 'NONE',  ( 176.9775198831545708, 292.4513829097897428, -2.718792113259059562 ) ) ;
#35364=CARTESIAN_POINT ( 'NONE',  ( 157.2168982216852555, 258.3393398020932636, 18.09635675623264106 ) ) ;
#35365=CARTESIAN_POINT ( 'NONE',  ( 47.97596991287763757, 210.0530062829863027, 1.101618078115930403E-13 ) ) ;
#35366=CARTESIAN_POINT ( 'NONE',  ( 208.2512496840233496, 269.9452501379965952, 1.821023623773176947 ) ) ;
#35369=CARTESIAN_POINT ( 'NONE',  ( 163.4222916751007801, 247.5912830598222172, -10.52132777929285012 ) ) ;
#35370=EDGE_LOOP ( 'NONE', ( #7918, #54106, #79016, #69605, #63955, #36591, #7735, #88459, #67846, #2234, #49322, #27021, #66629, #63124, #19892, #17998, #85066, #41691, #14181, #93705, #23370, #43214 ) ) ;
#35371=CARTESIAN_POINT ( 'NONE',  ( 194.6938575426807745, 266.4053782337838356, -7.878287061657681889 ) ) ;
#35372=CARTESIAN_POINT ( 'NONE',  ( 24.24733352825768407, 173.2592609112379876, 2.679491924311254714 ) ) ;
#35373=VECTOR ( 'NONE', #3893, 1000.000000000000000 ) ;
#35376=CARTESIAN_POINT ( 'NONE',  ( 133.7059490715648167, 241.8768266524159856, 9.188101187500098632 ) ) ;
#35377=CARTESIAN_POINT ( 'NONE',  ( 199.6189824786654299, 284.3965447663834425, 17.01103535422801727 ) ) ;
#35378=CARTESIAN_POINT ( 'NONE',  ( -17.42236680055705023, 149.2012482093457777, 0.000000000000000000 ) ) ;
#35380=CARTESIAN_POINT ( 'NONE',  ( 156.6941734481478079, 259.2447256682348211, 17.84224415335075520 ) ) ;
#35381=DIRECTION ( 'NONE',  ( 0.4999999999999992784, -0.8660254037844390407, 0.000000000000000000 ) ) ;
#35383=CARTESIAN_POINT ( 'NONE',  ( 189.9137270143924923, 269.8458973532920027, 15.23304003329433876 ) ) ;
#35384=CARTESIAN_POINT ( 'NONE',  ( 161.3723466847356178, 279.8813218052029583, -11.31205495863178179 ) ) ;
#35385=( BOUNDED_CURVE ( )  B_SPLINE_CURVE ( 2, ( #41397, #63713, #96151, #80967, #10522, #87083, #87593, #27222, #25205 ),
 .UNSPECIFIED., .F., .T. ) 
 B_SPLINE_CURVE_WITH_KNOTS ( ( 3, 2, 2, 2, 3 ),
 ( 0.1814516129032258118, 0.1827956989247311870, 0.1854838709677419373, 0.1881720430107526876, 0.1895161290322580627 ),
 .UNSPECIFIED. ) 
 CURVE ( )  GEOMETRIC_REPRESENTATION_ITEM ( )  RATIONAL_B_SPLINE_CURVE ( ( 0.9330127018922194093, 0.9330127018922194093, 1.000000000000000000, 0.8660254037844387076, 1.000000000000000000, 0.8660254037844387076, 1.000000000000000000, 0.9330127018922194093, 0.9330127018922194093 ) ) 
 REPRESENTATION_ITEM ( '' )  );
#35388=CARTESIAN_POINT ( 'NONE',  ( 196.1195470348416166, 280.1172796017575024, -16.75394804383025971 ) ) ;
#35389=CARTESIAN_POINT ( 'NONE',  ( 145.0633378486230072, 247.8927522451418213, 10.00000000000009948 ) ) ;
#35390=B_SPLINE_CURVE_WITH_KNOTS ( 'NONE', 3,
 ( #76730, #84865, #55401, #61010, #14441, #68623, #22532, #7323, #77748, #61520, #62499, #37714, #6829, #84370, #1232, #228, #70621, #53420, #721, #69121, #54918, #16422, #100048, #39199, #23506, #45806, #45323, #46825, #62002, #39692, #32115, #63024, #70111, #85375, #99545, #14917 ),
 .UNSPECIFIED., .F., .F.,
 ( 4, 2, 2, 2, 2, 2, 2, 2, 2, 2, 2, 2, 2, 2, 2, 2, 2, 4 ),
 ( 0.001249278581673068586, 0.001605651914841360042, 0.001962025248009651498, 0.002674771914346297727, 0.004100265247019663911, 0.004813011913356347003, 0.005169385246524688116, 0.005347571913108822676, 0.005436665246400925952, 0.005481211913047011851, 0.005525758579693097750, 0.005614851912985403988, 0.005703945246277711094, 0.005882131912862174385, 0.006060318579446638543, 0.006238505246031102701, 0.006594878579200030150, 0.006951251912368958466 ),
 .UNSPECIFIED. ) ;
#35393=AXIS2_PLACEMENT_3D ( 'NONE', #7836, #8332, #31609 ) ;
#35394=CARTESIAN_POINT ( 'NONE',  ( 167.6327783924723178, 249.9043753111564570, 7.633368920509352229 ) ) ;
#35395=CARTESIAN_POINT ( 'NONE',  ( -24.92236680055712483, 162.1916292661124999, 6.123233995736853057E-16 ) ) ;
#35396=CARTESIAN_POINT ( 'NONE',  ( 207.5959034698703078, 271.0803430774575418, -1.830000129038042544 ) ) ;
#35406=( NAMED_UNIT ( * ) SI_UNIT ( $, .STERADIAN. ) SOLID_ANGLE_UNIT ( ) );
#35407=CARTESIAN_POINT ( 'NONE',  ( 157.6219484825743393, 270.8997167613374017, -14.79150089323977468 ) ) ;
#35408=CARTESIAN_POINT ( 'NONE',  ( 206.0369695942839599, 273.2765813626796216, -9.363013045195234696 ) ) ;
#35410=CARTESIAN_POINT ( 'NONE',  ( 4.640666744108908226, 182.6744531367911577, 4.594050593750047540 ) ) ;
#35412=ORIENTED_EDGE ( 'NONE', *, *, #52830, .T. ) ;
#35414=B_SPLINE_CURVE_WITH_KNOTS ( 'NONE', 3,
 ( #55147, #54646, #63768, #87144 ),
 .UNSPECIFIED., .F., .F.,
 ( 4, 4 ),
 ( 0.009333216069306437407, 0.01375087555092867168 ),
 .UNSPECIFIED. ) ;
#35415=CARTESIAN_POINT ( 'NONE',  ( 191.3077102587145646, 274.7514833773715850, 16.90660339326615969 ) ) ;
#35417=CARTESIAN_POINT ( 'NONE',  ( 43.63930707798317599, 189.8768266524159856, -9.188101187500093303 ) ) ;
#35420=CARTESIAN_POINT ( 'NONE',  ( 161.8873598795597388, 250.2498629158519350, 13.90822209621415873 ) ) ;
#35421=CARTESIAN_POINT ( 'NONE',  ( 174.4935265407061706, 288.9661596538846879, 7.702119871588271494 ) ) ;
#35422=CARTESIAN_POINT ( 'NONE',  ( 147.2443490232117256, 275.6123016948292275, 5.226063659459642352 ) ) ;
#35424=CARTESIAN_POINT ( 'NONE',  ( 200.4845243426100012, 268.5102331880001998, -6.465539202158884002 ) ) ;
#35428=B_SPLINE_SURFACE_WITH_KNOTS ( 'NONE', 3, 1, ( 
 ( #11040, #57605 ),
 ( #33845, #49515 ),
 ( #95681, #41406 ),
 ( #72351, #2955 ),
 ( #26228, #57104 ),
 ( #41917, #72851 ),
 ( #3443, #60584 ),
 ( #68196, #99125 ),
 ( #20625, #75833 ),
 ( #5911, #68691 ),
 ( #4933, #30203 ),
 ( #76326, #91540 ),
 ( #97641, #28713 ),
 ( #21135, #28206 ),
 ( #6901, #37790 ),
 ( #29707, #52498 ),
 ( #21618, #52013 ),
 ( #37299, #5420 ),
 ( #36801, #36302 ),
 ( #99624, #91051 ),
 ( #82476, #92059 ),
 ( #61089, #22105 ),
 ( #82954, #59082 ),
 ( #53001, #83951 ),
 ( #51509, #6419 ),
 ( #67712, #43401 ),
 ( #51001, #90054 ),
 ( #74345, #44892 ),
 ( #83446, #14514 ),
 ( #14014, #45396 ),
 ( #81953, #35812 ),
 ( #29221, #12530 ),
 ( #98639, #59590 ),
 ( #13038, #66706 ) ),
 .UNSPECIFIED., .T., .F., .F.,
 ( 4, 2, 2, 2, 2, 2, 2, 2, 2, 2, 2, 2, 2, 2, 2, 2, 4 ),
 ( 2, 2 ),
 ( 0.000000000000000000, 0.06250000000000000000, 0.1250000000000000000, 0.1875000000000000000, 0.2500000000000000000, 0.3125000000000000000, 0.3750000000000000000, 0.4375000000000000000, 0.5000000000000000000, 0.5625000000000000000, 0.6250000000000000000, 0.6875000000000000000, 0.7500000000000000000, 0.8125000000000000000, 0.8750000000000000000, 0.9375000000000000000, 1.000000000000000000 ),
 ( 0.000000000000000000, 1.000000000000000000 ),
 .UNSPECIFIED. ) ;
#35430=CARTESIAN_POINT ( 'NONE',  ( 167.0269342199107143, 257.9714305878135860, -15.35314806562867318 ) ) ;
#35431=CARTESIAN_POINT ( 'NONE',  ( 175.0809028706871118, 261.2525943152746208, 15.25527675994286092 ) ) ;
#35432=CARTESIAN_POINT ( 'NONE',  ( 86.26382137438992004, 230.6115022471902876, -5.000000000000047962 ) ) ;
#35434=CARTESIAN_POINT ( 'NONE',  ( 161.6115930178048075, 267.7619094808129603, -17.27471002177463788 ) ) ;
#35436=CARTESIAN_POINT ( 'NONE',  ( 62.93552237999645627, 197.9548013555410080, -4.594050593750042211 ) ) ;
#35439=CARTESIAN_POINT ( 'NONE',  ( 183.9467679955122037, 297.5904300510428016, 0.04192798755140602490 ) ) ;
#35444=CARTESIAN_POINT ( 'NONE',  ( 164.3524132573224392, 245.9802652221976587, -2.749586949851067441 ) ) ;
#35447=CARTESIAN_POINT ( 'NONE',  ( 185.8388345170929199, 263.3051524106403463, 11.05951379595252071 ) ) ;
#35449=CARTESIAN_POINT ( 'NONE',  ( 174.5163211812949555, 257.2306003409090067, 11.39338901972694806 ) ) ;
#35460=CARTESIAN_POINT ( 'NONE',  ( 161.1750406344237661, 251.4836360396366501, -14.21198410781773802 ) ) ;
#35462=CARTESIAN_POINT ( 'NONE',  ( 149.2923684163597784, 272.0650280510108701, -12.99082738998495756 ) ) ;
#35466=CARTESIAN_POINT ( 'NONE',  ( 159.4574711498080433, 254.4585536525209477, 16.86100557095418395 ) ) ;
#35469=CARTESIAN_POINT ( 'NONE',  ( 117.8198823448352499, 229.6423013555409796, -4.594050593750043987 ) ) ;
#35472=CARTESIAN_POINT ( 'NONE',  ( 183.5989898313927142, 289.9010940570624939, -13.66799045760379627 ) ) ;
#35473=ORIENTED_EDGE ( 'NONE', *, *, #14166, .F. ) ;
#35475=CARTESIAN_POINT ( 'NONE',  ( 164.3602934812760452, 245.9666162739349318, -7.171958108566009571 ) ) ;
#35478=CARTESIAN_POINT ( 'NONE',  ( 159.8416255366773839, 253.7931787365127434, 16.77980437810719394 ) ) ;
#35480=CARTESIAN_POINT ( 'NONE',  ( 73.65258675182887771, 204.1423013555409796, -4.594050593750043987 ) ) ;
#35484=CARTESIAN_POINT ( 'NONE',  ( 198.7520972810255842, 286.3982647288286785, 17.58825518441947722 ) ) ;
#35485=CARTESIAN_POINT ( 'NONE',  ( 175.6165075620648963, 278.4664812795192574, 16.92304262170376461 ) ) ;
#35489=CARTESIAN_POINT ( 'NONE',  ( 203.3740894404336927, 278.3927394765486838, -15.19753795879846869 ) ) ;
#35491=CARTESIAN_POINT ( 'NONE',  ( 147.9190624158496803, 274.4436638182332899, 9.640318987393841965 ) ) ;
#35493=CARTESIAN_POINT ( 'NONE',  ( 161.8882824960653579, 250.2482648971885340, -13.83574485983625557 ) ) ;
#35494=CARTESIAN_POINT ( 'NONE',  ( 78.92295937046175425, 204.8262482093457777, 3.021315404115420679E-15 ) ) ;
#35495=CARTESIAN_POINT ( 'NONE',  ( 200.2074516942827245, 283.2632627625744135, -16.91194335012181327 ) ) ;
#35496=CARTESIAN_POINT ( 'NONE',  ( 169.8069776206597226, 261.6727971985682757, -16.70353856883196286 ) ) ;
#35499=CARTESIAN_POINT ( 'NONE',  ( 205.8610808625997208, 274.0851439753691920, 10.38803237360972531 ) ) ;
#35500=CARTESIAN_POINT ( 'NONE',  ( 134.7352435515850289, 237.0494855054051584, -2.679491924311248496 ) ) ;
#35502=CARTESIAN_POINT ( 'NONE',  ( 208.3135187673106543, 269.8373969220020285, 2.829653198597726682 ) ) ;
#35503=CARTESIAN_POINT ( 'NONE',  ( 114.8152493078691947, 249.3464784336661637, 1.353441290958777327E-15 ) ) ;
#35505=CARTESIAN_POINT ( 'NONE',  ( 146.5157004908022031, 276.8743579738231233, -0.1877253132609108255 ) ) ;
#35507=ADVANCED_FACE ( 'NONE', ( #67643 ), #50946, .F. ) ;
#35508=CARTESIAN_POINT ( 'NONE',  ( 155.4495868485232108, 261.4004128932040203, -18.48326470492642315 ) ) ;
#35516=CARTESIAN_POINT ( 'NONE',  ( 147.6729357283378192, 275.7175590154257065, 2.784006950529999358 ) ) ;
#35517=CARTESIAN_POINT ( 'NONE',  ( 29.78943643340442549, 199.5530062829863027, -4.648177544792955347E-16 ) ) ;
#35518=CARTESIAN_POINT ( 'NONE',  ( 198.5281735716552305, 266.2561165906912493, 0.8612751909359168678 ) ) ;
#35520=CARTESIAN_POINT ( 'NONE',  ( 195.3315847523439004, 263.4512225432230252, 0.8630184002952996369 ) ) ;
#35521=CARTESIAN_POINT ( 'NONE',  ( 147.2494378675467033, 275.6034875578896504, 3.639370109197119341 ) ) ;
#35523=CARTESIAN_POINT ( 'NONE',  ( 157.0978663001774862, 258.5455091378672137, -17.31223197570816552 ) ) ;
#35524=CARTESIAN_POINT ( 'NONE',  ( 174.6782577430604420, 252.0113062779471989, 3.549132482648186482 ) ) ;
#35527=EDGE_CURVE ( 'NONE', #983, #68725, #70881, .T. ) ;
#35528=CARTESIAN_POINT ( 'NONE',  ( 190.4841013044967042, 300.7188538369516095, 4.682298117523464143 ) ) ;
#35530=CARTESIAN_POINT ( 'NONE',  ( 198.0858447170796524, 287.5522480202560018, 18.44384186289807559 ) ) ;
#35531=CARTESIAN_POINT ( 'NONE',  ( 157.0103870222185662, 271.9336101705912370, -15.05502374871075766 ) ) ;
#35532=CARTESIAN_POINT ( 'NONE',  ( 141.9600801517288460, 242.7677522451417929, -5.000000000000041744 ) ) ;
#35533=CARTESIAN_POINT ( 'NONE',  ( 175.7051557773955324, 285.9761665229386836, -11.83304049905165911 ) ) ;
#35537=CARTESIAN_POINT ( 'NONE',  ( 151.2646864780760723, 268.6488729594320830, -14.38346604407754548 ) ) ;
#35538=CARTESIAN_POINT ( 'NONE',  ( -2.801652295722365071, 175.3149278399160949, -9.188101187500095079 ) ) ;
#35539=CARTESIAN_POINT ( 'NONE',  ( 53.57110205792969282, 210.9244531367911577, -4.594050593750046652 ) ) ;
#35544=FACE_OUTER_BOUND ( 'NONE', #79618, .T. ) ;
#35545=CARTESIAN_POINT ( 'NONE',  ( 188.9222141114651947, 290.4608455028081266, -14.68227143028564008 ) ) ;
#35547=EDGE_CURVE ( 'NONE', #45450, #37792, #31025, .T. ) ;
#35548=CARTESIAN_POINT ( 'NONE',  ( 171.4108528510993210, 258.3780868124931089, 14.19704647611232140 ) ) ;
#35549=CARTESIAN_POINT ( 'NONE',  ( 179.1925786807920815, 254.4794537879851362, -4.121526722083301841 ) ) ;
#35550=CARTESIAN_POINT ( 'NONE',  ( 150.8677798231829570, 269.3363354515693118, 13.85464777478129150 ) ) ;
#35553=CARTESIAN_POINT ( 'NONE',  ( 42.60170726692454224, 188.7365022471902023, 10.00000000000009592 ) ) ;
#35554=CARTESIAN_POINT ( 'NONE',  ( 181.1401942789648558, 292.7476587285891583, 9.359391415499011657 ) ) ;
#35555=CARTESIAN_POINT ( 'NONE',  ( 202.9685995779611858, 279.0950685203052899, 16.84977534244423580 ) ) ;
#35556=CARTESIAN_POINT ( 'NONE',  ( 10.54098545103790840, 167.7048013555410080, 4.594050593750051981 ) ) ;
#35557=CARTESIAN_POINT ( 'NONE',  ( 164.3059702326774243, 284.8567553647953332, 4.267327785685381514 ) ) ;
#35558=CARTESIAN_POINT ( 'NONE',  ( 192.2185419806677942, 297.7147144631093170, 12.45868041609393728 ) ) ;
#35560=CARTESIAN_POINT ( 'NONE',  ( 206.4229368915142686, 273.1119807867502800, 10.31819530520674810 ) ) ;
#35561=CARTESIAN_POINT ( 'NONE',  ( 207.0548180518391916, 272.0175305127218053, 7.721676452263806389 ) ) ;
#35562=EDGE_CURVE ( 'NONE', #20729, #62642, #45556, .T. ) ;
#35563=CARTESIAN_POINT ( 'NONE',  ( 193.8365934467825298, 294.9121671145370556, 14.14845633038902584 ) ) ;
#35564=CARTESIAN_POINT ( 'NONE',  ( 153.3682214589191517, 265.3887646446434587, -16.19041097722891109 ) ) ;
#35565=CARTESIAN_POINT ( 'NONE',  ( 146.3569154618635366, 243.7592609112379876, 2.679491924311254714 ) ) ;
#35573=CARTESIAN_POINT ( 'NONE',  ( 152.9138932732664671, 277.5051963946797287, -5.211359010245092627 ) ) ;
#35574=ORIENTED_EDGE ( 'NONE', *, *, #2894, .F. ) ;
#35575=CARTESIAN_POINT ( 'NONE',  ( 104.4503548538631463, 241.1115022471902876, -5.000000000000047962 ) ) ;
#35576=ADVANCED_FACE ( 'NONE', ( #85384 ), #24596, .F. ) ;
#35580=ORIENTED_EDGE ( 'NONE', *, *, #94392, .T. ) ;
#35581=CARTESIAN_POINT ( 'NONE',  ( 153.4242699508872647, 264.9083646613370320, 16.62000820703435267 ) ) ;
#35582=CARTESIAN_POINT ( 'NONE',  ( 148.8004271348772249, 276.2543922634745286, -5.595754242233163644 ) ) ;
#35584=CARTESIAN_POINT ( 'NONE',  ( 202.7676489560256528, 279.4431252073101746, -16.04062356091568020 ) ) ;
#35587=CARTESIAN_POINT ( 'NONE',  ( 165.1220565656817882, 246.3610340376649788, -4.369863341033457971 ) ) ;
#35588=CARTESIAN_POINT ( 'NONE',  ( 163.8147431267737204, 246.9115372060205118, 7.125417796469586840 ) ) ;
#35589=CARTESIAN_POINT ( 'NONE',  ( 153.0070714074088016, 265.6309737354857248, 17.74442213480098474 ) ) ;
#35597=ORIENTED_EDGE ( 'NONE', *, *, #40551, .F. ) ;
#35598=CARTESIAN_POINT ( 'NONE',  ( 177.0175048079005080, 269.3060889572638530, 16.09599001003793006 ) ) ;
#35599=CARTESIAN_POINT ( 'NONE',  ( 165.0020474182383339, 244.8550658491588479, 1.825383354618924425 ) ) ;
#35601=ORIENTED_EDGE ( 'NONE', *, *, #17188, .F. ) ;
#35602=CARTESIAN_POINT ( 'NONE',  ( 174.7676448104877807, 277.4213516129615869, -15.64693699161624352 ) ) ;
#35603=CARTESIAN_POINT ( 'NONE',  ( 169.6734611486750453, 261.6087119384134212, -16.67296044893563689 ) ) ;
#35604=VERTEX_POINT ( 'NONE', #72160 ) ;
#35606=B_SPLINE_CURVE_WITH_KNOTS ( 'NONE', 3,
 ( #21200, #12097, #13593, #36879 ),
 .UNSPECIFIED., .F., .F.,
 ( 4, 4 ),
 ( 0.01336260375758639186, 0.02197367245289875287 ),
 .UNSPECIFIED. ) ;
#35607=ORIENTED_EDGE ( 'NONE', *, *, #38002, .F. ) ;
#35609=EDGE_LOOP ( 'NONE', ( #94564, #23035, #2014, #43179 ) ) ;
#35610=CARTESIAN_POINT ( 'NONE',  ( 156.3075079012271260, 267.3199146548383283, -16.47880472041608968 ) ) ;
#35611=CARTESIAN_POINT ( 'NONE',  ( 190.6954410837624607, 300.3528026016029457, -5.728531842148099962 ) ) ;
#35614=CARTESIAN_POINT ( 'NONE',  ( 192.7944000592152634, 296.7172990131160759, 11.44860011299869740 ) ) ;
#35618=B_SPLINE_CURVE_WITH_KNOTS ( 'NONE', 3,
 ( #74049, #66433, #42616, #26941 ),
 .UNSPECIFIED., .F., .F.,
 ( 4, 4 ),
 ( 1.260064970365687123E-16, 0.004705947932869557031 ),
 .UNSPECIFIED. ) ;
#35620=CARTESIAN_POINT ( 'NONE',  ( 206.4695239676918845, 273.0312896038346366, 10.41704154450801667 ) ) ;
#35621=CARTESIAN_POINT ( 'NONE',  ( 149.4908848037268001, 271.7211875819559737, -12.92288068979413573 ) ) ;
#35622=CARTESIAN_POINT ( 'NONE',  ( 176.1545129615995791, 279.8491840402730304, -16.65846268951813158 ) ) ;
#35623=CARTESIAN_POINT ( 'NONE',  ( 159.6419305724666344, 254.1390605605417079, 16.92015248457581933 ) ) ;
#35624=ORIENTED_EDGE ( 'NONE', *, *, #41974, .T. ) ;
#35625=CARTESIAN_POINT ( 'NONE',  ( 176.5942392360894928, 290.0311217938273103, -9.473091939615279955 ) ) ;
#35626=VERTEX_POINT ( 'NONE', #86396 ) ;
#35627=CARTESIAN_POINT ( 'NONE',  ( 186.6370815005770112, 276.6162495332958997, 16.64778423223098613 ) ) ;
#35629=CARTESIAN_POINT ( 'NONE',  ( 163.7412020991711756, 247.5884774922407416, 7.473643870864920657 ) ) ;
#35631=CARTESIAN_POINT ( 'NONE',  ( 190.1092758455735918, 301.3680705757765850, -1.432918395251892019 ) ) ;
#35633=CARTESIAN_POINT ( 'NONE',  ( 170.5400372565194971, 255.6862325933128659, -12.52260723181821156 ) ) ;
#35635=CARTESIAN_POINT ( 'NONE',  ( 53.71569994882479193, 208.4865022471902876, -10.00000000000009592 ) ) ;
#35637=CARTESIAN_POINT ( 'NONE',  ( 21.94339294393528306, 190.1427522451419350, 10.00000000000009237 ) ) ;
#35638=CARTESIAN_POINT ( 'NONE',  ( 98.36111373172988692, 227.5958772461660260, -9.188101187500095079 ) ) ;
#35639=ADVANCED_FACE ( 'NONE', ( #16928 ), #93374, .F. ) ;
#35640=CARTESIAN_POINT ( 'NONE',  ( 169.5606897086885283, 261.7245448792994580, 16.76904778814408559 ) ) ;
#35642=CARTESIAN_POINT ( 'NONE',  ( 157.1606030646430554, 258.4368458743103361, 17.96998724893680688 ) ) ;
#35643=CARTESIAN_POINT ( 'NONE',  ( 163.1394982460384995, 248.0810956470044175, 11.48951572717839298 ) ) ;
#35644=CARTESIAN_POINT ( 'NONE',  ( 19.47135178391741661, 191.2369531367911293, -4.594050593750048428 ) ) ;
#35645=FACE_OUTER_BOUND ( 'NONE', #73719, .T. ) ;
#35646=ORIENTED_EDGE ( 'NONE', *, *, #23458, .T. ) ;
#35650=EDGE_CURVE ( 'NONE', #10047, #95964, #40971, .T. ) ;
#35655=CARTESIAN_POINT ( 'NONE',  ( 161.8408514536557163, 250.3304178724980318, -14.12919723462510646 ) ) ;
#35656=CARTESIAN_POINT ( 'NONE',  ( 179.1906477385719541, 287.9874793598855831, -12.80386165526534370 ) ) ;
#35657=CARTESIAN_POINT ( 'NONE',  ( 168.1482817187297485, 251.7781618965069299, 10.54809081625006328 ) ) ;
#35658=CARTESIAN_POINT ( 'NONE',  ( 42.82723471405275717, 195.5333772461660544, 9.188101187500095079 ) ) ;
#35659=CARTESIAN_POINT ( 'NONE',  ( 89.99855592466245469, 222.7677522451418781, 10.00000000000009592 ) ) ;
#35660=EDGE_LOOP ( 'NONE', ( #51543, #43856, #9727, #6446 ) ) ;
#35661=CARTESIAN_POINT ( 'NONE',  ( 194.7854625312828887, 266.3706711642819300, -7.713939373946292477 ) ) ;
#35662=CARTESIAN_POINT ( 'NONE',  ( 178.7744559918192806, 259.2102874926480354, -10.28428999224912843 ) ) ;
#35663=FACE_OUTER_BOUND ( 'NONE', #1469, .T. ) ;
#35664=CARTESIAN_POINT ( 'NONE',  ( 2.042590532755589994, 181.1744531367911577, 4.594050593750047540 ) ) ;
#35665=CARTESIAN_POINT ( 'NONE',  ( 199.2383506163646132, 285.5560492466715345, -17.78808061564097898 ) ) ;
#35668=CARTESIAN_POINT ( 'NONE',  ( 52.94873307290088604, 207.5024278399160949, 9.188101187500095079 ) ) ;
#35670=CARTESIAN_POINT ( 'NONE',  ( 203.8280627875664663, 275.9321709329971100, 13.16261023213589709 ) ) ;
#35673=ORIENTED_EDGE ( 'NONE', *, *, #79642, .T. ) ;
#35674=( BOUNDED_CURVE ( )  B_SPLINE_CURVE ( 2, ( #91608, #67275, #98202, #68767, #59664, #27793, #29292, #82031, #44969 ),
 .UNSPECIFIED., .F., .T. ) 
 B_SPLINE_CURVE_WITH_KNOTS ( ( 3, 2, 2, 2, 3 ),
 ( 0.4717741935483871218, 0.4731182795698924970, 0.4758064516129032473, 0.4784946236559139976, 0.4798387096774193727 ),
 .UNSPECIFIED. ) 
 CURVE ( )  GEOMETRIC_REPRESENTATION_ITEM ( )  RATIONAL_B_SPLINE_CURVE ( ( 0.9330127018922194093, 0.9330127018922194093, 1.000000000000000000, 0.8660254037844387076, 1.000000000000000000, 0.8660254037844387076, 1.000000000000000000, 0.9330127018922194093, 0.9330127018922194093 ) ) 
 REPRESENTATION_ITEM ( '' )  );
#35677=CARTESIAN_POINT ( 'NONE',  ( 8.826716519331432309, 169.2365022471902023, 10.00000000000009592 ) ) ;
#35679=CARTESIAN_POINT ( 'NONE',  ( 125.6948669907937415, 249.5024278399160949, 9.188101187500095079 ) ) ;
#35681=CARTESIAN_POINT ( 'NONE',  ( 207.4646420400604541, 271.3076945429622242, -8.143883892282612891 ) ) ;
#35683=B_SPLINE_CURVE_WITH_KNOTS ( 'NONE', 3,
 ( #48144, #31932, #16745, #78060 ),
 .UNSPECIFIED., .F., .F.,
 ( 4, 4 ),
 ( 0.007396415386818002910, 0.01554756812702462465 ),
 .UNSPECIFIED. ) ;
#35686=CARTESIAN_POINT ( 'NONE',  ( 188.9633349269510632, 289.6955772790231549, 14.43551268334040749 ) ) ;
#35687=EDGE_CURVE ( 'NONE', #18677, #20915, #21919, .T. ) ;
#35688=CARTESIAN_POINT ( 'NONE',  ( 150.3969908582963342, 270.1517658583956631, -13.88764202390153990 ) ) ;
#35689=ORIENTED_EDGE ( 'NONE', *, *, #54153, .F. ) ;
#35690=CARTESIAN_POINT ( 'NONE',  ( 196.7232418867741046, 263.8072851099263403, -0.2693295688966246271 ) ) ;
#35691=CARTESIAN_POINT ( 'NONE',  ( 207.6758789170519890, 270.9418215395808147, -0.5923825352568967695 ) ) ;
#35692=CARTESIAN_POINT ( 'NONE',  ( 181.6045319792032444, 288.0095535211878541, 13.87245391538852601 ) ) ;
#35693=CARTESIAN_POINT ( 'NONE',  ( 172.4831635826484444, 290.8796410925290843, -1.652085212636280609 ) ) ;
#35697=CARTESIAN_POINT ( 'NONE',  ( 171.0717129997618144, 284.5853248254017558, -11.57144567159876836 ) ) ;
#35698=EDGE_CURVE ( 'NONE', #33648, #99290, #63696, .T. ) ;
#35701=CARTESIAN_POINT ( 'NONE',  ( 182.1983635332545646, 295.7656116556308916, 4.955917269626422872 ) ) ;
#35704=CARTESIAN_POINT ( 'NONE',  ( 150.0648941724952863, 277.2273145327603174, -9.121012261533550361E-05 ) ) ;
#35705=CARTESIAN_POINT ( 'NONE',  ( 193.1829427640170422, 282.2301301676865819, 16.90027158358297044 ) ) ;
#35707=CARTESIAN_POINT ( 'NONE',  ( 93.10181362155671536, 217.8927522451418213, 10.00000000000009948 ) ) ;
#35710=CARTESIAN_POINT ( 'NONE',  ( 156.0362208818770569, 261.9694580292082264, -16.96406285719872642 ) ) ;
#35711=ORIENTED_EDGE ( 'NONE', *, *, #68305, .T. ) ;
#35712=CARTESIAN_POINT ( 'NONE',  ( 146.6138605399200117, 276.7043397814778132, -0.5394499176159462950 ) ) ;
#35713=CARTESIAN_POINT ( 'NONE',  ( 205.4834637267509549, 273.3784298103438459, -9.787331926331344079 ) ) ;
#35714=CARTESIAN_POINT ( 'NONE',  ( 204.9608076533459950, 275.6444629144898499, 14.31488288944633069 ) ) ;
#35717=CARTESIAN_POINT ( 'NONE',  ( 78.06346978264959091, 222.0024278399160949, -9.188101187500093303 ) ) ;
#35718=CARTESIAN_POINT ( 'NONE',  ( 203.4986178427917878, 278.1770499566792409, 15.08380016308619176 ) ) ;
#35721=CARTESIAN_POINT ( 'NONE',  ( 184.9950698617867886, 259.9054437811999492, -5.827971615141458450 ) ) ;
#35723=VERTEX_POINT ( 'NONE', #98449 ) ;
#35726=CARTESIAN_POINT ( 'NONE',  ( 192.6537829138044344, 294.0124578573780241, 14.33366951991050442 ) ) ;
#35727=B_SPLINE_CURVE_WITH_KNOTS ( 'NONE', 3,
 ( #16797, #93336, #54791, #8207 ),
 .UNSPECIFIED., .F., .F.,
 ( 4, 4 ),
 ( 0.009413270483557435037, 0.01469873868365958840 ),
 .UNSPECIFIED. ) ;
#35728=EDGE_CURVE ( 'NONE', #78211, #51310, #29780, .T. ) ;
#35731=DIRECTION ( 'NONE',  ( 0.8660254037844395958, 0.4999999999999985567, 0.000000000000000000 ) ) ;
#35733=CARTESIAN_POINT ( 'NONE',  ( 164.7596289686694888, 245.2749469205039929, 2.483240442660407776 ) ) ;
#35735=CARTESIAN_POINT ( 'NONE',  ( 181.0193311394079103, 261.5502185760933003, 13.24438261311760812 ) ) ;
#35738=CARTESIAN_POINT ( 'NONE',  ( 147.9133274879049793, 274.4535970048112290, -9.359166267164972908 ) ) ;
#35740=CARTESIAN_POINT ( 'NONE',  ( 168.3561001772640680, 267.2114426321716110, -17.22163279015371629 ) ) ;
#35746=CARTESIAN_POINT ( 'NONE',  ( 200.9124443442758832, 270.6563311349291894, 9.292281936012786403 ) ) ;
#35747=ORIENTED_EDGE ( 'NONE', *, *, #55395, .F. ) ;
#35750=CARTESIAN_POINT ( 'NONE',  ( 161.3049863899956335, 281.4170748028290063, -6.576827861606494352 ) ) ;
#35751=CARTESIAN_POINT ( 'NONE',  ( -17.42236680055705023, 149.2012482093457777, 0.000000000000000000 ) ) ;
#35752=B_SPLINE_CURVE_WITH_KNOTS ( 'NONE', 3,
 ( #40497, #1019, #3047, #16213, #32903, #16711, #31900, #78027, #70410, #62804, #49118, #32415, #80055, #24805, #2532, #72441, #33414, #33934, #17723, #93760, #63812, #48106, #79049, #78532, #56195, #94745 ),
 .UNSPECIFIED., .F., .F.,
 ( 4, 2, 2, 2, 2, 2, 2, 2, 2, 2, 2, 2, 4 ),
 ( 0.0002565227521606977881, 0.001765950409300323740, 0.001860289637871517755, 0.001907459252157120075, 0.001931044059299878409, 0.001954628866442637176, 0.002001798480728315607, 0.002048968095013994038, 0.002143307323585351334, 0.002331985780728105823, 0.002520664237870861180, 0.002898021152156497662, 0.003275378066442135010 ),
 .UNSPECIFIED. ) ;
#35756=ORIENTED_EDGE ( 'NONE', *, *, #87066, .T. ) ;
#35757=CARTESIAN_POINT ( 'NONE',  ( 181.4793763127861439, 271.1882028957970761, -15.96622495013739673 ) ) ;
#35759=ORIENTED_EDGE ( 'NONE', *, *, #25243, .T. ) ;
#35760=CARTESIAN_POINT ( 'NONE',  ( 159.9950753608005130, 276.8117990079294373, 13.35014033362692487 ) ) ;
#35761=EDGE_CURVE ( 'NONE', #73611, #97734, #79354, .T. ) ;
#35762=CARTESIAN_POINT ( 'NONE',  ( 174.6037846674788341, 281.1587274802971592, -14.18186885202987924 ) ) ;
#35763=CARTESIAN_POINT ( 'NONE',  ( 167.5505310038667517, 261.6318463984700315, 17.07012949051403439 ) ) ;
#35764=CARTESIAN_POINT ( 'NONE',  ( 190.2389970918280540, 301.1433867864428748, 4.601241515604689525 ) ) ;
#35765=CARTESIAN_POINT ( 'NONE',  ( 163.9695846725937542, 274.0645315248153224, 14.77959389856284389 ) ) ;
#35767=CARTESIAN_POINT ( 'NONE',  ( 151.2850021181167222, 275.2870477160321343, -9.752878341108868199 ) ) ;
#35775=CARTESIAN_POINT ( 'NONE',  ( 175.5786161558440881, 290.9456444599823044, 2.588591708581580608 ) ) ;
#35776=CARTESIAN_POINT ( 'NONE',  ( 153.4619471835925708, 264.8431057800031567, 16.95044998314351758 ) ) ;
#35777=ADVANCED_FACE ( 'NONE', ( #17832 ), #16499, .F. ) ;
#35780=CARTESIAN_POINT ( 'NONE',  ( 162.1260167985288376, 266.6785162637209510, 17.71249957499354366 ) ) ;
#35781=CARTESIAN_POINT ( 'NONE',  ( 10.18907585680922878, 170.5643266524159571, -9.188101187500093303 ) ) ;
#35782=CARTESIAN_POINT ( 'NONE',  ( 108.5912123618160763, 227.3768266524159856, -9.188101187500091527 ) ) ;
#35784=CARTESIAN_POINT ( 'NONE',  ( 183.5370458253748041, 294.2335165497496519, -7.795347451710910924 ) ) ;
#35787=CARTESIAN_POINT ( 'NONE',  ( 193.7901930790854976, 294.9925349088783264, 14.24765323155741115 ) ) ;
#35788=CARTESIAN_POINT ( 'NONE',  ( 147.9133274879049793, 274.4535970048112290, -9.359166267164972908 ) ) ;
#35790=CARTESIAN_POINT ( 'NONE',  ( 196.1785470034112109, 266.7132032025372723, 8.042115761827414389 ) ) ;
#35791=CARTESIAN_POINT ( 'NONE',  ( 170.7191605745771597, 286.8649585537148710, -9.393374115909271183 ) ) ;
#35797=CARTESIAN_POINT ( 'NONE',  ( 91.40610752940987993, 214.3923013555409796, 4.594050593750050204 ) ) ;
#35799=FACE_OUTER_BOUND ( 'NONE', #25002, .T. ) ;
#35800=CARTESIAN_POINT ( 'NONE',  ( 196.3021893095863959, 290.6416298092292436, 17.45656988653421138 ) ) ;
#35801=CARTESIAN_POINT ( 'NONE',  ( 152.4488546850150499, 266.5978334603062194, 15.77325388060940625 ) ) ;
#35802=CARTESIAN_POINT ( 'NONE',  ( 149.7453127691109387, 271.2805054190442888, 12.04833158289322981 ) ) ;
#35803=B_SPLINE_CURVE_WITH_KNOTS ( 'NONE', 3,
 ( #32937, #86701, #24348, #17757 ),
 .UNSPECIFIED., .F., .F.,
 ( 4, 4 ),
 ( 0.007593230830505486723, 0.01264584417670786519 ),
 .UNSPECIFIED. ) ;
#35807=CARTESIAN_POINT ( 'NONE',  ( 147.4563929227680603, 275.2450308873625886, -3.847749617713808412 ) ) ;
#35812=CARTESIAN_POINT ( 'NONE',  ( 146.8574506849497538, 276.2824292740633041, -4.888313306692038118 ) ) ;
#35813=CARTESIAN_POINT ( 'NONE',  ( 191.3641415966465900, 288.6821316927074008, -16.06258504083237071 ) ) ;
#35817=DIRECTION ( 'NONE',  ( -0.8660254037844387076, -0.4999999999999998890, -0.000000000000000000 ) ) ;
#35820=CARTESIAN_POINT ( 'NONE',  ( 138.7305270869972560, 244.2365022471902023, 10.00000000000009592 ) ) ;
#35821=CARTESIAN_POINT ( 'NONE',  ( 157.0978663001774862, 258.5455091378672137, -17.31223197570816552 ) ) ;
#35824=CARTESIAN_POINT ( 'NONE',  ( 169.5921219636811657, 248.4220618532164906, -1.949161244724071151 ) ) ;
#35826=FACE_OUTER_BOUND ( 'NONE', #10197, .T. ) ;
#35828=ORIENTED_EDGE ( 'NONE', *, *, #93311, .F. ) ;
#35831=CARTESIAN_POINT ( 'NONE',  ( 192.6276150426703850, 292.1813556936259033, 14.97627272081470018 ) ) ;
#35833=CARTESIAN_POINT ( 'NONE',  ( 150.1064787036151245, 245.2202760586659736, -5.415160957724236172E-17 ) ) ;
#35834=CARTESIAN_POINT ( 'NONE',  ( 204.0439772608724525, 272.7860293576995900, 11.11986000170599453 ) ) ;
#35835=CARTESIAN_POINT ( 'NONE',  ( 192.6636420411112169, 296.3681834598817773, -11.78089681376212638 ) ) ;
#35837=B_SPLINE_CURVE_WITH_KNOTS ( 'NONE', 3,
 ( #7883, #24563, #92997, #93509 ),
 .UNSPECIFIED., .F., .F.,
 ( 4, 4 ),
 ( 0.006163542666752603802, 0.01183985020392103529 ),
 .UNSPECIFIED. ) ;
#35840=CARTESIAN_POINT ( 'NONE',  ( 165.5076143076621520, 274.9436888840691040, 14.75253031382487556 ) ) ;
#35843=AXIS2_PLACEMENT_3D ( 'NONE', #67088, #90452, #1193 ) ;
#35844=ORIENTED_EDGE ( 'NONE', *, *, #68247, .T. ) ;
#35846=B_SPLINE_CURVE_WITH_KNOTS ( 'NONE', 3,
 ( #45425, #53527, #8437, #54010, #16030, #46932, #91569, #99653, #54505, #76360, #84968, #22141, #15513, #53031, #6931, #829, #83985, #85483, #84478, #31223, #39305, #69727, #93566, #45911, #332, #76830, #46415, #7427, #77849, #100156, #30742, #92574, #61619, #23118, #24133, #80382, #32727, #96079, #33753, #63631, #71252, #95082, #56006, #25646, #1342, #10952, #32227, #9437 ),
 .UNSPECIFIED., .F., .F.,
 ( 4, 2, 2, 2, 2, 2, 2, 2, 2, 2, 2, 2, 2, 2, 2, 2, 2, 2, 2, 2, 2, 2, 2, 4 ),
 ( 0.0002180751697494367309, 0.0006991417601631947807, 0.001180208350576952966, 0.001420741645783869843, 0.001541008293387322210, 0.001661274940990775011, 0.001781541588594227378, 0.001901808236197679962, 0.002142341531404522680, 0.002623408121818276203, 0.003104474712232029726, 0.004066607893059384984, 0.005028741073886740243, 0.005509807664300423076, 0.005750340959507223293, 0.005870607607110583069, 0.005990874254713943713, 0.006051007578515663066, 0.006111140902317381551, 0.006231407549920868830, 0.006471940845127756650, 0.006953007435541381370, 0.007434074025955006090, 0.007915140616368630810 ),
 .UNSPECIFIED. ) ;
#35847=DIRECTION ( 'NONE',  ( -0.8660254037844387076, -0.4999999999999998890, -0.000000000000000000 ) ) ;
#35848=CARTESIAN_POINT ( 'NONE',  ( 162.4690895575259901, 272.5881697659471570, -16.26466664224244241 ) ) ;
#35850=DIRECTION ( 'NONE',  ( 0.4999999999999992784, -0.8660254037844390407, 0.000000000000000000 ) ) ;
#35851=CARTESIAN_POINT ( 'NONE',  ( 152.9052392069962991, 268.7302753513774860, -15.74331135679841687 ) ) ;
#35854=CARTESIAN_POINT ( 'NONE',  ( 169.7687919401275565, 267.4058426616630300, 17.40508201545849687 ) ) ;
#35855=DIRECTION ( 'NONE',  ( 0.8660254037844395958, 0.4999999999999985567, 0.000000000000000000 ) ) ;
#35856=CARTESIAN_POINT ( 'NONE',  ( 100.4182711614829486, 216.5327760586659451, 1.948934522072303157E-15 ) ) ;
#35857=CARTESIAN_POINT ( 'NONE',  ( 148.4958247551113288, 275.2668892720577105, -7.172227964493664842 ) ) ;
#35858=CARTESIAN_POINT ( 'NONE',  ( 166.6214840706217046, 278.0950532397310440, -13.36420821935662318 ) ) ;
#35860=VERTEX_POINT ( 'NONE', #97830 ) ;
#35862=CARTESIAN_POINT ( 'NONE',  ( -22.42236680055709641, 157.8615022471902591, 0.000000000000000000 ) ) ;
#35863=CARTESIAN_POINT ( 'NONE',  ( 196.4390255720217908, 290.4046224503736653, 16.34739044515864848 ) ) ;
#35864=CARTESIAN_POINT ( 'NONE',  ( 164.0212554996149379, 272.3286311233993615, -16.82199824294186286 ) ) ;
#35868=LINE ( 'NONE', #82531, #51087 ) ;
#35870=B_SPLINE_CURVE_WITH_KNOTS ( 'NONE', 3,
 ( #10002, #86550, #9503, #40865, #94626, #26196, #87570, #39858, #72314, #2408, #32780, #63689, #63186, #40369 ),
 .UNSPECIFIED., .F., .F.,
 ( 4, 2, 2, 2, 2, 2, 4 ),
 ( 0.001036889160286317679, 0.001285291995625097812, 0.001533694830963879029, 0.001782097666302660246, 0.002030500501641441247, 0.002527306172318979395, 0.003024111842996517977 ),
 .UNSPECIFIED. ) ;
#35871=CARTESIAN_POINT ( 'NONE',  ( 191.4659329597417923, 264.0196791935998135, -7.956612423567304582 ) ) ;
#35872=CARTESIAN_POINT ( 'NONE',  ( 103.4423036115607601, 218.9824982072974251, 3.021315404115420679E-15 ) ) ;
#35874=CARTESIAN_POINT ( 'NONE',  ( 127.9681836757279001, 250.8149278399160949, 9.188101187500093303 ) ) ;
#35875=CARTESIAN_POINT ( 'NONE',  ( 198.9438511131552332, 284.5686006854416519, 17.54420169616632563 ) ) ;
#35878=CARTESIAN_POINT ( 'NONE',  ( 190.7569505155522904, 300.2462651405980978, -5.670926626284815697 ) ) ;
#35882=CARTESIAN_POINT ( 'NONE',  ( 178.5664908309598218, 285.2175874337613664, 13.98765452350090577 ) ) ;
#35885=CARTESIAN_POINT ( 'NONE',  ( 198.8109706115596964, 282.3938570165372539, -17.09471128148272356 ) ) ;
#35890=EDGE_CURVE ( 'NONE', #54644, #19179, #95144, .T. ) ;
#35891=CARTESIAN_POINT ( 'NONE',  ( 58.44249495421716745, 213.7369531367911293, -4.594050593750048428 ) ) ;
#35892=CARTESIAN_POINT ( 'NONE',  ( 159.5221561062548972, 254.3465160214695118, -16.91023001054109542 ) ) ;
#35894=CARTESIAN_POINT ( 'NONE',  ( 187.3153774383709163, 290.1783631386096545, -14.94016741271708248 ) ) ;
#35898=CARTESIAN_POINT ( 'NONE',  ( 185.9435401644106776, 265.4574032316044168, 13.60664360879022716 ) ) ;
#35901=CARTESIAN_POINT ( 'NONE',  ( -22.42236680055709641, 157.8615022471902591, 0.000000000000000000 ) ) ;
#35904=CARTESIAN_POINT ( 'NONE',  ( 6.805730253569997501, 183.9244531367911293, -4.594050593750046652 ) ) ;
#35907=CARTESIAN_POINT ( 'NONE',  ( 157.8740713127050981, 257.2010826190796706, 17.31862062017425075 ) ) ;
#35909=CARTESIAN_POINT ( 'NONE',  ( 35.67350403664903524, 184.7365022471902023, -10.00000000000009237 ) ) ;
#35910=CARTESIAN_POINT ( 'NONE',  ( 164.2090401137261892, 246.2285947913476889, -5.787448100099915393 ) ) ;
#35912=CARTESIAN_POINT ( 'NONE',  ( 51.05482314576993730, 188.0327760586659451, 1.948934522072302763E-15 ) ) ;
#35915=CARTESIAN_POINT ( 'NONE',  ( 146.8195026170398023, 276.3481572557323034, 4.765869558735466249 ) ) ;
#35918=CARTESIAN_POINT ( 'NONE',  ( 191.3413020738616410, 299.2341385521244774, -8.295023558158421295 ) ) ;
#35919=CARTESIAN_POINT ( 'NONE',  ( 177.2780219866808977, 275.6134775628974580, 17.64509040511156357 ) ) ;
#35924=CARTESIAN_POINT ( 'NONE',  ( 97.88299554183117834, 233.9865022471902876, -10.00000000000009415 ) ) ;
#35926=CARTESIAN_POINT ( 'NONE',  ( 163.3405847382477702, 268.5890301281064012, -16.46197277963260674 ) ) ;
#35927=ORIENTED_EDGE ( 'NONE', *, *, #94458, .F. ) ;
#35928=CARTESIAN_POINT ( 'NONE',  ( 60.41820218054165537, 211.8149278399160664, 9.188101187500093303 ) ) ;
#35930=CARTESIAN_POINT ( 'NONE',  ( 165.9205590267122830, 265.2445089552724085, 16.56339371490548729 ) ) ;
#35931=CARTESIAN_POINT ( 'NONE',  ( 190.6218339396177441, 300.4802939150614520, -4.178005820806754755 ) ) ;
#35934=CARTESIAN_POINT ( 'NONE',  ( 71.12873073640183463, 200.3262482093457777, 3.021315404115420679E-15 ) ) ;
#35935=CARTESIAN_POINT ( 'NONE',  ( 207.6209998424140792, 271.0368748851258260, 6.610167240481342965 ) ) ;
#35938=CARTESIAN_POINT ( 'NONE',  ( 186.0008503584107871, 263.4848601604851410, 10.99485596832306378 ) ) ;
#35939=CARTESIAN_POINT ( 'NONE',  ( 152.5994661946046449, 279.2824469453463507, 2.533033137138181345 ) ) ;
#35941=CARTESIAN_POINT ( 'NONE',  ( 156.7786475906069938, 259.0984121615696836, 17.12081851550279055 ) ) ;
#35949=CARTESIAN_POINT ( 'NONE',  ( 182.5313270724992663, 283.9550808915877269, 15.13072720056265297 ) ) ;
#35951=CARTESIAN_POINT ( 'NONE',  ( 206.8106726053982811, 272.4404028303941914, -10.47827087991598560 ) ) ;
#35953=CARTESIAN_POINT ( 'NONE',  ( 207.1019571622349815, 271.9358831784929293, -5.989975140547304733 ) ) ;
#35958=CARTESIAN_POINT ( 'NONE',  ( 198.0792648159935538, 287.5636447432459022, 17.04758482866669667 ) ) ;
#35959=CARTESIAN_POINT ( 'NONE',  ( 156.3551087084618700, 261.3239775484371989, -17.56576820129662053 ) ) ;
#35960=CARTESIAN_POINT ( 'NONE',  ( 204.7775947223805417, 271.9956584674009719, 9.991586326987553335 ) ) ;
#35961=EDGE_CURVE ( 'NONE', #52858, #39606, #76515, .T. ) ;
#35962=CARTESIAN_POINT ( 'NONE',  ( 122.0685591603289026, 241.2833772461660544, -9.188101187500095079 ) ) ;
#35966=ORIENTED_EDGE ( 'NONE', *, *, #51197, .F. ) ;
#35968=CARTESIAN_POINT ( 'NONE',  ( 198.5966822647444587, 286.6674514332866579, 17.25284514431582750 ) ) ;
#35970=CARTESIAN_POINT ( 'NONE',  ( 79.20030167299918844, 216.5333772461660544, 9.188101187500095079 ) ) ;
#35971=DIRECTION ( 'NONE',  ( 0.4999999999999992784, -0.8660254037844390407, 0.000000000000000000 ) ) ;
#35974=CARTESIAN_POINT ( 'NONE',  ( 150.8677798231829570, 269.3363354515693118, 13.85464777478129150 ) ) ;
#35975=CARTESIAN_POINT ( 'NONE',  ( 173.0842668126385888, 277.1454467833098079, 15.65064250236792809 ) ) ;
#35976=CARTESIAN_POINT ( 'NONE',  ( 182.1335790983844163, 257.1430377582902338, -6.167898280431136193 ) ) ;
#35977=EDGE_LOOP ( 'NONE', ( #27628, #15298, #8090, #41684 ) ) ;
#35980=CARTESIAN_POINT ( 'NONE',  ( 155.5066938333533528, 261.3015006940112244, -18.40036130547566273 ) ) ;
#35984=CARTESIAN_POINT ( 'NONE',  ( 165.1088727524893329, 246.3087121452358303, 4.054724759575032422 ) ) ;
#35986=CARTESIAN_POINT ( 'NONE',  ( 149.0244553356880886, 274.5290671187512999, 9.114935767028397251 ) ) ;
#35987=CARTESIAN_POINT ( 'NONE',  ( 149.2593905435863348, 272.1221474021800759, -12.98626158366800176 ) ) ;
#35988=CARTESIAN_POINT ( 'NONE',  ( 194.9232784475534856, 279.6201759093600572, 16.73569595568872614 ) ) ;
#35990=CARTESIAN_POINT ( 'NONE',  ( 207.5215400641004351, 271.2091442744748520, 2.886080616848571534 ) ) ;
#35991=CARTESIAN_POINT ( 'NONE',  ( 135.2211464324225858, 255.0024278399160949, -9.188101187500093303 ) ) ;
#35992=VERTEX_POINT ( 'NONE', #78011 ) ;
#35994=CARTESIAN_POINT ( 'NONE',  ( 182.7048629724877742, 257.5630761932868609, 6.780981931134482110 ) ) ;
#35997=CARTESIAN_POINT ( 'NONE',  ( 204.8523313866422484, 275.8323493198358847, 14.65426965484541100 ) ) ;
#35998=DIRECTION ( 'NONE',  ( -0.8660254037844387076, -0.4999999999999998890, -0.000000000000000000 ) ) ;
#35999=CARTESIAN_POINT ( 'NONE',  ( 178.7223853007603793, 254.2491090711346260, 4.616854984815845775 ) ) ;
#36002=CARTESIAN_POINT ( 'NONE',  ( 182.3945381577018736, 275.1057528038260784, -16.87030083329184649 ) ) ;
#36003=CARTESIAN_POINT ( 'NONE',  ( 167.1998709608827767, 248.9378275210275149, -5.484025092681479308 ) ) ;
#36004=CARTESIAN_POINT ( 'NONE',  ( 164.3104563928357322, 246.0529366432151051, -1.966241142131954334 ) ) ;
#36006=CARTESIAN_POINT ( 'NONE',  ( 198.4846960687163460, 266.2207596311699263, 0.7325185302305462498 ) ) ;
#36008=CARTESIAN_POINT ( 'NONE',  ( 147.4811722709131914, 275.2021117973970377, 3.890385073228495916 ) ) ;
#36009=CARTESIAN_POINT ( 'NONE',  ( 182.8590536091604406, 280.6449140202259969, 16.90169854257041848 ) ) ;
#36011=CARTESIAN_POINT ( 'NONE',  ( 157.3661765229227285, 258.0807821998820373, -18.27254492731150748 ) ) ;
#36012=CARTESIAN_POINT ( 'NONE',  ( 196.3706589808440981, 270.6234002145578756, 11.85799053031749040 ) ) ;
#36013=B_SPLINE_SURFACE_WITH_KNOTS ( 'NONE', 3, 1, ( 
 ( #66730, #44423 ),
 ( #90591, #67227 ),
 ( #97663, #59105 ),
 ( #28737, #21637 ),
 ( #20646, #21156 ),
 ( #82975, #75352 ),
 ( #34825, #3942 ),
 ( #36826, #91074 ),
 ( #80997, #42421 ),
 ( #45897, #46404 ),
 ( #91558, #99642 ),
 ( #77840, #39294 ),
 ( #7935, #92563 ),
 ( #22127, #92081 ),
 ( #31694, #76347 ),
 ( #7415, #15008 ),
 ( #84959, #37808 ),
 ( #8423, #14033 ),
 ( #69216, #84468 ),
 ( #53020, #68217 ),
 ( #6921, #61108 ),
 ( #46918, #83973 ),
 ( #62602, #77328 ),
 ( #70206, #38307 ),
 ( #45415, #100144 ),
 ( #14537, #15502 ),
 ( #23601, #69714 ),
 ( #38809, #44913 ),
 ( #30730, #99142 ),
 ( #30224, #52520 ),
 ( #68718, #75857 ),
 ( #61609, #23107 ),
 ( #322, #22629 ),
 ( #29729, #53998 ) ),
 .UNSPECIFIED., .T., .F., .F.,
 ( 4, 2, 2, 2, 2, 2, 2, 2, 2, 2, 2, 2, 2, 2, 2, 2, 4 ),
 ( 2, 2 ),
 ( 0.000000000000000000, 0.06250000000000000000, 0.1250000000000000000, 0.1875000000000000000, 0.2500000000000000000, 0.3125000000000000000, 0.3750000000000000000, 0.4375000000000000000, 0.5000000000000000000, 0.5625000000000000000, 0.6250000000000000000, 0.6875000000000000000, 0.7500000000000000000, 0.8125000000000000000, 0.8750000000000000000, 0.9375000000000000000, 1.000000000000000000 ),
 ( 0.000000000000000000, 1.000000000000000000 ),
 .UNSPECIFIED. ) ;
#36015=CARTESIAN_POINT ( 'NONE',  ( 149.6036070299368532, 271.5259469590175740, 11.63513718912356865 ) ) ;
#36016=CARTESIAN_POINT ( 'NONE',  ( 204.8583870631589150, 274.3003082388789267, 12.05194970354070527 ) ) ;
#36017=CARTESIAN_POINT ( 'NONE',  ( 159.4230536986738400, 254.5181664265525683, 16.83068086755798376 ) ) ;
#36020=CARTESIAN_POINT ( 'NONE',  ( 145.7850256851100994, 241.6427522451417644, 1.119607411625061291E-15 ) ) ;
#36021=CARTESIAN_POINT ( 'NONE',  ( 175.9868547499085025, 285.4643737892969853, -11.94532051846830534 ) ) ;
#36022=ORIENTED_EDGE ( 'NONE', *, *, #44100, .F. ) ;
#36024=CARTESIAN_POINT ( 'NONE',  ( 157.5710319558766344, 257.7259621817996162, 18.28704422422941533 ) ) ;
#36025=CARTESIAN_POINT ( 'NONE',  ( 198.4782858197754649, 286.8725200914082620, -17.44895083299520522 ) ) ;
#36026=CARTESIAN_POINT ( 'NONE',  ( 13.92363686274711299, 178.8458772461660544, 9.188101187500095079 ) ) ;
#36027=CARTESIAN_POINT ( 'NONE',  ( 51.92050145378936321, 200.7833772461660828, -9.188101187500095079 ) ) ;
#36030=CARTESIAN_POINT ( 'NONE',  ( 170.7953178271928039, 255.2457615276028093, -12.92277808742838374 ) ) ;
#36031=CARTESIAN_POINT ( 'NONE',  ( 157.7733463334721478, 257.3755434007023268, -16.94489513499352995 ) ) ;
#36032=CARTESIAN_POINT ( 'NONE',  ( 192.1286794796571940, 293.2256832552722017, -14.46936029153980918 ) ) ;
#36033=CARTESIAN_POINT ( 'NONE',  ( 150.0733278132864541, 276.4838168200450355, 3.709811967872132410 ) ) ;
#36034=CARTESIAN_POINT ( 'NONE',  ( 167.4857222457644070, 256.6955868355478287, 13.86207597102780653 ) ) ;
#36035=CARTESIAN_POINT ( 'NONE',  ( 65.38900070045460211, 221.8927522451419350, 2.944929066748280225E-16 ) ) ;
#36037=CARTESIAN_POINT ( 'NONE',  ( 198.7255181831150423, 286.4443010768291629, 17.42756903872921725 ) ) ;
#36038=CARTESIAN_POINT ( 'NONE',  ( 49.89075441544353851, 199.6115022471902591, 10.00000000000009592 ) ) ;
#36039=CARTESIAN_POINT ( 'NONE',  ( 181.8203573988056121, 291.6320214270799625, 9.291447165319489443 ) ) ;
#36040=CARTESIAN_POINT ( 'NONE',  ( 163.3706531435203146, 247.6807236201477735, 10.06957846017757241 ) ) ;
#36041=CARTESIAN_POINT ( 'NONE',  ( 18.76822678699008051, 172.4548013555409796, -4.594050593750042211 ) ) ;
#36042=CARTESIAN_POINT ( 'NONE',  ( 167.9632374571382343, 286.8488433775840463, 5.051339247087953233 ) ) ;
#36043=CARTESIAN_POINT ( 'NONE',  ( 3.558395312976033065, 182.8615022471903444, 5.000000000000046185 ) ) ;
#36046=CARTESIAN_POINT ( 'NONE',  ( 164.9586510554008782, 244.9302305544571823, -1.717556444319656039 ) ) ;
#36048=CARTESIAN_POINT ( 'NONE',  ( 153.2765620691255322, 265.6467114966280860, -16.15333212972641519 ) ) ;
#36049=CARTESIAN_POINT ( 'NONE',  ( 178.5819917554228482, 262.0706330385751812, -12.89024234665558488 ) ) ;
#36055=EDGE_CURVE ( 'NONE', #59501, #83319, #93879, .T. ) ;
#36056=CARTESIAN_POINT ( 'NONE',  ( 155.0929244053699847, 262.0181703658971628, 18.51426604808664678 ) ) ;
#36059=CARTESIAN_POINT ( 'NONE',  ( 156.7566617110267941, 276.4792909723148568, 10.26919381664546194 ) ) ;
#36060=B_SPLINE_CURVE_WITH_KNOTS ( 'NONE', 3,
 ( #66989, #35603, #51810, #89368, #4199, #73617, #43691, #82752, #75118, #36086, #81745, #12318, #74631, #42686, #74124, #19922, #66007, #28490, #43181, #96958, #59371, #27523, #50795, #89845, #66501, #97427, #58876, #6193, #20419, #90850, #83227, #27997, #13319, #90348, #51286, #20927, #5694, #29493, #36584, #67489, #98419, #29012, #59883, #21403, #52286, #13793, #44672, #75605, #37088, #67992 ),
 .UNSPECIFIED., .F., .F.,
 ( 4, 2, 2, 2, 2, 2, 2, 2, 2, 2, 2, 2, 2, 2, 2, 2, 2, 2, 2, 2, 2, 2, 2, 2, 4 ),
 ( 0.0004617987126954396912, 0.0009154468224893198055, 0.001142270877386221753, 0.001369094932283123917, 0.001482506959731604273, 0.001595918987180085062, 0.001709331014628565418, 0.001822743042077045773, 0.002276391151870667522, 0.003183687371458009466, 0.004090983591045351843, 0.004998279810632693353, 0.005451927920426320739, 0.005678751975323090631, 0.005792164002771485118, 0.005848870016495731801, 0.005905576030219976749, 0.005962282043944223432, 0.006018988057668470115, 0.006132400085116827305, 0.006359224140013545155, 0.006812872249806967845, 0.007266520359600390534, 0.007493344414497106649, 0.007720168469393822765 ),
 .UNSPECIFIED. ) ;
#36061=B_SPLINE_CURVE_WITH_KNOTS ( 'NONE', 3,
 ( #90393, #74168, #76163, #37617 ),
 .UNSPECIFIED., .F., .F.,
 ( 4, 4 ),
 ( 1.255848744284461856E-16, 0.002095492171155140856 ),
 .UNSPECIFIED. ) ;
#36063=ADVANCED_FACE ( 'NONE', ( #9101 ), #70908, .F. ) ;
#36064=VERTEX_POINT ( 'NONE', #40483 ) ;
#36066=CARTESIAN_POINT ( 'NONE',  ( 81.40501017803065054, 206.2592609112379876, 2.679491924311254714 ) ) ;
#36068=CARTESIAN_POINT ( 'NONE',  ( 155.6569868912636991, 261.0411854816857158, -17.75433477650897984 ) ) ;
#36069=ORIENTED_EDGE ( 'NONE', *, *, #28692, .T. ) ;
#36070=ORIENTED_EDGE ( 'NONE', *, *, #60429, .F. ) ;
#36071=CARTESIAN_POINT ( 'NONE',  ( 159.5819137999480120, 278.9358841718408257, -9.468475011818437537 ) ) ;
#36072=CARTESIAN_POINT ( 'NONE',  ( 204.3574891606595827, 276.6894411969685166, 13.41627538812899978 ) ) ;
#36073=CARTESIAN_POINT ( 'NONE',  ( 153.3127735718713609, 265.1014820546527631, 17.57722645152040641 ) ) ;
#36074=ORIENTED_EDGE ( 'NONE', *, *, #97454, .T. ) ;
#36077=CARTESIAN_POINT ( 'NONE',  ( 174.3461956351267474, 262.5478167486214716, 14.75061405228954747 ) ) ;
#36079=ADVANCED_FACE ( 'NONE', ( #2003 ), #32889, .T. ) ;
#36081=ORIENTED_EDGE ( 'NONE', *, *, #54687, .F. ) ;
#36082=CARTESIAN_POINT ( 'NONE',  ( 205.8452707775803390, 274.1125278458945900, 11.42742867493066328 ) ) ;
#36085=CARTESIAN_POINT ( 'NONE',  ( 177.7120326079455594, 279.3125840650498617, -16.15421593783462484 ) ) ;
#36086=CARTESIAN_POINT ( 'NONE',  ( 168.9473062510006116, 261.3660218479304831, -16.26153824055670327 ) ) ;
#36087=VECTOR ( 'NONE', #58573, 1000.000000000000000 ) ;
#36091=CARTESIAN_POINT ( 'NONE',  ( 192.4212750754384160, 297.3635704425909125, -12.73704185013552248 ) ) ;
#36093=CARTESIAN_POINT ( 'NONE',  ( 157.6602107013036402, 268.8732101254922213, 15.63420833100257212 ) ) ;
#36095=CARTESIAN_POINT ( 'NONE',  ( 156.2392164662131790, 267.4395022997947535, -16.72994906840104790 ) ) ;
#36096=CARTESIAN_POINT ( 'NONE',  ( 146.9324727656309335, 276.1524872186338371, 3.813717745456558728 ) ) ;
#36097=CARTESIAN_POINT ( 'NONE',  ( 188.6207918642060406, 298.5847884678960895, -4.298219847241822933 ) ) ;
#36099=CARTESIAN_POINT ( 'NONE',  ( 153.1314981037513121, 265.4154603756023789, 17.73969815997475408 ) ) ;
#36100=CARTESIAN_POINT ( 'NONE',  ( 31.19903945042937465, 195.4865022471903160, 10.00000000000009415 ) ) ;
#36101=CARTESIAN_POINT ( 'NONE',  ( 146.8859094598974480, 276.2331372299326517, -0.7994986043261681496 ) ) ;
#36102=ORIENTED_EDGE ( 'NONE', *, *, #28240, .F. ) ;
#36104=CARTESIAN_POINT ( 'NONE',  ( 149.1486417047969155, 272.3139700178423368, -11.47583619705022606 ) ) ;
#36105=CARTESIAN_POINT ( 'NONE',  ( 206.1215120922853146, 273.6340638536760821, 10.12238414215620885 ) ) ;
#36106=CARTESIAN_POINT ( 'NONE',  ( 198.4334039703542771, 286.9502577349437615, 18.47706603442866680 ) ) ;
#36107=ORIENTED_EDGE ( 'NONE', *, *, #16674, .F. ) ;
#36108=CARTESIAN_POINT ( 'NONE',  ( 167.9901196014850484, 286.8200544026590251, 3.506790081298479134 ) ) ;
#36109=CARTESIAN_POINT ( 'NONE',  ( 177.2041192817024182, 288.9686198354513635, -9.145765595030599826 ) ) ;
#36110=ORIENTED_EDGE ( 'NONE', *, *, #87057, .F. ) ;
#36115=CARTESIAN_POINT ( 'NONE',  ( 199.3683090308842907, 285.3309546698520762, -17.40861982076147285 ) ) ;
#36117=ORIENTED_EDGE ( 'NONE', *, *, #7089, .F. ) ;
#36118=CARTESIAN_POINT ( 'NONE',  ( 169.6774685567663710, 254.9819702002519932, -11.65141391084731026 ) ) ;
#36121=CARTESIAN_POINT ( 'NONE',  ( 200.8251833487811666, 282.8075743310126882, -16.74393672780000131 ) ) ;
#36122=CARTESIAN_POINT ( 'NONE',  ( 206.9408877595175511, 272.2148635675444552, 6.707071080545934372 ) ) ;
#36123=CARTESIAN_POINT ( 'NONE',  ( 30.24280306353617576, 188.2677522451418497, 10.00000000000009592 ) ) ;
#36124=CARTESIAN_POINT ( 'NONE',  ( 126.3990332750161087, 231.5327760586659736, 1.948934522072302763E-15 ) ) ;
#36125=CARTESIAN_POINT ( 'NONE',  ( 180.8688118873734254, 294.1367794693202313, -2.657154044881775867 ) ) ;
#36127=CARTESIAN_POINT ( 'NONE',  ( 167.8634577855056875, 282.1373012281606520, -10.74177425913053163 ) ) ;
#36128=CARTESIAN_POINT ( 'NONE',  ( 100.5532405368332007, 228.8615022471902591, -10.00000000000009592 ) ) ;
#36129=CARTESIAN_POINT ( 'NONE',  ( 162.4993287900620942, 249.1899016702093661, 10.54298717179175071 ) ) ;
#36130=CARTESIAN_POINT ( 'NONE',  ( 45.85867072306329817, 185.0327760586659451, 1.948934522072303157E-15 ) ) ;
#36135=CARTESIAN_POINT ( 'NONE',  ( 178.0914043118813765, 265.4878125568229166, 15.91409428133586168 ) ) ;
#36138=CARTESIAN_POINT ( 'NONE',  ( 146.8516045228164160, 276.2925551239072774, 3.995954059407343273 ) ) ;
#36141=CARTESIAN_POINT ( 'NONE',  ( 179.2274323333295740, 287.9912526978436063, -12.78748593997733352 ) ) ;
#36142=CARTESIAN_POINT ( 'NONE',  ( 164.1808077535702921, 250.0262784942443091, 10.25442190752840865 ) ) ;
#36143=CARTESIAN_POINT ( 'NONE',  ( 91.29759403033908427, 223.5177522451418781, -10.00000000000009592 ) ) ;
#36144=B_SPLINE_CURVE_WITH_KNOTS ( 'NONE', 3,
 ( #66928, #20860, #11276, #13259, #44119, #36526, #42137, #73068, #3666, #34544, #44613, #6643, #30928, #37518, #61319, #45614, #99351, #46618, #60806, #84670, #15212, #91766, #21833, #7627, #22331, #53230, #90790, #38518, #84182, #44, #54205, #85173, #15717, #39012, #77548, #69918, #6133, #52226, #28947, #59825, #52718, #21342, #83171, #37030, #67938, #47121, #2548, #48125, #47619, #9134 ),
 .UNSPECIFIED., .F., .F.,
 ( 4, 2, 2, 2, 2, 2, 2, 2, 2, 2, 2, 2, 2, 2, 2, 2, 2, 2, 2, 2, 2, 2, 2, 2, 4 ),
 ( 0.0004837326417408448816, 0.001489169143744289948, 0.001991887394746087725, 0.002117566957496566822, 0.002243246520247045919, 0.002368926082997524583, 0.002494605645748003246, 0.002745964771248944961, 0.002997323896749886675, 0.003500042147751701582, 0.004505478649755411194, 0.005510915151759121673, 0.006013633402760975612, 0.006264992528261860948, 0.006516351653762746284, 0.006579191435137916877, 0.006642031216513087470, 0.006704870997888258931, 0.006767710779263429524, 0.007019069904763931486, 0.007521788155764807908, 0.007773147281265280380, 0.008024506406765751984, 0.008275865532266224456, 0.008527224657766695193 ),
 .UNSPECIFIED. ) ;
#36146=CARTESIAN_POINT ( 'NONE',  ( 196.0351912666876615, 267.0317724427966368, -7.782412515619550497 ) ) ;
#36147=CARTESIAN_POINT ( 'NONE',  ( 155.4523213358487794, 279.7030401036391254, -1.715928067515927413 ) ) ;
#36148=CARTESIAN_POINT ( 'NONE',  ( 162.6757594134126350, 248.8843148665554281, -10.86406770146305867 ) ) ;
#36150=CARTESIAN_POINT ( 'NONE',  ( 13.46382118881039602, 169.3923013555410080, 4.594050593750050204 ) ) ;
#36155=CARTESIAN_POINT ( 'NONE',  ( 48.80796233711527776, 208.1744531367911293, 4.594050593750047540 ) ) ;
#36156=CARTESIAN_POINT ( 'NONE',  ( 196.1985894344492465, 280.6689076705129651, 17.57724957243723551 ) ) ;
#36157=CARTESIAN_POINT ( 'NONE',  ( 204.9780665305064531, 275.6145696623662502, 14.10615427165218883 ) ) ;
#36158=CARTESIAN_POINT ( 'NONE',  ( 186.2798660816079632, 264.0713031700501006, -12.82791401631097550 ) ) ;
#36161=CARTESIAN_POINT ( 'NONE',  ( 17.41480177352709191, 180.8615022471902591, -10.00000000000009592 ) ) ;
#36164=CARTESIAN_POINT ( 'NONE',  ( 127.8056303646358032, 256.8464784336661637, 1.353441290958777327E-15 ) ) ;
#36166=CARTESIAN_POINT ( 'NONE',  ( 164.8719015746727621, 245.0804850626086022, 0.9827678719136201391 ) ) ;
#36167=DIRECTION ( 'NONE',  ( -0.8660254037844387076, -0.4999999999999998890, -0.000000000000000000 ) ) ;
#36170=CARTESIAN_POINT ( 'NONE',  ( 196.4982648257524147, 290.3020170531091821, 16.69353242256149628 ) ) ;
#36174=CARTESIAN_POINT ( 'NONE',  ( 191.0816511748900268, 299.6838671013740623, 7.311127128005925790 ) ) ;
#36175=CARTESIAN_POINT ( 'NONE',  ( 207.6937983729889368, 270.9107841314541929, -1.514855854672175761 ) ) ;
#36177=CARTESIAN_POINT ( 'NONE',  ( 172.9630369837942965, 268.1244351977575207, -16.30034978024972858 ) ) ;
#36178=CARTESIAN_POINT ( 'NONE',  ( 195.4726663938093054, 272.0961244453007453, -13.40964562940238913 ) ) ;
#36183=CYLINDRICAL_SURFACE ( 'NONE', #35843, 10.00000000000010658 ) ;
#36184=CARTESIAN_POINT ( 'NONE',  ( 182.0881301589248551, 295.0157003455848894, 4.784192560878642198 ) ) ;
#36185=CARTESIAN_POINT ( 'NONE',  ( 163.0424334805279045, 248.2492167524936804, -9.671494865076915914 ) ) ;
#36192=CARTESIAN_POINT ( 'NONE',  ( 164.2981700896163773, 253.9203781951923133, 14.63367134977796802 ) ) ;
#36194=CARTESIAN_POINT ( 'NONE',  ( 156.1569981892633621, 261.6699882273320554, -17.05379912710613510 ) ) ;
#36195=VERTEX_POINT ( 'NONE', #11122 ) ;
#36197=CARTESIAN_POINT ( 'NONE',  ( 147.3047606266276546, 275.5076657283461827, -0.02269072295920609994 ) ) ;
#36198=CARTESIAN_POINT ( 'NONE',  ( 185.1256672880319911, 291.5517695480672842, 11.95305935706613276 ) ) ;
#36199=CARTESIAN_POINT ( 'NONE',  ( 204.7235752877335244, 276.0553614249301972, 14.82397698933823271 ) ) ;
#36201=CARTESIAN_POINT ( 'NONE',  ( 189.5698839646237843, 268.9756110371309887, -14.78084782106435391 ) ) ;
#36203=CARTESIAN_POINT ( 'NONE',  ( 92.94880205384217220, 212.2202760586659167, -5.415160957724236172E-17 ) ) ;
#36204=CARTESIAN_POINT ( 'NONE',  ( 155.4641461872872981, 261.3751953787398179, 17.01821821352853092 ) ) ;
#36206=CARTESIAN_POINT ( 'NONE',  ( 181.2844587369501141, 271.1666661326591452, -15.98216304377438490 ) ) ;
#36207=CARTESIAN_POINT ( 'NONE',  ( 185.6377146029830385, 259.0204853581686280, -6.791722753532964951 ) ) ;
#36211=B_SPLINE_CURVE_WITH_KNOTS ( 'NONE', 3,
 ( #63612, #71237, #16512, #94058 ),
 .UNSPECIFIED., .F., .F.,
 ( 4, 4 ),
 ( 0.03345425586890212605, 0.04234520293996446583 ),
 .UNSPECIFIED. ) ;
#36212=CARTESIAN_POINT ( 'NONE',  ( -3.965200385949115169, 158.5177522451418213, 5.000000000000051514 ) ) ;
#36214=EDGE_LOOP ( 'NONE', ( #25008, #22123, #56999, #91439 ) ) ;
#36218=CARTESIAN_POINT ( 'NONE',  ( 155.3716771045260714, 261.5353565282119348, -18.54934131471355840 ) ) ;
#36220=CARTESIAN_POINT ( 'NONE',  ( 182.9620665166839899, 279.7200058654210579, -17.04853919723895572 ) ) ;
#36222=CARTESIAN_POINT ( 'NONE',  ( 201.0356089830534643, 282.4431064412383989, -18.18835788025466371 ) ) ;
#36225=CARTESIAN_POINT ( 'NONE',  ( 166.1354066105388654, 265.9557281117362209, -16.63352449353996576 ) ) ;
#36230=CARTESIAN_POINT ( 'NONE',  ( 167.4082149272132085, 284.2775854637627049, 9.280720086700116056 ) ) ;
#36231=CARTESIAN_POINT ( 'NONE',  ( 201.1438721331022350, 270.7680306690247676, 9.304748580235882471 ) ) ;
#36232=EDGE_LOOP ( 'NONE', ( #69268, #100182, #52508, #72395, #16543 ) ) ;
#36234=DIRECTION ( 'NONE',  ( 0.8660254037844387076, 0.4999999999999998890, 0.000000000000000000 ) ) ;
#36236=CARTESIAN_POINT ( 'NONE',  ( 161.1037025896568764, 281.9537687873744289, -6.124960680995634732 ) ) ;
#36237=CARTESIAN_POINT ( 'NONE',  ( 177.3334602733804104, 257.8359255682534581, -11.87082999068797484 ) ) ;
#36238=CARTESIAN_POINT ( 'NONE',  ( 157.7111038903397571, 257.9445160749222055, 16.71092927711721998 ) ) ;
#36243=CARTESIAN_POINT ( 'NONE',  ( 181.8129903383622263, 270.5352787916219199, -16.24512204374439861 ) ) ;
#36247=CARTESIAN_POINT ( 'NONE',  ( 193.1030321335636586, 294.1827325794992021, -14.54662778306917481 ) ) ;
#36248=AXIS2_PLACEMENT_3D ( 'NONE', #64631, #9423, #64118 ) ;
#36250=CARTESIAN_POINT ( 'NONE',  ( 193.5354321533228301, 263.1006045986919730, 5.857068979672426678 ) ) ;
#36253=CARTESIAN_POINT ( 'NONE',  ( 160.8894027367712454, 272.6494381571178565, 15.39890601372860957 ) ) ;
#36254=CARTESIAN_POINT ( 'NONE',  ( -0.9067010812963882671, 158.0327760586659451, 1.948934522072303157E-15 ) ) ;
#36256=CARTESIAN_POINT ( 'NONE',  ( 189.0443830094626207, 297.0343580855736150, 8.140033191741938623 ) ) ;
#36259=B_SPLINE_SURFACE_WITH_KNOTS ( 'NONE', 3, 1, ( 
 ( #40562, #63379 ),
 ( #10190, #17793 ),
 ( #96316, #81129 ),
 ( #94318, #80125 ),
 ( #41056, #26387 ),
 ( #10687, #71498 ),
 ( #71992, #88240 ),
 ( #19311, #2598 ),
 ( #42073, #26884 ),
 ( #3117, #17274 ),
 ( #88739, #41566 ),
 ( #50176, #73006 ),
 ( #80628, #2092 ),
 ( #70997, #33483 ),
 ( #79122, #34476 ),
 ( #3595, #18791 ),
 ( #95343, #87259 ),
 ( #25900, #72509 ),
 ( #25375, #56773 ),
 ( #24873, #11203 ),
 ( #1600, #32969 ),
 ( #49671, #57763 ),
 ( #65374, #32484 ),
 ( #63877, #11696 ),
 ( #55746, #94813 ),
 ( #87754, #56266 ),
 ( #79627, #34003 ),
 ( #64888, #57265 ),
 ( #22140, #22640 ),
 ( #6930, #36837 ),
 ( #29739, #29251 ),
 ( #44922, #12184 ),
 ( #42555, #21647 ),
 ( #60119, #73489 ) ),
 .UNSPECIFIED., .T., .F., .F.,
 ( 4, 2, 2, 2, 2, 2, 2, 2, 2, 2, 2, 2, 2, 2, 2, 2, 4 ),
 ( 2, 2 ),
 ( 0.000000000000000000, 0.06250000000000000000, 0.1250000000000000000, 0.1875000000000000000, 0.2500000000000000000, 0.3125000000000000000, 0.3750000000000000000, 0.4375000000000000000, 0.5000000000000000000, 0.5625000000000000000, 0.6250000000000000000, 0.6875000000000000000, 0.7500000000000000000, 0.8125000000000000000, 0.8750000000000000000, 0.9375000000000000000, 1.000000000000000000 ),
 ( 0.000000000000000000, 1.000000000000000000 ),
 .UNSPECIFIED. ) ;
#36260=B_SPLINE_CURVE_WITH_KNOTS ( 'NONE', 3,
 ( #34526, #80174, #73051, #81664 ),
 .UNSPECIFIED., .F., .F.,
 ( 4, 4 ),
 ( 0.006461935089719096983, 0.01455589064683252346 ),
 .UNSPECIFIED. ) ;
#36263=CARTESIAN_POINT ( 'NONE',  ( 189.8274365450016319, 274.1967410140837274, -15.63878423788518290 ) ) ;
#36266=CARTESIAN_POINT ( 'NONE',  ( 175.3208435976894179, 291.5367879113061917, 3.470880399820767348 ) ) ;
#36267=CARTESIAN_POINT ( 'NONE',  ( 133.4825598088814047, 236.3262482093457493, 3.021315404115420679E-15 ) ) ;
#36270=CARTESIAN_POINT ( 'NONE',  ( 156.6812872898450735, 261.2670451491295012, 0.000000000000000000 ) ) ;
#36271=CARTESIAN_POINT ( 'NONE',  ( 3.585285057187872937, 179.0024278399160949, 9.188101187500095079 ) ) ;
#36272=CARTESIAN_POINT ( 'NONE',  ( 96.30395630197683943, 238.6589784336661637, -6.496448406907675876E-16 ) ) ;
#36273=CARTESIAN_POINT ( 'NONE',  ( 41.86197723097736656, 201.6427522451419350, -10.00000000000009592 ) ) ;
#36274=CARTESIAN_POINT ( 'NONE',  ( 186.7353386538602251, 295.9631457000137402, -7.534418545603307038 ) ) ;
#36279=CARTESIAN_POINT ( 'NONE',  ( 180.5329152982068877, 273.0640148049105278, 16.87540567491608101 ) ) ;
#36280=CARTESIAN_POINT ( 'NONE',  ( 194.7900911235093133, 293.2606606935473792, -14.66228443412922999 ) ) ;
#36283=CARTESIAN_POINT ( 'NONE',  ( 192.8548134607404165, 265.3588860054690031, 7.786932206011543123 ) ) ;
#36285=CARTESIAN_POINT ( 'NONE',  ( 184.4700260883318492, 268.6843530457092015, -15.41494737780146629 ) ) ;
#36286=CARTESIAN_POINT ( 'NONE',  ( 42.89584289395545369, 207.1199935810940929, 2.679491924311251605 ) ) ;
#36287=CARTESIAN_POINT ( 'NONE',  ( 172.5927298621351156, 263.8025790245163194, -15.44835621726458008 ) ) ;
#36289=CARTESIAN_POINT ( 'NONE',  ( 74.35571174875622091, 222.9244531367911293, -4.594050593750046652 ) ) ;
#36291=CYLINDRICAL_SURFACE ( 'NONE', #54660, 17.82106496071139645 ) ;
#36292=CARTESIAN_POINT ( 'NONE',  ( 157.4656258344471098, 257.9085309395441641, 18.30485740784190796 ) ) ;
#36293=CARTESIAN_POINT ( 'NONE',  ( 152.5098501883502706, 266.4921861494963196, 16.07965188502810605 ) ) ;
#36294=CARTESIAN_POINT ( 'NONE',  ( 196.9367784295097579, 289.5424892115916577, 16.51204079746186437 ) ) ;
#36295=CARTESIAN_POINT ( 'NONE',  ( 151.2646864780760723, 268.6488729594320830, -14.38346604407754548 ) ) ;
#36298=CARTESIAN_POINT ( 'NONE',  ( 192.4743214706506365, 297.2716913909250707, -12.17804856100553046 ) ) ;
#36302=CARTESIAN_POINT ( 'NONE',  ( 147.3379027498079381, 275.4502618871274535, -3.695260257281167249 ) ) ;
#36303=CARTESIAN_POINT ( 'NONE',  ( 191.6794403243964950, 288.1292005957208744, -15.80774595056399434 ) ) ;
#36306=CARTESIAN_POINT ( 'NONE',  ( 159.9307118030769175, 253.6388767968520881, 16.60600887889890487 ) ) ;
#36307=MECHANICAL_DESIGN_GEOMETRIC_PRESENTATION_REPRESENTATION('',(#23353),#799);
#36308=CARTESIAN_POINT ( 'NONE',  ( 153.6507061805664307, 266.9580362223465499, 16.55103579890343113 ) ) ;
#36309=CARTESIAN_POINT ( 'NONE',  ( 169.9051147537142299, 251.0516595293013040, -8.602792619013742481 ) ) ;
#36310=CARTESIAN_POINT ( 'NONE',  ( 149.8445197688975838, 243.9865022471901455, 1.119607411625061291E-15 ) ) ;
#36312=EDGE_LOOP ( 'NONE', ( #92551, #43604, #38174, #89485 ) ) ;
#36313=CARTESIAN_POINT ( 'NONE',  ( 193.0622221429366050, 289.4054684591471300, 16.71589558189321778 ) ) ;
#36315=CARTESIAN_POINT ( 'NONE',  ( 196.6281177133425899, 264.5552008573027933, -4.675636469121769778 ) ) ;
#36318=CARTESIAN_POINT ( 'NONE',  ( 185.3004367499268596, 292.5792462585945373, -10.68249092389169519 ) ) ;
#36322=CARTESIAN_POINT ( 'NONE',  ( 188.7930588916510999, 290.9633865388665299, 14.97457979531618832 ) ) ;
#36324=CARTESIAN_POINT ( 'NONE',  ( 157.5695214119805598, 258.1165995213424367, -16.71692661953962400 ) ) ;
#36325=CARTESIAN_POINT ( 'NONE',  ( 204.3267329952771831, 273.2094209704910099, 10.93732012634468909 ) ) ;
#36326=CARTESIAN_POINT ( 'NONE',  ( 153.1983976505312626, 265.2995869615763809, -17.69657798691567763 ) ) ;
#36335=ORIENTED_EDGE ( 'NONE', *, *, #45931, .F. ) ;
#36337=CARTESIAN_POINT ( 'NONE',  ( 164.3853877993040840, 245.9231516401292197, 5.995325337583643943 ) ) ;
#36338=CARTESIAN_POINT ( 'NONE',  ( 194.2154056360670040, 294.2560451561701029, -15.66696967429384557 ) ) ;
#36339=CARTESIAN_POINT ( 'NONE',  ( -22.42236680055709641, 157.8615022471902591, 0.000000000000000000 ) ) ;
#36340=CARTESIAN_POINT ( 'NONE',  ( 155.0929244053699847, 262.0181703658971628, 18.51426604808664678 ) ) ;
#36342=CARTESIAN_POINT ( 'NONE',  ( 148.2980785574368952, 273.7871886041155562, 9.134436720559454770 ) ) ;
#36343=CARTESIAN_POINT ( 'NONE',  ( 168.7909529993691251, 286.6037707115942226, -4.663693738437698855 ) ) ;
#36345=CARTESIAN_POINT ( 'NONE',  ( 181.9115977867584775, 256.5621209711902679, 5.178624687905984736 ) ) ;
#36346=CARTESIAN_POINT ( 'NONE',  ( 105.9931361504627603, 225.8768266524159856, -9.188101187500091527 ) ) ;
#36347=ORIENTED_EDGE ( 'NONE', *, *, #13609, .T. ) ;
#36349=CARTESIAN_POINT ( 'NONE',  ( 165.2491185908025102, 271.0061427863645349, 16.55936586366629015 ) ) ;
#36350=CARTESIAN_POINT ( 'NONE',  ( 191.9323033642516805, 275.2179287646682724, 16.63116605495289946 ) ) ;
#36352=ORIENTED_EDGE ( 'NONE', *, *, #48776, .F. ) ;
#36353=CARTESIAN_POINT ( 'NONE',  ( 180.1168005803277481, 295.2192856762299016, -2.191971455912026467 ) ) ;
#36354=CARTESIAN_POINT ( 'NONE',  ( 177.4877928417686803, 293.5951873982637608, -2.837372163671336267 ) ) ;
#36355=CARTESIAN_POINT ( 'NONE',  ( 157.1338510812060747, 258.4831816688264325, 17.88958125218800888 ) ) ;
#36356=CARTESIAN_POINT ( 'NONE',  ( 159.9470087484377814, 253.6106496594791508, -16.54933891566789939 ) ) ;
#36360=EDGE_CURVE ( 'NONE', #76328, #77324, #67276, .T. ) ;
#36361=CARTESIAN_POINT ( 'NONE',  ( 163.4218292706009095, 247.5920839679097014, -10.44611490715852042 ) ) ;
#36364=CARTESIAN_POINT ( 'NONE',  ( 101.7620676594010973, 222.8927522451417929, -10.00000000000009237 ) ) ;
#36365=CARTESIAN_POINT ( 'NONE',  ( 191.8812340238766581, 261.0126994209120426, -0.1972034713832918895 ) ) ;
#36366=CARTESIAN_POINT ( 'NONE',  ( 184.3049839938290972, 288.8408771957522276, -13.19264464187155639 ) ) ;
#36370=CARTESIAN_POINT ( 'NONE',  ( 205.0418338828961851, 275.5041213681629984, 14.30558627745945266 ) ) ;
#36374=CARTESIAN_POINT ( 'NONE',  ( 173.2783483489837408, 251.6438032808846970, -0.4401592383492047289 ) ) ;
#36380=CARTESIAN_POINT ( 'NONE',  ( 180.8044385370616567, 286.7361374272969101, 14.76499878110572439 ) ) ;
#36381=CARTESIAN_POINT ( 'NONE',  ( 206.4097941777342839, 271.6911524580777382, 7.546727351666162598 ) ) ;
#36382=CARTESIAN_POINT ( 'NONE',  ( 62.93552237999645627, 197.9548013555410080, -4.594050593750042211 ) ) ;
#36383=CARTESIAN_POINT ( 'NONE',  ( 206.0946696452135427, 273.6805563358039421, -10.19627505985792837 ) ) ;
#36385=FACE_OUTER_BOUND ( 'NONE', #67015, .T. ) ;
#36387=EDGE_CURVE ( 'NONE', #13192, #84442, #72153, .T. ) ;
#36388=CARTESIAN_POINT ( 'NONE',  ( 161.3145230519951951, 251.2420454056404822, -14.44869077440025151 ) ) ;
#36392=CARTESIAN_POINT ( 'NONE',  ( 160.7489855951974675, 254.2215850144021658, 15.85577744295692248 ) ) ;
#36395=CARTESIAN_POINT ( 'NONE',  ( 180.2261984326610218, 279.1782745765357276, -17.42438828499370729 ) ) ;
#36397=CARTESIAN_POINT ( 'NONE',  ( 26.96797095936772237, 192.5024278399160949, 9.188101187500095079 ) ) ;
#36399=CARTESIAN_POINT ( 'NONE',  ( 196.1573359623355088, 290.8925231663144473, 17.55680092534192482 ) ) ;
#36400=CARTESIAN_POINT ( 'NONE',  ( 166.1309782654906257, 249.2029336093187339, -9.347746458946922132 ) ) ;
#36401=CARTESIAN_POINT ( 'NONE',  ( 207.6172352878830907, 271.0433952848413810, 3.316653249540578496 ) ) ;
#36403=CARTESIAN_POINT ( 'NONE',  ( 51.08127902204942927, 209.4869531367911009, 4.594050593750046652 ) ) ;
#36404=B_SPLINE_CURVE_WITH_KNOTS ( 'NONE', 3,
 ( #90516, #52449, #75279, #13963, #55301, #98587 ),
 .UNSPECIFIED., .F., .F.,
 ( 4, 2, 4 ),
 ( 0.01937495045225347615, 0.02390856016151878677, 0.02844216987078409392 ),
 .UNSPECIFIED. ) ;
#36407=CARTESIAN_POINT ( 'NONE',  ( 199.1526122334580862, 285.7045524820243259, -17.32174362185583050 ) ) ;
#36410=CARTESIAN_POINT ( 'NONE',  ( 202.9861313035285377, 270.0111324708095708, -7.109816141738001249 ) ) ;
#36412=CARTESIAN_POINT ( 'NONE',  ( 179.8822850121538863, 276.6405008247433557, 16.37156656675600885 ) ) ;
#36413=CARTESIAN_POINT ( 'NONE',  ( 158.2129804214947058, 265.2348010298870236, 17.61986633405762603 ) ) ;
#36415=CARTESIAN_POINT ( 'NONE',  ( 192.6633363462123043, 266.5854721252571267, 11.55478091722345901 ) ) ;
#36418=CARTESIAN_POINT ( 'NONE',  ( 107.0484310652165476, 222.6115022471901739, -5.000000000000041744 ) ) ;
#36419=CARTESIAN_POINT ( 'NONE',  ( 179.4404154152157105, 291.3709498135804097, -10.08759257512885199 ) ) ;
#36420=CARTESIAN_POINT ( 'NONE',  ( 164.0800018754982261, 268.9966071389823696, -16.36617084150674728 ) ) ;
#36422=CARTESIAN_POINT ( 'NONE',  ( 65.10058588945754821, 199.2048013555409796, 4.594050593750051981 ) ) ;
#36424=CARTESIAN_POINT ( 'NONE',  ( 165.2047206435933902, 264.8326349929704406, 16.61084491559804732 ) ) ;
#36425=CARTESIAN_POINT ( 'NONE',  ( 190.1813752874636805, 301.2431906792259042, -4.710625539811892359 ) ) ;
#36426=B_SPLINE_CURVE_WITH_KNOTS ( 'NONE', 3,
 ( #96881, #12756, #42127, #73059 ),
 .UNSPECIFIED., .F., .F.,
 ( 4, 4 ),
 ( 0.009399112305859652974, 0.01497842902758104652 ),
 .UNSPECIFIED. ) ;
#36427=LINE ( 'NONE', #7527, #30480 ) ;
#36428=VERTEX_POINT ( 'NONE', #40360 ) ;
#36432=CARTESIAN_POINT ( 'NONE',  ( 187.7918093292738604, 264.8259943713989060, 10.76435498059212925 ) ) ;
#36434=CARTESIAN_POINT ( 'NONE',  ( 205.0418338828961851, 275.5041213681629984, 14.30558627745945266 ) ) ;
#36439=CARTESIAN_POINT ( 'NONE',  ( 172.2467550100553808, 258.4300157609564508, -14.58559033337875377 ) ) ;
#36440=B_SPLINE_CURVE_WITH_KNOTS ( 'NONE', 3,
 ( #71090, #71590, #17885, #62442 ),
 .UNSPECIFIED., .F., .F.,
 ( 4, 4 ),
 ( 0.01214016279898067277, 0.01831897122411682219 ),
 .UNSPECIFIED. ) ;
#36441=ORIENTED_EDGE ( 'NONE', *, *, #7280, .T. ) ;
#36442=CARTESIAN_POINT ( 'NONE',  ( 182.6210901421643769, 283.8088811521847106, 15.95401699950471652 ) ) ;
#36443=EDGE_CURVE ( 'NONE', #19809, #41237, #22607, .T. ) ;
#36444=CARTESIAN_POINT ( 'NONE',  ( 159.4491226731523454, 254.4730136382542582, -15.39140229921534520 ) ) ;
#36446=EDGE_CURVE ( 'NONE', #73023, #40420, #86716, .T. ) ;
#36449=CARTESIAN_POINT ( 'NONE',  ( 159.2440537178480042, 282.4524729739796385, -3.288764571076911114 ) ) ;
#36450=CARTESIAN_POINT ( 'NONE',  ( 165.4187906757635460, 280.8472404715405446, -12.62740765345973415 ) ) ;
#36453=EDGE_CURVE ( 'NONE', #98021, #86016, #26202, .T. ) ;
#36456=CARTESIAN_POINT ( 'NONE',  ( 163.7356037823865336, 264.5711151872889673, -16.68138376633201148 ) ) ;
#36457=EDGE_CURVE ( 'NONE', #36668, #99538, #90219, .T. ) ;
#36459=CARTESIAN_POINT ( 'NONE',  ( 129.7005815790617760, 239.5643266524159856, -9.188101187500093303 ) ) ;
#36462=CARTESIAN_POINT ( 'NONE',  ( 173.7177128658787240, 265.2567829307042757, 16.88771258197816039 ) ) ;
#36463=CARTESIAN_POINT ( 'NONE',  ( 27.19136022205111658, 198.0530062829863311, -4.648177544792955347E-16 ) ) ;
#36468=CARTESIAN_POINT ( 'NONE',  ( 198.6587626159274294, 286.5599251108861267, 17.99840276545888784 ) ) ;
#36470=CARTESIAN_POINT ( 'NONE',  ( 74.76226857436894591, 201.7202760586659167, -5.415160957724236172E-17 ) ) ;
#36473=CARTESIAN_POINT ( 'NONE',  ( 155.3017250444513024, 261.6565170503553190, 18.58368563027307374 ) ) ;
#36476=EDGE_LOOP ( 'NONE', ( #256, #7541, #79033, #42455 ) ) ;
#36478=CARTESIAN_POINT ( 'NONE',  ( 152.7375212135632125, 266.0978483664162582, -16.47968945089317572 ) ) ;
#36481=DIRECTION ( 'NONE',  ( 0.8660254037844395958, 0.4999999999999985567, 0.000000000000000000 ) ) ;
#36483=CARTESIAN_POINT ( 'NONE',  ( 174.7480863157453825, 254.3094501535669849, -7.405053707554171361 ) ) ;
#36486=B_SPLINE_CURVE_WITH_KNOTS ( 'NONE', 3,
 ( #58538, #36237, #28149, #57542 ),
 .UNSPECIFIED., .F., .F.,
 ( 4, 4 ),
 ( 0.009348827086400075120, 0.01504353011265674271 ),
 .UNSPECIFIED. ) ;
#36487=CARTESIAN_POINT ( 'NONE',  ( 205.8452707775803390, 274.1125278458945900, 11.42742867493066328 ) ) ;
#36489=CARTESIAN_POINT ( 'NONE',  ( 167.6278246310154714, 282.5728663012718584, -12.21306354836790220 ) ) ;
#36490=CARTESIAN_POINT ( 'NONE',  ( 194.9948854055928678, 279.4939489864826783, 16.52961264899888150 ) ) ;
#36492=CARTESIAN_POINT ( 'NONE',  ( 2.890834060677622830, 179.1427522451419350, -10.00000000000009592 ) ) ;
#36493=CARTESIAN_POINT ( 'NONE',  ( 139.3076170325891212, 260.4244531367911577, -4.594050593750046652 ) ) ;
#36497=CARTESIAN_POINT ( 'NONE',  ( 155.9594927221938292, 261.9410314534172244, -16.96711934140056499 ) ) ;
#36503=CARTESIAN_POINT ( 'NONE',  ( 182.4344152771883500, 275.0372901602324873, -17.25385560252001937 ) ) ;
#36504=CARTESIAN_POINT ( 'NONE',  ( 167.5910006351356287, 249.2382425172987723, -5.800627538551558438 ) ) ;
#36509=EDGE_CURVE ( 'NONE', #27272, #17277, #167, .T. ) ;
#36510=VECTOR ( 'NONE', #76414, 1000.000000000000000 ) ;
#36511=CARTESIAN_POINT ( 'NONE',  ( 157.5487431480040925, 257.7645675294749594, -18.29554785922338311 ) ) ;
#36512=CARTESIAN_POINT ( 'NONE',  ( 172.3986314675530309, 263.7922717222033384, -16.89442142407995107 ) ) ;
#36514=CARTESIAN_POINT ( 'NONE',  ( 48.88270317314112390, 187.4824982072973967, 3.021315404115420679E-15 ) ) ;
#36516=DIRECTION ( 'NONE',  ( -0.8660254037844387076, -0.4999999999999998890, -0.000000000000000000 ) ) ;
#36517=CARTESIAN_POINT ( 'NONE',  ( 159.8655504377736918, 253.7517395922482706, 15.51368179719542262 ) ) ;
#36519=CARTESIAN_POINT ( 'NONE',  ( 128.4645176094212502, 251.6427522451419350, 10.00000000000009237 ) ) ;
#36520=CARTESIAN_POINT ( 'NONE',  ( 175.5561847466084657, 285.0769009925375599, -12.03860467003484835 ) ) ;
#36524=CARTESIAN_POINT ( 'NONE',  ( 198.4860348845112981, 286.8590983175747056, -18.20461732983060088 ) ) ;
#36525=CARTESIAN_POINT ( 'NONE',  ( 8.998290926605621465, 169.8768266524160140, 9.188101187500096856 ) ) ;
#36526=CARTESIAN_POINT ( 'NONE',  ( 178.5956384695835482, 273.7284866639749907, -17.41459860866446263 ) ) ;
#36529=CARTESIAN_POINT ( 'NONE',  ( 157.3029956111992362, 258.1902147490555421, -18.22269824972649843 ) ) ;
#36531=CARTESIAN_POINT ( 'NONE',  ( -22.42236680055709641, 157.8615022471902591, 0.000000000000000000 ) ) ;
#36532=CARTESIAN_POINT ( 'NONE',  ( 196.2686502133740305, 269.5362150063830882, -10.79322297891937588 ) ) ;
#36533=CARTESIAN_POINT ( 'NONE',  ( 78.23504418992386888, 202.6427522451417644, 1.119607411625061291E-15 ) ) ;
#36534=CARTESIAN_POINT ( 'NONE',  ( 179.4307333220020553, 254.8376236813717526, -4.075317600375849558 ) ) ;
#36535=CARTESIAN_POINT ( 'NONE',  ( 197.9723018751917039, 287.7489099912414758, 17.92592712455262571 ) ) ;
#36536=CARTESIAN_POINT ( 'NONE',  ( 59.05618993882887224, 198.2365022471902023, -10.00000000000009059 ) ) ;
#36538=CARTESIAN_POINT ( 'NONE',  ( 189.8147415777049218, 301.8782188922952514, -0.5019643756309712934 ) ) ;
#36539=CARTESIAN_POINT ( 'NONE',  ( 15.06046875309669630, 173.3768266524159856, -9.188101187500091527 ) ) ;
#36540=CARTESIAN_POINT ( 'NONE',  ( 164.2551198995763002, 284.9701055883606386, 4.298724141468182935 ) ) ;
#36541=CARTESIAN_POINT ( 'NONE',  ( 192.1883190596398094, 297.7670620978826150, 12.41391288785556668 ) ) ;
#36543=CARTESIAN_POINT ( 'NONE',  ( 202.0335144746401284, 280.3352735051682885, -15.85562724245423105 ) ) ;
#36544=CARTESIAN_POINT ( 'NONE',  ( 164.2953672501826929, 246.0790718049323687, -2.576662677987826111 ) ) ;
#36545=DIRECTION ( 'NONE',  ( -0.8660254037844359321, -0.5000000000000051070, -0.000000000000000000 ) ) ;
#36547=CARTESIAN_POINT ( 'NONE',  ( 163.9286547936508782, 281.4788881291187863, 8.857336398642782882 ) ) ;
#36550=CARTESIAN_POINT ( 'NONE',  ( 164.9043417134678577, 286.5925546497160212, 0.04530247668140159611 ) ) ;
#36554=CARTESIAN_POINT ( 'NONE',  ( 194.4889937320412230, 293.7821766735966662, 14.99892588346621380 ) ) ;
#36555=ORIENTED_EDGE ( 'NONE', *, *, #93118, .F. ) ;
#36556=CARTESIAN_POINT ( 'NONE',  ( 181.5481620411168819, 289.3862663955354719, 12.74148585560425140 ) ) ;
#36560=( BOUNDED_CURVE ( )  B_SPLINE_CURVE ( 2, ( #75213, #13895, #37673, #90947, #68583, #28096, #60973, #6296, #37187 ),
 .UNSPECIFIED., .F., .T. ) 
 B_SPLINE_CURVE_WITH_KNOTS ( ( 3, 2, 2, 2, 3 ),
 ( 0.2459677419354838745, 0.2473118279569892497, 0.2500000000000000000, 0.2526881720430107503, 0.2540322580645161255 ),
 .UNSPECIFIED. ) 
 CURVE ( )  GEOMETRIC_REPRESENTATION_ITEM ( )  RATIONAL_B_SPLINE_CURVE ( ( 0.9330127018922194093, 0.9330127018922194093, 1.000000000000000000, 0.8660254037844387076, 1.000000000000000000, 0.8660254037844387076, 1.000000000000000000, 0.9330127018922194093, 0.9330127018922194093 ) ) 
 REPRESENTATION_ITEM ( '' )  );
#36561=CARTESIAN_POINT ( 'NONE',  ( 155.6368094659423207, 263.0761338075079721, 17.69820953191020152 ) ) ;
#36564=CARTESIAN_POINT ( 'NONE',  ( 155.3513572141771704, 261.5705516107003064, -17.00592413546589299 ) ) ;
#36565=ORIENTED_EDGE ( 'NONE', *, *, #39754, .F. ) ;
#36567=CARTESIAN_POINT ( 'NONE',  ( -22.42236680055709641, 157.8615022471902591, 0.000000000000000000 ) ) ;
#36568=CARTESIAN_POINT ( 'NONE',  ( 204.8189571845487080, 275.8901551335242175, 13.43702398685204358 ) ) ;
#36569=CARTESIAN_POINT ( 'NONE',  ( 153.3703256797887775, 265.0017988796566897, 16.44314709207578318 ) ) ;
#36574=EDGE_LOOP ( 'NONE', ( #18160, #32019, #18192 ) ) ;
#36579=CARTESIAN_POINT ( 'NONE',  ( 164.6869624841032191, 245.4008089637804346, 1.435659848726088317 ) ) ;
#36582=ORIENTED_EDGE ( 'NONE', *, *, #84624, .T. ) ;
#36583=CARTESIAN_POINT ( 'NONE',  ( 176.2580550267919932, 278.7780497695933946, -16.99066290002705060 ) ) ;
#36584=CARTESIAN_POINT ( 'NONE',  ( 172.3315061660855463, 263.8993054968007641, -15.56597864815643639 ) ) ;
#36585=ORIENTED_EDGE ( 'NONE', *, *, #48483, .F. ) ;
#36586=CYLINDRICAL_SURFACE ( 'NONE', #31942, 17.82106496071139645 ) ;
#36588=CARTESIAN_POINT ( 'NONE',  ( 147.4323331177958494, 275.2867036919951147, -5.064030047414062707 ) ) ;
#36591=ORIENTED_EDGE ( 'NONE', *, *, #59293, .T. ) ;
#36593=CARTESIAN_POINT ( 'NONE',  ( 168.9557235653834368, 272.5620232158073009, 16.16789404307498046 ) ) ;
#36594=CARTESIAN_POINT ( 'NONE',  ( 190.9586609929293104, 299.8968923453624598, -4.970176667899034229 ) ) ;
#36596=CARTESIAN_POINT ( 'NONE',  ( 190.0226014859668453, 301.5181949703289774, 3.835066345245774500 ) ) ;
#36597=CARTESIAN_POINT ( 'NONE',  ( 152.7153488183568300, 266.1362520814392951, 17.33540622643059237 ) ) ;
#36598=CARTESIAN_POINT ( 'NONE',  ( 191.1017707189859038, 299.6490190287749442, 8.670441576909594161 ) ) ;
#36599=CARTESIAN_POINT ( 'NONE',  ( 147.3047606266276546, 275.5076657283461827, -0.02269072295920609994 ) ) ;
#36600=VERTEX_POINT ( 'NONE', #50468 ) ;
#36601=CARTESIAN_POINT ( 'NONE',  ( 161.4250356354754672, 267.9004136800010656, 17.49898951125957680 ) ) ;
#36603=CARTESIAN_POINT ( 'NONE',  ( 164.3754245770190039, 245.9404084473339083, 1.667926061651832992 ) ) ;
#36605=CARTESIAN_POINT ( 'NONE',  ( 169.7005567072155259, 288.7155782076579271, 4.430715832634252394 ) ) ;
#36608=CARTESIAN_POINT ( 'NONE',  ( 190.1097268253669199, 301.3672894558616804, -3.549398112984228248 ) ) ;
#36610=CARTESIAN_POINT ( 'NONE',  ( 202.9764883503618478, 278.1159216087813775, 15.04054422000245594 ) ) ;
#36612=CARTESIAN_POINT ( 'NONE',  ( 179.5901059084964118, 282.7925552602970924, -15.57911077479886863 ) ) ;
#36613=CARTESIAN_POINT ( 'NONE',  ( 189.8565127379117428, 301.8058691205260402, -0.2865444372480985269 ) ) ;
#36614=ORIENTED_EDGE ( 'NONE', *, *, #92160, .F. ) ;
#36615=CARTESIAN_POINT ( 'NONE',  ( 208.3790849386676598, 269.7238329819538762, -1.525282248498321946 ) ) ;
#36617=CARTESIAN_POINT ( 'NONE',  ( 155.4926790358130688, 262.9189171763118225, 17.50096092146387505 ) ) ;
#36618=CARTESIAN_POINT ( 'NONE',  ( 41.93414601462609426, 195.0177522451418781, -10.00000000000009592 ) ) ;
#36619=CARTESIAN_POINT ( 'NONE',  ( 119.6601863278771845, 230.7048013555409796, 4.594050593750051981 ) ) ;
#36620=CARTESIAN_POINT ( 'NONE',  ( 151.3681950933278983, 268.4695907787949523, -15.50699599486383917 ) ) ;
#36622=CARTESIAN_POINT ( 'NONE',  ( 96.08673418588705317, 237.8297689869269220, -2.679491924311252493 ) ) ;
#36624=CARTESIAN_POINT ( 'NONE',  ( 29.24128764430186322, 193.8149278399160664, 9.188101187500093303 ) ) ;
#36629=VERTEX_POINT ( 'NONE', #42361 ) ;
#36632=CARTESIAN_POINT ( 'NONE',  ( -22.42236680055709641, 157.8615022471902591, 0.000000000000000000 ) ) ;
#36638=CARTESIAN_POINT ( 'NONE',  ( 68.64667992883292413, 198.8932355074535394, -2.679491924311248496 ) ) ;
#36639=CARTESIAN_POINT ( 'NONE',  ( 182.2453976510401219, 262.6361998111093499, 12.88021352968282152 ) ) ;
#36640=CARTESIAN_POINT ( 'NONE',  ( 97.79278455872238851, 227.2677522451418497, 10.00000000000009592 ) ) ;
#36644=CARTESIAN_POINT ( 'NONE',  ( 158.7916629078209496, 282.1994322289544925, -1.630852128393389666 ) ) ;
#36646=CARTESIAN_POINT ( 'NONE',  ( 5.696048431029936410, 186.3464784336661637, 1.353441290958777327E-15 ) ) ;
#36648=CARTESIAN_POINT ( 'NONE',  ( 195.7970677195757219, 273.6457781951527295, 14.65595583657620615 ) ) ;
#36650=CARTESIAN_POINT ( 'NONE',  ( 180.9072258576007073, 278.7294345915424287, 17.56943982383666736 ) ) ;
#36651=CARTESIAN_POINT ( 'NONE',  ( 58.41569198217266035, 204.5333772461660544, 9.188101187500095079 ) ) ;
#36652=CARTESIAN_POINT ( 'NONE',  ( 207.5570596878370679, 271.1476224814971374, 2.444960520848353358 ) ) ;
#36655=CARTESIAN_POINT ( 'NONE',  ( 207.6900289502458179, 270.9173129631602706, 7.178327969100043227 ) ) ;
#36658=CARTESIAN_POINT ( 'NONE',  ( 25.13686162393838330, 171.9865022471901739, 1.119607411625061291E-15 ) ) ;
#36659=CARTESIAN_POINT ( 'NONE',  ( 207.6172352878830907, 271.0433952848413810, 3.316653249540578496 ) ) ;
#36660=CARTESIAN_POINT ( 'NONE',  ( 144.1522069568320887, 254.0333772461660260, 9.188101187500095079 ) ) ;
#36662=CARTESIAN_POINT ( 'NONE',  ( 164.8095417749603939, 245.1884954040601201, 0.9289438697355421048 ) ) ;
#36664=CARTESIAN_POINT ( 'NONE',  ( 63.56442718099752653, 219.0530062829863027, -4.648177544792955347E-16 ) ) ;
#36666=CARTESIAN_POINT ( 'NONE',  ( 186.7527615248176858, 288.4939651830034677, 14.54212105726466753 ) ) ;
#36668=VERTEX_POINT ( 'NONE', #72815 ) ;
#36670=CARTESIAN_POINT ( 'NONE',  ( 207.7185302857748468, 270.8679472019405239, -1.571522964764315855 ) ) ;
#36671=CARTESIAN_POINT ( 'NONE',  ( 181.7713838635636137, 288.0101961225868763, 13.76523526626820626 ) ) ;
#36673=CARTESIAN_POINT ( 'NONE',  ( 197.2954959431661450, 273.3383094587030655, -14.52450022571995447 ) ) ;
#36683=CARTESIAN_POINT ( 'NONE',  ( 153.2906404175950854, 265.1398178023911782, -17.60231834963988007 ) ) ;
#36684=EDGE_LOOP ( 'NONE', ( #2767, #44779, #80103, #24392 ) ) ;
#36685=CARTESIAN_POINT ( 'NONE',  ( 163.9961211234992788, 256.9275610305372766, 16.20495027727189807 ) ) ;
#36687=CARTESIAN_POINT ( 'NONE',  ( 169.5762389015176552, 277.3387613457686030, 16.19092595284562108 ) ) ;
#36688=ORIENTED_EDGE ( 'NONE', *, *, #48703, .T. ) ;
#36693=CARTESIAN_POINT ( 'NONE',  ( 147.0276296945837373, 275.9876705829954062, 0.7617065417431535534 ) ) ;
#36695=CARTESIAN_POINT ( 'NONE',  ( 185.4098756247172162, 291.0786892564822210, 12.10185257883743759 ) ) ;
#36696=CARTESIAN_POINT ( 'NONE',  ( 163.8040269124969939, 246.9300982336122559, 6.025552750865228013 ) ) ;
#36697=CARTESIAN_POINT ( 'NONE',  ( 189.5154352181616844, 269.0707619020402035, -14.34315308920730558 ) ) ;
#36699=CARTESIAN_POINT ( 'NONE',  ( 88.80803131805656392, 212.8923013555409796, 4.594050593750050204 ) ) ;
#36700=CARTESIAN_POINT ( 'NONE',  ( 199.4204983887044591, 283.3295232521138587, 17.12415080298291059 ) ) ;
#36703=CARTESIAN_POINT ( 'NONE',  ( 177.9519160049562743, 269.0639553700436863, -16.55811740720082526 ) ) ;
#36707=EDGE_CURVE ( 'NONE', #21557, #78500, #64781, .T. ) ;
#36710=EDGE_LOOP ( 'NONE', ( #56666, #34903, #16903, #80116, #93178, #57287 ) ) ;
#36716=CARTESIAN_POINT ( 'NONE',  ( 165.0017188223714868, 244.8556349938953929, 2.184410744653827674 ) ) ;
#36722=CARTESIAN_POINT ( 'NONE',  ( 195.7108479875464297, 291.6658630236173622, -17.27467541470428714 ) ) ;
#36727=CARTESIAN_POINT ( 'NONE',  ( 165.7352987039666061, 282.5727979134155134, 8.872472809700889584 ) ) ;
#36731=CARTESIAN_POINT ( 'NONE',  ( 202.2712651538608668, 280.3028871727136675, 16.13191389836473988 ) ) ;
#36732=CARTESIAN_POINT ( 'NONE',  ( 188.2057398500588192, 260.7838726571292227, 2.785644019878456668 ) ) ;
#36733=CARTESIAN_POINT ( 'NONE',  ( 152.0629200551952351, 277.0898023037734674, -5.235464967198216080 ) ) ;
#36737=CARTESIAN_POINT ( 'NONE',  ( 157.8229873034836999, 281.2890896376861747, 1.531573202618901508 ) ) ;
#36738=ORIENTED_EDGE ( 'NONE', *, *, #85057, .T. ) ;
#36739=CARTESIAN_POINT ( 'NONE',  ( 181.8744732730408487, 270.4285964791639572, -16.45852818176540922 ) ) ;
#36743=CARTESIAN_POINT ( 'NONE',  ( 7.022496928113825199, 174.8615022471902591, -10.00000000000009592 ) ) ;
#36744=CARTESIAN_POINT ( 'NONE',  ( 0.2927578493243879754, 157.6427522451417360, 1.119607411625061291E-15 ) ) ;
#36745=CARTESIAN_POINT ( 'NONE',  ( 192.8093881745433578, 266.9317635038931940, -11.27160849829442668 ) ) ;
#36747=CARTESIAN_POINT ( 'NONE',  ( 170.1404595856897686, 280.7340597449264692, -14.11196382480607170 ) ) ;
#36749=CARTESIAN_POINT ( 'NONE',  ( 161.3667600300080380, 272.7931144062943076, 15.17166901843044080 ) ) ;
#36750=CARTESIAN_POINT ( 'NONE',  ( 1.691375130056927079, 159.5327760586659451, 1.948934522072303157E-15 ) ) ;
#36751=CARTESIAN_POINT ( 'NONE',  ( -4.037369169597886831, 175.1427522451419065, 10.00000000000009415 ) ) ;
#36753=CARTESIAN_POINT ( 'NONE',  ( 187.9452548533183460, 296.3769502305851233, 8.122909483408376374 ) ) ;
#36755=ORIENTED_EDGE ( 'NONE', *, *, #70139, .F. ) ;
#36758=EDGE_CURVE ( 'NONE', #88888, #38611, #59044, .T. ) ;
#36761=CARTESIAN_POINT ( 'NONE',  ( 202.5853389232562733, 279.7588954467959752, -15.97445231646760178 ) ) ;
#36762=CARTESIAN_POINT ( 'NONE',  ( 46.28462696178780789, 185.9824982072973967, 3.021315404115420679E-15 ) ) ;
#36763=CARTESIAN_POINT ( 'NONE',  ( 153.4741497343565868, 278.8061389251365654, 3.770324642130308934 ) ) ;
#36764=CARTESIAN_POINT ( 'NONE',  ( 20.58138070222250349, 176.5643266524160140, -9.188101187500093303 ) ) ;
#36765=CARTESIAN_POINT ( 'NONE',  ( 113.7873647845227225, 230.3768266524160140, -9.188101187500091527 ) ) ;
#36767=DIRECTION ( 'NONE',  ( -0.8660254037844387076, -0.4999999999999998890, -0.000000000000000000 ) ) ;
#36769=CARTESIAN_POINT ( 'NONE',  ( 206.2370539054256824, 271.7243903019979143, -8.078859316864654971 ) ) ;
#36770=CARTESIAN_POINT ( 'NONE',  ( 175.4961364399792672, 281.6643638624120172, -14.18804244962221794 ) ) ;
#36772=CARTESIAN_POINT ( 'NONE',  ( 65.31683191680592415, 208.5177522451418497, -10.00000000000009592 ) ) ;
#36774=CARTESIAN_POINT ( 'NONE',  ( 154.8838596469624349, 262.3802811495310152, 18.07457254681616021 ) ) ;
#36775=CARTESIAN_POINT ( 'NONE',  ( 184.4288184562230697, 274.3616139070439317, 17.06261365940633468 ) ) ;
#36780=CARTESIAN_POINT ( 'NONE',  ( 186.7681815113486437, 299.1371796739298361, -0.6084766120471760686 ) ) ;
#36782=CARTESIAN_POINT ( 'NONE',  ( 67.06923665261433598, 197.9824982072973967, 3.021315404115420679E-15 ) ) ;
#36783=ADVANCED_FACE ( 'NONE', ( #16331 ), #94214, .F. ) ;
#36784=DIRECTION ( 'NONE',  ( -0.8660254037844387076, -0.4999999999999998890, -0.000000000000000000 ) ) ;
#36786=CARTESIAN_POINT ( 'NONE',  ( 96.08779704679574252, 226.2833772461660260, -9.188101187500095079 ) ) ;
#36789=CARTESIAN_POINT ( 'NONE',  ( 187.6937625757019248, 280.4432552554100653, 17.79435256663161624 ) ) ;
#36790=CARTESIAN_POINT ( 'NONE',  ( 152.0771670635943451, 267.2416153051512424, 17.00512325015557380 ) ) ;
#36791=CARTESIAN_POINT ( 'NONE',  ( 196.3641580329410203, 290.5342968318988142, 17.59485314755329810 ) ) ;
#36792=CARTESIAN_POINT ( 'NONE',  ( 151.4428545556028780, 268.3402767968688067, -15.03309903163500749 ) ) ;
#36793=CARTESIAN_POINT ( 'NONE',  ( 173.4712241781546993, 267.5592519596314673, -16.59005366076430477 ) ) ;
#36795=CARTESIAN_POINT ( 'NONE',  ( 193.0142717932987182, 296.3364699985351081, -13.30037542329744937 ) ) ;
#36801=CARTESIAN_POINT ( 'NONE',  ( 193.0761489135300906, 296.2292956824684893, -11.99675185248219655 ) ) ;
#36802=CARTESIAN_POINT ( 'NONE',  ( 197.0184425104562820, 289.4010428742387262, -16.90752553128928426 ) ) ;
#36803=EDGE_CURVE ( 'NONE', #23266, #76921, #47519, .T. ) ;
#36804=B_SPLINE_CURVE_WITH_KNOTS ( 'NONE', 3,
 ( #45384, #14501, #13516, #22593 ),
 .UNSPECIFIED., .F., .F.,
 ( 4, 4 ),
 ( 0.009404506255995710717, 0.01466610642007075069 ),
 .UNSPECIFIED. ) ;
#36806=CARTESIAN_POINT ( 'NONE',  ( 198.6755293322981117, 286.5308843062557571, 17.86676876308990103 ) ) ;
#36807=CARTESIAN_POINT ( 'NONE',  ( 157.5527251258240256, 268.7623409241362538, 15.65735544631393772 ) ) ;
#36808=CARTESIAN_POINT ( 'NONE',  ( -17.42236680055705023, 149.2012482093457777, 0.000000000000000000 ) ) ;
#36809=CARTESIAN_POINT ( 'NONE',  ( 139.5965524907817041, 244.7365022471902023, -10.00000000000009059 ) ) ;
#36813=CARTESIAN_POINT ( 'NONE',  ( 190.2187748366491178, 299.5345473012424691, -6.575473572855297100 ) ) ;
#36814=ORIENTED_EDGE ( 'NONE', *, *, #27456, .F. ) ;
#36816=CARTESIAN_POINT ( 'NONE',  ( 167.6278246310154714, 282.5728663012718584, -12.21306354836790220 ) ) ;
#36820=B_SPLINE_CURVE_WITH_KNOTS ( 'NONE', 3,
 ( #54770, #47173, #39057, #86745 ),
 .UNSPECIFIED., .F., .F.,
 ( 4, 4 ),
 ( 0.01222404534472665630, 0.01842418820188282402 ),
 .UNSPECIFIED. ) ;
#36821=ORIENTED_EDGE ( 'NONE', *, *, #15771, .F. ) ;
#36822=CARTESIAN_POINT ( 'NONE',  ( 39.16110834368297589, 204.9637435831424739, 2.679491924311251605 ) ) ;
#36824=DIRECTION ( 'NONE',  ( 0.5000000000000007772, -0.8660254037844381525, 0.000000000000000000 ) ) ;
#36825=CARTESIAN_POINT ( 'NONE',  ( 191.6668504928946959, 279.4506890766722904, -16.59293083056063267 ) ) ;
#36826=CARTESIAN_POINT ( 'NONE',  ( 193.2920900494724492, 295.8552746635717767, -12.94670270598705031 ) ) ;
#36827=CARTESIAN_POINT ( 'NONE',  ( 152.6621968174709991, 266.2283140474973493, -17.02835521334403168 ) ) ;
#36833=CYLINDRICAL_SURFACE ( 'NONE', #22260, 17.82106496071139645 ) ;
#36837=CARTESIAN_POINT ( 'NONE',  ( 157.6500260163024620, 257.5891404556457474, -18.23450497588216379 ) ) ;
#36839=CARTESIAN_POINT ( 'NONE',  ( 173.8469137325424185, 256.4471593116459189, -12.44389045026504270 ) ) ;
#36840=CARTESIAN_POINT ( 'NONE',  ( 165.7305853283280612, 273.9508576969337241, -15.18882091205272289 ) ) ;
#36842=CARTESIAN_POINT ( 'NONE',  ( 197.6251864986240889, 273.3509762406971504, -13.38841307642727863 ) ) ;
#36843=CARTESIAN_POINT ( 'NONE',  ( 157.8143401782468800, 281.6959594171767662, 4.961866816185521500 ) ) ;
#36846=CARTESIAN_POINT ( 'NONE',  ( 170.5559173367651340, 288.6221555414043678, -4.098126037284842482 ) ) ;
#36849=CARTESIAN_POINT ( 'NONE',  ( 117.4951228184160783, 229.4548013555409796, -4.594050593750042211 ) ) ;
#36850=CARTESIAN_POINT ( 'NONE',  ( 148.1723659060776299, 275.6436025059589383, -5.668295273900294085 ) ) ;
#36852=CARTESIAN_POINT ( 'NONE',  ( 191.8882076080898003, 275.3147623427439044, 16.31405584673956355 ) ) ;
#36857=CARTESIAN_POINT ( 'NONE',  ( 180.7471050872008220, 294.1104588566450388, -2.489982966172171075 ) ) ;
#36859=CARTESIAN_POINT ( 'NONE',  ( 195.6986305151803549, 291.6870243064952888, 16.84182339398051909 ) ) ;
#36860=CARTESIAN_POINT ( 'NONE',  ( 190.4322164364161836, 300.4051867369805109, -0.3674591292211766835 ) ) ;
#36864=( BOUNDED_CURVE ( )  B_SPLINE_CURVE ( 2, ( #8753, #61444, #31045, #39624, #61932, #77151, #92396, #53832, #48254 ),
 .UNSPECIFIED., .F., .T. ) 
 B_SPLINE_CURVE_WITH_KNOTS ( ( 3, 2, 2, 2, 3 ),
 ( 0.3024193548387096864, 0.3037634408602150615, 0.3064516129032258118, 0.3091397849462365621, 0.3104838709677419373 ),
 .UNSPECIFIED. ) 
 CURVE ( )  GEOMETRIC_REPRESENTATION_ITEM ( )  RATIONAL_B_SPLINE_CURVE ( ( 0.9330127018922194093, 0.9330127018922194093, 1.000000000000000000, 0.8660254037844387076, 1.000000000000000000, 0.8660254037844387076, 1.000000000000000000, 0.9330127018922194093, 0.9330127018922194093 ) ) 
 REPRESENTATION_ITEM ( '' )  );
#36869=B_SPLINE_CURVE_WITH_KNOTS ( 'NONE', 3,
 ( #7045, #8061, #14155, #92201 ),
 .UNSPECIFIED., .F., .F.,
 ( 4, 4 ),
 ( 0.009708450334000175153, 0.01488528937472419038 ),
 .UNSPECIFIED. ) ;
#36870=CARTESIAN_POINT ( 'NONE',  ( 192.0312662756419968, 263.6944243638656644, -8.255564916146489907 ) ) ;
#36871=CARTESIAN_POINT ( 'NONE',  ( 191.2622316156482043, 288.8574828335728171, -16.55244734589887656 ) ) ;
#36873=CARTESIAN_POINT ( 'NONE',  ( 185.8658015726157942, 289.8550116424679572, -13.28855460030198188 ) ) ;
#36874=CARTESIAN_POINT ( 'NONE',  ( 160.3427821849308827, 281.3332481746720646, 5.617732255323795165 ) ) ;
#36875=CARTESIAN_POINT ( 'NONE',  ( 201.2535035105529744, 282.0657020489176716, -18.08976065250591958 ) ) ;
#36876=ORIENTED_EDGE ( 'NONE', *, *, #2303, .F. ) ;
#36877=CARTESIAN_POINT ( 'NONE',  ( 147.4811722709131914, 275.2021117973970377, 3.890385073228495916 ) ) ;
#36878=B_SPLINE_SURFACE_WITH_KNOTS ( 'NONE', 3, 1, ( 
 ( #92631, #31773 ),
 ( #23180, #16590 ),
 ( #47142, #9679 ),
 ( #8654, #2574 ),
 ( #17769, #2067 ),
 ( #25349, #63851 ),
 ( #47639, #64864 ),
 ( #78573, #71474 ),
 ( #94790, #41033 ),
 ( #33980, #93798 ),
 ( #25875, #24848 ),
 ( #62843, #40540 ),
 ( #56242, #39525 ),
 ( #3089, #71970 ),
 ( #70450, #16252 ),
 ( #9157, #32458 ),
 ( #79095, #32947 ),
 ( #33458, #31938 ),
 ( #86213, #95811 ),
 ( #10666, #48152 ),
 ( #87235, #56750 ),
 ( #1059, #70973 ),
 ( #64354, #48670 ),
 ( #40033, #87732 ),
 ( #79603, #55723 ),
 ( #1575, #63355 ),
 ( #10166, #95318 ),
 ( #16751, #24359 ),
 ( #72487, #94294 ),
 ( #55230, #18270 ),
 ( #49164, #86711 ),
 ( #17247, #80100 ),
 ( #41542, #54734 ),
 ( #85717, #78067 ) ),
 .UNSPECIFIED., .T., .F., .F.,
 ( 4, 2, 2, 2, 2, 2, 2, 2, 2, 2, 2, 2, 2, 2, 2, 2, 4 ),
 ( 2, 2 ),
 ( 0.000000000000000000, 0.06250000000000000000, 0.1250000000000000000, 0.1875000000000000000, 0.2500000000000000000, 0.3125000000000000000, 0.3750000000000000000, 0.4375000000000000000, 0.5000000000000000000, 0.5625000000000000000, 0.6250000000000000000, 0.6875000000000000000, 0.7500000000000000000, 0.8125000000000000000, 0.8750000000000000000, 0.9375000000000000000, 1.000000000000000000 ),
 ( 0.000000000000000000, 1.000000000000000000 ),
 .UNSPECIFIED. ) ;
#36879=CARTESIAN_POINT ( 'NONE',  ( 182.4502886106904214, 259.6876753163259650, 10.69873880494191631 ) ) ;
#36881=CARTESIAN_POINT ( 'NONE',  ( 170.3483830181634744, 248.6468970521230517, -0.2708202233927377578 ) ) ;
#36882=CARTESIAN_POINT ( 'NONE',  ( 189.1385169928410050, 270.1064989654813644, -14.07419399057638643 ) ) ;
#36885=AXIS2_PLACEMENT_3D ( 'NONE', #42246, #73182, #57449 ) ;
#36887=CARTESIAN_POINT ( 'NONE',  ( 75.51934661115029712, 226.6589784336661637, -6.496448406907675876E-16 ) ) ;
#36888=CARTESIAN_POINT ( 'NONE',  ( 206.6703863510205679, 272.6833857505801006, -10.72500664779635393 ) ) ;
#36891=ADVANCED_FACE ( 'NONE', ( #42 ), #96144, .T. ) ;
#36892=CARTESIAN_POINT ( 'NONE',  ( 207.1007598919583472, 271.9379569114424271, -6.086525981869248092 ) ) ;
#36896=EDGE_CURVE ( 'NONE', #63534, #31479, #27384, .T. ) ;
#36898=CARTESIAN_POINT ( 'NONE',  ( 149.7629758376029656, 272.4687595327688996, -11.42952473512502465 ) ) ;
#36902=CARTESIAN_POINT ( 'NONE',  ( 23.88258191050314494, 196.8464784336661637, 1.353441290958777327E-15 ) ) ;
#36903=CARTESIAN_POINT ( 'NONE',  ( 196.2255671652529259, 290.7743432561995860, 16.01325193769018185 ) ) ;
#36907=CARTESIAN_POINT ( 'NONE',  ( 54.19381813872350762, 202.0958772461660544, -9.188101187500095079 ) ) ;
#36908=VECTOR ( 'NONE', #89408, 1000.000000000000000 ) ;
#36910=CARTESIAN_POINT ( 'NONE',  ( 151.4376533647338476, 268.3492855237141725, -15.16853828792834236 ) ) ;
#36913=CARTESIAN_POINT ( 'NONE',  ( 204.9463377925012253, 275.6695254486514841, -14.15865086131798378 ) ) ;
#36914=CARTESIAN_POINT ( 'NONE',  ( 159.7106966763185483, 255.6638636138267486, -16.45402655586279650 ) ) ;
#36917=EDGE_LOOP ( 'NONE', ( #51542, #79550, #58050, #82506 ) ) ;
#36920=CARTESIAN_POINT ( 'NONE',  ( 163.8070446421170629, 255.0663642890118581, -15.42060242571707818 ) ) ;
#36921=DIRECTION ( 'NONE',  ( 0.4999999999999998335, -0.8660254037844389297, 0.000000000000000000 ) ) ;
#36922=CARTESIAN_POINT ( 'NONE',  ( 91.45997379709659469, 223.6115022471902307, 10.00000000000009592 ) ) ;
#36923=CARTESIAN_POINT ( 'NONE',  ( 161.7910648966377209, 250.4166507187868831, 13.19274492748169436 ) ) ;
#36925=CARTESIAN_POINT ( 'NONE',  ( 194.6544274154721563, 285.5701803447823295, -17.66485059694058180 ) ) ;
#36926=ORIENTED_EDGE ( 'NONE', *, *, #95791, .F. ) ;
#36927=CARTESIAN_POINT ( 'NONE',  ( 56.95410056540389832, 209.8149278399160949, -9.188101187500095079 ) ) ;
#36928=VERTEX_POINT ( 'NONE', #97624 ) ;
#36929=CARTESIAN_POINT ( 'NONE',  ( 166.2602210121610256, 265.2243045114799429, 16.56391771334216756 ) ) ;
#36931=FACE_OUTER_BOUND ( 'NONE', #97223, .T. ) ;
#36932=ORIENTED_EDGE ( 'NONE', *, *, #99358, .T. ) ;
#36934=B_SPLINE_CURVE_WITH_KNOTS ( 'NONE', 3,
 ( #50035, #78968, #40417, #87614 ),
 .UNSPECIFIED., .F., .F.,
 ( 4, 4 ),
 ( 0.007229077686816304769, 0.01226561482239176340 ),
 .UNSPECIFIED. ) ;
#36940=CARTESIAN_POINT ( 'NONE',  ( 206.7789538869637909, 271.7428703762204805, -6.364171105215885582 ) ) ;
#36941=EDGE_LOOP ( 'NONE', ( #5293, #44038, #80261, #21786, #90483, #66503, #23748, #60991, #93560, #75484, #61592, #13924, #54614, #22797, #39412, #57515, #73350, #81818, #98508, #31585 ) ) ;
#36944=CARTESIAN_POINT ( 'NONE',  ( 157.7255603307123408, 268.5163524934444013, 16.86592485641857309 ) ) ;
#36946=VERTEX_POINT ( 'NONE', #5404 ) ;
#36948=CARTESIAN_POINT ( 'NONE',  ( 206.8851632406098702, 272.3113812655195716, -9.957011741946159233 ) ) ;
#36950=ORIENTED_EDGE ( 'NONE', *, *, #15399, .F. ) ;
#36952=CARTESIAN_POINT ( 'NONE',  ( 160.4221878081525858, 282.4388110396778870, -3.172333647399238732 ) ) ;
#36954=CARTESIAN_POINT ( 'NONE',  ( 208.3764315856425640, 269.7284287242038658, -1.833640725398759441 ) ) ;
#36955=CARTESIAN_POINT ( 'NONE',  ( 204.6427704787179493, 276.1953194596412118, 13.28850621060895953 ) ) ;
#36956=CARTESIAN_POINT ( 'NONE',  ( 198.4334039703542771, 286.9502577349437615, 18.47706603442866680 ) ) ;
#36958=CARTESIAN_POINT ( 'NONE',  ( 204.2708887182014337, 271.6324151636133593, 9.900201553234905916 ) ) ;
#36959=CARTESIAN_POINT ( 'NONE',  ( 130.3772506997096343, 236.8923013555409796, 4.594050593750050204 ) ) ;
#36960=CARTESIAN_POINT ( 'NONE',  ( 83.28711936893076029, 209.7048013555409796, 4.594050593750051981 ) ) ;
#36961=ORIENTED_EDGE ( 'NONE', *, *, #3349, .F. ) ;
#36962=CARTESIAN_POINT ( 'NONE',  ( 173.8944842169933906, 265.3883602040215237, 16.80249544060196598 ) ) ;
#36965=AXIS2_PLACEMENT_3D ( 'NONE', #70399, #47595, #38491 ) ;
#36967=CARTESIAN_POINT ( 'NONE',  ( 161.1048434630436077, 252.8929743723557522, 14.67917439587344397 ) ) ;
#36972=CARTESIAN_POINT ( 'NONE',  ( 194.3054841547469778, 284.7826021230907259, 17.31190127946796409 ) ) ;
#36975=CARTESIAN_POINT ( 'NONE',  ( 193.9495889092963807, 294.7164532324382549, 15.46986001312306058 ) ) ;
#36978=ORIENTED_EDGE ( 'NONE', *, *, #53061, .T. ) ;
#36980=CARTESIAN_POINT ( 'NONE',  ( 153.2583947049096764, 265.1956690150883560, -17.64103123457563882 ) ) ;
#36981=CARTESIAN_POINT ( 'NONE',  ( 200.6563829895864615, 283.0999451294737241, -16.73778976840113586 ) ) ;
#36986=CARTESIAN_POINT ( 'NONE',  ( 163.8003088823192286, 260.8948240748503054, -17.39314492925268141 ) ) ;
#36987=CARTESIAN_POINT ( 'NONE',  ( 164.1360809937824001, 246.7355779274738268, 4.829182325609949089 ) ) ;
#36988=CARTESIAN_POINT ( 'NONE',  ( 206.5117639185820906, 272.9581278627833285, 11.28485531511759099 ) ) ;
#36989=CARTESIAN_POINT ( 'NONE',  ( 196.2379679265050925, 290.7528645076583871, -16.93678934971137906 ) ) ;
#36990=CARTESIAN_POINT ( 'NONE',  ( 38.99326808448932979, 199.9865022471903160, 10.00000000000009415 ) ) ;
#36991=CARTESIAN_POINT ( 'NONE',  ( 159.3000756570304475, 259.5621139873742322, 16.68461091752545755 ) ) ;
#36993=CARTESIAN_POINT ( 'NONE',  ( 137.4948102131217524, 244.0643266524159856, -9.188101187500093303 ) ) ;
#37002=AXIS2_PLACEMENT_3D ( 'NONE', #38543, #77044, #75572 ) ;
#37003=CARTESIAN_POINT ( 'NONE',  ( 182.1292595431042400, 275.5821809811551475, -16.44815416891946569 ) ) ;
#37007=CARTESIAN_POINT ( 'NONE',  ( 198.4797950122827217, 266.2212529384890445, 0.7508312083940900106 ) ) ;
#37008=CARTESIAN_POINT ( 'NONE',  ( 190.8683709797118411, 300.0532792356709706, -4.461919767133968762 ) ) ;
#37009=CARTESIAN_POINT ( 'NONE',  ( 186.8391812638637077, 282.1527847936219473, 16.55419741524866595 ) ) ;
#37011=CARTESIAN_POINT ( 'NONE',  ( 157.1002372043759010, 258.5414026113353430, -17.73553732786789539 ) ) ;
#37012=CARTESIAN_POINT ( 'NONE',  ( 195.5754259164033897, 270.4482758609249800, 12.00730134518774683 ) ) ;
#37016=CARTESIAN_POINT ( 'NONE',  ( 205.4596735342297791, 274.3777508883674727, 10.94792961590592029 ) ) ;
#37018=CARTESIAN_POINT ( 'NONE',  ( 198.5966822647444587, 286.6674514332866579, 17.25284514431582750 ) ) ;
#37020=CARTESIAN_POINT ( 'NONE',  ( 207.1728383846156589, 271.8131133000269983, 5.812426782309712436 ) ) ;
#37021=CARTESIAN_POINT ( 'NONE',  ( -2.801305199957352166, 163.0643266524159571, -9.188101187500093303 ) ) ;
#37022=B_SPLINE_CURVE_WITH_KNOTS ( 'NONE', 3,
 ( #8244, #17329, #39109, #48235 ),
 .UNSPECIFIED., .F., .F.,
 ( 4, 4 ),
 ( 0.008522409322521112135, 0.01490883787878987191 ),
 .UNSPECIFIED. ) ;
#37023=CARTESIAN_POINT ( 'NONE',  ( 175.5585873154026046, 286.2329552154398584, -11.98263329848505698 ) ) ;
#37024=ORIENTED_EDGE ( 'NONE', *, *, #77318, .F. ) ;
#37027=CARTESIAN_POINT ( 'NONE',  ( 65.93257831369518840, 197.3262482093457777, 3.021315404115420679E-15 ) ) ;
#37028=CARTESIAN_POINT ( 'NONE',  ( 150.6916211261701619, 269.6414512649903941, -15.44346024757110847 ) ) ;
#37029=CARTESIAN_POINT ( 'NONE',  ( 6.129408228687162286, 174.3458772461660828, 9.188101187500095079 ) ) ;
#37030=CARTESIAN_POINT ( 'NONE',  ( 181.6389525841213128, 276.3973689590053482, -17.23735931286679346 ) ) ;
#37035=CARTESIAN_POINT ( 'NONE',  ( 150.1477792844964938, 276.5081346559795747, 3.786615811811071541 ) ) ;
#37036=CARTESIAN_POINT ( 'NONE',  ( 179.2145810957732692, 255.1730852940781062, -3.979500447435403210 ) ) ;
#37037=CARTESIAN_POINT ( 'NONE',  ( 197.9637121306999461, 287.7637878651254937, 17.83088679657193865 ) ) ;
#37038=CARTESIAN_POINT ( 'NONE',  ( 47.72569090598240393, 208.3615022471902876, 5.000000000000046185 ) ) ;
#37040=EDGE_CURVE ( 'NONE', #15680, #59906, #33486, .T. ) ;
#37041=CARTESIAN_POINT ( 'NONE',  ( 148.1634546024981205, 274.0203641339852538, 9.324875965062235039 ) ) ;
#37043=CARTESIAN_POINT ( 'NONE',  ( 10.18872876104421366, 182.8149278399160949, -9.188101187500095079 ) ) ;
#37044=CARTESIAN_POINT ( 'NONE',  ( 164.7946292899401328, 284.8120369531133633, 4.194565866339356575 ) ) ;
#37047=CARTESIAN_POINT ( 'NONE',  ( 133.8285102913215212, 259.6199935810940929, 2.679491924311251605 ) ) ;
#37048=AXIS2_PLACEMENT_3D ( 'NONE', #87576, #57081, #71313 ) ;
#37049=CARTESIAN_POINT ( 'NONE',  ( 164.2578067403839555, 246.1441285162624126, -2.322300236470859591 ) ) ;
#37050=CARTESIAN_POINT ( 'NONE',  ( 187.7682546158083881, 267.7859742100430935, 13.35512656275608734 ) ) ;
#37052=CARTESIAN_POINT ( 'NONE',  ( 164.1994998312905807, 281.4989144817481588, 9.158350551505991533 ) ) ;
#37056=CARTESIAN_POINT ( 'NONE',  ( 147.6857584380539095, 274.8477581613835810, 8.112022437684441201 ) ) ;
#37058=CARTESIAN_POINT ( 'NONE',  ( 194.4165969972361552, 293.9075714965812267, 14.23342188338008718 ) ) ;
#37059=ORIENTED_EDGE ( 'NONE', *, *, #96740, .T. ) ;
#37061=CARTESIAN_POINT ( 'NONE',  ( 185.3905017119345473, 290.9592364371351323, 12.17893237875644452 ) ) ;
#37064=CARTESIAN_POINT ( 'NONE',  ( 4.262040950003053830, 163.2677522451418213, -5.000000000000041744 ) ) ;
#37069=CARTESIAN_POINT ( 'NONE',  ( 203.0498946958275326, 278.9542612457532869, -15.11479947333269003 ) ) ;
#37073=CARTESIAN_POINT ( 'NONE',  ( 186.5027827276450409, 272.0212515145463499, -16.58127060163710098 ) ) ;
#37074=CARTESIAN_POINT ( 'NONE',  ( 204.7610021263893429, 275.9905362388115577, 13.36619428527026976 ) ) ;
#37080=VERTEX_POINT ( 'NONE', #46882 ) ;
#37081=CARTESIAN_POINT ( 'NONE',  ( 189.8123550829396891, 301.8823524224806647, -0.5679054518196169354 ) ) ;
#37084=CARTESIAN_POINT ( 'NONE',  ( 205.7576124508049418, 274.2643565215761328, 10.88614016733041545 ) ) ;
#37087=CARTESIAN_POINT ( 'NONE',  ( 190.8153366230912411, 300.1451374358846920, 3.771947273125533684 ) ) ;
#37088=CARTESIAN_POINT ( 'NONE',  ( 172.3662264184933406, 263.8501619316954248, -16.86127397973819697 ) ) ;
#37096=B_SPLINE_CURVE_WITH_KNOTS ( 'NONE', 3,
 ( #8812, #55885, #32617, #94452, #49321, #86880, #39681, #9840, #40699, #64522, #71641, #41196, #2235, #94955, #95479, #26032, #72648, #95965, #70608, #89849, #88887, #88383, #20424, #28496, #58880, #36093, #59376, #51290, #18936, #35101, #42201, #12833, #49813, #82261, #43695, #74636, #73621, #5211, #4725, #66994, #57907, #57402, #96458, #97920 ),
 .UNSPECIFIED., .F., .F.,
 ( 4, 2, 2, 2, 2, 2, 2, 2, 2, 2, 2, 2, 2, 2, 2, 2, 2, 2, 2, 2, 2, 4 ),
 ( 0.002595982006264980872, 0.003006620947792503981, 0.003211940418556245153, 0.003314600153938147831, 0.003417259889320051376, 0.003622579360083736169, 0.003827898830847421829, 0.004238537772374822640, 0.005059815655429624262, 0.005881093538484426751, 0.006702371421539228373, 0.007523649304594030862, 0.007626309039975908387, 0.007677638907666772990, 0.007728968775357637593, 0.007780298643048502195, 0.007831628510739365931, 0.007934288246121141974, 0.008139607716884652427, 0.008344927187648159411, 0.008755566129175173379, 0.009166205070702187346 ),
 .UNSPECIFIED. ) ;
#37098=CARTESIAN_POINT ( 'NONE',  ( 190.8907028847385448, 300.0145992415348815, -5.421341690443150618 ) ) ;
#37099=CARTESIAN_POINT ( 'NONE',  ( 188.6208318395044614, 298.5876672984960010, -4.287592830512637398 ) ) ;
#37100=CARTESIAN_POINT ( 'NONE',  ( 153.1164404339926080, 265.4415410246681972, 16.15325778160653414 ) ) ;
#37101=CARTESIAN_POINT ( 'NONE',  ( 146.7529223504909908, 276.4634776601763519, 0.7434588459654100090 ) ) ;
#37102=CARTESIAN_POINT ( 'NONE',  ( 191.0933613939813540, 299.6635844069401173, -8.689828987424775164 ) ) ;
#37105=CARTESIAN_POINT ( 'NONE',  ( 149.2765980486851731, 272.0923431290771646, -11.40617906909507973 ) ) ;
#37110=CARTESIAN_POINT ( 'NONE',  ( 103.7198194655286017, 224.5643266524159856, -9.188101187500093303 ) ) ;
#37112=CARTESIAN_POINT ( 'NONE',  ( 149.6870021971257643, 271.3815022923409401, -11.82311727174023552 ) ) ;
#37113=DIRECTION ( 'NONE',  ( -0.8660254037844359321, -0.5000000000000051070, -0.000000000000000000 ) ) ;
#37114=CARTESIAN_POINT ( 'NONE',  ( 149.3865244398207892, 273.6028616444142472, 10.34018256803319069 ) ) ;
#37116=CARTESIAN_POINT ( 'NONE',  ( 183.0283589768903028, 284.4709846154196953, -14.99738598492708341 ) ) ;
#37117=CARTESIAN_POINT ( 'NONE',  ( 147.9781162831602899, 274.3413795196678961, -10.04506445315961294 ) ) ;
#37119=CARTESIAN_POINT ( 'NONE',  ( 167.3377213335115812, 253.1226028751397621, -12.07944002830884678 ) ) ;
#37120=CARTESIAN_POINT ( 'NONE',  ( 205.7188332128827994, 273.9225886963720882, 10.29739696992246856 ) ) ;
#37122=CARTESIAN_POINT ( 'NONE',  ( 47.05812965368407674, 184.6427522451417360, 1.119607411625061291E-15 ) ) ;
#37123=CARTESIAN_POINT ( 'NONE',  ( 110.8370318831756975, 243.9869531367911009, 4.594050593750046652 ) ) ;
#37127=CARTESIAN_POINT ( 'NONE',  ( 195.6986305151803549, 291.6870243064952888, 16.84182339398051909 ) ) ;
#37128=CARTESIAN_POINT ( 'NONE',  ( 175.6656071552219487, 253.2019425609971393, -4.750314916192522219 ) ) ;
#37129=CARTESIAN_POINT ( 'NONE',  ( 36.00728465925030974, 191.5958772461660544, -9.188101187500095079 ) ) ;
#37132=ORIENTED_EDGE ( 'NONE', *, *, #15275, .T. ) ;
#37134=CARTESIAN_POINT ( 'NONE',  ( 181.4829458551834591, 267.5981693230167480, 14.92975384738928213 ) ) ;
#37136=FACE_OUTER_BOUND ( 'NONE', #85985, .T. ) ;
#37137=CARTESIAN_POINT ( 'NONE',  ( 146.8201187048455267, 276.3470901603510015, 4.112223577763169047 ) ) ;
#37139=DIRECTION ( 'NONE',  ( -0.8660254037844387076, -0.4999999999999998890, -0.000000000000000000 ) ) ;
#37140=EDGE_CURVE ( 'NONE', #55652, #19593, #38308, .T. ) ;
#37142=( BOUNDED_CURVE ( )  B_SPLINE_CURVE ( 2, ( #51442, #3859, #88518, #26657, #50445, #89510, #34253, #34743, #74284 ),
 .UNSPECIFIED., .F., .T. ) 
 B_SPLINE_CURVE_WITH_KNOTS ( ( 3, 2, 2, 2, 3 ),
 ( 0.05241935483870967943, 0.05376344086021505458, 0.05645161290322580488, 0.05913978494623656212, 0.06048387096774193727 ),
 .UNSPECIFIED. ) 
 CURVE ( )  GEOMETRIC_REPRESENTATION_ITEM ( )  RATIONAL_B_SPLINE_CURVE ( ( 0.9330127018922194093, 0.9330127018922194093, 1.000000000000000000, 0.8660254037844387076, 1.000000000000000000, 0.8660254037844387076, 1.000000000000000000, 0.9330127018922194093, 0.9330127018922194093 ) ) 
 REPRESENTATION_ITEM ( '' )  );
#37143=CARTESIAN_POINT ( 'NONE',  ( 176.4843944339568793, 285.6110925004390992, -12.05111447379141154 ) ) ;
#37145=CARTESIAN_POINT ( 'NONE',  ( 107.6799079185947221, 239.6427522451419065, 10.00000000000009237 ) ) ;
#37146=EDGE_CURVE ( 'NONE', #14672, #14901, #20215, .T. ) ;
#37148=CARTESIAN_POINT ( 'NONE',  ( 198.7985463335893996, 267.7170212918624088, -8.201462806822382490 ) ) ;
#37150=CARTESIAN_POINT ( 'NONE',  ( 155.8667045217748637, 279.9326319796254552, -1.585803574218712875 ) ) ;
#37151=CARTESIAN_POINT ( 'NONE',  ( 208.3764315856425640, 269.7284287242038658, -1.833640725398759441 ) ) ;
#37153=CARTESIAN_POINT ( 'NONE',  ( 6.183361268541195166, 180.5024278399160949, 9.188101187500095079 ) ) ;
#37155=CARTESIAN_POINT ( 'NONE',  ( 192.1472537951952972, 272.2648030127336369, 14.59637687883535229 ) ) ;
#37156=CARTESIAN_POINT ( 'NONE',  ( 192.4663556654298588, 297.2854885702906245, -12.98646995774174684 ) ) ;
#37157=LINE ( 'NONE', #83299, #62041 ) ;
#37158=CARTESIAN_POINT ( 'NONE',  ( 198.2327445038538087, 277.3384089221707427, -15.34475411346854834 ) ) ;
#37159=CARTESIAN_POINT ( 'NONE',  ( 55.54680928425421627, 209.0024278399160949, 9.188101187500095079 ) ) ;
#37160=CARTESIAN_POINT ( 'NONE',  ( 164.1146561143383167, 246.3920726737087534, -7.362905700427413436 ) ) ;
#37166=CARTESIAN_POINT ( 'NONE',  ( 19.94070920123175839, 168.9865022471901455, 1.119607411625061291E-15 ) ) ;
#37167=CARTESIAN_POINT ( 'NONE',  ( 207.6590484093196096, 270.9709728340903894, 3.402057849327809524 ) ) ;
#37168=CARTESIAN_POINT ( 'NONE',  ( 131.9464011004214115, 256.1744531367911009, 4.594050593750047540 ) ) ;
#37172=CARTESIAN_POINT ( 'NONE',  ( 72.31720393073018727, 205.8927522451418213, 10.00000000000009948 ) ) ;
#37174=CARTESIAN_POINT ( 'NONE',  ( 189.5357902666890482, 289.6679798450429075, 15.45925615865311009 ) ) ;
#37176=ORIENTED_EDGE ( 'NONE', *, *, #15710, .F. ) ;
#37180=CARTESIAN_POINT ( 'NONE',  ( 169.5394568650638121, 265.9945832123831906, -17.16958432082164876 ) ) ;
#37184=CARTESIAN_POINT ( 'NONE',  ( 172.6012549852709412, 290.2025030293380610, -5.021894074213228087 ) ) ;
#37186=CARTESIAN_POINT ( 'NONE',  ( 148.7640267652926411, 273.4591307251904482, -8.961959150306132216 ) ) ;
#37187=CARTESIAN_POINT ( 'NONE',  ( 32.15758756610207314, 177.8262482093457777, 3.021315404115420679E-15 ) ) ;
#37188=CARTESIAN_POINT ( 'NONE',  ( 149.8622666665893632, 273.0779353264732663, 11.47145096717591528 ) ) ;
#37190=CARTESIAN_POINT ( 'NONE',  ( 153.4495116231415750, 264.8646448025247082, -16.73555355292144498 ) ) ;
#37191=CARTESIAN_POINT ( 'NONE',  ( 155.8152618860606253, 260.7670451491295012, 0.000000000000000000 ) ) ;
#37195=CARTESIAN_POINT ( 'NONE',  ( 190.8138402884741254, 300.1477291634665789, 4.037153726988762514 ) ) ;
#37197=CARTESIAN_POINT ( 'NONE',  ( 189.0975612648258846, 297.0756752416021982, 8.129472812105014157 ) ) ;
#37198=VERTEX_POINT ( 'NONE', #31664 ) ;
#37200=CARTESIAN_POINT ( 'NONE',  ( 191.8456210280128005, 298.3606325003146367, -9.135603544929113085 ) ) ;
#37202=CARTESIAN_POINT ( 'NONE',  ( 163.9587364689194260, 246.6621334214722481, 5.816126667419880825 ) ) ;
#37203=EDGE_CURVE ( 'NONE', #75103, #88081, #79810, .T. ) ;
#37205=ORIENTED_EDGE ( 'NONE', *, *, #81541, .T. ) ;
#37206=CARTESIAN_POINT ( 'NONE',  ( 99.63334886536203783, 219.1423013555409796, -4.594050593750043987 ) ) ;
#37207=CARTESIAN_POINT ( 'NONE',  ( 199.6663384057308690, 283.4776756693757420, 17.08414512188284817 ) ) ;
#37208=CARTESIAN_POINT ( 'NONE',  ( 178.0354895240675717, 269.1313736818431721, -16.48722257503622757 ) ) ;
#37212=ORIENTED_EDGE ( 'NONE', *, *, #24989, .T. ) ;
#37219=CARTESIAN_POINT ( 'NONE',  ( 207.6172352878830907, 271.0433952848413810, 3.316653249540578496 ) ) ;
#37222=EDGE_CURVE ( 'NONE', #44273, #80416, #65555, .T. ) ;
#37223=CARTESIAN_POINT ( 'NONE',  ( 12.14648056717172686, 184.4865022471903160, -10.00000000000009592 ) ) ;
#37225=CARTESIAN_POINT ( 'NONE',  ( 165.0834163913522445, 264.4347080444321136, -17.19626994086416261 ) ) ;
#37227=CARTESIAN_POINT ( 'NONE',  ( 175.3932935011599170, 269.2958584618301643, -17.65833184418574930 ) ) ;
#37232=CARTESIAN_POINT ( 'NONE',  ( 200.0873701903009021, 269.9495076100124038, 10.38151539442265836 ) ) ;
#37233=ORIENTED_EDGE ( 'NONE', *, *, #53520, .T. ) ;
#37234=CARTESIAN_POINT ( 'NONE',  ( 162.9148248802443106, 248.4702413316674381, 9.709394404200100581 ) ) ;
#37235=CARTESIAN_POINT ( 'NONE',  ( 187.7932394204981676, 260.5612834524825416, 2.855965374582485783 ) ) ;
#37236=CARTESIAN_POINT ( 'NONE',  ( 161.2744700912414828, 281.3972689067473993, -6.583020311435618943 ) ) ;
#37239=CARTESIAN_POINT ( 'NONE',  ( 168.5965412549398366, 253.6680249988097557, 11.50723466791552418 ) ) ;
#37241=ORIENTED_EDGE ( 'NONE', *, *, #87263, .F. ) ;
#37242=CARTESIAN_POINT ( 'NONE',  ( 181.6615078939564398, 271.3508032046874519, -15.97858828533330744 ) ) ;
#37244=CARTESIAN_POINT ( 'NONE',  ( 194.0351660592638439, 293.9963875260016266, -14.11356425598665432 ) ) ;
#37245=CARTESIAN_POINT ( 'NONE',  ( -0.5010987708114443828, 180.5177522451419350, 5.000000000000046185 ) ) ;
#37246=CARTESIAN_POINT ( 'NONE',  ( 192.9670459817621975, 266.8960202017726147, -11.36568172326798276 ) ) ;
#37248=CARTESIAN_POINT ( 'NONE',  ( 163.3597984219556167, 247.6995245493996833, -8.443090267489184342 ) ) ;
#37250=CARTESIAN_POINT ( 'NONE',  ( 160.7871907424899689, 272.7125984083364187, 15.60852731400909299 ) ) ;
#37251=CARTESIAN_POINT ( 'NONE',  ( -3.911334118262431936, 177.7369531367911293, -4.594050593750048428 ) ) ;
#37253=CARTESIAN_POINT ( 'NONE',  ( 189.1195168369542330, 296.9633965794964752, 8.417122978416381684 ) ) ;
#37254=VERTEX_POINT ( 'NONE', #93522 ) ;
#37259=CARTESIAN_POINT ( 'NONE',  ( 171.8934052655434073, 290.0727470064276190, 2.730291690633440016 ) ) ;
#37261=CARTESIAN_POINT ( 'NONE',  ( 162.4245261485180833, 249.3194636459039941, -11.14613848230852611 ) ) ;
#37264=CARTESIAN_POINT ( 'NONE',  ( 22.31343150979137846, 177.5643266524160708, 9.188101187500095079 ) ) ;
#37265=CARTESIAN_POINT ( 'NONE',  ( 120.1739550416679378, 246.3149278399160949, 9.188101187500093303 ) ) ;
#37266=CARTESIAN_POINT ( 'NONE',  ( 181.7448665231346467, 294.6636721014451155, -6.562496048646235813 ) ) ;
#37269=CARTESIAN_POINT ( 'NONE',  ( 206.6891045971790390, 272.2264157197300847, -7.035468968906900322 ) ) ;
#37270=EDGE_CURVE ( 'NONE', #81649, #48297, #74593, .T. ) ;
#37273=CARTESIAN_POINT ( 'NONE',  ( 60.96635096964421763, 217.5530062829863027, -4.648177544792955347E-16 ) ) ;
#37274=B_SPLINE_CURVE_WITH_KNOTS ( 'NONE', 3,
 ( #84562, #15101, #31799, #16614 ),
 .UNSPECIFIED., .F., .F.,
 ( 4, 4 ),
 ( 0.03043720490792996627, 0.03951895308350013292 ),
 .UNSPECIFIED. ) ;
#37276=CARTESIAN_POINT ( 'NONE',  ( 184.4054840374143680, 274.4020487136705810, 17.38799575625816374 ) ) ;
#37277=CARTESIAN_POINT ( 'NONE',  ( 189.9952630391477157, 284.7439679202585694, 16.81314581697001032 ) ) ;
#37278=CARTESIAN_POINT ( 'NONE',  ( 168.0280942669723458, 278.2301272409342232, 14.33002300203766488 ) ) ;
#37279=CARTESIAN_POINT ( 'NONE',  ( 192.6706003569902350, 265.2643762149980944, 7.794090319438162773 ) ) ;
#37283=AXIS2_PLACEMENT_3D ( 'NONE', #17708, #26307, #31882 ) ;
#37284=CARTESIAN_POINT ( 'NONE',  ( 184.7231325909508257, 269.5717479162897803, 15.41860894514769065 ) ) ;
#37285=CARTESIAN_POINT ( 'NONE',  ( 98.84807947347611901, 234.0024278399160664, -9.188101187500093303 ) ) ;
#37287=CARTESIAN_POINT ( 'NONE',  ( 150.7254409736883645, 269.5828735707850683, 14.54962197351449049 ) ) ;
#37291=CARTESIAN_POINT ( 'NONE',  ( 201.1561089954156500, 270.4184708626717111, -10.06927476064715066 ) ) ;
#37293=CARTESIAN_POINT ( 'NONE',  ( 163.2055398469344993, 284.3816007520933340, -6.092379576987982048 ) ) ;
#37294=CARTESIAN_POINT ( 'NONE',  ( 193.0065576635309412, 296.3498312632291913, -11.90044991639595295 ) ) ;
#37298=CARTESIAN_POINT ( 'NONE',  ( 153.2819058590468160, 274.2512448977743134, -12.24885634829186287 ) ) ;
#37299=CARTESIAN_POINT ( 'NONE',  ( 193.1028332910263998, 296.1830769848763225, -12.04975758233223893 ) ) ;
#37300=CARTESIAN_POINT ( 'NONE',  ( 196.9431415128477170, 289.5314680279574304, -16.61413060656005669 ) ) ;
#37302=CARTESIAN_POINT ( 'NONE',  ( 159.8416255366773839, 253.7931787365127434, 16.77980437810719394 ) ) ;
#37304=CARTESIAN_POINT ( 'NONE',  ( 172.6497489972219626, 253.7784896148466771, -8.913986932654800910 ) ) ;
#37306=CARTESIAN_POINT ( 'NONE',  ( 127.8330407560429904, 254.6115022471903160, -5.000000000000047962 ) ) ;
#37311=B_SPLINE_CURVE_WITH_KNOTS ( 'NONE', 3,
 ( #45229, #6237, #29542, #67534, #90895, #69022, #21445, #98464, #29057, #60414, #76166, #51853, #52331, #91881 ),
 .UNSPECIFIED., .F., .F.,
 ( 4, 2, 2, 2, 2, 2, 4 ),
 ( 0.0007405566181291618581, 0.001026655140925903124, 0.001312753663722644390, 0.001598852186519385439, 0.001884950709316126705, 0.002457147754909603382, 0.003029344800503079409 ),
 .UNSPECIFIED. ) ;
#37312=CARTESIAN_POINT ( 'NONE',  ( 183.9247570546335737, 291.7700146896927436, -10.70695736048003965 ) ) ;
#37315=CARTESIAN_POINT ( 'NONE',  ( 206.2281698397254956, 273.4493272160884771, 12.02209638042575612 ) ) ;
#37317=CARTESIAN_POINT ( 'NONE',  ( 201.0844796915553161, 282.3584598911111812, -16.59562674965125950 ) ) ;
#37318=DIRECTION ( 'NONE',  ( -0.8660254037844387076, -0.4999999999999998890, -0.000000000000000000 ) ) ;
#37325=ORIENTED_EDGE ( 'NONE', *, *, #19286, .T. ) ;
#37330=CARTESIAN_POINT ( 'NONE',  ( 165.9671773636226817, 274.1949923808492713, -15.14753692022039466 ) ) ;
#37332=CARTESIAN_POINT ( 'NONE',  ( 197.6821651709987577, 273.3821959209279271, -13.39123929363893062 ) ) ;
#37334=CARTESIAN_POINT ( 'NONE',  ( 148.1634546024981205, 274.0203641339852538, 9.324875965062235039 ) ) ;
#37335=CARTESIAN_POINT ( 'NONE',  ( 168.0124741839183855, 287.5020746026971779, -5.006766616574994444 ) ) ;
#37337=CARTESIAN_POINT ( 'NONE',  ( 165.8108829008523344, 266.0291451123555362, 17.22863011630727925 ) ) ;
#37338=CARTESIAN_POINT ( 'NONE',  ( 185.3484995286736421, 285.8968933059468895, -15.16821555540626854 ) ) ;
#37339=CARTESIAN_POINT ( 'NONE',  ( 116.0331843058823296, 246.9869531367911293, 4.594050593750046652 ) ) ;
#37343=CARTESIAN_POINT ( 'NONE',  ( 188.7546571689037194, 273.7569421533762011, 15.66845421830230478 ) ) ;
#37346=CARTESIAN_POINT ( 'NONE',  ( 162.9929399913377210, 248.7844230333444102, -9.774158786945124078 ) ) ;
#37347=CARTESIAN_POINT ( 'NONE',  ( 180.7478016446280549, 294.0847902074218609, -2.561698358318056368 ) ) ;
#37348=CARTESIAN_POINT ( 'NONE',  ( 147.2612474129807083, 275.5830328251833521, 2.671201371937485636 ) ) ;
#37349=CARTESIAN_POINT ( 'NONE',  ( 159.7692415128758228, 253.9185515433934768, -16.85856106119654285 ) ) ;
#37353=CARTESIAN_POINT ( 'NONE',  ( 195.4568363890616070, 292.1058240179047516, 16.34518427225309267 ) ) ;
#37358=CARTESIAN_POINT ( 'NONE',  ( 164.9103019330012216, 245.0139736909548560, 2.841678961959298810 ) ) ;
#37359=CARTESIAN_POINT ( 'NONE',  ( 194.9830273982886695, 264.9720653068531533, 4.415740111932965561 ) ) ;
#37362=CARTESIAN_POINT ( 'NONE',  ( 184.3650513960811281, 288.5837029191011993, -14.08819112931042916 ) ) ;
#37364=CARTESIAN_POINT ( 'NONE',  ( 153.3939648708017387, 264.9608545997728015, -16.49556533540763681 ) ) ;
#37366=CARTESIAN_POINT ( 'NONE',  ( 157.1517242151937523, 258.4522244926691883, 18.42395718741238042 ) ) ;
#37370=CARTESIAN_POINT ( 'NONE',  ( 173.1143141876224263, 251.5640903862351081, -0.2630518927552996100 ) ) ;
#37371=CARTESIAN_POINT ( 'NONE',  ( 192.3947780338729387, 271.6891214328757087, -14.51840760635450422 ) ) ;
#37374=CARTESIAN_POINT ( 'NONE',  ( 38.49039832772786696, 181.4824982072973683, 3.021315404115420679E-15 ) ) ;
#37376=CARTESIAN_POINT ( 'NONE',  ( 191.3096096579751304, 282.9911372872209654, -16.77114961036221530 ) ) ;
#37378=CARTESIAN_POINT ( 'NONE',  ( 80.33678646758374953, 223.3149278399160949, -9.188101187500095079 ) ) ;
#37379=DIRECTION ( 'NONE',  ( 0.2588190451025454974, 0.9659258262890615399, 0.000000000000000000 ) ) ;
#37381=CARTESIAN_POINT ( 'NONE',  ( 208.3764315856425640, 269.7284287242038658, -1.833640725398759441 ) ) ;
#37382=EDGE_CURVE ( 'NONE', #73834, #26527, #40631, .T. ) ;
#37383=CARTESIAN_POINT ( 'NONE',  ( 161.8935665241663457, 250.2391126920490194, -13.69501063978231770 ) ) ;
#37384=CARTESIAN_POINT ( 'NONE',  ( -22.42236680055709641, 157.8615022471902591, 0.000000000000000000 ) ) ;
#37388=CARTESIAN_POINT ( 'NONE',  ( 120.4921787521148246, 228.8262482093457777, 3.021315404115420679E-15 ) ) ;
#37394=CARTESIAN_POINT ( 'NONE',  ( 32.08336737017582152, 180.1423013555409796, -4.594050593750043987 ) ) ;
#37396=CARTESIAN_POINT ( 'NONE',  ( 199.4033704071922841, 277.6937026877216681, 15.29448692723246772 ) ) ;
#37399=CARTESIAN_POINT ( 'NONE',  ( 47.96943409690536697, 192.3768266524160140, 9.188101187500096856 ) ) ;
#37401=CARTESIAN_POINT ( 'NONE',  ( 170.7779774592389401, 287.5599273070118329, 7.147024354692598891 ) ) ;
#37402=CARTESIAN_POINT ( 'NONE',  ( 196.9319848161575806, 289.5507919934690335, -17.64330560362266453 ) ) ;
#37407=CARTESIAN_POINT ( 'NONE',  ( 179.4801981787712180, 276.6897665335758347, 16.30276041398731479 ) ) ;
#37409=CARTESIAN_POINT ( 'NONE',  ( 153.1524534015446761, 277.1654923934203225, 8.229120888094969999 ) ) ;
#37412=CARTESIAN_POINT ( 'NONE',  ( 88.86189758574322184, 232.1115022471902876, -5.000000000000047962 ) ) ;
#37413=CARTESIAN_POINT ( 'NONE',  ( 161.2313178023453588, 251.3861611254901618, 13.12937145726518473 ) ) ;
#37414=CARTESIAN_POINT ( 'NONE',  ( 164.8733870693940844, 270.4814310371710349, -16.86211258855632522 ) ) ;
#37416=CARTESIAN_POINT ( 'NONE',  ( 69.24135662524314228, 198.5327760586659451, 1.948934522072303157E-15 ) ) ;
#37417=ORIENTED_EDGE ( 'NONE', *, *, #68774, .F. ) ;
#37418=CARTESIAN_POINT ( 'NONE',  ( 166.3291615593880692, 265.1125154004245701, 16.59685441684288421 ) ) ;
#37419=CARTESIAN_POINT ( 'NONE',  ( 190.9441801652054096, 299.9219738747156043, -4.765040093794296716 ) ) ;
#37422=CYLINDRICAL_SURFACE ( 'NONE', #45695, 17.82106496071139645 ) ;
#37424=CARTESIAN_POINT ( 'NONE',  ( 194.9220242159064185, 293.0321458743159724, -14.92681063007793263 ) ) ;
#37426=CARTESIAN_POINT ( 'NONE',  ( 205.0608432903593155, 275.4711961086152883, 13.55071766891341412 ) ) ;
#37433=CARTESIAN_POINT ( 'NONE',  ( 200.7073644890481319, 268.7613916309068145, -8.767088900587291178 ) ) ;
#37434=CARTESIAN_POINT ( 'NONE',  ( 159.9894443651313338, 253.5371490153152081, -16.36035038356864391 ) ) ;
#37438=( BOUNDED_CURVE ( )  B_SPLINE_CURVE ( 2, ( #96432, #26995, #57880, #43159, #49295, #42663, #74100, #10802, #33089 ),
 .UNSPECIFIED., .F., .T. ) 
 B_SPLINE_CURVE_WITH_KNOTS ( ( 3, 2, 2, 2, 3 ),
 ( 0.8346774193548387455, 0.8360215053763441206, 0.8387096774193548709, 0.8413978494623656212, 0.8427419354838709964 ),
 .UNSPECIFIED. ) 
 CURVE ( )  GEOMETRIC_REPRESENTATION_ITEM ( )  RATIONAL_B_SPLINE_CURVE ( ( 0.9330127018922194093, 0.9330127018922194093, 1.000000000000000000, 0.8660254037844387076, 1.000000000000000000, 0.8660254037844387076, 1.000000000000000000, 0.9330127018922194093, 0.9330127018922194093 ) ) 
 REPRESENTATION_ITEM ( '' )  );
#37439=CARTESIAN_POINT ( 'NONE',  ( 163.0899802648238790, 283.6324727866974627, -3.105502518930082001 ) ) ;
#37440=CARTESIAN_POINT ( 'NONE',  ( 53.62548896571598078, 211.7677522451419350, -5.000000000000047962 ) ) ;
#37441=CARTESIAN_POINT ( 'NONE',  ( 208.3863431123642727, 269.7112614563416173, -1.693909372230378851 ) ) ;
#37442=CARTESIAN_POINT ( 'NONE',  ( 204.1953342137782954, 276.9703018036655067, 13.84727111424505885 ) ) ;
#37444=FACE_OUTER_BOUND ( 'NONE', #22787, .T. ) ;
#37445=CARTESIAN_POINT ( 'NONE',  ( 130.8910194135003735, 252.5024278399161233, 9.188101187500095079 ) ) ;
#37447=CARTESIAN_POINT ( 'NONE',  ( 176.9454523999648359, 269.2643027758560947, 16.09744801016948657 ) ) ;
#37448=CARTESIAN_POINT ( 'NONE',  ( 180.1735081377211429, 258.0673375898933841, 10.29486082622765686 ) ) ;
#37449=CARTESIAN_POINT ( 'NONE',  ( 68.48323730116675279, 210.3458772461660544, 9.188101187500095079 ) ) ;
#37451=CARTESIAN_POINT ( 'NONE',  ( 173.3416224425137671, 264.9983184062012356, 17.00855018129403007 ) ) ;
#37454=CARTESIAN_POINT ( 'NONE',  ( 160.6598419692975028, 254.0198957426222819, 15.58710629308137108 ) ) ;
#37459=CARTESIAN_POINT ( 'NONE',  ( 197.9023869102375386, 286.9431481333238594, 16.93429523346308230 ) ) ;
#37462=B_SPLINE_SURFACE_WITH_KNOTS ( 'NONE', 3, 1, ( 
 ( #18876, #17876 ),
 ( #32563, #72077 ),
 ( #40138, #8759 ),
 ( #87344, #34077 ),
 ( #57347, #95422 ),
 ( #62954, #47740 ),
 ( #95912, #93905 ),
 ( #48773, #2175 ),
 ( #79706, #41138 ),
 ( #86821, #10269 ),
 ( #3194, #33568 ),
 ( #9267, #39631 ),
 ( #64968, #25978 ),
 ( #9781, #56848 ),
 ( #71078, #49268 ),
 ( #26471, #55340 ),
 ( #80204, #40643 ),
 ( #32042, #78676 ),
 ( #33057, #10772 ),
 ( #88322, #70552 ),
 ( #1168, #86316 ),
 ( #16852, #60693 ),
 ( #73565, #45006 ),
 ( #91651, #11773 ),
 ( #75952, #4658 ),
 ( #4148, #21720 ),
 ( #73078, #42146 ),
 ( #52604, #6528 ),
 ( #36913, #65949 ),
 ( #61207, #76437 ),
 ( #96397, #98748 ),
 ( #67826, #7012 ),
 ( #53115, #35044 ),
 ( #30320, #42636 ) ),
 .UNSPECIFIED., .T., .F., .F.,
 ( 4, 2, 2, 2, 2, 2, 2, 2, 2, 2, 2, 2, 2, 2, 2, 2, 4 ),
 ( 2, 2 ),
 ( 0.000000000000000000, 0.06250000000000000000, 0.1250000000000000000, 0.1875000000000000000, 0.2500000000000000000, 0.3125000000000000000, 0.3750000000000000000, 0.4375000000000000000, 0.5000000000000000000, 0.5625000000000000000, 0.6250000000000000000, 0.6875000000000000000, 0.7500000000000000000, 0.8125000000000000000, 0.8750000000000000000, 0.9375000000000000000, 1.000000000000000000 ),
 ( 0.000000000000000000, 1.000000000000000000 ),
 .UNSPECIFIED. ) ;
#37465=B_SPLINE_CURVE_WITH_KNOTS ( 'NONE', 3,
 ( #38343, #67261, #6956, #36860, #37843, #61143 ),
 .UNSPECIFIED., .F., .F.,
 ( 4, 2, 4 ),
 ( 0.001016068118891022640, 0.001335860979828362455, 0.001655653840765702487 ),
 .UNSPECIFIED. ) ;
#37467=ADVANCED_FACE ( 'NONE', ( #75685 ), #63438, .F. ) ;
#37468=VERTEX_POINT ( 'NONE', #70050 ) ;
#37470=ORIENTED_EDGE ( 'NONE', *, *, #67208, .T. ) ;
#37471=CARTESIAN_POINT ( 'NONE',  ( 163.9330008582468849, 260.6526909249793107, -16.22567386398026912 ) ) ;
#37472=B_SPLINE_CURVE_WITH_KNOTS ( 'NONE', 3,
 ( #81930, #5885, #20601, #97616 ),
 .UNSPECIFIED., .F., .F.,
 ( 4, 4 ),
 ( 0.04352980446333042791, 0.04887066958154935581 ),
 .UNSPECIFIED. ) ;
#37473=CARTESIAN_POINT ( 'NONE',  ( 183.8084685968938459, 275.4580680932389782, 16.50770767648384663 ) ) ;
#37475=CARTESIAN_POINT ( 'NONE',  ( 195.2026777324871318, 279.1963207232482773, 16.32161989445632955 ) ) ;
#37476=CARTESIAN_POINT ( 'NONE',  ( 147.4771206202524354, 275.6046823160672830, -0.001107820683494442279 ) ) ;
#37477=CARTESIAN_POINT ( 'NONE',  ( 140.2550926398021147, 251.7833772461660544, -9.188101187500095079 ) ) ;
#37482=B_SPLINE_CURVE_WITH_KNOTS ( 'NONE', 3,
 ( #30748, #7951, #82988, #29746 ),
 .UNSPECIFIED., .F., .F.,
 ( 4, 4 ),
 ( 0.000000000000000000, 0.001018976964696252131 ),
 .UNSPECIFIED. ) ;
#37486=VERTEX_POINT ( 'NONE', #93911 ) ;
#37487=CARTESIAN_POINT ( 'NONE',  ( 197.0013005625082769, 266.0438005881301819, 4.442356137326111565 ) ) ;
#37489=CARTESIAN_POINT ( 'NONE',  ( 148.3780186227511138, 276.4204535841791994, -3.878789836482348985 ) ) ;
#37493=CARTESIAN_POINT ( 'NONE',  ( 198.0709943550380387, 266.0030824084365122, 0.8185462138619468142 ) ) ;
#37498=CARTESIAN_POINT ( 'NONE',  ( 186.6683070189575346, 282.4457408569519430, 16.24588814843900764 ) ) ;
#37499=CARTESIAN_POINT ( 'NONE',  ( 207.4826643481121664, 271.2764789897469768, 7.783310782367018454 ) ) ;
#37500=CARTESIAN_POINT ( 'NONE',  ( 177.8084161337914679, 264.6135516876653355, -15.81979285547498826 ) ) ;
#37502=EDGE_CURVE ( 'NONE', #76229, #18290, #30403, .T. ) ;
#37506=CARTESIAN_POINT ( 'NONE',  ( 205.4892939765805693, 274.2382912982014886, 10.85387586160992157 ) ) ;
#37508=CARTESIAN_POINT ( 'NONE',  ( 198.3150362131025588, 287.1552767044814800, 18.53472937702030521 ) ) ;
#37509=CARTESIAN_POINT ( 'NONE',  ( 192.7874605187217014, 292.5376213369709149, 15.36506066506490598 ) ) ;
#37510=CARTESIAN_POINT ( 'NONE',  ( -14.60124842228533915, 168.5024278399160949, 9.188101187500095079 ) ) ;
#37513=CARTESIAN_POINT ( 'NONE',  ( 178.4399924362400895, 256.1387041246245531, 8.807422250050599644 ) ) ;
#37515=CARTESIAN_POINT ( 'NONE',  ( 151.1230807375396807, 268.8941412966845519, -14.26613110909109849 ) ) ;
#37516=CARTESIAN_POINT ( 'NONE',  ( 10.97399815293012892, 167.9548013555409796, -4.594050593750042211 ) ) ;
#37518=CARTESIAN_POINT ( 'NONE',  ( 178.5166367657841135, 273.6876824058858801, -16.98119149330447897 ) ) ;
#37521=CARTESIAN_POINT ( 'NONE',  ( 170.7677701316179935, 271.1495265934172494, -17.63551025999282373 ) ) ;
#37523=DIRECTION ( 'NONE',  ( -0.8660254037844387076, -0.4999999999999998890, -0.000000000000000000 ) ) ;
#37524=CARTESIAN_POINT ( 'NONE',  ( 176.1144182152248447, 252.4374784436402308, -3.440074553853730066 ) ) ;
#37525=CARTESIAN_POINT ( 'NONE',  ( 150.7471914551857708, 269.5452006317422047, 15.29409085476701691 ) ) ;
#37526=CARTESIAN_POINT ( 'NONE',  ( 48.59171630976688760, 198.8615022471902591, -10.00000000000009592 ) ) ;
#37527=CARTESIAN_POINT ( 'NONE',  ( -22.42236680055709641, 157.8615022471902591, 0.000000000000000000 ) ) ;
#37528=CARTESIAN_POINT ( 'NONE',  ( 147.6207754342248961, 274.9603120256437592, 8.795690793376332195 ) ) ;
#37530=CARTESIAN_POINT ( 'NONE',  ( 17.98295739510416524, 187.3149278399160949, -9.188101187500095079 ) ) ;
#37532=ADVANCED_FACE ( 'NONE', ( #86827 ), #48067, .F. ) ;
#37533=CARTESIAN_POINT ( 'NONE',  ( 192.5049767439991513, 297.2185948999652965, 12.57567268027295881 ) ) ;
#37535=CARTESIAN_POINT ( 'NONE',  ( 201.1893450866852504, 280.1768276987904756, -16.82388990131531870 ) ) ;
#37536=DIRECTION ( 'NONE',  ( 0.4999999999999998890, -0.8660254037844385966, 0.000000000000000000 ) ) ;
#37537=CARTESIAN_POINT ( 'NONE',  ( 185.3440001858262178, 266.5832585216657549, 13.22870378338188324 ) ) ;
#37539=CARTESIAN_POINT ( 'NONE',  ( 153.5289410443318445, 265.1998938147651188, -16.31391090849110981 ) ) ;
#37542=CARTESIAN_POINT ( 'NONE',  ( 147.7157269441172218, 274.7958511862549926, 8.036290321896261801 ) ) ;
#37544=CARTESIAN_POINT ( 'NONE',  ( 155.4917600441137324, 261.3273667757233056, 17.14261720787171939 ) ) ;
#37546=CARTESIAN_POINT ( 'NONE',  ( 181.5361471459265204, 289.3569626564614055, 12.72074604773742834 ) ) ;
#37551=CARTESIAN_POINT ( 'NONE',  ( 149.0807665407234026, 276.4376266709116408, -5.539133476438467873 ) ) ;
#37553=CARTESIAN_POINT ( 'NONE',  ( 155.6048174803203210, 261.1315455520403361, -17.38645169541727498 ) ) ;
#37554=VERTEX_POINT ( 'NONE', #57352 ) ;
#37555=EDGE_LOOP ( 'NONE', ( #26140, #22294, #56408 ) ) ;
#37556=FACE_OUTER_BOUND ( 'NONE', #59245, .T. ) ;
#37557=CARTESIAN_POINT ( 'NONE',  ( 204.9427641582406636, 275.6757151647582305, 14.40446820030680897 ) ) ;
#37559=CARTESIAN_POINT ( 'NONE',  ( 191.4484954869714954, 299.0484741143815199, 8.684991747358081327 ) ) ;
#37564=CYLINDRICAL_SURFACE ( 'NONE', #32917, 17.82106496071139645 ) ;
#37566=CARTESIAN_POINT ( 'NONE',  ( 196.9431415128477170, 289.5314680279574304, -16.61413060656005669 ) ) ;
#37568=CARTESIAN_POINT ( 'NONE',  ( 206.4943150373521803, 272.9883502116088039, 11.34100825923693101 ) ) ;
#37571=CARTESIAN_POINT ( 'NONE',  ( 190.0445576990143195, 301.4801656937889902, 4.140328216824785912 ) ) ;
#37573=VERTEX_POINT ( 'NONE', #50745 ) ;
#37574=EDGE_CURVE ( 'NONE', #34618, #79381, #2094, .T. ) ;
#37580=EDGE_CURVE ( 'NONE', #32094, #34750, #42948, .T. ) ;
#37584=CARTESIAN_POINT ( 'NONE',  ( 190.2510882691990730, 301.1224442529128851, -5.480893437181090455 ) ) ;
#37585=CARTESIAN_POINT ( 'NONE',  ( 148.4049257185216106, 273.6021238924720365, 8.639190357831699529 ) ) ;
#37586=CARTESIAN_POINT ( 'NONE',  ( 190.4249800432324662, 300.8212548652687133, 3.085047376053959400 ) ) ;
#37587=CARTESIAN_POINT ( 'NONE',  ( 157.3797482626287092, 258.5641623508735165, -16.86146766721270396 ) ) ;
#37588=CARTESIAN_POINT ( 'NONE',  ( 147.1630655063547124, 275.7530888758436163, -0.6147864833414894425 ) ) ;
#37589=CARTESIAN_POINT ( 'NONE',  ( 191.5521510896938935, 298.8689373439769952, -9.847378829740700112 ) ) ;
#37590=CARTESIAN_POINT ( 'NONE',  ( 149.0323968763055689, 272.5153119669064949, 11.64231532207353403 ) ) ;
#37593=CARTESIAN_POINT ( 'NONE',  ( 196.4783028304046013, 290.3365922432724346, -16.37291435488387492 ) ) ;
#37596=CARTESIAN_POINT ( 'NONE',  ( 168.2319217786528327, 286.4071002536015840, 3.836160949525527997 ) ) ;
#37598=CARTESIAN_POINT ( 'NONE',  ( 102.5829875751790468, 230.0333772461660828, 9.188101187500095079 ) ) ;
#37600=CARTESIAN_POINT ( 'NONE',  ( 190.5599134601667117, 300.5875433314996030, -4.781267067655845082 ) ) ;
#37602=CARTESIAN_POINT ( 'NONE',  ( 203.0069541289995243, 278.2920787410731691, 14.98668837248997932 ) ) ;
#37604=CARTESIAN_POINT ( 'NONE',  ( 180.3507851124660135, 283.5217650176155075, -16.12320021977993534 ) ) ;
#37606=CARTESIAN_POINT ( 'NONE',  ( 169.2884693346459244, 285.2280652319857381, -7.815770310637231155 ) ) ;
#37608=CARTESIAN_POINT ( 'NONE',  ( 208.3226489551340990, 269.8215829728092103, -1.240262689467544366 ) ) ;
#37609=CARTESIAN_POINT ( 'NONE',  ( 206.8791291248445532, 272.3218326606039454, -10.16823074922856840 ) ) ;
#37612=CARTESIAN_POINT ( 'NONE',  ( 35.43895548624276159, 201.2677522451419350, -5.000000000000047962 ) ) ;
#37613=CARTESIAN_POINT ( 'NONE',  ( 108.2389556718223673, 242.4869531367911009, 4.594050593750046652 ) ) ;
#37616=DIRECTION ( 'NONE',  ( -0.8660254037844387076, -0.4999999999999998890, -0.000000000000000000 ) ) ;
#37617=CARTESIAN_POINT ( 'NONE',  ( 188.8544700204132880, 297.4231428397746413, 9.261439979758030461 ) ) ;
#37618=CARTESIAN_POINT ( 'NONE',  ( 175.4498787482802982, 253.5586827773643108, -4.041159264954998775 ) ) ;
#37619=CARTESIAN_POINT ( 'NONE',  ( 35.46636587765004123, 179.0327760586659736, 1.948934522072303157E-15 ) ) ;
#37621=ORIENTED_EDGE ( 'NONE', *, *, #57053, .F. ) ;
#37622=CARTESIAN_POINT ( 'NONE',  ( 181.2305971022323661, 265.9781236237157032, -15.82518789413146010 ) ) ;
#37623=CARTESIAN_POINT ( 'NONE',  ( 181.9045674196421203, 266.8808357545214562, 15.69428031596684114 ) ) ;
#37625=CARTESIAN_POINT ( 'NONE',  ( 16.54877636974260824, 190.3615022471903160, 5.000000000000046185 ) ) ;
#37627=CARTESIAN_POINT ( 'NONE',  ( 106.1564052266985101, 220.5494855054051584, -2.679491924311248496 ) ) ;
#37630=CARTESIAN_POINT ( 'NONE',  ( 106.9582200821076299, 245.8927522451419350, 2.944929066748280225E-16 ) ) ;
#37632=CARTESIAN_POINT ( 'NONE',  ( 207.8570869662935365, 270.6279599915536664, -5.669188455878507504 ) ) ;
#37633=CARTESIAN_POINT ( 'NONE',  ( 155.4352814124438282, 279.7207056978571131, -1.858304131775387003 ) ) ;
#37634=CARTESIAN_POINT ( 'NONE',  ( 154.3624839403327371, 263.9877490788467185, 16.80989463870938749 ) ) ;
#37635=ADVANCED_FACE ( 'NONE', ( #4663 ), #64276, .F. ) ;
#37636=CARTESIAN_POINT ( 'NONE',  ( 8.781437479894508513, 182.0024278399160949, 9.188101187500095079 ) ) ;
#37638=CARTESIAN_POINT ( 'NONE',  ( 192.5718708460708797, 272.1165744649917428, 14.18846852481804888 ) ) ;
#37640=CARTESIAN_POINT ( 'NONE',  ( 182.3667867738580242, 280.0318728379381241, 17.49684858827472667 ) ) ;
#37641=CARTESIAN_POINT ( 'NONE',  ( 194.7293364455423728, 275.0050812418281225, -15.92559422164948479 ) ) ;
#37642=CARTESIAN_POINT ( 'NONE',  ( 58.14488549560751807, 210.5024278399160949, 9.188101187500095079 ) ) ;
#37643=CARTESIAN_POINT ( 'NONE',  ( 197.4517085639775189, 281.7586087989938051, 17.62726178258972354 ) ) ;
#37648=B_SPLINE_CURVE_WITH_KNOTS ( 'NONE', 3,
 ( #3210, #64483, #49285, #63972, #72608, #95443, #79230, #80733, #47758, #64985, #62975, #25995, #49776, #56866, #95929, #55846, #87367, #48794, #9803, #87850, #70570, #1188, #93923, #40663, #79725, #2196, #33079, #94915, #25478, #10287, #41159, #96921, #66468, #97884, #65473, #28457, #26982, #65969, #42165, #21368, #58358, #5662, #13286, #90815, #58840, #36550 ),
 .UNSPECIFIED., .F., .F.,
 ( 4, 2, 2, 2, 2, 2, 2, 2, 2, 2, 2, 2, 2, 2, 2, 2, 2, 2, 2, 2, 2, 2, 4 ),
 ( 0.0003494839938075159236, 0.001366047292800560932, 0.001874328942297083652, 0.002001399354671171398, 0.002128469767045259361, 0.002255540179419347323, 0.002382610591793435720, 0.002636751416541610778, 0.002890892241289786703, 0.003399173890786319832, 0.004415737189779446806, 0.005432300488772573779, 0.005940582138269217063, 0.006194722963017495337, 0.006448863787765774479, 0.006512398993952864430, 0.006575934200139955249, 0.006639469406327046068, 0.006703004612514136019, 0.006957145437262477611, 0.007465427086759236254, 0.007973708736255996632, 0.008481990385752756142 ),
 .UNSPECIFIED. ) ;
#37649=CARTESIAN_POINT ( 'NONE',  ( 165.4619875320036329, 269.3508363939868673, 17.22119345129141266 ) ) ;
#37650=CARTESIAN_POINT ( 'NONE',  ( 6.156471524329347744, 184.3615022471903160, 5.000000000000046185 ) ) ;
#37651=CARTESIAN_POINT ( 'NONE',  ( 164.4405316900629259, 245.8276396196081350, -6.144538123479245328 ) ) ;
#37652=CARTESIAN_POINT ( 'NONE',  ( 133.0017827873424494, 259.8464784336661637, 1.353441290958777327E-15 ) ) ;
#37654=CARTESIAN_POINT ( 'NONE',  ( 206.7978835355532112, 272.4625541491475929, -7.782039308735489769 ) ) ;
#37657=CARTESIAN_POINT ( 'NONE',  ( 156.9694903541507074, 266.1758412851487492, -17.34135443527054576 ) ) ;
#37658=CARTESIAN_POINT ( 'NONE',  ( 175.7882114856885210, 291.4026636951798537, -6.622811550496607857 ) ) ;
#37660=EDGE_LOOP ( 'NONE', ( #96672, #9930, #90382 ) ) ;
#37662=CARTESIAN_POINT ( 'NONE',  ( 164.1353833742626591, 246.3561720064182339, 8.180808313729997394 ) ) ;
#37663=CARTESIAN_POINT ( 'NONE',  ( 151.6586017097065167, 268.5374266604292757, -14.66497191532962141 ) ) ;
#37665=CARTESIAN_POINT ( 'NONE',  ( 156.4703069145093650, 280.4439178849370364, -5.466162413456765456 ) ) ;
#37666=CARTESIAN_POINT ( 'NONE',  ( 197.2297097385163056, 273.4493452446096171, -13.71841916057935507 ) ) ;
#37668=FACE_OUTER_BOUND ( 'NONE', #52513, .T. ) ;
#37671=B_SPLINE_CURVE_WITH_KNOTS ( 'NONE', 3,
 ( #90825, #13770, #28467, #82727, #29472, #90325, #92310, #74610, #98891, #13299, #51788, #66964, #59348, #44157, #14764, #28986, #45646, #75583 ),
 .UNSPECIFIED., .F., .F.,
 ( 4, 2, 2, 2, 2, 2, 2, 2, 4 ),
 ( 7.954564953275306146E-05, 0.0004482884113075860004, 0.0008170311730824190207, 0.001185773934857251933, 0.001554516696632084844, 0.001923259458406917756, 0.002292002220181750885, 0.002660744981956583797, 0.003029487743731416709 ),
 .UNSPECIFIED. ) ;
#37672=CARTESIAN_POINT ( 'NONE',  ( 148.7588072053147243, 273.7711778218048835, -8.803803025135483296 ) ) ;
#37673=CARTESIAN_POINT ( 'NONE',  ( 21.74492879244924382, 193.3615022471903160, 5.000000000000046185 ) ) ;
#37675=CARTESIAN_POINT ( 'NONE',  ( 163.3723087697842971, 247.6778559913402091, -10.08585062664141319 ) ) ;
#37676=CARTESIAN_POINT ( 'NONE',  ( 152.8721808860877616, 265.8646109718731623, -17.65676496037632504 ) ) ;
#37677=CARTESIAN_POINT ( 'NONE',  ( 190.4940751089258129, 281.5363301538920950, 17.17439451701960706 ) ) ;
#37681=CYLINDRICAL_SURFACE ( 'NONE', #99783, 17.82106496071139645 ) ;
#37687=CIRCLE ( 'NONE', #99649, 17.82106496071138224 ) ;
#37688=AXIS2_PLACEMENT_3D ( 'NONE', #96160, #80470, #65705 ) ;
#37689=CARTESIAN_POINT ( 'NONE',  ( 204.9432097630379417, 275.6749433546094679, 13.74700047688257776 ) ) ;
#37692=CARTESIAN_POINT ( 'NONE',  ( 94.51795245455393513, 231.5024278399160949, 9.188101187500095079 ) ) ;
#37693=CARTESIAN_POINT ( 'NONE',  ( 185.2391986358457530, 295.7873944733689768, 8.585680893828113724 ) ) ;
#37694=CARTESIAN_POINT ( 'NONE',  ( 181.3482518238504611, 271.2696307585432578, -15.99940275358306607 ) ) ;
#37697=VERTEX_POINT ( 'NONE', #5648 ) ;
#37698=ORIENTED_EDGE ( 'NONE', *, *, #4972, .F. ) ;
#37700=VERTEX_POINT ( 'NONE', #59839 ) ;
#37702=ORIENTED_EDGE ( 'NONE', *, *, #91127, .T. ) ;
#37705=ORIENTED_EDGE ( 'NONE', *, *, #67390, .F. ) ;
#37706=CARTESIAN_POINT ( 'NONE',  ( 163.9910908123517288, 246.6060940548019289, -7.333295033952830444 ) ) ;
#37707=EDGE_CURVE ( 'NONE', #11091, #72615, #9069, .T. ) ;
#37708=CARTESIAN_POINT ( 'NONE',  ( 169.8557297738865941, 282.3553244834201337, 11.74113619686330701 ) ) ;
#37714=CARTESIAN_POINT ( 'NONE',  ( 198.8280325239424258, 277.6560935625093975, -15.37151893818075266 ) ) ;
#37718=CARTESIAN_POINT ( 'NONE',  ( 163.2835940097493790, 247.8315144631017404, 11.08416305054517359 ) ) ;
#37719=CARTESIAN_POINT ( 'NONE',  ( 187.7204020327498313, 260.5175946176191815, 2.856882547745535739 ) ) ;
#37721=B_SPLINE_CURVE_WITH_KNOTS ( 'NONE', 3,
 ( #84264, #45210, #76622, #29038, #21915, #21428, #38091, #91353, #59909, #60397, #13821, #68017, #44701, #75632, #37114, #83762 ),
 .UNSPECIFIED., .F., .F.,
 ( 4, 2, 2, 2, 2, 2, 2, 4 ),
 ( 0.0005218454421851866348, 0.0008352828619746982325, 0.001148720281764209830, 0.001462157701553721319, 0.001775595121343233026, 0.002089032541132744732, 0.002402469960922256221, 0.003029344800501365502 ),
 .UNSPECIFIED. ) ;
#37722=CARTESIAN_POINT ( 'NONE',  ( -27.42236680055714260, 166.5217562850347406, 1.224646799147364892E-15 ) ) ;
#37723=CARTESIAN_POINT ( 'NONE',  ( 172.0399293152837572, 254.5145317268123790, 11.42224199934888418 ) ) ;
#37724=CARTESIAN_POINT ( 'NONE',  ( 160.6911010070541863, 282.7964184354547683, 2.101448972218037614 ) ) ;
#37725=( BOUNDED_CURVE ( )  B_SPLINE_CURVE ( 2, ( #77726, #17402, #79257, #69602, #47295, #23486, #15897, #53709, #23314 ),
 .UNSPECIFIED., .F., .T. ) 
 B_SPLINE_CURVE_WITH_KNOTS ( ( 3, 2, 2, 2, 3 ),
 ( 0.9072580645161290036, 0.9086021505376343788, 0.9112903225806451291, 0.9139784946236558794, 0.9153225806451612545 ),
 .UNSPECIFIED. ) 
 CURVE ( )  GEOMETRIC_REPRESENTATION_ITEM ( )  RATIONAL_B_SPLINE_CURVE ( ( 0.9330127018922194093, 0.9330127018922194093, 1.000000000000000000, 0.8660254037844387076, 1.000000000000000000, 0.8660254037844387076, 1.000000000000000000, 0.9330127018922194093, 0.9330127018922194093 ) ) 
 REPRESENTATION_ITEM ( '' )  );
#37727=CARTESIAN_POINT ( 'NONE',  ( 194.6224351033329185, 293.5510494386875848, -14.91730472411656550 ) ) ;
#37730=CARTESIAN_POINT ( 'NONE',  ( 0.3649266329730349034, 171.0177522451418781, -10.00000000000009592 ) ) ;
#37731=CARTESIAN_POINT ( 'NONE',  ( 196.1039637098642459, 269.4745711467500087, -10.81934472805613545 ) ) ;
#37732=B_SPLINE_CURVE_WITH_KNOTS ( 'NONE', 3,
 ( #78032, #87698, #55689, #2540 ),
 .UNSPECIFIED., .F., .F.,
 ( 4, 4 ),
 ( 0.02958148137093116747, 0.03870913465764597161 ),
 .UNSPECIFIED. ) ;
#37733=CARTESIAN_POINT ( 'NONE',  ( 175.0403197011952159, 281.5117084114038448, -14.13282399009272261 ) ) ;
#37734=CARTESIAN_POINT ( 'NONE',  ( 163.5122523041594036, 247.4354666796116078, -8.835398473100831040 ) ) ;
#37737=CARTESIAN_POINT ( 'NONE',  ( -16.46870247313679059, 170.4869531367911293, 4.594050593750046652 ) ) ;
#37740=CARTESIAN_POINT ( 'NONE',  ( 189.0934591145252170, 297.0081427490579813, 8.814819132589450490 ) ) ;
#37741=ORIENTED_EDGE ( 'NONE', *, *, #51316, .F. ) ;
#37742=EDGE_LOOP ( 'NONE', ( #78369, #27002, #47571, #26780, #93200 ) ) ;
#37747=FACE_OUTER_BOUND ( 'NONE', #73209, .T. ) ;
#37749=CARTESIAN_POINT ( 'NONE',  ( 162.7089540403458159, 248.8268200861687376, -11.78833136687426553 ) ) ;
#37751=CARTESIAN_POINT ( 'NONE',  ( 153.6085985088494681, 279.1348322646095994, 3.818864634155017423 ) ) ;
#37752=CARTESIAN_POINT ( 'NONE',  ( 23.85612603422365297, 175.3923013555409796, 4.594050593750050204 ) ) ;
#37754=CARTESIAN_POINT ( 'NONE',  ( 111.5137010038235417, 241.3149278399161233, -9.188101187500095079 ) ) ;
#37755=CARTESIAN_POINT ( 'NONE',  ( 179.3642964896383205, 292.0887335915682002, -6.148695452510337667 ) ) ;
#37756=CARTESIAN_POINT ( 'NONE',  ( 168.7310635674097341, 283.4413295356843037, 12.00249716675341638 ) ) ;
#37757=CARTESIAN_POINT ( 'NONE',  ( 206.6750745834628731, 271.7034134901589368, -6.697661943153482511 ) ) ;
#37760=EDGE_CURVE ( 'NONE', #15004, #75836, #77976, .T. ) ;
#37761=CARTESIAN_POINT ( 'NONE',  ( 60.85032556585977659, 217.4860189848785410, -2.679491924311252493 ) ) ;
#37762=CARTESIAN_POINT ( 'NONE',  ( 195.7291534503633272, 291.6341570319625021, 16.44925029361851543 ) ) ;
#37763=CYLINDRICAL_SURFACE ( 'NONE', #51779, 10.00000000000010658 ) ;
#37764=CARTESIAN_POINT ( 'NONE',  ( 161.8882824960653579, 250.2482648971885340, -13.83574485983625557 ) ) ;
#37767=CARTESIAN_POINT ( 'NONE',  ( 196.4319357531070693, 266.2480072935647399, 8.325861693847476985 ) ) ;
#37772=CARTESIAN_POINT ( 'NONE',  ( -22.42236680055709641, 157.8615022471902591, 0.000000000000000000 ) ) ;
#37773=CARTESIAN_POINT ( 'NONE',  ( 181.5320323368239315, 267.9553237911030692, 15.00661790592713452 ) ) ;
#37775=CARTESIAN_POINT ( 'NONE',  ( 97.73839765093606502, 236.4244531367911009, -4.594050593750046652 ) ) ;
#37776=CARTESIAN_POINT ( 'NONE',  ( 161.8153478334749877, 250.3745914384277285, -14.21120979595050215 ) ) ;
#37777=CARTESIAN_POINT ( 'NONE',  ( 191.3638605175971747, 299.1950661814348678, 7.382965314423603154 ) ) ;
#37779=CARTESIAN_POINT ( 'NONE',  ( 145.0115229932138163, 242.9824982072973683, 3.021315404115420679E-15 ) ) ;
#37780=CARTESIAN_POINT ( 'NONE',  ( 194.0373140624720349, 278.4935463477126518, 16.30235809050098794 ) ) ;
#37781=CARTESIAN_POINT ( 'NONE',  ( 201.1568026402725877, 270.4843927660949134, -10.02948014338874039 ) ) ;
#37782=CARTESIAN_POINT ( 'NONE',  ( 198.4782858197754649, 286.8725200914082620, -17.44895083299520522 ) ) ;
#37786=CYLINDRICAL_SURFACE ( 'NONE', #44263, 17.82106496071139645 ) ;
#37790=CARTESIAN_POINT ( 'NONE',  ( 147.5118896528469179, 275.1489077312122049, -3.975523961781759930 ) ) ;
#37791=CARTESIAN_POINT ( 'NONE',  ( 196.8435556370661459, 289.7039558245273838, -16.43899056939217118 ) ) ;
#37792=VERTEX_POINT ( 'NONE', #9146 ) ;
#37794=CARTESIAN_POINT ( 'NONE',  ( 198.4264492142971221, 286.9623037257889564, 17.00126466006521397 ) ) ;
#37795=CARTESIAN_POINT ( 'NONE',  ( 180.3364889203162988, 263.1152589884272857, -12.84555436964710218 ) ) ;
#37796=CARTESIAN_POINT ( 'NONE',  ( 169.4616969408077978, 252.2111926658335221, -8.760020798663340713 ) ) ;
#37797=CARTESIAN_POINT ( 'NONE',  ( 152.8107382695299918, 265.9710327055011589, 16.32045346488711246 ) ) ;
#37802=CARTESIAN_POINT ( 'NONE',  ( 164.7636693376427388, 247.7456902508657492, 7.156984819320836522 ) ) ;
#37803=CARTESIAN_POINT ( 'NONE',  ( 184.9534712104859011, 293.2739629945884872, -10.43194920464371300 ) ) ;
#37806=CARTESIAN_POINT ( 'NONE',  ( 158.9588665712855118, 256.6514483001959661, 16.71440725461184940 ) ) ;
#37807=CARTESIAN_POINT ( 'NONE',  ( 190.5140674548521531, 278.6669388570777528, -16.50821822264429173 ) ) ;
#37808=CARTESIAN_POINT ( 'NONE',  ( 153.8198515416281964, 264.2231972476349711, -16.55097973663693978 ) ) ;
#37809=CARTESIAN_POINT ( 'NONE',  ( 200.7134601498536028, 283.0010845879393742, -16.98649239173277792 ) ) ;
#37812=CARTESIAN_POINT ( 'NONE',  ( 193.0126352936363503, 264.4189281174865869, 8.906082567666748773 ) ) ;
#37815=ORIENTED_EDGE ( 'NONE', *, *, #84417, .T. ) ;
#37816=CARTESIAN_POINT ( 'NONE',  ( 45.37789370152431445, 208.5530062829863027, -4.648177544792955347E-16 ) ) ;
#37817=VERTEX_POINT ( 'NONE', #17232 ) ;
#37820=CARTESIAN_POINT ( 'NONE',  ( 198.1516807435644409, 286.9647030927445144, 16.94921385266723490 ) ) ;
#37822=CARTESIAN_POINT ( 'NONE',  ( 174.3740210016665628, 256.9530918469817493, -12.27374415811068076 ) ) ;
#37823=CARTESIAN_POINT ( 'NONE',  ( 190.1235086622576773, 300.2499232672161043, -3.363423802915200156 ) ) ;
#37824=DIRECTION ( 'NONE',  ( -0.8660254037844387076, -0.4999999999999998890, -0.000000000000000000 ) ) ;
#37825=CARTESIAN_POINT ( 'NONE',  ( 197.8058269970693743, 272.4609363502503356, -13.32996429882288147 ) ) ;
#37827=CARTESIAN_POINT ( 'NONE',  ( 203.4776550330608416, 276.3243839139203715, 14.43342264677212405 ) ) ;
#37829=CARTESIAN_POINT ( 'NONE',  ( 168.2008345946905479, 248.1884056956802453, -5.064766917302788052 ) ) ;
#37830=ADVANCED_FACE ( 'NONE', ( #70960 ), #1561, .T. ) ;
#37833=CARTESIAN_POINT ( 'NONE',  ( 186.8266632922035910, 287.0577513604794149, -15.74549898466382203 ) ) ;
#37834=CARTESIAN_POINT ( 'NONE',  ( 106.3175485811169239, 238.3149278399160949, -9.188101187500095079 ) ) ;
#37838=CARTESIAN_POINT ( 'NONE',  ( 188.2014231658550898, 273.5110677970230313, 15.67131877287846287 ) ) ;
#37842=CARTESIAN_POINT ( 'NONE',  ( 198.2505066714982149, 285.2670451491296149, 0.000000000000000000 ) ) ;
#37843=CARTESIAN_POINT ( 'NONE',  ( 190.4495984692767649, 300.3985526752458668, -0.4774468551831849705 ) ) ;
#37844=CARTESIAN_POINT ( 'NONE',  ( 193.8698296682186992, 271.7227521665574841, -15.05645239061159479 ) ) ;
#37846=CARTESIAN_POINT ( 'NONE',  ( 195.4428138874578167, 292.1301117031320587, 15.46566957515385710 ) ) ;
#37847=ORIENTED_EDGE ( 'NONE', *, *, #95033, .T. ) ;
#37850=CARTESIAN_POINT ( 'NONE',  ( 190.8936203498974464, 267.5824989483721197, -12.06459381115725904 ) ) ;
#37851=CARTESIAN_POINT ( 'NONE',  ( 192.3722320044300034, 262.8214543474982179, 4.572296880953776288 ) ) ;
#37853=CARTESIAN_POINT ( 'NONE',  ( 6.406750531224583156, 186.0530062829863027, -4.648177544792955347E-16 ) ) ;
#37854=CARTESIAN_POINT ( 'NONE',  ( 184.2746014452833379, 288.7589902912345678, -13.23859099789902594 ) ) ;
#37855=CARTESIAN_POINT ( 'NONE',  ( 160.5389806683030827, 281.4356532093604528, 5.616753171805936695 ) ) ;
#37856=CARTESIAN_POINT ( 'NONE',  ( 197.4075646047015482, 273.1427705089788560, -14.69744958829762815 ) ) ;
#37858=CARTESIAN_POINT ( 'NONE',  ( 147.1249913145849177, 275.8190353104462815, 3.637773609013635223 ) ) ;
#37860=CARTESIAN_POINT ( 'NONE',  ( 190.5337456798271205, 263.9425320260396575, -9.625448268029721532 ) ) ;
#37861=CARTESIAN_POINT ( 'NONE',  ( 173.5418303646803793, 251.2005048794018194, -1.013737780652142151 ) ) ;
#37862=CARTESIAN_POINT ( 'NONE',  ( 163.2308556539849178, 280.6958281187306170, -11.57967609262591502 ) ) ;
#37866=CARTESIAN_POINT ( 'NONE',  ( 194.4165969972361552, 293.9075714965812267, 14.23342188338008718 ) ) ;
#37867=CARTESIAN_POINT ( 'NONE',  ( 191.4282566499900895, 282.7875431929116417, -17.14954741723730436 ) ) ;
#37869=CARTESIAN_POINT ( 'NONE',  ( 81.47361835793333285, 217.8458772461660544, 9.188101187500095079 ) ) ;
#37871=CARTESIAN_POINT ( 'NONE',  ( 147.5381343315788172, 275.1034506142203782, -4.056595942992749393 ) ) ;
#37873=ADVANCED_FACE ( 'NONE', ( #85182 ), #15729, .T. ) ;
#37874=CARTESIAN_POINT ( 'NONE',  ( 161.1232569692349443, 251.5733279787459367, -14.02750397520710557 ) ) ;
#37878=CARTESIAN_POINT ( 'NONE',  ( 193.8626392119275010, 262.2145712166342264, 1.470488869930418607 ) ) ;
#37880=CARTESIAN_POINT ( 'NONE',  ( 157.3305006125302441, 282.1378183958786963, 1.589776369934247979 ) ) ;
#37881=CARTESIAN_POINT ( 'NONE',  ( 157.5520850189458884, 257.7587792392113215, 16.71892742266126319 ) ) ;
#37883=VECTOR ( 'NONE', #62166, 1000.000000000000000 ) ;
#37884=CARTESIAN_POINT ( 'NONE',  ( 31.13589176296283156, 188.7833772461660544, -9.188101187500095079 ) ) ;
#37886=CARTESIAN_POINT ( 'NONE',  ( 56.57573509489573382, 191.2202760586659736, -5.415160957724236172E-17 ) ) ;
#37887=CARTESIAN_POINT ( 'NONE',  ( 196.4677102463732012, 290.3549391369982686, 16.45225250689336249 ) ) ;
#37891=CARTESIAN_POINT ( 'NONE',  ( -11.23620533500811725, 170.9865022471903444, -10.00000000000009415 ) ) ;
#37892=CARTESIAN_POINT ( 'NONE',  ( 57.73936995728981714, 194.9548013555410080, -4.594050593750042211 ) ) ;
#37894=CARTESIAN_POINT ( 'NONE',  ( 150.6626254231123880, 269.6916732958875969, -15.32062296289003811 ) ) ;
#37895=CARTESIAN_POINT ( 'NONE',  ( 196.8435556370661459, 289.7039558245273838, -16.43899056939217118 ) ) ;
#37899=CARTESIAN_POINT ( 'NONE',  ( 175.6477625036710606, 291.0204324385146037, 2.451421089737829906 ) ) ;
#37900=CARTESIAN_POINT ( 'NONE',  ( 159.4889735931715222, 254.4039898200529706, 16.88104032092801887 ) ) ;
#37902=CARTESIAN_POINT ( 'NONE',  ( 201.3272413420560554, 281.9379843783140700, 16.84531592925761601 ) ) ;
#37903=EDGE_CURVE ( 'NONE', #93443, #57499, #44223, .T. ) ;
#37904=DIRECTION ( 'NONE',  ( 0.5000000000000048850, -0.8660254037844358210, 0.000000000000000000 ) ) ;
#37905=CARTESIAN_POINT ( 'NONE',  ( 109.6465072765697641, 244.1115022471903160, -5.000000000000047962 ) ) ;
#37906=CARTESIAN_POINT ( 'NONE',  ( 161.8289209813647176, 250.3510820566641257, 13.28523796267037937 ) ) ;
#37907=CARTESIAN_POINT ( 'NONE',  ( 194.0058304551163531, 285.1060772508486707, -16.99837373451835631 ) ) ;
#37908=EDGE_LOOP ( 'NONE', ( #24816, #47423, #2860 ) ) ;
#37912=CARTESIAN_POINT ( 'NONE',  ( 194.1883405663843689, 293.5167174303800834, 14.56505799480749452 ) ) ;
#37913=DIRECTION ( 'NONE',  ( -0.8660254037844387076, -0.4999999999999998890, -0.000000000000000000 ) ) ;
#37915=CARTESIAN_POINT ( 'NONE',  ( 157.4068442735347446, 281.9945091197541274, 2.874377194828706905 ) ) ;
#37916=CARTESIAN_POINT ( 'NONE',  ( 207.6727254509676186, 270.9472835030587703, 7.315149605389819953 ) ) ;
#37917=CARTESIAN_POINT ( 'NONE',  ( 148.1004780136491377, 274.1294427855589788, -7.811560775291159331 ) ) ;
#37924=EDGE_CURVE ( 'NONE', #70463, #56261, #19757, .T. ) ;
#37927=CARTESIAN_POINT ( 'NONE',  ( 159.2122473525774069, 254.8832937285494609, -16.22689353966294590 ) ) ;
#37929=EDGE_CURVE ( 'NONE', #20151, #734, #97366, .T. ) ;
#37930=CARTESIAN_POINT ( 'NONE',  ( 174.6916540630883503, 286.2244833470182925, 10.52363204570947275 ) ) ;
#37931=CARTESIAN_POINT ( 'NONE',  ( 162.5729093422976916, 283.3574902375370925, -3.116333471781629783 ) ) ;
#37933=CARTESIAN_POINT ( 'NONE',  ( 207.8136982414359579, 270.7031114674828700, -0.9536989003868096004 ) ) ;
#37934=CARTESIAN_POINT ( 'NONE',  ( 164.4936379324916516, 245.7356569095223051, 6.719479797016231437 ) ) ;
#37936=CARTESIAN_POINT ( 'NONE',  ( 179.2728639618759985, 293.8282488962061620, 5.658163206248635113 ) ) ;
#37937=CARTESIAN_POINT ( 'NONE',  ( 133.7599021114188247, 248.0333772461660544, 9.188101187500095079 ) ) ;
#37939=CARTESIAN_POINT ( 'NONE',  ( 177.2759083163978744, 269.2989204424369518, 16.08029799372871338 ) ) ;
#37940=CARTESIAN_POINT ( 'NONE',  ( 181.9605180691946771, 260.3799461757151334, 9.466307468308277961 ) ) ;
#37941=CARTESIAN_POINT ( 'NONE',  ( 75.92590343676303632, 205.4548013555409796, -4.594050593750042211 ) ) ;
#37943=CARTESIAN_POINT ( 'NONE',  ( 171.2741013746033332, 249.3936815359432728, 2.927055546763141169 ) ) ;
#37944=FACE_OUTER_BOUND ( 'NONE', #70121, .T. ) ;
#37945=CARTESIAN_POINT ( 'NONE',  ( 189.4199209167946663, 300.3895034224956930, 3.306026617473488027 ) ) ;
#37947=CARTESIAN_POINT ( 'NONE',  ( 161.3383531994606699, 252.8394435820131605, 14.78188028638097506 ) ) ;
#37954=CARTESIAN_POINT ( 'NONE',  ( 194.1604701155857526, 284.7193346175499187, 17.50795125310741795 ) ) ;
#37957=CARTESIAN_POINT ( 'NONE',  ( 194.4263876777154394, 293.8906135405502482, 15.23185943445137802 ) ) ;
#37962=B_SPLINE_SURFACE_WITH_KNOTS ( 'NONE', 3, 1, ( 
 ( #38164, #21504 ),
 ( #5796, #69084 ),
 ( #76217, #30594 ),
 ( #83333, #37675 ),
 ( #99509, #99012 ),
 ( #52886, #100009 ),
 ( #83836, #14402 ),
 ( #6794, #68586 ),
 ( #51394, #36185 ),
 ( #60975, #67090 ),
 ( #91939, #77185 ),
 ( #93428, #22977 ),
 ( #53866, #84827 ),
 ( #46789, #190 ),
 ( #1708, #23981 ),
 ( #46264, #1195 ),
 ( #15366, #39160 ),
 ( #47278, #62462 ),
 ( #54878, #32589 ),
 ( #79241, #8294 ),
 ( #31075, #94425 ),
 ( #40674, #2207 ),
 ( #31570, #92429 ),
 ( #70073, #69582 ),
 ( #61963, #688 ),
 ( #16881, #7792 ),
 ( #61480, #85859 ),
 ( #38678, #16385 ),
 ( #63487, #24979 ),
 ( #78201, #92916 ),
 ( #23469, #86348 ),
 ( #54360, #8788 ),
 ( #32073, #15876 ),
 ( #62986, #93930 ) ),
 .UNSPECIFIED., .T., .F., .F.,
 ( 4, 2, 2, 2, 2, 2, 2, 2, 2, 2, 2, 2, 2, 2, 2, 2, 4 ),
 ( 2, 2 ),
 ( 0.000000000000000000, 0.06250000000000000000, 0.1250000000000000000, 0.1875000000000000000, 0.2500000000000000000, 0.3125000000000000000, 0.3750000000000000000, 0.4375000000000000000, 0.5000000000000000000, 0.5625000000000000000, 0.6250000000000000000, 0.6875000000000000000, 0.7500000000000000000, 0.8125000000000000000, 0.8750000000000000000, 0.9375000000000000000, 1.000000000000000000 ),
 ( 0.000000000000000000, 1.000000000000000000 ),
 .UNSPECIFIED. ) ;
#37968=CARTESIAN_POINT ( 'NONE',  ( 194.9160431658341395, 279.6352213503219559, 17.41133371011275699 ) ) ;
#37969=CARTESIAN_POINT ( 'NONE',  ( 162.9383048163760463, 261.5404076612216500, 17.29887017337560096 ) ) ;
#37970=CARTESIAN_POINT ( 'NONE',  ( 133.7599021114188247, 248.0333772461660544, 9.188101187500095079 ) ) ;
#37971=ORIENTED_EDGE ( 'NONE', *, *, #38134, .T. ) ;
#37975=CARTESIAN_POINT ( 'NONE',  ( 152.8328714238065515, 265.9326969577624027, -16.29536156676786263 ) ) ;
#37978=EDGE_LOOP ( 'NONE', ( #47533, #53072, #16677, #28726 ) ) ;
#37979=CARTESIAN_POINT ( 'NONE',  ( 199.4197156453936373, 266.8589959824688549, 4.580656179805971284 ) ) ;
#37980=CARTESIAN_POINT ( 'NONE',  ( 76.67083364154854053, 226.6199935810941213, 2.679491924311251605 ) ) ;
#37984=CARTESIAN_POINT ( 'NONE',  ( 196.5499765897077964, 265.0522732887451411, 0.8242394764280709385 ) ) ;
#37987=CARTESIAN_POINT ( 'NONE',  ( 183.0648203791300546, 280.6896956899441875, 16.60862611305853775 ) ) ;
#37990=CARTESIAN_POINT ( 'NONE',  ( 206.9676408587583296, 272.1685258403992975, 7.544050792475608169 ) ) ;
#37992=CARTESIAN_POINT ( 'NONE',  ( 196.8989084261116886, 269.7173827915191850, 12.31991664540137954 ) ) ;
#37993=EDGE_CURVE ( 'NONE', #39719, #54166, #26129, .T. ) ;
#37995=CARTESIAN_POINT ( 'NONE',  ( 28.09809348231459936, 175.4824982072973967, 3.021315404115420679E-15 ) ) ;
#37996=CARTESIAN_POINT ( 'NONE',  ( 164.8705138155180521, 286.2009910768602481, -3.373684704351256780 ) ) ;
#37999=CARTESIAN_POINT ( 'NONE',  ( -12.86919761471646773, 169.5024278399161233, -9.188101187500093303 ) ) ;
#38000=CARTESIAN_POINT ( 'NONE',  ( 75.63696797857046761, 221.1427522451419065, -10.00000000000009592 ) ) ;
#38002=EDGE_CURVE ( 'NONE', #68704, #73023, #46546, .T. ) ;
#38006=CARTESIAN_POINT ( 'NONE',  ( 16.17015057563676450, 170.9548013555409796, -4.594050593750042211 ) ) ;
#38009=CARTESIAN_POINT ( 'NONE',  ( 171.6054817282545741, 271.5228642886609123, -16.51620184496720611 ) ) ;
#38010=CARTESIAN_POINT ( 'NONE',  ( 150.1413706805870731, 276.5095333114461482, 3.755964711348897200 ) ) ;
#38011=CARTESIAN_POINT ( 'NONE',  ( 179.3677837486497992, 255.1410135168996192, -4.004816050580029874 ) ) ;
#38013=CARTESIAN_POINT ( 'NONE',  ( 189.4592384298869376, 261.1887071297708758, -0.7541892224000766864 ) ) ;
#38016=CARTESIAN_POINT ( 'NONE',  ( 183.0125666146673780, 295.6744899775687827, 1.024979532612127819 ) ) ;
#38017=CARTESIAN_POINT ( 'NONE',  ( 52.48883062679684741, 201.1115022471902591, 10.00000000000009592 ) ) ;
#38019=CARTESIAN_POINT ( 'NONE',  ( 190.4281805785508084, 300.8157113754859893, -1.233909217199055774 ) ) ;
#38020=CARTESIAN_POINT ( 'NONE',  ( 13.65283037618196893, 184.8149278399160664, 9.188101187500093303 ) ) ;
#38024=CARTESIAN_POINT ( 'NONE',  ( 202.1252189466871130, 279.3787218446790348, -15.92426048611617340 ) ) ;
#38026=CARTESIAN_POINT ( 'NONE',  ( 165.0509870607838252, 244.7702999017660375, -2.356357909806504392 ) ) ;
#38027=CARTESIAN_POINT ( 'NONE',  ( 188.6625213059338932, 268.1393303463237885, 13.54573900311840084 ) ) ;
#38029=CARTESIAN_POINT ( 'NONE',  ( 179.7179132322487192, 263.0089460524625906, -13.84971012364866638 ) ) ;
#38032=CARTESIAN_POINT ( 'NONE',  ( 189.8136646974935786, 301.8800841035353528, -0.6430783927310335102 ) ) ;
#38034=CARTESIAN_POINT ( 'NONE',  ( 155.4216552449402684, 261.4487918497463284, 18.51722274565528892 ) ) ;
#38040=EDGE_CURVE ( 'NONE', #65090, #42238, #92531, .T. ) ;
#38048=EDGE_CURVE ( 'NONE', #26850, #40206, #47805, .T. ) ;
#38049=CARTESIAN_POINT ( 'NONE',  ( -22.42236680055709641, 157.8615022471902591, 0.000000000000000000 ) ) ;
#38052=CARTESIAN_POINT ( 'NONE',  ( 201.1388841337167435, 282.2642286331299601, -18.17233400608081340 ) ) ;
#38055=CARTESIAN_POINT ( 'NONE',  ( 163.8003088823192286, 260.8948240748503054, -17.39314492925268141 ) ) ;
#38057=CARTESIAN_POINT ( 'NONE',  ( 147.6857584380539095, 274.8477581613835810, 8.112022437684441201 ) ) ;
#38060=CARTESIAN_POINT ( 'NONE',  ( 157.1837449796689725, 258.3967629017010381, 16.97243084443542216 ) ) ;
#38062=CARTESIAN_POINT ( 'NONE',  ( 158.1203932377468107, 265.1298614022592801, 17.32494200193550071 ) ) ;
#38068=CARTESIAN_POINT ( 'NONE',  ( 159.5199931099367063, 254.7822369541973728, 15.51695619349162669 ) ) ;
#38070=VECTOR ( 'NONE', #77227, 1000.000000000000000 ) ;
#38073=EDGE_LOOP ( 'NONE', ( #3792, #94784, #30616, #97817 ) ) ;
#38076=CARTESIAN_POINT ( 'NONE',  ( 148.1672759425158290, 274.0137453789218398, 7.847779094015780110 ) ) ;
#38077=CARTESIAN_POINT ( 'NONE',  ( 190.8138402884741254, 300.1477291634665789, 4.037153726988762514 ) ) ;
#38078=CARTESIAN_POINT ( 'NONE',  ( 170.6169145365665827, 275.3029056381844271, -16.38693344838593191 ) ) ;
#38079=CARTESIAN_POINT ( 'NONE',  ( 191.6193632569555803, 298.7525224553929206, 9.793282278935404150 ) ) ;
#38080=CARTESIAN_POINT ( 'NONE',  ( 191.8210230231139803, 298.4032374945642232, -8.800268167321144475 ) ) ;
#38081=CARTESIAN_POINT ( 'NONE',  ( 162.8769348986911609, 257.5139437324259006, 15.59328385742420231 ) ) ;
#38082=CYLINDRICAL_SURFACE ( 'NONE', #67234, 17.82106496071139645 ) ;
#38083=CARTESIAN_POINT ( 'NONE',  ( 149.1939152435731728, 272.2355539484436235, -11.44223522189843933 ) ) ;
#38084=FACE_OUTER_BOUND ( 'NONE', #71846, .T. ) ;
#38086=CARTESIAN_POINT ( 'NONE',  ( 168.3980180112511391, 286.3881167737972646, 4.061716199848717679 ) ) ;
#38089=CARTESIAN_POINT ( 'NONE',  ( 190.8340530982597727, 300.1127195499541926, -4.121419783134655290 ) ) ;
#38091=CARTESIAN_POINT ( 'NONE',  ( 148.8084825648000731, 273.2965378644469183, 9.141718298254820851 ) ) ;
#38094=CARTESIAN_POINT ( 'NONE',  ( 191.7051687561719575, 297.9732336099989425, -9.478784037103174853 ) ) ;
#38096=CARTESIAN_POINT ( 'NONE',  ( 169.0953906076103692, 285.0085978602089654, -7.951903769486427187 ) ) ;
#38097=VERTEX_POINT ( 'NONE', #6982 ) ;
#38098=CARTESIAN_POINT ( 'NONE',  ( 207.6163508138795635, 271.0449272387537576, -1.385071889578343152 ) ) ;
#38099=CARTESIAN_POINT ( 'NONE',  ( 159.5050723400634638, 254.3761059724978679, -15.34938048045353298 ) ) ;
#38101=CARTESIAN_POINT ( 'NONE',  ( 50.59440005247052596, 190.0177522451418213, 5.000000000000051514 ) ) ;
#38102=CARTESIAN_POINT ( 'NONE',  ( 123.3136442261515526, 235.8768266524159856, 9.188101187500096856 ) ) ;
#38103=CARTESIAN_POINT ( 'NONE',  ( 180.2882253864519839, 294.9333264195223592, -3.538453439748629137 ) ) ;
#38105=CARTESIAN_POINT ( 'NONE',  ( 157.8092552871339365, 257.3133472685137235, 17.04082256169242626 ) ) ;
#38106=CARTESIAN_POINT ( 'NONE',  ( 175.1838294155237463, 253.3695104272607352, -3.877482245682918105 ) ) ;
#38107=CARTESIAN_POINT ( 'NONE',  ( 43.80151329331025067, 196.0958772461660544, -9.188101187500095079 ) ) ;
#38110=ORIENTED_EDGE ( 'NONE', *, *, #47652, .T. ) ;
#38111=CARTESIAN_POINT ( 'NONE',  ( 196.4030970371012472, 264.3490001850324234, -4.693669024083267693 ) ) ;
#38112=CARTESIAN_POINT ( 'NONE',  ( 179.2088379982556035, 266.5293678400578301, 15.13748914936972589 ) ) ;
#38114=CARTESIAN_POINT ( 'NONE',  ( 147.5177358149801421, 275.1387818813681179, 4.867883209065928085 ) ) ;
#38115=DIRECTION ( 'NONE',  ( 0.3975764696564279554, -0.6886226453387660484, -0.6064089404866747079 ) ) ;
#38117=CARTESIAN_POINT ( 'NONE',  ( 181.0193311394079103, 261.5502185760933003, 13.24438261311760812 ) ) ;
#38118=CARTESIAN_POINT ( 'NONE',  ( 119.8042635715769251, 226.6427522451417644, 1.119607411625061291E-15 ) ) ;
#38119=DIRECTION ( 'NONE',  ( -0.8660254037844359321, -0.5000000000000051070, -0.000000000000000000 ) ) ;
#38121=EDGE_CURVE ( 'NONE', #39829, #45578, #3448, .T. ) ;
#38122=CARTESIAN_POINT ( 'NONE',  ( 158.7770781770005044, 282.1650295664360897, -1.628693105680839359 ) ) ;
#38125=CARTESIAN_POINT ( 'NONE',  ( 35.79112540406921283, 179.2202760586659736, -5.415160957724236172E-17 ) ) ;
#38127=CARTESIAN_POINT ( 'NONE',  ( 192.1384501294028553, 272.2803415673531049, 15.07942017704054471 ) ) ;
#38130=CARTESIAN_POINT ( 'NONE',  ( 195.7949008739993531, 275.8773930737895057, -15.42861398852914512 ) ) ;
#38131=CARTESIAN_POINT ( 'NONE',  ( 66.48072710279772934, 203.0643266524160424, 9.188101187500095079 ) ) ;
#38132=CARTESIAN_POINT ( 'NONE',  ( 200.1662314894802819, 283.9489124310637180, 17.19420058542677054 ) ) ;
#38134=EDGE_CURVE ( 'NONE', #42320, #93829, #15143, .T. ) ;
#38139=CARTESIAN_POINT ( 'NONE',  ( 161.9943004083856408, 267.2312384411657149, 16.48735601444852961 ) ) ;
#38140=CARTESIAN_POINT ( 'NONE',  ( 16.11576366785047654, 170.1115022471901739, -5.000000000000041744 ) ) ;
#38141=CARTESIAN_POINT ( 'NONE',  ( 207.8060684685902686, 270.7163266217015689, 2.015725026008670540 ) ) ;
#38142=CARTESIAN_POINT ( 'NONE',  ( 137.8192226437758450, 256.5024278399160949, -9.188101187500093303 ) ) ;
#38144=CARTESIAN_POINT ( 'NONE',  ( 164.0729100755626746, 260.4632643121815363, -16.14824515792620829 ) ) ;
#38145=CARTESIAN_POINT ( 'NONE',  ( 185.7793147125802875, 260.5841321348162865, 6.335720874329757279 ) ) ;
#38153=CARTESIAN_POINT ( 'NONE',  ( 179.5572819769699606, 286.1165802574137160, 13.07273523577711138 ) ) ;
#38154=CARTESIAN_POINT ( 'NONE',  ( 156.6893878665337638, 280.2375996934318323, -5.371908398693758357 ) ) ;
#38161=CARTESIAN_POINT ( 'NONE',  ( 200.5812521528945638, 281.4385583276488205, -17.14082239954941755 ) ) ;
#38163=AXIS2_PLACEMENT_3D ( 'NONE', #12373, #51344, #27577 ) ;
#38164=CARTESIAN_POINT ( 'NONE',  ( 208.3764315856425640, 269.7284287242038658, -1.833640725398759441 ) ) ;
#38166=VERTEX_POINT ( 'NONE', #1895 ) ;
#38167=ADVANCED_FACE ( 'NONE', ( #55069 ), #55560, .T. ) ;
#38168=CARTESIAN_POINT ( 'NONE',  ( 190.9259979929221913, 280.9477547779517863, 16.64741033664369141 ) ) ;
#38169=CARTESIAN_POINT ( 'NONE',  ( 167.0957737472305666, 246.8272050136007749, 1.963998143010642128 ) ) ;
#38171=CARTESIAN_POINT ( 'NONE',  ( 149.0761751337341821, 272.4394858007734683, 11.56094486755886130 ) ) ;
#38172=CARTESIAN_POINT ( 'NONE',  ( 6.406750531224583156, 186.0530062829863027, -4.648177544792955347E-16 ) ) ;
#38174=ORIENTED_EDGE ( 'NONE', *, *, #86110, .T. ) ;
#38175=CARTESIAN_POINT ( 'NONE',  ( 162.7435819479956933, 250.7668427907593411, -13.06080741167749082 ) ) ;
#38177=B_SPLINE_CURVE_WITH_KNOTS ( 'NONE', 3,
 ( #57117, #57619, #96674, #3934 ),
 .UNSPECIFIED., .F., .F.,
 ( 4, 4 ),
 ( 0.03227822889357200020, 0.04124890145165294175 ),
 .UNSPECIFIED. ) ;
#38182=CARTESIAN_POINT ( 'NONE',  ( 102.3121810886139116, 236.0024278399160949, 9.188101187500095079 ) ) ;
#38183=CARTESIAN_POINT ( 'NONE',  ( 200.2690241097007799, 283.7708703901988656, 16.96680019208369927 ) ) ;
#38185=CARTESIAN_POINT ( 'NONE',  ( 181.2482315834775477, 271.4898918969783495, -16.12830051190350034 ) ) ;
#38189=VERTEX_POINT ( 'NONE', #89538 ) ;
#38190=EDGE_LOOP ( 'NONE', ( #75328, #58654, #12349 ) ) ;
#38195=CARTESIAN_POINT ( 'NONE',  ( 208.3135187673106543, 269.8373969220020285, 2.829653198597726682 ) ) ;
#38196=CARTESIAN_POINT ( 'NONE',  ( 190.8429499865819707, 278.0757709512191695, -17.64141544901220371 ) ) ;
#38197=CARTESIAN_POINT ( 'NONE',  ( 171.0593044012981068, 283.5750802371461532, 12.19867815159854807 ) ) ;
#38198=CARTESIAN_POINT ( 'NONE',  ( 194.2223991963907963, 294.2439319543634610, -14.97294938100067441 ) ) ;
#38200=CARTESIAN_POINT ( 'NONE',  ( 200.0411626275569574, 270.6720010161316736, -11.59284015024147152 ) ) ;
#38203=CARTESIAN_POINT ( 'NONE',  ( 163.4923624983613024, 282.7451307114477572, 8.800724806903520658 ) ) ;
#38208=CARTESIAN_POINT ( 'NONE',  ( 202.9972156839127990, 279.0455039708822937, 16.77197898838388213 ) ) ;
#38209=FACE_OUTER_BOUND ( 'NONE', #53522, .T. ) ;
#38212=CARTESIAN_POINT ( 'NONE',  ( 180.3515574791316283, 255.6186696229350446, 6.159525720347461153 ) ) ;
#38215=CARTESIAN_POINT ( 'NONE',  ( 194.7902205010250043, 263.3917080119609295, -0.7864463132427590430 ) ) ;
#38217=CARTESIAN_POINT ( 'NONE',  ( 194.0373855506731502, 294.5643849888401746, -14.18241207909759538 ) ) ;
#38221=CARTESIAN_POINT ( 'NONE',  ( 5.561079055679667427, 174.0177522451418781, -10.00000000000009592 ) ) ;
#38223=CARTESIAN_POINT ( 'NONE',  ( 174.5125536636238621, 282.4638039902177979, -14.82547868367492327 ) ) ;
#38224=CARTESIAN_POINT ( 'NONE',  ( 203.6765436393997675, 277.8688734369772533, -15.81082241283986178 ) ) ;
#38226=CARTESIAN_POINT ( 'NONE',  ( 178.6423073663378602, 290.9544255387157818, 10.03153667033594765 ) ) ;
#38227=CARTESIAN_POINT ( 'NONE',  ( -7.212535326543083158, 157.4548013555409796, -4.594050593750042211 ) ) ;
#38229=CARTESIAN_POINT ( 'NONE',  ( 185.2391986358457530, 295.7873944733689768, 8.585680893828113724 ) ) ;
#38232=VERTEX_POINT ( 'NONE', #11510 ) ;
#38233=CARTESIAN_POINT ( 'NONE',  ( 151.9857020112045802, 279.0317921242573789, 1.822192154687843457 ) ) ;
#38237=LINE ( 'NONE', #30669, #25890 ) ;
#38238=CARTESIAN_POINT ( 'NONE',  ( 162.6464992788258144, 248.9349949062956284, -10.29443606917336496 ) ) ;
#38240=CARTESIAN_POINT ( 'NONE',  ( 150.1971333718279880, 276.5536166081793112, 3.687813122935997168 ) ) ;
#38241=CARTESIAN_POINT ( 'NONE',  ( 25.93973934025619599, 185.7833772461660544, -9.188101187500095079 ) ) ;
#38242=CARTESIAN_POINT ( 'NONE',  ( 116.0331843058823296, 246.9869531367911293, 4.594050593750046652 ) ) ;
#38243=CARTESIAN_POINT ( 'NONE',  ( 181.2440676231241241, 294.5520841294345473, -6.623935519155441654 ) ) ;
#38244=CARTESIAN_POINT ( 'NONE',  ( 196.0931812089658592, 275.1780562578900913, 15.95755391823183444 ) ) ;
#38245=CYLINDRICAL_SURFACE ( 'NONE', #2823, 17.82106496071139645 ) ;
#38246=B_SPLINE_CURVE_WITH_KNOTS ( 'NONE', 3,
 ( #51204, #3160, #34045, #64935 ),
 .UNSPECIFIED., .F., .F.,
 ( 4, 4 ),
 ( 0.005339423476618587738, 0.01094292413399224062 ),
 .UNSPECIFIED. ) ;
#38251=DIRECTION ( 'NONE',  ( -0.8660254037844387076, -0.4999999999999998890, -0.000000000000000000 ) ) ;
#38255=CARTESIAN_POINT ( 'NONE',  ( 171.3829901640632443, 279.8345946159657274, 13.89615929642840619 ) ) ;
#38256=CARTESIAN_POINT ( 'NONE',  ( 19.94070920123167312, 188.9865022471903160, -10.00000000000009592 ) ) ;
#38259=CARTESIAN_POINT ( 'NONE',  ( 207.3343352015242829, 271.1099079521872000, 2.793079588467688001 ) ) ;
#38260=CARTESIAN_POINT ( 'NONE',  ( 180.8886733632373591, 266.5746820064321128, -14.68068468162151596 ) ) ;
#38263=EDGE_CURVE ( 'NONE', #1077, #9692, #57958, .T. ) ;
#38264=B_SPLINE_CURVE_WITH_KNOTS ( 'NONE', 3,
 ( #71719, #9395, #10402, #2310 ),
 .UNSPECIFIED., .F., .F.,
 ( 4, 4 ),
 ( 0.0001948154735252194804, 0.0003149152481875766942 ),
 .UNSPECIFIED. ) ;
#38265=CARTESIAN_POINT ( 'NONE',  ( 184.4241326561383403, 269.4503056644531966, 15.31856924807197196 ) ) ;
#38268=CARTESIAN_POINT ( 'NONE',  ( 87.34609280552280097, 230.4244531367911009, -4.594050593750046652 ) ) ;
#38270=CARTESIAN_POINT ( 'NONE',  ( -7.266922234329370234, 156.6115022471902023, -5.000000000000041744 ) ) ;
#38272=CARTESIAN_POINT ( 'NONE',  ( 157.4177733328310467, 257.9914139036126812, 18.29188238796808363 ) ) ;
#38273=CARTESIAN_POINT ( 'NONE',  ( 195.6708441445795756, 278.3169109478037626, 17.04649191961062726 ) ) ;
#38274=CARTESIAN_POINT ( 'NONE',  ( 201.4550628388361417, 270.3106342360672443, -10.24027999735716854 ) ) ;
#38275=CARTESIAN_POINT ( 'NONE',  ( 181.5558742819051474, 255.2544784655372894, -2.503599602330015994 ) ) ;
#38277=AXIS2_PLACEMENT_3D ( 'NONE', #25705, #10003, #40867 ) ;
#38280=CARTESIAN_POINT ( 'NONE',  ( 7.313483791488072150, 163.4824982072973683, 3.021315404115420679E-15 ) ) ;
#38283=CARTESIAN_POINT ( 'NONE',  ( 178.5040461245142183, 280.6592112227464213, 16.58436230249095189 ) ) ;
#38285=CARTESIAN_POINT ( 'NONE',  ( 196.6512732745314906, 267.5067273676284003, 9.687024394805378691 ) ) ;
#38286=CARTESIAN_POINT ( 'NONE',  ( 65.93257831369518840, 197.3262482093457777, 3.021315404115420679E-15 ) ) ;
#38288=B_SPLINE_SURFACE_WITH_KNOTS ( 'NONE', 3, 1, ( 
 ( #74521, #35980 ),
 ( #74010, #34493 ),
 ( #50194, #65395 ),
 ( #42574, #26904 ),
 ( #96839, #57783 ),
 ( #19812, #81146 ),
 ( #50680, #28899 ),
 ( #82652, #13211 ),
 ( #66884, #4595 ),
 ( #19332, #81635 ),
 ( #28383, #58771 ),
 ( #35489, #75009 ),
 ( #89742, #20306 ),
 ( #4091, #5589 ),
 ( #65886, #52176 ),
 ( #51179, #100214 ),
 ( #77402, #85547 ),
 ( #86551, #38375 ),
 ( #1902, #54069 ),
 ( #8008, #16587 ),
 ( #394, #61679 ),
 ( #23670, #23178 ),
 ( #32781, #38880 ),
 ( #47483, #15569 ),
 ( #54562, #92629 ),
 ( #47973, #17083 ),
 ( #8989, #55075 ),
 ( #78918, #70794 ),
 ( #31282, #63691 ),
 ( #69289, #78408 ),
 ( #85025, #76884 ),
 ( #9505, #16088 ),
 ( #46994, #46473 ),
 ( #69784, #77908 ) ),
 .UNSPECIFIED., .T., .F., .F.,
 ( 4, 2, 2, 2, 2, 2, 2, 2, 2, 2, 2, 2, 2, 2, 2, 2, 4 ),
 ( 2, 2 ),
 ( 0.000000000000000000, 0.06250000000000000000, 0.1250000000000000000, 0.1875000000000000000, 0.2500000000000000000, 0.3125000000000000000, 0.3750000000000000000, 0.4375000000000000000, 0.5000000000000000000, 0.5625000000000000000, 0.6250000000000000000, 0.6875000000000000000, 0.7500000000000000000, 0.8125000000000000000, 0.8750000000000000000, 0.9375000000000000000, 1.000000000000000000 ),
 ( 0.000000000000000000, 1.000000000000000000 ),
 .UNSPECIFIED. ) ;
#38291=CARTESIAN_POINT ( 'NONE',  ( 198.2819808855875863, 287.2125302111982705, 18.53535247371401695 ) ) ;
#38292=CARTESIAN_POINT ( 'NONE',  ( 183.6672295643515440, 264.5222299264054868, -13.41344130462387518 ) ) ;
#38293=CARTESIAN_POINT ( 'NONE',  ( 169.4327616935881053, 251.8687907473509711, -8.483257748728734171 ) ) ;
#38294=CARTESIAN_POINT ( 'NONE',  ( 151.2157266582228772, 248.1115022471902023, -5.000000000000041744 ) ) ;
#38295=ORIENTED_EDGE ( 'NONE', *, *, #31070, .F. ) ;
#38296=EDGE_CURVE ( 'NONE', #4844, #7878, #55764, .T. ) ;
#38297=CARTESIAN_POINT ( 'NONE',  ( 187.5143746346354021, 278.9518094448188776, 17.63296374067274286 ) ) ;
#38301=DIRECTION ( 'NONE',  ( 0.4999999999999992784, -0.8660254037844390407, 0.000000000000000000 ) ) ;
#38302=CARTESIAN_POINT ( 'NONE',  ( 183.4092525909616711, 291.5038694251641687, -10.73000149755480948 ) ) ;
#38305=CARTESIAN_POINT ( 'NONE',  ( 206.2884309622781984, 273.3449518901063584, 11.80432421640126250 ) ) ;
#38307=CARTESIAN_POINT ( 'NONE',  ( 153.3658703804616152, 265.0095156844545272, -16.92037735142076826 ) ) ;
#38308=B_SPLINE_CURVE_WITH_KNOTS ( 'NONE', 3,
 ( #23069, #62061, #99107, #76310 ),
 .UNSPECIFIED., .F., .F.,
 ( 4, 4 ),
 ( 0.001669260644153817410, 0.003387224320680204057 ),
 .UNSPECIFIED. ) ;
#38309=CARTESIAN_POINT ( 'NONE',  ( 187.4167187180463259, 296.4074041626601002, 9.525756846988903348 ) ) ;
#38310=CARTESIAN_POINT ( 'NONE',  ( 182.7847760313759409, 280.0284915794045446, -17.53211380394024843 ) ) ;
#38311=AXIS2_PLACEMENT_3D ( 'NONE', #72011, #25916, #2615 ) ;
#38315=VERTEX_POINT ( 'NONE', #35780 ) ;
#38316=CARTESIAN_POINT ( 'NONE',  ( 162.8640727416213281, 249.5241558410263849, 11.11676342424593855 ) ) ;
#38319=VERTEX_POINT ( 'NONE', #97131 ) ;
#38321=( BOUNDED_CURVE ( )  B_SPLINE_CURVE ( 2, ( #24615, #55497, #8919, #18916, #78841, #32716, #17010, #63617, #3708 ),
 .UNSPECIFIED., .F., .F. ) 
 B_SPLINE_CURVE_WITH_KNOTS ( ( 3, 2, 2, 2, 3 ),
 ( 0.4879032258064516236, 0.4892473118279569988, 0.4919354838709677491, 0.4946236559139784994, 0.4959677419354838745 ),
 .UNSPECIFIED. ) 
 CURVE ( )  GEOMETRIC_REPRESENTATION_ITEM ( )  RATIONAL_B_SPLINE_CURVE ( ( 0.9330127018922194093, 0.9330127018922194093, 1.000000000000000000, 0.8660254037844387076, 1.000000000000000000, 0.8660254037844387076, 1.000000000000000000, 0.9330127018922194093, 0.9330127018922194093 ) ) 
 REPRESENTATION_ITEM ( '' )  );
#38322=CARTESIAN_POINT ( 'NONE',  ( 170.8944053752079810, 255.0871438150282700, -11.36895391432762636 ) ) ;
#38323=CARTESIAN_POINT ( 'NONE',  ( 190.5526305594705434, 299.9695577504274979, -4.324655322867677398 ) ) ;
#38324=CARTESIAN_POINT ( 'NONE',  ( 164.9402323277223275, 244.9621327266073081, -1.073314903116530106 ) ) ;
#38325=CARTESIAN_POINT ( 'NONE',  ( 197.4166373598459074, 273.1534249293282528, -13.33078627074450395 ) ) ;
#38328=CARTESIAN_POINT ( 'NONE',  ( 168.0467845603413366, 249.4717662844409176, -5.469034782820844320 ) ) ;
#38330=CARTESIAN_POINT ( 'NONE',  ( 178.1815451042072596, 255.1982646830548447, 5.740691749723041859 ) ) ;
#38331=CARTESIAN_POINT ( 'NONE',  ( 120.0931990297694085, 230.9548013555409796, -4.594050593750042211 ) ) ;
#38332=CARTESIAN_POINT ( 'NONE',  ( 187.0608580662972713, 262.1253545432567762, -10.24587999176721276 ) ) ;
#38334=CARTESIAN_POINT ( 'NONE',  ( 188.1875818435630663, 273.5226728761291497, 15.67860454874873355 ) ) ;
#38337=B_SPLINE_CURVE_WITH_KNOTS ( 'NONE', 3,
 ( #12553, #51534, #74860, #35834, #97180, #52035, #98154, #89591, #5932, #36325, #43426, #20156, #51024, #96682 ),
 .UNSPECIFIED., .F., .F.,
 ( 4, 2, 2, 2, 2, 2, 4 ),
 ( 0.002301009298598415652, 0.002438001431547676037, 0.002574993564496935988, 0.002711985697446196372, 0.002848977830395456323, 0.003396946362192322221, 0.004492883425785989399 ),
 .UNSPECIFIED. ) ;
#38340=CARTESIAN_POINT ( 'NONE',  ( 117.2783561438722586, 238.5177522451418497, -10.00000000000009592 ) ) ;
#38342=CARTESIAN_POINT ( 'NONE',  ( 192.6336181944592454, 296.9957813718090165, 11.10275837363962737 ) ) ;
#38343=CARTESIAN_POINT ( 'NONE',  ( 190.2204363742943656, 300.4646209966566062, -1.328626404316530739E-11 ) ) ;
#38345=ORIENTED_EDGE ( 'NONE', *, *, #76421, .F. ) ;
#38351=CARTESIAN_POINT ( 'NONE',  ( 192.5930808083610088, 262.6107660501119199, 4.653369615412138671 ) ) ;
#38352=CARTESIAN_POINT ( 'NONE',  ( 158.0314954405573644, 263.1485498153232356, 17.26347671721901023 ) ) ;
#38355=CARTESIAN_POINT ( 'NONE',  ( 197.8980529691977779, 285.8775128688180871, 17.80711829255526979 ) ) ;
#38356=CARTESIAN_POINT ( 'NONE',  ( 160.7022581417230356, 281.5213664053168827, 5.619168078228955920 ) ) ;
#38357=CARTESIAN_POINT ( 'NONE',  ( 201.2139346379346705, 282.1342373466909521, -16.65315141107179286 ) ) ;
#38360=CARTESIAN_POINT ( 'NONE',  ( 147.5634954182374372, 275.0595239235922236, 4.682022975662822439 ) ) ;
#38362=CARTESIAN_POINT ( 'NONE',  ( 188.2563532189512898, 263.5935347285679313, -9.073490670746114262 ) ) ;
#38363=CARTESIAN_POINT ( 'NONE',  ( 149.1870424807857489, 245.3932355074535678, -2.679491924311248496 ) ) ;
#38364=CARTESIAN_POINT ( 'NONE',  ( 192.7286328587738922, 271.7632531150862860, -14.68684183385635933 ) ) ;
#38365=CARTESIAN_POINT ( 'NONE',  ( 12.56145106960391011, 171.3927522451417929, 10.00000000000009948 ) ) ;
#38367=CARTESIAN_POINT ( 'NONE',  ( 38.37437292394342592, 181.4155109091896065, 2.679491924311254714 ) ) ;
#38369=CARTESIAN_POINT ( 'NONE',  ( 191.4422718808379500, 282.7623406846040552, -17.33968414145821058 ) ) ;
#38371=CARTESIAN_POINT ( 'NONE',  ( 78.87554214658000262, 216.3458772461660544, 9.188101187500095079 ) ) ;
#38373=CARTESIAN_POINT ( 'NONE',  ( 192.6679047218190135, 296.9363953644068488, -13.34486378385621386 ) ) ;
#38375=CARTESIAN_POINT ( 'NONE',  ( 154.9792334219179679, 262.2150889255981951, -17.21325849938693153 ) ) ;
#38376=CARTESIAN_POINT ( 'NONE',  ( 207.8232941427535536, 270.6864908788566026, -6.505149060073906142 ) ) ;
#38379=CARTESIAN_POINT ( 'NONE',  ( 46.33644181719702715, 190.8927522451418213, 10.00000000000009948 ) ) ;
#38380=DIRECTION ( 'NONE',  ( -0.8660254037844387076, -0.4999999999999998890, -0.000000000000000000 ) ) ;
#38382=DIRECTION ( 'NONE',  ( -0.5000000000000006661, 0.8660254037844382635, -1.877843081442121204E-16 ) ) ;
#38384=CARTESIAN_POINT ( 'NONE',  ( 204.8200301798767384, 275.8882966510998926, -12.76918925326218179 ) ) ;
#38385=EDGE_CURVE ( 'NONE', #84992, #6168, #27193, .T. ) ;
#38386=CARTESIAN_POINT ( 'NONE',  ( 157.7233946900069839, 257.4620621851055375, 16.86796251324260254 ) ) ;
#38388=EDGE_CURVE ( 'NONE', #92570, #47543, #80528, .T. ) ;
#38389=CARTESIAN_POINT ( 'NONE',  ( 25.93973934025619599, 185.7833772461660544, -9.188101187500095079 ) ) ;
#38392=CARTESIAN_POINT ( 'NONE',  ( 49.48463145776311478, 205.5024278399160949, -9.188101187500093303 ) ) ;
#38395=CARTESIAN_POINT ( 'NONE',  ( 165.7191908502203717, 249.0136070854895820, -9.415553735363799248 ) ) ;
#38396=CARTESIAN_POINT ( 'NONE',  ( -16.43235775771474749, 167.9865022471903160, -10.00000000000009415 ) ) ;
#38401=CARTESIAN_POINT ( 'NONE',  ( 149.4908848037268001, 271.7211875819559737, -12.92288068979413573 ) ) ;
#38403=CARTESIAN_POINT ( 'NONE',  ( 59.93088934303040105, 217.6589784336661353, -6.496448406907676862E-16 ) ) ;
#38405=CARTESIAN_POINT ( 'NONE',  ( 175.2603759342789829, 291.6537898291654187, 1.882018043770492977 ) ) ;
#38406=CARTESIAN_POINT ( 'NONE',  ( 159.8655504377736918, 253.7517395922482706, 15.51368179719542262 ) ) ;
#38407=CARTESIAN_POINT ( 'NONE',  ( 191.2557879401978198, 261.3776189723048446, -4.694998167070893125 ) ) ;
#38408=CARTESIAN_POINT ( 'NONE',  ( 150.0366313281010093, 275.4335823404518351, 7.372954474402361846 ) ) ;
#38410=CARTESIAN_POINT ( 'NONE',  ( 105.6772241758911264, 238.4865022471903444, -10.00000000000009415 ) ) ;
#38411=CARTESIAN_POINT ( 'NONE',  ( 161.1884843536000744, 251.4603508349806873, 13.21272898143761942 ) ) ;
#38412=CARTESIAN_POINT ( 'NONE',  ( 164.2600772519394923, 246.1401958748887182, -2.110785484364219311 ) ) ;
#38417=CARTESIAN_POINT ( 'NONE',  ( 159.7692415128758228, 253.9185515433934768, -16.85856106119654285 ) ) ;
#38418=CARTESIAN_POINT ( 'NONE',  ( 186.8942146390193955, 276.6477083451915178, -17.00271009909913289 ) ) ;
#38419=CARTESIAN_POINT ( 'NONE',  ( 115.5259514080638468, 249.0530062829863311, -4.648177544792955347E-16 ) ) ;
#38420=VERTEX_POINT ( 'NONE', #67169 ) ;
#38423=CARTESIAN_POINT ( 'NONE',  ( 148.4042165687623083, 273.6033521758856750, -8.709765892313745539 ) ) ;
#38431=FACE_OUTER_BOUND ( 'NONE', #13575, .T. ) ;
#38434=CARTESIAN_POINT ( 'NONE',  ( 159.9470087484377814, 253.6106496594791508, -16.54933891566789939 ) ) ;
#38435=VERTEX_POINT ( 'NONE', #57571 ) ;
#38436=CARTESIAN_POINT ( 'NONE',  ( 171.1617965414632749, 285.2369355936916691, 11.22781892977234719 ) ) ;
#38438=CARTESIAN_POINT ( 'NONE',  ( 162.9873704432093291, 283.5760391986459013, -3.109501405526100992 ) ) ;
#38441=CARTESIAN_POINT ( 'NONE',  ( 163.8670932201372352, 246.8208641845333773, 5.912697114930636211 ) ) ;
#38442=CARTESIAN_POINT ( 'NONE',  ( 198.5558597050348908, 286.7381581807989051, 17.16554469393394200 ) ) ;
#38443=CARTESIAN_POINT ( 'NONE',  ( 157.2777284163744582, 258.2339788142568864, -16.82360006463426316 ) ) ;
#38444=CARTESIAN_POINT ( 'NONE',  ( 131.9464011004214115, 256.1744531367911009, 4.594050593750047540 ) ) ;
#38445=CARTESIAN_POINT ( 'NONE',  ( 203.1999414577625203, 267.8405105413980891, 2.559446679431893301 ) ) ;
#38446=VECTOR ( 'NONE', #77057, 1000.000000000000000 ) ;
#38447=CARTESIAN_POINT ( 'NONE',  ( 195.4450401646303987, 290.4134588786556037, -16.67804988919992581 ) ) ;
#38448=CARTESIAN_POINT ( 'NONE',  ( 70.81050702595493362, 217.8149278399160664, 9.188101187500093303 ) ) ;
#38449=ORIENTED_EDGE ( 'NONE', *, *, #37040, .T. ) ;
#38450=CARTESIAN_POINT ( 'NONE',  ( 172.8011810764148208, 265.0538244599177347, 15.94685020396837238 ) ) ;
#38451=CARTESIAN_POINT ( 'NONE',  ( 204.0604753336787667, 271.4817813032398703, 9.862283393711939183 ) ) ;
#38454=CARTESIAN_POINT ( 'NONE',  ( 195.4711919121670860, 292.0809595225171620, -15.84858701701355521 ) ) ;
#38455=EDGE_LOOP ( 'NONE', ( #79879, #32077, #15657 ) ) ;
#38458=CARTESIAN_POINT ( 'NONE',  ( 197.6796757083432681, 286.6912785265818115, 16.92400811840941799 ) ) ;
#38459=CARTESIAN_POINT ( 'NONE',  ( 147.0660117096331874, 275.9211909828330249, -0.7354350123930680772 ) ) ;
#38461=CARTESIAN_POINT ( 'NONE',  ( 154.8596847415876994, 262.4221533139083817, 17.65401077761399762 ) ) ;
#38463=CARTESIAN_POINT ( 'NONE',  ( 77.90126356732251622, 215.7833772461660544, -9.188101187500095079 ) ) ;
#38464=ORIENTED_EDGE ( 'NONE', *, *, #48508, .T. ) ;
#38465=ADVANCED_FACE ( 'NONE', ( #57069 ), #18598, .T. ) ;
#38470=VERTEX_POINT ( 'NONE', #67673 ) ;
#38471=EDGE_CURVE ( 'NONE', #79855, #61965, #16420, .T. ) ;
#38473=CARTESIAN_POINT ( 'NONE',  ( 184.3174667830732574, 275.3152583799672470, 16.37424376149754934 ) ) ;
#38474=CARTESIAN_POINT ( 'NONE',  ( 165.0020474182383339, 244.8550658491588479, 1.825383354618924425 ) ) ;
#38475=CARTESIAN_POINT ( 'NONE',  ( 165.4191378457005897, 285.2699752501742978, 0.5081224057291762186 ) ) ;
#38477=DIRECTION ( 'NONE',  ( 0.5000000000000048850, -0.8660254037844358210, 0.000000000000000000 ) ) ;
#38479=CARTESIAN_POINT ( 'NONE',  ( 188.6582881733277191, 295.0323815393699647, 11.70685045119338774 ) ) ;
#38482=CARTESIAN_POINT ( 'NONE',  ( 200.8665851640556070, 282.7358642834317948, -16.69422397739980823 ) ) ;
#38485=ORIENTED_EDGE ( 'NONE', *, *, #38605, .F. ) ;
#38486=CARTESIAN_POINT ( 'NONE',  ( 196.0436306077152722, 265.5675073304090574, 4.427515145396084151 ) ) ;
#38487=CARTESIAN_POINT ( 'NONE',  ( 148.3216606269014619, 276.4951605611222476, -3.899572877788914482 ) ) ;
#38488=CARTESIAN_POINT ( 'NONE',  ( 22.53878541258498558, 190.4865022471903160, -10.00000000000009592 ) ) ;
#38491=DIRECTION ( 'NONE',  ( 0.4999999999999998890, -0.8660254037844385966, 0.000000000000000000 ) ) ;
#38492=CARTESIAN_POINT ( 'NONE',  ( 153.3323979404929958, 270.2931725392325575, 13.99377495420697137 ) ) ;
#38494=CARTESIAN_POINT ( 'NONE',  ( 147.3023124603499809, 275.5119060767245287, 5.196938859334171212 ) ) ;
#38495=CARTESIAN_POINT ( 'NONE',  ( 162.9466247808429102, 248.4151622881552441, 11.25765811906727443 ) ) ;
#38498=CARTESIAN_POINT ( 'NONE',  ( 206.9026071836525205, 272.2811674698855313, 7.240992997279449561 ) ) ;
#38499=CARTESIAN_POINT ( 'NONE',  ( 193.9495889092963807, 294.7164532324382549, 15.46986001312306058 ) ) ;
#38503=CARTESIAN_POINT ( 'NONE',  ( 163.3311208880642766, 283.7460365591649065, -3.269890911538303246 ) ) ;
#38507=CARTESIAN_POINT ( 'NONE',  ( 153.5792543191700474, 246.1427522451417644, 1.119607411625061291E-15 ) ) ;
#38509=ORIENTED_EDGE ( 'NONE', *, *, #28633, .T. ) ;
#38511=VECTOR ( 'NONE', #25545, 1000.000000000000000 ) ;
#38516=CARTESIAN_POINT ( 'NONE',  ( 10.56744132731740393, 189.1589784336661637, -6.496448406907676862E-16 ) ) ;
#38517=CARTESIAN_POINT ( 'NONE',  ( 176.1996253725332053, 265.6108028435369306, -16.12497321327553834 ) ) ;
#38518=CARTESIAN_POINT ( 'NONE',  ( 181.7343043149082291, 275.5595704463788138, -16.43090409027867693 ) ) ;
#38521=CARTESIAN_POINT ( 'NONE',  ( 205.0520875136525376, 275.4863615587311756, -14.16385635411862509 ) ) ;
#38524=CARTESIAN_POINT ( 'NONE',  ( 41.64315915125185086, 206.3967562850347122, -4.648177544792955347E-16 ) ) ;
#38526=B_SPLINE_CURVE_WITH_KNOTS ( 'NONE', 3,
 ( #56654, #64770, #80001, #12067 ),
 .UNSPECIFIED., .F., .F.,
 ( 4, 4 ),
 ( 0.02779447496634188455, 0.03699400560506550112 ),
 .UNSPECIFIED. ) ;
#38527=CARTESIAN_POINT ( 'NONE',  ( 182.8490516821578922, 296.1971294003607227, 1.821377340828691516 ) ) ;
#38528=CARTESIAN_POINT ( 'NONE',  ( 78.03658003843786162, 205.8615022471901739, 5.000000000000051514 ) ) ;
#38529=CYLINDRICAL_SURFACE ( 'NONE', #70068, 10.00000000000010658 ) ;
#38531=CARTESIAN_POINT ( 'NONE',  ( 147.6220714307702622, 274.9580672937808572, 8.392894244419288441 ) ) ;
#38532=CARTESIAN_POINT ( 'NONE',  ( 26.15589859543730000, 198.1589784336661637, -6.496448406907675876E-16 ) ) ;
#38534=CARTESIAN_POINT ( 'NONE',  ( 202.9990333130177191, 270.0056268523717335, -6.342944502012394459 ) ) ;
#38535=CARTESIAN_POINT ( 'NONE',  ( 150.8247211172754589, 269.4109153179094278, -14.37608026040300402 ) ) ;
#38536=CARTESIAN_POINT ( 'NONE',  ( 207.5338226493333025, 271.1878702128032614, 6.432541580693135863 ) ) ;
#38537=CARTESIAN_POINT ( 'NONE',  ( 155.2098048002210930, 261.8157275836062468, 16.98811268941991059 ) ) ;
#38538=CARTESIAN_POINT ( 'NONE',  ( -17.42236680055705023, 149.2012482093457777, 0.000000000000000000 ) ) ;
#38539=CARTESIAN_POINT ( 'NONE',  ( 202.8700503780948736, 278.3479282389285459, -15.15511564031462832 ) ) ;
#38540=CARTESIAN_POINT ( 'NONE',  ( 161.0050726372687393, 280.1669587882555561, 9.054279574223530247 ) ) ;
#38543=CARTESIAN_POINT ( 'NONE',  ( 198.2505066714982149, 285.2670451491296149, 0.000000000000000000 ) ) ;
#38545=CARTESIAN_POINT ( 'NONE',  ( 186.8465721486132907, 268.7342973959014216, -14.16766902808887174 ) ) ;
#38546=ORIENTED_EDGE ( 'NONE', *, *, #85833, .T. ) ;
#38550=ORIENTED_EDGE ( 'NONE', *, *, #87066, .F. ) ;
#38557=DIRECTION ( 'NONE',  ( -0.8660254037844387076, -0.4999999999999998890, -0.000000000000000000 ) ) ;
#38560=CARTESIAN_POINT ( 'NONE',  ( 201.2535035105529744, 282.0657020489176716, -18.08976065250591958 ) ) ;
#38563=CARTESIAN_POINT ( 'NONE',  ( 196.4030970371012472, 264.3490001850324234, -4.693669024083267693 ) ) ;
#38565=B_SPLINE_CURVE_WITH_KNOTS ( 'NONE', 3,
 ( #55207, #71444, #71942, #86188 ),
 .UNSPECIFIED., .F., .F.,
 ( 4, 4 ),
 ( 1.003144254802035469E-16, 0.005446537507594250913 ),
 .UNSPECIFIED. ) ;
#38566=ORIENTED_EDGE ( 'NONE', *, *, #80199, .T. ) ;
#38567=CARTESIAN_POINT ( 'NONE',  ( 147.7978300115112233, 274.6536445020713018, 7.902890709649431855 ) ) ;
#38570=EDGE_CURVE ( 'NONE', #53329, #38470, #57509, .T. ) ;
#38571=ORIENTED_EDGE ( 'NONE', *, *, #80453, .F. ) ;
#38572=CARTESIAN_POINT ( 'NONE',  ( 195.9920715006079490, 291.1787696107118677, 15.99608784761372071 ) ) ;
#38574=CARTESIAN_POINT ( 'NONE',  ( 158.9922026222019156, 265.5549985037428087, 16.88018579597198610 ) ) ;
#38581=CARTESIAN_POINT ( 'NONE',  ( 160.5772802285540024, 254.1801457531887536, 15.69096569341868452 ) ) ;
#38584=ORIENTED_EDGE ( 'NONE', *, *, #79610, .T. ) ;
#38586=VECTOR ( 'NONE', #84818, 1000.000000000000000 ) ;
#38587=CARTESIAN_POINT ( 'NONE',  ( 189.9686529740312153, 299.6116365339944423, 6.575253125843024016 ) ) ;
#38588=CARTESIAN_POINT ( 'NONE',  ( 70.44081555586384980, 218.1427522451419065, -10.00000000000009592 ) ) ;
#38589=CARTESIAN_POINT ( 'NONE',  ( 190.6084209867335915, 300.5035258309363826, -0.5505750481748228342 ) ) ;
#38590=CARTESIAN_POINT ( 'NONE',  ( 190.6661865267473104, 300.4034729807058852, 4.523489664447863490 ) ) ;
#38591=CARTESIAN_POINT ( 'NONE',  ( 136.9263074957796675, 249.8615022471902591, -10.00000000000009592 ) ) ;
#38592=EDGE_CURVE ( 'NONE', #63287, #21764, #20033, .T. ) ;
#38593=CARTESIAN_POINT ( 'NONE',  ( 191.1517988646461674, 299.5623677386828376, 8.533933079859274073 ) ) ;
#38594=CARTESIAN_POINT ( 'NONE',  ( 147.0456760057551833, 275.9564134551570760, -3.678503029046952033 ) ) ;
#38595=CARTESIAN_POINT ( 'NONE',  ( 163.1374594064594987, 257.6710164228418876, 15.57553777135039219 ) ) ;
#38597=AXIS2_PLACEMENT_3D ( 'NONE', #59852, #13760, #61719 ) ;
#38603=CARTESIAN_POINT ( 'NONE',  ( 190.4637805006824749, 300.7540505016085035, -3.224520439125855287 ) ) ;
#38605=EDGE_CURVE ( 'NONE', #45423, #78211, #59823, .T. ) ;
#38608=CARTESIAN_POINT ( 'NONE',  ( 179.5645164103034119, 282.8161413207554915, -15.65081265547478928 ) ) ;
#38609=CARTESIAN_POINT ( 'NONE',  ( 148.0336604448368405, 274.2451742095802842, -9.068513419098270134 ) ) ;
#38610=CARTESIAN_POINT ( 'NONE',  ( 169.2175156373457128, 285.3665543728620264, -7.678154704465813829 ) ) ;
#38611=VERTEX_POINT ( 'NONE', #94004 ) ;
#38612=CARTESIAN_POINT ( 'NONE',  ( 208.3586375946586315, 269.7592488206576604, -1.970210487958146128 ) ) ;
#38614=CARTESIAN_POINT ( 'NONE',  ( 43.23318412030275226, 195.7677522451418781, 10.00000000000009592 ) ) ;
#38615=CARTESIAN_POINT ( 'NONE',  ( 151.4376533647338476, 268.3492855237141725, -15.16853828792834236 ) ) ;
#38617=CARTESIAN_POINT ( 'NONE',  ( 196.2048238403250764, 290.8102717488927169, 17.53926796892840656 ) ) ;
#38618=CARTESIAN_POINT ( 'NONE',  ( 175.4671943841053690, 253.5411772790661757, -4.255739755355884668 ) ) ;
#38619=CARTESIAN_POINT ( 'NONE',  ( 50.02589733512838421, 205.8149278399161233, 9.188101187500093303 ) ) ;
#38620=CARTESIAN_POINT ( 'NONE',  ( 178.6804572816645589, 292.0409386983645277, -5.741727636564030846 ) ) ;
#38626=CARTESIAN_POINT ( 'NONE',  ( 26.84540973961100008, 174.7592609112379876, 2.679491924311254714 ) ) ;
#38627=CARTESIAN_POINT ( 'NONE',  ( 147.4368675721658519, 275.2788497866417288, 5.050119523016719292 ) ) ;
#38629=DIRECTION ( 'NONE',  ( 0.5000000000000048850, -0.8660254037844358210, 0.000000000000000000 ) ) ;
#38630=CARTESIAN_POINT ( 'NONE',  ( 180.9275591696145966, 262.4355116931648126, 12.34148954679617560 ) ) ;
#38632=CARTESIAN_POINT ( 'NONE',  ( 118.1443815476567352, 229.0177522451417929, 5.000000000000051514 ) ) ;
#38639=CARTESIAN_POINT ( 'NONE',  ( 147.6300909839706321, 274.9441770201837585, 8.328755691084779755 ) ) ;
#38640=CARTESIAN_POINT ( 'NONE',  ( 207.8446715390582540, 270.6494641423232679, -2.429516028743652800 ) ) ;
#38642=ADVANCED_FACE ( 'NONE', ( #58925 ), #58447, .T. ) ;
#38643=CARTESIAN_POINT ( 'NONE',  ( 26.10194555558328133, 192.0024278399160949, -9.188101187500093303 ) ) ;
#38647=CARTESIAN_POINT ( 'NONE',  ( 193.6523268064705974, 293.2313262976975352, 15.26490498002906193 ) ) ;
#38649=EDGE_CURVE ( 'NONE', #45893, #31631, #93401, .T. ) ;
#38650=CARTESIAN_POINT ( 'NONE',  ( 174.2270345836575132, 287.1587744952294088, 10.32173088169526842 ) ) ;
#38651=CARTESIAN_POINT ( 'NONE',  ( 75.14098114064213974, 208.0643266524159571, -9.188101187500093303 ) ) ;
#38652=DIRECTION ( 'NONE',  ( -0.8660254037844387076, -0.4999999999999998890, -0.000000000000000000 ) ) ;
#38658=CARTESIAN_POINT ( 'NONE',  ( 165.3960647433960673, 269.3279595906375334, 17.30649301441624743 ) ) ;
#38659=CARTESIAN_POINT ( 'NONE',  ( 35.52916646935165090, 177.9865022471901170, 1.119607411625061291E-15 ) ) ;
#38660=CARTESIAN_POINT ( 'NONE',  ( 208.0287371622045782, 270.3306531311065442, 3.558879245883286746 ) ) ;
#38661=CARTESIAN_POINT ( 'NONE',  ( -9.107486540969064848, 174.7369531367911293, -4.594050593750048428 ) ) ;
#38663=CARTESIAN_POINT ( 'NONE',  ( 167.7933980256991333, 262.5155890272394004, -16.76255740563084018 ) ) ;
#38664=CARTESIAN_POINT ( 'NONE',  ( 185.2721877113579012, 260.3715536164725677, 6.614250018501683037 ) ) ;
#38665=CARTESIAN_POINT ( 'NONE',  ( 164.5348324038273518, 245.6643059921780718, 1.473102934610569958 ) ) ;
#38674=CARTESIAN_POINT ( 'NONE',  ( 165.7158856635367670, 245.9455260183406153, -1.115825035939094878 ) ) ;
#38675=CARTESIAN_POINT ( 'NONE',  ( 200.8924071879331166, 282.0774472293816189, -16.63419059431211977 ) ) ;
#38676=CARTESIAN_POINT ( 'NONE',  ( 87.63502826371535548, 214.7365022471901739, -10.00000000000009237 ) ) ;
#38677=CARTESIAN_POINT ( 'NONE',  ( 98.24615118885414233, 215.9824982072973683, 3.021315404115420679E-15 ) ) ;
#38678=CARTESIAN_POINT ( 'NONE',  ( 208.1612901671020381, 270.1010645919285480, -2.401583477149568768 ) ) ;
#38679=CARTESIAN_POINT ( 'NONE',  ( 157.8501323257721083, 280.8042112442767007, -7.123878780571343050 ) ) ;
#38682=CARTESIAN_POINT ( 'NONE',  ( 190.4722783054066326, 281.5708337987511527, 17.36680661303515549 ) ) ;
#38685=CARTESIAN_POINT ( 'NONE',  ( 149.6896757981861583, 271.3768714794653647, 12.49809796062302603 ) ) ;
#38688=B_SPLINE_CURVE_WITH_KNOTS ( 'NONE', 3,
 ( #15708, #39493, #46610, #77540, #39005, #15204, #30921 ),
 .UNSPECIFIED., .F., .F.,
 ( 4, 3, 4 ),
 ( 0.000000000000000000, 0.001498044977029682010, 0.003457732078973784796 ),
 .UNSPECIFIED. ) ;
#38690=CARTESIAN_POINT ( 'NONE',  ( 191.0933613939813540, 299.6635844069401173, -8.689828987424775164 ) ) ;
#38692=B_SPLINE_CURVE_WITH_KNOTS ( 'NONE', 3,
 ( #17318, #32530, #79671, #33020, #78642, #9225, #25417, #55791, #49234, #86784, #56309, #94857, #48739, #63424, #95876, #10233, #41102, #48223, #40104, #87305, #94363, #72038, #2641, #33529, #63918, #80168, #79170, #25941, #56816, #24917, #71044, #80673, #18837, #40609, #10735, #96362, #87799, #9750, #18340, #72553, #3157, #71543, #88283, #34042, #64932, #26435, #1646, #57313, #11249, #3639 ),
 .UNSPECIFIED., .F., .F.,
 ( 4, 2, 2, 2, 2, 2, 2, 2, 2, 2, 2, 2, 2, 2, 2, 2, 2, 2, 2, 2, 2, 2, 2, 2, 4 ),
 ( 0.0008287262012033482601, 0.001030356982722712084, 0.001131172373482456717, 0.001231987764242201133, 0.001332803155001945766, 0.001433618545761690399, 0.001635249327281108325, 0.002038510890320054114, 0.002441772453359000554, 0.003248295579436893434, 0.004054818705514786313, 0.004861341831592680060, 0.005264603394631663796, 0.005466234176151118368, 0.005567049566910887287, 0.005617457262290818584, 0.005667864957670749881, 0.005718272653050681179, 0.005768680348430612476, 0.005869495739190313741, 0.006071126520709579227, 0.006474388083748255050, 0.006877649646786930873, 0.007079280428306236259, 0.007280911209825541644 ),
 .UNSPECIFIED. ) ;
#38693=CARTESIAN_POINT ( 'NONE',  ( 196.9728329903666122, 289.4800408803428695, -17.53478045286815856 ) ) ;
#38695=ORIENTED_EDGE ( 'NONE', *, *, #2021, .F. ) ;
#38696=CARTESIAN_POINT ( 'NONE',  ( 161.1027382213887336, 251.6088674925233022, 13.55451100897754557 ) ) ;
#38697=CARTESIAN_POINT ( 'NONE',  ( 191.4922467593309250, 298.9726946877590876, 7.604184559945784017 ) ) ;
#38698=CARTESIAN_POINT ( 'NONE',  ( 168.6888362159111523, 279.3388723634037660, -14.98891133512231377 ) ) ;
#38699=ORIENTED_EDGE ( 'NONE', *, *, #15402, .F. ) ;
#38700=ORIENTED_EDGE ( 'NONE', *, *, #87678, .T. ) ;
#38701=ORIENTED_EDGE ( 'NONE', *, *, #61502, .T. ) ;
#38708=CARTESIAN_POINT ( 'NONE',  ( 167.6203508625312963, 281.1962390192910561, 11.49557606910398633 ) ) ;
#38709=CARTESIAN_POINT ( 'NONE',  ( 194.7576540903134799, 293.3168432830895540, -14.62421624641040196 ) ) ;
#38710=EDGE_CURVE ( 'NONE', #16392, #45778, #68261, .T. ) ;
#38713=CARTESIAN_POINT ( 'NONE',  ( 203.9777429970372395, 272.3976805576900801, -11.01560090989651997 ) ) ;
#38715=CARTESIAN_POINT ( 'NONE',  ( 163.6954058318546004, 282.3930307436989438, 8.504173745411177876 ) ) ;
#38720=CARTESIAN_POINT ( 'NONE',  ( 171.1028772385554078, 259.1587979975018357, -13.89206456122039235 ) ) ;
#38721=CARTESIAN_POINT ( 'NONE',  ( 206.8775514429320026, 272.3245652858344670, -9.838455694836268250 ) ) ;
#38723=CARTESIAN_POINT ( 'NONE',  ( 165.5968251294584661, 246.8041483929534081, -2.409699260217772476 ) ) ;
#38726=CARTESIAN_POINT ( 'NONE',  ( 161.1089126327036354, 251.5981730984191529, 13.95161017039218976 ) ) ;
#38727=CARTESIAN_POINT ( 'NONE',  ( 161.2907445571653398, 283.4895778383536822, 2.139433395802937454 ) ) ;
#38729=ORIENTED_EDGE ( 'NONE', *, *, #84418, .T. ) ;
#38730=CARTESIAN_POINT ( 'NONE',  ( 155.7875766807000559, 260.8149973314318686, -17.66409480421729583 ) ) ;
#38733=CARTESIAN_POINT ( 'NONE',  ( 0.4370954166217684844, 164.3927522451417929, -10.00000000000009059 ) ) ;
#38734=CARTESIAN_POINT ( 'NONE',  ( 79.66011734693590540, 225.9869531367911293, 4.594050593750046652 ) ) ;
#38735=CARTESIAN_POINT ( 'NONE',  ( 195.3483670750180465, 269.0306795110596454, -10.80387254427798993 ) ) ;
#38736=CARTESIAN_POINT ( 'NONE',  ( 204.2446710276013846, 276.8848479354406322, -15.25810902262900193 ) ) ;
#38737=CARTESIAN_POINT ( 'NONE',  ( 173.4037495197947294, 288.6795182003594391, 9.022545291891718833 ) ) ;
#38738=CARTESIAN_POINT ( 'NONE',  ( 9.485603764116877556, 164.0327760586659451, 1.948934522072303157E-15 ) ) ;
#38739=CARTESIAN_POINT ( 'NONE',  ( 4.715407580134756138, 161.9824982072973683, 3.021315404115420679E-15 ) ) ;
#38740=VECTOR ( 'NONE', #58117, 1000.000000000000000 ) ;
#38741=CARTESIAN_POINT ( 'NONE',  ( 161.8662906133268393, 250.2863559554455719, 14.03735902266321744 ) ) ;
#38744=CARTESIAN_POINT ( 'NONE',  ( 154.0986224399686648, 280.1916420498395155, 2.233781007141098396 ) ) ;
#38747=CARTESIAN_POINT ( 'NONE',  ( 157.8811243250769110, 257.1888664433053009, -17.39256699147873064 ) ) ;
#38748=CARTESIAN_POINT ( 'NONE',  ( 162.6452507235760265, 248.9371574674245551, -11.74121925143418999 ) ) ;
#38749=CARTESIAN_POINT ( 'NONE',  ( 85.81045474425822306, 231.8967562850347122, -4.648177544792955347E-16 ) ) ;
#38750=CARTESIAN_POINT ( 'NONE',  ( 149.6148422561466305, 277.4437614652936190, 3.137689077364430368 ) ) ;
#38752=CARTESIAN_POINT ( 'NONE',  ( 15.03297158952216961, 188.6744531367911293, 4.594050593750047540 ) ) ;
#38753=CARTESIAN_POINT ( 'NONE',  ( 126.3990332750161087, 231.5327760586659736, 1.948934522072303157E-15 ) ) ;
#38755=EDGE_LOOP ( 'NONE', ( #81046, #33801, #22266, #22749 ) ) ;
#38756=CARTESIAN_POINT ( 'NONE',  ( 153.4539715540829548, 274.2402401102759768, -12.15832997750954725 ) ) ;
#38762=CARTESIAN_POINT ( 'NONE',  ( 207.1007598919583472, 271.9379569114424271, -6.086525981869248092 ) ) ;
#38763=CARTESIAN_POINT ( 'NONE',  ( 147.6095889327917803, 274.9796876144846465, -8.460961150142429332 ) ) ;
#38765=CARTESIAN_POINT ( 'NONE',  ( 189.3809998303445070, 262.9338621993890683, 7.973474124051453948 ) ) ;
#38766=CARTESIAN_POINT ( 'NONE',  ( 167.7277483666692035, 278.2164418835184279, 14.55005577363578695 ) ) ;
#38767=CARTESIAN_POINT ( 'NONE',  ( 192.5461644579549159, 265.2488509464530466, 7.905308701533972915 ) ) ;
#38769=CARTESIAN_POINT ( 'NONE',  ( 147.6947327179224487, 274.8322142526899370, 9.090449717876689206 ) ) ;
#38771=EDGE_LOOP ( 'NONE', ( #61725, #92801, #85686, #44763 ) ) ;
#38772=CARTESIAN_POINT ( 'NONE',  ( 152.7033526488152972, 266.7879839391151222, -15.74280670727761233 ) ) ;
#38773=CARTESIAN_POINT ( 'NONE',  ( 184.0878125373319847, 268.7792329301184964, 16.25146861396065390 ) ) ;
#38774=CARTESIAN_POINT ( 'NONE',  ( 100.2557178503908517, 222.5643266524160140, 9.188101187500095079 ) ) ;
#38776=CARTESIAN_POINT ( 'NONE',  ( -8.493791556357338735, 159.2365022471901455, -10.00000000000009237 ) ) ;
#38778=FACE_OUTER_BOUND ( 'NONE', #62436, .T. ) ;
#38779=CARTESIAN_POINT ( 'NONE',  ( 195.3033857398789621, 278.9466194944354811, 16.29485747049683297 ) ) ;
#38780=CARTESIAN_POINT ( 'NONE',  ( 196.4543326713419162, 290.3781097766342327, 17.78932051653062274 ) ) ;
#38781=CARTESIAN_POINT ( 'NONE',  ( 186.8613019359277985, 289.0675096450263482, -15.39881596941752839 ) ) ;
#38782=CARTESIAN_POINT ( 'NONE',  ( -22.42236680055709641, 157.8615022471902591, 0.000000000000000000 ) ) ;
#38784=CARTESIAN_POINT ( 'NONE',  ( 204.1793336335251468, 276.6190018376958051, 13.41972674969341206 ) ) ;
#38785=DIRECTION ( 'NONE',  ( -0.8660254037844387076, -0.4999999999999998890, -0.000000000000000000 ) ) ;
#38786=ORIENTED_EDGE ( 'NONE', *, *, #65428, .F. ) ;
#38787=CARTESIAN_POINT ( 'NONE',  ( 192.9292740511494912, 266.8656835997284702, 11.45998025205365423 ) ) ;
#38791=CARTESIAN_POINT ( 'NONE',  ( 196.7823306783968746, 289.8100005636337073, -17.85370042640856170 ) ) ;
#38795=CARTESIAN_POINT ( 'NONE',  ( 183.3038736369663582, 264.5073148912692886, -13.20120179016996254 ) ) ;
#38798=CARTESIAN_POINT ( 'NONE',  ( 192.1859061758433143, 297.7712413352111298, 11.15082371775444336 ) ) ;
#38799=CARTESIAN_POINT ( 'NONE',  ( 189.4188400755406292, 280.0569678547571471, 16.65366941511145527 ) ) ;
#38802=CARTESIAN_POINT ( 'NONE',  ( 169.2713223461767313, 284.8094741354592543, 10.92384103809050444 ) ) ;
#38804=CARTESIAN_POINT ( 'NONE',  ( -22.42236680055709641, 157.8615022471902591, 0.000000000000000000 ) ) ;
#38805=VERTEX_POINT ( 'NONE', #6246 ) ;
#38807=CARTESIAN_POINT ( 'NONE',  ( 159.0779171328172481, 255.1159604941658472, 17.23506282224926522 ) ) ;
#38809=CARTESIAN_POINT ( 'NONE',  ( 192.6084828143412437, 297.0393171272406221, -13.31966769178241705 ) ) ;
#38814=CARTESIAN_POINT ( 'NONE',  ( 175.7824178399792174, 285.8628427244275372, -13.39878279634721103 ) ) ;
#38819=ORIENTED_EDGE ( 'NONE', *, *, #57166, .F. ) ;
#38822=CARTESIAN_POINT ( 'NONE',  ( 190.6473439991314933, 300.0390052271857826, -3.781200630501462268 ) ) ;
#38823=CARTESIAN_POINT ( 'NONE',  ( 164.2901811315512077, 246.0880544258967575, -1.801919852217561235 ) ) ;
#38824=CARTESIAN_POINT ( 'NONE',  ( 199.2409351612726027, 274.1797303067421012, -13.51492913604719703 ) ) ;
#38827=CARTESIAN_POINT ( 'NONE',  ( 171.2101627772172492, 250.9235556046914155, -5.579768846723117015 ) ) ;
#38829=EDGE_CURVE ( 'NONE', #4704, #96078, #1721, .T. ) ;
#38830=CARTESIAN_POINT ( 'NONE',  ( 183.4135727292207605, 284.6015171189660578, -15.04630399923350659 ) ) ;
#38831=CARTESIAN_POINT ( 'NONE',  ( 113.4351080945290278, 245.4869531367911009, 4.594050593750046652 ) ) ;
#38832=CARTESIAN_POINT ( 'NONE',  ( 186.6240524511718206, 262.8751839256129301, -9.355389698624779982 ) ) ;
#38834=CARTESIAN_POINT ( 'NONE',  ( 177.0439216176413879, 289.2672441982131204, -10.54826698963404041 ) ) ;
#38836=EDGE_LOOP ( 'NONE', ( #40555, #51922, #7620, #32089, #29017 ) ) ;
#38839=CARTESIAN_POINT ( 'NONE',  ( 171.1102460733511066, 287.7606437450009480, -4.678464158645172510 ) ) ;
#38840=CARTESIAN_POINT ( 'NONE',  ( 196.2048238403250764, 290.8102717488927169, 17.53926796892840656 ) ) ;
#38843=DIRECTION ( 'NONE',  ( 0.4999999999999992784, -0.8660254037844390407, 0.000000000000000000 ) ) ;
#38845=ORIENTED_EDGE ( 'NONE', *, *, #80179, .F. ) ;
#38846=CARTESIAN_POINT ( 'NONE',  ( 153.5824857651062416, 266.9593715351384731, 16.60156113108486764 ) ) ;
#38847=EDGE_CURVE ( 'NONE', #55003, #91593, #59024, .T. ) ;
#38850=CARTESIAN_POINT ( 'NONE',  ( 148.3253847707240141, 273.7398928553401447, -9.074433450356286457 ) ) ;
#38851=CARTESIAN_POINT ( 'NONE',  ( 3.808674319871268921, 184.5530062829863027, -4.648177544792955347E-16 ) ) ;
#38853=CARTESIAN_POINT ( 'NONE',  ( 188.1446237001680970, 265.8515323599089584, -11.63103201079399440 ) ) ;
#38855=CARTESIAN_POINT ( 'NONE',  ( 190.6739029791876305, 284.0814300001334800, -17.04622756081775492 ) ) ;
#38856=CARTESIAN_POINT ( 'NONE',  ( 192.3824498117414237, 262.8597123339034738, 4.564481591547765227 ) ) ;
#38858=CARTESIAN_POINT ( 'NONE',  ( 204.6497552248077341, 273.0205207247614680, -10.58234289185253196 ) ) ;
#38859=CARTESIAN_POINT ( 'NONE',  ( 153.2402432998383972, 270.1751345723797044, 14.03626019444179818 ) ) ;
#38860=CARTESIAN_POINT ( 'NONE',  ( 156.8342227191775464, 280.4122116305982217, 5.959992801529873319 ) ) ;
#38861=CARTESIAN_POINT ( 'NONE',  ( 201.0844796915553161, 282.3584598911111812, -16.59562674965125950 ) ) ;
#38862=ORIENTED_EDGE ( 'NONE', *, *, #84985, .T. ) ;
#38863=CARTESIAN_POINT ( 'NONE',  ( 147.2443490232117256, 275.6123016948292275, 5.226063659459642352 ) ) ;
#38867=CARTESIAN_POINT ( 'NONE',  ( 26.27351996285747049, 192.6427522451419634, -10.00000000000009592 ) ) ;
#38868=CARTESIAN_POINT ( 'NONE',  ( 188.5899576770683836, 298.6136929722685522, -4.164154921440024637 ) ) ;
#38870=CARTESIAN_POINT ( 'NONE',  ( 170.7312474266366564, 253.4461053635303358, 11.28381232434868764 ) ) ;
#38872=CARTESIAN_POINT ( 'NONE',  ( -13.03246669095222998, 174.8297689869269220, -2.679491924311245832 ) ) ;
#38873=CARTESIAN_POINT ( 'NONE',  ( 191.5677310693528170, 283.6434865987201874, -16.60331218763614558 ) ) ;
#38874=EDGE_CURVE ( 'NONE', #39182, #31533, #19841, .T. ) ;
#38876=CARTESIAN_POINT ( 'NONE',  ( 74.97842782955004282, 214.0958772461660544, -9.188101187500095079 ) ) ;
#38879=CARTESIAN_POINT ( 'NONE',  ( 180.2008674086625888, 256.3788900776044102, -7.862092545524210330 ) ) ;
#38880=CARTESIAN_POINT ( 'NONE',  ( 154.8545429534089237, 262.4310591522755089, -17.81746354318405778 ) ) ;
#38881=B_SPLINE_CURVE_WITH_KNOTS ( 'NONE', 3,
 ( #93874, #94862, #2144, #62923, #32014, #39601, #24431, #25422, #47221, #33025, #31511, #41109, #17845, #78143, #86288, #56821, #62406, #15818, #70016, #93362, #8729, #79175, #25947, #95393, #78647, #54817, #85797, #63924, #71548, #70521, #23919, #32535, #55306, #39102, #48745, #1136, #9754, #24923, #16822, #46722 ),
 .UNSPECIFIED., .F., .F.,
 ( 4, 2, 2, 2, 2, 2, 2, 2, 2, 2, 2, 2, 2, 2, 2, 2, 2, 2, 2, 4 ),
 ( 0.0009045477389935737030, 0.0009985104552911751828, 0.001092473171588776446, 0.001280398604183980490, 0.001656249469374568989, 0.002407951199755620220, 0.003911354660517611659, 0.004663056390898655951, 0.005038907256089211056, 0.005226832688684499018, 0.005320795404982177693, 0.005414758121279858102, 0.005461739479428661878, 0.005508720837577467389, 0.005602683553875100961, 0.005790608986470392391, 0.005978534419065682087, 0.006166459851660971783, 0.006542310716851552910, 0.006918161582042132302 ),
 .UNSPECIFIED. ) ;
#38884=FACE_OUTER_BOUND ( 'NONE', #15903, .T. ) ;
#38888=CARTESIAN_POINT ( 'NONE',  ( 169.2950589356292710, 252.1013886194228348, -9.631404982488993127 ) ) ;
#38889=CARTESIAN_POINT ( 'NONE',  ( 204.9769638368455844, 275.6164795838122927, -13.69608158933077746 ) ) ;
#38890=CARTESIAN_POINT ( 'NONE',  ( 168.3110316854768485, 273.6977835318167536, 17.00254241999702387 ) ) ;
#38891=CARTESIAN_POINT ( 'NONE',  ( 157.7861133721078772, 257.3534302411229646, 18.03837896619386783 ) ) ;
#38893=CARTESIAN_POINT ( 'NONE',  ( 45.07374842694240868, 187.6423013555410080, -4.594050593750043987 ) ) ;
#38894=CARTESIAN_POINT ( 'NONE',  ( 64.36996372895568186, 195.7202760586659167, -5.415160957724236172E-17 ) ) ;
#38898=CARTESIAN_POINT ( 'NONE',  ( 139.4158702080621879, 260.4869531367911009, 4.594050593750046652 ) ) ;
#38899=EDGE_CURVE ( 'NONE', #78035, #60981, #35618, .T. ) ;
#38900=CARTESIAN_POINT ( 'NONE',  ( 197.1913910522388846, 270.0342516794337371, -10.84445706988983460 ) ) ;
#38902=CARTESIAN_POINT ( 'NONE',  ( 137.3333197629383449, 238.5494855054051868, -2.679491924311248496 ) ) ;
#38903=CARTESIAN_POINT ( 'NONE',  ( 148.9831146496684084, 272.6006712873522133, -12.63706091291043343 ) ) ;
#38905=CARTESIAN_POINT ( 'NONE',  ( 61.82584055745639517, 200.3768266524159856, -9.188101187500093303 ) ) ;
#38906=CARTESIAN_POINT ( 'NONE',  ( 159.0704364050992297, 255.7598713771850782, -16.06560598622004576 ) ) ;
#38908=CARTESIAN_POINT ( 'NONE',  ( 159.2303255284352304, 254.8519814094557603, 16.39103317446447150 ) ) ;
#38910=CARTESIAN_POINT ( 'NONE',  ( 153.3733417098790426, 276.7809054075530639, 7.651122506530271927 ) ) ;
#38912=CARTESIAN_POINT ( 'NONE',  ( 102.2852913444020686, 239.8615022471903160, 5.000000000000046185 ) ) ;
#38913=( BOUNDED_CURVE ( )  B_SPLINE_CURVE ( 2, ( #68760, #59658, #99685, #69263, #21193, #92607, #30268, #52071, #75902 ),
 .UNSPECIFIED., .F., .T. ) 
 B_SPLINE_CURVE_WITH_KNOTS ( ( 3, 2, 2, 2, 3 ),
 ( 0.02822580645161290591, 0.02956989247311828106, 0.03225806451612903136, 0.03494623655913978166, 0.03629032258064516375 ),
 .UNSPECIFIED. ) 
 CURVE ( )  GEOMETRIC_REPRESENTATION_ITEM ( )  RATIONAL_B_SPLINE_CURVE ( ( 0.9330127018922192983, 0.9330127018922194093, 1.000000000000000000, 0.8660254037844387076, 1.000000000000000000, 0.8660254037844387076, 1.000000000000000000, 0.9330127018922191873, 0.9330127018922194093 ) ) 
 REPRESENTATION_ITEM ( '' )  );
#38914=CARTESIAN_POINT ( 'NONE',  ( 161.6707029936031574, 250.6251236501384483, 14.45053103226186231 ) ) ;
#38915=CARTESIAN_POINT ( 'NONE',  ( 207.4285356523023154, 271.3702326410368642, 7.833982582429932506 ) ) ;
#38916=ORIENTED_EDGE ( 'NONE', *, *, #19780, .T. ) ;
#38920=CARTESIAN_POINT ( 'NONE',  ( 206.7923762329701276, 272.4720930770340033, -9.496103119940368487 ) ) ;
#38921=CARTESIAN_POINT ( 'NONE',  ( 186.8221477911302770, 276.5908659110200460, -17.12696914844746843 ) ) ;
#38923=ORIENTED_EDGE ( 'NONE', *, *, #48838, .T. ) ;
#38924=CARTESIAN_POINT ( 'NONE',  ( 173.6959472565854981, 251.9178171641904953, -0.2492449988941567163 ) ) ;
#38927=CARTESIAN_POINT ( 'NONE',  ( 194.6356465353167948, 293.5281665672507643, -16.13180903283129197 ) ) ;
#38928=DIRECTION ( 'NONE',  ( -0.8660254037844387076, -0.4999999999999998890, -0.000000000000000000 ) ) ;
#38932=CARTESIAN_POINT ( 'NONE',  ( 152.3360070569975449, 270.2436951681156643, -14.78697292633622951 ) ) ;
#38937=ORIENTED_EDGE ( 'NONE', *, *, #64057, .T. ) ;
#38938=AXIS2_PLACEMENT_3D ( 'NONE', #36567, #23356, #22371 ) ;
#38940=CARTESIAN_POINT ( 'NONE',  ( 163.2758796796684067, 283.7716228465783956, -2.991217566210298884 ) ) ;
#38942=CARTESIAN_POINT ( 'NONE',  ( 207.5886452961740076, 271.0929146030698007, -1.661373005306138184 ) ) ;
#38943=CARTESIAN_POINT ( 'NONE',  ( 164.1259971043086239, 246.3724295028720519, 5.761669507629934905 ) ) ;
#38945=CARTESIAN_POINT ( 'NONE',  ( 157.6668627405778409, 257.5599783937680058, -16.78811156090270629 ) ) ;
#38947=CARTESIAN_POINT ( 'NONE',  ( 144.4230134433972523, 248.0643266524160140, 9.188101187500095079 ) ) ;
#38948=CARTESIAN_POINT ( 'NONE',  ( 206.4992971559627506, 270.5621682591477111, 2.903359756976243933 ) ) ;
#38949=CARTESIAN_POINT ( 'NONE',  ( 178.8741573099551943, 257.7081751745919291, 10.05521247607878088 ) ) ;
#38950=CARTESIAN_POINT ( 'NONE',  ( 77.57650404090335883, 215.5958772461660544, -9.188101187500095079 ) ) ;
#38952=CARTESIAN_POINT ( 'NONE',  ( 191.3375250863502970, 299.2406804863936145, 8.828791580707859410 ) ) ;
#38955=CARTESIAN_POINT ( 'NONE',  ( 177.6444986370304946, 293.6980009803469329, 2.770296639708824227 ) ) ;
#38956=ORIENTED_EDGE ( 'NONE', *, *, #63360, .F. ) ;
#38957=B_SPLINE_CURVE_WITH_KNOTS ( 'NONE', 3,
 ( #7849, #92969, #46318, #76270 ),
 .UNSPECIFIED., .F., .F.,
 ( 4, 4 ),
 ( 0.002878795719159728261, 0.006003557113845784873 ),
 .UNSPECIFIED. ) ;
#38959=CARTESIAN_POINT ( 'NONE',  ( 191.5521510896938935, 298.8689373439769952, -9.847378829740700112 ) ) ;
#38962=EDGE_CURVE ( 'NONE', #46531, #81472, #48902, .T. ) ;
#38964=CARTESIAN_POINT ( 'NONE',  ( 76.33141897508073725, 221.0024278399160949, 9.188101187500095079 ) ) ;
#38968=CARTESIAN_POINT ( 'NONE',  ( 201.0785059933280650, 282.3688066399498098, -17.20790163225820280 ) ) ;
#38969=EDGE_CURVE ( 'NONE', #346, #87238, #88794, .T. ) ;
#38974=CARTESIAN_POINT ( 'NONE',  ( 196.4287751515431921, 269.1031666285815618, -12.09581130873691279 ) ) ;
#38975=DIRECTION ( 'NONE',  ( -0.8660254037844387076, -0.4999999999999998890, -0.000000000000000000 ) ) ;
#38976=CARTESIAN_POINT ( 'NONE',  ( 162.8777320348721673, 261.4784687625029278, 17.43788665286368911 ) ) ;
#38980=CARTESIAN_POINT ( 'NONE',  ( 155.8995516477446301, 262.1116139477605884, -16.97658656424888335 ) ) ;
#38981=CARTESIAN_POINT ( 'NONE',  ( 153.1961624462112752, 265.3034584490234806, -16.19494717845262954 ) ) ;
#38982=B_SPLINE_CURVE_WITH_KNOTS ( 'NONE', 3,
 ( #22177, #15058, #6485, #22683, #76395, #100195, #38860, #31262, #62149, #69266, #45949, #67780, #44966, #53070, #23157, #77382, #68268, #93095, #29289, #99191, #91605, #45462, #6971, #7984, #36874, #37855, #68764, #38356, #61161, #92610, #30780, #69766, #77890, #24174, #70261, #48479, #79421, #1883, #25687, #95122, #40847, #1386, #869, #40353, #62653, #17572, #39346, #86040, #56567, #71793 ),
 .UNSPECIFIED., .F., .F.,
 ( 4, 2, 2, 2, 2, 2, 2, 2, 2, 2, 2, 2, 2, 2, 2, 2, 2, 2, 2, 2, 2, 2, 2, 2, 4 ),
 ( 0.0005289711837892736640, 0.0009717741654603732774, 0.001193175656295859116, 0.001303876401713549397, 0.001414577147131239462, 0.001525277892548929960, 0.001635978637966619808, 0.001857380128802034198, 0.002300183110472862544, 0.003185789073814480638, 0.004071395037156097865, 0.004957001000497714659, 0.005399803982168523489, 0.005621205473003964767, 0.005731906218421648977, 0.005787256591130453785, 0.005842606963839258594, 0.005897957336548063402, 0.005953307709256868210, 0.006064008454674477827, 0.006285409945509695326, 0.006728212927180128589, 0.007171015908850563586, 0.007392417399685759401, 0.007613818890520955215 ),
 .UNSPECIFIED. ) ;
#38986=CARTESIAN_POINT ( 'NONE',  ( 199.8133446373031177, 266.7051771727681739, 4.672154848026198515 ) ) ;
#38987=CARTESIAN_POINT ( 'NONE',  ( 148.2604030792711853, 276.0951355443942248, -3.828504021689099979 ) ) ;
#38989=CARTESIAN_POINT ( 'NONE',  ( 187.8793669350804123, 266.2890599608011826, -12.74918944048514469 ) ) ;
#38990=CARTESIAN_POINT ( 'NONE',  ( 198.6619468263075419, 265.9559996360017635, 1.504078954549255220 ) ) ;
#38991=CARTESIAN_POINT ( 'NONE',  ( 156.6340579379407245, 272.3087899941822343, 14.25056221956334923 ) ) ;
#38992=ORIENTED_EDGE ( 'NONE', *, *, #5397, .F. ) ;
#38994=CARTESIAN_POINT ( 'NONE',  ( 202.3425522658138505, 280.1794142728863903, 15.86053073629060961 ) ) ;
#38995=CARTESIAN_POINT ( 'NONE',  ( 156.6084421796713002, 261.3932165810376205, -17.82046942966612590 ) ) ;
#38996=CARTESIAN_POINT ( 'NONE',  ( 194.4904290197884507, 293.7796906822950973, 14.50206953321744940 ) ) ;
#38998=CARTESIAN_POINT ( 'NONE',  ( 178.3271064952729716, 287.7206632098644263, -13.02025800059123561 ) ) ;
#39000=CARTESIAN_POINT ( 'NONE',  ( 168.6260063310307373, 273.1609051843404927, 15.95833444951868429 ) ) ;
#39002=CARTESIAN_POINT ( 'NONE',  ( 180.0662822340164269, 262.4007578510376675, -14.24330825748563534 ) ) ;
#39003=CARTESIAN_POINT ( 'NONE',  ( 188.2447773146031409, 260.7966381918191701, 3.249388362550839293 ) ) ;
#39004=CARTESIAN_POINT ( 'NONE',  ( -6.536213301660246167, 167.0333772461660828, 9.188101187500095079 ) ) ;
#39005=CARTESIAN_POINT ( 'NONE',  ( 189.6561516143011659, 295.9170104107913062, -11.61052802970076314 ) ) ;
#39007=CARTESIAN_POINT ( 'NONE',  ( 175.3074307085254020, 254.5436327766159650, 9.407465564047683415 ) ) ;
#39010=CARTESIAN_POINT ( 'NONE',  ( 20.93329029645117245, 173.7048013555409796, 4.594050593750051981 ) ) ;
#39012=CARTESIAN_POINT ( 'NONE',  ( 181.9693517213364089, 275.7599053639374915, -16.43459007604911548 ) ) ;
#39014=CARTESIAN_POINT ( 'NONE',  ( 147.2229325088103735, 275.6493961858936927, -0.4918294119671829390 ) ) ;
#39017=CARTESIAN_POINT ( 'NONE',  ( 187.7221740047435219, 259.7727845006203893, -0.7698188447816332047 ) ) ;
#39018=CARTESIAN_POINT ( 'NONE',  ( 71.97440221194672461, 212.3615022471902591, -10.00000000000009592 ) ) ;
#39020=DIRECTION ( 'NONE',  ( 0.4999999999999998890, -0.8660254037844385966, 0.000000000000000000 ) ) ;
#39021=CARTESIAN_POINT ( 'NONE',  ( 28.21305602519035460, 187.0958772461660544, -9.188101187500095079 ) ) ;
#39023=EDGE_CURVE ( 'NONE', #8043, #33367, #94865, .T. ) ;
#39025=CARTESIAN_POINT ( 'NONE',  ( 202.9963324477415654, 270.0117979724515749, -6.355055958317759490 ) ) ;
#39026=CARTESIAN_POINT ( 'NONE',  ( 198.9590707264871412, 286.0397762054715827, -17.05306195936250191 ) ) ;
#39029=CARTESIAN_POINT ( 'NONE',  ( 159.8940227261901157, 278.4197979795083597, -10.01923854142061998 ) ) ;
#39030=CARTESIAN_POINT ( 'NONE',  ( -16.26211276271276418, 167.1916292661124714, 6.123233995736853057E-16 ) ) ;
#39044=VERTEX_POINT ( 'NONE', #82685 ) ;
#39045=EDGE_LOOP ( 'NONE', ( #37132, #67012, #77015, #72028 ) ) ;
#39046=CARTESIAN_POINT ( 'NONE',  ( 189.6119997129436854, 274.5211355351512452, -16.98768979124082534 ) ) ;
#39048=ORIENTED_EDGE ( 'NONE', *, *, #38570, .T. ) ;
#39049=CARTESIAN_POINT ( 'NONE',  ( 191.1489696025915919, 299.5672681643093256, 8.892130899335590755 ) ) ;
#39053=CARTESIAN_POINT ( 'NONE',  ( 147.6430623265936219, 274.9217099957185155, 8.258152514891218487 ) ) ;
#39056=CARTESIAN_POINT ( 'NONE',  ( 195.7617614321055157, 291.5776783508526364, 16.33009124109666033 ) ) ;
#39057=CARTESIAN_POINT ( 'NONE',  ( 178.2682848727497742, 278.5227009152765163, -17.33614543379448136 ) ) ;
#39058=VERTEX_POINT ( 'NONE', #68416 ) ;
#39060=ADVANCED_FACE ( 'NONE', ( #400 ), #1983, .F. ) ;
#39061=CARTESIAN_POINT ( 'NONE',  ( 190.6023073677431512, 300.5141149296460981, 3.174888932019753973 ) ) ;
#39063=ORIENTED_EDGE ( 'NONE', *, *, #14341, .F. ) ;
#39064=CARTESIAN_POINT ( 'NONE',  ( 207.1610391518539984, 269.8335501706607715, 0.000000000000000000 ) ) ;
#39065=CARTESIAN_POINT ( 'NONE',  ( 184.1240780222136095, 289.0015729834078684, -14.54488561116068901 ) ) ;
#39066=CARTESIAN_POINT ( 'NONE',  ( 185.4867332780130766, 297.4061142773095412, 5.671143563000668131 ) ) ;
#39072=CARTESIAN_POINT ( 'NONE',  ( 199.9502294570856407, 265.6703872523112295, 6.360370400932541246E-13 ) ) ;
#39073=CARTESIAN_POINT ( 'NONE',  ( 147.6857584380539095, 274.8477581613835810, 8.112022437684441201 ) ) ;
#39075=CARTESIAN_POINT ( 'NONE',  ( 190.0896302098338424, 301.4020978150248311, 3.433521196325825642 ) ) ;
#39076=CARTESIAN_POINT ( 'NONE',  ( 132.4598011448335058, 258.8297689869269220, -2.679491924311252493 ) ) ;
#39077=CARTESIAN_POINT ( 'NONE',  ( 161.1061647010182583, 251.6029326557136585, -13.56144933775657613 ) ) ;
#39078=EDGE_CURVE ( 'NONE', #15116, #3513, #58571, .T. ) ;
#39079=CARTESIAN_POINT ( 'NONE',  ( 146.7842303614460207, 276.4092505945183689, -4.491116827832889236 ) ) ;
#39080=CARTESIAN_POINT ( 'NONE',  ( 159.9162261860523699, 255.4583558200632751, 16.33510284766913045 ) ) ;
#39082=CARTESIAN_POINT ( 'NONE',  ( 85.92648014804265699, 231.9637435831425023, 2.679491924311251605 ) ) ;
#39086=CARTESIAN_POINT ( 'NONE',  ( 121.0403275412173656, 234.5643266524160140, 9.188101187500095079 ) ) ;
#39088=CARTESIAN_POINT ( 'NONE',  ( 149.0702641876670214, 272.4497238596823649, -12.82991616757612974 ) ) ;
#39090=CARTESIAN_POINT ( 'NONE',  ( 176.5752601597114335, 288.5842064133888130, 11.38490813771325350 ) ) ;
#39091=CARTESIAN_POINT ( 'NONE',  ( 155.6048174803203210, 261.1315455520403361, -17.38645169541727498 ) ) ;
#39092=B_SPLINE_CURVE_WITH_KNOTS ( 'NONE', 3,
 ( #28293, #98221, #92153, #22197 ),
 .UNSPECIFIED., .F., .F.,
 ( 4, 4 ),
 ( 1.001342737176739535E-16, 0.002470176110450654407 ),
 .UNSPECIFIED. ) ;
#39093=CARTESIAN_POINT ( 'NONE',  ( 183.2867325885053731, 284.6525227658081008, -14.98979207437814942 ) ) ;
#39095=CARTESIAN_POINT ( 'NONE',  ( 169.3011938600986355, 285.2037582914177847, -7.848347211270669810 ) ) ;
#39096=ORIENTED_EDGE ( 'NONE', *, *, #90618, .F. ) ;
#39100=CARTESIAN_POINT ( 'NONE',  ( 128.5097966488581562, 238.8768266524159856, 9.188101187500096856 ) ) ;
#39101=CARTESIAN_POINT ( 'NONE',  ( 150.9115585710837877, 269.2605084359132093, -15.80434701481532578 ) ) ;
#39102=CARTESIAN_POINT ( 'NONE',  ( 185.6974139818678395, 297.0515939156086915, 4.189404417500578681 ) ) ;
#39103=CARTESIAN_POINT ( 'NONE',  ( 187.8012813670164007, 281.6076117757134512, -17.61501541281564442 ) ) ;
#39105=CARTESIAN_POINT ( 'NONE',  ( 40.25596147474394826, 203.2369531367911293, -4.594050593750048428 ) ) ;
#39107=VERTEX_POINT ( 'NONE', #53684 ) ;
#39109=CARTESIAN_POINT ( 'NONE',  ( 187.7806315037265108, 258.7815634600612498, -2.095649164382547003 ) ) ;
#39112=B_SPLINE_CURVE_WITH_KNOTS ( 'NONE', 3,
 ( #48410, #93544, #94047, #32200 ),
 .UNSPECIFIED., .F., .F.,
 ( 4, 4 ),
 ( 0.007058328506315592749, 0.01518834970152095967 ),
 .UNSPECIFIED. ) ;
#39115=CARTESIAN_POINT ( 'NONE',  ( 203.5258219653775313, 278.1299310341851765, -16.21052911601769608 ) ) ;
#39116=CARTESIAN_POINT ( 'NONE',  ( 178.3765882103122635, 261.1946448298811561, 12.30242364351752471 ) ) ;
#39117=CARTESIAN_POINT ( 'NONE',  ( 109.5562962934610738, 227.3927522451417929, -10.00000000000009059 ) ) ;
#39118=CARTESIAN_POINT ( 'NONE',  ( 193.9796946036068164, 292.6643086402947915, -15.64068455845557537 ) ) ;
#39120=CARTESIAN_POINT ( 'NONE',  ( 147.7157269441172218, 274.7958511862549926, 8.036290321896261801 ) ) ;
#39123=CARTESIAN_POINT ( 'NONE',  ( 29.05227845693028854, 178.3923013555409796, 4.594050593750050204 ) ) ;
#39128=CARTESIAN_POINT ( 'NONE',  ( 176.7336046869569088, 287.5723076295245733, 10.59130312256274564 ) ) ;
#39129=CARTESIAN_POINT ( 'NONE',  ( 69.56611615166231388, 198.7202760586659736, -5.415160957724236172E-17 ) ) ;
#39131=CARTESIAN_POINT ( 'NONE',  ( 208.3132655666949233, 269.8378354783333180, 2.688523655043302707 ) ) ;
#39136=CARTESIAN_POINT ( 'NONE',  ( 29.10614472461704949, 177.6115022471902023, -5.000000000000041744 ) ) ;
#39137=DIRECTION ( 'NONE',  ( 0.8660254037844395958, 0.4999999999999985567, 0.000000000000000000 ) ) ;
#39138=CARTESIAN_POINT ( 'NONE',  ( -7.645548028435306342, 157.2048013555409796, 4.594050593750051981 ) ) ;
#39140=CARTESIAN_POINT ( 'NONE',  ( 164.2175316724671177, 260.1791609587825178, -16.14942496352231416 ) ) ;
#39141=CARTESIAN_POINT ( 'NONE',  ( 200.2855905910826664, 282.2403571352788276, 17.19125751069146801 ) ) ;
#39142=ADVANCED_FACE ( 'NONE', ( #60283 ), #8113, .T. ) ;
#39143=CARTESIAN_POINT ( 'NONE',  ( 185.5939859232946674, 260.4830921086240210, 6.337058001680582642 ) ) ;
#39144=CARTESIAN_POINT ( 'NONE',  ( 164.8849641302980444, 245.0578600525887794, 2.884140591399200648 ) ) ;
#39148=CARTESIAN_POINT ( 'NONE',  ( 181.7987620307110603, 287.9999103646144363, 13.73581616295024688 ) ) ;
#39149=CARTESIAN_POINT ( 'NONE',  ( 196.6975304897132162, 289.5045102203591796, 16.45742868403355530 ) ) ;
#39151=ORIENTED_EDGE ( 'NONE', *, *, #29961, .F. ) ;
#39152=CARTESIAN_POINT ( 'NONE',  ( 206.4829433911860406, 273.0080464805345173, 8.621361281597655690 ) ) ;
#39153=CARTESIAN_POINT ( 'NONE',  ( 157.1002372043759010, 258.5414026113353430, -17.73553732786789539 ) ) ;
#39155=EDGE_CURVE ( 'NONE', #85624, #4197, #24659, .T. ) ;
#39156=CARTESIAN_POINT ( 'NONE',  ( 192.6470966816805230, 296.9724359471326807, 11.11268290051284424 ) ) ;
#39158=B_SPLINE_CURVE_WITH_KNOTS ( 'NONE', 3,
 ( #24259, #55137, #86122, #86616 ),
 .UNSPECIFIED., .F., .F.,
 ( 4, 4 ),
 ( 0.008993077315648693310, 0.01492662969474104623 ),
 .UNSPECIFIED. ) ;
#39159=CARTESIAN_POINT ( 'NONE',  ( 149.8083888948594335, 271.5779462620446338, 11.70101749353969645 ) ) ;
#39160=CARTESIAN_POINT ( 'NONE',  ( 162.6262389125959373, 248.9700868899859074, -10.50380342094597808 ) ) ;
#39161=CARTESIAN_POINT ( 'NONE',  ( 201.3505934466285510, 281.8975373467312693, -16.83770227898004279 ) ) ;
#39162=VERTEX_POINT ( 'NONE', #504 ) ;
#39167=CARTESIAN_POINT ( 'NONE',  ( 198.4097421844162170, 265.0824675037606539, -3.039349057205883664 ) ) ;
#39169=ORIENTED_EDGE ( 'NONE', *, *, #21839, .T. ) ;
#39172=CARTESIAN_POINT ( 'NONE',  ( 196.5114383562724072, 290.2791998289336561, -17.87308875047256862 ) ) ;
#39175=EDGE_LOOP ( 'NONE', ( #42597, #18688, #82131 ) ) ;
#39176=CARTESIAN_POINT ( 'NONE',  ( 200.5810378487751393, 283.2304467414622877, 18.38516374632547112 ) ) ;
#39177=CARTESIAN_POINT ( 'NONE',  ( 151.2648146047323507, 268.6486510375538614, 15.71323890031163550 ) ) ;
#39178=CARTESIAN_POINT ( 'NONE',  ( 179.4722142099873565, 269.7276464518548096, -17.35046799866735157 ) ) ;
#39180=EDGE_CURVE ( 'NONE', #13801, #16332, #60886, .T. ) ;
#39182=VERTEX_POINT ( 'NONE', #78016 ) ;
#39184=VERTEX_POINT ( 'NONE', #52691 ) ;
#39185=CARTESIAN_POINT ( 'NONE',  ( 160.5099781893591455, 258.1706592185460067, -17.21824937912870013 ) ) ;
#39188=CARTESIAN_POINT ( 'NONE',  ( 208.1876422586379647, 270.0554214305024630, 3.377638779759113863 ) ) ;
#39190=CARTESIAN_POINT ( 'NONE',  ( 167.7205243766922536, 281.0751846570960879, 11.60013190390802151 ) ) ;
#39191=CARTESIAN_POINT ( 'NONE',  ( 147.7467138384290308, 274.7421803109381813, -9.190172068879620682 ) ) ;
#39194=EDGE_CURVE ( 'NONE', #74996, #20915, #90151, .T. ) ;
#39195=CARTESIAN_POINT ( 'NONE',  ( 190.3443929803903814, 298.9608357525441420, -8.219721500574586059 ) ) ;
#39197=CARTESIAN_POINT ( 'NONE',  ( 164.5259176133158689, 246.1953198488120051, 1.882264443804981813 ) ) ;
#39199=CARTESIAN_POINT ( 'NONE',  ( 198.3993091967326166, 277.2393576875207373, -15.29194110241194160 ) ) ;
#39201=CARTESIAN_POINT ( 'NONE',  ( 198.1230806404959139, 287.4877535090322453, 17.00698319228197164 ) ) ;
#39202=VERTEX_POINT ( 'NONE', #46082 ) ;
#39206=EDGE_CURVE ( 'NONE', #62642, #82127, #44021, .T. ) ;
#39207=CARTESIAN_POINT ( 'NONE',  ( 159.8597520197352537, 253.7617827468940277, -16.74905990210778839 ) ) ;
#39209=( BOUNDED_CURVE ( )  B_SPLINE_CURVE ( 2, ( #17070, #71800, #94615, #9993, #48486, #87046, #25172, #32771, #56053 ),
 .UNSPECIFIED., .F., .T. ) 
 B_SPLINE_CURVE_WITH_KNOTS ( ( 3, 2, 2, 2, 3 ),
 ( 0.5685483870967742437, 0.5698924731182796188, 0.5725806451612903691, 0.5752688172043011194, 0.5766129032258064946 ),
 .UNSPECIFIED. ) 
 CURVE ( )  GEOMETRIC_REPRESENTATION_ITEM ( )  RATIONAL_B_SPLINE_CURVE ( ( 0.9330127018922194093, 0.9330127018922194093, 1.000000000000000000, 0.8660254037844387076, 1.000000000000000000, 0.8660254037844387076, 1.000000000000000000, 0.9330127018922194093, 0.9330127018922194093 ) ) 
 REPRESENTATION_ITEM ( '' )  );
#39214=B_SPLINE_CURVE_WITH_KNOTS ( 'NONE', 3,
 ( #44742, #15844, #45738, #23440, #29081, #68552, #45253, #37641, #21466, #159, #69048, #46753, #99978, #77154, #30562, #76188, #53353, #60945, #38130, #52354, #69554, #85301, #77680, #13863, #92886, #6262, #61446, #37158, #68057, #53834, #84794, #7756, #71574, #86817, #94890, #39627, #93393, #62950, #40134, #47736, #87340, #2171, #85825, #41642, #49263, #17872, #48769, #8755 ),
 .UNSPECIFIED., .F., .F.,
 ( 4, 2, 2, 2, 2, 2, 2, 2, 2, 2, 2, 2, 2, 2, 2, 2, 2, 2, 2, 2, 2, 2, 2, 4 ),
 ( 0.002781645625483006659, 0.003194136222294276066, 0.003297258871497089731, 0.003400381520699903397, 0.003503504169902717062, 0.003606626819105530728, 0.003812872117511218774, 0.004019117415916907687, 0.004431608012728316739, 0.005256589206351068057, 0.006081570399973819374, 0.006906551593596570691, 0.007731532787219322009, 0.007834655436422123531, 0.007886216761023559854, 0.007937778085624996177, 0.007989339410226430765, 0.008040900734827867088, 0.008144023384030739734, 0.008556513980842487058, 0.008762759279248379801, 0.008969004577654274279, 0.009175249876060167023, 0.009381495174466059767 ),
 .UNSPECIFIED. ) ;
#39215=CARTESIAN_POINT ( 'NONE',  ( 193.8198143686853712, 294.9412293303058732, -14.86391783401530553 ) ) ;
#39216=CARTESIAN_POINT ( 'NONE',  ( 137.2172943591538967, 238.4824982072973967, 3.021315404115420679E-15 ) ) ;
#39217=CARTESIAN_POINT ( 'NONE',  ( -22.42236680055709641, 157.8615022471902591, 0.000000000000000000 ) ) ;
#39218=CARTESIAN_POINT ( 'NONE',  ( 9.458193372709645885, 176.2677522451418497, 10.00000000000009592 ) ) ;
#39219=CARTESIAN_POINT ( 'NONE',  ( 87.02133327910362937, 230.2369531367911009, -4.594050593750048428 ) ) ;
#39221=FACE_OUTER_BOUND ( 'NONE', #81467, .T. ) ;
#39222=CARTESIAN_POINT ( 'NONE',  ( 168.4958712465444819, 279.2003023517014526, -13.40781613193690802 ) ) ;
#39223=CARTESIAN_POINT ( 'NONE',  ( 4.424420716760506522, 173.3615022471902591, -10.00000000000009592 ) ) ;
#39224=CARTESIAN_POINT ( 'NONE',  ( 5.371288904610766579, 186.1589784336661637, -6.496448406907675876E-16 ) ) ;
#39226=CARTESIAN_POINT ( 'NONE',  ( 161.0952649348064938, 251.6218116045831437, 13.81854265722852482 ) ) ;
#39227=ORIENTED_EDGE ( 'NONE', *, *, #50081, .F. ) ;
#39231=CARTESIAN_POINT ( 'NONE',  ( 189.0804396436501236, 261.2380845551991229, -6.138920082207003581 ) ) ;
#39233=CARTESIAN_POINT ( 'NONE',  ( 202.1579274701688291, 280.4991937992804765, -15.90174466444106649 ) ) ;
#39235=CARTESIAN_POINT ( 'NONE',  ( 37.36027580478098287, 198.5024278399160664, 9.188101187500095079 ) ) ;
#39236=CARTESIAN_POINT ( 'NONE',  ( 196.7621536703766196, 275.9285207744129025, 15.30025596421527467 ) ) ;
#39237=ORIENTED_EDGE ( 'NONE', *, *, #39446, .T. ) ;
#39239=CARTESIAN_POINT ( 'NONE',  ( 182.3105792408025820, 260.2671590519555025, -11.01268989705850743 ) ) ;
#39241=ADVANCED_FACE ( 'NONE', ( #2520 ), #86970, .F. ) ;
#39242=CARTESIAN_POINT ( 'NONE',  ( 164.8705138155180521, 286.2009910768602481, -3.373684704351256780 ) ) ;
#39244=CARTESIAN_POINT ( 'NONE',  ( 155.4186054393023255, 261.4540742680644598, 17.05753227160644769 ) ) ;
#39245=CARTESIAN_POINT ( 'NONE',  ( 57.23161641937173982, 215.3967562850347122, -4.648177544792955347E-16 ) ) ;
#39246=DIRECTION ( 'NONE',  ( -0.8660254037844387076, -0.4999999999999998890, -0.000000000000000000 ) ) ;
#39247=CARTESIAN_POINT ( 'NONE',  ( 147.7112127936102866, 274.8036699242858276, -9.124700685424272706 ) ) ;
#39249=CARTESIAN_POINT ( 'NONE',  ( 190.9986981037068290, 264.2499144972765066, 7.795840479274263046 ) ) ;
#39251=CARTESIAN_POINT ( 'NONE',  ( 176.4011637054438495, 256.6761881497252489, -11.13936515825015228 ) ) ;
#39252=CARTESIAN_POINT ( 'NONE',  ( 191.1000148935602567, 299.6520602076213891, -9.462302242170249400 ) ) ;
#39253=CARTESIAN_POINT ( 'NONE',  ( 190.4750160083620472, 300.7345900314585947, -1.159659205620361400 ) ) ;
#39255=ORIENTED_EDGE ( 'NONE', *, *, #32602, .T. ) ;
#39256=CARTESIAN_POINT ( 'NONE',  ( 149.9060791885465846, 273.0020498124315509, -11.57482514211843849 ) ) ;
#39257=CARTESIAN_POINT ( 'NONE',  ( 163.7183543885751078, 247.0784873978576854, -6.786164904910574336 ) ) ;
#39258=CARTESIAN_POINT ( 'NONE',  ( 183.5291393727272009, 269.0254755003825267, 15.13985252155338834 ) ) ;
#39259=CARTESIAN_POINT ( 'NONE',  ( 101.4461556848294492, 235.5024278399160949, -9.188101187500093303 ) ) ;
#39261=CARTESIAN_POINT ( 'NONE',  ( -6.697530200413229551, 155.3932355074535963, -2.679491924311250717 ) ) ;
#39265=CARTESIAN_POINT ( 'NONE',  ( 136.7639277290220718, 259.7677522451419350, -5.000000000000047962 ) ) ;
#39266=CARTESIAN_POINT ( 'NONE',  ( 191.5813027864163587, 276.8931351878708256, 16.99066381371337187 ) ) ;
#39267=CARTESIAN_POINT ( 'NONE',  ( 204.6600721283745372, 272.9583799553993231, -9.753926932682416506 ) ) ;
#39269=CARTESIAN_POINT ( 'NONE',  ( 149.9431819415206348, 271.6515743903611906, -11.68441791719118328 ) ) ;
#39270=CARTESIAN_POINT ( 'NONE',  ( 105.1336465626505969, 243.0530062829863027, -4.648177544792955347E-16 ) ) ;
#39274=CARTESIAN_POINT ( 'NONE',  ( 163.2954787364450340, 255.9746288828553702, -14.88763456503479787 ) ) ;
#39275=CARTESIAN_POINT ( 'NONE',  ( 178.1322669947267343, 280.4903793975759640, 16.69614814349041509 ) ) ;
#39276=CARTESIAN_POINT ( 'NONE',  ( 197.3934918644919776, 268.5675634807000733, 9.323123344629930642 ) ) ;
#39277=EDGE_CURVE ( 'NONE', #32845, #469, #79067, .T. ) ;
#39279=EDGE_CURVE ( 'NONE', #1341, #29582, #80339, .T. ) ;
#39281=CARTESIAN_POINT ( 'NONE',  ( 179.9888841032236257, 262.5618594283533298, -12.69062350693043761 ) ) ;
#39284=VERTEX_POINT ( 'NONE', #50100 ) ;
#39287=EDGE_LOOP ( 'NONE', ( #7529, #58993, #97795, #18652 ) ) ;
#39288=CARTESIAN_POINT ( 'NONE',  ( 167.3868433433993630, 249.7561290667149194, 6.957693806426012983 ) ) ;
#39289=CARTESIAN_POINT ( 'NONE',  ( 194.3442947553755005, 294.0328026529847421, -15.97648891113594871 ) ) ;
#39290=CARTESIAN_POINT ( 'NONE',  ( 157.0150015346687553, 258.6890351218854676, 16.85538724311808068 ) ) ;
#39294=CARTESIAN_POINT ( 'NONE',  ( 154.0741575860427304, 263.7827262580370871, -16.96155047328870680 ) ) ;
#39296=CARTESIAN_POINT ( 'NONE',  ( 120.7424577590100654, 230.5177522451417929, 5.000000000000051514 ) ) ;
#39298=ORIENTED_EDGE ( 'NONE', *, *, #84109, .F. ) ;
#39299=ORIENTED_EDGE ( 'NONE', *, *, #5774, .T. ) ;
#39300=CARTESIAN_POINT ( 'NONE',  ( 162.6627524694667954, 249.2999192911965167, 10.54795694096488745 ) ) ;
#39301=B_SPLINE_CURVE_WITH_KNOTS ( 'NONE', 3,
 ( #62539, #16949, #9363, #62034 ),
 .UNSPECIFIED., .F., .F.,
 ( 4, 4 ),
 ( 0.000000000000000000, 0.007566978283060982885 ),
 .UNSPECIFIED. ) ;
#39302=ORIENTED_EDGE ( 'NONE', *, *, #43944, .F. ) ;
#39305=CARTESIAN_POINT ( 'NONE',  ( 170.2702171900916710, 269.5895188327120877, 16.72394520728834522 ) ) ;
#39308=ADVANCED_FACE ( 'NONE', ( #21206 ), #39693, .T. ) ;
#39309=CARTESIAN_POINT ( 'NONE',  ( 190.6193642582544499, 300.0591430953767258, -3.705976999785533632 ) ) ;
#39311=CARTESIAN_POINT ( 'NONE',  ( 190.0646458372534937, 301.4453720177293121, 2.091788150666768153 ) ) ;
#39312=CARTESIAN_POINT ( 'NONE',  ( 206.6389649419900536, 271.5030152196637800, -6.665702415263554670 ) ) ;
#39314=CARTESIAN_POINT ( 'NONE',  ( 168.7460418684975139, 249.8756972425479148, -5.467426467192338713 ) ) ;
#39317=CARTESIAN_POINT ( 'NONE',  ( 183.5877099323311370, 284.2622598002585050, -15.59430947663861566 ) ) ;
#39319=CARTESIAN_POINT ( 'NONE',  ( 128.5097966488581562, 238.8768266524159856, 9.188101187500098632 ) ) ;
#39320=CARTESIAN_POINT ( 'NONE',  ( 186.6224779119422408, 262.8828560441721720, -9.606717503673682046 ) ) ;
#39322=CARTESIAN_POINT ( 'NONE',  ( 179.3876637460693928, 290.2313054047237983, -9.427853318526828730 ) ) ;
#39325=CARTESIAN_POINT ( 'NONE',  ( 203.3725562006430039, 276.0788499616656395, 13.32272411125720701 ) ) ;
#39326=CARTESIAN_POINT ( 'NONE',  ( 180.7648415157122486, 256.2425494826519525, 1.247752698343054467 ) ) ;
#39327=AXIS2_PLACEMENT_3D ( 'NONE', #6029, #92182, #60205 ) ;
#39328=EDGE_CURVE ( 'NONE', #90496, #81863, #97200, .T. ) ;
#39329=CARTESIAN_POINT ( 'NONE',  ( 174.0430117795368972, 289.9400120375415213, -4.743096007750332355 ) ) ;
#39330=DIRECTION ( 'NONE',  ( 0.5000000000000048850, -0.8660254037844358210, 0.000000000000000000 ) ) ;
#39331=CARTESIAN_POINT ( 'NONE',  ( -22.42236680055709641, 157.8615022471902591, 0.000000000000000000 ) ) ;
#39333=CARTESIAN_POINT ( 'NONE',  ( 180.2260403442535051, 295.0423342771414923, -3.480517403894910711 ) ) ;
#39334=CARTESIAN_POINT ( 'NONE',  ( 148.5730530464635706, 273.3109188183360061, 10.25868201370624888 ) ) ;
#39335=CARTESIAN_POINT ( 'NONE',  ( 165.0169426809697768, 246.6514736266339298, 5.598232276327055779 ) ) ;
#39337=CARTESIAN_POINT ( 'NONE',  ( 194.8598199529639317, 293.1398868181796615, -15.91766051364927570 ) ) ;
#39341=CARTESIAN_POINT ( 'NONE',  ( 191.0217486410549839, 283.4676459628224165, -16.57262105235832905 ) ) ;
#39342=CARTESIAN_POINT ( 'NONE',  ( 178.2544296081904918, 259.9720107254665322, -13.27066457805568866 ) ) ;
#39344=CARTESIAN_POINT ( 'NONE',  ( 204.6823371430232896, 272.9704135290961062, -9.754921121218281144 ) ) ;
#39345=CARTESIAN_POINT ( 'NONE',  ( 164.7124473124548558, 284.1078844219010193, -6.876237286123044967 ) ) ;
#39346=CARTESIAN_POINT ( 'NONE',  ( 160.5163443890054964, 282.2647654489487081, 6.663140935368019768 ) ) ;
#39347=FACE_OUTER_BOUND ( 'NONE', #88210, .T. ) ;
#39352=CARTESIAN_POINT ( 'NONE',  ( 164.2681401592249699, 247.4123488826276969, -7.457225004184277140 ) ) ;
#39353=CARTESIAN_POINT ( 'NONE',  ( 156.6812872898450735, 261.2670451491295012, 0.000000000000000000 ) ) ;
#39354=CARTESIAN_POINT ( 'NONE',  ( 173.7407999030873498, 250.8548675950284519, -1.041279177761091912 ) ) ;
#39355=CARTESIAN_POINT ( 'NONE',  ( 185.8592955827088531, 297.1117474649988708, -4.290889079375690862 ) ) ;
#39356=CARTESIAN_POINT ( 'NONE',  ( 204.3095277081791892, 275.7254174276451977, 13.16468475777854863 ) ) ;
#39357=CARTESIAN_POINT ( 'NONE',  ( 193.6455285480667783, 269.4045135959429444, 13.67829860818159027 ) ) ;
#39360=CARTESIAN_POINT ( 'NONE',  ( -7.320788502016136512, 157.3923013555410080, 4.594050593750050204 ) ) ;
#39361=CARTESIAN_POINT ( 'NONE',  ( 87.45434598099585344, 230.4869531367911293, 4.594050593750046652 ) ) ;
#39363=CARTESIAN_POINT ( 'NONE',  ( 193.1977289678065404, 296.0187128512746995, -12.37159405312863925 ) ) ;
#39365=ADVANCED_FACE ( 'NONE', ( #86387 ), #40779, .F. ) ;
#39367=FACE_OUTER_BOUND ( 'NONE', #52383, .T. ) ;
#39369=CARTESIAN_POINT ( 'NONE',  ( 37.58366506746438773, 204.0530062829863027, 1.101618078115930403E-13 ) ) ;
#39373=CARTESIAN_POINT ( 'NONE',  ( 169.4383027745296602, 251.8538218511134232, -9.888297047301421117 ) ) ;
#39374=CARTESIAN_POINT ( 'NONE',  ( 164.7584947292794766, 245.2769114807558140, -5.139043669254925284 ) ) ;
#39375=CARTESIAN_POINT ( 'NONE',  ( 196.4390255720217908, 290.4046224503736653, 16.34739044515864848 ) ) ;
#39378=CARTESIAN_POINT ( 'NONE',  ( 44.64073572505018461, 187.3923013555410080, 4.594050593750050204 ) ) ;
#39379=CARTESIAN_POINT ( 'NONE',  ( 69.15955932604958889, 219.9244531367911293, -4.594050593750046652 ) ) ;
#39383=CARTESIAN_POINT ( 'NONE',  ( 167.2628569450862699, 259.7336296457672233, 16.26364047457860096 ) ) ;
#39384=CARTESIAN_POINT ( 'NONE',  ( -6.040052912301403509, 153.9865022471901455, 1.119607411625061291E-15 ) ) ;
#39389=CARTESIAN_POINT ( 'NONE',  ( 150.8247211172754589, 269.4109153179094278, -14.37608026040300402 ) ) ;
#39392=CARTESIAN_POINT ( 'NONE',  ( 61.98804677278346986, 206.5958772461660828, -9.188101187500095079 ) ) ;
#39395=CARTESIAN_POINT ( 'NONE',  ( 159.2077906806335932, 254.8910129107889588, 16.14624949541834553 ) ) ;
#39397=CARTESIAN_POINT ( 'NONE',  ( 201.3152185631758186, 281.9588084421832264, 17.09304993608981604 ) ) ;
#39402=CARTESIAN_POINT ( 'NONE',  ( 112.2445834879231796, 225.6115022471901739, -5.000000000000041744 ) ) ;
#39404=CARTESIAN_POINT ( 'NONE',  ( 206.9408877595175511, 272.2148635675444552, 6.707071080545934372 ) ) ;
#39407=CARTESIAN_POINT ( 'NONE',  ( 184.7589102698180454, 271.2641373520414163, 16.13988341988741482 ) ) ;
#39409=CARTESIAN_POINT ( 'NONE',  ( 206.7680519836501958, 272.5142239127119979, -10.57935479673322021 ) ) ;
#39410=CARTESIAN_POINT ( 'NONE',  ( 187.3045064622214682, 276.9103046244464394, -16.79128408433122033 ) ) ;
#39412=ORIENTED_EDGE ( 'NONE', *, *, #90160, .F. ) ;
#39413=CARTESIAN_POINT ( 'NONE',  ( 173.5969002525141605, 251.1178000409413187, 0.5105381496963667942 ) ) ;
#39416=CARTESIAN_POINT ( 'NONE',  ( 148.3025927079438304, 273.7793698660844939, -8.046026357031887954 ) ) ;
#39417=CARTESIAN_POINT ( 'NONE',  ( 155.8152618860606538, 260.7670451491295012, 0.000000000000000000 ) ) ;
#39418=VERTEX_POINT ( 'NONE', #96975 ) ;
#39424=DIRECTION ( 'NONE',  ( -0.8660254037844387076, -0.4999999999999998890, -0.000000000000000000 ) ) ;
#39425=ORIENTED_EDGE ( 'NONE', *, *, #8433, .F. ) ;
#39431=CARTESIAN_POINT ( 'NONE',  ( 182.8258399896172648, 294.6916754291505072, 8.116841955439214829 ) ) ;
#39432=CARTESIAN_POINT ( 'NONE',  ( 185.3862244519964406, 292.5652162196358859, -10.75470610306963515 ) ) ;
#39433=CARTESIAN_POINT ( 'NONE',  ( 205.3465787480556344, 274.9762877783610406, -13.79319041940166279 ) ) ;
#39434=CARTESIAN_POINT ( 'NONE',  ( 139.7406297344813311, 260.6744531367911009, 4.594050593750047540 ) ) ;
#39435=CARTESIAN_POINT ( 'NONE',  ( 203.5602143330212641, 268.7753616305579385, 2.467715433455414331 ) ) ;
#39436=CARTESIAN_POINT ( 'NONE',  ( 179.0261547916831546, 258.3138165185279149, 9.736748159590288054 ) ) ;
#39437=CARTESIAN_POINT ( 'NONE',  ( 88.13101510164371177, 227.8149278399160949, -9.188101187500095079 ) ) ;
#39439=CARTESIAN_POINT ( 'NONE',  ( 151.4025156491502742, 268.4101458323662541, 14.71049357081981235 ) ) ;
#39441=VERTEX_POINT ( 'NONE', #57921 ) ;
#39442=CARTESIAN_POINT ( 'NONE',  ( 156.9377365471174812, 258.8228620059706486, -16.89686783298308015 ) ) ;
#39446=EDGE_CURVE ( 'NONE', #78211, #86358, #34363, .T. ) ;
#39447=CARTESIAN_POINT ( 'NONE',  ( 147.0276296945837373, 275.9876705829954062, 0.7617065417431535534 ) ) ;
#39450=CARTESIAN_POINT ( 'NONE',  ( 163.0682440866927720, 248.2045114712421423, 11.63988583931958942 ) ) ;
#39451=CARTESIAN_POINT ( 'NONE',  ( 82.93520977470207356, 212.5643266524159856, -9.188101187500093303 ) ) ;
#39453=ORIENTED_EDGE ( 'NONE', *, *, #7066, .F. ) ;
#39454=CARTESIAN_POINT ( 'NONE',  ( 208.3790849386676598, 269.7238329819538762, -1.525282248498321946 ) ) ;
#39459=CARTESIAN_POINT ( 'NONE',  ( 207.0644055248061761, 269.7777976096807038, -0.04004023774084553011 ) ) ;
#39463=CARTESIAN_POINT ( 'NONE',  ( 188.8759260044885764, 294.9136311979676748, 11.52016544153279654 ) ) ;
#39466=CARTESIAN_POINT ( 'NONE',  ( 153.0308080659177392, 265.5898606369461277, -17.74682723936668438 ) ) ;
#39471=CARTESIAN_POINT ( 'NONE',  ( 195.8540013720623278, 265.4683100572506191, 4.431129527759733122 ) ) ;
#39472=CARTESIAN_POINT ( 'NONE',  ( 86.96746701141694302, 211.0177522451417929, 5.000000000000051514 ) ) ;
#39474=CARTESIAN_POINT ( 'NONE',  ( 171.1784097330638872, 251.6294428635012537, 7.086366496291955919 ) ) ;
#39477=DIRECTION ( 'NONE',  ( 0.4999999999999998890, -0.8660254037844385966, 0.000000000000000000 ) ) ;
#39480=CARTESIAN_POINT ( 'NONE',  ( 165.8866640751390094, 265.8956478032751534, 17.81115609982314751 ) ) ;
#39483=CARTESIAN_POINT ( 'NONE',  ( 194.2199708651012600, 294.2481379475345875, 15.50834247347371253 ) ) ;
#39488=CARTESIAN_POINT ( 'NONE',  ( 174.5508403973756515, 260.3590064504865040, -14.93617697178709314 ) ) ;
#39490=CARTESIAN_POINT ( 'NONE',  ( 161.7767236248226084, 250.4414905302161287, -13.15904643207033153 ) ) ;
#39491=( BOUNDED_CURVE ( )  B_SPLINE_CURVE ( 2, ( #22546, #5363, #91479, #28647, #6841, #67646, #29650, #21558, #53432 ),
 .UNSPECIFIED., .F., .T. ) 
 B_SPLINE_CURVE_WITH_KNOTS ( ( 3, 2, 2, 2, 3 ),
 ( 0.6895161290322581182, 0.6908602150537634934, 0.6935483870967742437, 0.6962365591397849940, 0.6975806451612903691 ),
 .UNSPECIFIED. ) 
 CURVE ( )  GEOMETRIC_REPRESENTATION_ITEM ( )  RATIONAL_B_SPLINE_CURVE ( ( 0.9330127018922194093, 0.9330127018922194093, 1.000000000000000000, 0.8660254037844387076, 1.000000000000000000, 0.8660254037844387076, 1.000000000000000000, 0.9330127018922194093, 0.9330127018922194093 ) ) 
 REPRESENTATION_ITEM ( '' )  );
#39492=CARTESIAN_POINT ( 'NONE',  ( -6.807019788225388446, 173.0024278399160949, 9.188101187500095079 ) ) ;
#39493=CARTESIAN_POINT ( 'NONE',  ( 191.1597575862519705, 296.5656282560291288, -11.82805995379970021 ) ) ;
#39496=CARTESIAN_POINT ( 'NONE',  ( 177.3028647534693789, 256.5043743002872816, 8.298765593072630509 ) ) ;
#39499=CARTESIAN_POINT ( 'NONE',  ( 28.05084980986327281, 180.8768266524160424, -9.188101187500093303 ) ) ;
#39503=CARTESIAN_POINT ( 'NONE',  ( 173.3031365584441232, 273.4220882896894409, -17.43855797201185354 ) ) ;
#39504=CARTESIAN_POINT ( 'NONE',  ( 133.7124848875370731, 259.5530062829863596, -4.648177544792955347E-16 ) ) ;
#39505=CARTESIAN_POINT ( 'NONE',  ( 186.9795881944451423, 295.9919572693598866, -7.697386768984371130 ) ) ;
#39506=CARTESIAN_POINT ( 'NONE',  ( 189.1827640625472782, 261.0025008612562942, -0.7550638320438417539 ) ) ;
#39508=ADVANCED_FACE ( 'NONE', ( #7705 ), #54281, .T. ) ;
#39509=CARTESIAN_POINT ( 'NONE',  ( 193.0616670940060828, 295.8427809175656762, -12.31989297540982697 ) ) ;
#39510=CARTESIAN_POINT ( 'NONE',  ( 78.46959274033007148, 206.1115022471901739, -5.000000000000041744 ) ) ;
#39514=CARTESIAN_POINT ( 'NONE',  ( 34.70824655357364463, 190.8458772461660544, 9.188101187500095079 ) ) ;
#39518=CARTESIAN_POINT ( 'NONE',  ( 206.6389649419900536, 271.5030152196637800, -6.665702415263554670 ) ) ;
#39519=CARTESIAN_POINT ( 'NONE',  ( 151.3124059063077311, 268.5662204852269497, -14.45542936000225609 ) ) ;
#39521=CARTESIAN_POINT ( 'NONE',  ( 0.5273063997305368344, 171.1115022471902591, 10.00000000000009592 ) ) ;
#39525=CARTESIAN_POINT ( 'NONE',  ( 162.6937333994314656, 248.8531830095558632, 10.02305144031113926 ) ) ;
#39526=CARTESIAN_POINT ( 'NONE',  ( 105.5870131927823508, 231.7677522451418497, 10.00000000000009592 ) ) ;
#39527=CARTESIAN_POINT ( 'NONE',  ( 175.0279472884096776, 256.8441564353742592, 11.93536191757501363 ) ) ;
#39529=B_SPLINE_CURVE_WITH_KNOTS ( 'NONE', 3,
 ( #65922, #72565, #3169, #63933 ),
 .UNSPECIFIED., .F., .F.,
 ( 4, 4 ),
 ( 0.04541327962301634075, 0.04887120950165262795 ),
 .UNSPECIFIED. ) ;
#39535=LINE ( 'NONE', #31450, #65177 ) ;
#39537=CARTESIAN_POINT ( 'NONE',  ( 190.7851751463332164, 300.1973786460605425, 8.237717828100052486 ) ) ;
#39538=CARTESIAN_POINT ( 'NONE',  ( 181.2136957205551084, 257.4508974852847700, -7.654872872151471164 ) ) ;
#39545=CARTESIAN_POINT ( 'NONE',  ( 201.4214977800931763, 281.7747274386935601, -17.04225209925078133 ) ) ;
#39548=CARTESIAN_POINT ( 'NONE',  ( 147.9748066657072627, 274.3471119452502762, 9.387104374042873900 ) ) ;
#39551=CARTESIAN_POINT ( 'NONE',  ( 181.3700392331832631, 287.2969061643829036, -13.32859413632180434 ) ) ;
#39554=CARTESIAN_POINT ( 'NONE',  ( 160.2389756875691944, 266.2308171109146429, 16.63061643655940713 ) ) ;
#39559=CARTESIAN_POINT ( 'NONE',  ( 64.36996372895569607, 195.7202760586659736, -5.415160957724236172E-17 ) ) ;
#39561=CARTESIAN_POINT ( 'NONE',  ( 193.7609008727193043, 262.8443104439116951, 4.759103018491034121 ) ) ;
#39562=CARTESIAN_POINT ( 'NONE',  ( 159.8276996530030090, 255.3946308028359624, 16.30222759331605786 ) ) ;
#39563=CARTESIAN_POINT ( 'NONE',  ( 89.49337443912149581, 229.1427522451419065, 10.00000000000009415 ) ) ;
#39564=CARTESIAN_POINT ( 'NONE',  ( 172.7335680787827528, 271.6338345647230312, 16.60374280657107349 ) ) ;
#39566=CARTESIAN_POINT ( 'NONE',  ( 189.9548861516039722, 299.9966941760355326, 5.043691249193295256 ) ) ;
#39568=CARTESIAN_POINT ( 'NONE',  ( 73.11106055086588640, 213.0177522451418497, -10.00000000000009592 ) ) ;
#39569=CARTESIAN_POINT ( 'NONE',  ( 190.5674408456512765, 300.5745055173924811, -0.9151048603553563199 ) ) ;
#39571=CARTESIAN_POINT ( 'NONE',  ( 174.9895866936052471, 261.2018727689135176, -14.15269007960848313 ) ) ;
#39573=CARTESIAN_POINT ( 'NONE',  ( 191.0536258616249370, 299.7324083678473130, 8.935283001608469888 ) ) ;
#39574=CARTESIAN_POINT ( 'NONE',  ( 192.6789561813392595, 296.9172536750198219, -11.84591848451790952 ) ) ;
#39575=CARTESIAN_POINT ( 'NONE',  ( 163.3485124243574091, 257.7923317456250629, 15.56224772009493229 ) ) ;
#39579=CARTESIAN_POINT ( 'NONE',  ( 206.1932826529868805, 273.5097535960530877, 11.72208607728249241 ) ) ;
#39583=B_SPLINE_CURVE_WITH_KNOTS ( 'NONE', 3,
 ( #37188, #30593, #21990, #91427, #61479, #8293, #92428, #99508, #22976, #39159 ),
 .UNSPECIFIED., .F., .F.,
 ( 4, 2, 2, 2, 4 ),
 ( 0.000000000000000000, 0.0004172351265548456087, 0.0008344702531096912174, 0.001251705379664536880, 0.001668940506219382435 ),
 .UNSPECIFIED. ) ;
#39584=CARTESIAN_POINT ( 'NONE',  ( 107.7791399978856930, 233.0333772461660828, 9.188101187500095079 ) ) ;
#39586=CARTESIAN_POINT ( 'NONE',  ( 190.2594329105515101, 301.1079909101196108, -4.731131889240534960 ) ) ;
#39588=CARTESIAN_POINT ( 'NONE',  ( 193.7609008727193043, 262.8443104439116951, 4.759103018491034121 ) ) ;
#39589=CARTESIAN_POINT ( 'NONE',  ( 154.9792334219179679, 262.2150889255981951, -17.21325849938693153 ) ) ;
#39590=B_SPLINE_CURVE_WITH_KNOTS ( 'NONE', 3,
 ( #68951, #61352, #35200, #30460, #34698, #58488, #20518, #12420, #66105, #27622, #97529, #4819, #74731, #92307 ),
 .UNSPECIFIED., .F., .F.,
 ( 4, 2, 2, 2, 2, 2, 4 ),
 ( 0.0009458495952914972114, 0.001465415157218448623, 0.001725197938181909692, 0.001984980719145370762, 0.002244763500108832265, 0.002504546281072293334, 0.003024111842999374633 ),
 .UNSPECIFIED. ) ;
#39591=CARTESIAN_POINT ( 'NONE',  ( 163.7136804588959649, 247.0865828815331042, 6.783386239354816105 ) ) ;
#39593=CARTESIAN_POINT ( 'NONE',  ( 165.4298696296856690, 283.8953809392911580, -8.443581878439131216 ) ) ;
#39595=CARTESIAN_POINT ( 'NONE',  ( 162.7459776558209228, 248.7626933030860812, -9.895605163646791880 ) ) ;
#39596=CARTESIAN_POINT ( 'NONE',  ( 181.9913924001663759, 260.5072070915913400, 9.621015379077912044 ) ) ;
#39597=EDGE_CURVE ( 'NONE', #28763, #84992, #27976, .T. ) ;
#39599=CARTESIAN_POINT ( 'NONE',  ( 132.6505673846437503, 238.2048013555409796, 4.594050593750051981 ) ) ;
#39600=CARTESIAN_POINT ( 'NONE',  ( 198.4782858197754649, 286.8725200914082620, -17.44895083299520522 ) ) ;
#39601=CARTESIAN_POINT ( 'NONE',  ( 189.1685910125652299, 299.5261110243415033, 4.889329439728404836 ) ) ;
#39602=CARTESIAN_POINT ( 'NONE',  ( 187.3694706215540862, 281.3094075288585714, -17.25064062178364566 ) ) ;
#39604=CARTESIAN_POINT ( 'NONE',  ( 47.42782112377506820, 204.3149278399160664, 9.188101187500093303 ) ) ;
#39606=VERTEX_POINT ( 'NONE', #77628 ) ;
#39610=CARTESIAN_POINT ( 'NONE',  ( 174.5571948831425857, 262.1308976863569455, 14.30389198049646282 ) ) ;
#39612=CARTESIAN_POINT ( 'NONE',  ( 203.4696564630250464, 278.2272125378923988, -16.38980782817167636 ) ) ;
#39613=CARTESIAN_POINT ( 'NONE',  ( 179.2813879323843196, 261.6109213834521938, 12.22300016988861415 ) ) ;
#39614=CARTESIAN_POINT ( 'NONE',  ( 124.2065593741477301, 252.5177522451419350, 5.000000000000046185 ) ) ;
#39615=B_SPLINE_SURFACE_WITH_KNOTS ( 'NONE', 3, 1, ( 
 ( #88735, #90211 ),
 ( #69332, #76924 ),
 ( #71350, #48023 ),
 ( #9034, #92668 ),
 ( #16133, #61721 ),
 ( #16628, #84575 ),
 ( #31325, #30835 ),
 ( #86592, #1450 ),
 ( #38920, #40416 ),
 ( #938, #23221 ),
 ( #24237, #8537 ),
 ( #39906, #85067 ),
 ( #69825, #54110 ),
 ( #62715, #31814 ),
 ( #62212, #85592 ),
 ( #15615, #78452 ),
 ( #32330, #24725 ),
 ( #70324, #22740 ),
 ( #436, #17127 ),
 ( #47031, #55608 ),
 ( #63231, #46513 ),
 ( #61223, #47524 ),
 ( #77948, #93673 ),
 ( #78967, #77451 ),
 ( #100253, #70839 ),
 ( #9554, #55115 ),
 ( #30333, #94173 ),
 ( #23714, #53619 ),
 ( #8047, #38417 ),
 ( #92187, #93164 ),
 ( #15113, #7525 ),
 ( #46007, #54609 ),
 ( #39409, #86102 ),
 ( #72362, #25751 ) ),
 .UNSPECIFIED., .T., .F., .F.,
 ( 4, 2, 2, 2, 2, 2, 2, 2, 2, 2, 2, 2, 2, 2, 2, 2, 4 ),
 ( 2, 2 ),
 ( 0.000000000000000000, 0.06250000000000000000, 0.1250000000000000000, 0.1875000000000000000, 0.2500000000000000000, 0.3125000000000000000, 0.3750000000000000000, 0.4375000000000000000, 0.5000000000000000000, 0.5625000000000000000, 0.6250000000000000000, 0.6875000000000000000, 0.7500000000000000000, 0.8125000000000000000, 0.8750000000000000000, 0.9375000000000000000, 1.000000000000000000 ),
 ( 0.000000000000000000, 1.000000000000000000 ),
 .UNSPECIFIED. ) ;
#39616=CARTESIAN_POINT ( 'NONE',  ( 147.8791740781505837, 276.5127524457575987, 2.771564245682613947 ) ) ;
#39617=ORIENTED_EDGE ( 'NONE', *, *, #79934, .T. ) ;
#39619=CARTESIAN_POINT ( 'NONE',  ( 202.9685995779611858, 279.0950685203052899, 16.84977534244423580 ) ) ;
#39621=CARTESIAN_POINT ( 'NONE',  ( 25.42527643493543366, 194.6744531367911293, 4.594050593750047540 ) ) ;
#39624=CARTESIAN_POINT ( 'NONE',  ( 38.27158024800235125, 186.2365022471901739, -10.00000000000009237 ) ) ;
#39627=CARTESIAN_POINT ( 'NONE',  ( 198.2339335403562472, 277.5049642442517097, -15.43335200160522902 ) ) ;
#39628=CARTESIAN_POINT ( 'NONE',  ( 63.88265089144443465, 201.5643266524160424, 9.188101187500095079 ) ) ;
#39629=CARTESIAN_POINT ( 'NONE',  ( 174.0414442612575954, 288.4808356476244739, 7.602831793599980514 ) ) ;
#39630=CARTESIAN_POINT ( 'NONE',  ( 183.6498318386265396, 256.3252116762061519, 1.424693195823348635 ) ) ;
#39631=CARTESIAN_POINT ( 'NONE',  ( 157.4805323096970255, 257.8827121670497036, -16.70238855805511591 ) ) ;
#39634=CARTESIAN_POINT ( 'NONE',  ( 23.90999230191033575, 194.6115022471903160, -5.000000000000047962 ) ) ;
#39635=CARTESIAN_POINT ( 'NONE',  ( 185.0112656319525115, 294.4118031042779080, 9.900635645151082187 ) ) ;
#39637=CARTESIAN_POINT ( 'NONE',  ( -10.21716836350912949, 177.1589784336661637, -6.496448406907675876E-16 ) ) ;
#39639=CARTESIAN_POINT ( 'NONE',  ( 164.1930575273928810, 260.6154384242434503, -16.15766538543017816 ) ) ;
#39640=CARTESIAN_POINT ( 'NONE',  ( 170.5783285705315961, 263.4208030108840717, 15.80046225904663260 ) ) ;
#39642=CARTESIAN_POINT ( 'NONE',  ( 188.9382125046037117, 261.1427886392369828, 6.789719310133031982 ) ) ;
#39644=CARTESIAN_POINT ( 'NONE',  ( 187.0838235210196672, 259.2678003084403144, -2.401093518989122266 ) ) ;
#39646=ORIENTED_EDGE ( 'NONE', *, *, #53934, .F. ) ;
#39647=CARTESIAN_POINT ( 'NONE',  ( 136.0602820919951341, 259.3615022471902876, 5.000000000000046185 ) ) ;
#39648=CARTESIAN_POINT ( 'NONE',  ( 144.2948532952960932, 258.0163529461947292, -10.00000000000009592 ) ) ;
#39649=CARTESIAN_POINT ( 'NONE',  ( 155.3647120480568162, 278.9503195987401796, -5.223984518467562843 ) ) ;
#39651=CARTESIAN_POINT ( 'NONE',  ( 206.9483995484939101, 272.2018527673814106, 9.530154192725417417 ) ) ;
#39653=CARTESIAN_POINT ( 'NONE',  ( 159.3237119419271437, 254.6902313965507858, -15.56765445935501191 ) ) ;
#39654=DIRECTION ( 'NONE',  ( 0.4999999999999992784, -0.8660254037844390407, 0.000000000000000000 ) ) ;
#39655=CARTESIAN_POINT ( 'NONE',  ( 88.86189758574333553, 212.1115022471902023, -5.000000000000041744 ) ) ;
#39656=CARTESIAN_POINT ( 'NONE',  ( 191.4149729938089592, 298.5499520618976135, 8.351909744838231120 ) ) ;
#39661=CARTESIAN_POINT ( 'NONE',  ( 156.2183318835597561, 276.9731782824784432, -10.13063037517403231 ) ) ;
#39665=CARTESIAN_POINT ( 'NONE',  ( 188.7627825353981166, 297.5844699726765725, 7.724845922223074979 ) ) ;
#39669=CARTESIAN_POINT ( 'NONE',  ( 196.6800254274587019, 289.9871984561398222, -17.90749311895638129 ) ) ;
#39672=CARTESIAN_POINT ( 'NONE',  ( 203.2795549558504433, 278.5564780069144035, 16.55170960561796889 ) ) ;
#39674=CARTESIAN_POINT ( 'NONE',  ( 175.4606724842758751, 268.3091254637062661, -17.51855393743042910 ) ) ;
#39675=ORIENTED_EDGE ( 'NONE', *, *, #74606, .F. ) ;
#39680=VERTEX_POINT ( 'NONE', #6211 ) ;
#39681=CARTESIAN_POINT ( 'NONE',  ( 161.1429874292947488, 271.1544374080688726, 16.26257973483764729 ) ) ;
#39685=CARTESIAN_POINT ( 'NONE',  ( 177.9925615710933755, 254.8251403409008731, -7.350624415798725053 ) ) ;
#39686=CARTESIAN_POINT ( 'NONE',  ( 194.9636675848471441, 292.9600174435121289, -15.57898232594655319 ) ) ;
#39688=DIRECTION ( 'NONE',  ( 0.5000000000000048850, -0.8660254037844358210, 0.000000000000000000 ) ) ;
#39692=CARTESIAN_POINT ( 'NONE',  ( 198.6255909461775104, 276.8423615036599585, -15.32991266925497342 ) ) ;
#39693=CYLINDRICAL_SURFACE ( 'NONE', #46667, 17.82106496071139645 ) ;
#39694=FACE_OUTER_BOUND ( 'NONE', #74493, .T. ) ;
#39696=CARTESIAN_POINT ( 'NONE',  ( 147.4105755286778106, 275.3243889417975083, -3.778870683123901397 ) ) ;
#39697=CARTESIAN_POINT ( 'NONE',  ( 191.2557879401978198, 261.3776189723048446, -4.694998167070893125 ) ) ;
#39698=CARTESIAN_POINT ( 'NONE',  ( 206.7923762329701276, 272.4720930770340033, -9.496103119940368487 ) ) ;
#39702=CARTESIAN_POINT ( 'NONE',  ( 161.8873598795597388, 250.2498629158519350, 13.90822209621415873 ) ) ;
#39703=CARTESIAN_POINT ( 'NONE',  ( 106.5432495796755603, 238.9865022471903160, 10.00000000000009415 ) ) ;
#39706=B_SPLINE_CURVE_WITH_KNOTS ( 'NONE', 3,
 ( #91634, #51608, #22202, #6995 ),
 .UNSPECIFIED., .F., .F.,
 ( 4, 4 ),
 ( 0.01573702636073541841, 0.02454403038988591315 ),
 .UNSPECIFIED. ) ;
#39709=EDGE_CURVE ( 'NONE', #68725, #33752, #60888, .T. ) ;
#39710=CARTESIAN_POINT ( 'NONE',  ( 17.25242200676955306, 190.7677522451419065, -5.000000000000047962 ) ) ;
#39711=CARTESIAN_POINT ( 'NONE',  ( 89.26784699199328088, 222.3458772461660544, 9.188101187500095079 ) ) ;
#39714=CARTESIAN_POINT ( 'NONE',  ( 167.6527552166903376, 278.6792754734481719, -13.36931194722780170 ) ) ;
#39715=CARTESIAN_POINT ( 'NONE',  ( 6.129408228687162286, 174.3458772461660828, 9.188101187500095079 ) ) ;
#39719=VERTEX_POINT ( 'NONE', #7200 ) ;
#39722=CARTESIAN_POINT ( 'NONE',  ( 197.5944296959598319, 265.4027214831109518, -2.921024236943222885 ) ) ;
#39725=FACE_OUTER_BOUND ( 'NONE', #38455, .T. ) ;
#39727=CARTESIAN_POINT ( 'NONE',  ( 30.18841615574984516, 197.4244531367911293, -4.594050593750046652 ) ) ;
#39728=CARTESIAN_POINT ( 'NONE',  ( 100.8960422556166634, 222.3927522451418213, 10.00000000000009948 ) ) ;
#39730=CARTESIAN_POINT ( 'NONE',  ( 150.0434472053995307, 271.6953193618362548, -11.68999578780283244 ) ) ;
#39731=CARTESIAN_POINT ( 'NONE',  ( 182.6142383756292418, 260.6848368803231892, -10.84370499219341077 ) ) ;
#39732=CARTESIAN_POINT ( 'NONE',  ( 152.2705230281304409, 271.0405980996342237, 14.27451841150712042 ) ) ;
#39733=CARTESIAN_POINT ( 'NONE',  ( 157.2464636617698375, 258.2881309577184652, 18.14284729738657731 ) ) ;
#39734=CARTESIAN_POINT ( 'NONE',  ( 155.4216552449402684, 261.4487918497463284, 18.51722274565528892 ) ) ;
#39735=CARTESIAN_POINT ( 'NONE',  ( 161.3773209892555371, 251.1332761876949746, -14.50043705923759241 ) ) ;
#39736=VECTOR ( 'NONE', #25689, 1000.000000000000000 ) ;
#39738=CARTESIAN_POINT ( 'NONE',  ( 148.0346525705264469, 274.2434557974783615, -9.381294579651672905 ) ) ;
#39739=ADVANCED_FACE ( 'NONE', ( #38084 ), #71029, .T. ) ;
#39741=CARTESIAN_POINT ( 'NONE',  ( 190.7982574810033611, 262.8194055429554510, 8.405793748174573921 ) ) ;
#39742=CARTESIAN_POINT ( 'NONE',  ( 171.7060500237028862, 279.6726968596310030, 14.88215948178559245 ) ) ;
#39743=CARTESIAN_POINT ( 'NONE',  ( 189.9686529740312153, 299.6116365339944423, 6.575253125843024016 ) ) ;
#39745=CARTESIAN_POINT ( 'NONE',  ( 147.6430623265936219, 274.9217099957185155, 8.258152514891218487 ) ) ;
#39750=CARTESIAN_POINT ( 'NONE',  ( 161.8840393808384022, 251.8702681966305477, -13.97960957670215087 ) ) ;
#39751=CARTESIAN_POINT ( 'NONE',  ( 104.9102572999672276, 237.5024278399160949, 9.188101187500095079 ) ) ;
#39753=CARTESIAN_POINT ( 'NONE',  ( -15.06115086838940442, 172.1115022471903160, -5.000000000000047962 ) ) ;
#39754=EDGE_CURVE ( 'NONE', #48297, #68650, #66064, .T. ) ;
#39756=CARTESIAN_POINT ( 'NONE',  ( 157.5520850189458884, 257.7587792392113215, 16.71892742266126319 ) ) ;
#39757=CARTESIAN_POINT ( 'NONE',  ( 191.5711784964392166, 276.9236626822979588, 16.85412083571288022 ) ) ;
#39758=CARTESIAN_POINT ( 'NONE',  ( 150.8870980228296332, 269.3028753482705611, -13.88216063016896307 ) ) ;
#39759=CARTESIAN_POINT ( 'NONE',  ( 192.9146452215483123, 263.8600050127276972, -4.623449015741573298 ) ) ;
#39760=CARTESIAN_POINT ( 'NONE',  ( 149.8974208606144600, 271.7624278638419355, -11.58230692921836358 ) ) ;
#39761=CARTESIAN_POINT ( 'NONE',  ( 116.3166592645429205, 226.4155109091896350, 2.679491924311254714 ) ) ;
#39765=CARTESIAN_POINT ( 'NONE',  ( 190.2885894641050868, 266.2465236892521148, 10.78400978751670003 ) ) ;
#39766=CARTESIAN_POINT ( 'NONE',  ( 178.9380535331071655, 280.8279290640091403, 16.38556303516354262 ) ) ;
#39767=CARTESIAN_POINT ( 'NONE',  ( 196.5175218668017862, 267.6197207801589002, 9.577823450216618184 ) ) ;
#39768=EDGE_CURVE ( 'NONE', #57662, #82888, #59638, .T. ) ;
#39769=ADVANCED_FACE ( 'NONE', ( #56294 ), #79683, .F. ) ;
#39770=ORIENTED_EDGE ( 'NONE', *, *, #54704, .F. ) ;
#39772=CARTESIAN_POINT ( 'NONE',  ( 183.5722823471954257, 264.5482469279784823, -13.32579016364044655 ) ) ;
#39774=CARTESIAN_POINT ( 'NONE',  ( 192.0523540417460993, 298.0025604169266558, 12.03387399082417275 ) ) ;
#39775=ORIENTED_EDGE ( 'NONE', *, *, #33012, .T. ) ;
#39776=CARTESIAN_POINT ( 'NONE',  ( 201.0718222649304607, 273.3369752706136069, -13.40913439694983289 ) ) ;
#39780=CARTESIAN_POINT ( 'NONE',  ( 167.1424731200726228, 249.5982725804538802, 6.966350190857109048 ) ) ;
#39782=DIRECTION ( 'NONE',  ( -0.8660254037844387076, -0.4999999999999998890, -0.000000000000000000 ) ) ;
#39790=CARTESIAN_POINT ( 'NONE',  ( 203.2187760522547819, 278.6617501559703101, -15.08675642319914978 ) ) ;
#39791=VERTEX_POINT ( 'NONE', #4607 ) ;
#39792=( BOUNDED_CURVE ( )  B_SPLINE_CURVE ( 2, ( #35494, #81151, #11718, #42580, #96341, #17818, #57291, #65400, #26413 ),
 .UNSPECIFIED., .F., .T. ) 
 B_SPLINE_CURVE_WITH_KNOTS ( ( 3, 2, 2, 2, 3 ),
 ( 0.5443548387096773800, 0.5456989247311827551, 0.5483870967741935054, 0.5510752688172042557, 0.5524193548387096309 ),
 .UNSPECIFIED. ) 
 CURVE ( )  GEOMETRIC_REPRESENTATION_ITEM ( )  RATIONAL_B_SPLINE_CURVE ( ( 0.9330127018922194093, 0.9330127018922194093, 1.000000000000000000, 0.8660254037844387076, 1.000000000000000000, 0.8660254037844387076, 1.000000000000000000, 0.9330127018922194093, 0.9330127018922194093 ) ) 
 REPRESENTATION_ITEM ( '' )  );
#39794=CARTESIAN_POINT ( 'NONE',  ( 175.7956577457310345, 258.6345868136107242, 13.14558633677379973 ) ) ;
#39800=CARTESIAN_POINT ( 'NONE',  ( 155.6066474290145720, 261.1283759879266881, -18.16552045242181279 ) ) ;
#39802=CARTESIAN_POINT ( 'NONE',  ( 165.7267109360765573, 274.6484224846600455, -15.16830425928928072 ) ) ;
#39803=CARTESIAN_POINT ( 'NONE',  ( 206.4839639422192192, 273.0062788342933118, -11.22308919026441210 ) ) ;
#39804=CARTESIAN_POINT ( 'NONE',  ( 190.5841104648970088, 300.5456328899159644, 3.298325803792328870 ) ) ;
#39805=CARTESIAN_POINT ( 'NONE',  ( 196.1252721995043942, 284.4712197134549001, -17.81715240067734030 ) ) ;
#39808=CARTESIAN_POINT ( 'NONE',  ( 171.5407152967187017, 250.9167206134208072, -5.638389805452348469 ) ) ;
#39810=CARTESIAN_POINT ( 'NONE',  ( 156.9561170169907030, 280.4813240094630373, 2.086493405815429636 ) ) ;
#39811=CARTESIAN_POINT ( 'NONE',  ( 130.4855038751826726, 236.9548013555409796, -4.594050593750042211 ) ) ;
#39813=CARTESIAN_POINT ( 'NONE',  ( 186.5674233539620275, 262.7087872174366225, -9.046917918335617870 ) ) ;
#39815=EDGE_LOOP ( 'NONE', ( #41976, #11086, #74851, #62014 ) ) ;
#39818=CARTESIAN_POINT ( 'NONE',  ( 200.0648741936326189, 273.7901900051996336, 13.73784782553251205 ) ) ;
#39819=CARTESIAN_POINT ( 'NONE',  ( 180.5509916577576348, 256.1221220636168141, 1.304812651851478433 ) ) ;
#39822=CARTESIAN_POINT ( 'NONE',  ( 147.4382974802994113, 275.2763731131041141, 3.664996198306503583 ) ) ;
#39828=CARTESIAN_POINT ( 'NONE',  ( 176.5702065357462516, 255.6409285000345619, -7.288246984450118759 ) ) ;
#39829=VERTEX_POINT ( 'NONE', #75900 ) ;
#39830=CARTESIAN_POINT ( 'NONE',  ( 194.9220242159064185, 293.0321458743159724, -14.92681063007793263 ) ) ;
#39833=CARTESIAN_POINT ( 'NONE',  ( 188.3791492419724420, 266.3799810227098419, -11.83448844734568794 ) ) ;
#39834=EDGE_CURVE ( 'NONE', #94451, #94798, #18583, .T. ) ;
#39835=CARTESIAN_POINT ( 'NONE',  ( 160.0965860327900145, 279.1799484724489275, 10.77100507046937139 ) ) ;
#39836=CARTESIAN_POINT ( 'NONE',  ( 152.4791540838723449, 266.5453533620465691, -15.88447083262123272 ) ) ;
#39837=CARTESIAN_POINT ( 'NONE',  ( 148.9694607950094394, 272.6243204573405592, 11.81236034532910573 ) ) ;
#39839=CARTESIAN_POINT ( 'NONE',  ( 161.5256564828909234, 281.5214332243310196, -6.610724726001431684 ) ) ;
#39840=CARTESIAN_POINT ( 'NONE',  ( 151.4835999992953930, 274.9817874143876111, -8.672836155307052763 ) ) ;
#39842=ORIENTED_EDGE ( 'NONE', *, *, #16554, .F. ) ;
#39843=CARTESIAN_POINT ( 'NONE',  ( 190.1696443193688708, 301.2635093119881162, -4.804312979389741223 ) ) ;
#39844=CARTESIAN_POINT ( 'NONE',  ( 187.2655409194766207, 261.7880714798743043, -8.837611146579153143 ) ) ;
#39845=CARTESIAN_POINT ( 'NONE',  ( 155.7631971310857750, 279.9683759737790183, 6.348568169051404197 ) ) ;
#39846=CARTESIAN_POINT ( 'NONE',  ( 194.7023383591533161, 288.5740446449341334, -17.20894952458154137 ) ) ;
#39848=CARTESIAN_POINT ( 'NONE',  ( 184.7240172173571295, 296.8390834670735785, -4.377300740651686617 ) ) ;
#39854=CARTESIAN_POINT ( 'NONE',  ( -10.43332761869022640, 164.7833772461660544, -9.188101187500095079 ) ) ;
#39855=CARTESIAN_POINT ( 'NONE',  ( 84.85626976964255164, 228.9869531367911293, 4.594050593750046652 ) ) ;
#39857=CARTESIAN_POINT ( 'NONE',  ( 146.8153075009282134, 276.3554234099810287, -4.113808735271278216 ) ) ;
#39858=CARTESIAN_POINT ( 'NONE',  ( 147.7963747854073802, 275.1547895869376248, 4.489566192750358731 ) ) ;
#39859=DIRECTION ( 'NONE',  ( -0.8660254037844387076, -0.4999999999999998890, -0.000000000000000000 ) ) ;
#39860=CARTESIAN_POINT ( 'NONE',  ( 207.8575108622103755, 270.6272257822888037, -6.381720258959569847 ) ) ;
#39863=CARTESIAN_POINT ( 'NONE',  ( -22.42236680055709641, 157.8615022471902591, 0.000000000000000000 ) ) ;
#39866=CARTESIAN_POINT ( 'NONE',  ( 177.9223291652669445, 289.9174720514999990, 9.664897302444829918 ) ) ;
#39868=CARTESIAN_POINT ( 'NONE',  ( 193.7563803396631670, 267.3524183776476661, 11.90297280730822571 ) ) ;
#39869=CARTESIAN_POINT ( 'NONE',  ( 161.4733487491374717, 251.3868574054517921, 13.04233661072845329 ) ) ;
#39870=CARTESIAN_POINT ( 'NONE',  ( 196.4994169513186364, 290.3000215130921902, 16.82935102260526961 ) ) ;
#39875=CARTESIAN_POINT ( 'NONE',  ( 38.41565749170202082, 202.1744531367911293, 4.594050593750047540 ) ) ;
#39876=CARTESIAN_POINT ( 'NONE',  ( 63.34103791831414298, 213.5024278399161233, 9.188101187500095079 ) ) ;
#39877=CARTESIAN_POINT ( 'NONE',  ( 65.47921168356349142, 198.6115022471902023, -5.000000000000041744 ) ) ;
#39883=CARTESIAN_POINT ( 'NONE',  ( 200.2233614854171435, 270.9342182064973485, -11.47649089687903334 ) ) ;
#39884=EDGE_CURVE ( 'NONE', #5726, #41965, #20866, .T. ) ;
#39886=CARTESIAN_POINT ( 'NONE',  ( 198.6894790592683080, 286.5067226703918095, -17.06774375037124614 ) ) ;
#39887=CARTESIAN_POINT ( 'NONE',  ( 148.9504735598738137, 272.6572073132907690, -11.88406006066344744 ) ) ;
#39889=CARTESIAN_POINT ( 'NONE',  ( 59.38997056143013964, 205.0958772461660828, -9.188101187500095079 ) ) ;
#39891=CYLINDRICAL_SURFACE ( 'NONE', #59139, 10.00000000000010658 ) ;
#39893=CARTESIAN_POINT ( 'NONE',  ( 159.9671766634011192, 253.5757178060795809, 16.49140845334465411 ) ) ;
#39895=CARTESIAN_POINT ( 'NONE',  ( 198.9721957120447655, 281.0613474150461570, 17.36564602955951386 ) ) ;
#39898=CARTESIAN_POINT ( 'NONE',  ( 149.0247308281161622, 274.5285899518638075, 9.115861392502811356 ) ) ;
#39899=CARTESIAN_POINT ( 'NONE',  ( 113.6157903772485298, 229.7365022471902023, -10.00000000000009059 ) ) ;
#39901=CARTESIAN_POINT ( 'NONE',  ( 207.1122325394003951, 271.9180857031755636, 7.794245785756032774 ) ) ;
#39904=CARTESIAN_POINT ( 'NONE',  ( 188.0932163354825093, 273.3618889904262801, 15.64081734860616990 ) ) ;
#39905=ORIENTED_EDGE ( 'NONE', *, *, #40464, .F. ) ;
#39906=CARTESIAN_POINT ( 'NONE',  ( 206.5081929095101998, 272.9643130319303737, -9.215516226794479238 ) ) ;
#39907=CARTESIAN_POINT ( 'NONE',  ( 187.4304084080513348, 276.9874324135936376, -16.75430557518339825 ) ) ;
#39909=ORIENTED_EDGE ( 'NONE', *, *, #98038, .T. ) ;
#39910=CARTESIAN_POINT ( 'NONE',  ( 177.2936775833025251, 253.0977458076815765, -0.2642580955292048728 ) ) ;
#39913=CARTESIAN_POINT ( 'NONE',  ( 166.2081174782295534, 287.2918692684091297, 1.312827985884416737 ) ) ;
#39914=CARTESIAN_POINT ( 'NONE',  ( 176.9878821292914211, 283.3466992399841615, -15.40003107629192769 ) ) ;
#39915=ORIENTED_EDGE ( 'NONE', *, *, #14341, .T. ) ;
#39918=CARTESIAN_POINT ( 'NONE',  ( 29.01593374150824189, 180.8927522451417929, -10.00000000000009237 ) ) ;
#39922=CARTESIAN_POINT ( 'NONE',  ( 167.7129959498070093, 276.7492194616727375, 15.67174948013163061 ) ) ;
#39924=VERTEX_POINT ( 'NONE', #63663 ) ;
#39925=CARTESIAN_POINT ( 'NONE',  ( 170.8911557219925612, 284.9263958063596078, 11.11643632232859602 ) ) ;
#39929=CARTESIAN_POINT ( 'NONE',  ( 155.4216552449402684, 261.4487918497463284, 18.51722274565528892 ) ) ;
#39930=CARTESIAN_POINT ( 'NONE',  ( 185.4339105455779304, 292.4495553130619214, -11.40531104680791152 ) ) ;
#39931=CARTESIAN_POINT ( 'NONE',  ( 164.3024481966923531, 265.7778226775905068, -17.31441928355125270 ) ) ;
#39932=CARTESIAN_POINT ( 'NONE',  ( 208.0534104968160420, 270.2879176619674695, -3.858664761683422206 ) ) ;
#39933=CARTESIAN_POINT ( 'NONE',  ( 204.6979730149710690, 269.6043557618498880, 2.446051969963311201 ) ) ;
#39935=CARTESIAN_POINT ( 'NONE',  ( 87.96880888631662287, 221.5958772461660544, -9.188101187500095079 ) ) ;
#39937=CARTESIAN_POINT ( 'NONE',  ( 151.1926529451685326, 268.7736386982768408, 14.30343427984827365 ) ) ;
#39938=B_SPLINE_CURVE_WITH_KNOTS ( 'NONE', 3,
 ( #26928, #57807, #12232, #82672 ),
 .UNSPECIFIED., .F., .F.,
 ( 4, 4 ),
 ( 0.002905392229856628220, 0.01085320331254635735 ),
 .UNSPECIFIED. ) ;
#39942=ORIENTED_EDGE ( 'NONE', *, *, #27450, .T. ) ;
#39943=CARTESIAN_POINT ( 'NONE',  ( 195.9349871089815167, 291.2776426773277194, -17.14268251872402971 ) ) ;
#39945=ORIENTED_EDGE ( 'NONE', *, *, #14466, .T. ) ;
#39949=B_SPLINE_SURFACE_WITH_KNOTS ( 'NONE', 3, 1, ( 
 ( #69500, #92838 ),
 ( #62899, #24406 ),
 ( #23389, #54279 ),
 ( #53301, #6712 ),
 ( #84254, #23894 ),
 ( #78118, #37590 ),
 ( #68502, #45684 ),
 ( #99424, #42096 ),
 ( #72534, #48204 ),
 ( #48721, #87782 ),
 ( #80652, #11230 ),
 ( #71527, #86262 ),
 ( #64913, #17300 ),
 ( #80150, #10217 ),
 ( #9733, #25924 ),
 ( #78622, #47687 ),
 ( #56797, #49219 ),
 ( #55774, #86766 ),
 ( #16801, #79151 ),
 ( #9209, #41084 ),
 ( #71027, #17820 ),
 ( #57295, #40588 ),
 ( #96343, #79653 ),
 ( #26414, #49699 ),
 ( #34025, #72020 ),
 ( #2117, #40082 ),
 ( #32513, #1629 ),
 ( #95858, #2624 ),
 ( #64408, #63405 ),
 ( #65402, #18320 ),
 ( #26910, #18814 ),
 ( #95371, #33001 ),
 ( #10716, #41592 ),
 ( #73028, #33513 ) ),
 .UNSPECIFIED., .T., .F., .F.,
 ( 4, 2, 2, 2, 2, 2, 2, 2, 2, 2, 2, 2, 2, 2, 2, 2, 4 ),
 ( 2, 2 ),
 ( 0.000000000000000000, 0.06250000000000000000, 0.1250000000000000000, 0.1875000000000000000, 0.2500000000000000000, 0.3125000000000000000, 0.3750000000000000000, 0.4375000000000000000, 0.5000000000000000000, 0.5625000000000000000, 0.6250000000000000000, 0.6875000000000000000, 0.7500000000000000000, 0.8125000000000000000, 0.8750000000000000000, 0.9375000000000000000, 1.000000000000000000 ),
 ( 0.000000000000000000, 1.000000000000000000 ),
 .UNSPECIFIED. ) ;
#39952=CARTESIAN_POINT ( 'NONE',  ( 162.4702972292363086, 249.2401858085828508, 11.41296778546566060 ) ) ;
#39953=CARTESIAN_POINT ( 'NONE',  ( 79.95842099707557793, 204.7202760586659167, -5.415160957724236172E-17 ) ) ;
#39957=CARTESIAN_POINT ( 'NONE',  ( 124.1108878986028543, 230.9155109091896065, 2.679491924311254714 ) ) ;
#39958=CARTESIAN_POINT ( 'NONE',  ( 200.3443106254163411, 283.6404703198547850, -17.85865425939682538 ) ) ;
#39959=ORIENTED_EDGE ( 'NONE', *, *, #45700, .T. ) ;
#39962=CARTESIAN_POINT ( 'NONE',  ( 161.7013249288979182, 284.4161495234801009, 0.5351470228536304719 ) ) ;
#39963=CARTESIAN_POINT ( 'NONE',  ( 183.8183646926467816, 261.3479267577503720, -11.63888974307716495 ) ) ;
#39967=CARTESIAN_POINT ( 'NONE',  ( 188.6809246227683445, 295.1128069315126368, 11.75850413834363550 ) ) ;
#39968=CARTESIAN_POINT ( 'NONE',  ( 184.8538874427280518, 260.0470281449409526, 6.326053503214689400 ) ) ;
#39969=CARTESIAN_POINT ( 'NONE',  ( 206.8775514429320026, 272.3245652858344670, -9.838455694836268250 ) ) ;
#39970=CARTESIAN_POINT ( 'NONE',  ( 191.3077102587145646, 274.7514833773715850, 16.90660339326615969 ) ) ;
#39973=CARTESIAN_POINT ( 'NONE',  ( 198.7408816115379864, 285.9624092822338071, -17.04496721243561197 ) ) ;
#39977=CARTESIAN_POINT ( 'NONE',  ( 203.5562810614256364, 277.6620430705328317, -14.30492976707583708 ) ) ;
#39978=CARTESIAN_POINT ( 'NONE',  ( 200.8769374536528858, 282.7179335918746688, 17.26928237494566787 ) ) ;
#39981=CARTESIAN_POINT ( 'NONE',  ( 171.5357040741050980, 251.2175910118344859, 7.330095994321424335 ) ) ;
#39983=CARTESIAN_POINT ( 'NONE',  ( 156.4350627803543148, 272.1488426913780927, 14.19226130382477358 ) ) ;
#39984=VERTEX_POINT ( 'NONE', #96613 ) ;
#39986=CARTESIAN_POINT ( 'NONE',  ( 164.9971748156432056, 244.8635054444190757, -1.825016704039769788 ) ) ;
#39988=CARTESIAN_POINT ( 'NONE',  ( 176.0413199817918724, 285.4093408875521618, -13.23764318957976371 ) ) ;
#39991=CARTESIAN_POINT ( 'NONE',  ( 172.0067041090704549, 274.8475428133772311, 16.34631960249475569 ) ) ;
#39992=CARTESIAN_POINT ( 'NONE',  ( 163.1007186844803982, 284.1234281835157276, -3.987921137952420647 ) ) ;
#39995=CARTESIAN_POINT ( 'NONE',  ( 195.3642010211272861, 265.2768603898356332, -7.559402155732556139 ) ) ;
#39997=CARTESIAN_POINT ( 'NONE',  ( -1.069254392388470976, 164.0643266524160140, 9.188101187500095079 ) ) ;
#39999=EDGE_LOOP ( 'NONE', ( #39425, #73606, #28167, #18300 ) ) ;
#40000=CARTESIAN_POINT ( 'NONE',  ( 174.9585859693524696, 255.2860589088032839, 8.263831412499913043 ) ) ;
#40002=LINE ( 'NONE', #25321, #45110 ) ;
#40004=CARTESIAN_POINT ( 'NONE',  ( 17.98295739510416524, 187.3149278399160949, -9.188101187500095079 ) ) ;
#40008=CARTESIAN_POINT ( 'NONE',  ( 191.6517533181996100, 265.3842329497505261, -11.14382704138352054 ) ) ;
#40009=CARTESIAN_POINT ( 'NONE',  ( 191.6723191112861855, 298.6608002251342100, -9.737039817265848995 ) ) ;
#40010=VECTOR ( 'NONE', #82829, 1000.000000000000000 ) ;
#40012=CARTESIAN_POINT ( 'NONE',  ( 172.1631122144370920, 275.2657131827085664, -17.28304708590200889 ) ) ;
#40013=B_SPLINE_CURVE_WITH_KNOTS ( 'NONE', 3,
 ( #32574, #16863, #39141, #1179, #93915, #31553, #55836, #25467, #72086, #24959, #54861, #81573, #86832, #86326, #85840, #17364 ),
 .UNSPECIFIED., .F., .F.,
 ( 4, 2, 2, 2, 2, 2, 2, 4 ),
 ( 8.156114889773229926E-15, 0.0005317649415277559332, 0.0007976474122876054925, 0.001063529883047454943, 0.001329412353807304719, 0.001595294824567154062, 0.001861177295327003838, 0.002127059766086853397 ),
 .UNSPECIFIED. ) ;
#40016=CARTESIAN_POINT ( 'NONE',  ( 198.0355408163131585, 287.6393769322024241, 18.20720360189982756 ) ) ;
#40017=CARTESIAN_POINT ( 'NONE',  ( 69.37632600059342280, 210.8615022471902591, -10.00000000000009592 ) ) ;
#40020=CARTESIAN_POINT ( 'NONE',  ( 206.3531636607249879, 271.3592212809042508, 6.161143238982110582 ) ) ;
#40021=CARTESIAN_POINT ( 'NONE',  ( 28.05084980986327281, 180.8768266524160140, -9.188101187500091527 ) ) ;
#40022=CARTESIAN_POINT ( 'NONE',  ( 159.2554912534056939, 254.8083930951974878, 16.49944922174842432 ) ) ;
#40024=CARTESIAN_POINT ( 'NONE',  ( 198.9369963555428740, 286.0780101374919013, -18.58432392708837710 ) ) ;
#40028=CARTESIAN_POINT ( 'NONE',  ( 78.13225151398272317, 227.4637435831425023, 2.679491924311251605 ) ) ;
#40029=CARTESIAN_POINT ( 'NONE',  ( 167.6278246310154714, 282.5728663012718584, -12.21306354836790220 ) ) ;
#40030=CARTESIAN_POINT ( 'NONE',  ( 163.1717563955264438, 281.1342508170415613, -10.22479631152172352 ) ) ;
#40033=CARTESIAN_POINT ( 'NONE',  ( 202.9216520459657147, 279.1763840310111391, 15.75371595331685803 ) ) ;
#40034=CARTESIAN_POINT ( 'NONE',  ( 111.1205068418362742, 223.4155109091896065, 2.679491924311254714 ) ) ;
#40035=CARTESIAN_POINT ( 'NONE',  ( 185.5354357917608752, 267.5855751454028564, -14.72482343138568339 ) ) ;
#40036=EDGE_LOOP ( 'NONE', ( #27547, #89212, #66831, #27064 ) ) ;
#40042=CARTESIAN_POINT ( 'NONE',  ( 185.1775619574503366, 280.9945881611855043, 17.59732015342263267 ) ) ;
#40044=B_SPLINE_CURVE_WITH_KNOTS ( 'NONE', 3,
 ( #95340, #18292, #78087, #55743 ),
 .UNSPECIFIED., .F., .F.,
 ( 4, 4 ),
 ( 0.008346957882847750101, 0.01470164726671086691 ),
 .UNSPECIFIED. ) ;
#40045=CARTESIAN_POINT ( 'NONE',  ( 151.3284628043366524, 268.5384091220288383, 14.49047510809488237 ) ) ;
#40046=CARTESIAN_POINT ( 'NONE',  ( 181.0230527394317619, 257.6990957149607198, -7.502503115033712255 ) ) ;
#40049=CARTESIAN_POINT ( 'NONE',  ( 207.8575108622103755, 270.6272257822888037, -6.381720258959569847 ) ) ;
#40052=CARTESIAN_POINT ( 'NONE',  ( 200.7134601498536028, 283.0010845879393742, -16.98649239173277792 ) ) ;
#40057=CARTESIAN_POINT ( 'NONE',  ( 189.9052851100924215, 301.7213928939034986, -1.077181946533001256 ) ) ;
#40058=CARTESIAN_POINT ( 'NONE',  ( 91.43256340568937901, 235.8464784336661637, 1.353441290958777525E-15 ) ) ;
#40059=B_SPLINE_CURVE_WITH_KNOTS ( 'NONE', 3,
 ( #50821, #87911, #11852, #89395, #89869, #19946 ),
 .UNSPECIFIED., .F., .F.,
 ( 4, 2, 4 ),
 ( 0.01904094441108342833, 0.02356434879539306276, 0.02808775317970270066 ),
 .UNSPECIFIED. ) ;
#40060=CARTESIAN_POINT ( 'NONE',  ( 203.3286960320409094, 267.8359400968079171, 2.569349860321338941 ) ) ;
#40062=CARTESIAN_POINT ( 'NONE',  ( 161.8637969276452679, 267.0824340876292240, 16.50456879414842959 ) ) ;
#40065=CARTESIAN_POINT ( 'NONE',  ( 197.9952413503812352, 287.7091776547143809, 17.17611241386010690 ) ) ;
#40067=CARTESIAN_POINT ( 'NONE',  ( 52.94873307290090025, 207.5024278399160949, 9.188101187500095079 ) ) ;
#40069=CARTESIAN_POINT ( 'NONE',  ( 160.7489855951974675, 254.2215850144021658, 15.85577744295692248 ) ) ;
#40070=CARTESIAN_POINT ( 'NONE',  ( 198.0384979254556015, 287.6342550689238351, 17.28192639992792579 ) ) ;
#40071=CARTESIAN_POINT ( 'NONE',  ( 176.4670716382853470, 273.1881962802569319, 17.38719208580632269 ) ) ;
#40072=ORIENTED_EDGE ( 'NONE', *, *, #83049, .T. ) ;
#40073=DIRECTION ( 'NONE',  ( -0.8660254037844387076, -0.4999999999999998890, -0.000000000000000000 ) ) ;
#40074=CARTESIAN_POINT ( 'NONE',  ( 190.2648877593310317, 301.0985428348857340, -4.426259207433023590 ) ) ;
#40075=CARTESIAN_POINT ( 'NONE',  ( 147.6618183892331331, 274.8892235422768522, 8.990680574201936892 ) ) ;
#40077=ORIENTED_EDGE ( 'NONE', *, *, #99481, .T. ) ;
#40078=CARTESIAN_POINT ( 'NONE',  ( 175.4521479476684647, 261.2799168608980267, -14.40428220072110932 ) ) ;
#40079=CARTESIAN_POINT ( 'NONE',  ( 170.6367097137389806, 275.3559257912166345, -16.50175916787543784 ) ) ;
#40080=CARTESIAN_POINT ( 'NONE',  ( 207.5462191418491500, 271.1663988579299485, -5.239401497773396699 ) ) ;
#40081=CARTESIAN_POINT ( 'NONE',  ( 147.3236643320416022, 275.4749235501183193, -5.185334239426818037 ) ) ;
#40082=CARTESIAN_POINT ( 'NONE',  ( 149.2561433752359505, 272.1277716627430436, 12.99353668144589946 ) ) ;
#40084=CARTESIAN_POINT ( 'NONE',  ( 179.7440261010970062, 270.5841209280236512, 17.43403005247386517 ) ) ;
#40085=DIRECTION ( 'NONE',  ( 0.4999999999999998890, -0.8660254037844385966, 0.000000000000000000 ) ) ;
#40087=CARTESIAN_POINT ( 'NONE',  ( 154.6934824199911702, 264.1949505326113581, -17.20522734258247866 ) ) ;
#40088=CARTESIAN_POINT ( 'NONE',  ( 207.5583741822599393, 271.1453457103705205, 3.140867606700001424 ) ) ;
#40090=CARTESIAN_POINT ( 'NONE',  ( 109.6190968851625911, 246.3464784336661353, 1.353441290958777327E-15 ) ) ;
#40091=EDGE_LOOP ( 'NONE', ( #33249, #8111, #32350, #53130 ) ) ;
#40092=CARTESIAN_POINT ( 'NONE',  ( 149.0458102676470560, 272.4920792916013284, -12.77276851155236059 ) ) ;
#40094=CARTESIAN_POINT ( 'NONE',  ( 155.5587153255869453, 261.2113968263770971, -18.30500480654006878 ) ) ;
#40095=EDGE_CURVE ( 'NONE', #100032, #947, #43810, .T. ) ;
#40096=CARTESIAN_POINT ( 'NONE',  ( 163.8040269124969939, 246.9300982336122559, 6.025552750865228013 ) ) ;
#40099=CARTESIAN_POINT ( 'NONE',  ( 176.2336582595617358, 254.2209709748362627, 4.925071008084640489 ) ) ;
#40101=CARTESIAN_POINT ( 'NONE',  ( 162.7738416911812180, 248.7144313781379310, -11.09964294874192525 ) ) ;
#40104=CARTESIAN_POINT ( 'NONE',  ( 156.1631927981498222, 273.8066032555324796, -12.73205779767400969 ) ) ;
#40105=CARTESIAN_POINT ( 'NONE',  ( 184.2589036364679771, 261.5973822520062413, 9.577938735879747867 ) ) ;
#40106=CARTESIAN_POINT ( 'NONE',  ( 206.2410742340367165, 271.7831106908868719, 8.101945950764607218 ) ) ;
#40107=CARTESIAN_POINT ( 'NONE',  ( 137.1700506867025808, 243.8768266524160140, -9.188101187500093303 ) ) ;
#40108=CARTESIAN_POINT ( 'NONE',  ( 198.6894790592683080, 286.5067226703918095, -17.06774375037124614 ) ) ;
#40111=CARTESIAN_POINT ( 'NONE',  ( 196.4351339088274813, 290.4113630087520050, 17.20526457544535504 ) ) ;
#40113=CARTESIAN_POINT ( 'NONE',  ( 49.94514132322986910, 190.4548013555409796, -4.594050593750042211 ) ) ;
#40117=CARTESIAN_POINT ( 'NONE',  ( 171.3314046892768090, 260.1076107119635026, 14.81378772054287474 ) ) ;
#40119=CARTESIAN_POINT ( 'NONE',  ( 178.8916920429171000, 291.7792318689755007, -6.177336454205645033 ) ) ;
#40121=CARTESIAN_POINT ( 'NONE',  ( 9.004826742577897392, 187.5530062829863027, -4.648177544792955347E-16 ) ) ;
#40123=EDGE_CURVE ( 'NONE', #62531, #22014, #66161, .T. ) ;
#40124=CARTESIAN_POINT ( 'NONE',  ( 112.8760603413013399, 242.6427522451419350, 10.00000000000009237 ) ) ;
#40127=CARTESIAN_POINT ( 'NONE',  ( 202.3139361598622372, 280.2289788223093865, 15.93832709035092421 ) ) ;
#40129=CARTESIAN_POINT ( 'NONE',  ( 19.79611131033658111, 191.4244531367911293, -4.594050593750046652 ) ) ;
#40131=CARTESIAN_POINT ( 'NONE',  ( 81.77131458871032521, 208.0177522451417929, 5.000000000000051514 ) ) ;
#40134=CARTESIAN_POINT ( 'NONE',  ( 198.1230357675706557, 277.7030879543556239, -15.67994595731362217 ) ) ;
#40135=CARTESIAN_POINT ( 'NONE',  ( 52.32645086003936541, 201.0177522451418497, -10.00000000000009592 ) ) ;
#40136=CARTESIAN_POINT ( 'NONE',  ( 172.8524532584847861, 287.5566872288061404, 7.496887191024062425 ) ) ;
#40137=CARTESIAN_POINT ( 'NONE',  ( 184.7866525864025107, 257.7151715236021232, 1.373357544146073250 ) ) ;
#40138=CARTESIAN_POINT ( 'NONE',  ( 205.2941531242069857, 275.0670916224857478, -13.92605142593109058 ) ) ;
#40141=CARTESIAN_POINT ( 'NONE',  ( 161.5791065876047128, 267.6385769225021249, 16.61089899141252246 ) ) ;
#40142=CARTESIAN_POINT ( 'NONE',  ( 32.93109025799834200, 176.4865022471901455, 1.119607411625061291E-15 ) ) ;
#40143=CARTESIAN_POINT ( 'NONE',  ( 150.1604317434691325, 251.3768266524160140, -9.188101187500091527 ) ) ;
#40144=CARTESIAN_POINT ( 'NONE',  ( 202.5511585997265911, 279.8180975037686835, 17.12781264818056925 ) ) ;
#40145=VECTOR ( 'NONE', #76614, 1000.000000000000000 ) ;
#40146=CARTESIAN_POINT ( 'NONE',  ( -8.322217149083147802, 159.8768266524159856, -9.188101187500091527 ) ) ;
#40149=CARTESIAN_POINT ( 'NONE',  ( 170.2387432371133684, 263.6005831635989125, 15.83122915802868214 ) ) ;
#40150=CARTESIAN_POINT ( 'NONE',  ( 188.3259911839309098, 288.6587601801259098, -15.98176789963882349 ) ) ;
#40151=CARTESIAN_POINT ( 'NONE',  ( 206.4943150373521803, 272.9883502116088039, 11.34100825923693101 ) ) ;
#40152=CARTESIAN_POINT ( 'NONE',  ( 186.2095639655686341, 259.2069574296129417, -2.346516652132980774 ) ) ;
#40157=EDGE_CURVE ( 'NONE', #90906, #30881, #6319, .T. ) ;
#40158=CARTESIAN_POINT ( 'NONE',  ( 180.3366176027714971, 286.6329442896284263, 13.14786923958608966 ) ) ;
#40159=CARTESIAN_POINT ( 'NONE',  ( 153.2950423568359781, 277.6701191893376972, -5.326679232739844672 ) ) ;
#40161=CARTESIAN_POINT ( 'NONE',  ( 160.5941949179546384, 252.4896903319198600, 14.95613949087054628 ) ) ;
#40163=CARTESIAN_POINT ( 'NONE',  ( 206.5081929095101998, 272.9643130319303737, -9.215516226794479238 ) ) ;
#40164=CARTESIAN_POINT ( 'NONE',  ( 192.0963028965829551, 297.9264387674147656, 11.34530024772836754 ) ) ;
#40168=CARTESIAN_POINT ( 'NONE',  ( 193.7118145980225279, 295.1282904202991517, 14.61271143546694162 ) ) ;
#40172=CARTESIAN_POINT ( 'NONE',  ( 136.9984762794283881, 243.2365022471901739, -10.00000000000009237 ) ) ;
#40174=EDGE_LOOP ( 'NONE', ( #55988, #97573, #83478, #19764 ) ) ;
#40176=CARTESIAN_POINT ( 'NONE',  ( 199.9502294570856407, 265.6703872523112295, 6.360370400932541246E-13 ) ) ;
#40178=CARTESIAN_POINT ( 'NONE',  ( 191.0702043019150835, 299.7036936669546776, -8.800021049343948576 ) ) ;
#40184=CARTESIAN_POINT ( 'NONE',  ( 190.8094645593471341, 300.1553081486349015, 8.399847186519689757 ) ) ;
#40186=B_SPLINE_SURFACE_WITH_KNOTS ( 'NONE', 3, 1, ( 
 ( #8256, #17341 ),
 ( #46222, #38639 ),
 ( #85292, #1157 ),
 ( #77144, #62423 ),
 ( #61927, #39120 ),
 ( #92879, #48249 ),
 ( #32031, #62941 ),
 ( #24448, #23433 ),
 ( #9255, #54320 ),
 ( #80696, #11271 ),
 ( #41631, #18359 ),
 ( #3663, #50725 ),
 ( #3179, #65934 ),
 ( #34541, #26947 ),
 ( #19859, #42134 ),
 ( #42623, #81681 ),
 ( #96888, #73065 ),
 ( #17863, #11759 ),
 ( #88811, #80189 ),
 ( #57831, #27458 ),
 ( #19377, #63942 ),
 ( #40630, #65439 ),
 ( #72573, #56333 ),
 ( #71566, #96384 ),
 ( #87331, #25965 ),
 ( #73552, #58329 ),
 ( #48761, #50236 ),
 ( #94879, #49252 ),
 ( #2162, #34064 ),
 ( #81191, #35030 ),
 ( #89304, #57334 ),
 ( #33043, #25443 ),
 ( #79694, #41125 ),
 ( #4136, #64955 ) ),
 .UNSPECIFIED., .T., .F., .F.,
 ( 4, 2, 2, 2, 2, 2, 2, 2, 2, 2, 2, 2, 2, 2, 2, 2, 4 ),
 ( 2, 2 ),
 ( 0.000000000000000000, 0.06250000000000000000, 0.1250000000000000000, 0.1875000000000000000, 0.2500000000000000000, 0.3125000000000000000, 0.3750000000000000000, 0.4375000000000000000, 0.5000000000000000000, 0.5625000000000000000, 0.6250000000000000000, 0.6875000000000000000, 0.7500000000000000000, 0.8125000000000000000, 0.8750000000000000000, 0.9375000000000000000, 1.000000000000000000 ),
 ( 0.000000000000000000, 1.000000000000000000 ),
 .UNSPECIFIED. ) ;
#40188=CARTESIAN_POINT ( 'NONE',  ( 195.6968381273587454, 265.0589268724819476, 7.395276693337085483 ) ) ;
#40189=ORIENTED_EDGE ( 'NONE', *, *, #12103, .T. ) ;
#40193=CARTESIAN_POINT ( 'NONE',  ( 164.0781508658037637, 275.4055464209769752, 15.63836535835214114 ) ) ;
#40198=CARTESIAN_POINT ( 'NONE',  ( 194.1789525331299728, 294.3191837825503967, -15.34533909744314961 ) ) ;
#40200=CARTESIAN_POINT ( 'NONE',  ( 8.774901663922227257, 164.3262482093457777, 3.021315404115420679E-15 ) ) ;
#40203=CARTESIAN_POINT ( 'NONE',  ( 164.2813349609167517, 246.1033764428878214, 1.949810150281061638 ) ) ;
#40206=VERTEX_POINT ( 'NONE', #20575 ) ;
#40209=CARTESIAN_POINT ( 'NONE',  ( 206.6703863510205679, 272.6833857505801006, -10.72500664779635393 ) ) ;
#40211=EDGE_CURVE ( 'NONE', #69571, #6423, #70365, .T. ) ;
#40212=CARTESIAN_POINT ( 'NONE',  ( 200.4775477985258760, 283.4096967665721536, 16.80647240730505487 ) ) ;
#40216=CARTESIAN_POINT ( 'NONE',  ( 155.4594742945911321, 261.3832873342573180, -17.01475918255801645 ) ) ;
#40217=DIRECTION ( 'NONE',  ( 0.4999999999999998890, -0.8660254037844385966, 0.000000000000000000 ) ) ;
#40222=EDGE_CURVE ( 'NONE', #88994, #19414, #38957, .T. ) ;
#40223=CARTESIAN_POINT ( 'NONE',  ( 20.35567970366385993, 175.8927522451418213, 10.00000000000009592 ) ) ;
#40224=CARTESIAN_POINT ( 'NONE',  ( 90.56688509766992468, 223.0958772461660260, -9.188101187500095079 ) ) ;
#40227=CARTESIAN_POINT ( 'NONE',  ( 174.5555281753831025, 282.3909387449837709, -14.50095961335927264 ) ) ;
#40228=CARTESIAN_POINT ( 'NONE',  ( 166.7187202459675746, 278.5591580196478958, -14.78021074750266273 ) ) ;
#40230=CARTESIAN_POINT ( 'NONE',  ( 0.1751364819041374699, 183.1589784336661637, -6.496448406907675876E-16 ) ) ;
#40232=CARTESIAN_POINT ( 'NONE',  ( 200.4403816905005158, 283.4740703539914648, 16.81798557643505987 ) ) ;
#40233=VERTEX_POINT ( 'NONE', #244 ) ;
#40237=CARTESIAN_POINT ( 'NONE',  ( 197.7056209715021851, 265.0177529662663574, -2.988310547816667828 ) ) ;
#40244=CARTESIAN_POINT ( 'NONE',  ( 28.70002176693659379, 193.5024278399160949, -9.188101187500093303 ) ) ;
#40245=CARTESIAN_POINT ( 'NONE',  ( 73.03889176721715160, 219.6427522451419065, -10.00000000000009415 ) ) ;
#40246=CARTESIAN_POINT ( 'NONE',  ( 199.2997933464620530, 277.4527719018980747, 15.18799710326758579 ) ) ;
#40247=ORIENTED_EDGE ( 'NONE', *, *, #82211, .F. ) ;
#40248=CARTESIAN_POINT ( 'NONE',  ( 153.0823121780915983, 273.6142464696663410, -11.82140495845541039 ) ) ;
#40249=B_SPLINE_CURVE_WITH_KNOTS ( 'NONE', 3,
 ( #68245, #76375, #75377, #75886, #5466, #82997, #36350, #14061, #98686, #5961, #91096, #36852, #6946, #13574, #67761, #21664, #28761, #67253, #84492, #53541, #52544, #69242, #37343, #99169, #98180, #15035, #44444, #29757, #59642, #45927, #90613, #37838, #38334, #60629, #91583, #22157, #53047, #68744, #99667, #30253, #92111, #76844, #7442, #30758, #61636, #92588 ),
 .UNSPECIFIED., .F., .F.,
 ( 4, 2, 2, 2, 2, 2, 2, 2, 2, 2, 2, 2, 2, 2, 2, 2, 2, 2, 2, 2, 2, 2, 4 ),
 ( 0.0004441887608673076183, 0.0008957827227663670705, 0.001121579703715850067, 0.001347376684665332848, 0.001460275175140070443, 0.001573173665614808038, 0.001798970646564274989, 0.002250564608463331839, 0.003153752532261445973, 0.004056940456059559240, 0.004960128379857672506, 0.005411722341756729573, 0.005637519322706221678, 0.005750417813181006761, 0.005806867058418394532, 0.005863316303655782304, 0.005919765548893170075, 0.005976214794130558713, 0.006089113284605340327, 0.006314910265554874932, 0.006766504227453943275, 0.007218098189353012485, 0.007669692151252081695 ),
 .UNSPECIFIED. ) ;
#40250=CARTESIAN_POINT ( 'NONE',  ( 175.1808269137907246, 281.3498469887747433, -14.26151238791351261 ) ) ;
#40252=CARTESIAN_POINT ( 'NONE',  ( -10.43332761869022640, 164.7833772461660544, -9.188101187500095079 ) ) ;
#40255=CARTESIAN_POINT ( 'NONE',  ( 151.1451503555562113, 268.8559155969762742, -15.81507177720227553 ) ) ;
#40256=CARTESIAN_POINT ( 'NONE',  ( 186.1033490533799579, 283.4419393130733624, 16.98975762302446668 ) ) ;
#40257=CARTESIAN_POINT ( 'NONE',  ( 194.8598199529639317, 293.1398868181796615, -15.91766051364927570 ) ) ;
#40259=CARTESIAN_POINT ( 'NONE',  ( 164.2712161151136172, 246.1209027979328710, 7.276091357954241445 ) ) ;
#40260=CARTESIAN_POINT ( 'NONE',  ( 191.0481192767711036, 299.7419460525905492, -9.103377665618040737 ) ) ;
#40261=CARTESIAN_POINT ( 'NONE',  ( 190.5726849661229210, 300.5654224342945326, -0.2192718484028965964 ) ) ;
#40263=CARTESIAN_POINT ( 'NONE',  ( 153.2106226585791831, 267.1006197558320991, -16.38176366188328359 ) ) ;
#40264=CARTESIAN_POINT ( 'NONE',  ( 161.5029716424245407, 251.3413373469583973, -13.00020995489466458 ) ) ;
#40265=CARTESIAN_POINT ( 'NONE',  ( 106.3178956768819319, 226.0643266524159856, -9.188101187500093303 ) ) ;
#40269=CARTESIAN_POINT ( 'NONE',  ( 157.2168982216852555, 258.3393398020932636, 18.09635675623264106 ) ) ;
#40271=CARTESIAN_POINT ( 'NONE',  ( 191.3729584906539003, 299.1793080298546101, -7.317708866624486497 ) ) ;
#40272=CARTESIAN_POINT ( 'NONE',  ( 196.5806080813426888, 290.1593943507663766, -16.31912166233602690 ) ) ;
#40274=CARTESIAN_POINT ( 'NONE',  ( 181.8129518053731033, 270.5384970965435514, -17.23398818032472946 ) ) ;
#40275=CARTESIAN_POINT ( 'NONE',  ( 173.1810892923022038, 289.7194164501482305, -1.146283512214450351 ) ) ;
#40279=CARTESIAN_POINT ( 'NONE',  ( 196.5361253761390685, 267.7136571270361287, 9.529754956671661503 ) ) ;
#40281=CARTESIAN_POINT ( 'NONE',  ( 176.7131714061462162, 273.8257724863759108, 17.80520185479879203 ) ) ;
#40282=CARTESIAN_POINT ( 'NONE',  ( 183.6324539711410750, 256.9743827782117478, 4.698106744110496891 ) ) ;
#40284=CARTESIAN_POINT ( 'NONE',  ( 184.7157775894015117, 297.3647472220100099, -4.497232409310948142 ) ) ;
#40285=CARTESIAN_POINT ( 'NONE',  ( 174.3506819931331506, 286.9267872025895940, 11.76311152586403885 ) ) ;
#40292=CARTESIAN_POINT ( 'NONE',  ( 164.1828665376937408, 279.9707757242401840, 12.51912677511460181 ) ) ;
#40294=CYLINDRICAL_SURFACE ( 'NONE', #82323, 10.00000000000010658 ) ;
#40299=CARTESIAN_POINT ( 'NONE',  ( 164.0741338217690668, 246.4622593432776796, 7.359073626423302983 ) ) ;
#40305=CARTESIAN_POINT ( 'NONE',  ( 155.5211745099813356, 261.2764194263634749, -17.18163098020766810 ) ) ;
#40308=FACE_OUTER_BOUND ( 'NONE', #92446, .T. ) ;
#40313=VECTOR ( 'NONE', #31340, 1000.000000000000000 ) ;
#40317=CARTESIAN_POINT ( 'NONE',  ( 190.6865851974790473, 300.3681414465920625, 2.985923517389160509 ) ) ;
#40319=FACE_OUTER_BOUND ( 'NONE', #54881, .T. ) ;
#40320=CARTESIAN_POINT ( 'NONE',  ( 185.5568049818104726, 266.1438378612298834, 14.60334785453874140 ) ) ;
#40321=CARTESIAN_POINT ( 'NONE',  ( 45.12761469462908792, 206.8615022471902876, 5.000000000000046185 ) ) ;
#40322=B_SPLINE_CURVE_WITH_KNOTS ( 'NONE', 3,
 ( #7967, #100177, #23139, #16053 ),
 .UNSPECIFIED., .F., .F.,
 ( 4, 4 ),
 ( 0.003503662168842324939, 0.007090156351249257347 ),
 .UNSPECIFIED. ) ;
#40323=CARTESIAN_POINT ( 'NONE',  ( 156.7043981061308102, 280.3628295831616697, 2.089248679677577325 ) ) ;
#40324=CARTESIAN_POINT ( 'NONE',  ( 132.6505673846437503, 238.2048013555409796, 4.594050593750051981 ) ) ;
#40325=CARTESIAN_POINT ( 'NONE',  ( 184.2837900991036690, 261.1937265540972817, -9.136837574883312385 ) ) ;
#40327=VERTEX_POINT ( 'NONE', #84383 ) ;
#40331=CARTESIAN_POINT ( 'NONE',  ( 203.5079006281358431, 276.1533853654332802, 13.32764713983298499 ) ) ;
#40333=CARTESIAN_POINT ( 'NONE',  ( 181.1417631960959511, 255.6584326465087713, 0.5790604069595610692 ) ) ;
#40334=CARTESIAN_POINT ( 'NONE',  ( 176.0127109592394277, 252.6004560315867593, -4.768680066900455650 ) ) ;
#40335=CARTESIAN_POINT ( 'NONE',  ( 192.1174645699329346, 297.8897856739996541, 12.27388818933617110 ) ) ;
#40336=CYLINDRICAL_SURFACE ( 'NONE', #98577, 10.00000000000010658 ) ;
#40338=CARTESIAN_POINT ( 'NONE',  ( 174.7842343859746563, 287.5387069739456365, -9.405270440949729860 ) ) ;
#40341=ORIENTED_EDGE ( 'NONE', *, *, #76713, .T. ) ;
#40342=CARTESIAN_POINT ( 'NONE',  ( 194.8708600166808651, 293.1207648669033006, -14.79199694356877970 ) ) ;
#40343=CARTESIAN_POINT ( 'NONE',  ( 3.808674319871268921, 184.5530062829863027, -4.648177544792955347E-16 ) ) ;
#40347=ADVANCED_FACE ( 'NONE', ( #61536 ), #16438, .T. ) ;
#40348=CARTESIAN_POINT ( 'NONE',  ( 190.6445454741162280, 284.1381220441062396, -17.32122990259229667 ) ) ;
#40349=CARTESIAN_POINT ( 'NONE',  ( 192.1722555058605337, 297.7948849891782857, -10.50817311975818491 ) ) ;
#40350=CARTESIAN_POINT ( 'NONE',  ( 149.0323968763055689, 272.5153119669064949, 11.64231532207353403 ) ) ;
#40351=CARTESIAN_POINT ( 'NONE',  ( 163.2437751800324293, 247.9004826992694461, 9.806027032984305336 ) ) ;
#40352=CARTESIAN_POINT ( 'NONE',  ( 161.6984845383829565, 281.6232062658947939, -6.601711233045046257 ) ) ;
#40353=CARTESIAN_POINT ( 'NONE',  ( 160.7277267915518451, 281.8993980653820017, 6.551854072316369404 ) ) ;
#40354=CARTESIAN_POINT ( 'NONE',  ( 199.9279498498847261, 267.4457311908202541, 6.228283794749674307 ) ) ;
#40356=CARTESIAN_POINT ( 'NONE',  ( 190.1607982559816890, 301.2788311432216233, -4.972636536415983244 ) ) ;
#40357=CARTESIAN_POINT ( 'NONE',  ( 187.1961889814599544, 261.9078172817692121, -8.752267960438080863 ) ) ;
#40360=CARTESIAN_POINT ( 'NONE',  ( 129.9777503372646095, 257.3967562850347122, -4.648177544792955347E-16 ) ) ;
#40361=CARTESIAN_POINT ( 'NONE',  ( 153.3703256797887775, 265.0017988796566897, 16.44314709207578318 ) ) ;
#40363=CARTESIAN_POINT ( 'NONE',  ( 193.9495889092963807, 294.7164532324382549, 15.46986001312306058 ) ) ;
#40365=CARTESIAN_POINT ( 'NONE',  ( -6.184650803196579893, 176.4244531367911293, -4.594050593750046652 ) ) ;
#40366=CARTESIAN_POINT ( 'NONE',  ( 90.56688509766992468, 223.0958772461660260, -9.188101187500095079 ) ) ;
#40369=CARTESIAN_POINT ( 'NONE',  ( 148.1316126177475496, 276.0755160693871630, 5.020219949272568094 ) ) ;
#40373=CARTESIAN_POINT ( 'NONE',  ( -22.42236680055709641, 157.8615022471902591, 0.000000000000000000 ) ) ;
#40376=CARTESIAN_POINT ( 'NONE',  ( 163.4055107321044318, 247.6203485056908846, -10.24153090796238530 ) ) ;
#40377=CARTESIAN_POINT ( 'NONE',  ( 178.4671845014859741, 289.9579026316837371, 9.503558631820238745 ) ) ;
#40378=CARTESIAN_POINT ( 'NONE',  ( 166.0486951412649148, 249.5559827260773886, -9.134215000997858880 ) ) ;
#40380=CARTESIAN_POINT ( 'NONE',  ( -13.92449252947024263, 172.7677522451419350, -5.000000000000047962 ) ) ;
#40381=CARTESIAN_POINT ( 'NONE',  ( 161.8750289368003621, 250.2712207352165592, -13.97436367953006098 ) ) ;
#40383=CARTESIAN_POINT ( 'NONE',  ( 37.90188877791127453, 186.5643266524160424, 9.188101187500095079 ) ) ;
#40385=CARTESIAN_POINT ( 'NONE',  ( 74.27495573685767738, 207.5643266524160424, 9.188101187500095079 ) ) ;
#40386=CARTESIAN_POINT ( 'NONE',  ( 183.2462649708989773, 258.1020939971272128, 7.820152278097399545 ) ) ;
#40388=CARTESIAN_POINT ( 'NONE',  ( 166.9983013567537000, 259.4879522421344973, 16.46229539392700048 ) ) ;
#40391=CARTESIAN_POINT ( 'NONE',  ( 176.1400978288397994, 269.8946129783859078, -16.59496141468774510 ) ) ;
#40399=CARTESIAN_POINT ( 'NONE',  ( 57.33281313167710636, 216.1589784336662206, -6.496448406907676862E-16 ) ) ;
#40402=CARTESIAN_POINT ( 'NONE',  ( 173.1206616589821010, 289.7470628071918668, -0.8130285733345999910 ) ) ;
#40404=CARTESIAN_POINT ( 'NONE',  ( 153.9658056652968980, 263.9703972898665825, 16.69902601383360619 ) ) ;
#40408=( BOUNDED_CURVE ( )  B_SPLINE_CURVE ( 2, ( #37779, #77296, #8395, #92048, #68681, #24085, #39265, #84434, #31669 ),
 .UNSPECIFIED., .F., .T. ) 
 B_SPLINE_CURVE_WITH_KNOTS ( ( 3, 2, 2, 2, 3 ),
 ( 0.9475806451612903691, 0.9489247311827957443, 0.9516129032258064946, 0.9543010752688172449, 0.9556451612903226200 ),
 .UNSPECIFIED. ) 
 CURVE ( )  GEOMETRIC_REPRESENTATION_ITEM ( )  RATIONAL_B_SPLINE_CURVE ( ( 0.9330127018922194093, 0.9330127018922194093, 1.000000000000000000, 0.8660254037844387076, 1.000000000000000000, 0.8660254037844387076, 1.000000000000000000, 0.9330127018922194093, 0.9330127018922194093 ) ) 
 REPRESENTATION_ITEM ( '' )  );
#40409=CARTESIAN_POINT ( 'NONE',  ( 192.4413533297683330, 287.8524838211871497, 16.04042031060856033 ) ) ;
#40410=CARTESIAN_POINT ( 'NONE',  ( 123.0699010352285825, 251.8615022471902876, 5.000000000000046185 ) ) ;
#40411=CARTESIAN_POINT ( 'NONE',  ( 20.30386484825465132, 170.9824982072973967, 3.021315404115420679E-15 ) ) ;
#40412=DIRECTION ( 'NONE',  ( -0.8660254037844387076, -0.4999999999999998890, -0.000000000000000000 ) ) ;
#40413=CARTESIAN_POINT ( 'NONE',  ( 149.3545991938273971, 273.9572411826421217, -10.14243178476390028 ) ) ;
#40414=CARTESIAN_POINT ( 'NONE',  ( 188.3480435840147322, 273.1765081552686070, 15.60535422690979424 ) ) ;
#40415=ORIENTED_EDGE ( 'NONE', *, *, #4791, .T. ) ;
#40416=CARTESIAN_POINT ( 'NONE',  ( 159.8188415394622268, 253.8326417772889840, -15.43862849427313222 ) ) ;
#40417=CARTESIAN_POINT ( 'NONE',  ( 151.9706434441667113, 279.1253449119590186, -0.3226571599251377709 ) ) ;
#40418=EDGE_CURVE ( 'NONE', #65011, #86855, #75940, .T. ) ;
#40420=VERTEX_POINT ( 'NONE', #70124 ) ;
#40421=CARTESIAN_POINT ( 'NONE',  ( 177.1809705214487849, 253.2799522049397751, -0.2609578167311901176 ) ) ;
#40422=ORIENTED_EDGE ( 'NONE', *, *, #88325, .T. ) ;
#40424=CARTESIAN_POINT ( 'NONE',  ( 167.5224888712764084, 247.9179630693595300, 3.541551421311048387 ) ) ;
#40425=CARTESIAN_POINT ( 'NONE',  ( 148.8264412599648097, 273.9886447002814975, 8.871318654940013815 ) ) ;
#40431=CARTESIAN_POINT ( 'NONE',  ( 167.0784635423869986, 276.4927169897987369, 15.85967558429602775 ) ) ;
#40433=CARTESIAN_POINT ( 'NONE',  ( 165.3929592122126451, 286.2279243276498732, 4.432946431554212197 ) ) ;
#40437=CARTESIAN_POINT ( 'NONE',  ( 183.1883525905292913, 295.7849739342112798, 1.003725237841741613 ) ) ;
#40439=CARTESIAN_POINT ( 'NONE',  ( 147.6095889327917803, 274.9796876144846465, -8.460961150142429332 ) ) ;
#40441=CARTESIAN_POINT ( 'NONE',  ( 193.7261517370125432, 295.1034577671335342, 14.97744313279139661 ) ) ;
#40442=CARTESIAN_POINT ( 'NONE',  ( 185.4422274959847527, 292.4385988784968617, -11.34057656226370447 ) ) ;
#40443=CARTESIAN_POINT ( 'NONE',  ( 205.2391015854675516, 275.1624436846170738, -14.01434138479280911 ) ) ;
#40444=CARTESIAN_POINT ( 'NONE',  ( 145.4512450625087467, 254.7833772461660544, -9.188101187500095079 ) ) ;
#40448=CARTESIAN_POINT ( 'NONE',  ( 80.17458025225667484, 217.0958772461660544, -9.188101187500095079 ) ) ;
#40450=CARTESIAN_POINT ( 'NONE',  ( 190.8443993347725325, 300.0947993426467519, 8.522468760355437212 ) ) ;
#40452=ORIENTED_EDGE ( 'NONE', *, *, #43624, .T. ) ;
#40453=CARTESIAN_POINT ( 'NONE',  ( 180.1800635485680573, 295.0721525882481160, 3.264262412682620962 ) ) ;
#40455=EDGE_CURVE ( 'NONE', #79518, #79225, #71662, .T. ) ;
#40458=CARTESIAN_POINT ( 'NONE',  ( 198.2505066714982149, 285.2670451491296149, 0.000000000000000000 ) ) ;
#40460=CARTESIAN_POINT ( 'NONE',  ( 207.9312334543074599, 270.4995345071110933, 1.552289074598145469 ) ) ;
#40461=CARTESIAN_POINT ( 'NONE',  ( 91.40610752940987993, 214.3923013555409796, 4.594050593750050204 ) ) ;
#40464=EDGE_CURVE ( 'NONE', #31220, #8428, #736, .T. ) ;
#40473=CARTESIAN_POINT ( 'NONE',  ( 99.68721513304873838, 238.3615022471903160, 5.000000000000046185 ) ) ;
#40475=ORIENTED_EDGE ( 'NONE', *, *, #69116, .T. ) ;
#40479=CARTESIAN_POINT ( 'NONE',  ( 206.6298919378964740, 272.7535241315335384, -9.267551915974392429 ) ) ;
#40480=EDGE_CURVE ( 'NONE', #87662, #53811, #83047, .T. ) ;
#40482=CARTESIAN_POINT ( 'NONE',  ( 177.1365833152386244, 284.6974615985632795, 13.05344454345314986 ) ) ;
#40483=CARTESIAN_POINT ( 'NONE',  ( 162.8839417982861448, 263.3994626277539055, 17.77684832337497767 ) ) ;
#40484=CARTESIAN_POINT ( 'NONE',  ( 195.4347729807024905, 279.6077732330228400, -17.24073704596056089 ) ) ;
#40485=VERTEX_POINT ( 'NONE', #63537 ) ;
#40486=CARTESIAN_POINT ( 'NONE',  ( 202.7724833007839891, 277.6125776806421186, -15.34270362070550497 ) ) ;
#40487=CARTESIAN_POINT ( 'NONE',  ( 200.3765029811139584, 283.5847115241710981, 16.85207472104531590 ) ) ;
#40491=CARTESIAN_POINT ( 'NONE',  ( 175.0130774361952035, 290.1460611646906500, -6.342396626919687641 ) ) ;
#40492=FACE_OUTER_BOUND ( 'NONE', #25260, .T. ) ;
#40494=CARTESIAN_POINT ( 'NONE',  ( 168.6156890688689884, 286.4116463664167895, -8.226575548882113509 ) ) ;
#40495=CARTESIAN_POINT ( 'NONE',  ( 206.9408877595175511, 272.2148635675444552, 6.707071080545934372 ) ) ;
#40497=CARTESIAN_POINT ( 'NONE',  ( 200.5914588262792222, 282.7033700937254821, -16.73555027083989444 ) ) ;
#40500=CARTESIAN_POINT ( 'NONE',  ( 168.8069195673892580, 272.9388147432762253, 15.96133530879710172 ) ) ;
#40501=CARTESIAN_POINT ( 'NONE',  ( 183.5555461010262661, 274.8638377643932813, 16.36404075196846364 ) ) ;
#40503=CARTESIAN_POINT ( 'NONE',  ( 188.8764293144468240, 259.6972905960182061, 3.583694637520717041 ) ) ;
#40505=CARTESIAN_POINT ( 'NONE',  ( 4.126898030318161936, 167.0643266524160424, 9.188101187500095079 ) ) ;
#40507=ORIENTED_EDGE ( 'NONE', *, *, #98843, .T. ) ;
#40508=CARTESIAN_POINT ( 'NONE',  ( 174.9245405914076343, 255.2035582809694176, 9.090376104202114504 ) ) ;
#40511=CARTESIAN_POINT ( 'NONE',  ( 14.27519936121077926, 188.2369531367911293, -4.594050593750048428 ) ) ;
#40512=CARTESIAN_POINT ( 'NONE',  ( 175.0125019719911847, 292.0719086349095051, 3.303583340955516423 ) ) ;
#40514=CARTESIAN_POINT ( 'NONE',  ( 177.8194257969418288, 292.8449071177858514, 6.006967295066290013 ) ) ;
#40515=CARTESIAN_POINT ( 'NONE',  ( 173.5658952278579363, 272.9572349787487724, -16.37894178319135818 ) ) ;
#40516=CARTESIAN_POINT ( 'NONE',  ( 196.6640600515679580, 290.0148512983446949, 16.35009042604046314 ) ) ;
#40517=CARTESIAN_POINT ( 'NONE',  ( 133.5964594837526533, 259.4860189848785694, -2.679491924311252493 ) ) ;
#40518=CARTESIAN_POINT ( 'NONE',  ( 169.9907874252009492, 274.9766311711105118, 17.04400878134698161 ) ) ;
#40520=CARTESIAN_POINT ( 'NONE',  ( 187.1121570753812193, 296.0775264014479831, -7.699669239627596973 ) ) ;
#40523=CARTESIAN_POINT ( 'NONE',  ( 192.9866187040997829, 295.5921736933902935, -12.74678698041507197 ) ) ;
#40524=CARTESIAN_POINT ( 'NONE',  ( 68.07728789491679322, 200.1115022471901739, -5.000000000000041744 ) ) ;
#40527=CARTESIAN_POINT ( 'NONE',  ( 203.3903727158224228, 270.0836496803775049, 6.045350443737255830 ) ) ;
#40528=CARTESIAN_POINT ( 'NONE',  ( 34.97905304013878691, 184.8768266524159856, 9.188101187500098632 ) ) ;
#40529=CARTESIAN_POINT ( 'NONE',  ( 198.0792648159935538, 287.5636447432459022, 17.04758482866669667 ) ) ;
#40531=CARTESIAN_POINT ( 'NONE',  ( 150.6916211261701619, 269.6414512649903941, -15.44346024757110847 ) ) ;
#40534=VERTEX_POINT ( 'NONE', #18968 ) ;
#40535=CARTESIAN_POINT ( 'NONE',  ( 3.630564096624801174, 166.2365022471902307, 10.00000000000009948 ) ) ;
#40536=CARTESIAN_POINT ( 'NONE',  ( 144.9899443387551798, 254.5170451491295296, 0.000000000000000000 ) ) ;
#40537=FACE_OUTER_BOUND ( 'NONE', #69328, .T. ) ;
#40538=CARTESIAN_POINT ( 'NONE',  ( 162.8839417982861448, 263.3994626277539055, 17.77684832337497767 ) ) ;
#40540=CARTESIAN_POINT ( 'NONE',  ( 162.6626107288841467, 248.9070890562113902, 10.12509462564867313 ) ) ;
#40541=CARTESIAN_POINT ( 'NONE',  ( 149.4908848037268001, 271.7211875819559737, -12.92288068979413573 ) ) ;
#40542=CARTESIAN_POINT ( 'NONE',  ( 185.6900645067668165, 267.8684138037842786, -14.44923933729529963 ) ) ;
#40548=ORIENTED_EDGE ( 'NONE', *, *, #25961, .T. ) ;
#40549=CARTESIAN_POINT ( 'NONE',  ( 106.0403798229140619, 220.4824982072973683, 3.021315404115420679E-15 ) ) ;
#40551=EDGE_CURVE ( 'NONE', #86134, #30236, #29295, .T. ) ;
#40552=CARTESIAN_POINT ( 'NONE',  ( 177.3939513230285172, 256.1386864175269125, -7.257050990210307084 ) ) ;
#40553=CARTESIAN_POINT ( 'NONE',  ( 190.4841013044967042, 300.7188538369516095, 4.682298117523464143 ) ) ;
#40555=ORIENTED_EDGE ( 'NONE', *, *, #9370, .T. ) ;
#40556=CARTESIAN_POINT ( 'NONE',  ( 186.3138662162842820, 272.0885644523062865, -16.12950033991073795 ) ) ;
#40557=ORIENTED_EDGE ( 'NONE', *, *, #81441, .F. ) ;
#40562=CARTESIAN_POINT ( 'NONE',  ( 205.2391015854675516, 275.1624436846170738, -14.01434138479280911 ) ) ;
#40563=CARTESIAN_POINT ( 'NONE',  ( 106.4801018922090066, 232.2833772461660544, -9.188101187500095079 ) ) ;
#40564=CARTESIAN_POINT ( 'NONE',  ( 199.0746189151364831, 265.2438329385483939, 1.559867394473611002 ) ) ;
#40566=CARTESIAN_POINT ( 'NONE',  ( 161.7243182998967939, 267.0551689734765546, 16.50076583471866343 ) ) ;
#40571=CARTESIAN_POINT ( 'NONE',  ( 59.55252387252222945, 199.0643266524159856, -9.188101187500093303 ) ) ;
#40573=CARTESIAN_POINT ( 'NONE',  ( 191.1489696025915919, 299.5672681643093256, 8.892130899335590755 ) ) ;
#40574=DIRECTION ( 'NONE',  ( -0.8660254037844387076, -0.4999999999999998890, -0.000000000000000000 ) ) ;
#40575=CARTESIAN_POINT ( 'NONE',  ( 176.2720603235588612, 273.0790378244862495, 17.50981446612852821 ) ) ;
#40580=CARTESIAN_POINT ( 'NONE',  ( 189.8763472015711216, 301.7715148217271803, -0.1184663095182975079 ) ) ;
#40582=CARTESIAN_POINT ( 'NONE',  ( 175.4182666330609095, 261.1119833641568562, -14.60109906219532228 ) ) ;
#40584=CARTESIAN_POINT ( 'NONE',  ( 161.1492466472929266, 251.5283125358769212, -13.33353587056634915 ) ) ;
#40585=CARTESIAN_POINT ( 'NONE',  ( 192.5143468344189728, 297.2023654272867361, -12.06830393602581530 ) ) ;
#40588=CARTESIAN_POINT ( 'NONE',  ( 149.6071296322179194, 271.5198456328920997, 12.75640156477042453 ) ) ;
#40589=CARTESIAN_POINT ( 'NONE',  ( 180.0263293189807143, 270.7602331593356553, 17.37738868372918333 ) ) ;
#40593=FACE_OUTER_BOUND ( 'NONE', #35977, .T. ) ;
#40594=ADVANCED_FACE ( 'NONE', ( #1762 ), #48914, .F. ) ;
#40595=CARTESIAN_POINT ( 'NONE',  ( 113.3268549190559753, 245.4244531367911293, -4.594050593750046652 ) ) ;
#40596=EDGE_LOOP ( 'NONE', ( #89140, #18220, #15802, #86894 ) ) ;
#40597=CARTESIAN_POINT ( 'NONE',  ( 147.2999496562918296, 275.5159985734018164, -0.1418322875769767455 ) ) ;
#40600=ADVANCED_FACE ( 'NONE', ( #44216 ), #81287, .T. ) ;
#40601=CARTESIAN_POINT ( 'NONE',  ( 155.4661767250933622, 261.3716783840932294, -17.10192542004562810 ) ) ;
#40602=CARTESIAN_POINT ( 'NONE',  ( 163.9149533033796047, 246.7379680887036670, 7.273005089308705706 ) ) ;
#40605=CARTESIAN_POINT ( 'NONE',  ( 177.4875709022480805, 255.0843569672325373, 4.885038851980863406 ) ) ;
#40607=CARTESIAN_POINT ( 'NONE',  ( 172.3986314675530309, 263.7922717222033384, -16.89442142407995107 ) ) ;
#40608=B_SPLINE_CURVE_WITH_KNOTS ( 'NONE', 3,
 ( #36512, #45112, #83662, #14224 ),
 .UNSPECIFIED., .F., .F.,
 ( 4, 4 ),
 ( 0.009430154199042148702, 0.01486991593141949626 ),
 .UNSPECIFIED. ) ;
#40609=CARTESIAN_POINT ( 'NONE',  ( 158.5191741753731094, 275.0318726483118894, -12.49859467851711514 ) ) ;
#40610=CARTESIAN_POINT ( 'NONE',  ( 185.6923914186591276, 262.0522634787053562, 9.806237466387484503 ) ) ;
#40611=CARTESIAN_POINT ( 'NONE',  ( 206.0977829604818510, 273.6751639155793896, -9.820003938885891515 ) ) ;
#40612=CARTESIAN_POINT ( 'NONE',  ( 131.6216415740022398, 255.9869531367911009, 4.594050593750046652 ) ) ;
#40613=CARTESIAN_POINT ( 'NONE',  ( 198.7136873185829984, 286.4647927352960437, -18.57144721070432070 ) ) ;
#40614=CARTESIAN_POINT ( 'NONE',  ( 190.1413301607522044, 298.8649611522849341, -8.184056379218567656 ) ) ;
#40616=CARTESIAN_POINT ( 'NONE',  ( 63.55789136502527015, 201.3768266524160140, 9.188101187500098632 ) ) ;
#40620=CARTESIAN_POINT ( 'NONE',  ( 171.6722295479746947, 260.3874344878792044, 14.68526897012709220 ) ) ;
#40621=CARTESIAN_POINT ( 'NONE',  ( 155.0819613845161768, 280.3159068740167186, -0.8634000510104499204 ) ) ;
#40622=CARTESIAN_POINT ( 'NONE',  ( 178.8456940037896743, 291.7693823845650059, -6.757125974697903992 ) ) ;
#40624=CARTESIAN_POINT ( 'NONE',  ( 203.3349860717029571, 278.4604684979374838, -16.59553970625579566 ) ) ;
#40625=CARTESIAN_POINT ( 'NONE',  ( 157.2843776208655697, 270.8446288838524652, -14.72886913550468257 ) ) ;
#40626=CARTESIAN_POINT ( 'NONE',  ( 120.7424577590100654, 230.5177522451417929, 5.000000000000051514 ) ) ;
#40628=ORIENTED_EDGE ( 'NONE', *, *, #93507, .F. ) ;
#40629=EDGE_CURVE ( 'NONE', #25829, #6621, #93371, .T. ) ;
#40630=CARTESIAN_POINT ( 'NONE',  ( 190.5154909595809727, 300.6644853595138329, -0.04129855346138300298 ) ) ;
#40631=B_SPLINE_CURVE_WITH_KNOTS ( 'NONE', 3,
 ( #19516, #67066, #81329, #51368 ),
 .UNSPECIFIED., .F., .F.,
 ( 4, 4 ),
 ( 0.008479649949678834397, 0.01357937252561114416 ),
 .UNSPECIFIED. ) ;
#40632=B_SPLINE_CURVE_WITH_KNOTS ( 'NONE', 3,
 ( #78703, #53864, #84825, #46261, #93928, #7790, #32071 ),
 .UNSPECIFIED., .F., .F.,
 ( 4, 3, 4 ),
 ( 6.109341443789230770E-15, 0.001498044977023242066, 0.004247078789804528687 ),
 .UNSPECIFIED. ) ;
#40633=CARTESIAN_POINT ( 'NONE',  ( 35.03300607999280913, 191.0333772461660544, 9.188101187500095079 ) ) ;
#40635=CARTESIAN_POINT ( 'NONE',  ( 43.57052534665006505, 184.4155109091896065, 2.679491924311254714 ) ) ;
#40636=CARTESIAN_POINT ( 'NONE',  ( 188.7612856390439333, 290.4500619787207825, -14.79637974347269491 ) ) ;
#40640=CARTESIAN_POINT ( 'NONE',  ( 59.32682287396359300, 198.3927522451418213, 10.00000000000009592 ) ) ;
#40641=CARTESIAN_POINT ( 'NONE',  ( 128.4024327899592208, 233.3932355074535678, -2.679491924311248496 ) ) ;
#40642=CARTESIAN_POINT ( 'NONE',  ( 184.3152199276001966, 257.8157294273448201, 1.347602273921576499 ) ) ;
#40643=CARTESIAN_POINT ( 'NONE',  ( 157.1850763439666139, 258.3944569110938687, -16.98181238659443437 ) ) ;
#40646=CARTESIAN_POINT ( 'NONE',  ( 28.67313202272483252, 177.3615022471902023, 5.000000000000051514 ) ) ;
#40647=CARTESIAN_POINT ( 'NONE',  ( 147.7245617474428911, 256.0958772461660828, -9.188101187500095079 ) ) ;
#40648=CARTESIAN_POINT ( 'NONE',  ( 202.6560281492536717, 279.6364581158209717, 17.15553667345918853 ) ) ;
#40649=CARTESIAN_POINT ( 'NONE',  ( 148.9967968810750563, 247.6423013555410080, -4.594050593750043987 ) ) ;
#40652=CARTESIAN_POINT ( 'NONE',  ( 170.4714877815671343, 263.5862471893055954, 15.80051778782658900 ) ) ;
#40653=CARTESIAN_POINT ( 'NONE',  ( 192.4202172926039793, 297.3654025762033370, 10.98569444949570872 ) ) ;
#40655=CARTESIAN_POINT ( 'NONE',  ( 164.2545401858843945, 246.1497863546213978, 2.275217130759496609 ) ) ;
#40660=CARTESIAN_POINT ( 'NONE',  ( 193.2752197284765998, 263.9480352582601768, 7.898392093415175452 ) ) ;
#40661=CARTESIAN_POINT ( 'NONE',  ( 55.77019854693759271, 214.5530062829863311, -4.648177544792955347E-16 ) ) ;
#40663=CARTESIAN_POINT ( 'NONE',  ( 166.4691412992503672, 285.8895934590825050, 0.4981257345838445705 ) ) ;
#40665=CARTESIAN_POINT ( 'NONE',  ( 160.4469838632686844, 252.7446673580718368, 14.71213094057149995 ) ) ;
#40667=CARTESIAN_POINT ( 'NONE',  ( 159.2289198208967775, 254.8544161663325838, -15.88961297684315888 ) ) ;
#40669=VERTEX_POINT ( 'NONE', #92366 ) ;
#40670=CYLINDRICAL_SURFACE ( 'NONE', #79759, 10.00000000000010658 ) ;
#40671=CARTESIAN_POINT ( 'NONE',  ( 164.9836323268835940, 244.8869617230113249, -2.696511969808454534 ) ) ;
#40674=CARTESIAN_POINT ( 'NONE',  ( 207.6523394534040392, 270.9825930866021508, -2.115019688068903392 ) ) ;
#40675=CARTESIAN_POINT ( 'NONE',  ( 194.1493756275458793, 294.3704124857528655, 13.94613522129020744 ) ) ;
#40678=CARTESIAN_POINT ( 'NONE',  ( 157.0110656778546740, 277.1938971196430543, -9.979977716902725504 ) ) ;
#40680=EDGE_LOOP ( 'NONE', ( #4444, #93383, #71977, #72397 ) ) ;
#40682=CARTESIAN_POINT ( 'NONE',  ( 188.5140216088474006, 298.0167532018325005, 7.839324137471839649 ) ) ;
#40688=CARTESIAN_POINT ( 'NONE',  ( 200.3414094930810165, 283.6454952284590263, 16.87912319229835489 ) ) ;
#40690=CARTESIAN_POINT ( 'NONE',  ( 191.2729698983822288, 299.3524933518466469, 8.871011392605806734 ) ) ;
#40691=CARTESIAN_POINT ( 'NONE',  ( 151.4273961969814764, 275.0250855714808154, -8.568716987504124916 ) ) ;
#40692=ORIENTED_EDGE ( 'NONE', *, *, #92076, .T. ) ;
#40693=CARTESIAN_POINT ( 'NONE',  ( 170.6620473226114143, 255.5658883142887703, -11.58147698829965222 ) ) ;
#40694=CARTESIAN_POINT ( 'NONE',  ( 163.1691520398773321, 248.0297337694385931, 11.21816141384514331 ) ) ;
#40699=CARTESIAN_POINT ( 'NONE',  ( 161.1561989937922021, 271.1185073049681478, 16.16522359423900923 ) ) ;
#40700=ORIENTED_EDGE ( 'NONE', *, *, #89795, .T. ) ;
#40701=( BOUNDED_CURVE ( )  B_SPLINE_CURVE ( 2, ( #21991, #13417, #43785, #98014, #68090, #5308, #7285, #20517, #13897 ),
 .UNSPECIFIED., .F., .T. ) 
 B_SPLINE_CURVE_WITH_KNOTS ( ( 3, 2, 2, 2, 3 ),
 ( 0.9717741935483871218, 0.9731182795698924970, 0.9758064516129032473, 0.9784946236559139976, 0.9798387096774193727 ),
 .UNSPECIFIED. ) 
 CURVE ( )  GEOMETRIC_REPRESENTATION_ITEM ( )  RATIONAL_B_SPLINE_CURVE ( ( 0.9330127018922194093, 0.9330127018922194093, 1.000000000000000000, 0.8660254037844387076, 1.000000000000000000, 0.8660254037844387076, 1.000000000000000000, 0.9330127018922194093, 0.9330127018922194093 ) ) 
 REPRESENTATION_ITEM ( '' )  );
#40705=B_SPLINE_CURVE_WITH_KNOTS ( 'NONE', 3,
 ( #18716, #86664, #26314, #84773, #49598, #87181, #72936, #94244, #95260, #71922, #3527, #80047, #17196, #40491, #71421, #48099, #94738, #56187, #25300, #95762, #57189, #48617, #18218, #1525, #79040, #88168, #79556, #25826, #34404, #10111, #2524, #10614, #53809, #15309, #72435, #77126, #7732, #38620, #52091, #4500, #90139, #42483, #59680, #65789 ),
 .UNSPECIFIED., .F., .F.,
 ( 4, 2, 2, 2, 2, 2, 2, 2, 2, 2, 2, 2, 2, 2, 2, 2, 2, 2, 2, 2, 2, 4 ),
 ( 0.001166255102719954443, 0.001645796290616598646, 0.002125337478513243065, 0.002365108072461565708, 0.002604878666409887918, 0.002724763963384048589, 0.002844649260358210127, 0.002964534557332370798, 0.003084419854306532337, 0.003563961042203122112, 0.004043502230099711020, 0.005002584605892812508, 0.005961666981685913996, 0.006441208169582427444, 0.006920749357478940891, 0.007040634654453109369, 0.007100577302940112509, 0.007160519951427115649, 0.007400290545375051883, 0.007879831733270893993, 0.008359372921166736969, 0.008838914109062578212 ),
 .UNSPECIFIED. ) ;
#40707=CARTESIAN_POINT ( 'NONE',  ( 192.0332533962074706, 298.0356437054567778, 11.70630383928353346 ) ) ;
#40709=CARTESIAN_POINT ( 'NONE',  ( 123.0902549634681407, 230.3262482093457777, 3.021315404115420679E-15 ) ) ;
#40710=VERTEX_POINT ( 'NONE', #16818 ) ;
#40713=CARTESIAN_POINT ( 'NONE',  ( 164.7762319088960794, 245.2461897844768828, 2.994040459560653122 ) ) ;
#40714=CARTESIAN_POINT ( 'NONE',  ( 190.3443929803903814, 298.9608357525441420, -8.219721500574586059 ) ) ;
#40715=CARTESIAN_POINT ( 'NONE',  ( 207.0309969265819063, 271.4803781728614354, 5.109250008308237945 ) ) ;
#40718=CARTESIAN_POINT ( 'NONE',  ( 168.4288024578681302, 257.2676070226289085, -14.34928285719503727 ) ) ;
#40719=EDGE_CURVE ( 'NONE', #82888, #73927, #72925, .T. ) ;
#40721=CARTESIAN_POINT ( 'NONE',  ( 161.7910648966377209, 250.4166507187868831, 13.19274492748169436 ) ) ;
#40722=CARTESIAN_POINT ( 'NONE',  ( 190.9750444319660119, 261.6428408136690109, -0.08634532216184034881 ) ) ;
#40725=CARTESIAN_POINT ( 'NONE',  ( 139.8153705705071843, 239.9824982072973967, 3.021315404115420679E-15 ) ) ;
#40726=CARTESIAN_POINT ( 'NONE',  ( 207.6727254509676186, 270.9472835030587703, 7.315149605389819953 ) ) ;
#40727=CARTESIAN_POINT ( 'NONE',  ( 21.07736754015091662, 169.6427522451417644, 1.119607411625061291E-15 ) ) ;
#40728=CARTESIAN_POINT ( 'NONE',  ( 96.71051312758956442, 217.4548013555409511, -4.594050593750042211 ) ) ;
#40730=CARTESIAN_POINT ( 'NONE',  ( 90.43156862655462191, 233.0177522451419350, 5.000000000000046185 ) ) ;
#40731=CARTESIAN_POINT ( 'NONE',  ( 207.9670239186021377, 270.4375436045261836, 3.151456135821919968 ) ) ;
#40733=CARTESIAN_POINT ( 'NONE',  ( -0.2035760843690503918, 176.8149278399160949, -9.188101187500095079 ) ) ;
#40734=CYLINDRICAL_SURFACE ( 'NONE', #88554, 10.00000000000010658 ) ;
#40735=CARTESIAN_POINT ( 'NONE',  ( 200.7079229450794173, 283.0106753079404029, 16.90512463913211505 ) ) ;
#40738=DIRECTION ( 'NONE',  ( -0.4999999999999998890, 0.8660254037844387076, 0.000000000000000000 ) ) ;
#40741=CARTESIAN_POINT ( 'NONE',  ( 161.8935665241663457, 250.2391126920490194, -13.69501063978231770 ) ) ;
#40742=CARTESIAN_POINT ( 'NONE',  ( 182.9576018746647890, 284.4981050466655006, 14.97526635527638739 ) ) ;
#40744=CARTESIAN_POINT ( 'NONE',  ( 26.10194555558327778, 192.0024278399160949, -9.188101187500093303 ) ) ;
#40745=CARTESIAN_POINT ( 'NONE',  ( 83.57553417992789946, 212.3927522451417929, -10.00000000000009059 ) ) ;
#40746=CARTESIAN_POINT ( 'NONE',  ( 92.25929090966846502, 235.6199935810940929, 2.679491924311251605 ) ) ;
#40750=CARTESIAN_POINT ( 'NONE',  ( -6.887775800123916881, 157.6423013555410080, -4.594050593750043987 ) ) ;
#40752=CARTESIAN_POINT ( 'NONE',  ( 207.8431546909062320, 270.6520914003897360, -6.441273666418043220 ) ) ;
#40753=CARTESIAN_POINT ( 'NONE',  ( 192.0969986600162827, 271.0201763999182845, -15.22553433325905736 ) ) ;
#40754=CARTESIAN_POINT ( 'NONE',  ( 148.2670916631250861, 273.8408594794321971, -7.980554973576580835 ) ) ;
#40756=CARTESIAN_POINT ( 'NONE',  ( 171.4574698082410009, 280.1005400806686225, 15.30362981370621611 ) ) ;
#40757=CARTESIAN_POINT ( 'NONE',  ( 146.9235493515124062, 276.1679430252639804, 0.7994986043261682607 ) ) ;
#40758=FACE_OUTER_BOUND ( 'NONE', #38771, .T. ) ;
#40760=CARTESIAN_POINT ( 'NONE',  ( 164.4678285797544106, 245.7803600197737524, -6.875991496205872799 ) ) ;
#40762=CARTESIAN_POINT ( 'NONE',  ( 110.0256537107753161, 225.1423013555409796, -4.594050593750043987 ) ) ;
#40765=DIRECTION ( 'NONE',  ( -0.8660254037844387076, -0.4999999999999998890, -0.000000000000000000 ) ) ;
#40768=CARTESIAN_POINT ( 'NONE',  ( 204.3238350981471001, 272.7781662703540064, -9.746153380280240697 ) ) ;
#40769=CARTESIAN_POINT ( 'NONE',  ( 190.0900669226457751, 261.8932147952297669, -4.414057574442162846 ) ) ;
#40770=CARTESIAN_POINT ( 'NONE',  ( 148.9194629746633893, 272.7109192224475009, -12.27648025871169679 ) ) ;
#40771=CARTESIAN_POINT ( 'NONE',  ( 110.7831656154889970, 234.7677522451418497, 10.00000000000009592 ) ) ;
#40772=CARTESIAN_POINT ( 'NONE',  ( 203.5517807763935991, 276.4131063546051337, 14.32831804246049678 ) ) ;
#40777=CARTESIAN_POINT ( 'NONE',  ( 167.9438064097205370, 271.4634641811414895, -17.49863926106802126 ) ) ;
#40779=B_SPLINE_SURFACE_WITH_KNOTS ( 'NONE', 3, 1, ( 
 ( #64535, #8824 ),
 ( #79778, #80276 ),
 ( #64029, #94971 ),
 ( #87419, #10343 ),
 ( #72149, #16919 ),
 ( #2754, #33644 ),
 ( #95494, #78243 ),
 ( #47808, #1749 ),
 ( #56916, #18447 ),
 ( #94465, #32116 ),
 ( #86892, #49336 ),
 ( #63025, #93970 ),
 ( #32628, #63525 ),
 ( #17426, #57415 ),
 ( #34622, #50320 ),
 ( #4219, #12849 ),
 ( #66520, #36603 ),
 ( #80787, #81763 ),
 ( #20946, #51304 ),
 ( #42215, #97447 ),
 ( #82276, #59391 ),
 ( #44201, #81272 ),
 ( #36105, #88902 ),
 ( #43708, #12337 ),
 ( #11846, #74650 ),
 ( #73635, #18950 ),
 ( #28017, #20436 ),
 ( #42703, #28510 ),
 ( #65522, #58891 ),
 ( #35117, #50814 ),
 ( #90367, #96471 ),
 ( #43202, #82769 ),
 ( #5714, #5227 ),
 ( #11361, #27039 ) ),
 .UNSPECIFIED., .T., .F., .F.,
 ( 4, 2, 2, 2, 2, 2, 2, 2, 2, 2, 2, 2, 2, 2, 2, 2, 4 ),
 ( 2, 2 ),
 ( 0.000000000000000000, 0.06250000000000000000, 0.1250000000000000000, 0.1875000000000000000, 0.2500000000000000000, 0.3125000000000000000, 0.3750000000000000000, 0.4375000000000000000, 0.5000000000000000000, 0.5625000000000000000, 0.6250000000000000000, 0.6875000000000000000, 0.7500000000000000000, 0.8125000000000000000, 0.8750000000000000000, 0.9375000000000000000, 1.000000000000000000 ),
 ( 0.000000000000000000, 1.000000000000000000 ),
 .UNSPECIFIED. ) ;
#40780=EDGE_CURVE ( 'NONE', #91328, #99484, #88558, .T. ) ;
#40781=CARTESIAN_POINT ( 'NONE',  ( 198.1925917153872376, 271.8148388623765186, 12.14180242448621527 ) ) ;
#40786=CARTESIAN_POINT ( 'NONE',  ( 192.7259387352017939, 296.8358775046606297, 11.24705370801146209 ) ) ;
#40788=CYLINDRICAL_SURFACE ( 'NONE', #18073, 10.00000000000010658 ) ;
#40789=ADVANCED_FACE ( 'NONE', ( #91983 ), #99546, .T. ) ;
#40791=CARTESIAN_POINT ( 'NONE',  ( 174.1430845602542945, 272.9649943977126441, -16.36010906446035307 ) ) ;
#40792=ORIENTED_EDGE ( 'NONE', *, *, #53213, .F. ) ;
#40795=CARTESIAN_POINT ( 'NONE',  ( -22.42236680055709641, 157.8615022471902591, 0.000000000000000000 ) ) ;
#40796=CARTESIAN_POINT ( 'NONE',  ( 164.4430760075033788, 246.2065693058222564, -1.743745055932603538 ) ) ;
#40799=CARTESIAN_POINT ( 'NONE',  ( 187.6671935738553714, 292.4988616513966235, 12.35105147068263065 ) ) ;
#40802=CARTESIAN_POINT ( 'NONE',  ( 202.9547455376043672, 279.1190644220934018, -15.19669173352461478 ) ) ;
#40805=CARTESIAN_POINT ( 'NONE',  ( 178.6928612807282946, 260.5973771377355774, 11.99803804170878863 ) ) ;
#40813=CARTESIAN_POINT ( 'NONE',  ( 190.5561904564986833, 300.5939917630097966, 3.348721477520653966 ) ) ;
#40814=CARTESIAN_POINT ( 'NONE',  ( 196.7432902728890269, 284.8136100218615070, -17.21513713512148058 ) ) ;
#40816=CARTESIAN_POINT ( 'NONE',  ( 201.4520623681621316, 281.7217880192456505, -17.56577389517433119 ) ) ;
#40818=CARTESIAN_POINT ( 'NONE',  ( 157.8621261317385915, 281.2061543397735477, 2.756635258921121601 ) ) ;
#40819=CARTESIAN_POINT ( 'NONE',  ( 121.9060058492368483, 247.3149278399160949, -9.188101187500095079 ) ) ;
#40827=CARTESIAN_POINT ( 'NONE',  ( 203.5517529213690295, 276.4076950671145596, 13.56830733209305251 ) ) ;
#40830=CARTESIAN_POINT ( 'NONE',  ( 192.0519773745460554, 298.0032128236547351, 11.68523422658327249 ) ) ;
#40831=CARTESIAN_POINT ( 'NONE',  ( 153.3750525283932689, 276.8757596813744044, 7.147645658179857087 ) ) ;
#40833=CARTESIAN_POINT ( 'NONE',  ( 174.3376866340771869, 288.4003068613999972, -10.07124184041177450 ) ) ;
#40834=CARTESIAN_POINT ( 'NONE',  ( 192.6470520760290981, 292.3461483602033013, -14.37014842569768192 ) ) ;
#40837=CARTESIAN_POINT ( 'NONE',  ( 147.9133274879049793, 274.4535970048112290, -9.359166267164972908 ) ) ;
#40838=CARTESIAN_POINT ( 'NONE',  ( 152.5693996133281587, 273.3850609750195417, 11.87574206830028878 ) ) ;
#40839=ORIENTED_EDGE ( 'NONE', *, *, #32486, .F. ) ;
#40841=CARTESIAN_POINT ( 'NONE',  ( 191.0043802832096844, 283.4987559632036778, -16.57480583703641130 ) ) ;
#40842=CARTESIAN_POINT ( 'NONE',  ( 191.7656802644930849, 298.4990939643267893, -9.391040447064041174 ) ) ;
#40843=CARTESIAN_POINT ( 'NONE',  ( 149.6877696051026305, 271.3801731027346591, 11.89134584187677390 ) ) ;
#40845=CARTESIAN_POINT ( 'NONE',  ( 202.4017613376760494, 280.0768611521521620, 15.73960524502980540 ) ) ;
#40846=CARTESIAN_POINT ( 'NONE',  ( 153.5022104429997398, 269.9741907477366567, 14.95430817309988747 ) ) ;
#40847=CARTESIAN_POINT ( 'NONE',  ( 160.9022227064159836, 281.5926560585749598, 6.018336957399161413 ) ) ;
#40849=CARTESIAN_POINT ( 'NONE',  ( 152.8721808860877616, 265.8646109718731623, -17.65676496037632504 ) ) ;
#40850=EDGE_LOOP ( 'NONE', ( #76497, #72688, #10305, #2369 ) ) ;
#40851=CARTESIAN_POINT ( 'NONE',  ( 164.6353421851925702, 280.3989608998424501, -11.20704416911448753 ) ) ;
#40853=CARTESIAN_POINT ( 'NONE',  ( 193.0512205562391159, 275.6825563886401369, -16.88465587640301280 ) ) ;
#40854=DIRECTION ( 'NONE',  ( -0.8660254037844387076, -0.4999999999999998890, -0.000000000000000000 ) ) ;
#40856=CARTESIAN_POINT ( 'NONE',  ( 14.99168702176358892, 167.9155109091896065, 2.679491924311228512 ) ) ;
#40861=CARTESIAN_POINT ( 'NONE',  ( -17.68663747114990770, 172.8464784336661353, 1.353441290958777525E-15 ) ) ;
#40862=CARTESIAN_POINT ( 'NONE',  ( 89.26784699199328088, 222.3458772461660544, 9.188101187500095079 ) ) ;
#40863=CARTESIAN_POINT ( 'NONE',  ( 155.5211745099813356, 261.2764194263634749, -17.18163098020766810 ) ) ;
#40864=CARTESIAN_POINT ( 'NONE',  ( 192.4867975473904949, 297.2500821921321972, -13.04960750009181325 ) ) ;
#40865=CARTESIAN_POINT ( 'NONE',  ( 147.7236348786572933, 275.2192751642206190, 4.007618914242884856 ) ) ;
#40866=EDGE_CURVE ( 'NONE', #50800, #2973, #22107, .T. ) ;
#40867=DIRECTION ( 'NONE',  ( 0.4999999999999998890, -0.8660254037844385966, 0.000000000000000000 ) ) ;
#40869=CARTESIAN_POINT ( 'NONE',  ( 161.0423214198712856, 281.7177014927175946, 5.594616910120793207 ) ) ;
#40871=CARTESIAN_POINT ( 'NONE',  ( 162.8480293090835005, 248.5859346546387769, -9.753154585358942086 ) ) ;
#40872=CARTESIAN_POINT ( 'NONE',  ( 177.8711684648900757, 290.0939523432613214, 9.786701248066272285 ) ) ;
#40874=CARTESIAN_POINT ( 'NONE',  ( 151.1237910559533475, 270.8929109891034841, -13.93008610078706688 ) ) ;
#40878=CARTESIAN_POINT ( 'NONE',  ( 36.84650709099022947, 182.8923013555409796, 4.594050593750050204 ) ) ;
#40880=CARTESIAN_POINT ( 'NONE',  ( 70.62149783858335184, 202.3923013555409796, 4.594050593750050204 ) ) ;
#40881=CARTESIAN_POINT ( 'NONE',  ( 161.1747502674735415, 251.4841389699472529, -13.25152330924089839 ) ) ;
#40883=CARTESIAN_POINT ( 'NONE',  ( 165.3184754677606918, 258.9335273930299195, 15.57829592379341044 ) ) ;
#40884=CARTESIAN_POINT ( 'NONE',  ( 198.4146594612899719, 286.4472197769862873, -17.06352273131960473 ) ) ;
#40885=CARTESIAN_POINT ( 'NONE',  ( 199.9968460962569452, 284.2422965381864515, 16.92744394710046762 ) ) ;
#40886=CARTESIAN_POINT ( 'NONE',  ( 173.6170773432991155, 268.4804802943822892, -16.29536237713207569 ) ) ;
#40890=ORIENTED_EDGE ( 'NONE', *, *, #98844, .T. ) ;
#40892=CARTESIAN_POINT ( 'NONE',  ( 78.52397964811635234, 206.9548013555409796, -4.594050593750042211 ) ) ;
#40893=CARTESIAN_POINT ( 'NONE',  ( 193.7190926099759736, 281.1151242756019997, 17.77946842270920413 ) ) ;
#40894=CARTESIAN_POINT ( 'NONE',  ( 169.1636391637144357, 288.4733247442767379, -1.122355453443255602 ) ) ;
#40897=B_SPLINE_CURVE_WITH_KNOTS ( 'NONE', 3,
 ( #89766, #20336, #64434, #89291 ),
 .UNSPECIFIED., .F., .F.,
 ( 4, 4 ),
 ( 0.02882533845999755637, 0.03798746942113730152 ),
 .UNSPECIFIED. ) ;
#40898=VERTEX_POINT ( 'NONE', #68129 ) ;
#40900=CARTESIAN_POINT ( 'NONE',  ( 189.7676554596182825, 286.5697828033414112, 16.74390813620514251 ) ) ;
#40901=CARTESIAN_POINT ( 'NONE',  ( 122.6368883333363584, 251.6115022471903160, -5.000000000000047962 ) ) ;
#40902=CARTESIAN_POINT ( 'NONE',  ( 161.8811854682448939, 250.2605573099562264, 13.51112293479948789 ) ) ;
#40904=ORIENTED_EDGE ( 'NONE', *, *, #90380, .F. ) ;
#40905=CARTESIAN_POINT ( 'NONE',  ( 188.6573459026649857, 272.6511070077579575, 15.94497187152243356 ) ) ;
#40906=ORIENTED_EDGE ( 'NONE', *, *, #32915, .F. ) ;
#40907=CARTESIAN_POINT ( 'NONE',  ( 162.8042930031641049, 248.6616881586264469, 11.14389129512055554 ) ) ;
#40911=ORIENTED_EDGE ( 'NONE', *, *, #14721, .T. ) ;
#40915=CARTESIAN_POINT ( 'NONE',  ( 164.9101359252495627, 286.5608941336866451, 1.040025780022917790 ) ) ;
#40916=CARTESIAN_POINT ( 'NONE',  ( 182.8075329105516289, 285.5996758505444291, -15.91971760981349071 ) ) ;
#40923=CARTESIAN_POINT ( 'NONE',  ( 167.5026854337390034, 276.6728444866564587, 15.74913442802015950 ) ) ;
#40924=CARTESIAN_POINT ( 'NONE',  ( 75.41814989884494480, 225.8967562850346837, -4.648177544792955347E-16 ) ) ;
#40925=ORIENTED_EDGE ( 'NONE', *, *, #50313, .F. ) ;
#40926=ORIENTED_EDGE ( 'NONE', *, *, #2150, .T. ) ;
#40927=CARTESIAN_POINT ( 'NONE',  ( 198.2943784004556846, 286.7604802059595954, 16.98915255761611576 ) ) ;
#40928=CARTESIAN_POINT ( 'NONE',  ( 162.6094341192679735, 284.9563523671238272, -2.779506450940901541 ) ) ;
#40929=CARTESIAN_POINT ( 'NONE',  ( 147.9311236323648870, 274.4227731784279172, -7.799459659034405412 ) ) ;
#40930=CARTESIAN_POINT ( 'NONE',  ( 163.4222916751007801, 247.5912830598222172, -10.52132777929285012 ) ) ;
#40931=CARTESIAN_POINT ( 'NONE',  ( 155.2098048002210930, 261.8157275836062468, 16.98811268941991059 ) ) ;
#40933=DIRECTION ( 'NONE',  ( -0.8660254037844387076, -0.4999999999999998890, -0.000000000000000000 ) ) ;
#40934=CARTESIAN_POINT ( 'NONE',  ( 207.5716517802669046, 271.1223482360200023, -3.664688748148826836 ) ) ;
#40935=CARTESIAN_POINT ( 'NONE',  ( 206.4636530084236483, 270.6281364296536367, 2.534735893817217089 ) ) ;
#40937=CARTESIAN_POINT ( 'NONE',  ( 175.7824178399792174, 285.8628427244275372, -13.39878279634721103 ) ) ;
#40938=CARTESIAN_POINT ( 'NONE',  ( 86.94057726720511425, 214.8768266524160140, 9.188101187500098632 ) ) ;
#40939=ORIENTED_EDGE ( 'NONE', *, *, #17705, .T. ) ;
#40940=CARTESIAN_POINT ( 'NONE',  ( 149.8083888948594335, 271.5779462620446338, 11.70101749353969645 ) ) ;
#40943=CARTESIAN_POINT ( 'NONE',  ( 167.5469267500292574, 266.7168544022062520, -17.80679023418265672 ) ) ;
#40946=CARTESIAN_POINT ( 'NONE',  ( 78.46959274033001464, 216.1115022471902591, 10.00000000000009592 ) ) ;
#40950=CARTESIAN_POINT ( 'NONE',  ( 162.9968728533147271, 248.3281300736514652, 11.73082768548638910 ) ) ;
#40951=CARTESIAN_POINT ( 'NONE',  ( 90.89164462408909628, 223.2833772461660260, -9.188101187500095079 ) ) ;
#40953=ORIENTED_EDGE ( 'NONE', *, *, #50076, .F. ) ;
#40955=CARTESIAN_POINT ( 'NONE',  ( 161.2859416640352208, 251.2915498217379024, -13.80521263047813996 ) ) ;
#40959=CARTESIAN_POINT ( 'NONE',  ( 165.4994878024789102, 285.5423758539902792, 1.070543995922314862 ) ) ;
#40960=CARTESIAN_POINT ( 'NONE',  ( -6.563276597302431625, 157.0177522451417929, 5.000000000000051514 ) ) ;
#40962=ORIENTED_EDGE ( 'NONE', *, *, #29723, .T. ) ;
#40963=CARTESIAN_POINT ( 'NONE',  ( 204.7462429809936282, 276.0160998285135179, 13.10238900943261342 ) ) ;
#40964=CARTESIAN_POINT ( 'NONE',  ( 159.4491226731523454, 254.4730136382542582, -15.39140229921534520 ) ) ;
#40965=CARTESIAN_POINT ( 'NONE',  ( 188.8614500713004247, 269.5370965013109412, 14.80401887895223645 ) ) ;
#40966=CARTESIAN_POINT ( 'NONE',  ( 176.2504776146596157, 284.2477974488793961, 13.12230192542356910 ) ) ;
#40971=( BOUNDED_CURVE ( )  B_SPLINE_CURVE ( 2, ( #18960, #13345, #34149, #65041, #7716, #30518, #67519, #44703, #91355 ),
 .UNSPECIFIED., .F., .T. ) 
 B_SPLINE_CURVE_WITH_KNOTS ( ( 3, 2, 2, 2, 3 ),
 ( 0.3508064516129032473, 0.3521505376344086224, 0.3548387096774193727, 0.3575268817204301230, 0.3588709677419354982 ),
 .UNSPECIFIED. ) 
 CURVE ( )  GEOMETRIC_REPRESENTATION_ITEM ( )  RATIONAL_B_SPLINE_CURVE ( ( 0.9330127018922194093, 0.9330127018922194093, 1.000000000000000000, 0.8660254037844387076, 1.000000000000000000, 0.8660254037844387076, 1.000000000000000000, 0.9330127018922194093, 0.9330127018922194093 ) ) 
 REPRESENTATION_ITEM ( '' )  );
#40972=CARTESIAN_POINT ( 'NONE',  ( 200.3414094930810165, 283.6454952284590263, 16.87912319229835489 ) ) ;
#40974=CARTESIAN_POINT ( 'NONE',  ( 171.4444819528139021, 251.6572025020039121, 7.136088224024340398 ) ) ;
#40982=CARTESIAN_POINT ( 'NONE',  ( 182.5087044554237252, 264.6871601893720936, 13.42516869467857532 ) ) ;
#40987=CARTESIAN_POINT ( 'NONE',  ( 172.2755583984224756, 275.1251726850771320, 16.76863583107396138 ) ) ;
#40988=( BOUNDED_CURVE ( )  B_SPLINE_CURVE ( 2, ( #46, #46109, #63329, #78548, #15719, #47621, #1038, #78046, #61321 ),
 .UNSPECIFIED., .F., .T. ) 
 B_SPLINE_CURVE_WITH_KNOTS ( ( 3, 2, 2, 2, 3 ),
 ( 0.8588709677419354982, 0.8602150537634408733, 0.8629032258064516236, 0.8655913978494623739, 0.8669354838709677491 ),
 .UNSPECIFIED. ) 
 CURVE ( )  GEOMETRIC_REPRESENTATION_ITEM ( )  RATIONAL_B_SPLINE_CURVE ( ( 0.9330127018922194093, 0.9330127018922194093, 1.000000000000000000, 0.8660254037844387076, 1.000000000000000000, 0.8660254037844387076, 1.000000000000000000, 0.9330127018922194093, 0.9330127018922194093 ) ) 
 REPRESENTATION_ITEM ( '' )  );
#40991=CARTESIAN_POINT ( 'NONE',  ( 188.4939758497592379, 260.3566504396036976, 3.747743627288043555 ) ) ;
#40993=CARTESIAN_POINT ( 'NONE',  ( 1.609577830863368586, 180.9244531367911577, -4.594050593750046652 ) ) ;
#40995=CARTESIAN_POINT ( 'NONE',  ( 123.3201800421238090, 253.5530062829863311, -4.648177544792955347E-16 ) ) ;
#40996=ORIENTED_EDGE ( 'NONE', *, *, #76851, .F. ) ;
#40997=B_SPLINE_CURVE_WITH_KNOTS ( 'NONE', 3,
 ( #53839, #16360, #78174, #62955, #94398, #24459, #55341, #86317, #78677, #16853, #47741, #9268, #32564, #58343, #94895, #72078, #64969, #26472, #10270, #79707, #96903, #11287, #96398, #57348 ),
 .UNSPECIFIED., .F., .F.,
 ( 4, 2, 2, 2, 2, 2, 2, 2, 2, 2, 2, 4 ),
 ( 0.0002136614537458351754, 0.0007436913151772940860, 0.001008706245893013905, 0.001074959978571868834, 0.001108086844911295972, 0.001141213711250723328, 0.001207467443929577822, 0.001273721176608432317, 0.001538736107323809095, 0.001803751038039185439, 0.002068765968754562434, 0.002333780899469938778 ),
 .UNSPECIFIED. ) ;
#40999=CARTESIAN_POINT ( 'NONE',  ( 175.0114272764108136, 255.3094567315552581, 8.250059182469716035 ) ) ;
#41002=CARTESIAN_POINT ( 'NONE',  ( 33.57141466322406131, 196.3149278399160949, -9.188101187500095079 ) ) ;
#41003=CARTESIAN_POINT ( 'NONE',  ( 161.4844649541891499, 250.9476973967054789, 12.93553496455142415 ) ) ;
#41006=CARTESIAN_POINT ( 'NONE',  ( 181.6818972446956195, 294.4829896772180859, 6.439555545740881293 ) ) ;
#41008=CARTESIAN_POINT ( 'NONE',  ( 196.9152821016313339, 289.5797219436533396, 17.82432002680865679 ) ) ;
#41012=EDGE_CURVE ( 'NONE', #86855, #37817, #12779, .T. ) ;
#41014=CARTESIAN_POINT ( 'NONE',  ( 186.8244161705717374, 295.8837896403537684, -7.711110150879106229 ) ) ;
#41015=DIRECTION ( 'NONE',  ( -0.8660254037844387076, -0.4999999999999998890, -0.000000000000000000 ) ) ;
#41017=CARTESIAN_POINT ( 'NONE',  ( 88.86189758574327868, 222.1115022471902591, 10.00000000000009592 ) ) ;
#41019=CARTESIAN_POINT ( 'NONE',  ( 203.3519541875798495, 270.1197850214451819, 6.287554717287071604 ) ) ;
#41020=CARTESIAN_POINT ( 'NONE',  ( 47.69862761034023180, 198.3458772461660544, 9.188101187500095079 ) ) ;
#41021=CARTESIAN_POINT ( 'NONE',  ( 197.9598023461055902, 287.7705598106892921, 18.23120408239484291 ) ) ;
#41022=EDGE_LOOP ( 'NONE', ( #15765, #49357, #10106 ) ) ;
#41024=CARTESIAN_POINT ( 'NONE',  ( 147.1249913145849177, 275.8190353104462815, 3.637773609013635223 ) ) ;
#41026=ADVANCED_FACE ( 'NONE', ( #63367 ), #68199, .F. ) ;
#41029=CARTESIAN_POINT ( 'NONE',  ( 168.0713720833696811, 281.8093708158166351, -11.21549903910966250 ) ) ;
#41033=CARTESIAN_POINT ( 'NONE',  ( 162.6476498368881494, 248.9330020812748785, 10.75824100428386743 ) ) ;
#41034=CARTESIAN_POINT ( 'NONE',  ( 149.7072529793668707, 271.3464269086063041, -11.98883662638834657 ) ) ;
#41035=CARTESIAN_POINT ( 'NONE',  ( 157.1187995864133882, 258.5092516225370218, 18.42986330599266509 ) ) ;
#41039=CARTESIAN_POINT ( 'NONE',  ( 171.7522488252528206, 252.8251119870537025, 8.533298209578807914 ) ) ;
#41040=DIRECTION ( 'NONE',  ( -0.4999999999999987788, 0.8660254037844392627, 0.000000000000000000 ) ) ;
#41043=CYLINDRICAL_SURFACE ( 'NONE', #61076, 17.82106496071139645 ) ;
#41044=CARTESIAN_POINT ( 'NONE',  ( 191.0170959869219303, 299.7956799668270946, 7.353346939903929069 ) ) ;
#41048=ORIENTED_EDGE ( 'NONE', *, *, #35890, .T. ) ;
#41049=CARTESIAN_POINT ( 'NONE',  ( 189.7066971257315231, 274.2939208849840043, -15.68303241876299658 ) ) ;
#41050=CARTESIAN_POINT ( 'NONE',  ( 151.2479124125312921, 269.2699359884643400, -14.13957473936566167 ) ) ;
#41052=CARTESIAN_POINT ( 'NONE',  ( 201.1060504099706350, 282.3210983108598384, -18.18000168485860257 ) ) ;
#41056=CARTESIAN_POINT ( 'NONE',  ( 205.3708847852691406, 274.9341884869767227, -13.70973585089674174 ) ) ;
#41057=CARTESIAN_POINT ( 'NONE',  ( 111.6762543149156386, 235.2833772461660544, -9.188101187500095079 ) ) ;
#41058=CARTESIAN_POINT ( 'NONE',  ( 148.9504735598738137, 272.6572073132907690, -11.88406006066344744 ) ) ;
#41059=CARTESIAN_POINT ( 'NONE',  ( 180.3887555915763414, 287.0315616845538216, -13.66997111987796032 ) ) ;
#41061=CARTESIAN_POINT ( 'NONE',  ( 164.3545367017254364, 245.9765873086048487, -5.942639963102972267 ) ) ;
#41062=ORIENTED_EDGE ( 'NONE', *, *, #9669, .F. ) ;
#41064=CARTESIAN_POINT ( 'NONE',  ( 159.2077906806335932, 254.8910129107889588, 16.14624949541834553 ) ) ;
#41066=CARTESIAN_POINT ( 'NONE',  ( 66.48072710279772934, 203.0643266524160140, 9.188101187500095079 ) ) ;
#41068=CARTESIAN_POINT ( 'NONE',  ( 151.3284628043366524, 268.5384091220288383, 14.49047510809488237 ) ) ;
#41069=CARTESIAN_POINT ( 'NONE',  ( 150.5461004505574181, 269.8935004687035644, 13.73913105907748111 ) ) ;
#41075=CARTESIAN_POINT ( 'NONE',  ( 177.9640863285869159, 288.6651767168248170, 10.86720228571057945 ) ) ;
#41076=CARTESIAN_POINT ( 'NONE',  ( 147.6947327179224487, 274.8322142526899370, 9.090449717876689206 ) ) ;
#41077=VERTEX_POINT ( 'NONE', #57749 ) ;
#41078=CARTESIAN_POINT ( 'NONE',  ( 105.7493929595398470, 231.8615022471902591, -10.00000000000009592 ) ) ;
#41080=B_SPLINE_CURVE_WITH_KNOTS ( 'NONE', 3,
 ( #27781, #20190, #51058, #82019 ),
 .UNSPECIFIED., .F., .F.,
 ( 4, 4 ),
 ( 0.02373679057857851910, 0.03297336722804258130 ),
 .UNSPECIFIED. ) ;
#41081=CARTESIAN_POINT ( 'NONE',  ( 191.0481356132114570, 299.7419177570458828, 9.104177228535229816 ) ) ;
#41084=CARTESIAN_POINT ( 'NONE',  ( 149.6896757981861583, 271.3768714794653647, 12.49809796062302603 ) ) ;
#41086=ADVANCED_FACE ( 'NONE', ( #89231 ), #19781, .T. ) ;
#41087=CARTESIAN_POINT ( 'NONE',  ( 164.6241018286200699, 245.5096868128744632, 3.031483545445131433 ) ) ;
#41089=CARTESIAN_POINT ( 'NONE',  ( 167.8759064645936689, 255.9993705094734651, 13.57746339537463598 ) ) ;
#41091=CARTESIAN_POINT ( 'NONE',  ( 114.4365367415960293, 243.0024278399160949, -9.188101187500093303 ) ) ;
#41095=EDGE_CURVE ( 'NONE', #33095, #7074, #25712, .T. ) ;
#41096=CARTESIAN_POINT ( 'NONE',  ( 202.7754741559590173, 279.4295715634463022, -15.65855077192107636 ) ) ;
#41097=CARTESIAN_POINT ( 'NONE',  ( 204.3951397407346064, 276.6242284793436852, 14.79595971842109137 ) ) ;
#41102=CARTESIAN_POINT ( 'NONE',  ( 155.5521066005403554, 273.5621557416596943, -12.84016899138273260 ) ) ;
#41105=CARTESIAN_POINT ( 'NONE',  ( 165.0817809681736037, 244.7169632896033136, -1.727194264083430131 ) ) ;
#41106=CARTESIAN_POINT ( 'NONE',  ( 140.8778087205959650, 242.9548013555409796, -4.594050593750042211 ) ) ;
#41107=EDGE_CURVE ( 'NONE', #52411, #90599, #36440, .T. ) ;
#41108=CARTESIAN_POINT ( 'NONE',  ( 101.3989120123781191, 240.8967562850346837, -4.648177544792955347E-16 ) ) ;
#41109=CARTESIAN_POINT ( 'NONE',  ( 188.0009137200860039, 298.2175614353434412, 4.729959318426725012 ) ) ;
#41110=CARTESIAN_POINT ( 'NONE',  ( -22.42236680055709641, 157.8615022471902591, 0.000000000000000000 ) ) ;
#41111=CARTESIAN_POINT ( 'NONE',  ( 59.55217677675723564, 211.3149278399160949, -9.188101187500095079 ) ) ;
#41112=CARTESIAN_POINT ( 'NONE',  ( 207.6007741873543750, 271.0719067473055475, 7.587922723682903658 ) ) ;
#41113=CARTESIAN_POINT ( 'NONE',  ( 155.9742855435482909, 281.1012582971416123, 3.224975351481907282 ) ) ;
#41114=EDGE_CURVE ( 'NONE', #75611, #13298, #40013, .T. ) ;
#41119=CARTESIAN_POINT ( 'NONE',  ( 169.6667690310781893, 285.3286781044860163, -7.966101626908379529 ) ) ;
#41120=CARTESIAN_POINT ( 'NONE',  ( 203.5629025532486196, 278.0657055720176913, -15.85226727704602823 ) ) ;
#41121=CARTESIAN_POINT ( 'NONE',  ( 193.0622221429366050, 289.4054684591471300, 16.71589558189321778 ) ) ;
#41122=CARTESIAN_POINT ( 'NONE',  ( 130.1965684169902033, 232.6427522451417644, 1.119607411625061291E-15 ) ) ;
#41125=CARTESIAN_POINT ( 'NONE',  ( 147.6140518775699491, 274.9719575673779559, 8.457032797753797126 ) ) ;
#41126=CARTESIAN_POINT ( 'NONE',  ( 166.8965953329662568, 259.4083194189263963, 16.50658842888446642 ) ) ;
#41127=CARTESIAN_POINT ( 'NONE',  ( 38.76791418169571557, 187.0643266524159856, -9.188101187500093303 ) ) ;
#41129=CARTESIAN_POINT ( 'NONE',  ( 192.9064638172013417, 270.9369261147751331, 14.92505667092759758 ) ) ;
#41131=CARTESIAN_POINT ( 'NONE',  ( 147.3984236761635884, 275.3454365677582700, 5.108566646342994844 ) ) ;
#41135=CARTESIAN_POINT ( 'NONE',  ( 68.78093353194373094, 200.5177522451417929, 5.000000000000051514 ) ) ;
#41136=CARTESIAN_POINT ( 'NONE',  ( 174.4928008983406471, 289.3651385215947585, 7.878677603660426243 ) ) ;
#41137=CARTESIAN_POINT ( 'NONE',  ( 180.8112268592145426, 256.2796902623131245, 1.435307982165026752 ) ) ;
#41138=CARTESIAN_POINT ( 'NONE',  ( 157.7733463334721478, 257.3755434007023268, -16.94489513499352995 ) ) ;
#41140=AXIS2_PLACEMENT_3D ( 'NONE', #25724, #58099, #66208 ) ;
#41142=CARTESIAN_POINT ( 'NONE',  ( 39.49844957003031709, 183.6115022471902023, -5.000000000000041744 ) ) ;
#41143=CARTESIAN_POINT ( 'NONE',  ( 184.8810468967335225, 294.4243617658604535, 9.952176429897862775 ) ) ;
#41144=CARTESIAN_POINT ( 'NONE',  ( 162.8042930031641049, 248.6616881586264469, 11.14389129512055554 ) ) ;
#41145=CARTESIAN_POINT ( 'NONE',  ( 11.59636713795893925, 171.3768266524160140, 9.188101187500098632 ) ) ;
#41147=CARTESIAN_POINT ( 'NONE',  ( 164.3310316338254609, 252.4241088064557061, 13.56221488630103345 ) ) ;
#41148=CARTESIAN_POINT ( 'NONE',  ( 170.8728180971433801, 262.9177787688888088, 16.18685465067498797 ) ) ;
#41149=CARTESIAN_POINT ( 'NONE',  ( 27.64472685218285264, 186.7677522451418497, 10.00000000000009592 ) ) ;
#41151=CARTESIAN_POINT ( 'NONE',  ( 164.9617201910520237, 244.9249146555742414, 2.745022583679548767 ) ) ;
#41153=CARTESIAN_POINT ( 'NONE',  ( 183.2116848952928194, 257.8133941036112446, -2.270876890648756863 ) ) ;
#41156=CARTESIAN_POINT ( 'NONE',  ( 65.02584505343169496, 219.8967562850346837, -4.648177544792955347E-16 ) ) ;
#41159=CARTESIAN_POINT ( 'NONE',  ( 165.7072790779917284, 285.4338682230774111, 0.4788325442398248533 ) ) ;
#41161=CARTESIAN_POINT ( 'NONE',  ( 76.32488315910845245, 203.3262482093458061, 3.021315404115420679E-15 ) ) ;
#41163=CARTESIAN_POINT ( 'NONE',  ( 153.8401448635538600, 275.1610109593079869, 10.49742240986545028 ) ) ;
#41164=CARTESIAN_POINT ( 'NONE',  ( 159.9531724557437826, 253.5999738052623229, -15.71074128491364874 ) ) ;
#41165=CARTESIAN_POINT ( 'NONE',  ( 62.88113547221017541, 197.1115022471902023, -5.000000000000041744 ) ) ;
#41166=ORIENTED_EDGE ( 'NONE', *, *, #98793, .F. ) ;
#41167=CARTESIAN_POINT ( 'NONE',  ( 192.0523540417460993, 298.0025604169266558, 12.03387399082417275 ) ) ;
#41168=CARTESIAN_POINT ( 'NONE',  ( 206.9676408587583296, 272.1685258403992975, 7.544050792475608169 ) ) ;
#41171=CARTESIAN_POINT ( 'NONE',  ( 154.8838596469624349, 262.3802811495310152, 18.07457254681616021 ) ) ;
#41172=ORIENTED_EDGE ( 'NONE', *, *, #52337, .T. ) ;
#41173=ORIENTED_EDGE ( 'NONE', *, *, #61638, .F. ) ;
#41174=CARTESIAN_POINT ( 'NONE',  ( 159.4726537399769200, 278.3283626346205892, -9.792651960952584389 ) ) ;
#41175=B_SPLINE_CURVE_WITH_KNOTS ( 'NONE', 3,
 ( #12753, #3650, #4125, #34053 ),
 .UNSPECIFIED., .F., .F.,
 ( 4, 4 ),
 ( 0.01409801504582384665, 0.02276995735195360901 ),
 .UNSPECIFIED. ) ;
#41177=ORIENTED_EDGE ( 'NONE', *, *, #546, .T. ) ;
#41179=DIRECTION ( 'NONE',  ( -0.8660254037844387076, -0.4999999999999998890, -0.000000000000000000 ) ) ;
#41184=VERTEX_POINT ( 'NONE', #35431 ) ;
#41185=CARTESIAN_POINT ( 'NONE',  ( 161.5056331467593225, 250.9110330116698435, 14.52719814064025528 ) ) ;
#41186=CARTESIAN_POINT ( 'NONE',  ( 169.4855280223256102, 276.4705657850510079, -15.92413266703292329 ) ) ;
#41189=ORIENTED_EDGE ( 'NONE', *, *, #7852, .T. ) ;
#41192=VERTEX_POINT ( 'NONE', #5043 ) ;
#41196=CARTESIAN_POINT ( 'NONE',  ( 160.9880467243960140, 270.9392944726602082, 15.98296159911883763 ) ) ;
#41199=CARTESIAN_POINT ( 'NONE',  ( 194.0720430060108015, 294.5043565153341660, 13.95655032404117435 ) ) ;
#41200=CARTESIAN_POINT ( 'NONE',  ( 177.3359723029854820, 288.7904352073793461, -9.432456604021657753 ) ) ;
#41202=CARTESIAN_POINT ( 'NONE',  ( 192.1149248854976861, 297.8941845364767005, 12.26771790733441314 ) ) ;
#41203=CARTESIAN_POINT ( 'NONE',  ( 175.4967466201937611, 291.2628096033125189, 6.560984766252938805 ) ) ;
#41205=ORIENTED_EDGE ( 'NONE', *, *, #917, .F. ) ;
#41208=CARTESIAN_POINT ( 'NONE',  ( 205.9240884482826175, 273.9760116357041966, 10.27504561427317142 ) ) ;
#41209=CARTESIAN_POINT ( 'NONE',  ( 168.1726423428391399, 255.4859975196775963, 14.21197738914692366 ) ) ;
#41210=CARTESIAN_POINT ( 'NONE',  ( 190.9468710165551784, 298.7780173384815043, -8.169303778663410398 ) ) ;
#41212=VERTEX_POINT ( 'NONE', #13151 ) ;
#41214=CARTESIAN_POINT ( 'NONE',  ( 146.7017019969479463, 276.5521939148946444, -3.698925540390689104 ) ) ;
#41215=CARTESIAN_POINT ( 'NONE',  ( 197.6616696696203803, 265.4270972886941991, 5.703842229917075457 ) ) ;
#41219=CARTESIAN_POINT ( 'NONE',  ( 161.8662906133268393, 250.2863559554455719, 14.03735902266321744 ) ) ;
#41225=CARTESIAN_POINT ( 'NONE',  ( 164.7243055739305078, 245.3361288348881999, -1.445094907380085170 ) ) ;
#41226=CARTESIAN_POINT ( 'NONE',  ( 10.75723147838630034, 177.0177522451418497, -10.00000000000009592 ) ) ;
#41227=CARTESIAN_POINT ( 'NONE',  ( 102.5290345353249961, 223.8768266524159856, 9.188101187500096856 ) ) ;
#41232=CARTESIAN_POINT ( 'NONE',  ( 170.2950668402331758, 280.6084956370413579, -13.85235648845468326 ) ) ;
#41233=CARTESIAN_POINT ( 'NONE',  ( 21.71786549680706102, 183.3458772461660544, 9.188101187500095079 ) ) ;
#41236=PRODUCT_DEFINITION_CONTEXT ( 'detailed design', #61525, 'design' ) ;
#41237=VERTEX_POINT ( 'NONE', #66825 ) ;
#41238=CARTESIAN_POINT ( 'NONE',  ( -16.26211276271276063, 167.1916292661125283, 0.000000000000000000 ) ) ;
#41241=EDGE_CURVE ( 'NONE', #21768, #24856, #60632, .T. ) ;
#41245=CARTESIAN_POINT ( 'NONE',  ( 181.9320025749308627, 285.0146321948373043, 15.19111020286634428 ) ) ;
#41247=CARTESIAN_POINT ( 'NONE',  ( 36.49425040099653472, 198.0024278399160949, -9.188101187500093303 ) ) ;
#41248=CARTESIAN_POINT ( 'NONE',  ( 87.40047971330916710, 211.2677522451417929, -5.000000000000041744 ) ) ;
#41249=EDGE_LOOP ( 'NONE', ( #48923, #12574, #30718, #1388 ) ) ;
#41251=CARTESIAN_POINT ( 'NONE',  ( 178.8406086741226204, 259.2614543872599597, -10.29665073561374733 ) ) ;
#41253=CARTESIAN_POINT ( 'NONE',  ( -0.5819415548772214342, 158.2202760586659736, -5.415160957724236172E-17 ) ) ;
#41255=CARTESIAN_POINT ( 'NONE',  ( 198.6894790592683080, 286.5067226703918095, -17.06774375037124614 ) ) ;
#41256=CARTESIAN_POINT ( 'NONE',  ( 186.7303744183177230, 282.7117158418231497, 16.18601837252264630 ) ) ;
#41257=CARTESIAN_POINT ( 'NONE',  ( 147.4824818982269790, 275.1998434563504929, -4.972419998968698351 ) ) ;
#41258=CARTESIAN_POINT ( 'NONE',  ( 172.2547787113288678, 266.8662971372079369, 17.58576446449312058 ) ) ;
#41259=FACE_OUTER_BOUND ( 'NONE', #32994, .T. ) ;
#41260=CARTESIAN_POINT ( 'NONE',  ( 191.7934382699952494, 298.4510156884799699, -8.680100145728863126 ) ) ;
#41261=CARTESIAN_POINT ( 'NONE',  ( 207.0200405408487541, 272.0777669287182334, 6.494273599193515878 ) ) ;
#41263=EDGE_CURVE ( 'NONE', #82867, #20583, #77553, .T. ) ;
#41264=CARTESIAN_POINT ( 'NONE',  ( 145.6409484414103588, 245.7048013555409511, 4.594050593750051981 ) ) ;
#41266=CARTESIAN_POINT ( 'NONE',  ( 123.6384037525706958, 236.0643266524160140, 9.188101187500095079 ) ) ;
#41270=CARTESIAN_POINT ( 'NONE',  ( 144.9899443387551798, 254.5170451491295296, 0.000000000000000000 ) ) ;
#41271=DIRECTION ( 'NONE',  ( 0.4999999999999998890, -0.8660254037844385966, 0.000000000000000000 ) ) ;
#41273=CARTESIAN_POINT ( 'NONE',  ( 151.0363639623897996, 269.0443391571128018, -14.33469264561397516 ) ) ;
#41274=ORIENTED_EDGE ( 'NONE', *, *, #75091, .F. ) ;
#41275=CARTESIAN_POINT ( 'NONE',  ( 192.9426785658947381, 263.8201562504407320, -4.863779990015462573 ) ) ;
#41276=CARTESIAN_POINT ( 'NONE',  ( 196.4808189786114951, 290.3322341467384717, -17.84817245450773271 ) ) ;
#41277=CARTESIAN_POINT ( 'NONE',  ( 182.2052959828711494, 288.8764495671124450, 13.90737013350400986 ) ) ;
#41278=CARTESIAN_POINT ( 'NONE',  ( 172.8470737319805721, 290.2464512094754241, -1.885184669499159194 ) ) ;
#41282=CARTESIAN_POINT ( 'NONE',  ( 177.1415970308396481, 279.4433984593848663, 15.53509258474510979 ) ) ;
#41286=AXIS2_PLACEMENT_3D ( 'NONE', #88372, #4196, #74628 ) ;
#41289=CARTESIAN_POINT ( 'NONE',  ( 150.5438776023515004, 278.3016033182416322, -9.804454847755098641E-05 ) ) ;
#41290=( BOUNDED_CURVE ( )  B_SPLINE_CURVE ( 2, ( #43738, #37627, #59423, #28047, #58922, #60422, #14835, #76646, #20469 ),
 .UNSPECIFIED., .F., .T. ) 
 B_SPLINE_CURVE_WITH_KNOTS ( ( 3, 2, 2, 2, 3 ),
 ( 0.7056451612903226200, 0.7069892473118279952, 0.7096774193548387455, 0.7123655913978494958, 0.7137096774193548709 ),
 .UNSPECIFIED. ) 
 CURVE ( )  GEOMETRIC_REPRESENTATION_ITEM ( )  RATIONAL_B_SPLINE_CURVE ( ( 0.9330127018922194093, 0.9330127018922194093, 1.000000000000000000, 0.8660254037844387076, 1.000000000000000000, 0.8660254037844387076, 1.000000000000000000, 0.9330127018922194093, 0.9330127018922194093 ) ) 
 REPRESENTATION_ITEM ( '' )  );
#41292=CARTESIAN_POINT ( 'NONE',  ( 164.9009427471078766, 270.4319544559331234, -17.40525121274953335 ) ) ;
#41295=CARTESIAN_POINT ( 'NONE',  ( 173.7847068915813793, 272.6461794896769675, -16.37293504331134741 ) ) ;
#41296=VERTEX_POINT ( 'NONE', #60699 ) ;
#41298=CARTESIAN_POINT ( 'NONE',  ( 194.9757425430702824, 292.9391030023704161, -15.21392314336593365 ) ) ;
#41301=CARTESIAN_POINT ( 'NONE',  ( 186.5927565586945036, 291.7418713830221009, 12.22326468075236860 ) ) ;
#41308=VERTEX_POINT ( 'NONE', #66334 ) ;
#41309=CARTESIAN_POINT ( 'NONE',  ( 175.1720010258828495, 258.8074648690770800, 12.63278887511889081 ) ) ;
#41314=ORIENTED_EDGE ( 'NONE', *, *, #23774, .T. ) ;
#41319=CARTESIAN_POINT ( 'NONE',  ( 190.3365032855578249, 300.9745011048501624, 3.518936879699320563 ) ) ;
#41321=CARTESIAN_POINT ( 'NONE',  ( 146.9370072200009645, 276.1446333132804511, -3.799807221059707363 ) ) ;
#41322=CARTESIAN_POINT ( 'NONE',  ( 201.3715986869907510, 281.8611552031986776, -17.89433714524984964 ) ) ;
#41325=CARTESIAN_POINT ( 'NONE',  ( 153.9970851639660623, 279.5717529699742840, 2.172531455066414097 ) ) ;
#41326=B_SPLINE_CURVE_WITH_KNOTS ( 'NONE', 3,
 ( #90908, #44240, #89899, #60428, #59431, #37148, #51868, #50853, #82805, #5751, #83792, #27584, #68049, #74689, #19977, #43744, #81803, #82316, #12379, #36146, #91385, #21457, #12888, #13854, #52345, #90410, #20477, #58929, #20985, #98971, #35661, #29556, #43245, #58451, #89423, #66561, #13374, #1540, #32422, #1026, #17209, #62809, #63318, #70934, #39995, #24812, #9645, #71437 ),
 .UNSPECIFIED., .F., .F.,
 ( 4, 2, 2, 2, 2, 2, 2, 2, 2, 2, 2, 2, 2, 2, 2, 2, 2, 2, 2, 2, 2, 2, 2, 4 ),
 ( 0.0005856873627484591917, 0.001016685950634623565, 0.001232185244577682116, 0.001339934891549285009, 0.001447684538520887902, 0.001663183832464095856, 0.001878683126407304027, 0.002309681714293799950, 0.003171678890066790928, 0.004033676065839783206, 0.004895673241612774618, 0.005326671829499233027, 0.005542171123442425802, 0.005649920770414057318, 0.005703795593899839249, 0.005757670417385620312, 0.005811545240871401376, 0.005865420064357183307, 0.005973169711328742831, 0.006188669005271752593, 0.006619667593157770383, 0.007050666181043788172, 0.007266165474986736351, 0.007481664768929684531 ),
 .UNSPECIFIED. ) ;
#41327=CARTESIAN_POINT ( 'NONE',  ( 133.4351425849996531, 247.8458772461660544, 9.188101187500095079 ) ) ;
#41328=VERTEX_POINT ( 'NONE', #29337 ) ;
#41330=FACE_OUTER_BOUND ( 'NONE', #29641, .T. ) ;
#41337=CARTESIAN_POINT ( 'NONE',  ( 180.3486785659322891, 255.9976438602005260, 1.309110463909484157 ) ) ;
#41340=CARTESIAN_POINT ( 'NONE',  ( 156.6370339646614411, 279.1166159043581843, 7.320210838852614366 ) ) ;
#41342=DIRECTION ( 'NONE',  ( -0.8660254037844387076, -0.4999999999999998890, -0.000000000000000000 ) ) ;
#41344=CARTESIAN_POINT ( 'NONE',  ( 172.8794231584638226, 280.7410324931668697, 13.92705740956398053 ) ) ;
#41346=CARTESIAN_POINT ( 'NONE',  ( 177.0478225817679458, 255.9438551104777275, -7.283735771377678248 ) ) ;
#41348=CARTESIAN_POINT ( 'NONE',  ( 185.0903458666867891, 273.1516923159391581, -16.67643005644730536 ) ) ;
#41349=CARTESIAN_POINT ( 'NONE',  ( 193.7862695136616651, 274.3493697269946097, 16.30071627112327803 ) ) ;
#41350=ORIENTED_EDGE ( 'NONE', *, *, #36896, .F. ) ;
#41352=CARTESIAN_POINT ( 'NONE',  ( 205.0491312206212342, 269.1753787081169662, -2.999829222793530370 ) ) ;
#41353=CARTESIAN_POINT ( 'NONE',  ( 191.5024861053093730, 298.9549596202882640, -10.70987072427270803 ) ) ;
#41354=CARTESIAN_POINT ( 'NONE',  ( 149.7128599965862463, 271.3367152699035501, 12.33532264622322394 ) ) ;
#41355=CARTESIAN_POINT ( 'NONE',  ( 163.1014434023538513, 248.1470085697407058, 9.692260209037655727 ) ) ;
#41356=CARTESIAN_POINT ( 'NONE',  ( 160.4962995477943650, 275.9333967852908813, 14.18032076246626794 ) ) ;
#41357=CARTESIAN_POINT ( 'NONE',  ( 151.4940044683453095, 274.9262206533563813, -9.273972269532857027 ) ) ;
#41358=CARTESIAN_POINT ( 'NONE',  ( 200.1754978754242984, 267.3235950566412953, 6.315888745726680575 ) ) ;
#41362=CARTESIAN_POINT ( 'NONE',  ( 193.4852642841095189, 276.0130112962725093, -16.67970642947549464 ) ) ;
#41363=ADVANCED_FACE ( 'NONE', ( #52611 ), #59718, .T. ) ;
#41366=CARTESIAN_POINT ( 'NONE',  ( 152.9262073036446168, 265.7710344717137900, 16.19159804214501008 ) ) ;
#41370=CARTESIAN_POINT ( 'NONE',  ( -7.294332625736643649, 178.8464784336661637, 1.353441290958777525E-15 ) ) ;
#41372=CARTESIAN_POINT ( 'NONE',  ( 93.32716752435031538, 230.8149278399160949, -9.188101187500095079 ) ) ;
#41373=CARTESIAN_POINT ( 'NONE',  ( 203.5080190724872011, 278.1607665491929993, -15.47044080916498743 ) ) ;
#41377=CARTESIAN_POINT ( 'NONE',  ( 180.9780804914473720, 282.7163897586885923, -16.62997927953544774 ) ) ;
#41380=CARTESIAN_POINT ( 'NONE',  ( 161.7651517240504688, 282.1360828662558902, 5.605791128093589037 ) ) ;
#41382=CARTESIAN_POINT ( 'NONE',  ( 207.6555576926778883, 270.9770189326688410, -1.235081510489080436 ) ) ;
#41383=CARTESIAN_POINT ( 'NONE',  ( 177.8726909305742652, 289.9607890038341793, 9.707458997688759084 ) ) ;
#41384=CARTESIAN_POINT ( 'NONE',  ( 158.3585752585947262, 263.3710999200782226, 17.79390465796247156 ) ) ;
#41386=CARTESIAN_POINT ( 'NONE',  ( 147.1562325744354496, 245.7677522451417929, -5.000000000000041744 ) ) ;
#41387=CARTESIAN_POINT ( 'NONE',  ( 82.20432729060244981, 228.2677522451419350, -5.000000000000047962 ) ) ;
#41389=EDGE_CURVE ( 'NONE', #83009, #86318, #43613, .T. ) ;
#41391=CARTESIAN_POINT ( 'NONE',  ( 63.96340690334295687, 216.9244531367911293, -4.594050593750046652 ) ) ;
#41392=CARTESIAN_POINT ( 'NONE',  ( 161.1061647010182583, 251.6029326557136585, -13.56144933775657613 ) ) ;
#41396=CARTESIAN_POINT ( 'NONE',  ( 199.8780930708521453, 284.4479828117403031, 17.00188320299317368 ) ) ;
#41397=CARTESIAN_POINT ( 'NONE',  ( 11.60290295393121696, 189.0530062829863027, -4.648177544792955347E-16 ) ) ;
#41403=CARTESIAN_POINT ( 'NONE',  ( 81.12205585946965414, 208.4548013555409796, -4.594050593750042211 ) ) ;
#41404=CARTESIAN_POINT ( 'NONE',  ( 94.05805000844991071, 225.1115022471902307, 10.00000000000009592 ) ) ;
#41406=CARTESIAN_POINT ( 'NONE',  ( 147.0314375879888757, 275.9810751181479986, -5.168577011192616588 ) ) ;
#41410=CARTESIAN_POINT ( 'NONE',  ( 189.7553949637821802, 286.5528735061270140, 16.71718042389977654 ) ) ;
#41412=CARTESIAN_POINT ( 'NONE',  ( 133.5343746642906524, 241.2365022471902307, 10.00000000000009592 ) ) ;
#41413=CARTESIAN_POINT ( 'NONE',  ( 13.06432082636536762, 189.8967562850346837, -4.648177544792955347E-16 ) ) ;
#41416=CARTESIAN_POINT ( 'NONE',  ( 185.7548115650120906, 271.5664750103190954, 16.84803787444293022 ) ) ;
#41418=CARTESIAN_POINT ( 'NONE',  ( 162.6937333994314656, 248.8531830095558632, 10.02305144031113926 ) ) ;
#41420=CARTESIAN_POINT ( 'NONE',  ( 201.1755594471486859, 282.2007051268825535, -18.15567516623250910 ) ) ;
#41421=ORIENTED_EDGE ( 'NONE', *, *, #88809, .F. ) ;
#41424=CARTESIAN_POINT ( 'NONE',  ( 192.3546171244506411, 291.9418057657312602, 14.85604634385901690 ) ) ;
#41425=CARTESIAN_POINT ( 'NONE',  ( 167.3984581500753848, 247.5600430218893280, 3.593632883392327670 ) ) ;
#41427=EDGE_CURVE ( 'NONE', #8285, #8043, #96264, .T. ) ;
#41434=CARTESIAN_POINT ( 'NONE',  ( 167.7832046799460954, 276.7730461828406874, 15.64290657898813031 ) ) ;
#41439=CARTESIAN_POINT ( 'NONE',  ( 186.2875372408365990, 298.3389836698145814, 1.055114130040206710 ) ) ;
#41440=CARTESIAN_POINT ( 'NONE',  ( 163.7064929935861244, 247.0990319366274548, 6.401263337036986023 ) ) ;
#41441=CARTESIAN_POINT ( 'NONE',  ( 148.0826818691893152, 274.1602666119424043, -9.371267383421741926 ) ) ;
#41443=CARTESIAN_POINT ( 'NONE',  ( 155.6435836392643637, 261.0644005951349982, 17.58841156286628049 ) ) ;
#41446=CARTESIAN_POINT ( 'NONE',  ( 207.4225649187019087, 271.3805742549917568, -3.927239063805231023 ) ) ;
#41447=CARTESIAN_POINT ( 'NONE',  ( 166.1957201800340442, 265.4536997604227508, 16.55608710447817344 ) ) ;
#41449=CARTESIAN_POINT ( 'NONE',  ( 92.62404252742298638, 212.0327760586659451, 1.948934522072303157E-15 ) ) ;
#41452=CARTESIAN_POINT ( 'NONE',  ( 166.8158164543628459, 278.2249326526564914, -13.34744090285348683 ) ) ;
#41454=ORIENTED_EDGE ( 'NONE', *, *, #7583, .T. ) ;
#41456=CARTESIAN_POINT ( 'NONE',  ( 164.1828359708729863, 281.6525977458860552, 8.811343294891619493 ) ) ;
#41457=CARTESIAN_POINT ( 'NONE',  ( 146.5046981847821428, 276.8934145268504494, 0.02269072295920678689 ) ) ;
#41459=CARTESIAN_POINT ( 'NONE',  ( 206.8775514429320026, 272.3245652858344670, -9.838455694836268250 ) ) ;
#41460=CARTESIAN_POINT ( 'NONE',  ( 207.9670239186021377, 270.4375436045261836, 3.151456135821919968 ) ) ;
#41461=B_SPLINE_CURVE_WITH_KNOTS ( 'NONE', 3,
 ( #54995, #54480, #47397, #79358 ),
 .UNSPECIFIED., .F., .F.,
 ( 4, 4 ),
 ( 0.01697285580833185481, 0.02587605460899505133 ),
 .UNSPECIFIED. ) ;
#41462=CARTESIAN_POINT ( 'NONE',  ( 84.74801659416949917, 228.9244531367911293, -4.594050593750046652 ) ) ;
#41464=CARTESIAN_POINT ( 'NONE',  ( 200.4606599504492408, 283.4389473774714361, -18.16209435128261873 ) ) ;
#41466=B_SPLINE_CURVE_WITH_KNOTS ( 'NONE', 3,
 ( #49028, #25215, #49514, #95169, #65217, #88585, #40894, #48531, #95680, #2954, #80469, #25738, #96159, #11039, #72850, #33844, #10032, #41916, #33319, #3442, #34319, #26722, #96658, #57604, #79468, #50020, #73333, #80974, #63722, #11539, #42399, #50503, #56617, #89093, #3920, #58112, #19642, #40402, #71843, #81457, #71339, #1931, #32817, #56100, #87091, #17628, #2441, #28712, #90566, #74344 ),
 .UNSPECIFIED., .F., .F.,
 ( 4, 2, 2, 2, 2, 2, 2, 2, 2, 2, 2, 2, 2, 2, 2, 2, 2, 2, 2, 2, 2, 2, 2, 2, 4 ),
 ( 0.0004158906835773414643, 0.001427088945389863150, 0.001932688076296212518, 0.002185487641749338846, 0.002311887424475821563, 0.002438287207202304279, 0.002564686989928787429, 0.002691086772655270579, 0.002943886338108236012, 0.003449485469014167312, 0.004460683730825979604, 0.005471881992637791028, 0.005977481123543697608, 0.006230280688996726358, 0.006483080254449755109, 0.006546280145813108790, 0.006609480037176460737, 0.006672679928539813551, 0.006735879819903165498, 0.006988679385356588031, 0.007494278516263348962, 0.007747078081716728126, 0.007999877647170108158, 0.008252677212623488190, 0.008505476778076868222 ),
 .UNSPECIFIED. ) ;
#41468=CARTESIAN_POINT ( 'NONE',  ( 192.3713340522295709, 271.8780416168410170, 15.57788208939756380 ) ) ;
#41472=AXIS2_PLACEMENT_3D ( 'NONE', #98705, #76866, #7464 ) ;
#41473=CARTESIAN_POINT ( 'NONE',  ( 156.6823612109870396, 259.2651850631482375, 17.57884712310819708 ) ) ;
#41474=CARTESIAN_POINT ( 'NONE',  ( 160.7043946034031308, 275.5602053013725481, 12.99197331405084910 ) ) ;
#41475=CARTESIAN_POINT ( 'NONE',  ( 206.6703863510205679, 272.6833857505801006, -10.72500664779635393 ) ) ;
#41476=CARTESIAN_POINT ( 'NONE',  ( 191.5959239871531850, 271.5537089687533694, 14.17158143004904325 ) ) ;
#41477=CARTESIAN_POINT ( 'NONE',  ( 174.7055293015415600, 283.6856165666803236, 13.49174788089805865 ) ) ;
#41484=CARTESIAN_POINT ( 'NONE',  ( 149.0570874715264154, 274.4997098312325079, 9.090637939377691268 ) ) ;
#41485=B_SPLINE_CURVE_WITH_KNOTS ( 'NONE', 3,
 ( #12010, #68177, #91031, #4909 ),
 .UNSPECIFIED., .F., .F.,
 ( 4, 4 ),
 ( 0.01048086686357619333, 0.01574798419196724725 ),
 .UNSPECIFIED. ) ;
#41486=CARTESIAN_POINT ( 'NONE',  ( 178.3666971430922672, 291.5231582936299333, 9.051735255157939974 ) ) ;
#41488=CARTESIAN_POINT ( 'NONE',  ( 167.6848733776141671, 249.9537906194314303, 6.968395254000899541 ) ) ;
#41493=ORIENTED_EDGE ( 'NONE', *, *, #100184, .F. ) ;
#41494=CYLINDRICAL_SURFACE ( 'NONE', #35263, 17.82106496071139645 ) ;
#41498=CARTESIAN_POINT ( 'NONE',  ( 180.4957999564819886, 267.2278171865779086, -15.18777883605170409 ) ) ;
#41503=CARTESIAN_POINT ( 'NONE',  ( 203.1526193585190470, 278.7763369107815379, -16.67658907091021447 ) ) ;
#41506=CARTESIAN_POINT ( 'NONE',  ( 205.8387202508380653, 272.3240174465572636, -9.430873374051206071 ) ) ;
#41507=CARTESIAN_POINT ( 'NONE',  ( 161.1232569692349443, 251.5733279787459367, -14.02750397520710557 ) ) ;
#41508=CARTESIAN_POINT ( 'NONE',  ( 10.18907585680922878, 170.5643266524159571, -9.188101187500093303 ) ) ;
#41512=CARTESIAN_POINT ( 'NONE',  ( 181.4283053378885597, 267.7238133557910373, 16.48022347432943135 ) ) ;
#41514=CARTESIAN_POINT ( 'NONE',  ( 30.97333845187074175, 194.8149278399160664, -9.188101187500095079 ) ) ;
#41515=FACE_OUTER_BOUND ( 'NONE', #75342, .T. ) ;
#41516=CARTESIAN_POINT ( 'NONE',  ( 146.8358616138309571, 276.3198226421291679, 4.054088818585255716 ) ) ;
#41518=CARTESIAN_POINT ( 'NONE',  ( 178.1014170928845033, 292.3538449268187378, 5.578751321692007714 ) ) ;
#41520=CARTESIAN_POINT ( 'NONE',  ( 177.4918489660068417, 292.2262405376345669, 2.581417131937560061 ) ) ;
#41521=CARTESIAN_POINT ( 'NONE',  ( 149.3412472373495063, 271.9803674496423014, 11.49645634555178297 ) ) ;
#41522=CARTESIAN_POINT ( 'NONE',  ( 179.3634369656868728, 278.6207563196031174, -17.18449886317435826 ) ) ;
#41523=CARTESIAN_POINT ( 'NONE',  ( 173.2412943989675398, 277.7050541934257240, 16.79641741871846250 ) ) ;
#41524=CARTESIAN_POINT ( 'NONE',  ( 167.0813381624552392, 257.8573864978880579, -15.59453214358795137 ) ) ;
#41526=CARTESIAN_POINT ( 'NONE',  ( 182.6015398117219490, 296.6291243770974120, 1.816064570435409253 ) ) ;
#41527=CARTESIAN_POINT ( 'NONE',  ( 84.17092664857760553, 212.7365022471902023, 10.00000000000009592 ) ) ;
#41528=CARTESIAN_POINT ( 'NONE',  ( 177.8222571804544430, 286.5223583772871621, 13.77940225188420875 ) ) ;
#41529=CARTESIAN_POINT ( 'NONE',  ( 178.2087173759056498, 281.9494420025493469, 16.33014707258442755 ) ) ;
#41530=CARTESIAN_POINT ( 'NONE',  ( 56.25097556847656932, 191.0327760586659451, 1.948934522072303157E-15 ) ) ;
#41531=CARTESIAN_POINT ( 'NONE',  ( 197.9002057575219453, 287.8737841300738296, 18.01270164875645818 ) ) ;
#41532=ORIENTED_EDGE ( 'NONE', *, *, #59842, .F. ) ;
#41534=CARTESIAN_POINT ( 'NONE',  ( 151.0426280674448378, 269.0334894088936153, -15.84467774422408581 ) ) ;
#41536=VERTEX_POINT ( 'NONE', #57109 ) ;
#41537=CARTESIAN_POINT ( 'NONE',  ( 171.1309707950161680, 286.4780903314298826, 7.470031319074768028 ) ) ;
#41538=CARTESIAN_POINT ( 'NONE',  ( 164.6649740431187183, 245.4388940607451843, -1.430729255012818557 ) ) ;
#41539=CARTESIAN_POINT ( 'NONE',  ( 193.3266656173557294, 295.7953880232976758, 13.75377347669239825 ) ) ;
#41540=CARTESIAN_POINT ( 'NONE',  ( 95.19470834736912934, 215.7677522451417929, -5.000000000000041744 ) ) ;
#41542=CARTESIAN_POINT ( 'NONE',  ( 202.8787628851569593, 279.2506702366259788, 17.01435431865322556 ) ) ;
#41548=CARTESIAN_POINT ( 'NONE',  ( 171.7111136159620344, 252.7683153775072071, 8.549686029849182134 ) ) ;
#41550=ORIENTED_EDGE ( 'NONE', *, *, #86564, .T. ) ;
#41557=ORIENTED_EDGE ( 'NONE', *, *, #12926, .F. ) ;
#41558=CARTESIAN_POINT ( 'NONE',  ( 207.3646600298985447, 271.4808684644054324, -5.284084612275558257 ) ) ;
#41559=CARTESIAN_POINT ( 'NONE',  ( 151.0156108440694425, 269.4662454610033251, -13.81341911168381564 ) ) ;
#41561=CARTESIAN_POINT ( 'NONE',  ( 153.1627746953036535, 265.3612877299463548, -17.72069958822647351 ) ) ;
#41565=EDGE_CURVE ( 'NONE', #19653, #92570, #72739, .T. ) ;
#41566=CARTESIAN_POINT ( 'NONE',  ( 157.6036818288543486, 257.6694109429415107, -16.73826488331764395 ) ) ;
#41567=CARTESIAN_POINT ( 'NONE',  ( 111.8384605302426991, 241.5024278399160949, -9.188101187500093303 ) ) ;
#41568=CARTESIAN_POINT ( 'NONE',  ( 149.2223635749290622, 272.1862799931444670, -12.97307652490353647 ) ) ;
#41569=CARTESIAN_POINT ( 'NONE',  ( 184.1784204912316909, 288.8332414524454634, -13.14701115336322346 ) ) ;
#41573=CARTESIAN_POINT ( 'NONE',  ( 201.4453672590843212, 280.6253616217601916, 16.44210273926617560 ) ) ;
#41576=CARTESIAN_POINT ( 'NONE',  ( 159.3528137482544196, 254.6398255893999476, 16.73628156321660398 ) ) ;
#41578=CARTESIAN_POINT ( 'NONE',  ( 57.11665387649598813, 203.7833772461660828, -9.188101187500095079 ) ) ;
#41580=CARTESIAN_POINT ( 'NONE',  ( 191.0816511748900268, 299.6838671013740623, 7.311127128005925790 ) ) ;
#41581=CARTESIAN_POINT ( 'NONE',  ( 151.0254882145115971, 269.0631765050081299, 14.78274390654921078 ) ) ;
#41586=CARTESIAN_POINT ( 'NONE',  ( 147.6140518775699491, 274.9719575673779559, 8.457032797753797126 ) ) ;
#41587=ORIENTED_EDGE ( 'NONE', *, *, #63578, .T. ) ;
#41588=CARTESIAN_POINT ( 'NONE',  ( 171.6932237194176025, 259.4651268520354961, -13.84549871016380607 ) ) ;
#41590=CARTESIAN_POINT ( 'NONE',  ( 160.4864031019297954, 258.1637219028588675, -17.19673236967974006 ) ) ;
#41592=CARTESIAN_POINT ( 'NONE',  ( 148.9232972370683399, 272.7042780851529642, 12.27045554427055940 ) ) ;
#41593=CARTESIAN_POINT ( 'NONE',  ( 177.0733235261513983, 269.7023525544009885, 16.22382760421824699 ) ) ;
#41594=CARTESIAN_POINT ( 'NONE',  ( 205.7668501412109663, 274.2483563724483133, 11.09689540819876896 ) ) ;
#41596=CARTESIAN_POINT ( 'NONE',  ( 153.9188684017919968, 264.4466852765838212, -16.50884978456451790 ) ) ;
#41597=CARTESIAN_POINT ( 'NONE',  ( 208.1415148974628266, 270.1353163636768500, 3.453641150550738725 ) ) ;
#41598=CARTESIAN_POINT ( 'NONE',  ( 123.7191597644692393, 251.4244531367911293, -4.594050593750046652 ) ) ;
#41599=ORIENTED_EDGE ( 'NONE', *, *, #85845, .T. ) ;
#41602=EDGE_CURVE ( 'NONE', #29582, #45874, #82453, .T. ) ;
#41603=CARTESIAN_POINT ( 'NONE',  ( 205.7160570675956137, 273.8316721655138508, -10.27501494681582805 ) ) ;
#41604=CARTESIAN_POINT ( 'NONE',  ( 164.4990934228277411, 245.7262077230798809, 6.470820838822735510 ) ) ;
#41606=CARTESIAN_POINT ( 'NONE',  ( 177.9260618338437041, 255.3518848370148078, 4.867121141759041869 ) ) ;
#41610=CARTESIAN_POINT ( 'NONE',  ( 185.8136036613169324, 262.0491945824166464, 9.850964508789044061 ) ) ;
#41611=CARTESIAN_POINT ( 'NONE',  ( 164.2877295051262934, 246.0923007674255416, -1.726861278304287373 ) ) ;
#41612=CARTESIAN_POINT ( 'NONE',  ( 137.4944631173567018, 256.3149278399160380, -9.188101187500095079 ) ) ;
#41613=EDGE_CURVE ( 'NONE', #43017, #49470, #90062, .T. ) ;
#41616=CARTESIAN_POINT ( 'NONE',  ( 63.63864737692379236, 216.7369531367911293, -4.594050593750048428 ) ) ;
#41617=AXIS2_PLACEMENT_3D ( 'NONE', #68511, #60894, #21913 ) ;
#41619=CARTESIAN_POINT ( 'NONE',  ( 170.6781199183338344, 250.4769293299289927, 3.472362579247760372 ) ) ;
#41622=CARTESIAN_POINT ( 'NONE',  ( 190.8187029736043883, 300.1393067457597681, 3.941064102378585954 ) ) ;
#41623=CARTESIAN_POINT ( 'NONE',  ( 154.8332767207531901, 280.7459370637686220, -0.9958211956073632631 ) ) ;
#41624=CARTESIAN_POINT ( 'NONE',  ( 170.2435210885388983, 285.6843656190501406, -7.971347355553285219 ) ) ;
#41625=CARTESIAN_POINT ( 'NONE',  ( 198.0006249058153003, 287.6998530631771587, 18.31850453277666801 ) ) ;
#41628=CARTESIAN_POINT ( 'NONE',  ( 117.3505249275209366, 251.8927522451419634, 2.944929066748280225E-16 ) ) ;
#41631=CARTESIAN_POINT ( 'NONE',  ( 190.3144310910409445, 301.0127312671879167, -1.334877248546042949 ) ) ;
#41632=CARTESIAN_POINT ( 'NONE',  ( -6.102853504003020291, 155.0327760586659167, 1.948934522072302763E-15 ) ) ;
#41633=CARTESIAN_POINT ( 'NONE',  ( 31.67681054456310008, 201.3464784336661353, 1.353441290958777327E-15 ) ) ;
#41634=CARTESIAN_POINT ( 'NONE',  ( 27.07746054717988571, 174.8932355074535678, -2.679491924311248496 ) ) ;
#41637=AXIS2_PLACEMENT_3D ( 'NONE', #49709, #11729, #96354 ) ;
#41640=CARTESIAN_POINT ( 'NONE',  ( 147.0538900202505488, 275.9421863647172017, 5.192507380313251986 ) ) ;
#41642=CARTESIAN_POINT ( 'NONE',  ( 198.0913710030449408, 277.7585867100321479, -16.26773035892281882 ) ) ;
#41643=CARTESIAN_POINT ( 'NONE',  ( 58.82164138842269097, 194.7677522451418213, -5.000000000000041744 ) ) ;
#41644=CARTESIAN_POINT ( 'NONE',  ( 163.1128098473768375, 255.9724106907921168, -14.93599513872953821 ) ) ;
#41645=CARTESIAN_POINT ( 'NONE',  ( -2.640161845538968599, 180.8297689869269504, -2.679491924311240503 ) ) ;
#41647=B_SPLINE_CURVE_WITH_KNOTS ( 'NONE', 3,
 ( #58469, #89442, #19997, #50877 ),
 .UNSPECIFIED., .F., .F.,
 ( 4, 4 ),
 ( 0.01207516581926863092, 0.01741691159609244990 ),
 .UNSPECIFIED. ) ;
#41648=CARTESIAN_POINT ( 'NONE',  ( 161.9621149929554065, 267.2142435603461763, 16.48812087427357653 ) ) ;
#41649=CARTESIAN_POINT ( 'NONE',  ( 39.93146227192245590, 203.8615022471903160, 5.000000000000046185 ) ) ;
#41650=CARTESIAN_POINT ( 'NONE',  ( 41.20449994286561690, 183.0494855054052152, -2.679491924311248496 ) ) ;
#41652=CARTESIAN_POINT ( 'NONE',  ( 163.4004183463084416, 247.6291687766210146, 10.19167732382099345 ) ) ;
#41653=CARTESIAN_POINT ( 'NONE',  ( 5.858601742122021783, 180.3149278399161233, 9.188101187500093303 ) ) ;
#41655=CARTESIAN_POINT ( 'NONE',  ( 163.9254889395286341, 247.2708555043535625, 6.667454687248093315 ) ) ;
#41656=CARTESIAN_POINT ( 'NONE',  ( 192.0523540417460993, 298.0025604169266558, 12.03387399082417275 ) ) ;
#41658=CARTESIAN_POINT ( 'NONE',  ( 165.0565241268390366, 244.7607094220335568, 2.191926263411719589 ) ) ;
#41659=CARTESIAN_POINT ( 'NONE',  ( 180.1282168372663079, 277.0805460213222204, 16.30842645680661818 ) ) ;
#41666=EDGE_CURVE ( 'NONE', #41308, #70064, #61734, .T. ) ;
#41667=DIRECTION ( 'NONE',  ( -0.8660254037844387076, -0.4999999999999998890, -0.000000000000000000 ) ) ;
#41672=CARTESIAN_POINT ( 'NONE',  ( 192.6797324865049745, 296.9159090750308110, 12.42053959885222625 ) ) ;
#41673=CARTESIAN_POINT ( 'NONE',  ( 164.9779129355220562, 244.8968679994381148, -1.771286574179712803 ) ) ;
#41676=ORIENTED_EDGE ( 'NONE', *, *, #51526, .T. ) ;
#41678=CARTESIAN_POINT ( 'NONE',  ( 134.3282312844263231, 248.3615022471902591, -10.00000000000009592 ) ) ;
#41683=CARTESIAN_POINT ( 'NONE',  ( 177.2673766539031988, 263.0841653866659158, 15.51101798395150944 ) ) ;
#41684=ORIENTED_EDGE ( 'NONE', *, *, #38263, .T. ) ;
#41688=CARTESIAN_POINT ( 'NONE',  ( 196.4808189786114951, 290.3322341467384717, -17.84817245450773271 ) ) ;
#41691=ORIENTED_EDGE ( 'NONE', *, *, #41819, .F. ) ;
#41692=CARTESIAN_POINT ( 'NONE',  ( 200.6449165581618956, 283.1198055712825976, 18.35107460171532523 ) ) ;
#41693=CARTESIAN_POINT ( 'NONE',  ( 166.1079261098780080, 274.0347854768993443, -15.23724750118056193 ) ) ;
#41694=AXIS2_PLACEMENT_3D ( 'NONE', #86328, #70564, #32056 ) ;
#41696=ORIENTED_EDGE ( 'NONE', *, *, #99048, .F. ) ;
#41697=CARTESIAN_POINT ( 'NONE',  ( 170.6619951277876623, 255.5210136367033726, -11.54849001391199970 ) ) ;
#41698=CARTESIAN_POINT ( 'NONE',  ( 202.8787628851569593, 279.2506702366259788, 17.01435431865322556 ) ) ;
#41699=EDGE_CURVE ( 'NONE', #89234, #70505, #26773, .T. ) ;
#41701=EDGE_CURVE ( 'NONE', #21534, #30468, #90877, .T. ) ;
#41703=CARTESIAN_POINT ( 'NONE',  ( 157.0136551185426868, 266.0997186349934509, -17.02801493162102986 ) ) ;
#41704=B_SPLINE_CURVE_WITH_KNOTS ( 'NONE', 3,
 ( #11196, #42066, #65368, #5074 ),
 .UNSPECIFIED., .F., .F.,
 ( 4, 4 ),
 ( 0.008546822710145150076, 0.01492985447388818325 ),
 .UNSPECIFIED. ) ;
#41708=CARTESIAN_POINT ( 'NONE',  ( 147.8435824263222855, 274.5743989950495347, 6.098816573078369885 ) ) ;
#41709=CARTESIAN_POINT ( 'NONE',  ( 180.5039422260482240, 291.5977753851293528, -9.856995586095885997 ) ) ;
#41710=CARTESIAN_POINT ( 'NONE',  ( 188.2520712372829621, 265.6420100395978920, -13.17850047611677766 ) ) ;
#41712=CARTESIAN_POINT ( 'NONE',  ( 158.3623000859935246, 256.3554455780269450, -16.52320444293775381 ) ) ;
#41713=ORIENTED_EDGE ( 'NONE', *, *, #87410, .F. ) ;
#41714=CARTESIAN_POINT ( 'NONE',  ( 100.9602528039918923, 217.5494855054051868, -2.679491924311248496 ) ) ;
#41716=CARTESIAN_POINT ( 'NONE',  ( 196.7823306783968746, 289.8100005636337073, -17.85370042640856170 ) ) ;
#41717=CARTESIAN_POINT ( 'NONE',  ( 190.4646797940841623, 298.9332177302380842, -8.185516204028834508 ) ) ;
#41720=AXIS2_PLACEMENT_3D ( 'NONE', #13563, #37824, #84481 ) ;
#41722=CARTESIAN_POINT ( 'NONE',  ( 187.6504252453685240, 277.1264514418339786, 17.28725775733853709 ) ) ;
#41723=EDGE_CURVE ( 'NONE', #66637, #85448, #44868, .T. ) ;
#41724=CARTESIAN_POINT ( 'NONE',  ( 171.5016553172604574, 259.7020436333838802, -14.14659924787457435 ) ) ;
#41725=CYLINDRICAL_SURFACE ( 'NONE', #44718, 17.82106496071139645 ) ;
#41727=CARTESIAN_POINT ( 'NONE',  ( 161.8948331661419218, 250.2369188037922356, 13.64419044796309777 ) ) ;
#41728=CARTESIAN_POINT ( 'NONE',  ( 148.4341346725819051, 273.5515325000037024, -10.40428456760419884 ) ) ;
#41732=DIRECTION ( 'NONE',  ( -0.8660254037844387076, -0.4999999999999998890, -0.000000000000000000 ) ) ;
#41733=CARTESIAN_POINT ( 'NONE',  ( 42.77981749017101976, 207.0530062829863311, -4.648177544792955347E-16 ) ) ;
#41734=CARTESIAN_POINT ( 'NONE',  ( 164.5416088356626290, 245.6525688679454618, -1.463507744092769292 ) ) ;
#41735=CARTESIAN_POINT ( 'NONE',  ( 27.64472685218290238, 176.7677522451417929, -5.000000000000041744 ) ) ;
#41736=CARTESIAN_POINT ( 'NONE',  ( 98.90203251333015544, 240.1589784336661637, -6.496448406907676862E-16 ) ) ;
#41737=CARTESIAN_POINT ( 'NONE',  ( 180.7892034029179626, 294.0795370620815561, -2.813581583843308032 ) ) ;
#41741=CARTESIAN_POINT ( 'NONE',  ( 13.16551753867071461, 190.6589784336661921, -6.496448406907675876E-16 ) ) ;
#41744=ORIENTED_EDGE ( 'NONE', *, *, #80771, .T. ) ;
#41745=ORIENTED_EDGE ( 'NONE', *, *, #13280, .F. ) ;
#41747=CARTESIAN_POINT ( 'NONE',  ( 186.7200758071169275, 260.8107248425581020, -5.831653652513626440 ) ) ;
#41748=CARTESIAN_POINT ( 'NONE',  ( 181.8404918915032340, 261.1361780761246223, 12.51250699268308786 ) ) ;
#41750=CARTESIAN_POINT ( 'NONE',  ( 193.0206257540501156, 263.7076866269070479, -4.037792959707156015 ) ) ;
#41751=CARTESIAN_POINT ( 'NONE',  ( 161.1150691641480535, 251.5875096731584506, -13.48836942566120101 ) ) ;
#41752=CARTESIAN_POINT ( 'NONE',  ( 182.0419006976227934, 284.8263522540155464, 14.99106680293229843 ) ) ;
#41754=CARTESIAN_POINT ( 'NONE',  ( 45.69611741197122257, 191.0643266524160140, 9.188101187500095079 ) ) ;
#41755=CARTESIAN_POINT ( 'NONE',  ( 87.90566119885008334, 214.8927522451418213, 10.00000000000009592 ) ) ;
#41757=ORIENTED_EDGE ( 'NONE', *, *, #5261, .T. ) ;
#41759=CARTESIAN_POINT ( 'NONE',  ( 158.3433012654136292, 282.4888899867655141, -1.676262827589547921 ) ) ;
#41761=CARTESIAN_POINT ( 'NONE',  ( 8.267668766103758671, 166.3923013555410080, 4.594050593750050204 ) ) ;
#41764=CARTESIAN_POINT ( 'NONE',  ( 198.5970767652345899, 286.6667681383942181, -17.17073100918929640 ) ) ;
#41766=CARTESIAN_POINT ( 'NONE',  ( 147.5540328368684300, 275.0759135952944234, -4.750028533202499403 ) ) ;
#41768=CARTESIAN_POINT ( 'NONE',  ( 163.7729086741176161, 246.9839966035275438, 6.099406794390714204 ) ) ;
#41769=CARTESIAN_POINT ( 'NONE',  ( 191.2211340522693774, 299.4422756709672626, -8.405362570633277741 ) ) ;
#41770=CARTESIAN_POINT ( 'NONE',  ( 206.9878665138179770, 272.1334939782196329, 6.566295309274049252 ) ) ;
#41773=CARTESIAN_POINT ( 'NONE',  ( -3.441976700948170542, 175.4865022471903160, -10.00000000000009415 ) ) ;
#41775=CARTESIAN_POINT ( 'NONE',  ( 125.6141109788952122, 234.1423013555409796, -4.594050593750043987 ) ) ;
#41778=CARTESIAN_POINT ( 'NONE',  ( 150.9724347302981187, 269.6954501832723849, 13.74844370660301784 ) ) ;
#41779=VECTOR ( 'NONE', #35998, 1000.000000000000000 ) ;
#41780=CARTESIAN_POINT ( 'NONE',  ( 196.0034224882197975, 291.1591091234520263, 17.53794140922627776 ) ) ;
#41783=ORIENTED_EDGE ( 'NONE', *, *, #44414, .T. ) ;
#41784=CARTESIAN_POINT ( 'NONE',  ( 189.8675696937700650, 261.6596842279012662, -4.438983720181640891 ) ) ;
#41785=CARTESIAN_POINT ( 'NONE',  ( 196.2379679265050925, 290.7528645076583871, -16.93678934971137906 ) ) ;
#41786=CARTESIAN_POINT ( 'NONE',  ( 190.4937053644069920, 299.9959326328678912, 4.274138836246343942 ) ) ;
#41787=CARTESIAN_POINT ( 'NONE',  ( 176.1878198624884249, 292.0021934572283158, -1.093827943886815923 ) ) ;
#41791=CARTESIAN_POINT ( 'NONE',  ( -22.42236680055709641, 157.8615022471902591, 0.000000000000000000 ) ) ;
#41792=CARTESIAN_POINT ( 'NONE',  ( 168.8502749405928398, 271.8395537308506960, -16.79921431673894361 ) ) ;
#41796=CARTESIAN_POINT ( 'NONE',  ( 176.9361943346061992, 287.9860272245114174, 12.19037568368620938 ) ) ;
#41799=CARTESIAN_POINT ( 'NONE',  ( 167.5505310038667517, 261.6318463984700315, 17.07012949051403439 ) ) ;
#41801=CARTESIAN_POINT ( 'NONE',  ( 192.3683084660635529, 288.2966816650776423, -15.88566354911130674 ) ) ;
#41802=VERTEX_POINT ( 'NONE', #88471 ) ;
#41803=CARTESIAN_POINT ( 'NONE',  ( 164.8075539017095252, 280.4672370525465226, 12.63796469268613265 ) ) ;
#41804=CARTESIAN_POINT ( 'NONE',  ( 194.9455394410084921, 292.9914163096879065, -15.01116663483170655 ) ) ;
#41805=CARTESIAN_POINT ( 'NONE',  ( 165.0319151415814645, 246.0072716476385608, -1.061671501984392751 ) ) ;
#41807=EDGE_CURVE ( 'NONE', #6621, #14175, #17067, .T. ) ;
#41813=FACE_OUTER_BOUND ( 'NONE', #80499, .T. ) ;
#41814=CARTESIAN_POINT ( 'NONE',  ( 203.3740894404336927, 278.3927394765486838, -15.19753795879846869 ) ) ;
#41818=CARTESIAN_POINT ( 'NONE',  ( 106.0403798229140477, 220.4824982072973683, 3.021315404115420679E-15 ) ) ;
#41819=EDGE_CURVE ( 'NONE', #62607, #72102, #79922, .T. ) ;
#41820=ORIENTED_EDGE ( 'NONE', *, *, #40464, .T. ) ;
#41824=CARTESIAN_POINT ( 'NONE',  ( 154.9903553346911735, 262.1958252075976361, -18.39016733948542637 ) ) ;
#41825=ORIENTED_EDGE ( 'NONE', *, *, #93643, .T. ) ;
#41826=CARTESIAN_POINT ( 'NONE',  ( 183.3723276922390539, 280.6706895461819045, -16.13205748088399005 ) ) ;
#41828=CARTESIAN_POINT ( 'NONE',  ( 160.9268025830670865, 254.5507503617475038, -15.18711876478708511 ) ) ;
#41829=CARTESIAN_POINT ( 'NONE',  ( 161.9036870859828809, 277.5393705136012272, -13.14925469141188508 ) ) ;
#41830=CARTESIAN_POINT ( 'NONE',  ( 192.5076277540105423, 297.2140032159341558, -13.10094381206144298 ) ) ;
#41832=CARTESIAN_POINT ( 'NONE',  ( 200.8665851640556070, 282.7358642834317948, -16.69422397739980823 ) ) ;
#41835=CARTESIAN_POINT ( 'NONE',  ( 155.1556490571049949, 279.7438825265072069, 2.118603912366986197 ) ) ;
#41836=CARTESIAN_POINT ( 'NONE',  ( 130.0789470495699618, 258.1589784336661637, -6.496448406907675876E-16 ) ) ;
#41843=EDGE_LOOP ( 'NONE', ( #97452, #7961, #59113, #50723, #5365 ) ) ;
#41844=CARTESIAN_POINT ( 'NONE',  ( 202.3894997978090373, 280.0980987621804275, 16.95659012541789323 ) ) ;
#41846=CARTESIAN_POINT ( 'NONE',  ( 190.0601721553029222, 300.2863949309033842, 3.228815124723532382 ) ) ;
#41848=CARTESIAN_POINT ( 'NONE',  ( 152.9273493951901628, 265.7690563111299298, -17.70273273795505631 ) ) ;
#41850=CARTESIAN_POINT ( 'NONE',  ( 192.8911265895718827, 292.5243652962839747, -14.36741178004102970 ) ) ;
#41854=ORIENTED_EDGE ( 'NONE', *, *, #9669, .T. ) ;
#41855=CARTESIAN_POINT ( 'NONE',  ( 194.1852025340051284, 294.3083584634874796, -15.46421316575964688 ) ) ;
#41856=EDGE_CURVE ( 'NONE', #31200, #64025, #14736, .T. ) ;
#41860=ADVANCED_FACE ( 'NONE', ( #16995 ), #97051, .T. ) ;
#41862=EDGE_CURVE ( 'NONE', #65003, #74614, #12240, .T. ) ;
#41863=CARTESIAN_POINT ( 'NONE',  ( 201.2353357416039614, 267.9535537611733957, -2.850234977744889431 ) ) ;
#41864=CARTESIAN_POINT ( 'NONE',  ( 192.0275136246134196, 298.0455852814817490, -9.520297513543107826 ) ) ;
#41866=CARTESIAN_POINT ( 'NONE',  ( 202.2576150004249200, 280.3265299319959354, 16.24828394350762295 ) ) ;
#41871=VERTEX_POINT ( 'NONE', #44285 ) ;
#41873=CARTESIAN_POINT ( 'NONE',  ( 11.62325688217078223, 167.5177522451418213, 5.000000000000051514 ) ) ;
#41874=EDGE_CURVE ( 'NONE', #96323, #54644, #83327, .T. ) ;
#41878=CARTESIAN_POINT ( 'NONE',  ( 192.2185419806677942, 297.7147144631093170, 12.45868041609393728 ) ) ;
#41881=CARTESIAN_POINT ( 'NONE',  ( 202.5245888501533216, 279.8641176599742266, 15.60152447840272494 ) ) ;
#41882=CARTESIAN_POINT ( 'NONE',  ( 3.856091543753019213, 173.0333772461660828, 9.188101187500095079 ) ) ;
#41883=CARTESIAN_POINT ( 'NONE',  ( 97.84665082640911749, 236.4869531367911293, 4.594050593750046652 ) ) ;
#41884=CARTESIAN_POINT ( 'NONE',  ( 192.4663556654298588, 297.2854885702906245, -12.98646995774174684 ) ) ;
#41885=CARTESIAN_POINT ( 'NONE',  ( 181.9272638006293619, 257.0174299096278219, -2.314174031938120102 ) ) ;
#41888=CARTESIAN_POINT ( 'NONE',  ( 163.5826848823411410, 283.4162327659261678, 5.679725392094765013 ) ) ;
#41890=CARTESIAN_POINT ( 'NONE',  ( 207.9528294584847288, 270.4621291306354465, 5.874671256616545101 ) ) ;
#41892=CARTESIAN_POINT ( 'NONE',  ( 184.5847840940699598, 267.9585090317841036, 15.85480517954647084 ) ) ;
#41896=EDGE_CURVE ( 'NONE', #3452, #77804, #13775, .T. ) ;
#41897=CARTESIAN_POINT ( 'NONE',  ( 75.30318735596920021, 214.2833772461660544, -9.188101187500095079 ) ) ;
#41898=CARTESIAN_POINT ( 'NONE',  ( 207.5785076975260779, 271.1104734389944042, -6.824813054587777650 ) ) ;
#41900=VECTOR ( 'NONE', #33560, 1000.000000000000000 ) ;
#41908=CARTESIAN_POINT ( 'NONE',  ( 173.3300473466945277, 268.3110915217967545, -16.29280547201360818 ) ) ;
#41911=DIRECTION ( 'NONE',  ( -0.8660254037844387076, -0.4999999999999998890, -0.000000000000000000 ) ) ;
#41914=CARTESIAN_POINT ( 'NONE',  ( 68.21243081460160340, 216.3149278399160664, 9.188101187500093303 ) ) ;
#41915=CARTESIAN_POINT ( 'NONE',  ( 198.7134558283731280, 282.8386145195935910, 17.66748989068429054 ) ) ;
#41916=CARTESIAN_POINT ( 'NONE',  ( 169.9373325680253117, 288.2255053123109860, -1.082792927354846446 ) ) ;
#41917=CARTESIAN_POINT ( 'NONE',  ( 192.7705129102570822, 296.7586727687594816, -13.39629674907774692 ) ) ;
#41918=CARTESIAN_POINT ( 'NONE',  ( 199.3579472636792786, 281.3827632249817725, 17.38534755126016407 ) ) ;
#41920=CARTESIAN_POINT ( 'NONE',  ( 189.7468387718738541, 286.5256409918453073, 16.65683580306518863 ) ) ;
#41923=CARTESIAN_POINT ( 'NONE',  ( 118.7397740163064128, 239.3615022471902307, -10.00000000000009592 ) ) ;
#41924=CARTESIAN_POINT ( 'NONE',  ( 205.3704330671644414, 274.9349708856848338, -13.01557521325596944 ) ) ;
#41927=CARTESIAN_POINT ( 'NONE',  ( 165.9969153545198708, 246.1123342570000716, -1.176638740111072723 ) ) ;
#41928=VERTEX_POINT ( 'NONE', #45283 ) ;
#41929=CARTESIAN_POINT ( 'NONE',  ( 162.8789161433191452, 248.5324370884573568, 9.731756914259689140 ) ) ;
#41932=ORIENTED_EDGE ( 'NONE', *, *, #44688, .T. ) ;
#41934=ORIENTED_EDGE ( 'NONE', *, *, #36509, .F. ) ;
#41935=EDGE_CURVE ( 'NONE', #98181, #76921, #73273, .T. ) ;
#41936=CARTESIAN_POINT ( 'NONE',  ( 159.9635946688021022, 268.7707599091479551, -17.14635356962945778 ) ) ;
#41937=FACE_OUTER_BOUND ( 'NONE', #64883, .T. ) ;
#41938=CARTESIAN_POINT ( 'NONE',  ( 194.1483379205519100, 280.7941404440221049, -17.33680858677280767 ) ) ;
#41950=CARTESIAN_POINT ( 'NONE',  ( 198.8081898473356262, 282.3983615885804284, -17.60554210735202574 ) ) ;
#41951=CARTESIAN_POINT ( 'NONE',  ( 204.3276935076901850, 276.7410487817560920, 13.46217427333259309 ) ) ;
#41952=CARTESIAN_POINT ( 'NONE',  ( 194.8432095198904221, 293.1686569321988145, -14.74101036184996616 ) ) ;
#41954=DIRECTION ( 'NONE',  ( -0.8660254037844387076, -0.4999999999999998890, -0.000000000000000000 ) ) ;
#41955=CARTESIAN_POINT ( 'NONE',  ( 129.4748805805031395, 238.8927522451418781, 10.00000000000009948 ) ) ;
#41956=CARTESIAN_POINT ( 'NONE',  ( 187.6335173687660927, 291.4025380883284697, -13.88432507550760953 ) ) ;
#41957=CARTESIAN_POINT ( 'NONE',  ( 207.6895561066261280, 270.9181319523335674, -5.172192454743582246 ) ) ;
#41958=CARTESIAN_POINT ( 'NONE',  ( 166.8954640849737530, 265.8187516957161165, 16.54619064527818395 ) ) ;
#41960=CARTESIAN_POINT ( 'NONE',  ( 104.8563042601131770, 231.3458772461660544, 9.188101187500095079 ) ) ;
#41964=CARTESIAN_POINT ( 'NONE',  ( 163.1341141637884959, 276.8030541846430310, -14.24718853740416868 ) ) ;
#41965=VERTEX_POINT ( 'NONE', #69083 ) ;
#41970=CARTESIAN_POINT ( 'NONE',  ( 206.8106726053982811, 272.4404028303941914, -10.47827087991598560 ) ) ;
#41971=CARTESIAN_POINT ( 'NONE',  ( 94.51795245455393513, 231.5024278399160949, 9.188101187500095079 ) ) ;
#41974=EDGE_CURVE ( 'NONE', #23996, #14901, #25511, .T. ) ;
#41975=CARTESIAN_POINT ( 'NONE',  ( 208.1612901671020381, 270.1010645919285480, -2.401583477149568768 ) ) ;
#41976=ORIENTED_EDGE ( 'NONE', *, *, #50591, .T. ) ;
#41979=CARTESIAN_POINT ( 'NONE',  ( 94.62531631345288474, 236.9860189848785410, -2.679491924311252493 ) ) ;
#41980=CARTESIAN_POINT ( 'NONE',  ( 165.5677502601071183, 285.3540468067780580, 0.5650785607410294675 ) ) ;
#41981=CARTESIAN_POINT ( 'NONE',  ( 134.8963869060034142, 254.8149278399161233, -9.188101187500095079 ) ) ;
#41982=CARTESIAN_POINT ( 'NONE',  ( 198.8170977036201066, 284.5390304616801700, 17.67078396476120261 ) ) ;
#41987=CARTESIAN_POINT ( 'NONE',  ( 204.3341445623842674, 276.7298752272635625, 14.23430099947301031 ) ) ;
#41988=CARTESIAN_POINT ( 'NONE',  ( 160.7782940569628920, 275.4437765362630444, 13.33882116160937237 ) ) ;
#41990=CARTESIAN_POINT ( 'NONE',  ( 192.2804853811905730, 271.9156663614426179, 14.15980414719692604 ) ) ;
#41993=CARTESIAN_POINT ( 'NONE',  ( 198.8081898473356262, 282.3983615885804284, -17.60554210735202574 ) ) ;
#41996=CARTESIAN_POINT ( 'NONE',  ( 153.4689407916852701, 266.8309924954582470, 16.62268559038933091 ) ) ;
#41998=CARTESIAN_POINT ( 'NONE',  ( 206.7893622945242385, 272.4773133715531230, -10.52881283832460291 ) ) ;
#42000=CARTESIAN_POINT ( 'NONE',  ( 118.0101279445459284, 227.3932355074535394, -2.679491924311248496 ) ) ;
#42002=CARTESIAN_POINT ( 'NONE',  ( 188.5410240070633563, 293.7196559869043426, 13.01390607220156248 ) ) ;
#42003=EDGE_CURVE ( 'NONE', #21873, #33698, #84752, .T. ) ;
#42005=CARTESIAN_POINT ( 'NONE',  ( 164.3524132573224392, 245.9802652221976587, -2.749586949851067441 ) ) ;
#42006=CARTESIAN_POINT ( 'NONE',  ( 180.4743659044432036, 267.2657980451650133, -15.36156412806984406 ) ) ;
#42011=CYLINDRICAL_SURFACE ( 'NONE', #63795, 10.00000000000010658 ) ;
#42013=CARTESIAN_POINT ( 'NONE',  ( 160.9546831504796387, 273.1595514402344520, -15.05126160413894176 ) ) ;
#42015=CARTESIAN_POINT ( 'NONE',  ( 25.39882055865593458, 173.2202760586659736, -5.415160957724236172E-17 ) ) ;
#42019=CARTESIAN_POINT ( 'NONE',  ( 37.35373998880870516, 180.8262482093457493, 3.021315404115420679E-15 ) ) ;
#42020=CARTESIAN_POINT ( 'NONE',  ( 164.0179800784044915, 246.5595204798204065, -5.772998092557310557 ) ) ;
#42022=CARTESIAN_POINT ( 'NONE',  ( 34.70824655357364463, 190.8458772461660544, 9.188101187500095079 ) ) ;
#42023=CARTESIAN_POINT ( 'NONE',  ( 161.8662906133268393, 250.2863559554455719, 14.03735902266321744 ) ) ;
#42024=CARTESIAN_POINT ( 'NONE',  ( 190.3791419447713906, 300.9006487807255326, -5.688668718458480988 ) ) ;
#42026=CARTESIAN_POINT ( 'NONE',  ( 178.8069409143749340, 291.7769763296440715, 6.074930007927774156 ) ) ;
#42027=CARTESIAN_POINT ( 'NONE',  ( 146.5157004908022031, 276.8743579738231233, -0.1877253132609108255 ) ) ;
#42028=CARTESIAN_POINT ( 'NONE',  ( 179.1308850641379138, 278.3362884085181008, -16.57857069867015554 ) ) ;
#42030=CARTESIAN_POINT ( 'NONE',  ( 165.7783219637343848, 257.4631878547201609, -15.00105737115166527 ) ) ;
#42033=CARTESIAN_POINT ( 'NONE',  ( 73.27344031762333998, 223.1115022471903160, -5.000000000000047962 ) ) ;
#42036=CARTESIAN_POINT ( 'NONE',  ( 52.11020483269097525, 191.7048013555409796, 4.594050593750051981 ) ) ;
#42039=CARTESIAN_POINT ( 'NONE',  ( 150.6626254231123880, 269.6916732958875969, -15.32062296289003811 ) ) ;
#42040=VECTOR ( 'NONE', #55636, 1000.000000000000000 ) ;
#42042=ORIENTED_EDGE ( 'NONE', *, *, #98548, .T. ) ;
#42043=CARTESIAN_POINT ( 'NONE',  ( 167.6793603611326944, 285.0233743312336969, 7.699659890578392840 ) ) ;
#42044=CARTESIAN_POINT ( 'NONE',  ( 207.4764081617721843, 271.2873150223495600, 6.359972247200924578 ) ) ;
#42045=CARTESIAN_POINT ( 'NONE',  ( -17.42236680055705023, 149.2012482093457777, 0.000000000000000000 ) ) ;
#42049=CARTESIAN_POINT ( 'NONE',  ( 171.3238289833617500, 255.7752812501198889, 11.47896718753802858 ) ) ;
#42056=DIRECTION ( 'NONE',  ( -0.8660254037844387076, -0.4999999999999998890, -0.000000000000000000 ) ) ;
#42057=CARTESIAN_POINT ( 'NONE',  ( 177.9144328244200040, 254.9604715414552345, -7.067334745369662663 ) ) ;
#42059=ADVANCED_FACE ( 'NONE', ( #85331 ), #100008, .T. ) ;
#42060=ORIENTED_EDGE ( 'NONE', *, *, #153, .T. ) ;
#42063=CARTESIAN_POINT ( 'NONE',  ( 207.8232941427535536, 270.6864908788566026, -6.505149060073906142 ) ) ;
#42065=B_SPLINE_CURVE_WITH_KNOTS ( 'NONE', 3,
 ( #10010, #8997, #23186, #93634, #62681, #70806, #69296, #30805, #25191, #31290, #40378, #55082, #401, #54571, #55575, #54079, #8503, #70288, #69791, #100220, #56073, #77410, #24201, #85032, #87067, #61685, #86068, #8015, #16594, #17599, #92637, #79445, #63699, #1909, #32294, #32790, #47490, #38888, #86558, #39373, #900, #15578 ),
 .UNSPECIFIED., .F., .F.,
 ( 4, 2, 2, 2, 2, 2, 2, 2, 2, 2, 2, 2, 2, 2, 2, 2, 2, 2, 2, 2, 4 ),
 ( 0.0009151626340143699393, 0.001011832196295166806, 0.001108501758575963780, 0.001205171320856760755, 0.001301840883137557730, 0.001495180007699081857, 0.001688519132260605984, 0.002461875630506861218, 0.004008588626999308804, 0.004781945125245484242, 0.005168623374368607956, 0.005361962498930214482, 0.005458632061211052440, 0.005555301623491891265, 0.005603636404632282055, 0.005651971185772672844, 0.005748640748053380697, 0.005941979872614794669, 0.006328658121737632154, 0.006715336370860470507, 0.007102014619983307124 ),
 .UNSPECIFIED. ) ;
#42066=CARTESIAN_POINT ( 'NONE',  ( 186.2990562447640741, 264.8370073322022336, -13.43280071233020934 ) ) ;
#42067=ORIENTED_EDGE ( 'NONE', *, *, #60928, .F. ) ;
#42069=EDGE_CURVE ( 'NONE', #40669, #13902, #39583, .T. ) ;
#42073=CARTESIAN_POINT ( 'NONE',  ( 205.3704330671644414, 274.9349708856848338, -13.01557521325596944 ) ) ;
#42075=CARTESIAN_POINT ( 'NONE',  ( 109.6190968851625769, 246.3464784336661353, 1.353441290958777525E-15 ) ) ;
#42076=B_SPLINE_CURVE_WITH_KNOTS ( 'NONE', 3,
 ( #14538, #38309, #69217, #100145 ),
 .UNSPECIFIED., .F., .F.,
 ( 4, 4 ),
 ( 0.002091524323244029187, 0.007431800589236895946 ),
 .UNSPECIFIED. ) ;
#42077=CARTESIAN_POINT ( 'NONE',  ( 164.4915767550571957, 245.7392269735623529, -6.407198159945809657 ) ) ;
#42080=CARTESIAN_POINT ( 'NONE',  ( 198.3523905153085423, 287.0905771551796306, 18.52598547438866206 ) ) ;
#42081=CARTESIAN_POINT ( 'NONE',  ( 204.7753828612366931, 275.5785558422823556, -12.39807726186342052 ) ) ;
#42082=CARTESIAN_POINT ( 'NONE',  ( 69.59257202794182717, 220.1744531367911293, 4.594050593750047540 ) ) ;
#42084=CARTESIAN_POINT ( 'NONE',  ( 191.0170959869219303, 299.7956799668270946, 7.353346939903929069 ) ) ;
#42085=CARTESIAN_POINT ( 'NONE',  ( 198.7255181831150423, 286.4443010768291629, 17.42756903872921725 ) ) ;
#42086=CARTESIAN_POINT ( 'NONE',  ( 175.6569888586722072, 278.3733240093107497, 15.53892781902675857 ) ) ;
#42087=VERTEX_POINT ( 'NONE', #8787 ) ;
#42092=CARTESIAN_POINT ( 'NONE',  ( 191.4738032422262677, 260.7793432447242594, -0.2951778641931921410 ) ) ;
#42094=CARTESIAN_POINT ( 'NONE',  ( 160.9608998348622890, 258.6124335639508445, -16.62975727638092494 ) ) ;
#42095=CARTESIAN_POINT ( 'NONE',  ( 206.5803147552910275, 270.4199738506200674, 1.964338299035684576 ) ) ;
#42096=CARTESIAN_POINT ( 'NONE',  ( 149.1856130393175306, 272.2499337880290682, 11.44243872309708188 ) ) ;
#42097=CARTESIAN_POINT ( 'NONE',  ( 176.9380622633689768, 269.9288259353154444, 16.55129804831395646 ) ) ;
#42098=CARTESIAN_POINT ( 'NONE',  ( 165.0020474182383339, 244.8550658491588479, 1.825383354618924425 ) ) ;
#42099=CARTESIAN_POINT ( 'NONE',  ( -22.42236680055709641, 157.8615022471902591, 0.000000000000000000 ) ) ;
#42100=CARTESIAN_POINT ( 'NONE',  ( 164.8383744266741928, 254.7166954803307704, 14.02974467908927814 ) ) ;
#42101=CARTESIAN_POINT ( 'NONE',  ( 164.4405316900629259, 245.8276396196081350, -6.144538123479245328 ) ) ;
#42102=CARTESIAN_POINT ( 'NONE',  ( 115.9249311304092771, 246.9244531367911293, -4.594050593750046652 ) ) ;
#42103=ORIENTED_EDGE ( 'NONE', *, *, #41935, .F. ) ;
#42106=CARTESIAN_POINT ( 'NONE',  ( 203.2369479875374623, 278.6302754407888074, -16.66242713208754367 ) ) ;
#42107=CARTESIAN_POINT ( 'NONE',  ( 163.9942050550062049, 246.6007000282974673, 5.791111691696777974 ) ) ;
#42109=CARTESIAN_POINT ( 'NONE',  ( 177.8766753057446408, 255.3238193400180194, 4.872644976819591633 ) ) ;
#42110=EDGE_LOOP ( 'NONE', ( #71596, #74362, #85756, #66750, #90845, #29725, #13055, #50868, #58399, #57989, #13915, #77697, #70188, #18926, #28848, #58992, #65234, #23343, #29013, #25073 ) ) ;
#42113=CARTESIAN_POINT ( 'NONE',  ( 147.6620395981771878, 275.3265400130114244, 3.458083620816670312 ) ) ;
#42115=CARTESIAN_POINT ( 'NONE',  ( 164.7349053118283564, 245.3177695503021027, -2.492200678360605437 ) ) ;
#42116=CARTESIAN_POINT ( 'NONE',  ( 139.7681268980558968, 245.3768266524160140, -9.188101187500093303 ) ) ;
#42118=CARTESIAN_POINT ( 'NONE',  ( 146.8729474948188454, 276.2555880120147549, 3.934020695290606273 ) ) ;
#42120=EDGE_CURVE ( 'NONE', #68198, #67601, #86928, .T. ) ;
#42121=CARTESIAN_POINT ( 'NONE',  ( 171.3262007583307138, 250.8544493858235285, 3.410168526935229760 ) ) ;
#42124=CARTESIAN_POINT ( 'NONE',  ( 149.2511585606875428, 272.1364056148075292, 11.40684181024752242 ) ) ;
#42125=CARTESIAN_POINT ( 'NONE',  ( 154.9848759717382336, 280.4844015978009111, -0.8777400808273079225 ) ) ;
#42126=CARTESIAN_POINT ( 'NONE',  ( 171.4620503856968412, 287.6916138556427995, -8.596052341455351353 ) ) ;
#42127=CARTESIAN_POINT ( 'NONE',  ( 160.7872435741957133, 280.1341495971591939, 10.66000836593391199 ) ) ;
#42128=CARTESIAN_POINT ( 'NONE',  ( 157.4866207245044052, 271.0942435755181350, -14.66448764132394089 ) ) ;
#42129=CARTESIAN_POINT ( 'NONE',  ( 132.8668134119921547, 247.5177522451418497, -10.00000000000009592 ) ) ;
#42133=CARTESIAN_POINT ( 'NONE',  ( 196.2609093297512857, 290.7131288316392670, 16.03897268885959448 ) ) ;
#42134=CARTESIAN_POINT ( 'NONE',  ( 148.4016473149517594, 273.6078022540229426, 8.470066617688926769 ) ) ;
#42135=CARTESIAN_POINT ( 'NONE',  ( -4.262896616726100874, 168.3458772461660544, 9.188101187500095079 ) ) ;
#42136=CARTESIAN_POINT ( 'NONE',  ( 43.58535403812915376, 183.7202760586659736, -5.415160957724236172E-17 ) ) ;
#42137=CARTESIAN_POINT ( 'NONE',  ( 178.5646908849556951, 273.7108284848578705, -17.39287981145522721 ) ) ;
#42139=DIRECTION ( 'NONE',  ( -0.8660254037844387076, -0.4999999999999998890, -0.000000000000000000 ) ) ;
#42141=CARTESIAN_POINT ( 'NONE',  ( 190.7569505155522904, 300.2462651405980978, -5.670926626284815697 ) ) ;
#42143=CARTESIAN_POINT ( 'NONE',  ( 166.5497620933320775, 284.9599651698292178, -8.643830016708903941 ) ) ;
#42144=CARTESIAN_POINT ( 'NONE',  ( 64.01779381112933720, 197.7677522451418213, -5.000000000000041744 ) ) ;
#42145=CARTESIAN_POINT ( 'NONE',  ( 181.0761428174893126, 255.7875309544736524, 2.145717405531494926 ) ) ;
#42146=CARTESIAN_POINT ( 'NONE',  ( 157.3661765229227285, 258.0807821998820373, -18.27254492731150748 ) ) ;
#42147=CARTESIAN_POINT ( 'NONE',  ( 167.4564344753456453, 270.0695307704535821, -17.68371939062425824 ) ) ;
#42148=CARTESIAN_POINT ( 'NONE',  ( 161.6411385815104609, 267.5259986109867327, 16.53943407798323761 ) ) ;
#42149=CARTESIAN_POINT ( 'NONE',  ( 52.48883062679690426, 191.1115022471902023, -5.000000000000041744 ) ) ;
#42150=CARTESIAN_POINT ( 'NONE',  ( 181.6034186054171187, 291.9446207410121019, 9.020533753185340231 ) ) ;
#42152=CARTESIAN_POINT ( 'NONE',  ( 5.344833028331274605, 164.7048013555410080, 4.594050593750051981 ) ) ;
#42154=B_SPLINE_CURVE_WITH_KNOTS ( 'NONE', 3,
 ( #24122, #76349, #85991, #16518 ),
 .UNSPECIFIED., .F., .F.,
 ( 4, 4 ),
 ( 0.007172802622825931278, 0.01294203102117486362 ),
 .UNSPECIFIED. ) ;
#42155=CARTESIAN_POINT ( 'NONE',  ( 165.0735250206753619, 246.7312630101393722, 5.989302113854410692 ) ) ;
#42156=CARTESIAN_POINT ( 'NONE',  ( 152.6757560589063303, 266.2048287524194166, 16.73757896668104195 ) ) ;
#42158=CARTESIAN_POINT ( 'NONE',  ( 206.5117639185820906, 272.9581278627833285, 11.28485531511759099 ) ) ;
#42159=CARTESIAN_POINT ( 'NONE',  ( 182.5090719219444395, 278.4899130783974215, 16.60092655590875310 ) ) ;
#42161=CARTESIAN_POINT ( 'NONE',  ( 196.2293283710122012, 290.7678286567270902, -17.07152402978540096 ) ) ;
#42162=CARTESIAN_POINT ( 'NONE',  ( 176.5849886759608864, 260.5643506436040866, -13.27287686889044593 ) ) ;
#42165=CARTESIAN_POINT ( 'NONE',  ( 165.5685896552094221, 285.4467981318400120, 0.1671104821641794524 ) ) ;
#42167=CARTESIAN_POINT ( 'NONE',  ( 159.1502228898632154, 259.4266978733254518, 16.68670530085068648 ) ) ;
#42168=CARTESIAN_POINT ( 'NONE',  ( 152.9700320981889092, 277.5340873795012726, -5.209865602531399631 ) ) ;
#42169=CARTESIAN_POINT ( 'NONE',  ( 156.8724508569020202, 276.4746155548443198, 10.35837630302414425 ) ) ;
#42170=B_SPLINE_CURVE_WITH_KNOTS ( 'NONE', 3,
 ( #5312, #35202, #97054, #75217 ),
 .UNSPECIFIED., .F., .F.,
 ( 4, 4 ),
 ( 0.009368188378409090036, 0.01456212696257992191 ),
 .UNSPECIFIED. ) ;
#42171=CARTESIAN_POINT ( 'NONE',  ( 159.7132918459648181, 254.0154592091499239, -16.90058287995827158 ) ) ;
#42172=EDGE_CURVE ( 'NONE', #70733, #68153, #43177, .T. ) ;
#42175=CARTESIAN_POINT ( 'NONE',  ( 206.8968397926183229, 272.2911568841838061, 7.145103750817420440 ) ) ;
#42176=CARTESIAN_POINT ( 'NONE',  ( 203.1399666651039695, 272.9695736541691531, -12.09293310806949684 ) ) ;
#42178=ORIENTED_EDGE ( 'NONE', *, *, #11686, .F. ) ;
#42180=ORIENTED_EDGE ( 'NONE', *, *, #88176, .T. ) ;
#42181=CARTESIAN_POINT ( 'NONE',  ( 159.5098919638083146, 279.0616708731288327, -9.454383224537151520 ) ) ;
#42185=CARTESIAN_POINT ( 'NONE',  ( 174.3232990571352730, 262.5854648150144044, 14.90850430120301340 ) ) ;
#42190=CARTESIAN_POINT ( 'NONE',  ( 149.7072529793668707, 271.3464269086063041, -11.98883662638834657 ) ) ;
#42191=CARTESIAN_POINT ( 'NONE',  ( 43.23318412030279489, 185.7677522451417929, -5.000000000000041744 ) ) ;
#42193=CARTESIAN_POINT ( 'NONE',  ( 161.6673510627899191, 250.6309293646106653, 13.01175935005004192 ) ) ;
#42194=CARTESIAN_POINT ( 'NONE',  ( 166.1236709775900238, 274.1391546445065615, -15.19174922871369837 ) ) ;
#42197=CARTESIAN_POINT ( 'NONE',  ( 174.6250001500969518, 276.7190186761092150, -16.51844552091739615 ) ) ;
#42198=VERTEX_POINT ( 'NONE', #78705 ) ;
#42199=CARTESIAN_POINT ( 'NONE',  ( 156.9962301082478859, 266.1307905592512952, -17.22057167171774950 ) ) ;
#42200=ORIENTED_EDGE ( 'NONE', *, *, #42792, .F. ) ;
#42201=CARTESIAN_POINT ( 'NONE',  ( 157.5483139352812998, 268.8664552472071705, 15.62089565001041791 ) ) ;
#42203=VERTEX_POINT ( 'NONE', #79240 ) ;
#42204=CARTESIAN_POINT ( 'NONE',  ( 193.6030392054437357, 295.3166949268590997, 13.33385638216535263 ) ) ;
#42205=CARTESIAN_POINT ( 'NONE',  ( 189.5599828453989346, 263.0657735508838186, -9.804501003715218488 ) ) ;
#42207=CARTESIAN_POINT ( 'NONE',  ( 192.4380962356868281, 295.3344353383980661, 13.50754959408193656 ) ) ;
#42209=CARTESIAN_POINT ( 'NONE',  ( 158.6799548824769772, 255.8052513312497638, -17.63511970826639441 ) ) ;
#42210=EDGE_LOOP ( 'NONE', ( #90831, #20622, #68364, #24247, #28547 ) ) ;
#42211=CARTESIAN_POINT ( 'NONE',  ( 92.59663213601572807, 234.2677522451419065, -5.000000000000047962 ) ) ;
#42213=CARTESIAN_POINT ( 'NONE',  ( 205.8452707775803390, 274.1125278458945900, 11.42742867493066328 ) ) ;
#42214=CARTESIAN_POINT ( 'NONE',  ( 166.8906917922102480, 254.4375966883865487, 14.01000126778575527 ) ) ;
#42215=CARTESIAN_POINT ( 'NONE',  ( 205.9240884482826175, 273.9760116357041966, 10.27504561427317142 ) ) ;
#42216=CARTESIAN_POINT ( 'NONE',  ( 159.9671766634011192, 253.5757178060795809, 16.49140845334465411 ) ) ;
#42217=ORIENTED_EDGE ( 'NONE', *, *, #53027, .T. ) ;
#42219=CARTESIAN_POINT ( 'NONE',  ( 146.6676967921120820, 276.6110926573920779, -3.425452920967749115 ) ) ;
#42223=CARTESIAN_POINT ( 'NONE',  ( 198.8820006463426182, 286.1732655000252521, -17.07140226101661185 ) ) ;
#42224=CARTESIAN_POINT ( 'NONE',  ( 190.4787930012176105, 300.7280480879330753, -0.07093684169630354308 ) ) ;
#42228=CARTESIAN_POINT ( 'NONE',  ( 51.48077938449444702, 188.9824982072973967, 3.021315404115420679E-15 ) ) ;
#42229=CARTESIAN_POINT ( 'NONE',  ( -5.967884128652756637, 167.3615022471902591, -10.00000000000009592 ) ) ;
#42230=CARTESIAN_POINT ( 'NONE',  ( 33.34606076043043998, 183.3927522451418213, 10.00000000000009592 ) ) ;
#42231=CARTESIAN_POINT ( 'NONE',  ( 91.10780387927019319, 235.6589784336661353, -6.496448406907676862E-16 ) ) ;
#42234=CARTESIAN_POINT ( 'NONE',  ( 163.0076983195990294, 254.4055174419354159, -15.32059749880538568 ) ) ;
#42235=CARTESIAN_POINT ( 'NONE',  ( 12.11013585174968554, 186.9869531367911293, 4.594050593750046652 ) ) ;
#42237=CARTESIAN_POINT ( 'NONE',  ( 161.5056331467593225, 250.9110330116698435, 14.52719814064025528 ) ) ;
#42238=VERTEX_POINT ( 'NONE', #55856 ) ;
#42239=ORIENTED_EDGE ( 'NONE', *, *, #30639, .T. ) ;
#42240=CARTESIAN_POINT ( 'NONE',  ( 185.2106478887846777, 259.7847997664600257, -5.498830920350593843 ) ) ;
#42244=CARTESIAN_POINT ( 'NONE',  ( 193.1049081091807125, 263.9287996605999638, -4.331719323007160227 ) ) ;
#42245=CARTESIAN_POINT ( 'NONE',  ( 161.3773209892555371, 251.1332761876949746, -14.50043705923759241 ) ) ;
#42246=CARTESIAN_POINT ( 'NONE',  ( 144.9899443387551798, 254.5170451491295296, 0.000000000000000000 ) ) ;
#42247=CARTESIAN_POINT ( 'NONE',  ( 168.1916425577783514, 251.6829154642088895, 10.62658168803038095 ) ) ;
#42248=CARTESIAN_POINT ( 'NONE',  ( 49.16021902710897251, 193.0643266524159856, -9.188101187500093303 ) ) ;
#42249=CARTESIAN_POINT ( 'NONE',  ( 88.62734903533704767, 228.6427522451418781, -10.00000000000009415 ) ) ;
#42254=CARTESIAN_POINT ( 'NONE',  ( -2.639098984630277922, 169.2833772461660828, -9.188101187500095079 ) ) ;
#42256=CARTESIAN_POINT ( 'NONE',  ( 198.7357616895271804, 286.4265588032756114, -17.04018524297827497 ) ) ;
#42257=CARTESIAN_POINT ( 'NONE',  ( 179.0080424117914220, 253.6959867325634264, -1.969551310178471404 ) ) ;
#42258=CARTESIAN_POINT ( 'NONE',  ( 146.7944005049231180, 276.3916353892955726, -4.243051111306586520 ) ) ;
#42261=CARTESIAN_POINT ( 'NONE',  ( 78.03658003843786162, 205.8615022471901739, 5.000000000000051514 ) ) ;
#42262=CARTESIAN_POINT ( 'NONE',  ( 164.9335952247126045, 244.9736285262353306, -1.661461410667423255 ) ) ;
#42263=EDGE_CURVE ( 'NONE', #18147, #88849, #44446, .T. ) ;
#42266=CARTESIAN_POINT ( 'NONE',  ( 6.228640307978117185, 167.7365022471902023, 10.00000000000009592 ) ) ;
#42268=CARTESIAN_POINT ( 'NONE',  ( 122.5830220656496579, 232.3923013555409796, 4.594050593750050204 ) ) ;
#42271=CARTESIAN_POINT ( 'NONE',  ( 46.28462696178780789, 185.9824982072973967, 3.021315404115420679E-15 ) ) ;
#42272=CARTESIAN_POINT ( 'NONE',  ( 182.8798658535135928, 295.3622947365996083, -6.914253198550406765 ) ) ;
#42273=FACE_OUTER_BOUND ( 'NONE', #61271, .T. ) ;
#42275=ORIENTED_EDGE ( 'NONE', *, *, #78363, .F. ) ;
#42276=CARTESIAN_POINT ( 'NONE',  ( 191.5281967176683509, 298.9104275333885994, 7.715154960566919407 ) ) ;
#42277=CARTESIAN_POINT ( 'NONE',  ( 196.9431415128477170, 289.5314680279574304, -16.61413060656005669 ) ) ;
#42278=CARTESIAN_POINT ( 'NONE',  ( 180.6665526851674599, 287.6815954905284798, 14.11204521094005671 ) ) ;
#42279=CARTESIAN_POINT ( 'NONE',  ( 176.3588661899402439, 292.5224010984320557, -1.117630640333412639 ) ) ;
#42281=ORIENTED_EDGE ( 'NONE', *, *, #58382, .F. ) ;
#42282=CARTESIAN_POINT ( 'NONE',  ( 189.2748339612899144, 265.2827144222970333, 12.02701514401042360 ) ) ;
#42283=CARTESIAN_POINT ( 'NONE',  ( 168.3417633411148984, 271.6681995330380346, -17.37814367259023740 ) ) ;
#42285=EDGE_CURVE ( 'NONE', #56545, #66866, #97597, .T. ) ;
#42288=CARTESIAN_POINT ( 'NONE',  ( 196.2991918319561364, 270.8780335082191755, 12.03491514832104592 ) ) ;
#42289=CARTESIAN_POINT ( 'NONE',  ( 185.6543263943590603, 297.1164544966914605, 5.613520220585219711 ) ) ;
#42291=CARTESIAN_POINT ( 'NONE',  ( 148.1700451075146532, 274.5003607289000342, 6.655253088558737318 ) ) ;
#42293=CYLINDRICAL_SURFACE ( 'NONE', #58398, 10.00000000000010658 ) ;
#42295=CARTESIAN_POINT ( 'NONE',  ( 173.7786751825973681, 272.6665995263483637, -16.36869263761786897 ) ) ;
#42299=CARTESIAN_POINT ( 'NONE',  ( 156.1849287808383338, 261.6246031306073974, -17.08462936727468673 ) ) ;
#42303=CARTESIAN_POINT ( 'NONE',  ( 185.5025673201750749, 291.0580338203257611, 12.15717963013472769 ) ) ;
#42305=ORIENTED_EDGE ( 'NONE', *, *, #57869, .T. ) ;
#42309=CARTESIAN_POINT ( 'NONE',  ( 185.0126953839742896, 259.9172543619729936, -5.831654218434374926 ) ) ;
#42313=ORIENTED_EDGE ( 'NONE', *, *, #34981, .T. ) ;
#42314=CARTESIAN_POINT ( 'NONE',  ( 178.1963635607110916, 260.9795737440591097, 12.20855421423478404 ) ) ;
#42317=EDGE_LOOP ( 'NONE', ( #11494, #42956, #87157, #88247, #69342 ) ) ;
#42319=CARTESIAN_POINT ( 'NONE',  ( 155.4661767250933622, 261.3716783840932294, -17.10192542004562810 ) ) ;
#42320=VERTEX_POINT ( 'NONE', #45163 ) ;
#42321=CARTESIAN_POINT ( 'NONE',  ( 182.8342258324622378, 279.9465444586228386, -16.27734326228908301 ) ) ;
#42324=CARTESIAN_POINT ( 'NONE',  ( 160.5053574735698021, 276.1538589699120507, -12.57604534192124746 ) ) ;
#42325=CARTESIAN_POINT ( 'NONE',  ( 192.8011239859581849, 296.7056528303708660, -11.79847971295421694 ) ) ;
#42326=CARTESIAN_POINT ( 'NONE',  ( 200.6737073311291795, 283.0699384897140476, -17.61533935526990291 ) ) ;
#42328=CARTESIAN_POINT ( 'NONE',  ( 0.07393976959879319799, 182.3967562850347406, 2.649461200531984646E-14 ) ) ;
#42329=CARTESIAN_POINT ( 'NONE',  ( 140.9585647324944659, 258.3149278399160380, 9.188101187500093303 ) ) ;
#42330=VERTEX_POINT ( 'NONE', #99387 ) ;
#42334=CARTESIAN_POINT ( 'NONE',  ( 204.0750558719120988, 271.6231733279527703, 9.785492889829541241 ) ) ;
#42337=CARTESIAN_POINT ( 'NONE',  ( 122.4023397829301700, 248.1427522451419065, -10.00000000000009592 ) ) ;
#42338=CARTESIAN_POINT ( 'NONE',  ( 153.3256299635001483, 276.8936154282524171, 7.080213329903488173 ) ) ;
#42340=CARTESIAN_POINT ( 'NONE',  ( 171.6775608579050925, 280.0339643969739427, 13.87834783768247071 ) ) ;
#42347=ORIENTED_EDGE ( 'NONE', *, *, #63578, .F. ) ;
#42349=CARTESIAN_POINT ( 'NONE',  ( 200.9372752118609640, 267.7768021933786144, -2.766562499730290448 ) ) ;
#42352=CARTESIAN_POINT ( 'NONE',  ( 203.0398866899141126, 278.9715956204779559, 16.57839218037009132 ) ) ;
#42353=CARTESIAN_POINT ( 'NONE',  ( 170.3620333804029485, 268.1781345414723319, 17.80501103880222402 ) ) ;
#42356=CARTESIAN_POINT ( 'NONE',  ( 62.71875570545262946, 207.0177522451418497, -10.00000000000009592 ) ) ;
#42358=B_SPLINE_CURVE_WITH_KNOTS ( 'NONE', 3,
 ( #21679, #30267, #62145, #31258, #30776, #85521, #60150, #38351, #46445, #23153, #77886, #93091, #92606, #37851, #38856, #77378, #6968, #76391, #84021, #68759, #69762, #44962, #7980, #865, #23648, #91113, #37359, #61157, #53066, #45945, #54044, #52558, #99684, #60645, #370, #75901, #16065, #54538, #22172, #92126, #83514, #76862, #85002, #6481, #22679, #68264 ),
 .UNSPECIFIED., .F., .F.,
 ( 4, 2, 2, 2, 2, 2, 2, 2, 2, 2, 2, 2, 2, 2, 2, 2, 2, 2, 2, 2, 2, 2, 4 ),
 ( 0.001386463054751980182, 0.001851836421151829490, 0.002317209787551679015, 0.002549896470751603778, 0.002666239812351530163, 0.002782583153951456983, 0.002898926495551383802, 0.003015269837151310188, 0.003247956520351133903, 0.003713329886750830339, 0.004178703253150526341, 0.005109449985949853293, 0.006040196718749181112, 0.006505570085148845889, 0.006970943451548509799, 0.007087286793148386312, 0.007145458463948324568, 0.007203630134748261957, 0.007319973476348140204, 0.007436316817948018451, 0.007901690184347711851, 0.008367063550747406986, 0.008832436917147098651 ),
 .UNSPECIFIED. ) ;
#42361=CARTESIAN_POINT ( 'NONE',  ( 194.3094773688834778, 284.8302703302293253, 17.74979085435418469 ) ) ;
#42362=CARTESIAN_POINT ( 'NONE',  ( -22.42236680055709641, 157.8615022471902591, 0.000000000000000000 ) ) ;
#42364=DIRECTION ( 'NONE',  ( 0.8660254037844395958, 0.4999999999999985567, 0.000000000000000000 ) ) ;
#42365=CARTESIAN_POINT ( 'NONE',  ( 5.317335864756744357, 180.0024278399160949, -9.188101187500093303 ) ) ;
#42366=CARTESIAN_POINT ( 'NONE',  ( 111.1892885731694065, 228.8768266524159856, -9.188101187500091527 ) ) ;
#42367=CARTESIAN_POINT ( 'NONE',  ( 202.7754741559590173, 279.4295715634463022, -15.65855077192107636 ) ) ;
#42369=CARTESIAN_POINT ( 'NONE',  ( 186.3053879374282928, 296.7155014134779663, -7.306349104823136820 ) ) ;
#42374=FACE_OUTER_BOUND ( 'NONE', #89028, .T. ) ;
#42375=CARTESIAN_POINT ( 'NONE',  ( 194.3011251241114508, 294.1075746476782342, -14.76047579547631905 ) ) ;
#42376=CARTESIAN_POINT ( 'NONE',  ( 181.7502977777323281, 291.5405758491393726, 9.349876991887354549 ) ) ;
#42379=CARTESIAN_POINT ( 'NONE',  ( 164.5782759443297039, 245.5890595727670984, -5.697842221573455213 ) ) ;
#42381=DIRECTION ( 'NONE',  ( 0.8660254037844395958, 0.4999999999999985567, 0.000000000000000000 ) ) ;
#42383=CARTESIAN_POINT ( 'NONE',  ( 90.45192255479418009, 211.4824982072973683, 3.021315404115420679E-15 ) ) ;
#42386=CARTESIAN_POINT ( 'NONE',  ( 84.39645409570583467, 219.5333772461660544, 9.188101187500095079 ) ) ;
#42387=CARTESIAN_POINT ( 'NONE',  ( 161.4816992964961742, 250.9524876563463067, -12.92750327687364198 ) ) ;
#42388=CARTESIAN_POINT ( 'NONE',  ( 163.4945121521897988, 257.9090426894093184, 15.56564318970484884 ) ) ;
#42389=CARTESIAN_POINT ( 'NONE',  ( 157.8763546842245376, 257.1971277035954699, 17.68444922773363004 ) ) ;
#42391=CARTESIAN_POINT ( 'NONE',  ( 151.0013883899287066, 269.1049186256390726, -14.25461351222133466 ) ) ;
#42392=CARTESIAN_POINT ( 'NONE',  ( 175.9975959079605161, 269.8183398160408046, -16.55671884903257407 ) ) ;
#42395=CARTESIAN_POINT ( 'NONE',  ( 127.2636487221268311, 255.8297689869269504, -2.679491924311252493 ) ) ;
#42398=CARTESIAN_POINT ( 'NONE',  ( 77.03558525930309031, 203.0327760586659451, 1.948934522072302763E-15 ) ) ;
#42399=CARTESIAN_POINT ( 'NONE',  ( 173.0455529495148141, 289.6430652088176885, -1.041919219315089906 ) ) ;
#42403=CARTESIAN_POINT ( 'NONE',  ( 190.1859351024625369, 286.6565765330755085, 16.32613358219952104 ) ) ;
#42405=CARTESIAN_POINT ( 'NONE',  ( 118.6676052326576922, 245.9865022471903444, -10.00000000000009415 ) ) ;
#42406=FACE_OUTER_BOUND ( 'NONE', #55427, .T. ) ;
#42410=CARTESIAN_POINT ( 'NONE',  ( 165.6072792903335937, 246.7937695405969976, -1.477711117505905225 ) ) ;
#42412=CARTESIAN_POINT ( 'NONE',  ( 202.5245888501533216, 279.8641176599742266, 15.60152447840272494 ) ) ;
#42413=CARTESIAN_POINT ( 'NONE',  ( 207.2032113364036547, 269.9913168956704794, -0.07087847770824695637 ) ) ;
#42417=CARTESIAN_POINT ( 'NONE',  ( 188.8306723507383538, 290.8947323270112975, 14.73421016979825282 ) ) ;
#42418=ADVANCED_FACE ( 'NONE', ( #14909 ), #81349, .F. ) ;
#42419=CARTESIAN_POINT ( 'NONE',  ( 205.8346909429602363, 274.1308526569923742, 12.31208841938360976 ) ) ;
#42420=CARTESIAN_POINT ( 'NONE',  ( 78.92295937046175425, 204.8262482093457777, 3.021315404115420679E-15 ) ) ;
#42421=CARTESIAN_POINT ( 'NONE',  ( 154.0923235371355986, 263.7512619077765521, -17.59436137934181232 ) ) ;
#42426=CARTESIAN_POINT ( 'NONE',  ( -22.42236680055709641, 157.8615022471902591, 0.000000000000000000 ) ) ;
#42427=CARTESIAN_POINT ( 'NONE',  ( 173.8469137325424185, 256.4471593116459189, -12.44389045026504270 ) ) ;
#42430=CARTESIAN_POINT ( 'NONE',  ( 196.1252721995043942, 284.4712197134549001, -17.81715240067734030 ) ) ;
#42431=CARTESIAN_POINT ( 'NONE',  ( 204.2129321040862919, 276.9398213635460024, 14.41515352680879758 ) ) ;
#42432=CARTESIAN_POINT ( 'NONE',  ( 147.6884207308302450, 274.8431469350302336, -8.096293592099874203 ) ) ;
#42434=CARTESIAN_POINT ( 'NONE',  ( 193.9844289374573520, 294.6561085335266625, 15.49818881749970245 ) ) ;
#42435=CARTESIAN_POINT ( 'NONE',  ( 120.7221038307704788, 252.0530062829862743, -4.648177544792955347E-16 ) ) ;
#42436=CARTESIAN_POINT ( 'NONE',  ( 157.8043799545718286, 257.3217915922150496, -17.97575562758749257 ) ) ;
#42437=CARTESIAN_POINT ( 'NONE',  ( 164.1144691085127647, 246.3923965773001328, 5.648579756269943353 ) ) ;
#42438=CARTESIAN_POINT ( 'NONE',  ( 166.3040822299595050, 265.4869683937334912, 16.55097390736193219 ) ) ;
#42439=CARTESIAN_POINT ( 'NONE',  ( 179.3484401907847996, 256.1569968345440884, 4.890721239772626738 ) ) ;
#42440=CARTESIAN_POINT ( 'NONE',  ( 91.10780387927019319, 235.6589784336661353, -6.496448406907675876E-16 ) ) ;
#42444=CARTESIAN_POINT ( 'NONE',  ( 166.8095580818603025, 278.3619912271652765, -13.27947376363879251 ) ) ;
#42445=ORIENTED_EDGE ( 'NONE', *, *, #64757, .F. ) ;
#42449=CARTESIAN_POINT ( 'NONE',  ( 196.0760950258556363, 286.0837363073127904, -17.73048769406821279 ) ) ;
#42450=B_SPLINE_SURFACE_WITH_KNOTS ( 'NONE', 3, 1, ( 
 ( #72503, #8308 ),
 ( #39172, #95828 ),
 ( #64374, #18289 ),
 ( #92443, #46276 ),
 ( #39669, #70595 ),
 ( #49183, #61493 ),
 ( #76704, #70089 ),
 ( #69095, #7807 ),
 ( #38693, #22989 ),
 ( #1207, #7298 ),
 ( #53879, #699 ),
 ( #84840, #31582 ),
 ( #95336, #62475 ),
 ( #23994, #25894 ),
 ( #10681, #3109 ),
 ( #33997, #53397 ),
 ( #84347, #14893 ),
 ( #26878, #51673 ),
 ( #59233, #18785 ),
 ( #19786, #13185 ),
 ( #27866, #73982 ),
 ( #66367, #65856 ),
 ( #67355, #96817 ),
 ( #81607, #90209 ),
 ( #82117, #42549 ),
 ( #34469, #81122 ),
 ( #96310, #58745 ),
 ( #4566, #58259 ),
 ( #57259, #43038 ),
 ( #97786, #80621 ),
 ( #50655, #88733 ),
 ( #26381, #20279 ),
 ( #89718, #34956 ),
 ( #19303, #35462 ) ),
 .UNSPECIFIED., .T., .F., .F.,
 ( 4, 2, 2, 2, 2, 2, 2, 2, 2, 2, 2, 2, 2, 2, 2, 2, 4 ),
 ( 2, 2 ),
 ( 0.000000000000000000, 0.06250000000000000000, 0.1250000000000000000, 0.1875000000000000000, 0.2500000000000000000, 0.3125000000000000000, 0.3750000000000000000, 0.4375000000000000000, 0.5000000000000000000, 0.5625000000000000000, 0.6250000000000000000, 0.6875000000000000000, 0.7500000000000000000, 0.8125000000000000000, 0.8750000000000000000, 0.9375000000000000000, 1.000000000000000000 ),
 ( 0.000000000000000000, 1.000000000000000000 ),
 .UNSPECIFIED. ) ;
#42453=CARTESIAN_POINT ( 'NONE',  ( 208.2726345668874615, 269.9082104343620472, 2.818736869262927769 ) ) ;
#42454=CARTESIAN_POINT ( 'NONE',  ( 94.03063961704269502, 237.3464784336661637, 1.353441290958777327E-15 ) ) ;
#42455=ORIENTED_EDGE ( 'NONE', *, *, #5206, .F. ) ;
#42457=CARTESIAN_POINT ( 'NONE',  ( 162.6425574510925003, 248.9418223522047526, -10.70838742014210077 ) ) ;
#42459=EDGE_CURVE ( 'NONE', #99984, #72868, #38337, .T. ) ;
#42461=CARTESIAN_POINT ( 'NONE',  ( 170.4855375986076638, 248.6613294790634541, -0.2716024841417116753 ) ) ;
#42463=CARTESIAN_POINT ( 'NONE',  ( 165.5562080735016082, 285.3469202611815376, 0.5477150056637907216 ) ) ;
#42464=CARTESIAN_POINT ( 'NONE',  ( 124.8827946268633298, 255.1589784336661069, -6.496448406907675876E-16 ) ) ;
#42466=CARTESIAN_POINT ( 'NONE',  ( -12.69762320744227502, 170.1427522451419350, -10.00000000000009415 ) ) ;
#42469=CARTESIAN_POINT ( 'NONE',  ( 156.9781162866021589, 258.7529222455866034, 16.87007551417546480 ) ) ;
#42472=CARTESIAN_POINT ( 'NONE',  ( 188.8600501376575096, 269.6449448202791359, 14.64833052561093396 ) ) ;
#42474=( BOUNDED_CURVE ( )  B_SPLINE_CURVE ( 2, ( #47276, #94423, #39655, #38676, #188, #1705, #78199, #70577, #16879 ),
 .UNSPECIFIED., .F., .T. ) 
 B_SPLINE_CURVE_WITH_KNOTS ( ( 3, 2, 2, 2, 3 ),
 ( 0.6088709677419354982, 0.6102150537634408733, 0.6129032258064516236, 0.6155913978494623739, 0.6169354838709677491 ),
 .UNSPECIFIED. ) 
 CURVE ( )  GEOMETRIC_REPRESENTATION_ITEM ( )  RATIONAL_B_SPLINE_CURVE ( ( 0.9330127018922194093, 0.9330127018922194093, 1.000000000000000000, 0.8660254037844387076, 1.000000000000000000, 0.8660254037844387076, 1.000000000000000000, 0.9330127018922194093, 0.9330127018922194093 ) ) 
 REPRESENTATION_ITEM ( '' )  );
#42478=( BOUNDED_CURVE ( )  B_SPLINE_CURVE ( 2, ( #12147, #89689, #10652, #97269, #72970, #73453, #64849, #11166, #50138 ),
 .UNSPECIFIED., .F., .T. ) 
 B_SPLINE_CURVE_WITH_KNOTS ( ( 3, 2, 2, 2, 3 ),
 ( 0.1653225806451612823, 0.1666666666666666574, 0.1693548387096774077, 0.1720430107526881858, 0.1733870967741935609 ),
 .UNSPECIFIED. ) 
 CURVE ( )  GEOMETRIC_REPRESENTATION_ITEM ( )  RATIONAL_B_SPLINE_CURVE ( ( 0.9330127018922194093, 0.9330127018922194093, 1.000000000000000000, 0.8660254037844387076, 1.000000000000000000, 0.8660254037844387076, 1.000000000000000000, 0.9330127018922194093, 0.9330127018922194093 ) ) 
 REPRESENTATION_ITEM ( '' )  );
#42483=CARTESIAN_POINT ( 'NONE',  ( 178.2245750143592602, 292.8343567999519337, -5.806686789501219970 ) ) ;
#42485=ADVANCED_FACE ( 'NONE', ( #60108 ), #36013, .F. ) ;
#42487=CARTESIAN_POINT ( 'NONE',  ( 185.2191211618261661, 266.4373919749868378, 13.17776240725820358 ) ) ;
#42491=CARTESIAN_POINT ( 'NONE',  ( 192.2185419806677942, 297.7147144631093170, 12.45868041609393728 ) ) ;
#42495=ADVANCED_FACE ( 'NONE', ( #85473 ), #16019, .T. ) ;
#42496=CARTESIAN_POINT ( 'NONE',  ( 15.70964071017000663, 186.0024278399160949, -9.188101187500093303 ) ) ;
#42501=CARTESIAN_POINT ( 'NONE',  ( 207.7655736232174206, 270.7864657513322300, 3.530742899761726949 ) ) ;
#42503=CARTESIAN_POINT ( 'NONE',  ( 37.03551627836181837, 198.3149278399161233, 9.188101187500093303 ) ) ;
#42506=CARTESIAN_POINT ( 'NONE',  ( 147.1249913145849177, 275.8190353104462815, 3.637773609013635223 ) ) ;
#42508=CARTESIAN_POINT ( 'NONE',  ( 199.6009500900462115, 267.6840532653818059, -6.578795037453118333 ) ) ;
#42509=CARTESIAN_POINT ( 'NONE',  ( 178.8777897842755920, 293.7479682644459444, 2.680126103812829896 ) ) ;
#42510=CARTESIAN_POINT ( 'NONE',  ( 179.3350525740847274, 278.4300550830843690, -16.48020194126838334 ) ) ;
#42515=B_SPLINE_CURVE_WITH_KNOTS ( 'NONE', 3,
 ( #14142, #75454, #44017, #45030 ),
 .UNSPECIFIED., .F., .F.,
 ( 4, 4 ),
 ( 0.01114144257808264912, 0.01698608932288061743 ),
 .UNSPECIFIED. ) ;
#42516=CARTESIAN_POINT ( 'NONE',  ( 192.6198018426369458, 295.4256716423112152, -13.24907985865837468 ) ) ;
#42517=CARTESIAN_POINT ( 'NONE',  ( 77.24272341830202038, 228.7365022471903444, 2.944929066748280225E-16 ) ) ;
#42521=VERTEX_POINT ( 'NONE', #94062 ) ;
#42522=CARTESIAN_POINT ( 'NONE',  ( 39.63359248971512017, 199.8149278399161233, 9.188101187500093303 ) ) ;
#42524=CARTESIAN_POINT ( 'NONE',  ( 162.5372704899184839, 263.2211447608169692, 17.50793036557484683 ) ) ;
#42525=CARTESIAN_POINT ( 'NONE',  ( 198.5201458116119397, 286.8000164587433005, -18.30276554821096013 ) ) ;
#42527=ORIENTED_EDGE ( 'NONE', *, *, #51096, .T. ) ;
#42529=CARTESIAN_POINT ( 'NONE',  ( 168.1331800941538006, 285.1077698243100258, 7.621536105887456003 ) ) ;
#42530=CARTESIAN_POINT ( 'NONE',  ( 207.5686001603237116, 271.1276337968068333, 7.659944433763431704 ) ) ;
#42533=CARTESIAN_POINT ( 'NONE',  ( 186.0925163355340999, 262.9831289636886140, 11.40996487886282651 ) ) ;
#42534=CARTESIAN_POINT ( 'NONE',  ( -13.76211276271269668, 162.8615022471902591, -10.00000000000007816 ) ) ;
#42535=CARTESIAN_POINT ( 'NONE',  ( 171.3620354993367130, 255.7207998885352538, 11.34474888520862201 ) ) ;
#42536=VERTEX_POINT ( 'NONE', #47900 ) ;
#42539=CARTESIAN_POINT ( 'NONE',  ( 172.3741624485570867, 252.4865239976215037, 8.880853820034850798 ) ) ;
#42543=CARTESIAN_POINT ( 'NONE',  ( 182.5039235484258882, 284.0050300796905276, 15.07559313791482403 ) ) ;
#42544=CARTESIAN_POINT ( 'NONE',  ( 151.0099717111976076, 269.0900518771037468, 15.84752309685681659 ) ) ;
#42545=DIRECTION ( 'NONE',  ( 0.4999999999999998890, -0.8660254037844385966, 0.000000000000000000 ) ) ;
#42547=CARTESIAN_POINT ( 'NONE',  ( 161.3145230519951951, 251.2420454056404822, -14.44869077440025151 ) ) ;
#42549=CARTESIAN_POINT ( 'NONE',  ( 148.9285945872975390, 272.6951028054104427, -12.01265727652413240 ) ) ;
#42550=EDGE_LOOP ( 'NONE', ( #81380, #2345, #20441, #10156 ) ) ;
#42552=CARTESIAN_POINT ( 'NONE',  ( 159.5764336135613632, 254.2525046211064819, 15.32981087583629076 ) ) ;
#42555=CARTESIAN_POINT ( 'NONE',  ( 205.2121761402296443, 275.2090799237855094, -14.05269615702442465 ) ) ;
#42556=CARTESIAN_POINT ( 'NONE',  ( 114.1121243109418799, 230.5643266524159856, -9.188101187500093303 ) ) ;
#42557=FACE_OUTER_BOUND ( 'NONE', #91494, .T. ) ;
#42559=ORIENTED_EDGE ( 'NONE', *, *, #55165, .F. ) ;
#42560=CARTESIAN_POINT ( 'NONE',  ( 164.0179800784044915, 246.5595204798204065, -5.772998092557310557 ) ) ;
#42565=CARTESIAN_POINT ( 'NONE',  ( 73.73334276372742124, 219.5024278399160949, 9.188101187500095079 ) ) ;
#42567=CARTESIAN_POINT ( 'NONE',  ( 14.20097916528452942, 190.5530062829863311, -4.648177544792955347E-16 ) ) ;
#42568=CARTESIAN_POINT ( 'NONE',  ( 155.9200296242932495, 280.3860598674420430, -5.539708607631867565 ) ) ;
#42569=CARTESIAN_POINT ( 'NONE',  ( 150.9950855294679570, 269.1158355001903715, 14.12809338255366320 ) ) ;
#42570=CARTESIAN_POINT ( 'NONE',  ( 171.9138461029266409, 276.7610644589011031, 16.36093085335564723 ) ) ;
#42571=VERTEX_POINT ( 'NONE', #78337 ) ;
#42574=CARTESIAN_POINT ( 'NONE',  ( 203.4357368910538355, 278.2859629599173559, -16.45855118664066197 ) ) ;
#42576=CARTESIAN_POINT ( 'NONE',  ( 195.5097554423081760, 292.0141655289934874, 16.05747864979548112 ) ) ;
#42579=CARTESIAN_POINT ( 'NONE',  ( 207.8431546909062320, 270.6520914003897360, -6.441273666418043220 ) ) ;
#42580=CARTESIAN_POINT ( 'NONE',  ( 77.24272341830209143, 208.7365022471902023, -10.00000000000009237 ) ) ;
#42581=CARTESIAN_POINT ( 'NONE',  ( 149.9060791885465846, 273.0020498124315509, -11.57482514211843849 ) ) ;
#42582=CARTESIAN_POINT ( 'NONE',  ( 176.9166214895533642, 269.9654513595619960, 17.05290727745522972 ) ) ;
#42584=CARTESIAN_POINT ( 'NONE',  ( 151.5781362109140105, 269.4382799247086382, -14.31326077235408079 ) ) ;
#42586=CARTESIAN_POINT ( 'NONE',  ( 164.2414282675923403, 253.9130995731632083, 14.60178471863180327 ) ) ;
#42587=CARTESIAN_POINT ( 'NONE',  ( 163.7085541710205234, 247.0954618725873217, -6.713544974106887331 ) ) ;
#42588=CARTESIAN_POINT ( 'NONE',  ( 131.4326323866306439, 240.5643266524160140, 9.188101187500095079 ) ) ;
#42592=CIRCLE ( 'NONE', #78196, 17.82106496071138935 ) ;
#42593=CARTESIAN_POINT ( 'NONE',  ( 202.8549823380854491, 279.2918593523859272, -16.39745931995414807 ) ) ;
#42597=ORIENTED_EDGE ( 'NONE', *, *, #80108, .F. ) ;
#42600=CARTESIAN_POINT ( 'NONE',  ( 167.5662050468191637, 249.1799470243284986, -5.491780700972443974 ) ) ;
#42601=CARTESIAN_POINT ( 'NONE',  ( 164.8012313184158018, 245.2028895370295913, -2.462952685407667097 ) ) ;
#42602=CARTESIAN_POINT ( 'NONE',  ( 144.9642793207625004, 248.3768266524159856, -9.188101187500093303 ) ) ;
#42607=CARTESIAN_POINT ( 'NONE',  ( 157.7593757092099906, 257.3997412317380054, -18.08445832352326121 ) ) ;
#42608=CARTESIAN_POINT ( 'NONE',  ( 173.3722461183258190, 251.8737700704222107, 3.437992158665448272 ) ) ;
#42611=CARTESIAN_POINT ( 'NONE',  ( 190.7862358025146534, 300.1955415356651429, 3.573119809004446257 ) ) ;
#42612=CARTESIAN_POINT ( 'NONE',  ( 155.3570097178104277, 279.6568258031100527, -1.565792345466651359 ) ) ;
#42613=CARTESIAN_POINT ( 'NONE',  ( 169.3954986152665754, 285.0806455033480233, -8.523934259276524372 ) ) ;
#42614=CARTESIAN_POINT ( 'NONE',  ( 159.4889735931715222, 254.4039898200529706, 16.88104032092801887 ) ) ;
#42615=EDGE_CURVE ( 'NONE', #64780, #48318, #38321, .T. ) ;
#42616=CARTESIAN_POINT ( 'NONE',  ( 187.4307896699236835, 297.8422539827560058, -7.210019786355569060 ) ) ;
#42617=CARTESIAN_POINT ( 'NONE',  ( 137.1969404309142817, 260.0177522451418781, 5.000000000000046185 ) ) ;
#42618=ADVANCED_FACE ( 'NONE', ( #34587 ), #95944, .T. ) ;
#42621=ADVANCED_FACE ( 'NONE', ( #65487 ), #87811, .F. ) ;
#42622=CARTESIAN_POINT ( 'NONE',  ( 196.3519702320103590, 290.5554067223432639, 17.39042812051341969 ) ) ;
#42623=CARTESIAN_POINT ( 'NONE',  ( 190.5969391768923913, 300.5234129089444650, -0.7564693504096553500 ) ) ;
#42624=CARTESIAN_POINT ( 'NONE',  ( -9.729855525997878729, 171.3149278399161233, 9.188101187500093303 ) ) ;
#42625=CARTESIAN_POINT ( 'NONE',  ( 42.04265951369687571, 185.8923013555410080, 4.594050593750050204 ) ) ;
#42626=CARTESIAN_POINT ( 'NONE',  ( 175.4247336203138445, 256.7083858149467233, -10.72411828751436325 ) ) ;
#42629=CYLINDRICAL_SURFACE ( 'NONE', #91658, 10.00000000000010658 ) ;
#42631=CARTESIAN_POINT ( 'NONE',  ( 147.2494378675467033, 275.6034875578896504, 3.639370109197119341 ) ) ;
#42633=CARTESIAN_POINT ( 'NONE',  ( 167.4001030851802057, 256.8364653434372258, 14.17688984365114280 ) ) ;
#42634=CARTESIAN_POINT ( 'NONE',  ( 69.21394623383592659, 210.7677522451418497, 10.00000000000009592 ) ) ;
#42636=CARTESIAN_POINT ( 'NONE',  ( 157.8043799545718286, 257.3217915922150496, -17.97575562758749257 ) ) ;
#42638=CARTESIAN_POINT ( 'NONE',  ( 40.79748767570693246, 194.3615022471902591, -10.00000000000009592 ) ) ;
#42640=CARTESIAN_POINT ( 'NONE',  ( 163.2919429874875448, 247.8170536094679903, 9.876785378511263147 ) ) ;
#42641=CARTESIAN_POINT ( 'NONE',  ( 13.13906166239122619, 169.2048013555410080, 4.594050593750051981 ) ) ;
#42642=CARTESIAN_POINT ( 'NONE',  ( 168.1388510285085260, 286.2295795236503864, 4.095240327730098606 ) ) ;
#42643=FACE_OUTER_BOUND ( 'NONE', #57235, .T. ) ;
#42645=LINE ( 'NONE', #4159, #82174 ) ;
#42646=CARTESIAN_POINT ( 'NONE',  ( 207.6727254509676186, 270.9472835030587703, 7.315149605389819953 ) ) ;
#42647=CARTESIAN_POINT ( 'NONE',  ( 193.7261517370125432, 295.1034577671335342, 14.97744313279139661 ) ) ;
#42649=CARTESIAN_POINT ( 'NONE',  ( 176.5733983122591439, 260.2598607953340775, -13.59682439435957946 ) ) ;
#42653=CARTESIAN_POINT ( 'NONE',  ( 159.1730915527162438, 259.4008141402116507, 16.68298605874345597 ) ) ;
#42655=CARTESIAN_POINT ( 'NONE',  ( 152.7657949578753289, 278.5609422129916766, -4.697314451781300804 ) ) ;
#42657=CARTESIAN_POINT ( 'NONE',  ( 156.8398918776343294, 276.5535896746492313, 11.26052967366049806 ) ) ;
#42658=CARTESIAN_POINT ( 'NONE',  ( 159.8946522441011382, 253.7013337850969492, -16.68230890105693121 ) ) ;
#42659=ORIENTED_EDGE ( 'NONE', *, *, #96221, .T. ) ;
#42661=CARTESIAN_POINT ( 'NONE',  ( 206.9377610035629118, 272.2202792677204002, 7.440532334334675646 ) ) ;
#42663=CARTESIAN_POINT ( 'NONE',  ( 118.6676052326576922, 245.9865022471902876, -10.00000000000009592 ) ) ;
#42665=ORIENTED_EDGE ( 'NONE', *, *, #100184, .T. ) ;
#42667=CARTESIAN_POINT ( 'NONE',  ( 164.1571068132817857, 246.7865404346968035, -5.088878239364682976 ) ) ;
#42669=CARTESIAN_POINT ( 'NONE',  ( 153.4578721839791342, 264.8501638863745029, 16.85421393845643223 ) ) ;
#42672=CARTESIAN_POINT ( 'NONE',  ( 174.6205011729852856, 262.3198158003589242, 14.36378246763594468 ) ) ;
#42673=ORIENTED_EDGE ( 'NONE', *, *, #20368, .F. ) ;
#42675=CARTESIAN_POINT ( 'NONE',  ( 159.8822213732012756, 255.7228646850775533, -16.63148941946954196 ) ) ;
#42676=CARTESIAN_POINT ( 'NONE',  ( 149.6230451358742926, 271.4922791719315001, -12.72565967355361671 ) ) ;
#42678=CARTESIAN_POINT ( 'NONE',  ( 170.6178593158246315, 266.5408558992322696, -17.65857870869936974 ) ) ;
#42679=ORIENTED_EDGE ( 'NONE', *, *, #97840, .F. ) ;
#42680=CARTESIAN_POINT ( 'NONE',  ( 174.1176602439136332, 267.3798616381827173, 17.23308470258429992 ) ) ;
#42681=CARTESIAN_POINT ( 'NONE',  ( 166.0506673010352472, 274.1027903476490337, -16.62009509085023851 ) ) ;
#42684=ORIENTED_EDGE ( 'NONE', *, *, #3882, .F. ) ;
#42685=CARTESIAN_POINT ( 'NONE',  ( 176.8603533460532162, 279.0893642389937099, -16.89033693841190242 ) ) ;
#42686=CARTESIAN_POINT ( 'NONE',  ( 169.0226874675672661, 261.4850206712534373, -16.08682720245705156 ) ) ;
#42688=CARTESIAN_POINT ( 'NONE',  ( 179.4037581149374034, 257.9870511612666064, -10.76565914641300736 ) ) ;
#42689=ORIENTED_EDGE ( 'NONE', *, *, #89860, .T. ) ;
#42690=DIRECTION ( 'NONE',  ( -0.8660254037844387076, -0.4999999999999998890, -0.000000000000000000 ) ) ;
#42691=ORIENTED_EDGE ( 'NONE', *, *, #153, .F. ) ;
#42692=CARTESIAN_POINT ( 'NONE',  ( 158.8103961591765767, 260.0426163253080745, 17.56740887531538675 ) ) ;
#42697=CARTESIAN_POINT ( 'NONE',  ( 178.4964614385565653, 291.5674140005135087, 6.117148090635161850 ) ) ;
#42698=CARTESIAN_POINT ( 'NONE',  ( 158.3372743204232336, 256.3987914754929420, -17.01754169342242662 ) ) ;
#42703=CARTESIAN_POINT ( 'NONE',  ( 206.5318754762992910, 272.9232936229979032, 10.63244694018452741 ) ) ;
#42706=ORIENTED_EDGE ( 'NONE', *, *, #6227, .T. ) ;
#42707=CARTESIAN_POINT ( 'NONE',  ( 190.6453198962280453, 300.4396150449484821, 6.790521636783821258 ) ) ;
#42708=CARTESIAN_POINT ( 'NONE',  ( 171.4644772550263667, 259.7729622726477601, -14.70397530572840417 ) ) ;
#42711=CARTESIAN_POINT ( 'NONE',  ( 199.2085059260846549, 285.6077417665728149, -18.52696122218391750 ) ) ;
#42712=CARTESIAN_POINT ( 'NONE',  ( 190.1621882522046576, 301.2764235991409123, 0.1320823580815838616 ) ) ;
#42714=CARTESIAN_POINT ( 'NONE',  ( 167.2444082654604642, 252.9089594313395537, -12.21390469949916557 ) ) ;
#42715=CARTESIAN_POINT ( 'NONE',  ( 205.7543183366283870, 273.7119534119829609, 10.15442286887563839 ) ) ;
#42716=CYLINDRICAL_SURFACE ( 'NONE', #30127, 17.82106496071139645 ) ;
#42717=CARTESIAN_POINT ( 'NONE',  ( 165.0509870607838252, 244.7702999017660375, -2.356357909806504392 ) ) ;
#42718=CARTESIAN_POINT ( 'NONE',  ( 30.24280306353621128, 178.2677522451417929, -5.000000000000041744 ) ) ;
#42719=CARTESIAN_POINT ( 'NONE',  ( 111.8659576938172364, 226.2048013555410080, 4.594050593750051981 ) ) ;
#42721=CARTESIAN_POINT ( 'NONE',  ( 164.2369440024486664, 280.7661753373989768, -11.66746695687372615 ) ) ;
#42723=CARTESIAN_POINT ( 'NONE',  ( 207.7679535393632477, 270.7823436156499497, 1.643001479255987274 ) ) ;
#42724=CARTESIAN_POINT ( 'NONE',  ( 17.30628827445631401, 189.9869531367911293, 4.594050593750046652 ) ) ;
#42725=CARTESIAN_POINT ( 'NONE',  ( 176.5750811079351763, 290.0661888821730372, -9.631901365267058424 ) ) ;
#42727=EDGE_LOOP ( 'NONE', ( #74736, #77061, #87874, #14178 ) ) ;
#42729=CARTESIAN_POINT ( 'NONE',  ( 185.4335740946144711, 259.3911566074018538, -5.299005558259515247 ) ) ;
#42731=CARTESIAN_POINT ( 'NONE',  ( 147.4317198359019301, 275.2877659273946733, 3.797273160043843188 ) ) ;
#42734=CARTESIAN_POINT ( 'NONE',  ( 161.1232569692349443, 251.5733279787459367, -14.02750397520710557 ) ) ;
#42735=CARTESIAN_POINT ( 'NONE',  ( 182.3344119359328488, 284.3327036968043444, 14.89823965017127172 ) ) ;
#42736=CARTESIAN_POINT ( 'NONE',  ( -22.42236680055709641, 157.8615022471902591, 0.000000000000000000 ) ) ;
#42738=CARTESIAN_POINT ( 'NONE',  ( 38.41565749170202082, 202.1744531367911293, 4.594050593750047540 ) ) ;
#42739=CARTESIAN_POINT ( 'NONE',  ( 100.8960422556166634, 222.3927522451418213, 10.00000000000009592 ) ) ;
#42740=ORIENTED_EDGE ( 'NONE', *, *, #6844, .F. ) ;
#42742=EDGE_CURVE ( 'NONE', #92439, #21055, #21386, .T. ) ;
#42743=VECTOR ( 'NONE', #50424, 1000.000000000000000 ) ;
#42744=CARTESIAN_POINT ( 'NONE',  ( 178.9500347670535234, 258.7740023882205378, -10.02348361398978760 ) ) ;
#42745=CARTESIAN_POINT ( 'NONE',  ( -6.184650803196579893, 176.4244531367911293, -4.594050593750046652 ) ) ;
#42747=CARTESIAN_POINT ( 'NONE',  ( 198.4427928769277969, 286.9339956717308837, -17.97122743692687763 ) ) ;
#42749=CARTESIAN_POINT ( 'NONE',  ( 192.5551423381268989, 297.1317055421444024, -13.20528585388119858 ) ) ;
#42751=CARTESIAN_POINT ( 'NONE',  ( 204.1090098116124238, 275.4430282029952082, 13.26781899738782222 ) ) ;
#42753=CARTESIAN_POINT ( 'NONE',  ( 206.8986117509267899, 272.2880877623646825, 6.975890063856878598 ) ) ;
#42754=ORIENTED_EDGE ( 'NONE', *, *, #21470, .F. ) ;
#42755=( BOUNDED_CURVE ( )  B_SPLINE_CURVE ( 2, ( #35132, #73651, #11859, #4752, #19952, #19478, #73166, #27560, #4232 ),
 .UNSPECIFIED., .F., .T. ) 
 B_SPLINE_CURVE_WITH_KNOTS ( ( 3, 2, 2, 2, 3 ),
 ( 0.8750000000000000000, 0.8763440860215053752, 0.8790322580645161255, 0.8817204301075268758, 0.8830645161290322509 ),
 .UNSPECIFIED. ) 
 CURVE ( )  GEOMETRIC_REPRESENTATION_ITEM ( )  RATIONAL_B_SPLINE_CURVE ( ( 0.9330127018922194093, 0.9330127018922194093, 1.000000000000000000, 0.8660254037844387076, 1.000000000000000000, 0.8660254037844387076, 1.000000000000000000, 0.9330127018922194093, 0.9330127018922194093 ) ) 
 REPRESENTATION_ITEM ( '' )  );
#42756=CARTESIAN_POINT ( 'NONE',  ( 164.9872103004705082, 269.1319161758361247, 17.53557708690383876 ) ) ;
#42757=CARTESIAN_POINT ( 'NONE',  ( 7.888522331898304429, 165.3615022471902023, 5.000000000000051514 ) ) ;
#42759=CARTESIAN_POINT ( 'NONE',  ( 127.1025053677084742, 238.0643266524160424, -9.188101187500093303 ) ) ;
#42762=CARTESIAN_POINT ( 'NONE',  ( 150.9781172735503390, 269.9373692962728910, 13.75123450916632883 ) ) ;
#42763=CARTESIAN_POINT ( 'NONE',  ( 196.3021893095863959, 290.6416298092292436, 17.45656988653421138 ) ) ;
#42764=CARTESIAN_POINT ( 'NONE',  ( 189.4648164480647381, 289.7840259140004378, 14.59263643371816954 ) ) ;
#42768=CARTESIAN_POINT ( 'NONE',  ( 162.5148320529283126, 285.2034568178174254, 0.5437328601018158736 ) ) ;
#42769=CARTESIAN_POINT ( 'NONE',  ( 163.3761757142922875, 247.6711582469822019, 7.822525700913879554 ) ) ;
#42771=CARTESIAN_POINT ( 'NONE',  ( 173.0221673524149537, 268.1772831482880974, -16.30159817659111354 ) ) ;
#42774=DIRECTION ( 'NONE',  ( -0.8660254037844387076, -0.4999999999999998890, -0.000000000000000000 ) ) ;
#42775=CARTESIAN_POINT ( 'NONE',  ( 165.4631639692057092, 269.4820744690946981, -16.38125699399958890 ) ) ;
#42777=CARTESIAN_POINT ( 'NONE',  ( 149.3083371557971475, 273.7923365791965580, -10.10007029348708585 ) ) ;
#42779=CARTESIAN_POINT ( 'NONE',  ( 181.8748162431300273, 295.1086854819222367, 4.838109536733072424 ) ) ;
#42781=DIRECTION ( 'NONE',  ( -0.8660254037844387076, -0.4999999999999998890, -0.000000000000000000 ) ) ;
#42782=CARTESIAN_POINT ( 'NONE',  ( 193.4106419289095413, 282.3615967192327503, 16.94929546279620780 ) ) ;
#42784=CARTESIAN_POINT ( 'NONE',  ( -22.42236680055709641, 157.8615022471902591, 0.000000000000000000 ) ) ;
#42787=CARTESIAN_POINT ( 'NONE',  ( 194.1972774922283236, 294.2874440223457100, -15.09915398317898649 ) ) ;
#42788=CARTESIAN_POINT ( 'NONE',  ( 159.6845851668356602, 264.1119169267814186, -17.40983169896417593 ) ) ;
#42789=ORIENTED_EDGE ( 'NONE', *, *, #15658, .T. ) ;
#42792=EDGE_CURVE ( 'NONE', #40669, #99571, #56467, .T. ) ;
#42794=EDGE_LOOP ( 'NONE', ( #28842, #4179, #95475 ) ) ;
#42795=CARTESIAN_POINT ( 'NONE',  ( 90.72943840876205002, 217.0643266524159856, -9.188101187500093303 ) ) ;
#42798=CARTESIAN_POINT ( 'NONE',  ( 183.0029883054649247, 258.5817195840489262, -5.861537397372212688 ) ) ;
#42800=CARTESIAN_POINT ( 'NONE',  ( 191.3843761966370209, 282.8631020262318430, -17.76976768207862278 ) ) ;
#42801=VERTEX_POINT ( 'NONE', #6176 ) ;
#42802=CARTESIAN_POINT ( 'NONE',  ( 175.4039180538638050, 286.4985578832265105, -12.71199677751706503 ) ) ;
#42803=AXIS2_PLACEMENT_3D ( 'NONE', #42099, #96346, #88771 ) ;
#42807=CARTESIAN_POINT ( 'NONE',  ( 203.3740894404336927, 278.3927394765486838, -15.19753795879846869 ) ) ;
#42811=CARTESIAN_POINT ( 'NONE',  ( 162.6510684159478899, 255.6836685834286698, -14.96140778093960044 ) ) ;
#42812=CARTESIAN_POINT ( 'NONE',  ( 158.6360470686486792, 274.9027906808635180, -12.66648404655886395 ) ) ;
#42818=CARTESIAN_POINT ( 'NONE',  ( 147.5623555321158165, 249.8768266524159856, -9.188101187500091527 ) ) ;
#42819=CARTESIAN_POINT ( 'NONE',  ( 168.1596581537996542, 267.1068951904059645, -17.02861468427176206 ) ) ;
#42822=ORIENTED_EDGE ( 'NONE', *, *, #34421, .F. ) ;
#42823=CARTESIAN_POINT ( 'NONE',  ( 204.0811171663250150, 271.5389168563704061, 9.836206406191243090 ) ) ;
#42824=ORIENTED_EDGE ( 'NONE', *, *, #18207, .F. ) ;
#42825=CARTESIAN_POINT ( 'NONE',  ( 203.2757866645317222, 269.5093088776978334, -7.514607224931010521 ) ) ;
#42826=CARTESIAN_POINT ( 'NONE',  ( 163.1008115941903895, 248.1481028935802442, 11.25332017433677834 ) ) ;
#42830=CARTESIAN_POINT ( 'NONE',  ( 174.5324672201822409, 281.8837275374356750, 14.18752577204586274 ) ) ;
#42833=ORIENTED_EDGE ( 'NONE', *, *, #16316, .T. ) ;
#42836=CARTESIAN_POINT ( 'NONE',  ( 194.3496232524742879, 293.5687256674401056, -14.39162217157957890 ) ) ;
#42837=CARTESIAN_POINT ( 'NONE',  ( 201.0634398150303070, 267.8636890061912368, -2.845120707021614237 ) ) ;
#42838=CARTESIAN_POINT ( 'NONE',  ( 163.7706638094790605, 246.9878848231379038, -7.366147995746058719 ) ) ;
#42839=CARTESIAN_POINT ( 'NONE',  ( 193.7796494901127744, 262.2143583836045764, -1.898228983734132846 ) ) ;
#42840=CARTESIAN_POINT ( 'NONE',  ( 160.7802298691281351, 272.6907373984244032, 15.57769528675181903 ) ) ;
#42841=CARTESIAN_POINT ( 'NONE',  ( 161.0749639472951742, 282.0180817886167688, -7.709404307391809930 ) ) ;
#42844=CARTESIAN_POINT ( 'NONE',  ( 168.2356071464602962, 248.8554872198452301, 6.669745218284529820 ) ) ;
#42851=CARTESIAN_POINT ( 'NONE',  ( 175.0125019719911847, 292.0719086349095051, 3.303583340955516423 ) ) ;
#42852=CARTESIAN_POINT ( 'NONE',  ( 192.1883190596398094, 297.7670620978826150, 12.41391288785556668 ) ) ;
#42855=CARTESIAN_POINT ( 'NONE',  ( 11.92112666437810908, 171.5643266524160140, 9.188101187500095079 ) ) ;
#42856=CARTESIAN_POINT ( 'NONE',  ( 101.1213961584103060, 235.3149278399160949, -9.188101187500095079 ) ) ;
#42859=CARTESIAN_POINT ( 'NONE',  ( 180.3719397577650625, 255.7858912907505271, -2.354358376422963417 ) ) ;
#42863=CARTESIAN_POINT ( 'NONE',  ( 163.7018558908529826, 283.5206950014648442, 5.691029027290803732 ) ) ;
#42864=CARTESIAN_POINT ( 'NONE',  ( 194.9385458806846430, 293.0035295114944347, -15.70518692812489192 ) ) ;
#42867=CARTESIAN_POINT ( 'NONE',  ( 189.2845499996045930, 259.5340837477176024, -0.8149847707460528001 ) ) ;
#42868=CARTESIAN_POINT ( 'NONE',  ( 165.7619395286449162, 253.6454674417704780, -13.15779432277202865 ) ) ;
#42870=CARTESIAN_POINT ( 'NONE',  ( 172.5158698997361171, 263.7363841177182735, -15.44335349234447108 ) ) ;
#42871=CARTESIAN_POINT ( 'NONE',  ( 83.61187889534991768, 209.8923013555409796, 4.594050593750050204 ) ) ;
#42872=CARTESIAN_POINT ( 'NONE',  ( 207.8984236726843164, 270.5563627158673512, -6.084369154771423815 ) ) ;
#42874=DIRECTION ( 'NONE',  ( -0.8660254037844387076, -0.4999999999999998890, -0.000000000000000000 ) ) ;
#42875=CARTESIAN_POINT ( 'NONE',  ( 196.0034224882197975, 291.1591091234520263, 17.53794140922627776 ) ) ;
#42878=CARTESIAN_POINT ( 'NONE',  ( 173.2357414004084717, 267.9835125820733310, -16.29977483448695708 ) ) ;
#42880=CARTESIAN_POINT ( 'NONE',  ( 146.8868584395697781, 276.2314935489248455, -3.891417269505058396 ) ) ;
#42881=CARTESIAN_POINT ( 'NONE',  ( 136.0806360202347491, 237.8262482093457493, 3.021315404115420679E-15 ) ) ;
#42886=CARTESIAN_POINT ( 'NONE',  ( 190.6592569510245596, 287.2925400494787027, -15.83648776903241817 ) ) ;
#42887=EDGE_LOOP ( 'NONE', ( #100077, #45937, #55522, #20408 ) ) ;
#42889=CARTESIAN_POINT ( 'NONE',  ( 157.2276673882269051, 268.6185831692512238, 15.65931871386393226 ) ) ;
#42891=CARTESIAN_POINT ( 'NONE',  ( 142.1224599184862711, 252.8615022471902307, -10.00000000000009592 ) ) ;
#42896=VERTEX_POINT ( 'NONE', #2085 ) ;
#42897=CARTESIAN_POINT ( 'NONE',  ( 162.7561251957091031, 248.7451172484279027, 11.07313294959361194 ) ) ;
#42904=CARTESIAN_POINT ( 'NONE',  ( 157.9182071844803943, 257.7446772440080736, -16.73371276857705681 ) ) ;
#42906=FACE_OUTER_BOUND ( 'NONE', #98403, .T. ) ;
#42908=EDGE_CURVE ( 'NONE', #94798, #77324, #29913, .T. ) ;
#42911=EDGE_CURVE ( 'NONE', #71353, #12301, #100095, .T. ) ;
#42912=CARTESIAN_POINT ( 'NONE',  ( 167.7466885841891724, 276.4027061906341487, 15.04260431868030068 ) ) ;
#42913=CARTESIAN_POINT ( 'NONE',  ( 82.65769392073423205, 206.9824982072973967, 3.021315404115420679E-15 ) ) ;
#42916=ORIENTED_EDGE ( 'NONE', *, *, #78197, .T. ) ;
#42918=CARTESIAN_POINT ( 'NONE',  ( 204.1793240545508752, 276.9980322128846524, 14.17550310845996187 ) ) ;
#42919=CARTESIAN_POINT ( 'NONE',  ( 162.3140616334688389, 272.4534376533870841, -16.17207721611645965 ) ) ;
#42920=B_SPLINE_CURVE_WITH_KNOTS ( 'NONE', 3,
 ( #63551, #46854, #78773, #62031, #92982, #77777, #1264, #39231, #70138, #70650, #32148, #94492, #63055, #55429, #86418, #25052, #49359, #72691, #2787, #3768, #3284, #41747, #88421, #10871, #33671, #50348, #11389, #57443, #35147, #34165, #18981, #65057, #18472, #49853, #4768, #80819, #81301, #88933, #42240, #20464, #73178, #11874, #42729, #73667, #4247, #34650, #96007, #66056, #58920, #65550 ),
 .UNSPECIFIED., .F., .F.,
 ( 4, 2, 2, 2, 2, 2, 2, 2, 2, 2, 2, 2, 2, 2, 2, 2, 2, 2, 2, 2, 2, 2, 2, 2, 4 ),
 ( 0.0001133116680782004403, 0.001133496570739383601, 0.001643589022070062779, 0.001771112134902744824, 0.001898635247735426653, 0.002026158360568108482, 0.002153681473400790528, 0.002408727699066037526, 0.002663773924731284957, 0.003173866376061861352, 0.004194051278722935212, 0.005214236181384009940, 0.005724328632714509139, 0.005979374858379796036, 0.006234421084045082932, 0.006298182640461369962, 0.006361944196877656124, 0.006425705753293943154, 0.006489467309710230183, 0.006744513535375672338, 0.006999559761041115359, 0.007254605986706557513, 0.007509652212371999667, 0.007764698438037443556, 0.008274790889368326130 ),
 .UNSPECIFIED. ) ;
#42922=CARTESIAN_POINT ( 'NONE',  ( 194.1153812227096864, 294.4292925221022870, 15.54001482840963710 ) ) ;
#42925=CARTESIAN_POINT ( 'NONE',  ( 207.8721260090728720, 270.6019116053632843, -5.149293805580906991 ) ) ;
#42927=CARTESIAN_POINT ( 'NONE',  ( 167.6797392981326595, 266.2679195731100776, 16.57304949636104752 ) ) ;
#42928=CARTESIAN_POINT ( 'NONE',  ( 181.6314276487895540, 257.0242095793732915, 5.011107819272414332 ) ) ;
#42929=CARTESIAN_POINT ( 'NONE',  ( 95.76303752037657091, 226.0958772461660260, -9.188101187500095079 ) ) ;
#42932=CARTESIAN_POINT ( 'NONE',  ( 166.2700931250637666, 279.3192040119241142, -14.00315165249155669 ) ) ;
#42935=ORIENTED_EDGE ( 'NONE', *, *, #50326, .T. ) ;
#42938=CARTESIAN_POINT ( 'NONE',  ( 180.4853699739515775, 293.9068444078645825, -2.637950556201079877 ) ) ;
#42939=CARTESIAN_POINT ( 'NONE',  ( 196.2609093297512857, 290.7131288316392670, 16.03897268885959448 ) ) ;
#42940=CARTESIAN_POINT ( 'NONE',  ( 159.9788992190088948, 253.5554137441726255, -15.81862932303382330 ) ) ;
#42941=CARTESIAN_POINT ( 'NONE',  ( 207.2149758913051585, 271.2477481997252085, -3.868811482646887789 ) ) ;
#42943=ORIENTED_EDGE ( 'NONE', *, *, #82167, .F. ) ;
#42945=ORIENTED_EDGE ( 'NONE', *, *, #85707, .T. ) ;
#42946=CARTESIAN_POINT ( 'NONE',  ( 208.0421103033489771, 270.3074901711881353, -2.473242163239977476 ) ) ;
#42948=B_SPLINE_CURVE_WITH_KNOTS ( 'NONE', 3,
 ( #11779, #73570, #80717, #89794 ),
 .UNSPECIFIED., .F., .F.,
 ( 4, 4 ),
 ( 0.009049921839384984096, 0.01512907757492281194 ),
 .UNSPECIFIED. ) ;
#42949=B_SPLINE_CURVE_WITH_KNOTS ( 'NONE', 3,
 ( #20161, #52041, #82980, #11566 ),
 .UNSPECIFIED., .F., .F.,
 ( 4, 4 ),
 ( 0.03276373770747892378, 0.04170172322417993460 ),
 .UNSPECIFIED. ) ;
#42950=CARTESIAN_POINT ( 'NONE',  ( 194.5803990493530478, 266.2842781977357163, -7.755041682219012245 ) ) ;
#42953=CARTESIAN_POINT ( 'NONE',  ( 128.2389901622930495, 244.8458772461660544, 9.188101187500095079 ) ) ;
#42954=CARTESIAN_POINT ( 'NONE',  ( 199.7528798840209276, 284.2810620923601164, 16.93803948313987817 ) ) ;
#42956=ORIENTED_EDGE ( 'NONE', *, *, #85085, .T. ) ;
#42957=CARTESIAN_POINT ( 'NONE',  ( 204.8109598484962532, 275.9040069258922472, 13.12942483889034762 ) ) ;
#42958=CARTESIAN_POINT ( 'NONE',  ( 54.58172535260923297, 208.9865022471903160, 10.00000000000009415 ) ) ;
#42959=ADVANCED_FACE ( 'NONE', ( #63870 ), #10680, .T. ) ;
#42961=CARTESIAN_POINT ( 'NONE',  ( 191.8644938906121808, 271.7084166993448662, 14.16934409235493320 ) ) ;
#42962=CARTESIAN_POINT ( 'NONE',  ( 123.2062803672525604, 230.3932355074535394, -2.679491924311248496 ) ) ;
#42963=DIRECTION ( 'NONE',  ( -0.8660254037844387076, -0.4999999999999998890, -0.000000000000000000 ) ) ;
#42965=FACE_OUTER_BOUND ( 'NONE', #4946, .T. ) ;
#42966=ADVANCED_FACE ( 'NONE', ( #88732 ), #88233, .T. ) ;
#42967=CARTESIAN_POINT ( 'NONE',  ( 200.7523954295751594, 282.9336467052548869, 18.23634913067694185 ) ) ;
#42968=CARTESIAN_POINT ( 'NONE',  ( 206.6509060984486155, 272.1412184117673974, 7.097787738138362279 ) ) ;
#42969=CARTESIAN_POINT ( 'NONE',  ( 159.8188415394622268, 253.8326417772889840, -15.43862849427313222 ) ) ;
#42970=LINE ( 'NONE', #29793, #22434 ) ;
#42971=CARTESIAN_POINT ( 'NONE',  ( -10.31836507581447471, 176.3967562850347406, -4.648177544792955347E-16 ) ) ;
#42975=EDGE_CURVE ( 'NONE', #4228, #63881, #21496, .T. ) ;
#42978=CARTESIAN_POINT ( 'NONE',  ( 185.3757608622346709, 266.4090302586452594, 13.11668907775444204 ) ) ;
#42979=EDGE_CURVE ( 'NONE', #89111, #47191, #97250, .T. ) ;
#42980=CARTESIAN_POINT ( 'NONE',  ( 68.87660500748863512, 222.1199935810940929, 2.679491924311251605 ) ) ;
#42982=CARTESIAN_POINT ( 'NONE',  ( 149.7318359886737937, 272.2261244477465993, -11.42674851380234813 ) ) ;
#42984=CARTESIAN_POINT ( 'NONE',  ( 157.6161041218087746, 270.9124938997304639, -14.78071789165227834 ) ) ;
#42985=AXIS2_PLACEMENT_3D ( 'NONE', #59145, #11603, #82023 ) ;
#42987=B_SPLINE_CURVE_WITH_KNOTS ( 'NONE', 3,
 ( #22890, #62375, #84738, #15279 ),
 .UNSPECIFIED., .F., .F.,
 ( 4, 4 ),
 ( 0.02551283278911079672, 0.03475741272028291112 ),
 .UNSPECIFIED. ) ;
#42988=CARTESIAN_POINT ( 'NONE',  ( 7.238742955462222461, 184.1744531367911293, 4.594050593750047540 ) ) ;
#42989=CARTESIAN_POINT ( 'NONE',  ( 41.64315915125185086, 206.3967562850347122, -4.648177544792955347E-16 ) ) ;
#42994=CARTESIAN_POINT ( 'NONE',  ( 35.46636587765004123, 179.0327760586659736, 1.948934522072302763E-15 ) ) ;
#42996=CARTESIAN_POINT ( 'NONE',  ( 174.6041121390431670, 289.2630556414907801, 7.804972839359269443 ) ) ;
#42997=CARTESIAN_POINT ( 'NONE',  ( 190.3286155001717930, 300.9881631498979004, -5.624828231725103045 ) ) ;
#42999=CARTESIAN_POINT ( 'NONE',  ( 203.1203444092346899, 269.7784739467876420, -7.400015971792329061 ) ) ;
#43000=CARTESIAN_POINT ( 'NONE',  ( 146.5913834600193582, 276.7432712258716947, -0.4909717733184599253 ) ) ;
#43003=CARTESIAN_POINT ( 'NONE',  ( 147.8791740781505837, 276.5127524457575987, 2.771564245682613947 ) ) ;
#43007=CARTESIAN_POINT ( 'NONE',  ( 160.8891438268352374, 281.0495864612497599, 9.578199528566821996 ) ) ;
#43008=CARTESIAN_POINT ( 'NONE',  ( 75.87151652897667020, 224.6115022471903160, -5.000000000000047962 ) ) ;
#43010=CARTESIAN_POINT ( 'NONE',  ( 162.0192538899617318, 268.0510789565263394, -17.53028463913764057 ) ) ;
#43012=CARTESIAN_POINT ( 'NONE',  ( 59.93088934303040816, 217.6589784336661637, -6.496448406907675876E-16 ) ) ;
#43014=CARTESIAN_POINT ( 'NONE',  ( 162.8839417982861448, 263.3994626277539055, 17.77684832337497767 ) ) ;
#43015=CARTESIAN_POINT ( 'NONE',  ( 146.8358616138309571, 276.3198226421291679, 4.054088818585255716 ) ) ;
#43017=VERTEX_POINT ( 'NONE', #44541 ) ;
#43018=CARTESIAN_POINT ( 'NONE',  ( 167.5553568848317525, 285.0228605941855449, 7.731127579155963048 ) ) ;
#43019=CARTESIAN_POINT ( 'NONE',  ( 164.2672861321391053, 246.1277097281173667, -2.417001679502223777 ) ) ;
#43020=CARTESIAN_POINT ( 'NONE',  ( 188.9122134955663910, 290.7695941481946988, -15.11888497690123678 ) ) ;
#43022=CARTESIAN_POINT ( 'NONE',  ( 189.2086094880577889, 265.3749622005305469, 10.54437259076535227 ) ) ;
#43024=CARTESIAN_POINT ( 'NONE',  ( 171.3037854771465618, 255.8038501838435934, 11.58489188490385224 ) ) ;
#43025=ORIENTED_EDGE ( 'NONE', *, *, #77665, .F. ) ;
#43028=CARTESIAN_POINT ( 'NONE',  ( 22.68312297988245163, 177.2365022471902023, -10.00000000000009237 ) ) ;
#43031=CARTESIAN_POINT ( 'NONE',  ( 26.96143514339544467, 174.8262482093457777, 3.021315404115420679E-15 ) ) ;
#43032=CARTESIAN_POINT ( 'NONE',  ( 167.2952297142404632, 261.5110431333442307, 16.99354490899708381 ) ) ;
#43034=ORIENTED_EDGE ( 'NONE', *, *, #45353, .T. ) ;
#43036=CARTESIAN_POINT ( 'NONE',  ( 207.8996209429610360, 270.5542889829179103, -5.987818313449536411 ) ) ;
#43038=CARTESIAN_POINT ( 'NONE',  ( 149.0203866098534888, 272.5361143586139860, -12.73049804737905255 ) ) ;
#43039=ORIENTED_EDGE ( 'NONE', *, *, #44744, .T. ) ;
#43045=CARTESIAN_POINT ( 'NONE',  ( 112.1907172202364080, 226.3923013555410080, 4.594050593750050204 ) ) ;
#43046=ADVANCED_FACE ( 'NONE', ( #99275 ), #90717, .T. ) ;
#43047=CARTESIAN_POINT ( 'NONE',  ( 204.8284483594339065, 275.8737159363993214, 14.69997973035875383 ) ) ;
#43048=DIRECTION ( 'NONE',  ( 0.4999999999999998890, -0.8660254037844385966, 0.000000000000000000 ) ) ;
#43049=ORIENTED_EDGE ( 'NONE', *, *, #44948, .T. ) ;
#43050=CARTESIAN_POINT ( 'NONE',  ( 163.8111161534324935, 246.9178193081252743, -7.110480325054721717 ) ) ;
#43055=CARTESIAN_POINT ( 'NONE',  ( 73.24602992621615272, 225.3464784336661353, 1.353441290958777525E-15 ) ) ;
#43057=EDGE_CURVE ( 'NONE', #8187, #68859, #74980, .T. ) ;
#43058=CARTESIAN_POINT ( 'NONE',  ( 170.5993847053230468, 287.8722104901659691, 7.679145147933459370 ) ) ;
#43061=CARTESIAN_POINT ( 'NONE',  ( 198.4688822609874137, 286.8888075330012839, 18.53129255230862071 ) ) ;
#43063=CARTESIAN_POINT ( 'NONE',  ( 172.1403850395635118, 276.9566470737562440, 16.52013608218327079 ) ) ;
#43069=CARTESIAN_POINT ( 'NONE',  ( 195.5000684248051073, 292.0309439354826964, 16.15209601369885206 ) ) ;
#43071=CARTESIAN_POINT ( 'NONE',  ( 207.1432938686257046, 271.8642859028066141, -6.405155839440290322 ) ) ;
#43075=CARTESIAN_POINT ( 'NONE',  ( 205.9642072045669465, 273.9065239114831911, 10.22128930895731536 ) ) ;
#43076=CARTESIAN_POINT ( 'NONE',  ( 125.9182562534771677, 255.0530062829863311, -4.648177544792955347E-16 ) ) ;
#43078=CARTESIAN_POINT ( 'NONE',  ( 207.8725590214046406, 270.6011616060040410, 1.988011721677743093 ) ) ;
#43079=CARTESIAN_POINT ( 'NONE',  ( 126.7237928014352804, 231.7202760586659736, -5.415160957724236172E-17 ) ) ;
#43084=CARTESIAN_POINT ( 'NONE',  ( 205.8889072768004951, 273.5716727396786041, -9.812782715980612025 ) ) ;
#43085=CARTESIAN_POINT ( 'NONE',  ( 164.2712161151136172, 246.1209027979328710, 7.276091357954241445 ) ) ;
#43087=FACE_OUTER_BOUND ( 'NONE', #99267, .T. ) ;
#43090=CARTESIAN_POINT ( 'NONE',  ( 182.2429953966146172, 275.8324561883076171, -16.43557028755543215 ) ) ;
#43092=CARTESIAN_POINT ( 'NONE',  ( 166.9253229281109157, 248.7550762113961582, -5.490293681429817774 ) ) ;
#43093=CARTESIAN_POINT ( 'NONE',  ( 0.07393976959879319799, 182.3967562850347406, 2.649461200531984646E-14 ) ) ;
#43094=CARTESIAN_POINT ( 'NONE',  ( 30.24280306353613312, 198.2677522451419350, -5.000000000000047962 ) ) ;
#43096=CARTESIAN_POINT ( 'NONE',  ( 190.3286155001717930, 300.9881631498979004, -5.624828231725103045 ) ) ;
#43099=CARTESIAN_POINT ( 'NONE',  ( 170.8035993136612376, 250.5442460706725569, 3.418796778386401947 ) ) ;
#43102=CARTESIAN_POINT ( 'NONE',  ( 149.6071296322179194, 271.5198456328920997, 12.75640156477042453 ) ) ;
#43103=CARTESIAN_POINT ( 'NONE',  ( -22.42236680055709641, 157.8615022471902591, 0.000000000000000000 ) ) ;
#43104=CARTESIAN_POINT ( 'NONE',  ( 169.0232266158229208, 285.7259705221371746, -9.141046413429966933 ) ) ;
#43105=CARTESIAN_POINT ( 'NONE',  ( 159.4574711498080433, 254.4585536525209477, 16.86100557095418395 ) ) ;
#43106=CARTESIAN_POINT ( 'NONE',  ( 193.1232865735839539, 289.3006304592061610, 16.37785481887425476 ) ) ;
#43107=CARTESIAN_POINT ( 'NONE',  ( 131.5677753063154682, 256.7677522451419350, -5.000000000000047962 ) ) ;
#43108=CARTESIAN_POINT ( 'NONE',  ( 183.3171886181362140, 279.0376548180590817, 17.18391320931595345 ) ) ;
#43110=CARTESIAN_POINT ( 'NONE',  ( 157.6286460899086137, 257.6261715744221306, 18.25526781158026779 ) ) ;
#43111=CARTESIAN_POINT ( 'NONE',  ( 198.5970767652345899, 286.6667681383942181, -17.17073100918929640 ) ) ;
#43112=CARTESIAN_POINT ( 'NONE',  ( -12.05712525078605069, 163.8458772461660544, 9.188101187500095079 ) ) ;
#43114=CARTESIAN_POINT ( 'NONE',  ( 56.95444766116892055, 197.5643266524159856, -9.188101187500093303 ) ) ;
#43115=CARTESIAN_POINT ( 'NONE',  ( 178.0613071443478930, 258.8060421996208902, -10.32626121482724102 ) ) ;
#43118=CARTESIAN_POINT ( 'NONE',  ( 157.8719920515997046, 257.2046840049564480, -17.69857783492101433 ) ) ;
#43123=CARTESIAN_POINT ( 'NONE',  ( 174.9671601572613326, 281.6994072225486434, -15.63500919100072473 ) ) ;
#43124=CARTESIAN_POINT ( 'NONE',  ( 68.70876474829496772, 217.1427522451419065, 10.00000000000009237 ) ) ;
#43127=CARTESIAN_POINT ( 'NONE',  ( 198.4688822609874137, 286.8888075330012839, 18.53129255230862071 ) ) ;
#43129=CARTESIAN_POINT ( 'NONE',  ( 179.1040650366922193, 294.2007529456641919, 1.056493710678918729 ) ) ;
#43130=CARTESIAN_POINT ( 'NONE',  ( 41.66351307949141614, 184.8615022471902023, 5.000000000000051514 ) ) ;
#43131=CARTESIAN_POINT ( 'NONE',  ( 183.6907499062894260, 292.8494268563325136, 9.428801131153548454 ) ) ;
#43132=CARTESIAN_POINT ( 'NONE',  ( 163.2437751800324293, 247.9004826992694461, 9.806027032984305336 ) ) ;
#43133=CARTESIAN_POINT ( 'NONE',  ( -2.801652295722365071, 175.3149278399160949, -9.188101187500095079 ) ) ;
#43134=CARTESIAN_POINT ( 'NONE',  ( 167.5854134468545169, 285.9299511827676383, 4.087413415166947672 ) ) ;
#43139=CARTESIAN_POINT ( 'NONE',  ( 179.9113681451759135, 276.9646501146019659, 16.30242976572636238 ) ) ;
#43140=CARTESIAN_POINT ( 'NONE',  ( 193.7901930790854976, 294.9925349088783264, 14.24765323155741115 ) ) ;
#43141=FACE_OUTER_BOUND ( 'NONE', #35660, .T. ) ;
#43142=CARTESIAN_POINT ( 'NONE',  ( 141.9699493749754140, 259.7505386000626686, -7.968025677899344572 ) ) ;
#43147=CARTESIAN_POINT ( 'NONE',  ( 159.1565304511513546, 259.4205487488260360, 16.68562774920905056 ) ) ;
#43151=CARTESIAN_POINT ( 'NONE',  ( 156.3599523370786244, 276.2775748563693696, 10.27199958061185114 ) ) ;
#43153=CARTESIAN_POINT ( 'NONE',  ( 160.0166746459236435, 283.6086068001695253, 2.232576205374148248 ) ) ;
#43155=CARTESIAN_POINT ( 'NONE',  ( 192.8132846206021611, 296.6845899933152850, 11.53748932578252351 ) ) ;
#43156=CARTESIAN_POINT ( 'NONE',  ( 70.33802287992277513, 222.9637435831424739, 2.679491924311251605 ) ) ;
#43159=CARTESIAN_POINT ( 'NONE',  ( 124.0080952226617796, 235.7365022471901739, -10.00000000000009237 ) ) ;
#43161=ORIENTED_EDGE ( 'NONE', *, *, #72896, .F. ) ;
#43164=CARTESIAN_POINT ( 'NONE',  ( 153.4242699508872647, 264.9083646613370320, 16.62000820703435267 ) ) ;
#43165=VERTEX_POINT ( 'NONE', #66856 ) ;
#43166=CARTESIAN_POINT ( 'NONE',  ( 190.8443993347725325, 300.0947993426467519, 8.522468760355437212 ) ) ;
#43168=CARTESIAN_POINT ( 'NONE',  ( 174.3516257938615865, 262.5322562012714798, 15.40078459836708547 ) ) ;
#43169=VERTEX_POINT ( 'NONE', #97785 ) ;
#43175=CARTESIAN_POINT ( 'NONE',  ( 175.6563521628115438, 268.5095984484888731, 16.17594149762453171 ) ) ;
#43176=CARTESIAN_POINT ( 'NONE',  ( 168.8056409514728102, 275.8157205250771540, -15.38912072102792905 ) ) ;
#43177=B_SPLINE_CURVE_WITH_KNOTS ( 'NONE', 3,
 ( #70579, #17383, #63486, #85858, #16880, #24484, #94927, #17905, #16384, #26498, #32072, #39656, #1194, #62984 ),
 .UNSPECIFIED., .F., .F.,
 ( 4, 2, 2, 2, 2, 2, 4 ),
 ( 2.907926436840383405E-17, 0.0005042492132239927323, 0.001008498426447956408, 0.001260623033059940631, 0.001512747639671924637, 0.001764872246283908860, 0.002016996852895892867 ),
 .UNSPECIFIED. ) ;
#43179=ORIENTED_EDGE ( 'NONE', *, *, #917, .T. ) ;
#43180=CARTESIAN_POINT ( 'NONE',  ( 174.3697573357644899, 277.1653490889620457, -17.12727634137145571 ) ) ;
#43181=CARTESIAN_POINT ( 'NONE',  ( 169.8694959362524628, 262.1277198426760151, -15.72963479151413502 ) ) ;
#43184=B_SPLINE_CURVE_WITH_KNOTS ( 'NONE', 3,
 ( #74972, #51660, #28860, #22243, #28344, #61234 ),
 .UNSPECIFIED., .F., .F.,
 ( 4, 2, 4 ),
 ( 0.01996523517852847110, 0.02451540668050315036, 0.02906557818247782615 ),
 .UNSPECIFIED. ) ;
#43185=CARTESIAN_POINT ( 'NONE',  ( 160.3724000868533324, 268.8946452163862659, -16.80276685773084822 ) ) ;
#43186=ORIENTED_EDGE ( 'NONE', *, *, #12730, .T. ) ;
#43194=CARTESIAN_POINT ( 'NONE',  ( 157.2548874775783929, 258.6822847665750942, -16.83730550228635181 ) ) ;
#43195=CARTESIAN_POINT ( 'NONE',  ( 162.7898368507877933, 277.9903003075606875, -13.67957419982492162 ) ) ;
#43196=CARTESIAN_POINT ( 'NONE',  ( 197.2241483131352027, 289.0447499725873399, -16.69872125311100319 ) ) ;
#43200=CARTESIAN_POINT ( 'NONE',  ( 206.5117639185820906, 272.9581278627833285, 11.28485531511759099 ) ) ;
#43201=CARTESIAN_POINT ( 'NONE',  ( 149.4456112649506281, 271.7996036513546869, -12.95648166494593667 ) ) ;
#43202=CARTESIAN_POINT ( 'NONE',  ( 206.5280879940269756, 272.9298537347264642, 11.21709153681466731 ) ) ;
#43203=CARTESIAN_POINT ( 'NONE',  ( 198.2819808855875863, 287.2125302111982705, 18.53535247371401695 ) ) ;
#43204=EDGE_LOOP ( 'NONE', ( #54242, #96259, #327, #82523 ) ) ;
#43206=EDGE_LOOP ( 'NONE', ( #83400, #47770, #1584, #61013 ) ) ;
#43207=CARTESIAN_POINT ( 'NONE',  ( 147.2227856845451583, 275.6496504929807543, -2.633553040037199366 ) ) ;
#43208=CARTESIAN_POINT ( 'NONE',  ( 171.5754110937450889, 259.5470102351253558, -13.93953539574996725 ) ) ;
#43209=CARTESIAN_POINT ( 'NONE',  ( 164.2961018905060087, 247.3365041451504851, 7.253309886448856325 ) ) ;
#43211=B_SPLINE_CURVE_WITH_KNOTS ( 'NONE', 3,
 ( #50639, #57241, #35939, #11672 ),
 .UNSPECIFIED., .F., .F.,
 ( 4, 4 ),
 ( 0.001999640796707240990, 0.007335658808800400027 ),
 .UNSPECIFIED. ) ;
#43212=CARTESIAN_POINT ( 'NONE',  ( 160.1153909744335806, 253.3190030889627735, -14.69843286118399561 ) ) ;
#43213=CARTESIAN_POINT ( 'NONE',  ( 148.2043552425267876, 273.9495221473935089, -8.865305688972465958 ) ) ;
#43214=ORIENTED_EDGE ( 'NONE', *, *, #84637, .F. ) ;
#43215=CARTESIAN_POINT ( 'NONE',  ( 170.5758582599388262, 255.6247867453906224, -12.63526933594605950 ) ) ;
#43219=FACE_OUTER_BOUND ( 'NONE', #18471, .T. ) ;
#43220=CARTESIAN_POINT ( 'NONE',  ( 206.9377610035629118, 272.2202792677204002, 7.440532334334675646 ) ) ;
#43222=CARTESIAN_POINT ( 'NONE',  ( 23.81978131880152816, 197.8927522451419634, 2.944929066748280225E-16 ) ) ;
#43223=CARTESIAN_POINT ( 'NONE',  ( 105.9931361504627745, 225.8768266524159856, -9.188101187500093303 ) ) ;
#43224=CARTESIAN_POINT ( 'NONE',  ( 184.0101390881002033, 296.9595158201846630, -2.782362052833078359 ) ) ;
#43226=CARTESIAN_POINT ( 'NONE',  ( 157.2464636617698375, 258.2881309577184652, 18.14284729738657731 ) ) ;
#43228=CARTESIAN_POINT ( 'NONE',  ( 28.05084980986327281, 180.8768266524160140, -9.188101187500091527 ) ) ;
#43229=CARTESIAN_POINT ( 'NONE',  ( 175.8939073520130592, 252.7054158260212375, 5.280091837693253964 ) ) ;
#43234=CARTESIAN_POINT ( 'NONE',  ( 147.5539660880823192, 275.8630805544623286, -0.6031081523752792606 ) ) ;
#43236=CARTESIAN_POINT ( 'NONE',  ( 146.8358616138309571, 276.3198226421291679, 4.054088818585255716 ) ) ;
#43239=CARTESIAN_POINT ( 'NONE',  ( 179.3912532575458272, 287.9620500955485340, -12.67217938249804732 ) ) ;
#43240=CARTESIAN_POINT ( 'NONE',  ( 108.5224306304829582, 221.9155109091896350, 2.679491924311254714 ) ) ;
#43242=CARTESIAN_POINT ( 'NONE',  ( 50.26990084964904071, 190.6423013555410080, -4.594050593750043987 ) ) ;
#43243=CARTESIAN_POINT ( 'NONE',  ( 94.68952686182812783, 232.1427522451419065, 10.00000000000009237 ) ) ;
#43245=CARTESIAN_POINT ( 'NONE',  ( 194.7749398255589881, 266.3361531225978069, -7.673830273753635467 ) ) ;
#43246=CARTESIAN_POINT ( 'NONE',  ( 179.3989088880254030, 257.9931946406668430, -10.60009870068524052 ) ) ;
#43247=CARTESIAN_POINT ( 'NONE',  ( 207.8136982414359579, 270.7031114674828700, -0.9536989003868096004 ) ) ;
#43249=CARTESIAN_POINT ( 'NONE',  ( 6.102605256642664067, 165.1423013555410080, -4.594050593750043987 ) ) ;
#43250=CARTESIAN_POINT ( 'NONE',  ( 151.4376533647338476, 268.3492855237141725, -15.16853828792834236 ) ) ;
#43252=CARTESIAN_POINT ( 'NONE',  ( 192.6789561813392595, 296.9172536750198219, -11.84591848451790952 ) ) ;
#43254=CARTESIAN_POINT ( 'NONE',  ( 54.51857766514267212, 202.2833772461660828, -9.188101187500095079 ) ) ;
#43255=CARTESIAN_POINT ( 'NONE',  ( 207.5792673731680793, 271.1091576421853233, 2.359198794924813214 ) ) ;
#43260=CARTESIAN_POINT ( 'NONE',  ( 208.3152833949211526, 269.8343404973242059, 2.763633873278860342 ) ) ;
#43261=CARTESIAN_POINT ( 'NONE',  ( 1.898513289055925979, 165.2365022471902023, -10.00000000000009059 ) ) ;
#43263=CARTESIAN_POINT ( 'NONE',  ( 117.0346129529493311, 244.5024278399160949, -9.188101187500093303 ) ) ;
#43265=CARTESIAN_POINT ( 'NONE',  ( 164.2866824732684279, 246.0941142798005785, 1.717120327741293195 ) ) ;
#43268=CARTESIAN_POINT ( 'NONE',  ( 189.5210412211111191, 289.6957050120914801, 15.52021532872637266 ) ) ;
#43269=B_SPLINE_CURVE_WITH_KNOTS ( 'NONE', 3,
 ( #77025, #84674, #67943, #67433 ),
 .UNSPECIFIED., .F., .F.,
 ( 4, 4 ),
 ( 0.008266395780886143241, 0.01413511161970297005 ),
 .UNSPECIFIED. ) ;
#43270=CARTESIAN_POINT ( 'NONE',  ( 150.3208749327335738, 270.2836025087354415, -14.97713178109939847 ) ) ;
#43272=CARTESIAN_POINT ( 'NONE',  ( 190.8443993347725325, 300.0947993426467519, 8.522468760355437212 ) ) ;
#43273=CARTESIAN_POINT ( 'NONE',  ( 163.8785059224672409, 246.8010968042466118, 7.414532662353326309 ) ) ;
#43278=ORIENTED_EDGE ( 'NONE', *, *, #36387, .F. ) ;
#43281=CARTESIAN_POINT ( 'NONE',  ( 171.2611302217239029, 284.5690204168765831, -11.47485418152970560 ) ) ;
#43282=B_SPLINE_SURFACE_WITH_KNOTS ( 'NONE', 3, 1, ( 
 ( #41998, #89649 ),
 ( #72934, #12109 ),
 ( #51082, #3525 ),
 ( #11620, #81537 ),
 ( #34403, #65302 ),
 ( #26805, #88666 ),
 ( #19233, #50102 ),
 ( #81057, #73415 ),
 ( #65787, #42969 ),
 ( #73911, #20210 ),
 ( #52580, #68285 ),
 ( #67287, #21697 ),
 ( #66794, #83035 ),
 ( #5500, #97719 ),
 ( #68780, #29792 ),
 ( #44479, #75410 ),
 ( #45964, #5994 ),
 ( #60168, #99703 ),
 ( #60664, #21209 ),
 ( #13117, #59678 ),
 ( #74918, #75921 ),
 ( #28287, #91133 ),
 ( #36383, #98214 ),
 ( #5012, #28798 ),
 ( #30291, #84531 ),
 ( #14098, #35892 ),
 ( #61179, #92146 ),
 ( #84041, #22699 ),
 ( #43976, #90651 ),
 ( #22193, #98722 ),
 ( #36888, #13606 ),
 ( #52089, #67797 ),
 ( #83534, #29306 ),
 ( #44980, #6502 ) ),
 .UNSPECIFIED., .T., .F., .F.,
 ( 4, 2, 2, 2, 2, 2, 2, 2, 2, 2, 2, 2, 2, 2, 2, 2, 4 ),
 ( 2, 2 ),
 ( 0.000000000000000000, 0.06250000000000000000, 0.1250000000000000000, 0.1875000000000000000, 0.2500000000000000000, 0.3125000000000000000, 0.3750000000000000000, 0.4375000000000000000, 0.5000000000000000000, 0.5625000000000000000, 0.6250000000000000000, 0.6875000000000000000, 0.7500000000000000000, 0.8125000000000000000, 0.8750000000000000000, 0.9375000000000000000, 1.000000000000000000 ),
 ( 0.000000000000000000, 1.000000000000000000 ),
 .UNSPECIFIED. ) ;
#43284=CARTESIAN_POINT ( 'NONE',  ( 196.4164021072083983, 270.5621661862001019, 13.33908636140236936 ) ) ;
#43285=CARTESIAN_POINT ( 'NONE',  ( 185.2313369549983406, 296.3301568530737882, 4.659716315438352296 ) ) ;
#43297=DIRECTION ( 'NONE',  ( -0.8660254037844387076, -0.4999999999999998890, -0.000000000000000000 ) ) ;
#43298=CARTESIAN_POINT ( 'NONE',  ( 184.8651805647570256, 291.9995124747351838, 12.23147168373134264 ) ) ;
#43299=VECTOR ( 'NONE', #25242, 1000.000000000000000 ) ;
#43300=CARTESIAN_POINT ( 'NONE',  ( 164.4761815919938215, 245.7658921781788592, 6.833796894895563412 ) ) ;
#43303=CARTESIAN_POINT ( 'NONE',  ( 80.49933977867583224, 217.2833772461660544, -9.188101187500095079 ) ) ;
#43304=CARTESIAN_POINT ( 'NONE',  ( 203.3686379427449253, 278.4021817475232297, 14.97501784957458426 ) ) ;
#43307=ORIENTED_EDGE ( 'NONE', *, *, #60787, .T. ) ;
#43308=ORIENTED_EDGE ( 'NONE', *, *, #52337, .F. ) ;
#43309=EDGE_CURVE ( 'NONE', #99407, #63534, #95292, .T. ) ;
#43310=DIRECTION ( 'NONE',  ( -0.8660254037844359321, -0.5000000000000051070, -0.000000000000000000 ) ) ;
#43311=VERTEX_POINT ( 'NONE', #94690 ) ;
#43313=EDGE_LOOP ( 'NONE', ( #52259, #56003, #79386, #95557 ) ) ;
#43314=ADVANCED_FACE ( 'NONE', ( #49063 ), #72400, .F. ) ;
#43315=LINE ( 'NONE', #83360, #42743 ) ;
#43316=CARTESIAN_POINT ( 'NONE',  ( 155.0453531195792038, 262.1005662498678817, -18.46987289964740953 ) ) ;
#43317=ORIENTED_EDGE ( 'NONE', *, *, #27586, .T. ) ;
#43318=CARTESIAN_POINT ( 'NONE',  ( 207.5409781303276588, 271.1754765561682348, -7.231270017877110767 ) ) ;
#43323=CARTESIAN_POINT ( 'NONE',  ( 153.0308080659177392, 265.5898606369461277, -17.74682723936668438 ) ) ;
#43327=CARTESIAN_POINT ( 'NONE',  ( 140.8778087205959650, 242.9548013555409796, -4.594050593750042211 ) ) ;
#43328=CARTESIAN_POINT ( 'NONE',  ( 195.8767001660183951, 291.3785986239582826, -17.20508890422931003 ) ) ;
#43329=EDGE_LOOP ( 'NONE', ( #12441, #8536, #75743, #85430 ) ) ;
#43334=CARTESIAN_POINT ( 'NONE',  ( 200.0523276869015206, 270.2207466263407696, 9.267919080221707517 ) ) ;
#43335=ORIENTED_EDGE ( 'NONE', *, *, #92560, .F. ) ;
#43338=CARTESIAN_POINT ( 'NONE',  ( 161.1767284389501071, 281.8257712043616152, -6.166458447416498956 ) ) ;
#43343=ORIENTED_EDGE ( 'NONE', *, *, #80799, .F. ) ;
#43344=CARTESIAN_POINT ( 'NONE',  ( 184.6274781232527573, 272.9621770304452184, -16.38896422655171392 ) ) ;
#43349=CARTESIAN_POINT ( 'NONE',  ( 171.7367047606329038, 279.7472062399093602, -14.55191673240434902 ) ) ;
#43356=CARTESIAN_POINT ( 'NONE',  ( 203.5077069180501042, 269.8384169519572993, 5.656147133308556896 ) ) ;
#43357=ORIENTED_EDGE ( 'NONE', *, *, #56472, .T. ) ;
#43362=CARTESIAN_POINT ( 'NONE',  ( 175.6384468060905988, 290.9795127648189350, 2.794533193917200453 ) ) ;
#43364=AXIS2_PLACEMENT_3D ( 'NONE', #35901, #75935, #99218 ) ;
#43365=( BOUNDED_CURVE ( )  B_SPLINE_CURVE ( 2, ( #95726, #88628, #19196, #50066, #81024, #97204, #27769, #12577, #43453 ),
 .UNSPECIFIED., .F., .T. ) 
 B_SPLINE_CURVE_WITH_KNOTS ( ( 3, 2, 2, 2, 3 ),
 ( 0.7862903225806451291, 0.7876344086021505042, 0.7903225806451612545, 0.7930107526881720048, 0.7943548387096773800 ),
 .UNSPECIFIED. ) 
 CURVE ( )  GEOMETRIC_REPRESENTATION_ITEM ( )  RATIONAL_B_SPLINE_CURVE ( ( 0.9330127018922194093, 0.9330127018922194093, 1.000000000000000000, 0.8660254037844387076, 1.000000000000000000, 0.8660254037844387076, 1.000000000000000000, 0.9330127018922194093, 0.9330127018922194093 ) ) 
 REPRESENTATION_ITEM ( '' )  );
#43366=LINE ( 'NONE', #96626, #46487 ) ;
#43368=CARTESIAN_POINT ( 'NONE',  ( 2.557053438076354990, 172.2833772461660828, -9.188101187500095079 ) ) ;
#43369=CARTESIAN_POINT ( 'NONE',  ( 107.1028179730028285, 223.4548013555409796, -4.594050593750042211 ) ) ;
#43371=CARTESIAN_POINT ( 'NONE',  ( 184.9305274905498493, 294.8224435932747838, -7.698895662769760229 ) ) ;
#43373=VECTOR ( 'NONE', #69513, 1000.000000000000000 ) ;
#43374=EDGE_CURVE ( 'NONE', #9838, #77732, #22750, .T. ) ;
#43376=B_SPLINE_CURVE_WITH_KNOTS ( 'NONE', 3,
 ( #85694, #40008, #70948, #15214 ),
 .UNSPECIFIED., .F., .F.,
 ( 4, 4 ),
 ( 0.01311470161809044112, 0.02170404453345711054 ),
 .UNSPECIFIED. ) ;
#43377=CARTESIAN_POINT ( 'NONE',  ( 154.8556227199321427, 262.4291889417971788, 17.77326384500479861 ) ) ;
#43378=CARTESIAN_POINT ( 'NONE',  ( 194.5298665426430489, 293.7113828889860656, -16.13302716640051315 ) ) ;
#43380=CARTESIAN_POINT ( 'NONE',  ( 196.4695417320205024, 266.7097263680378205, 8.121914006708831124 ) ) ;
#43381=CARTESIAN_POINT ( 'NONE',  ( 79.69646206235792363, 223.4865022471902591, -10.00000000000009592 ) ) ;
#43382=CARTESIAN_POINT ( 'NONE',  ( 181.5716216444320992, 267.3631569497555915, -14.78134104179376784 ) ) ;
#43386=CARTESIAN_POINT ( 'NONE',  ( 81.52757139778736928, 224.0024278399160949, 9.188101187500095079 ) ) ;
#43388=CARTESIAN_POINT ( 'NONE',  ( 191.4922467593309250, 298.9726946877590876, 7.604184559945784017 ) ) ;
#43390=CARTESIAN_POINT ( 'NONE',  ( 157.8562613713738472, 257.2319303423452652, 17.81420683562559404 ) ) ;
#43392=CARTESIAN_POINT ( 'NONE',  ( 196.9726513669839107, 289.4803554612698235, 16.57669625517693746 ) ) ;
#43393=CARTESIAN_POINT ( 'NONE',  ( 198.9369963555428740, 286.0780101374919013, -18.58432392708837710 ) ) ;
#43394=CARTESIAN_POINT ( 'NONE',  ( 173.1825648917232172, 268.0947487749845095, -16.28828717342791421 ) ) ;
#43396=CARTESIAN_POINT ( 'NONE',  ( 193.1977289678065404, 296.0187128512746995, -12.37159405312863925 ) ) ;
#43397=CARTESIAN_POINT ( 'NONE',  ( -27.42236680055714260, 166.5217562850347406, 1.224646799147364892E-15 ) ) ;
#43398=VERTEX_POINT ( 'NONE', #31711 ) ;
#43401=CARTESIAN_POINT ( 'NONE',  ( 146.8153075009282134, 276.3554234099810287, -4.113808735271278216 ) ) ;
#43402=CARTESIAN_POINT ( 'NONE',  ( 191.7535527499152579, 287.9627823321743563, -15.84076656666959160 ) ) ;
#43405=FACE_OUTER_BOUND ( 'NONE', #9253, .T. ) ;
#43406=CARTESIAN_POINT ( 'NONE',  ( 157.7704454140505277, 268.4375085597957309, 16.01069904446985603 ) ) ;
#43409=CARTESIAN_POINT ( 'NONE',  ( 145.5865615336240353, 244.8615022471901739, 5.000000000000051514 ) ) ;
#43410=CARTESIAN_POINT ( 'NONE',  ( 157.8159121039657293, 257.3018173235443555, -17.05074702406642118 ) ) ;
#43413=CARTESIAN_POINT ( 'NONE',  ( 190.1016529815521210, 299.5590995676359967, -6.615970321355634454 ) ) ;
#43414=AXIS2_PLACEMENT_3D ( 'NONE', #15287, #116, #21907 ) ;
#43415=CARTESIAN_POINT ( 'NONE',  ( 167.5388416099013966, 248.0610247611899695, -1.869801589506421724 ) ) ;
#43417=CARTESIAN_POINT ( 'NONE',  ( 196.8310340268163543, 265.3144059923225768, -4.523882790829159894 ) ) ;
#43423=CARTESIAN_POINT ( 'NONE',  ( 192.8339539104745768, 292.5331237600439636, 15.31903378033653773 ) ) ;
#43424=CARTESIAN_POINT ( 'NONE',  ( 158.3813060601511893, 256.3225262651385492, 16.44677913423000959 ) ) ;
#43426=CARTESIAN_POINT ( 'NONE',  ( 204.4652362847643303, 273.3276312005621094, 10.91026480097475293 ) ) ;
#43427=CARTESIAN_POINT ( 'NONE',  ( 192.5395560493205949, 296.4429067975564180, -11.74828324584324868 ) ) ;
#43428=VECTOR ( 'NONE', #52317, 1000.000000000000000 ) ;
#43432=EDGE_CURVE ( 'NONE', #73019, #39791, #17720, .T. ) ;
#43433=CARTESIAN_POINT ( 'NONE',  ( 164.0653621983113339, 275.4287311911768370, 15.31700800437514864 ) ) ;
#43440=CARTESIAN_POINT ( 'NONE',  ( 165.9755981782961953, 274.1598679360748179, -15.15796544636562260 ) ) ;
#43442=CARTESIAN_POINT ( 'NONE',  ( 193.9495889092963807, 294.7164532324382549, 15.46986001312306058 ) ) ;
#43443=CARTESIAN_POINT ( 'NONE',  ( 186.6970606014003522, 295.2539764206142081, -10.47640868448896434 ) ) ;
#43446=CARTESIAN_POINT ( 'NONE',  ( 170.8091510057469691, 288.1825902081931190, -4.081328050745901770 ) ) ;
#43447=EDGE_CURVE ( 'NONE', #11106, #30511, #30976, .T. ) ;
#43449=CARTESIAN_POINT ( 'NONE',  ( 180.5366697149694062, 256.7075445286905619, 4.926626485048444692 ) ) ;
#43450=CARTESIAN_POINT ( 'NONE',  ( 92.65049840370248546, 233.4869531367911293, 4.594050593750046652 ) ) ;
#43451=ORIENTED_EDGE ( 'NONE', *, *, #20031, .T. ) ;
#43453=CARTESIAN_POINT ( 'NONE',  ( 110.3297989853572005, 246.0530062829863311, -4.648177544792955347E-16 ) ) ;
#43457=CARTESIAN_POINT ( 'NONE',  ( 179.5498935473132747, 293.3807426002626357, -2.640407830033155268 ) ) ;
#43458=CARTESIAN_POINT ( 'NONE',  ( 157.8763546842245376, 257.1971277035954699, 17.68444922773363004 ) ) ;
#43459=CARTESIAN_POINT ( 'NONE',  ( 160.0061168334508750, 253.5082714530983026, -16.02306982074888708 ) ) ;
#43460=CARTESIAN_POINT ( 'NONE',  ( 162.8491774010308575, 248.5839461010540390, 10.21539626359008146 ) ) ;
#43461=ORIENTED_EDGE ( 'NONE', *, *, #90057, .T. ) ;
#43462=EDGE_LOOP ( 'NONE', ( #49927, #22992, #6815, #56776, #4711 ) ) ;
#43463=CARTESIAN_POINT ( 'NONE',  ( 207.9743173328493526, 270.4249110404894054, -2.481515874287090639 ) ) ;
#43465=CARTESIAN_POINT ( 'NONE',  ( 191.3753129921931873, 263.8116507527752788, -8.027821554704329898 ) ) ;
#43468=CARTESIAN_POINT ( 'NONE',  ( 131.6216415740022398, 255.9869531367911009, 4.594050593750046652 ) ) ;
#43469=CARTESIAN_POINT ( 'NONE',  ( 198.7045056313791633, 284.4806958840320021, 17.79791830837532274 ) ) ;
#43472=CARTESIAN_POINT ( 'NONE',  ( 146.8729474948188454, 276.2555880120147549, 3.934020695290606273 ) ) ;
#43474=CARTESIAN_POINT ( 'NONE',  ( 206.6268150440956504, 272.7588534679261443, -10.76664753678610609 ) ) ;
#43475=CARTESIAN_POINT ( 'NONE',  ( 173.2003599206826436, 251.6178260009447456, -0.2735355138943916242 ) ) ;
#43476=CARTESIAN_POINT ( 'NONE',  ( 178.4715894149740052, 285.3467937416216955, 13.10955772305596945 ) ) ;
#43478=CARTESIAN_POINT ( 'NONE',  ( 199.0630536459244411, 281.9549554678117715, -16.62110652460417626 ) ) ;
#43479=CARTESIAN_POINT ( 'NONE',  ( 147.4935738007826842, 244.4155109091896065, 2.679491924311254714 ) ) ;
#43480=CARTESIAN_POINT ( 'NONE',  ( 185.9608592076092464, 288.5956984647530703, 15.36535719480430018 ) ) ;
#43483=CARTESIAN_POINT ( 'NONE',  ( 57.33281313167710636, 216.1589784336661921, -6.496448406907675876E-16 ) ) ;
#43486=CARTESIAN_POINT ( 'NONE',  ( 162.6757594134126350, 248.8843148665554281, -10.86406770146305867 ) ) ;
#43488=CARTESIAN_POINT ( 'NONE',  ( 191.1363710586135198, 294.8022764895544583, 13.34403287223599222 ) ) ;
#43491=AXIS2_PLACEMENT_3D ( 'NONE', #5565, #74500, #97790 ) ;
#43492=CARTESIAN_POINT ( 'NONE',  ( 156.6812872898450735, 261.2670451491295012, 0.000000000000000000 ) ) ;
#43494=CARTESIAN_POINT ( 'NONE',  ( 161.8385268298191306, 255.1149155613134951, 15.97321096069992308 ) ) ;
#43500=CARTESIAN_POINT ( 'NONE',  ( 207.1019571622349815, 271.9358831784929293, -5.989975140547304733 ) ) ;
#43502=CARTESIAN_POINT ( 'NONE',  ( 15.00651571324267763, 167.2202760586659736, -5.415160957724236172E-17 ) ) ;
#43503=B_SPLINE_CURVE_WITH_KNOTS ( 'NONE', 3,
 ( #23576, #54986, #54467, #40274 ),
 .UNSPECIFIED., .F., .F.,
 ( 4, 4 ),
 ( 0.01796415739704124506, 0.02693908509615394742 ),
 .UNSPECIFIED. ) ;
#43504=CARTESIAN_POINT ( 'NONE',  ( 207.2586958963831023, 270.9687488091540217, 3.100303027002558665 ) ) ;
#43505=ORIENTED_EDGE ( 'NONE', *, *, #60920, .T. ) ;
#43509=CARTESIAN_POINT ( 'NONE',  ( 164.3545367017254364, 245.9765873086048487, -5.942639963102972267 ) ) ;
#43511=CARTESIAN_POINT ( 'NONE',  ( 59.22776434610305785, 198.8768266524159571, -9.188101187500093303 ) ) ;
#43512=CARTESIAN_POINT ( 'NONE',  ( 161.5056331467593225, 250.9110330116698435, 14.52719814064025528 ) ) ;
#43513=CARTESIAN_POINT ( 'NONE',  ( 151.1126408083691501, 268.9122237844355254, -15.82705194100464396 ) ) ;
#43514=CARTESIAN_POINT ( 'NONE',  ( 147.3984236761635884, 275.3454365677582700, 5.108566646342994844 ) ) ;
#43516=CARTESIAN_POINT ( 'NONE',  ( 202.8423703034144694, 269.9731342184576874, -6.433654896179251459 ) ) ;
#43517=CARTESIAN_POINT ( 'NONE',  ( 146.5310397537613483, 276.8477895910274356, -0.2793038414862049068 ) ) ;
#43518=CARTESIAN_POINT ( 'NONE',  ( 179.6700249023918730, 276.7835841873084064, 16.30426102577613534 ) ) ;
#43521=PRODUCT ( 'Lead Screw Acme Drive Shaft', 'Lead Screw Acme Drive Shaft', '', ( #69448 ) ) ;
#43522=CARTESIAN_POINT ( 'NONE',  ( 167.0324277405701139, 257.7922078709543143, -15.65539679637635651 ) ) ;
#43523=EDGE_CURVE ( 'NONE', #80622, #75397, #50362, .T. ) ;
#43525=CARTESIAN_POINT ( 'NONE',  ( 102.3574601280508176, 223.2365022471902023, 10.00000000000009592 ) ) ;
#43528=ORIENTED_EDGE ( 'NONE', *, *, #15045, .F. ) ;
#43529=CARTESIAN_POINT ( 'NONE',  ( 52.13666070897046012, 213.1589784336661637, -6.496448406907675876E-16 ) ) ;
#43531=CARTESIAN_POINT ( 'NONE',  ( 192.5076277540105423, 297.2140032159341558, -13.10094381206144298 ) ) ;
#43532=CARTESIAN_POINT ( 'NONE',  ( 147.2443490232117256, 275.6123016948292275, 5.226063659459642352 ) ) ;
#43533=CARTESIAN_POINT ( 'NONE',  ( -17.42236680055705023, 149.2012482093457777, 0.000000000000000000 ) ) ;
#43534=VERTEX_POINT ( 'NONE', #97561 ) ;
#43535=CARTESIAN_POINT ( 'NONE',  ( 70.24235140437789937, 201.3615022471901739, 5.000000000000051514 ) ) ;
#43536=CARTESIAN_POINT ( 'NONE',  ( 206.9026071836525205, 272.2811674698855313, 7.240992997279449561 ) ) ;
#43537=CARTESIAN_POINT ( 'NONE',  ( 162.0192538899617318, 268.0510789565263394, -17.53028463913764057 ) ) ;
#43541=CARTESIAN_POINT ( 'NONE',  ( 157.4725523017146429, 257.8965339463198916, 17.43710027717953892 ) ) ;
#43547=EDGE_CURVE ( 'NONE', #44921, #93452, #96349, .T. ) ;
#43549=CARTESIAN_POINT ( 'NONE',  ( 182.4419837166206548, 284.0818805488852377, 15.00679419155397554 ) ) ;
#43550=CARTESIAN_POINT ( 'NONE',  ( 151.4327733764141612, 268.3577379114237829, 14.90862905801242100 ) ) ;
#43551=CARTESIAN_POINT ( 'NONE',  ( 206.2809287719926488, 273.3579460648492159, -10.70911012174624588 ) ) ;
#43553=VERTEX_POINT ( 'NONE', #89969 ) ;
#43555=CARTESIAN_POINT ( 'NONE',  ( 161.3773209892555371, 251.1332761876949746, -14.50043705923759241 ) ) ;
#43557=DIRECTION ( 'NONE',  ( 0.5000000000000048850, -0.8660254037844358210, 0.000000000000000000 ) ) ;
#43560=CARTESIAN_POINT ( 'NONE',  ( 159.2303255284352304, 254.8519814094557603, 16.39103317446447150 ) ) ;
#43564=CARTESIAN_POINT ( 'NONE',  ( 126.2364799639240402, 237.5643266524160140, 9.188101187500095079 ) ) ;
#43566=EDGE_CURVE ( 'NONE', #53916, #22854, #58780, .T. ) ;
#43569=AXIS2_PLACEMENT_3D ( 'NONE', #13484, #44356, #97600 ) ;
#43570=CARTESIAN_POINT ( 'NONE',  ( 201.5099656766716976, 280.8415660465722112, 16.32132609628684605 ) ) ;
#43572=EDGE_LOOP ( 'NONE', ( #93678, #31383, #18507, #46381 ) ) ;
#43576=ADVANCED_FACE ( 'NONE', ( #58519 ), #18185, .F. ) ;
#43577=CARTESIAN_POINT ( 'NONE',  ( 76.33141897508073725, 221.0024278399160949, 9.188101187500095079 ) ) ;
#43580=CARTESIAN_POINT ( 'NONE',  ( 198.7430995078048284, 286.4138493292020371, 18.01120443222870193 ) ) ;
#43581=CARTESIAN_POINT ( 'NONE',  ( 173.9825871881620571, 277.6148033471986878, 15.53242809676506830 ) ) ;
#43585=CARTESIAN_POINT ( 'NONE',  ( 152.9251141908703175, 265.7729277985770864, -16.20110192949203309 ) ) ;
#43588=CARTESIAN_POINT ( 'NONE',  ( 206.9395787313233939, 270.0782334019143605, 3.375702725593451969 ) ) ;
#43589=CARTESIAN_POINT ( 'NONE',  ( 207.8232941427535536, 270.6864908788566026, -6.505149060073906142 ) ) ;
#43590=CARTESIAN_POINT ( 'NONE',  ( 174.8967126845354869, 253.3500105558054827, -7.849478773564977807 ) ) ;
#43592=B_SPLINE_CURVE_WITH_KNOTS ( 'NONE', 3,
 ( #570, #8668, #79, #30466, #15247, #62345, #53747, #94308, #76577, #39538, #69464, #30961, #61358, #61850, #92798, #70986, #40046, #31953, #1589, #62856, #32471, #54238, #93812, #24372, #7159, #16761, #47650, #78587, #63368, #24860, #55735, #17262, #2586, #72498, #40552, #3584, #33472, #96302, #56253, #49177, #65362, #71980, #80112, #87247, #34464, #26871, #88226, #50163, #10676, #33990, #26375, #42057, #48681, #57253 ),
 .UNSPECIFIED., .F., .F.,
 ( 4, 2, 2, 2, 2, 2, 2, 2, 2, 2, 2, 2, 2, 2, 2, 2, 2, 2, 2, 2, 2, 2, 2, 2, 2, 2, 4 ),
 ( 0.0008417762867302816879, 0.001328145691676835142, 0.001814515096623388595, 0.002057699799096665214, 0.002300884501569942266, 0.002422476852806596838, 0.002544069204043251410, 0.002665661555279905982, 0.002787253906516560555, 0.003030438608989949496, 0.003273623311463338438, 0.003759992716410036958, 0.004732731526303299123, 0.005705470336196561722, 0.006191839741143153122, 0.006435024443616449256, 0.006678209146089744523, 0.006739005321708050125, 0.006799801497326356595, 0.006860597672944663064, 0.006921393848562969534, 0.007042986199799565993, 0.007164578551036161584, 0.007407763253509473331, 0.007650947955982785945, 0.008137317360929409438, 0.008623686765876034666 ),
 .UNSPECIFIED. ) ;
#43594=CARTESIAN_POINT ( 'NONE',  ( 9.458193372709686741, 166.2677522451418213, -5.000000000000041744 ) ) ;
#43595=CARTESIAN_POINT ( 'NONE',  ( 131.1618259000655371, 246.5333772461660544, 9.188101187500095079 ) ) ;
#43599=CARTESIAN_POINT ( 'NONE',  ( 202.9490938173916561, 279.1288534886517709, -16.56031645010252973 ) ) ;
#43600=B_SPLINE_CURVE_WITH_KNOTS ( 'NONE', 3,
 ( #1278, #77270, #39732, #46867 ),
 .UNSPECIFIED., .F., .F.,
 ( 4, 4 ),
 ( 0.000000000000000000, 0.001628043935741951614 ),
 .UNSPECIFIED. ) ;
#43601=CARTESIAN_POINT ( 'NONE',  ( 204.2556901454867955, 276.8657622634082713, 13.61111001399713949 ) ) ;
#43604=ORIENTED_EDGE ( 'NONE', *, *, #49962, .T. ) ;
#43606=CARTESIAN_POINT ( 'NONE',  ( 182.3261756823741564, 275.2222332755986827, -16.67497698087158753 ) ) ;
#43608=CARTESIAN_POINT ( 'NONE',  ( 38.49039832772786696, 181.4824982072973683, 3.021315404115420679E-15 ) ) ;
#43610=CARTESIAN_POINT ( 'NONE',  ( 195.7820092358261093, 263.4657121749461339, 0.8738221391051791409 ) ) ;
#43611=CARTESIAN_POINT ( 'NONE',  ( 28.67313202272483252, 177.3615022471902023, 5.000000000000051514 ) ) ;
#43613=B_SPLINE_CURVE_WITH_KNOTS ( 'NONE', 3,
 ( #39898, #14631, #45512, #69323 ),
 .UNSPECIFIED., .F., .F.,
 ( 4, 4 ),
 ( 0.000000000000000000, 0.007933777700369805050 ),
 .UNSPECIFIED. ) ;
#43614=CARTESIAN_POINT ( 'NONE',  ( 192.9666104369811990, 268.2690024003410372, 12.61864968089833638 ) ) ;
#43616=CARTESIAN_POINT ( 'NONE',  ( 148.9498507103374152, 272.6582861203333437, 11.90061892622094852 ) ) ;
#43617=CARTESIAN_POINT ( 'NONE',  ( 71.24263041127305485, 223.4860189848785410, -2.679491924311252493 ) ) ;
#43618=LINE ( 'NONE', #5135, #51501 ) ;
#43619=FACE_OUTER_BOUND ( 'NONE', #93995, .T. ) ;
#43621=CARTESIAN_POINT ( 'NONE',  ( 140.7332108297008801, 245.3927522451417929, -10.00000000000009059 ) ) ;
#43622=CARTESIAN_POINT ( 'NONE',  ( 175.9939695555370065, 285.4482173679398898, -11.95632612277833040 ) ) ;
#43624=EDGE_CURVE ( 'NONE', #56647, #74262, #53930, .T. ) ;
#43627=CARTESIAN_POINT ( 'NONE',  ( 150.9363692955544991, 269.2175350005573478, -14.27857383982596140 ) ) ;
#43628=CARTESIAN_POINT ( 'NONE',  ( -6.076397627723526540, 176.4869531367911293, 4.594050593750046652 ) ) ;
#43629=CARTESIAN_POINT ( 'NONE',  ( 63.26028190641562787, 198.1423013555410080, -4.594050593750043987 ) ) ;
#43630=CARTESIAN_POINT ( 'NONE',  ( 178.6427318236586359, 259.2647235818225226, -10.45271603834399876 ) ) ;
#43633=CARTESIAN_POINT ( 'NONE',  ( 204.6475128369918082, 276.1871054541632020, -13.72068618491070779 ) ) ;
#43634=CARTESIAN_POINT ( 'NONE',  ( 190.8458701802819064, 291.3353758386331833, -14.35470056613957723 ) ) ;
#43635=CARTESIAN_POINT ( 'NONE',  ( 148.9635810001525726, 275.9368111177387846, 3.718913479852709703 ) ) ;
#43636=CARTESIAN_POINT ( 'NONE',  ( 167.3905708005187591, 256.8461950526155988, 14.46083098827760693 ) ) ;
#43639=CARTESIAN_POINT ( 'NONE',  ( 150.2494575935072874, 270.4073009688167986, 14.61449051812962985 ) ) ;
#43642=CARTESIAN_POINT ( 'NONE',  ( 62.44812277031795134, 196.8615022471901739, 5.000000000000051514 ) ) ;
#43643=CARTESIAN_POINT ( 'NONE',  ( 182.4321081115337222, 291.9834752246442235, 9.344615119188279806 ) ) ;
#43644=CARTESIAN_POINT ( 'NONE',  ( 189.8480911035503880, 301.8204558191226283, -0.8992086515915015399 ) ) ;
#43645=CARTESIAN_POINT ( 'NONE',  ( 23.01690360248371903, 184.0958772461660544, -9.188101187500095079 ) ) ;
#43646=CARTESIAN_POINT ( 'NONE',  ( 168.2447061861834072, 286.2798532801800775, 4.135845175375446381 ) ) ;
#43647=CARTESIAN_POINT ( 'NONE',  ( 192.4454213697443095, 297.3217478340386606, 12.58566886711101596 ) ) ;
#43649=CARTESIAN_POINT ( 'NONE',  ( 144.1251436611898953, 244.0177522451417644, 5.000000000000051514 ) ) ;
#43650=CARTESIAN_POINT ( 'NONE',  ( 180.4127669783307795, 277.2432443295738267, 16.31949751863770359 ) ) ;
#43652=CARTESIAN_POINT ( 'NONE',  ( 114.3892930691446850, 248.3967562850347122, -4.648177544792955347E-16 ) ) ;
#43657=CARTESIAN_POINT ( 'NONE',  ( 201.5232667746729760, 270.7243246684459450, 10.73244273373618718 ) ) ;
#43658=CARTESIAN_POINT ( 'NONE',  ( 185.6872253078315964, 257.5179133167785608, -1.638249339750624589 ) ) ;
#43659=CARTESIAN_POINT ( 'NONE',  ( 191.2663728242109187, 269.6285576558835260, -14.72094365787478232 ) ) ;
#43661=CARTESIAN_POINT ( 'NONE',  ( 181.7743748161887822, 289.6841531283870381, 12.89587171145656974 ) ) ;
#43662=CARTESIAN_POINT ( 'NONE',  ( 156.7717313778066455, 276.4859198570546255, 10.27056923680294354 ) ) ;
#43665=ORIENTED_EDGE ( 'NONE', *, *, #47299, .T. ) ;
#43666=( BOUNDED_CURVE ( )  B_SPLINE_CURVE ( 2, ( #53757, #51801, #68471, #46153, #84230, #83725, #98407, #84716, #14283 ),
 .UNSPECIFIED., .F., .T. ) 
 B_SPLINE_CURVE_WITH_KNOTS ( ( 3, 2, 2, 2, 3 ),
 ( 0.3830645161290322509, 0.3844086021505376261, 0.3870967741935483764, 0.3897849462365591267, 0.3911290322580645018 ),
 .UNSPECIFIED. ) 
 CURVE ( )  GEOMETRIC_REPRESENTATION_ITEM ( )  RATIONAL_B_SPLINE_CURVE ( ( 0.9330127018922194093, 0.9330127018922194093, 1.000000000000000000, 0.8660254037844387076, 1.000000000000000000, 0.8660254037844387076, 1.000000000000000000, 0.9330127018922194093, 0.9330127018922194093 ) ) 
 REPRESENTATION_ITEM ( '' )  );
#43667=CARTESIAN_POINT ( 'NONE',  ( 152.6364317663293946, 268.0951475544519553, 15.85731527355114778 ) ) ;
#43669=CARTESIAN_POINT ( 'NONE',  ( 176.6558404752379090, 252.2237374370411942, -0.2705739152901737166 ) ) ;
#43670=CARTESIAN_POINT ( 'NONE',  ( 154.9048824156581361, 262.3438686460345366, -17.40627786727128168 ) ) ;
#43672=VERTEX_POINT ( 'NONE', #12399 ) ;
#43673=EDGE_CURVE ( 'NONE', #4704, #35604, #76910, .T. ) ;
#43675=CARTESIAN_POINT ( 'NONE',  ( 204.4781092559247782, 276.4805210635553863, 13.30606382016679490 ) ) ;
#43676=CARTESIAN_POINT ( 'NONE',  ( 152.6615646578087819, 266.2294089801508221, 16.94722993326405813 ) ) ;
#43678=CARTESIAN_POINT ( 'NONE',  ( 194.3452430042056847, 293.4673175397701357, -14.50972866970454866 ) ) ;
#43680=CARTESIAN_POINT ( 'NONE',  ( 174.4937798827906192, 262.3286410478639823, 14.41242922277202965 ) ) ;
#43682=DIRECTION ( 'NONE',  ( -0.8660254037844387076, -0.4999999999999998890, -0.000000000000000000 ) ) ;
#43685=EDGE_LOOP ( 'NONE', ( #1312, #97512, #97271, #37971, #82875 ) ) ;
#43686=CARTESIAN_POINT ( 'NONE',  ( 165.0565241268390366, 244.7607094220335568, 2.191926263411719589 ) ) ;
#43687=EDGE_CURVE ( 'NONE', #47416, #7762, #18996, .T. ) ;
#43688=CARTESIAN_POINT ( 'NONE',  ( 151.1866278134736206, 275.4563625138778207, -8.238537655447901287 ) ) ;
#43690=CARTESIAN_POINT ( 'NONE',  ( 177.6370681238493603, 279.4364947633008569, -16.61177670297263376 ) ) ;
#43691=CARTESIAN_POINT ( 'NONE',  ( 169.0811126367664485, 261.3667313283961562, -16.44051657199686289 ) ) ;
#43695=CARTESIAN_POINT ( 'NONE',  ( 157.4694053559891529, 268.9764842683514985, 15.59267564261065431 ) ) ;
#43697=CARTESIAN_POINT ( 'NONE',  ( 156.6075427607332244, 266.5381846890032875, -16.22512947928903415 ) ) ;
#43698=CARTESIAN_POINT ( 'NONE',  ( 190.1752790837055045, 301.2537496138681945, -5.177773110520776711 ) ) ;
#43700=CARTESIAN_POINT ( 'NONE',  ( 148.9230895364621574, 272.7046378331555161, 12.20434325797056019 ) ) ;
#43701=CARTESIAN_POINT ( 'NONE',  ( 192.8323852661406761, 296.6515067047851062, 11.86505947732313615 ) ) ;
#43704=CARTESIAN_POINT ( 'NONE',  ( 158.8123895076641077, 255.5758678317443469, -17.62141936352351479 ) ) ;
#43708=CARTESIAN_POINT ( 'NONE',  ( 206.2456893945931142, 273.4189824569319285, 10.13882547285618152 ) ) ;
#43709=CARTESIAN_POINT ( 'NONE',  ( 159.8655504377736918, 253.7517395922482706, 15.51368179719542262 ) ) ;
#43710=CARTESIAN_POINT ( 'NONE',  ( 206.3023480738090996, 271.3208467458289874, 7.632938913807082670 ) ) ;
#43711=CARTESIAN_POINT ( 'NONE',  ( 176.8206666507760474, 289.6423215265738804, -9.013642675727712827 ) ) ;
#43715=CARTESIAN_POINT ( 'NONE',  ( 198.6774775476553714, 286.5275098982731379, -17.42299212369177752 ) ) ;
#43716=CARTESIAN_POINT ( 'NONE',  ( 99.75938391669748739, 221.7365022471902023, 10.00000000000009948 ) ) ;
#43720=CARTESIAN_POINT ( 'NONE',  ( 205.6720057621449484, 274.0264657029327964, 10.42642860073514299 ) ) ;
#43721=CARTESIAN_POINT ( 'NONE',  ( 200.9521687275011175, 282.5876292032514243, -18.16013154125647944 ) ) ;
#43722=CARTESIAN_POINT ( 'NONE',  ( 164.3524132573224392, 245.9802652221976587, -2.749586949851067441 ) ) ;
#43724=CARTESIAN_POINT ( 'NONE',  ( 41.86197723097744472, 181.6427522451417644, 1.119607411625061291E-15 ) ) ;
#43725=CARTESIAN_POINT ( 'NONE',  ( 106.6962611473900893, 244.6589784336661069, -6.496448406907676862E-16 ) ) ;
#43726=CARTESIAN_POINT ( 'NONE',  ( 180.8261506122944979, 294.1084290502871568, -2.669056545970062810 ) ) ;
#43727=CARTESIAN_POINT ( 'NONE',  ( 167.9232164608807807, 282.0145233034614876, -10.83756476677490710 ) ) ;
#43729=CARTESIAN_POINT ( 'NONE',  ( 208.3490404761574553, 269.7758715175073689, 2.423947743236856578 ) ) ;
#43730=CARTESIAN_POINT ( 'NONE',  ( 32.46173284068399312, 198.7369531367911293, -4.594050593750048428 ) ) ;
#43733=ORIENTED_EDGE ( 'NONE', *, *, #77679, .F. ) ;
#43734=CARTESIAN_POINT ( 'NONE',  ( 191.3941823605357229, 298.7337486089482468, 7.883234235473491225 ) ) ;
#43736=CYLINDRICAL_SURFACE ( 'NONE', #15812, 10.00000000000010658 ) ;
#43737=CARTESIAN_POINT ( 'NONE',  ( 190.3791419447713906, 300.9006487807255326, -5.688668718458480988 ) ) ;
#43738=CARTESIAN_POINT ( 'NONE',  ( 106.0403798229140477, 220.4824982072973683, 3.021315404115420679E-15 ) ) ;
#43739=CARTESIAN_POINT ( 'NONE',  ( 161.8839333999304415, 250.2557977526613229, -13.90128376743482441 ) ) ;
#43741=CARTESIAN_POINT ( 'NONE',  ( 164.2609264239344213, 250.0470742514019378, 10.21728485584155699 ) ) ;
#43742=CARTESIAN_POINT ( 'NONE',  ( 92.59663213601572807, 234.2677522451419065, -5.000000000000047962 ) ) ;
#43744=CARTESIAN_POINT ( 'NONE',  ( 197.6218578199255376, 267.6909935936381544, -7.901084308168314863 ) ) ;
#43746=CARTESIAN_POINT ( 'NONE',  ( 162.8042930031641049, 248.6616881586264469, 11.14389129512055554 ) ) ;
#43747=CARTESIAN_POINT ( 'NONE',  ( 207.5959034698703078, 271.0803430774575418, -1.830000129038042544 ) ) ;
#43748=CARTESIAN_POINT ( 'NONE',  ( 19.71535529843806245, 176.0643266524160424, 9.188101187500095079 ) ) ;
#43753=CARTESIAN_POINT ( 'NONE',  ( 207.5195222358739784, 271.2126392554839640, 2.810970398613041432 ) ) ;
#43754=CARTESIAN_POINT ( 'NONE',  ( 203.6857291523390074, 276.2442838610515423, 13.33094155839203587 ) ) ;
#43757=CARTESIAN_POINT ( 'NONE',  ( 207.4764081617721843, 271.2873150223495600, 6.359972247200924578 ) ) ;
#43758=ORIENTED_EDGE ( 'NONE', *, *, #8741, .F. ) ;
#43761=CARTESIAN_POINT ( 'NONE',  ( 164.4989226152910646, 245.7265035704120351, -6.575810094723514965 ) ) ;
#43762=CARTESIAN_POINT ( 'NONE',  ( 12.21864935082045456, 177.8615022471902591, -10.00000000000009592 ) ) ;
#43764=CARTESIAN_POINT ( 'NONE',  ( 130.8910194135003735, 252.5024278399160949, 9.188101187500095079 ) ) ;
#43766=CARTESIAN_POINT ( 'NONE',  ( 164.2980263007286226, 246.0744661942869982, 1.511195434064211529 ) ) ;
#43768=CARTESIAN_POINT ( 'NONE',  ( 177.7634369230092091, 252.8608366103077856, -4.270187854574569275E-12 ) ) ;
#43769=CARTESIAN_POINT ( 'NONE',  ( 180.6665526851674599, 287.6815954905284798, 14.11204521094005671 ) ) ;
#43773=CARTESIAN_POINT ( 'NONE',  ( 151.2648146047323507, 268.6486510375538614, 15.71323890031163550 ) ) ;
#43774=CARTESIAN_POINT ( 'NONE',  ( 163.6887036115909666, 247.1298440500783613, 7.368436217261104204 ) ) ;
#43776=CARTESIAN_POINT ( 'NONE',  ( 170.3310799939524429, 266.5390996155348944, -16.61713687241611836 ) ) ;
#43778=ORIENTED_EDGE ( 'NONE', *, *, #25483, .F. ) ;
#43780=CARTESIAN_POINT ( 'NONE',  ( 168.8507326547640162, 282.4667480612920372, -10.92933487478789445 ) ) ;
#43784=CARTESIAN_POINT ( 'NONE',  ( 185.4867332780130766, 297.4061142773095412, 5.671143563000668131 ) ) ;
#43785=CARTESIAN_POINT ( 'NONE',  ( 138.6583583033484786, 260.8615022471902876, 5.000000000000046185 ) ) ;
#43786=AXIS2_PLACEMENT_3D ( 'NONE', #92482, #63542, #15941 ) ;
#43787=CARTESIAN_POINT ( 'NONE',  ( 148.8081469520198539, 276.3561860483582109, -0.0002503201696655007265 ) ) ;
#43789=EDGE_CURVE ( 'NONE', #20199, #17038, #27421, .T. ) ;
#43796=CARTESIAN_POINT ( 'NONE',  ( 156.0331829292964017, 261.8985861856509700, -16.97186308071531258 ) ) ;
#43797=B_SPLINE_CURVE_WITH_KNOTS ( 'NONE', 3,
 ( #55578, #16100, #85035, #47003 ),
 .UNSPECIFIED., .F., .F.,
 ( 4, 4 ),
 ( 0.04853013625147470367, 0.04887120950165269734 ),
 .UNSPECIFIED. ) ;
#43799=CARTESIAN_POINT ( 'NONE',  ( 191.7741832257749195, 298.4843664033717801, -8.615487418695501276 ) ) ;
#43800=CARTESIAN_POINT ( 'NONE',  ( 185.7027875752530406, 291.1743587175776611, 12.16933810580360387 ) ) ;
#43801=B_SPLINE_CURVE_WITH_KNOTS ( 'NONE', 3,
 ( #8404, #45395, #39275, #38283, #62577, #54991, #70185, #793, #39766, #94041, #84444, #14989, #24592, #24095, #47392, #14513, #76325, #45876, #68690, #30201, #7393, #61588, #2320, #41282, #79352, #10412, #72737, #33200, #3328, #16988, #65100, #33719, #48912, #64101, #32696, #87971, #71727, #95047, #55970, #82216, #25610, #34208, #2829, #94536, #72224, #18515, #47879, #79846, #64609, #12788, #56497, #20377 ),
 .UNSPECIFIED., .F., .F.,
 ( 4, 2, 2, 2, 2, 2, 2, 2, 2, 2, 2, 2, 2, 2, 2, 2, 2, 2, 2, 2, 2, 2, 2, 2, 2, 4 ),
 ( 9.788385118261326871E-05, 0.001114237024482954202, 0.001368325317808037796, 0.001622413611133120956, 0.001749457757795665463, 0.001876501904458209753, 0.002003546051120754044, 0.002130590197783298334, 0.002384678491108393854, 0.002638766784433488506, 0.003146943371083746766, 0.004163296544384260250, 0.005179649717684773301, 0.005687826304335072761, 0.005941914597660264558, 0.006068958744322860456, 0.006196002890985456354, 0.006259524964316822392, 0.006323047037648188429, 0.006450091184311090506, 0.006704179477637036040, 0.006958267770962981574, 0.007212356064288926241, 0.007466444357614864837, 0.007720532650940801697, 0.008228709237592696235 ),
 .UNSPECIFIED. ) ;
#43802=CARTESIAN_POINT ( 'NONE',  ( 166.0742539356187706, 262.7740412608126803, -17.50261138965781527 ) ) ;
#43804=ORIENTED_EDGE ( 'NONE', *, *, #21458, .T. ) ;
#43805=CARTESIAN_POINT ( 'NONE',  ( 84.74801659416949917, 228.9244531367911293, -4.594050593750046652 ) ) ;
#43806=CARTESIAN_POINT ( 'NONE',  ( 155.2775459039818315, 261.6983965501318039, 17.03612935257831040 ) ) ;
#43808=CARTESIAN_POINT ( 'NONE',  ( 181.3346534254663140, 271.3440730695800767, -17.45372068697093226 ) ) ;
#43809=CARTESIAN_POINT ( 'NONE',  ( 184.9070598923041473, 259.8481512251225354, -5.813936190556519890 ) ) ;
#43810=B_SPLINE_CURVE_WITH_KNOTS ( 'NONE', 3,
 ( #56040, #17565, #33793, #79414, #80925, #3393, #88034, #48473, #26175, #95626, #34267, #19091, #2385, #64167, #27176, #33265, #58064, #88530, #25680, #49970, #65162, #57052, #18582, #11495, #58547, #4879, #50457, #89999, #59533, #51961, #12987, #74296, #60033, #5858, #97111, #13956, #90512, #51454, #27680, #89520, #73773, #44837, #13473, #90998, #81903, #82901, #43847, #74786, #12480, #44342, #20080, #35760 ),
 .UNSPECIFIED., .F., .F.,
 ( 4, 2, 2, 2, 2, 2, 2, 2, 2, 2, 2, 2, 2, 2, 2, 2, 2, 2, 2, 2, 2, 2, 2, 2, 2, 4 ),
 ( 0.001584306797643239388, 0.002043180208590379687, 0.002502053619537519553, 0.002731490325011090570, 0.002846208677747904918, 0.002960927030484718833, 0.003075645383221533181, 0.003190363735958347095, 0.003419800441431977527, 0.003878673852379238389, 0.004337547263326498384, 0.005255294085221049599, 0.006173040907115600814, 0.006631914318062911984, 0.007090787729010222286, 0.007205506081747125972, 0.007262865258115577816, 0.007320224434484028792, 0.007434942787220981918, 0.007549661139957934176, 0.007779097845431880327, 0.008008534550905825611, 0.008237971256379771762, 0.008467407961853717913, 0.008696844667327664063, 0.008926281372801610214 ),
 .UNSPECIFIED. ) ;
#43811=ORIENTED_EDGE ( 'NONE', *, *, #64237, .F. ) ;
#43812=EDGE_CURVE ( 'NONE', #64017, #99390, #44245, .T. ) ;
#43814=CARTESIAN_POINT ( 'NONE',  ( -11.83159780365783398, 170.6427522451419065, 10.00000000000009415 ) ) ;
#43815=ORIENTED_EDGE ( 'NONE', *, *, #67126, .T. ) ;
#43818=CARTESIAN_POINT ( 'NONE',  ( 205.4228510824199248, 268.8300068208707785, 0.2998358105646597993 ) ) ;
#43819=CARTESIAN_POINT ( 'NONE',  ( 155.3250150347760723, 261.6161776038049425, -18.57420904020362684 ) ) ;
#43820=ORIENTED_EDGE ( 'NONE', *, *, #4708, .T. ) ;
#43821=CARTESIAN_POINT ( 'NONE',  ( 206.8268337557409211, 272.4124108968919131, -7.200219557041771523 ) ) ;
#43824=CARTESIAN_POINT ( 'NONE',  ( 19.28323191311993057, 170.3932355074535678, -2.679491924311248496 ) ) ;
#43826=CARTESIAN_POINT ( 'NONE',  ( 157.1282499545302755, 258.4928831048084135, -18.43070736571433699 ) ) ;
#43830=ADVANCED_FACE ( 'NONE', ( #73089 ), #3683, .T. ) ;
#43831=ORIENTED_EDGE ( 'NONE', *, *, #67764, .F. ) ;
#43833=CARTESIAN_POINT ( 'NONE',  ( 204.0830486605019871, 271.5957195856256590, 9.804030348223873759 ) ) ;
#43834=ORIENTED_EDGE ( 'NONE', *, *, #8899, .T. ) ;
#43838=CARTESIAN_POINT ( 'NONE',  ( 161.3490137394416877, 281.4934520396691369, -6.492417838214519676 ) ) ;
#43839=DIRECTION ( 'NONE',  ( -0.8660254037844387076, -0.4999999999999998890, -0.000000000000000000 ) ) ;
#43840=CARTESIAN_POINT ( 'NONE',  ( 158.4533830096545159, 257.7614088891019719, 17.16045812922167002 ) ) ;
#43841=CARTESIAN_POINT ( 'NONE',  ( 168.0428203547336921, 252.9999441337117503, 11.78450787674390199 ) ) ;
#43847=CARTESIAN_POINT ( 'NONE',  ( 160.1046313666135177, 276.6195463108357444, 12.87142096350444120 ) ) ;
#43850=CARTESIAN_POINT ( 'NONE',  ( 190.1519139143167081, 301.2942192743771557, 4.481136594690903863 ) ) ;
#43851=CARTESIAN_POINT ( 'NONE',  ( 164.8351683237598024, 274.0798523170363410, 15.21690876053529706 ) ) ;
#43852=CARTESIAN_POINT ( 'NONE',  ( -4.533703103291247594, 174.3149278399161233, 9.188101187500093303 ) ) ;
#43854=CARTESIAN_POINT ( 'NONE',  ( 203.1946125585645859, 269.9679951457329139, 6.014315348829343044 ) ) ;
#43856=ORIENTED_EDGE ( 'NONE', *, *, #19358, .F. ) ;
#43860=CARTESIAN_POINT ( 'NONE',  ( 175.5246756310037028, 290.9156563365580723, 2.576511661195814540 ) ) ;
#43861=CARTESIAN_POINT ( 'NONE',  ( 153.3920560952016956, 264.9641606960921649, 16.50453917291963535 ) ) ;
#43865=CARTESIAN_POINT ( 'NONE',  ( -3.586574591843265658, 177.9244531367911577, -4.594050593750046652 ) ) ;
#43866=CARTESIAN_POINT ( 'NONE',  ( 99.66015183740654493, 228.3458772461660544, 9.188101187500095079 ) ) ;
#43867=CARTESIAN_POINT ( 'NONE',  ( 47.20246722098146108, 191.3927522451417929, -10.00000000000009237 ) ) ;
#43868=CARTESIAN_POINT ( 'NONE',  ( 181.1221284655866270, 256.4354403611804969, -2.327941025046529777 ) ) ;
#43870=CARTESIAN_POINT ( 'NONE',  ( 177.8561250001070846, 283.2065401683831283, -14.44526047890849796 ) ) ;
#43871=CARTESIAN_POINT ( 'NONE',  ( 190.6839247239546751, 299.7689920197724973, -5.111333485343316774 ) ) ;
#43873=CARTESIAN_POINT ( 'NONE',  ( 182.6908602801013899, 274.3648995712160286, 16.39508407896753539 ) ) ;
#43874=CARTESIAN_POINT ( 'NONE',  ( 148.1004780136491377, 274.1294427855589788, -7.811560775291159331 ) ) ;
#43877=CARTESIAN_POINT ( 'NONE',  ( 193.2553405396020025, 265.5685525206544639, 7.793004429795182375 ) ) ;
#43879=CARTESIAN_POINT ( 'NONE',  ( 184.7157775894015117, 297.3647472220100099, -4.497232409310948142 ) ) ;
#43880=CARTESIAN_POINT ( 'NONE',  ( 183.4233717680499467, 267.7550803107557158, -15.99514032604573011 ) ) ;
#43886=CARTESIAN_POINT ( 'NONE',  ( 85.69549220138247847, 220.2833772461660544, -9.188101187500095079 ) ) ;
#43888=CARTESIAN_POINT ( 'NONE',  ( 191.2056514706806070, 299.4690922889112699, 7.290007621276087590 ) ) ;
#43889=CARTESIAN_POINT ( 'NONE',  ( 158.7250054796891732, 259.1391378321184220, -17.13534898805800211 ) ) ;
#43890=CARTESIAN_POINT ( 'NONE',  ( 195.8627871995700502, 291.4026965887302936, 17.41145040657729481 ) ) ;
#43891=CARTESIAN_POINT ( 'NONE',  ( 152.4944416537803988, 266.5188745142414746, 15.96416334701886086 ) ) ;
#43892=CARTESIAN_POINT ( 'NONE',  ( 199.1216527653377000, 285.7581758537840528, -18.37739894744384728 ) ) ;
#43893=CARTESIAN_POINT ( 'NONE',  ( 173.2161758961336488, 268.0191514601266931, -16.29353906404126562 ) ) ;
#43895=CARTESIAN_POINT ( 'NONE',  ( 147.4271219180435253, 275.2957297547342819, -3.800519706258907782 ) ) ;
#43897=ORIENTED_EDGE ( 'NONE', *, *, #83804, .T. ) ;
#43901=CARTESIAN_POINT ( 'NONE',  ( 188.0102668379925035, 285.9726363770864168, -16.35593525032086148 ) ) ;
#43902=ORIENTED_EDGE ( 'NONE', *, *, #4660, .F. ) ;
#43904=CARTESIAN_POINT ( 'NONE',  ( 160.0105735053945182, 253.5005522708592594, 16.10371386499367929 ) ) ;
#43905=CARTESIAN_POINT ( 'NONE',  ( 157.3351601172205676, 268.6802943510268733, 15.65239677815443287 ) ) ;
#43908=CARTESIAN_POINT ( 'NONE',  ( 146.5247557210571756, 248.7365022471902023, 10.00000000000009592 ) ) ;
#43913=CARTESIAN_POINT ( 'NONE',  ( 196.9914202414729232, 265.2248154332262970, -4.566998097189091332 ) ) ;
#43916=CARTESIAN_POINT ( 'NONE',  ( 181.4406354472745591, 291.0628233767851043, -11.23432871412726541 ) ) ;
#43917=EDGE_LOOP ( 'NONE', ( #71652, #51401, #73288 ) ) ;
#43918=CARTESIAN_POINT ( 'NONE',  ( 201.9316232165379859, 267.4154334901691072, 4.302177643393134687 ) ) ;
#43919=CARTESIAN_POINT ( 'NONE',  ( 158.9201382803563547, 255.3892414829881261, 16.13706509051041138 ) ) ;
#43920=CARTESIAN_POINT ( 'NONE',  ( 144.1522069568320887, 254.0333772461660260, 9.188101187500095079 ) ) ;
#43925=CARTESIAN_POINT ( 'NONE',  ( 164.4315604333902172, 274.7944110612714894, 14.66686579097542875 ) ) ;
#43926=CARTESIAN_POINT ( 'NONE',  ( 171.7726240267592175, 270.5206136648362190, -17.82399101355076709 ) ) ;
#43927=ORIENTED_EDGE ( 'NONE', *, *, #32161, .F. ) ;
#43931=CARTESIAN_POINT ( 'NONE',  ( 204.8189571845487080, 275.8901551335242175, 13.43702398685204358 ) ) ;
#43933=CARTESIAN_POINT ( 'NONE',  ( 164.6359882590319899, 245.4890989114802551, -0.8957991669032092652 ) ) ;
#43935=CARTESIAN_POINT ( 'NONE',  ( 155.4618104034866235, 280.5061703920193281, 4.424633671028313842 ) ) ;
#43937=CARTESIAN_POINT ( 'NONE',  ( 171.0227729602065665, 287.7541690653450814, -4.552090657951240793 ) ) ;
#43939=CARTESIAN_POINT ( 'NONE',  ( 178.4848498230702489, 255.6885313391786951, 4.886089711317160855 ) ) ;
#43940=CARTESIAN_POINT ( 'NONE',  ( 104.5047417616495125, 221.9548013555409511, -4.594050593750042211 ) ) ;
#43941=ORIENTED_EDGE ( 'NONE', *, *, #84717, .F. ) ;
#43942=CARTESIAN_POINT ( 'NONE',  ( 148.3835077007541088, 274.9253393602572260, -7.051312147027137378 ) ) ;
#43943=CARTESIAN_POINT ( 'NONE',  ( 179.7302837102534738, 291.4774734579422102, -10.05131855248582795 ) ) ;
#43944=EDGE_CURVE ( 'NONE', #83615, #59645, #35837, .T. ) ;
#43947=CARTESIAN_POINT ( 'NONE',  ( 183.4553195968295256, 297.0403188216897661, -2.838562726794640056 ) ) ;
#43949=CARTESIAN_POINT ( 'NONE',  ( 195.7578697689113199, 291.5844189092309193, 17.18796537138345215 ) ) ;
#43950=CARTESIAN_POINT ( 'NONE',  ( 159.3451320108506764, 254.6531307488737355, -16.72997986213134425 ) ) ;
#43951=CARTESIAN_POINT ( 'NONE',  ( 197.4075646047015482, 273.1427705089788560, -14.69744958829762815 ) ) ;
#43952=ORIENTED_EDGE ( 'NONE', *, *, #83954, .T. ) ;
#43953=( BOUNDED_CURVE ( )  B_SPLINE_CURVE ( 2, ( #74340, #64726, #87596, #18631, #49509, #30198, #14509, #67708, #38280 ),
 .UNSPECIFIED., .F., .T. ) 
 B_SPLINE_CURVE_WITH_KNOTS ( ( 3, 2, 2, 2, 3 ),
 ( 0.08467741935483871774, 0.08602150537634409289, 0.08870967741935484319, 0.09139784946236559349, 0.09274193548387096864 ),
 .UNSPECIFIED. ) 
 CURVE ( )  GEOMETRIC_REPRESENTATION_ITEM ( )  RATIONAL_B_SPLINE_CURVE ( ( 0.9330127018922192983, 0.9330127018922196314, 1.000000000000000000, 0.8660254037844387076, 1.000000000000000000, 0.8660254037844387076, 1.000000000000000000, 0.9330127018922194093, 0.9330127018922194093 ) ) 
 REPRESENTATION_ITEM ( '' )  );
#43955=CARTESIAN_POINT ( 'NONE',  ( 162.6257765080958677, 248.9708877980734485, -10.42859054881151160 ) ) ;
#43956=VERTEX_POINT ( 'NONE', #100094 ) ;
#43957=ADVANCED_FACE ( 'NONE', ( #24067 ), #68664, .T. ) ;
#43958=CARTESIAN_POINT ( 'NONE',  ( 191.8042499109635060, 263.6573267499654207, -8.212264930826352227 ) ) ;
#43959=CYLINDRICAL_SURFACE ( 'NONE', #42985, 17.82106496071139645 ) ;
#43961=CARTESIAN_POINT ( 'NONE',  ( 132.6505673846437503, 238.2048013555409796, 4.594050593750051981 ) ) ;
#43965=CARTESIAN_POINT ( 'NONE',  ( 157.3094609834150788, 258.1790163958882545, 18.30007615310968916 ) ) ;
#43966=CARTESIAN_POINT ( 'NONE',  ( 57.68498304950349365, 204.1115022471902591, 10.00000000000009592 ) ) ;
#43967=CARTESIAN_POINT ( 'NONE',  ( 190.3403783070287432, 264.3467331185190119, -9.331392502024449698 ) ) ;
#43968=CARTESIAN_POINT ( 'NONE',  ( 170.5500411757033419, 249.6187539556079855, -0.2597110160622304043 ) ) ;
#43969=CARTESIAN_POINT ( 'NONE',  ( 123.0902549634681407, 230.3262482093458061, 3.021315404115420679E-15 ) ) ;
#43972=CARTESIAN_POINT ( 'NONE',  ( 138.8568224548344858, 257.6427522451418781, 10.00000000000009415 ) ) ;
#43973=CARTESIAN_POINT ( 'NONE',  ( 161.5056331467593225, 250.9110330116698435, 14.52719814064025528 ) ) ;
#43975=CARTESIAN_POINT ( 'NONE',  ( 56.27743144475606130, 212.4869531367911009, 4.594050593750046652 ) ) ;
#43976=CARTESIAN_POINT ( 'NONE',  ( 206.5237403681858552, 272.9373840435757188, -10.81420335655575116 ) ) ;
#43977=DIRECTION ( 'NONE',  ( -0.8660254037844387076, -0.4999999999999998890, -0.000000000000000000 ) ) ;
#43978=CARTESIAN_POINT ( 'NONE',  ( 163.4178923001155681, 247.5989030008181260, -10.38047187240561442 ) ) ;
#43980=DIRECTION ( 'NONE',  ( 0.8660254037844395958, 0.4999999999999985567, 0.000000000000000000 ) ) ;
#43985=CARTESIAN_POINT ( 'NONE',  ( 149.8100742315740774, 272.7067330206335782, -11.46274738871846566 ) ) ;
#43988=CARTESIAN_POINT ( 'NONE',  ( 18.68642948779652002, 193.8464784336661637, 1.353441290958777327E-15 ) ) ;
#43989=CARTESIAN_POINT ( 'NONE',  ( 207.1829395897571260, 270.7610514960755381, 3.262445449933754293 ) ) ;
#43990=ADVANCED_FACE ( 'NONE', ( #92029 ), #83005, .F. ) ;
#43991=CARTESIAN_POINT ( 'NONE',  ( 157.2744851780909414, 258.2395962677452985, 18.17792129701959070 ) ) ;
#43992=CARTESIAN_POINT ( 'NONE',  ( 200.6957962653111167, 278.2105254787464901, 15.28271896800693952 ) ) ;
#43995=CARTESIAN_POINT ( 'NONE',  ( 40.25596147474394826, 203.2369531367911293, -4.594050593750048428 ) ) ;
#43997=CARTESIAN_POINT ( 'NONE',  ( 170.8906340425221799, 287.3599720229358923, 7.052392840008895547 ) ) ;
#43998=CARTESIAN_POINT ( 'NONE',  ( -18.11259370987442452, 171.8967562850347690, 9.296355089585912665E-16 ) ) ;
#44000=CARTESIAN_POINT ( 'NONE',  ( 203.2757866645317222, 269.5093088776978334, -7.514607224931010521 ) ) ;
#44002=CARTESIAN_POINT ( 'NONE',  ( 176.4077479315872665, 274.9858714345624549, 16.74632039004189465 ) ) ;
#44003=CARTESIAN_POINT ( 'NONE',  ( 155.0568450317760494, 264.0806616740677555, 17.52241723436104337 ) ) ;
#44005=CARTESIAN_POINT ( 'NONE',  ( 193.0433938349725338, 267.1203275631486349, 11.31873111441719182 ) ) ;
#44007=CARTESIAN_POINT ( 'NONE',  ( 108.2753003872445134, 219.9865022471901739, 1.119607411625061291E-15 ) ) ;
#44008=FACE_OUTER_BOUND ( 'NONE', #18541, .T. ) ;
#44011=CARTESIAN_POINT ( 'NONE',  ( 51.08127902204942927, 209.4869531367911009, 4.594050593750046652 ) ) ;
#44017=CARTESIAN_POINT ( 'NONE',  ( 177.1052724318428773, 289.8048150823444757, 10.36495476014435901 ) ) ;
#44018=CARTESIAN_POINT ( 'NONE',  ( 204.0604753336787667, 271.4817813032398703, 9.862283393711939183 ) ) ;
#44019=B_SPLINE_CURVE_WITH_KNOTS ( 'NONE', 3,
 ( #58185, #59156, #3994, #90126, #20701, #65780 ),
 .UNSPECIFIED., .F., .F.,
 ( 4, 2, 4 ),
 ( 0.01962962394112050674, 0.02417033321900810550, 0.02871104249689570426 ),
 .UNSPECIFIED. ) ;
#44021=B_SPLINE_CURVE_WITH_KNOTS ( 'NONE', 3,
 ( #91241, #49106, #41486, #70914 ),
 .UNSPECIFIED., .F., .F.,
 ( 4, 4 ),
 ( 0.02844990342440924941, 0.03762721602985887731 ),
 .UNSPECIFIED. ) ;
#44023=CARTESIAN_POINT ( 'NONE',  ( 188.6489399924155066, 265.3460165191049214, 10.74106153545168318 ) ) ;
#44024=CARTESIAN_POINT ( 'NONE',  ( 149.2593905435863348, 272.1221474021800759, -12.98626158366800176 ) ) ;
#44025=CARTESIAN_POINT ( 'NONE',  ( 157.3812306876618266, 258.0547076216885785, 17.10114491953027027 ) ) ;
#44027=ORIENTED_EDGE ( 'NONE', *, *, #31217, .T. ) ;
#44031=CARTESIAN_POINT ( 'NONE',  ( 175.6063544791335573, 254.0105997054014040, 8.344378697908656051 ) ) ;
#44033=ORIENTED_EDGE ( 'NONE', *, *, #84494, .T. ) ;
#44034=CARTESIAN_POINT ( 'NONE',  ( -22.42236680055709641, 157.8615022471902591, 0.000000000000000000 ) ) ;
#44035=CARTESIAN_POINT ( 'NONE',  ( 166.9027035012226463, 261.4283233817405971, 16.57751465251748257 ) ) ;
#44036=CARTESIAN_POINT ( 'NONE',  ( 159.9997000813754084, 253.5193855937126841, -16.28798248637880519 ) ) ;
#44038=ORIENTED_EDGE ( 'NONE', *, *, #27553, .T. ) ;
#44039=CARTESIAN_POINT ( 'NONE',  ( 159.2607205968722042, 282.5689587104361635, -3.306452599273326243 ) ) ;
#44043=CARTESIAN_POINT ( 'NONE',  ( 159.3528137482544196, 254.6398255893999476, 16.73628156321660398 ) ) ;
#44045=CARTESIAN_POINT ( 'NONE',  ( 164.5705541677141923, 265.2993310360931787, -16.66072161617881164 ) ) ;
#44046=CARTESIAN_POINT ( 'NONE',  ( 132.9753269110629503, 238.3923013555409796, 4.594050593750050204 ) ) ;
#44048=VERTEX_POINT ( 'NONE', #97855 ) ;
#44049=CARTESIAN_POINT ( 'NONE',  ( 170.3043206595384902, 263.9273437261221602, 15.94611219504030508 ) ) ;
#44051=CARTESIAN_POINT ( 'NONE',  ( 183.6331817901053682, 289.8384269728442177, -13.45033778474055808 ) ) ;
#44053=ORIENTED_EDGE ( 'NONE', *, *, #22537, .T. ) ;
#44056=ORIENTED_EDGE ( 'NONE', *, *, #86935, .F. ) ;
#44057=CARTESIAN_POINT ( 'NONE',  ( 198.2819808855875863, 287.2125302111982705, 18.53535247371401695 ) ) ;
#44059=CARTESIAN_POINT ( 'NONE',  ( 75.81765026128996965, 205.3923013555409796, 4.594050593750050204 ) ) ;
#44060=CARTESIAN_POINT ( 'NONE',  ( -22.42236680055709641, 157.8615022471902591, 0.000000000000000000 ) ) ;
#44062=CARTESIAN_POINT ( 'NONE',  ( 194.1011995340913074, 294.4538559273262877, 13.93949783759920713 ) ) ;
#44063=CARTESIAN_POINT ( 'NONE',  ( 175.3207465333977950, 278.3523610338168623, 15.46700679219081209 ) ) ;
#44068=CARTESIAN_POINT ( 'NONE',  ( 153.2906404175950854, 265.1398178023911782, -17.60231834963988007 ) ) ;
#44074=CARTESIAN_POINT ( 'NONE',  ( 174.2670700365113134, 253.8381489143473004, -7.486906580229475416 ) ) ;
#44076=CARTESIAN_POINT ( 'NONE',  ( 164.3939401533646958, 245.9083385283718712, 2.844462461176849200 ) ) ;
#44078=CARTESIAN_POINT ( 'NONE',  ( 195.7846125890239364, 279.4931724946097233, 16.34764129634911711 ) ) ;
#44079=CARTESIAN_POINT ( 'NONE',  ( 163.8111161534324935, 246.9178193081252743, -7.110480325054721717 ) ) ;
#44080=CARTESIAN_POINT ( 'NONE',  ( 138.9560545341254851, 251.0333772461660260, 9.188101187500095079 ) ) ;
#44081=EDGE_LOOP ( 'NONE', ( #40452, #60017, #14816, #34980 ) ) ;
#44084=CARTESIAN_POINT ( 'NONE',  ( 181.7383033065034112, 289.1381347789208007, -13.52584881963807284 ) ) ;
#44086=CARTESIAN_POINT ( 'NONE',  ( -27.42236680055714260, 166.5217562850347406, 1.224646799147364892E-15 ) ) ;
#44087=CARTESIAN_POINT ( 'NONE',  ( 178.3148920459139788, 254.9549173854477999, 4.342301552106668794 ) ) ;
#44090=CARTESIAN_POINT ( 'NONE',  ( 182.3761579831538313, 275.1398338757759348, -16.79997168648350936 ) ) ;
#44091=CARTESIAN_POINT ( 'NONE',  ( 164.5641499066685469, 246.8022252770303169, -5.664862832761055955 ) ) ;
#44093=CARTESIAN_POINT ( 'NONE',  ( 186.2798660816079632, 264.0713031700501006, -12.82791401631097550 ) ) ;
#44095=CARTESIAN_POINT ( 'NONE',  ( 146.8358616138309571, 276.3198226421291679, 4.054088818585255716 ) ) ;
#44100=EDGE_CURVE ( 'NONE', #34942, #33130, #64919, .T. ) ;
#44101=ADVANCED_FACE ( 'NONE', ( #69912 ), #23311, .T. ) ;
#44103=B_SPLINE_SURFACE_WITH_KNOTS ( 'NONE', 3, 1, ( 
 ( #11751, #42614 ),
 ( #27448, #43105 ),
 ( #58322, #36017 ),
 ( #89297, #74048 ),
 ( #35530, #97849 ),
 ( #41625, #57327 ),
 ( #28420, #66431 ),
 ( #59298, #90279 ),
 ( #97359, #49246 ),
 ( #10749, #98346 ),
 ( #44108, #15202 ),
 ( #83161, #22319 ),
 ( #59814, #76536 ),
 ( #68912, #90780 ),
 ( #13726, #29922 ),
 ( #29426, #28937 ),
 ( #61310, #5623 ),
 ( #6122, #14230 ),
 ( #67926, #75537 ),
 ( #45117, #36517 ),
 ( #67418, #76051 ),
 ( #46098, #21331 ),
 ( #37018, #82684 ),
 ( #7617, #52215 ),
 ( #30420, #6631 ),
 ( #44603, #98849 ),
 ( #60300, #91259 ),
 ( #21822, #92272 ),
 ( #53222, #60794 ),
 ( #20851, #22820 ),
 ( #13251, #52708 ),
 ( #83667, #84173 ),
 ( #37508, #53701 ),
 ( #99836, #68415 ) ),
 .UNSPECIFIED., .T., .F., .F.,
 ( 4, 2, 2, 2, 2, 2, 2, 2, 2, 2, 2, 2, 2, 2, 2, 2, 4 ),
 ( 2, 2 ),
 ( 0.000000000000000000, 0.06250000000000000000, 0.1250000000000000000, 0.1875000000000000000, 0.2500000000000000000, 0.3125000000000000000, 0.3750000000000000000, 0.4375000000000000000, 0.5000000000000000000, 0.5625000000000000000, 0.6250000000000000000, 0.6875000000000000000, 0.7500000000000000000, 0.8125000000000000000, 0.8750000000000000000, 0.9375000000000000000, 1.000000000000000000 ),
 ( 0.000000000000000000, 1.000000000000000000 ),
 .UNSPECIFIED. ) ;
#44105=CARTESIAN_POINT ( 'NONE',  ( 148.9230895364621574, 272.7046378331555161, 12.20434325797056019 ) ) ;
#44106=CARTESIAN_POINT ( 'NONE',  ( 73.03889176721716581, 219.6427522451419065, -10.00000000000009592 ) ) ;
#44108=CARTESIAN_POINT ( 'NONE',  ( 197.8977219949227049, 287.8780861330898801, 17.48564646125164046 ) ) ;
#44109=CARTESIAN_POINT ( 'NONE',  ( 161.4317887380794900, 251.0389352793577871, 14.14184562255241318 ) ) ;
#44110=EDGE_CURVE ( 'NONE', #68650, #79972, #32244, .T. ) ;
#44111=CARTESIAN_POINT ( 'NONE',  ( 143.3312870410541677, 246.8927522451417929, -10.00000000000009059 ) ) ;
#44112=CARTESIAN_POINT ( 'NONE',  ( 175.5934154519829633, 286.1723408421822228, -11.93597657450535188 ) ) ;
#44117=CARTESIAN_POINT ( 'NONE',  ( 150.8168331730346949, 269.4245776381016526, -15.71017957295074652 ) ) ;
#44118=CARTESIAN_POINT ( 'NONE',  ( 7.942909239684589728, 166.2048013555410080, 4.594050593750051981 ) ) ;
#44119=CARTESIAN_POINT ( 'NONE',  ( 178.7548933528066470, 273.8195275360004075, -17.51453903275912793 ) ) ;
#44122=CARTESIAN_POINT ( 'NONE',  ( 157.6036818288543486, 257.6694109429415107, -16.73826488331764395 ) ) ;
#44124=DIRECTION ( 'NONE',  ( 0.4999999999999998890, -0.8660254037844385966, 0.000000000000000000 ) ) ;
#44126=B_SPLINE_SURFACE_WITH_KNOTS ( 'NONE', 3, 1, ( 
 ( #63890, #25913 ),
 ( #79639, #55269 ),
 ( #17287, #86249 ),
 ( #69978, #71013 ),
 ( #16787, #94332 ),
 ( #9195, #592 ),
 ( #79138, #9719 ),
 ( #40070, #24885 ),
 ( #86753, #48191 ),
 ( #17806, #93326 ),
 ( #71515, #2105 ),
 ( #94826, #41069 ),
 ( #2611, #31477 ),
 ( #64395, #33499 ),
 ( #56785, #62368 ),
 ( #58766, #50189 ),
 ( #97317, #35974 ),
 ( #27884, #34016 ),
 ( #42085, #51696 ),
 ( #35484, #42569 ),
 ( #73017, #34977 ),
 ( #57280, #96330 ),
 ( #43580, #66876 ),
 ( #10703, #41581 ),
 ( #82139, #12200 ),
 ( #74004, #3609 ),
 ( #43061, #18803 ),
 ( #88256, #64901 ),
 ( #5093, #11708 ),
 ( #59255, #49686 ),
 ( #80641, #12709 ),
 ( #3131, #4590 ),
 ( #66388, #51174 ),
 ( #89736, #97809 ) ),
 .UNSPECIFIED., .T., .F., .F.,
 ( 4, 2, 2, 2, 2, 2, 2, 2, 2, 2, 2, 2, 2, 2, 2, 2, 4 ),
 ( 2, 2 ),
 ( 0.000000000000000000, 0.06250000000000000000, 0.1250000000000000000, 0.1875000000000000000, 0.2500000000000000000, 0.3125000000000000000, 0.3750000000000000000, 0.4375000000000000000, 0.5000000000000000000, 0.5625000000000000000, 0.6250000000000000000, 0.6875000000000000000, 0.7500000000000000000, 0.8125000000000000000, 0.8750000000000000000, 0.9375000000000000000, 1.000000000000000000 ),
 ( 0.000000000000000000, 1.000000000000000000 ),
 .UNSPECIFIED. ) ;
#44127=CARTESIAN_POINT ( 'NONE',  ( 18.55146011244625370, 181.5177522451418497, -10.00000000000009592 ) ) ;
#44128=CARTESIAN_POINT ( 'NONE',  ( 73.18322933451463541, 206.3927522451418213, -10.00000000000009059 ) ) ;
#44131=CARTESIAN_POINT ( 'NONE',  ( 198.5328126748496516, 286.7780768080430676, 18.48542741931266775 ) ) ;
#44133=CARTESIAN_POINT ( 'NONE',  ( 55.08690683815012790, 212.6115022471903444, -5.000000000000047962 ) ) ;
#44134=CARTESIAN_POINT ( 'NONE',  ( 181.9135216713392538, 291.6657426544036298, 9.319931514330358269 ) ) ;
#44135=CARTESIAN_POINT ( 'NONE',  ( 189.8533352240220893, 301.8113727360248504, -0.2033756396389863053 ) ) ;
#44136=CARTESIAN_POINT ( 'NONE',  ( 16.52171307410043255, 180.3458772461660544, 9.188101187500095079 ) ) ;
#44137=CARTESIAN_POINT ( 'NONE',  ( 168.2555426073723481, 286.2821508661389771, 4.155022024279104720 ) ) ;
#44138=CARTESIAN_POINT ( 'NONE',  ( 192.3401793061076717, 297.5040324353506094, 12.56432540404525611 ) ) ;
#44141=CARTESIAN_POINT ( 'NONE',  ( 207.6209998424140792, 271.0368748851258260, 6.610167240481342965 ) ) ;
#44142=LINE ( 'NONE', #38538, #81542 ) ;
#44143=CARTESIAN_POINT ( 'NONE',  ( 123.1420698188773315, 235.2365022471902023, 10.00000000000009948 ) ) ;
#44144=CARTESIAN_POINT ( 'NONE',  ( 160.6358730764160612, 280.0761735822365495, 9.121476281160894928 ) ) ;
#44147=CARTESIAN_POINT ( 'NONE',  ( 121.1754704609022468, 240.7677522451418497, 10.00000000000009592 ) ) ;
#44149=CARTESIAN_POINT ( 'NONE',  ( 159.4515169353164197, 258.9283067265839122, 16.83560305343668517 ) ) ;
#44150=CARTESIAN_POINT ( 'NONE',  ( 155.6126298223767890, 261.1180141786725244, 18.15400560664037855 ) ) ;
#44151=ORIENTED_EDGE ( 'NONE', *, *, #80813, .T. ) ;
#44152=CARTESIAN_POINT ( 'NONE',  ( 181.8673996824255710, 289.2482696471543022, 12.44316705411579882 ) ) ;
#44157=CARTESIAN_POINT ( 'NONE',  ( 196.4830298217786435, 289.2019227521179232, -16.84636831274811897 ) ) ;
#44159=B_SPLINE_CURVE_WITH_KNOTS ( 'NONE', 3,
 ( #9396, #32687, #63588, #63087 ),
 .UNSPECIFIED., .F., .F.,
 ( 4, 4 ),
 ( 0.000000000000000000, 0.005356180736718595299 ),
 .UNSPECIFIED. ) ;
#44161=CARTESIAN_POINT ( 'NONE',  ( 202.8874463667715133, 279.2356300052831557, -15.29930322226033468 ) ) ;
#44164=CARTESIAN_POINT ( 'NONE',  ( 159.2788173922416775, 279.4644734097240644, -9.612199085998382131 ) ) ;
#44165=CARTESIAN_POINT ( 'NONE',  ( 204.9780665305064531, 275.6145696623662502, 14.10615427165218883 ) ) ;
#44166=CARTESIAN_POINT ( 'NONE',  ( 192.4202172926039793, 297.3654025762033370, 10.98569444949570872 ) ) ;
#44168=CARTESIAN_POINT ( 'NONE',  ( 151.3589047706063582, 268.4856820897672378, 14.56544807350869419 ) ) ;
#44171=VERTEX_POINT ( 'NONE', #22715 ) ;
#44176=CARTESIAN_POINT ( 'NONE',  ( 164.6241018286200699, 245.5096868128744632, 3.031483545445131433 ) ) ;
#44177=CARTESIAN_POINT ( 'NONE',  ( 158.2296914707421820, 265.1721668954002666, 17.20786077318715712 ) ) ;
#44179=CARTESIAN_POINT ( 'NONE',  ( 174.5677109544117229, 276.8219974751209520, -15.95664790871851757 ) ) ;
#44180=CARTESIAN_POINT ( 'NONE',  ( -22.42236680055709641, 157.8615022471902591, 0.000000000000000000 ) ) ;
#44181=CIRCLE ( 'NONE', #79821, 16.82106496071157764 ) ;
#44182=EDGE_CURVE ( 'NONE', #10482, #67335, #26157, .T. ) ;
#44185=CARTESIAN_POINT ( 'NONE',  ( 146.9700173529739970, 276.0874580858064746, -5.099093031535578469 ) ) ;
#44187=ORIENTED_EDGE ( 'NONE', *, *, #98839, .F. ) ;
#44189=CARTESIAN_POINT ( 'NONE',  ( 147.5813496936708020, 275.0285994114094592, 4.516581957185684004 ) ) ;
#44192=CARTESIAN_POINT ( 'NONE',  ( 157.0719585813440062, 259.1361147967522243, -16.97184851174986164 ) ) ;
#44194=CARTESIAN_POINT ( 'NONE',  ( 191.7916824445696591, 298.4540568673266421, 9.471960810989466850 ) ) ;
#44195=CARTESIAN_POINT ( 'NONE',  ( 146.7373254022577100, 276.4904923669593586, -0.7242168585908188572 ) ) ;
#44200=CARTESIAN_POINT ( 'NONE',  ( 149.5390997184345281, 271.6376768999995761, -11.52989534384373016 ) ) ;
#44201=CARTESIAN_POINT ( 'NONE',  ( 206.0627831668701901, 273.7357853363691902, 10.14454147593459687 ) ) ;
#44202=LINE ( 'NONE', #59903, #54156 ) ;
#44203=CARTESIAN_POINT ( 'NONE',  ( 189.3832291599495079, 300.6256203239445313, 1.753828516883770838 ) ) ;
#44205=CARTESIAN_POINT ( 'NONE',  ( 149.6097189538088230, 271.5153607963395075, -12.93833707350289330 ) ) ;
#44207=DIRECTION ( 'NONE',  ( 0.5000000000000003331, -0.8660254037844384856, 0.000000000000000000 ) ) ;
#44211=CARTESIAN_POINT ( 'NONE',  ( 198.8190325544414634, 286.2823294344537999, -18.51269608589847948 ) ) ;
#44214=CARTESIAN_POINT ( 'NONE',  ( 167.7412147458803133, 253.5458412874411636, -11.91840095923254417 ) ) ;
#44216=FACE_OUTER_BOUND ( 'NONE', #9417, .T. ) ;
#44217=CARTESIAN_POINT ( 'NONE',  ( 32.33569778934854355, 196.1427522451419065, 10.00000000000009237 ) ) ;
#44218=CARTESIAN_POINT ( 'NONE',  ( 118.6312605172356598, 248.4869531367911293, 4.594050593750046652 ) ) ;
#44219=CARTESIAN_POINT ( 'NONE',  ( 151.1811967613751335, 268.7934813906678642, -15.79361349403328418 ) ) ;
#44223=B_SPLINE_CURVE_WITH_KNOTS ( 'NONE', 3,
 ( #96278, #57723, #18255, #19273 ),
 .UNSPECIFIED., .F., .F.,
 ( 4, 4 ),
 ( 0.008754644785881138605, 0.01505839894353219049 ),
 .UNSPECIFIED. ) ;
#44224=CARTESIAN_POINT ( 'NONE',  ( 37.65788526339063225, 201.7369531367911293, -4.594050593750048428 ) ) ;
#44235=CARTESIAN_POINT ( 'NONE',  ( 178.0385697874355060, 286.6247767869483596, -12.15384962285411952 ) ) ;
#44236=CARTESIAN_POINT ( 'NONE',  ( 181.2921530440871720, 261.7463096819169550, 13.20693057592762010 ) ) ;
#44238=CARTESIAN_POINT ( 'NONE',  ( 87.40047971330908183, 231.2677522451419065, -5.000000000000047962 ) ) ;
#44240=CARTESIAN_POINT ( 'NONE',  ( 198.5188009505039872, 267.2797725955071542, -8.327816907216345044 ) ) ;
#44242=CARTESIAN_POINT ( 'NONE',  ( 155.2811537424576329, 279.9766836497481108, -2.298807824649978571 ) ) ;
#44244=CARTESIAN_POINT ( 'NONE',  ( 10.18907585680922878, 170.5643266524159571, -9.188101187500093303 ) ) ;
#44245=B_SPLINE_CURVE_WITH_KNOTS ( 'NONE', 3,
 ( #33577, #95919, #25466, #41655, #65462, #17884, #32573, #64472, #26479, #57355, #49766, #80722, #11295, #42155 ),
 .UNSPECIFIED., .F., .F.,
 ( 4, 2, 2, 2, 2, 2, 4 ),
 ( 0.0004313387020570975386, 0.001079531987292708202, 0.001403628629910513587, 0.001727725272528318756, 0.002051821915146123925, 0.002375918557763929528, 0.003024111842999565019 ),
 .UNSPECIFIED. ) ;
#44246=ADVANCED_FACE ( 'NONE', ( #95156 ), #73319, .T. ) ;
#44248=CARTESIAN_POINT ( 'NONE',  ( 195.8823446862052151, 273.2863346474129003, 15.24343364205054208 ) ) ;
#44252=CARTESIAN_POINT ( 'NONE',  ( 60.22919299317007358, 196.3923013555409796, 4.594050593750050204 ) ) ;
#44253=CARTESIAN_POINT ( 'NONE',  ( 208.1415148974628266, 270.1353163636768500, 3.453641150550738725 ) ) ;
#44256=CARTESIAN_POINT ( 'NONE',  ( 151.3511865740561007, 278.6745403919405248, -1.693856907688049862 ) ) ;
#44258=ORIENTED_EDGE ( 'NONE', *, *, #84447, .T. ) ;
#44259=VECTOR ( 'NONE', #83213, 1000.000000000000000 ) ;
#44261=CARTESIAN_POINT ( 'NONE',  ( 14.74455677852512636, 165.9865022471901739, 1.119607411625061291E-15 ) ) ;
#44262=CARTESIAN_POINT ( 'NONE',  ( 207.5408646414791178, 271.1756731246201753, 3.050859480894625886 ) ) ;
#44263=AXIS2_PLACEMENT_3D ( 'NONE', #29703, #59078, #60580 ) ;
#44264=CARTESIAN_POINT ( 'NONE',  ( 134.0307085979840167, 242.0643266524160140, 9.188101187500095079 ) ) ;
#44266=CARTESIAN_POINT ( 'NONE',  ( 191.2557879401978198, 261.3776189723048446, -4.694998167070893125 ) ) ;
#44270=CARTESIAN_POINT ( 'NONE',  ( 157.5710319558766344, 257.7259621817996162, 18.28704422422941533 ) ) ;
#44271=CARTESIAN_POINT ( 'NONE',  ( 189.2663724790391200, 289.8708104362821700, 14.44557331680590195 ) ) ;
#44273=VERTEX_POINT ( 'NONE', #56603 ) ;
#44274=CARTESIAN_POINT ( 'NONE',  ( 155.5494399783600272, 273.4016498944568525, 13.96529472218679224 ) ) ;
#44275=CARTESIAN_POINT ( 'NONE',  ( 163.5327758489833059, 247.3999188572254013, 7.475710045443520357 ) ) ;
#44276=CARTESIAN_POINT ( 'NONE',  ( 180.8098011652053003, 287.7440423659127191, 14.08944922001110633 ) ) ;
#44277=CARTESIAN_POINT ( 'NONE',  ( 173.0248719821516090, 268.2920160064722950, -16.32364012504238460 ) ) ;
#44278=CARTESIAN_POINT ( 'NONE',  ( 194.2215157464497111, 270.7474829811882273, -14.13497883233823416 ) ) ;
#44281=CARTESIAN_POINT ( 'NONE',  ( 168.2714446481795960, 282.1153207652979518, -10.92340985837064338 ) ) ;
#44284=CARTESIAN_POINT ( 'NONE',  ( 196.2975913249615587, 270.7692368477389664, 13.22270430323884938 ) ) ;
#44285=CARTESIAN_POINT ( 'NONE',  ( 175.1183745746886871, 267.9007702990796247, 17.47926410801357022 ) ) ;
#44286=FACE_OUTER_BOUND ( 'NONE', #15695, .T. ) ;
#44287=CARTESIAN_POINT ( 'NONE',  ( 150.0209462876923396, 271.4416770187968382, -12.09856010893388678 ) ) ;
#44288=CARTESIAN_POINT ( 'NONE',  ( 194.3931393306973234, 282.9231816806054098, 17.79127136852465441 ) ) ;
#44291=ORIENTED_EDGE ( 'NONE', *, *, #72061, .T. ) ;
#44292=CARTESIAN_POINT ( 'NONE',  ( 167.5680495833038322, 281.2627909971289455, 12.96205408629257150 ) ) ;
#44293=B_SPLINE_CURVE_WITH_KNOTS ( 'NONE', 3,
 ( #25183, #93624, #55074, #78406, #56063, #1403, #87056, #17591, #94129, #24684, #97135, #59557, #50477, #96135, #35784, #65187, #4383, #49992, #43371, #20595, #80439, #73794, #35283, #66677, #74318, #20104, #80947, #5388, #11515, #13008, #72823, #36274, #66190, #67173, #19116, #50974, #27703, #98096, #97612, #42369, #27198, #21104, #81430, #58569 ),
 .UNSPECIFIED., .F., .F.,
 ( 4, 2, 2, 2, 2, 2, 2, 2, 2, 2, 2, 2, 2, 2, 2, 2, 2, 2, 2, 2, 2, 4 ),
 ( 0.002656945797708354200, 0.003073439877435233704, 0.003281686917298652639, 0.003385810437230362107, 0.003489933957162071575, 0.003698180997025623216, 0.003906428036889175726, 0.004322922116616358806, 0.005155910276070672059, 0.005988898435524985311, 0.006821886594979298564, 0.007654874754433611816, 0.007758998274365423199, 0.007811060034331282487, 0.007863121794297142642, 0.007967245314228861217, 0.008071368834160581526, 0.008487862913887627564, 0.008696109953751200022, 0.008904356993614772481, 0.009112604033478348409, 0.009320851073341920867 ),
 .UNSPECIFIED. ) ;
#44295=CARTESIAN_POINT ( 'NONE',  ( 156.0396634953594628, 261.8849338628862711, -16.97419079234479611 ) ) ;
#44297=CARTESIAN_POINT ( 'NONE',  ( 147.0721334091522294, 275.9105878882373304, 0.7242168585908188572 ) ) ;
#44298=CARTESIAN_POINT ( 'NONE',  ( 204.8067230205685689, 273.0357175708630848, -9.758814814642425617 ) ) ;
#44299=CARTESIAN_POINT ( 'NONE',  ( 163.9149533033796047, 246.7379680887036670, 7.273005089308705706 ) ) ;
#44300=CYLINDRICAL_SURFACE ( 'NONE', #78665, 10.00000000000010658 ) ;
#44302=CARTESIAN_POINT ( 'NONE',  ( 92.19068272976576850, 224.0333772461660544, 9.188101187500095079 ) ) ;
#44303=CARTESIAN_POINT ( 'NONE',  ( 199.0624198797852955, 283.1069319285825827, 17.22852181067409916 ) ) ;
#44309=VERTEX_POINT ( 'NONE', #89082 ) ;
#44312=CARTESIAN_POINT ( 'NONE',  ( 159.4780960521576674, 258.5615967792256811, 17.42390817850915141 ) ) ;
#44315=CARTESIAN_POINT ( 'NONE',  ( 164.3663504224794565, 247.9561253440330972, -9.019399920391260039 ) ) ;
#44317=CARTESIAN_POINT ( 'NONE',  ( 152.7729059155601021, 266.0365602647466972, -17.50667083025758686 ) ) ;
#44321=CARTESIAN_POINT ( 'NONE',  ( 195.8418359169588427, 291.4389852746969041, -17.23329826360656014 ) ) ;
#44326=CARTESIAN_POINT ( 'NONE',  ( 166.5387429586460257, 283.1419806720085148, 8.930908821604470305 ) ) ;
#44327=CARTESIAN_POINT ( 'NONE',  ( 17.75760349231054391, 174.3927522451418213, 10.00000000000009948 ) ) ;
#44328=ORIENTED_EDGE ( 'NONE', *, *, #41263, .F. ) ;
#44329=CARTESIAN_POINT ( 'NONE',  ( 202.9093905060991005, 279.1976216410395182, 16.97070083370504179 ) ) ;
#44330=CARTESIAN_POINT ( 'NONE',  ( 185.3339162672891973, 258.7583632471134933, 2.918957613551585339 ) ) ;
#44331=CARTESIAN_POINT ( 'NONE',  ( 151.3711344188577925, 276.7819027391564077, -5.262085087660871352 ) ) ;
#44333=CYLINDRICAL_SURFACE ( 'NONE', #3661, 10.00000000000010658 ) ;
#44334=DIRECTION ( 'NONE',  ( -0.8660254037844303809, -0.5000000000000144329, 0.000000000000000000 ) ) ;
#44336=VECTOR ( 'NONE', #6985, 1000.000000000000000 ) ;
#44338=CARTESIAN_POINT ( 'NONE',  ( 193.8212943487757514, 292.9386659295947197, 15.46346239154970625 ) ) ;
#44340=CARTESIAN_POINT ( 'NONE',  ( 181.8761527141526813, 271.4782540734216809, -15.98508151632294094 ) ) ;
#44342=CARTESIAN_POINT ( 'NONE',  ( 160.0078452925083354, 276.7889099177259595, 13.19893458269325670 ) ) ;
#44343=CARTESIAN_POINT ( 'NONE',  ( -4.831225789733595732, 168.0177522451418781, -10.00000000000009592 ) ) ;
#44345=CARTESIAN_POINT ( 'NONE',  ( 194.7112710368652131, 268.6419340635496837, -10.81822129561431822 ) ) ;
#44346=CARTESIAN_POINT ( 'NONE',  ( 175.0303541417597160, 281.4344200042963280, -14.16194463650028901 ) ) ;
#44349=CARTESIAN_POINT ( 'NONE',  ( 164.6715181915554069, 274.3332101388145361, 14.81878660653080892 ) ) ;
#44350=CARTESIAN_POINT ( 'NONE',  ( -14.92600794870451253, 168.3149278399160664, 9.188101187500093303 ) ) ;
#44352=CARTESIAN_POINT ( 'NONE',  ( 163.9407385976260798, 248.4868885448184415, 9.894533935068681174 ) ) ;
#44353=ORIENTED_EDGE ( 'NONE', *, *, #37903, .F. ) ;
#44354=B_SPLINE_SURFACE_WITH_KNOTS ( 'NONE', 3, 1, ( 
 ( #81444, #95666 ),
 ( #89554, #64206 ),
 ( #80962, #4399 ),
 ( #42872, #95155 ),
 ( #11526, #19133 ),
 ( #57590, #20117 ),
 ( #26709, #88074 ),
 ( #18113, #89081 ),
 ( #34305, #49016 ),
 ( #79949, #42387 ),
 ( #79454, #34789 ),
 ( #35296, #73318 ),
 ( #73805, #10019 ),
 ( #66207, #40881 ),
 ( #88571, #97148 ),
 ( #11026, #3908 ),
 ( #71830, #41392 ),
 ( #26214, #65692 ),
 ( #2427, #96646 ),
 ( #50006, #27714 ),
 ( #27216, #56602 ),
 ( #58098, #33828 ),
 ( #80455, #33304 ),
 ( #87588, #10515 ),
 ( #72335, #19631 ),
 ( #2940, #57091 ),
 ( #18622, #49500 ),
 ( #41898, #72837 ),
 ( #3430, #65205 ),
 ( #96146, #37776 ),
 ( #76312, #21604 ),
 ( #44383, #90038 ),
 ( #61073, #59068 ),
 ( #14499, #52484 ) ),
 .UNSPECIFIED., .T., .F., .F.,
 ( 4, 2, 2, 2, 2, 2, 2, 2, 2, 2, 2, 2, 2, 2, 2, 2, 4 ),
 ( 2, 2 ),
 ( 0.000000000000000000, 0.06250000000000000000, 0.1250000000000000000, 0.1875000000000000000, 0.2500000000000000000, 0.3125000000000000000, 0.3750000000000000000, 0.4375000000000000000, 0.5000000000000000000, 0.5625000000000000000, 0.6250000000000000000, 0.6875000000000000000, 0.7500000000000000000, 0.8125000000000000000, 0.8750000000000000000, 0.9375000000000000000, 1.000000000000000000 ),
 ( 0.000000000000000000, 1.000000000000000000 ),
 .UNSPECIFIED. ) ;
#44356=DIRECTION ( 'NONE',  ( 0.8660254037844395958, 0.4999999999999985567, 0.000000000000000000 ) ) ;
#44359=CARTESIAN_POINT ( 'NONE',  ( 175.6186723166894126, 290.9646728346197619, 2.631908926450905017 ) ) ;
#44361=CARTESIAN_POINT ( 'NONE',  ( 202.7395715537438150, 279.4917566946068064, -16.55506732176026219 ) ) ;
#44363=CARTESIAN_POINT ( 'NONE',  ( 153.1852539850606547, 279.2954070424707993, 3.897478566824396307 ) ) ;
#44365=CARTESIAN_POINT ( 'NONE',  ( 24.64070123457955219, 185.0333772461660544, 9.188101187500095079 ) ) ;
#44366=CARTESIAN_POINT ( 'NONE',  ( 120.7155680147981940, 234.3768266524159856, 9.188101187500098632 ) ) ;
#44367=CARTESIAN_POINT ( 'NONE',  ( 45.14796862286864609, 185.3262482093457209, 3.021315404115420679E-15 ) ) ;
#44370=EDGE_CURVE ( 'NONE', #53564, #38420, #75671, .T. ) ;
#44371=CARTESIAN_POINT ( 'NONE',  ( 177.1851337456532178, 282.7301262368820858, -14.31388644062017690 ) ) ;
#44372=CARTESIAN_POINT ( 'NONE',  ( 154.9344967692067598, 262.2925750810547356, 17.30210568643136781 ) ) ;
#44373=CARTESIAN_POINT ( 'NONE',  ( 207.2707369601997982, 271.6435479931266173, -5.381413637561199614 ) ) ;
#44374=CARTESIAN_POINT ( 'NONE',  ( 148.0637215040603394, 274.1931069276759558, -7.795633835291665648 ) ) ;
#44375=EDGE_CURVE ( 'NONE', #93452, #35100, #12035, .T. ) ;
#44377=CARTESIAN_POINT ( 'NONE',  ( 188.2332182273270291, 299.2236753513818712, -0.5858898820902108673 ) ) ;
#44379=CARTESIAN_POINT ( 'NONE',  ( 165.4117122400764401, 253.5151701492806069, -13.08392429282121050 ) ) ;
#44381=CARTESIAN_POINT ( 'NONE',  ( 175.4548110154385938, 265.3612680696711550, -15.70463155788832310 ) ) ;
#44382=CARTESIAN_POINT ( 'NONE',  ( 91.91987624320061911, 230.0024278399160949, 9.188101187500095079 ) ) ;
#44383=CARTESIAN_POINT ( 'NONE',  ( 207.8232941427535536, 270.6864908788566026, -6.505149060073906142 ) ) ;
#44385=CARTESIAN_POINT ( 'NONE',  ( 196.4982648257524147, 290.3020170531091821, 16.69353242256149628 ) ) ;
#44387=CARTESIAN_POINT ( 'NONE',  ( 192.3589614934448946, 289.7923222231842715, -16.44823055510686771 ) ) ;
#44391=CARTESIAN_POINT ( 'NONE',  ( 193.1028332910263998, 296.1830769848763225, -12.04975758233223893 ) ) ;
#44396=CARTESIAN_POINT ( 'NONE',  ( 197.0600256462842026, 267.5279731586389858, 9.811020786235678415 ) ) ;
#44397=CARTESIAN_POINT ( 'NONE',  ( 187.9898463188184223, 285.9731239514064214, -16.38654393692524991 ) ) ;
#44403=ADVANCED_FACE ( 'NONE', ( #20613 ), #21499, .F. ) ;
#44404=CARTESIAN_POINT ( 'NONE',  ( 173.1900044977692232, 253.8258194800205274, -9.054949657387052042 ) ) ;
#44406=CARTESIAN_POINT ( 'NONE',  ( 144.7205361298395871, 254.3615022471902307, -10.00000000000009592 ) ) ;
#44407=CARTESIAN_POINT ( 'NONE',  ( 157.4893260420801653, 257.8674809757739013, -18.30842125257398223 ) ) ;
#44409=CARTESIAN_POINT ( 'NONE',  ( 95.64807497750081211, 214.4824982072973683, 3.021315404115420679E-15 ) ) ;
#44410=B_SPLINE_SURFACE_WITH_KNOTS ( 'NONE', 3, 1, ( 
 ( #87236, #63356 ),
 ( #79096, #33459 ),
 ( #56751, #63852 ),
 ( #94295, #47640 ),
 ( #70451, #40541 ),
 ( #62844, #24849 ),
 ( #48153, #56243 ),
 ( #93799, #79604 ),
 ( #17248, #25350 ),
 ( #70974, #17770 ),
 ( #95812, #41034 ),
 ( #64355, #9680 ),
 ( #71475, #1576 ),
 ( #55724, #24360 ),
 ( #55231, #86214 ),
 ( #86712, #16752 ),
 ( #32459, #78574 ),
 ( #87733, #18271 ),
 ( #9158, #94791 ),
 ( #2575, #71971 ),
 ( #49165, #2068 ),
 ( #32948, #80101 ),
 ( #48671, #10667 ),
 ( #72488, #3090 ),
 ( #33981, #64865 ),
 ( #26366, #85718 ),
 ( #28339, #12672 ),
 ( #82604, #13170 ),
 ( #34454, #80603 ),
 ( #96801, #5059 ),
 ( #96291, #73962 ),
 ( #3573, #67340 ),
 ( #89222, #44024 ),
 ( #19285, #59217 ) ),
 .UNSPECIFIED., .T., .F., .F.,
 ( 4, 2, 2, 2, 2, 2, 2, 2, 2, 2, 2, 2, 2, 2, 2, 2, 4 ),
 ( 2, 2 ),
 ( 0.000000000000000000, 0.06250000000000000000, 0.1250000000000000000, 0.1875000000000000000, 0.2500000000000000000, 0.3125000000000000000, 0.3750000000000000000, 0.4375000000000000000, 0.5000000000000000000, 0.5625000000000000000, 0.6250000000000000000, 0.6875000000000000000, 0.7500000000000000000, 0.8125000000000000000, 0.8750000000000000000, 0.9375000000000000000, 1.000000000000000000 ),
 ( 0.000000000000000000, 1.000000000000000000 ),
 .UNSPECIFIED. ) ;
#44412=CARTESIAN_POINT ( 'NONE',  ( 202.8499463704053198, 279.3005819042728604, 17.04674939340617001 ) ) ;
#44414=EDGE_CURVE ( 'NONE', #18565, #10368, #62279, .T. ) ;
#44418=ORIENTED_EDGE ( 'NONE', *, *, #47040, .F. ) ;
#44419=DIRECTION ( 'NONE',  ( 0.4999999999999998890, -0.8660254037844385966, 0.000000000000000000 ) ) ;
#44420=CARTESIAN_POINT ( 'NONE',  ( 205.5942821894498422, 274.5472528326565680, 11.03599490385640003 ) ) ;
#44421=CARTESIAN_POINT ( 'NONE',  ( 190.5112993737188560, 278.7663833916702174, -16.51125563584619726 ) ) ;
#44422=B_SPLINE_CURVE_WITH_KNOTS ( 'NONE', 3,
 ( #54396, #93967, #24520, #31111, #78739, #84863, #99543, #16917, #78240, #30632, #8821, #93466, #23504, #85372, #23010, #39197 ),
 .UNSPECIFIED., .F., .F.,
 ( 4, 2, 2, 2, 2, 2, 2, 4 ),
 ( 0.002922212478766483476, 0.003107388242815427911, 0.003199976124839900345, 0.003292564006864372780, 0.003477739770913328490, 0.003662915534962284635, 0.004403618591158125692, 0.005885024703549807806 ),
 .UNSPECIFIED. ) ;
#44423=CARTESIAN_POINT ( 'NONE',  ( 153.6416917630915862, 264.5317790359255810, -18.09859318578890708 ) ) ;
#44424=CARTESIAN_POINT ( 'NONE',  ( 200.8147387322574957, 282.8256649374973790, -18.02438097732020239 ) ) ;
#44429=CARTESIAN_POINT ( 'NONE',  ( 62.54379424586281289, 218.4637435831424739, 2.679491924311251605 ) ) ;
#44430=ORIENTED_EDGE ( 'NONE', *, *, #52211, .T. ) ;
#44431=ORIENTED_EDGE ( 'NONE', *, *, #9240, .F. ) ;
#44433=CARTESIAN_POINT ( 'NONE',  ( 164.4272222519600746, 245.8506922426221593, 7.021336339662529902 ) ) ;
#44434=CARTESIAN_POINT ( 'NONE',  ( 164.1635987429686736, 273.1024144199500370, -15.31708653229989814 ) ) ;
#44435=CARTESIAN_POINT ( 'NONE',  ( 204.1633547645365638, 275.3510256380408237, 13.36249479004741580 ) ) ;
#44436=CARTESIAN_POINT ( 'NONE',  ( 200.7780343897620980, 274.8121090555061983, -13.81066045772921314 ) ) ;
#44439=CARTESIAN_POINT ( 'NONE',  ( 167.0623087134214302, 286.3931234802170707, -4.864607199251016922 ) ) ;
#44440=CARTESIAN_POINT ( 'NONE',  ( 165.8284142803885857, 265.9971752285911180, 17.07883704590099327 ) ) ;
#44441=CARTESIAN_POINT ( 'NONE',  ( 178.1291671650300543, 255.4875147564563065, 4.904221248299380775 ) ) ;
#44442=CARTESIAN_POINT ( 'NONE',  ( 113.9495709998497688, 236.5958772461660544, -9.188101187500095079 ) ) ;
#44443=CARTESIAN_POINT ( 'NONE',  ( 148.0510481135471252, 274.9194765995500802, -5.872114088031683110 ) ) ;
#44444=CARTESIAN_POINT ( 'NONE',  ( 188.3599285997746051, 273.5439987038621439, 15.65562976607134260 ) ) ;
#44446=B_SPLINE_CURVE_WITH_KNOTS ( 'NONE', 3,
 ( #43669, #13301, #11806, #28470 ),
 .UNSPECIFIED., .F., .F.,
 ( 4, 4 ),
 ( 0.01303476720425170501, 0.02161825251906693626 ),
 .UNSPECIFIED. ) ;
#44448=CARTESIAN_POINT ( 'NONE',  ( 164.4286791602839912, 246.2317698387275300, -2.006671165488138175 ) ) ;
#44449=CARTESIAN_POINT ( 'NONE',  ( 157.3988263959001870, 258.0242309610243865, 16.72376558639979294 ) ) ;
#44453=CARTESIAN_POINT ( 'NONE',  ( -17.42236680055705023, 149.2012482093457777, 0.000000000000000000 ) ) ;
#44460=CARTESIAN_POINT ( 'NONE',  ( 158.0966096247271366, 263.1875288115938929, 17.28628307208229842 ) ) ;
#44461=CYLINDRICAL_SURFACE ( 'NONE', #59686, 10.00000000000010658 ) ;
#44462=CARTESIAN_POINT ( 'NONE',  ( 185.1766543017484139, 289.3992658934859037, -13.22389641140907024 ) ) ;
#44466=CARTESIAN_POINT ( 'NONE',  ( 190.2236813008869660, 301.1699145145108218, -5.401374690107298093 ) ) ;
#44469=CARTESIAN_POINT ( 'NONE',  ( 170.0428130633470687, 248.7678227811192926, -0.2667965012368537780 ) ) ;
#44478=CARTESIAN_POINT ( 'NONE',  ( 74.46396492422927338, 222.9869531367911293, 4.594050593750046652 ) ) ;
#44479=CARTESIAN_POINT ( 'NONE',  ( 206.2313482792274328, 273.4438219973828268, -9.403385562213845361 ) ) ;
#44480=DIRECTION ( 'NONE',  ( -0.8660254037844387076, -0.4999999999999998890, -0.000000000000000000 ) ) ;
#44481=CARTESIAN_POINT ( 'NONE',  ( 162.6541320028305506, 248.9217746405196294, -10.16950121496441817 ) ) ;
#44482=B_SPLINE_CURVE_WITH_KNOTS ( 'NONE', 3,
 ( #48984, #63170, #87040, #94114 ),
 .UNSPECIFIED., .F., .F.,
 ( 4, 4 ),
 ( 0.01172131844875056762, 0.02019504072144193141 ),
 .UNSPECIFIED. ) ;
#44483=CARTESIAN_POINT ( 'NONE',  ( 196.6222993919940905, 288.9791602159129411, -16.90160481779407320 ) ) ;
#44484=CARTESIAN_POINT ( 'NONE',  ( 207.3646600298985447, 271.4808684644054324, -5.284084612275558257 ) ) ;
#44485=CARTESIAN_POINT ( 'NONE',  ( 165.0179060354396370, 286.2867116390483488, 3.417988829560836272 ) ) ;
#44487=CARTESIAN_POINT ( 'NONE',  ( 185.9406580756425171, 265.4572926502605128, 14.02042132963198817 ) ) ;
#44491=CARTESIAN_POINT ( 'NONE',  ( 157.2744851780909414, 258.2395962677452985, 18.17792129701959070 ) ) ;
#44493=CARTESIAN_POINT ( 'NONE',  ( 23.34166312890287998, 184.2833772461660544, -9.188101187500095079 ) ) ;
#44495=CARTESIAN_POINT ( 'NONE',  ( 187.4171132689631634, 261.5282790321019206, -9.397869408254909018 ) ) ;
#44497=CARTESIAN_POINT ( 'NONE',  ( 194.2900850603946310, 294.1266965989547657, -15.88613936555681505 ) ) ;
#44499=CARTESIAN_POINT ( 'NONE',  ( 43.96371950863733247, 202.3149278399160949, -9.188101187500095079 ) ) ;
#44506=CARTESIAN_POINT ( 'NONE',  ( 202.5450565896906596, 269.8107279373824099, -6.424806493487884573 ) ) ;
#44507=CARTESIAN_POINT ( 'NONE',  ( 175.7185668582631592, 291.0393361692799772, 2.533717797835123964 ) ) ;
#44508=CARTESIAN_POINT ( 'NONE',  ( 176.2779124731408444, 274.9878774502150236, 17.29739640835781245 ) ) ;
#44513=CARTESIAN_POINT ( 'NONE',  ( 87.63502826371527021, 234.7365022471903444, 2.944929066748280225E-16 ) ) ;
#44514=CARTESIAN_POINT ( 'NONE',  ( 161.6673510627899191, 250.6309293646106653, 13.01175935005004192 ) ) ;
#44515=CARTESIAN_POINT ( 'NONE',  ( 165.1836928371452018, 269.6304300936849359, -16.29016501675020123 ) ) ;
#44517=CARTESIAN_POINT ( 'NONE',  ( 49.53858449761714411, 211.6589784336661637, -6.496448406907675876E-16 ) ) ;
#44518=EDGE_LOOP ( 'NONE', ( #54182, #30922, #55240 ) ) ;
#44520=CARTESIAN_POINT ( 'NONE',  ( 146.8881680668833951, 276.2292252078784145, 4.973452195244782104 ) ) ;
#44521=CYLINDRICAL_SURFACE ( 'NONE', #75852, 17.82106496071139645 ) ;
#44522=ORIENTED_EDGE ( 'NONE', *, *, #50435, .F. ) ;
#44526=CARTESIAN_POINT ( 'NONE',  ( 176.9245165359646990, 274.6851866283708432, -17.45875439271293317 ) ) ;
#44528=CARTESIAN_POINT ( 'NONE',  ( 204.6163864379986705, 276.2410179586759682, 14.66911174422491726 ) ) ;
#44529=ORIENTED_EDGE ( 'NONE', *, *, #97601, .F. ) ;
#44533=CARTESIAN_POINT ( 'NONE',  ( 154.2194984598485519, 265.5309884801890234, 17.12742652472672944 ) ) ;
#44538=VERTEX_POINT ( 'NONE', #96036 ) ;
#44539=( BOUNDED_CURVE ( )  B_SPLINE_CURVE ( 2, ( #26207, #18613, #65199, #49490, #26701, #88561, #19126, #14492, #83928 ),
 .UNSPECIFIED., .F., .T. ) 
 B_SPLINE_CURVE_WITH_KNOTS ( ( 3, 2, 2, 2, 3 ),
 ( 0.09274193548387096864, 0.09408602150537634379, 0.09677419354838709409, 0.09946236559139784439, 0.1008064516129032334 ),
 .UNSPECIFIED. ) 
 CURVE ( )  GEOMETRIC_REPRESENTATION_ITEM ( )  RATIONAL_B_SPLINE_CURVE ( ( 0.9330127018922194093, 0.9330127018922194093, 1.000000000000000000, 0.8660254037844387076, 1.000000000000000000, 0.8660254037844387076, 1.000000000000000000, 0.9330127018922189652, 0.9330127018922192983 ) ) 
 REPRESENTATION_ITEM ( '' )  );
#44540=CARTESIAN_POINT ( 'NONE',  ( 170.4623819437503016, 288.8056674672355939, -5.476885062779371260 ) ) ;
#44541=CARTESIAN_POINT ( 'NONE',  ( 20.85854946042532276, 194.3967562850347122, -4.648177544792955347E-16 ) ) ;
#44542=CARTESIAN_POINT ( 'NONE',  ( 162.8223739550644211, 248.6303710312858186, -11.16939803179192658 ) ) ;
#44544=CARTESIAN_POINT ( 'NONE',  ( 188.0431710233438309, 294.4895058550014824, -10.95648900967039197 ) ) ;
#44546=CARTESIAN_POINT ( 'NONE',  ( 205.5791761573774181, 272.5734172477073116, 10.13670412909801044 ) ) ;
#44548=CARTESIAN_POINT ( 'NONE',  ( 120.0114017305758267, 252.3464784336661353, 1.353441290958777525E-15 ) ) ;
#44549=CARTESIAN_POINT ( 'NONE',  ( 76.00665944866153723, 220.8149278399160664, 9.188101187500093303 ) ) ;
#44550=EDGE_LOOP ( 'NONE', ( #88976, #67263, #35747, #55180 ) ) ;
#44551=CARTESIAN_POINT ( 'NONE',  ( 170.4098397670617828, 263.7867033673382480, 15.85021430837907630 ) ) ;
#44553=VERTEX_POINT ( 'NONE', #3798 ) ;
#44554=CARTESIAN_POINT ( 'NONE',  ( 200.5237418414733384, 281.6908991433180631, 17.12490243155320613 ) ) ;
#44559=CARTESIAN_POINT ( 'NONE',  ( -6.699655929326435277, 178.4860189848785410, -2.679491924311252493 ) ) ;
#44562=CARTESIAN_POINT ( 'NONE',  ( 194.3252252352508265, 294.0658320307167628, 14.07225870721148731 ) ) ;
#44567=CARTESIAN_POINT ( 'NONE',  ( 200.6583719735737645, 283.0965001081523269, -17.35266956530146132 ) ) ;
#44568=CARTESIAN_POINT ( 'NONE',  ( 189.4308808934198680, 289.8491723414206831, 15.72891001903047048 ) ) ;
#44569=EDGE_LOOP ( 'NONE', ( #59358, #59970, #45593, #65247 ) ) ;
#44574=CARTESIAN_POINT ( 'NONE',  ( 164.9171241593586217, 245.0021572482830550, 1.622680932994367220 ) ) ;
#44576=CARTESIAN_POINT ( 'NONE',  ( 46.85966550219804816, 187.8615022471902023, 5.000000000000051514 ) ) ;
#44577=CARTESIAN_POINT ( 'NONE',  ( 163.9354095869165633, 246.7025367662834014, -7.289870401565430313 ) ) ;
#44578=CARTESIAN_POINT ( 'NONE',  ( 136.6287848093373043, 243.5643266524160140, 9.188101187500095079 ) ) ;
#44581=CARTESIAN_POINT ( 'NONE',  ( 182.4211569912797586, 258.2722588617187967, 6.464551942522600569 ) ) ;
#44582=CARTESIAN_POINT ( 'NONE',  ( 179.8841377953208109, 288.3657013325343428, -13.30019851817003307 ) ) ;
#44588=CARTESIAN_POINT ( 'NONE',  ( 184.3179147726750386, 277.0395465893940354, -16.62992345926578253 ) ) ;
#44589=CARTESIAN_POINT ( 'NONE',  ( 167.9496373820661290, 248.6204696539478789, -6.517719931589019744 ) ) ;
#44592=CARTESIAN_POINT ( 'NONE',  ( 195.9531395617315752, 264.6018537701219202, 0.8289104891173008083 ) ) ;
#44593=CARTESIAN_POINT ( 'NONE',  ( 146.8058449195592061, 276.3718130816831149, 4.181814292810413392 ) ) ;
#44596=CARTESIAN_POINT ( 'NONE',  ( 204.6149525604204769, 276.2435015074934199, -13.22810747389629960 ) ) ;
#44597=CARTESIAN_POINT ( 'NONE',  ( 196.2612106832813481, 270.7781520464870937, 11.97022677330632412 ) ) ;
#44601=CARTESIAN_POINT ( 'NONE',  ( -22.42236680055709641, 157.8615022471902591, 0.000000000000000000 ) ) ;
#44603=CARTESIAN_POINT ( 'NONE',  ( 198.6755293322981117, 286.5308843062557571, 17.86676876308990103 ) ) ;
#44604=CARTESIAN_POINT ( 'NONE',  ( 207.5570812576139303, 271.1475851215477064, 6.450149787450828676 ) ) ;
#44605=CARTESIAN_POINT ( 'NONE',  ( -11.38080322590321281, 173.4244531367911293, -4.594050593750046652 ) ) ;
#44606=CARTESIAN_POINT ( 'NONE',  ( 176.0078709123280589, 285.3975443765536397, -11.99210929984988816 ) ) ;
#44610=CARTESIAN_POINT ( 'NONE',  ( 150.9584389135710865, 269.1793093008492406, -15.82751450793727699 ) ) ;
#44611=CARTESIAN_POINT ( 'NONE',  ( -2.422939729449180124, 181.6589784336661637, -6.496448406907676862E-16 ) ) ;
#44612=EDGE_CURVE ( 'NONE', #62907, #99632, #64832, .T. ) ;
#44613=CARTESIAN_POINT ( 'NONE',  ( 178.4187001493748426, 273.6290048830982755, -17.20285326387372038 ) ) ;
#44616=CARTESIAN_POINT ( 'NONE',  ( 67.91490812815924016, 210.0177522451418497, -10.00000000000009592 ) ) ;
#44619=CARTESIAN_POINT ( 'NONE',  ( 198.6654679441890892, 270.7080073051427007, -10.97714029729529983 ) ) ;
#44620=CARTESIAN_POINT ( 'NONE',  ( 69.21394623383588396, 220.7677522451419065, -5.000000000000047962 ) ) ;
#44621=CARTESIAN_POINT ( 'NONE',  ( 175.9315981478186472, 252.7514783800165503, -3.278135643623982354 ) ) ;
#44622=CARTESIAN_POINT ( 'NONE',  ( 150.2761558193201381, 270.3610582852369930, 14.81920478290713028 ) ) ;
#44623=ADVANCED_FACE ( 'NONE', ( #9752 ), #83831, .F. ) ;
#44624=CARTESIAN_POINT ( 'NONE',  ( 61.58209736653347477, 206.3615022471902307, -10.00000000000009592 ) ) ;
#44626=CARTESIAN_POINT ( 'NONE',  ( 148.4049257185216106, 273.6021238924720365, 8.639190357831699529 ) ) ;
#44627=CARTESIAN_POINT ( 'NONE',  ( 23.96437920969670898, 175.4548013555409796, -4.594050593750042211 ) ) ;
#44630=CARTESIAN_POINT ( 'NONE',  ( 153.3127735718713609, 265.1014820546527631, 17.57722645152040641 ) ) ;
#44634=CARTESIAN_POINT ( 'NONE',  ( 185.2853394675401830, 266.6322772215058876, 13.29842321144261774 ) ) ;
#44638=CARTESIAN_POINT ( 'NONE',  ( 147.8503508990560533, 274.5626756563852950, 7.845851077393495743 ) ) ;
#44642=CARTESIAN_POINT ( 'NONE',  ( 155.2419697281468416, 261.7600162942170527, 18.58580762350309357 ) ) ;
#44643=ORIENTED_EDGE ( 'NONE', *, *, #63101, .T. ) ;
#44644=CARTESIAN_POINT ( 'NONE',  ( 181.6645495853941839, 289.2224369541009992, 12.52750095734821123 ) ) ;
#44652=CARTESIAN_POINT ( 'NONE',  ( 203.0026270830780675, 279.0361311525880978, -16.61345826058821373 ) ) ;
#44656=CARTESIAN_POINT ( 'NONE',  ( 164.2851776226980860, 246.0967207574460929, 5.847738044744511754 ) ) ;
#44657=VERTEX_POINT ( 'NONE', #19835 ) ;
#44658=CARTESIAN_POINT ( 'NONE',  ( 150.8757650385446993, 269.3225046528533539, 14.31332712971473953 ) ) ;
#44663=CARTESIAN_POINT ( 'NONE',  ( 156.0916382163451601, 277.5285333452508212, -10.52960063827285886 ) ) ;
#44665=CARTESIAN_POINT ( 'NONE',  ( 164.3022921857394749, 246.0670774647090582, 1.862798784958315856 ) ) ;
#44668=B_SPLINE_CURVE_WITH_KNOTS ( 'NONE', 3,
 ( #56191, #32408, #8120, #94247 ),
 .UNSPECIFIED., .F., .F.,
 ( 4, 4 ),
 ( 0.008701075091435968994, 0.01503270840399712274 ),
 .UNSPECIFIED. ) ;
#44670=EDGE_CURVE ( 'NONE', #82029, #3452, #89576, .T. ) ;
#44671=CARTESIAN_POINT ( 'NONE',  ( 190.6661865267473104, 300.4034729807058852, 4.523489664447863490 ) ) ;
#44672=CARTESIAN_POINT ( 'NONE',  ( 172.2817675467364609, 263.9987076400973933, -16.71829096631468659 ) ) ;
#44674=CARTESIAN_POINT ( 'NONE',  ( 158.6532002544261104, 274.8663221026905603, -12.72708391612727574 ) ) ;
#44675=CARTESIAN_POINT ( 'NONE',  ( 187.4061870533930971, 294.1816329134088619, 12.04041381263369814 ) ) ;
#44677=CARTESIAN_POINT ( 'NONE',  ( 170.5993847053230468, 287.8722104901659691, 7.679145147933459370 ) ) ;
#44682=FACE_OUTER_BOUND ( 'NONE', #79379, .T. ) ;
#44684=CARTESIAN_POINT ( 'NONE',  ( 149.0323968763055689, 272.5153119669064949, 11.64231532207353403 ) ) ;
#44685=CARTESIAN_POINT ( 'NONE',  ( 152.7531861616124615, 266.0707158804971186, 17.45453282433162556 ) ) ;
#44687=CARTESIAN_POINT ( 'NONE',  ( 146.8175579285427546, 276.3515255550140068, 0.7851837772504086654 ) ) ;
#44688=EDGE_CURVE ( 'NONE', #36928, #71064, #38246, .T. ) ;
#44689=CARTESIAN_POINT ( 'NONE',  ( 191.1687199697037443, 299.5330595250031820, -8.491751560014430211 ) ) ;
#44690=ORIENTED_EDGE ( 'NONE', *, *, #37574, .F. ) ;
#44693=CARTESIAN_POINT ( 'NONE',  ( 196.9976074755333286, 289.4371302133026802, -16.79549473444794216 ) ) ;
#44695=CARTESIAN_POINT ( 'NONE',  ( 169.5742172260261214, 287.1141421671970875, 4.090594757681383697 ) ) ;
#44697=CARTESIAN_POINT ( 'NONE',  ( 104.8295012880686699, 222.1423013555409796, -4.594050593750043987 ) ) ;
#44699=CARTESIAN_POINT ( 'NONE',  ( 149.3744903853108212, 271.9227886283697444, -13.09816371469833740 ) ) ;
#44701=CARTESIAN_POINT ( 'NONE',  ( 149.1694037875916194, 273.2954204789498363, 9.972691433298622954 ) ) ;
#44703=CARTESIAN_POINT ( 'NONE',  ( 38.92905753611409381, 204.8297689869269220, -2.679491924311252493 ) ) ;
#44706=CARTESIAN_POINT ( 'NONE',  ( 169.0084691738961737, 254.5285646557595669, -11.70697648969032301 ) ) ;
#44708=CARTESIAN_POINT ( 'NONE',  ( 206.9059968923335475, 272.2752963222270068, 6.902135944297345560 ) ) ;
#44709=CARTESIAN_POINT ( 'NONE',  ( 47.13029843733273339, 198.0177522451418781, -10.00000000000009592 ) ) ;
#44710=CARTESIAN_POINT ( 'NONE',  ( 114.4904897814500373, 249.1589784336661069, -6.496448406907676862E-16 ) ) ;
#44713=DIRECTION ( 'NONE',  ( 0.4999999999999998890, -0.8660254037844385966, 0.000000000000000000 ) ) ;
#44714=CARTESIAN_POINT ( 'NONE',  ( 172.9698904924519240, 250.6642211707864476, -4.168778760986519671 ) ) ;
#44715=CARTESIAN_POINT ( 'NONE',  ( 36.16949087457737733, 197.8149278399160949, -9.188101187500095079 ) ) ;
#44716=CIRCLE ( 'NONE', #14006, 17.82106496071138224 ) ;
#44718=AXIS2_PLACEMENT_3D ( 'NONE', #58418, #88907, #19470 ) ;
#44719=ORIENTED_EDGE ( 'NONE', *, *, #9126, .F. ) ;
#44724=CARTESIAN_POINT ( 'NONE',  ( 190.7403173041394950, 300.2750747078583800, -4.254144485856557800 ) ) ;
#44727=CARTESIAN_POINT ( 'NONE',  ( 179.3575481875710693, 287.7525672830279291, -12.49454744750270585 ) ) ;
#44728=CARTESIAN_POINT ( 'NONE',  ( 164.3438181478333036, 250.0973453384040113, 10.21369496864028292 ) ) ;
#44729=CARTESIAN_POINT ( 'NONE',  ( 112.9482291249501174, 226.0177522451418213, 5.000000000000051514 ) ) ;
#44732=CARTESIAN_POINT ( 'NONE',  ( 202.7041331321765938, 279.5531378413010657, 17.14708438049711248 ) ) ;
#44735=AXIS2_PLACEMENT_3D ( 'NONE', #63450, #93894, #62424 ) ;
#44736=CARTESIAN_POINT ( 'NONE',  ( 4.207654042216683266, 182.4244531367911293, -4.594050593750046652 ) ) ;
#44739=CARTESIAN_POINT ( 'NONE',  ( 192.2315437480665992, 272.1294165976894988, 14.32756029153346056 ) ) ;
#44742=CARTESIAN_POINT ( 'NONE',  ( 195.2495212664957194, 275.1290853193528392, -16.26662379558266380 ) ) ;
#44743=CARTESIAN_POINT ( 'NONE',  ( 59.17381130624904273, 192.7202760586659736, -5.415160957724236172E-17 ) ) ;
#44744=EDGE_CURVE ( 'NONE', #20065, #39184, #11740, .T. ) ;
#44745=CARTESIAN_POINT ( 'NONE',  ( 207.5215400641004351, 271.2091442744748520, 2.886080616848571534 ) ) ;
#44751=CARTESIAN_POINT ( 'NONE',  ( 16.62094515339138212, 173.7365022471902307, 10.00000000000009592 ) ) ;
#44752=B_SPLINE_CURVE_WITH_KNOTS ( 'NONE', 3,
 ( #41512, #73929, #34424, #65324 ),
 .UNSPECIFIED., .F., .F.,
 ( 4, 4 ),
 ( 0.01189126407362384348, 0.01800151522966263185 ),
 .UNSPECIFIED. ) ;
#44753=CARTESIAN_POINT ( 'NONE',  ( 164.0179800784044915, 246.5595204798204065, -5.772998092557310557 ) ) ;
#44754=CARTESIAN_POINT ( 'NONE',  ( 131.5133883985292016, 255.9244531367911293, -4.594050593750046652 ) ) ;
#44756=CARTESIAN_POINT ( 'NONE',  ( 165.0728006432024699, 244.7325176687217549, 1.503174307937145793 ) ) ;
#44758=CARTESIAN_POINT ( 'NONE',  ( -17.42236680055705023, 149.2012482093457777, 0.000000000000000000 ) ) ;
#44759=CARTESIAN_POINT ( 'NONE',  ( 203.3946109532447224, 276.3571951737117729, -14.55139583984842133 ) ) ;
#44763=ORIENTED_EDGE ( 'NONE', *, *, #65679, .F. ) ;
#44765=CARTESIAN_POINT ( 'NONE',  ( 207.8229629847965612, 270.6870644612629917, -0.3253519274997035415 ) ) ;
#44768=CARTESIAN_POINT ( 'NONE',  ( 197.3243759857185182, 273.2497805167799356, -13.42310424059574636 ) ) ;
#44769=ORIENTED_EDGE ( 'NONE', *, *, #9594, .F. ) ;
#44772=EDGE_CURVE ( 'NONE', #33315, #71254, #69660, .T. ) ;
#44775=CARTESIAN_POINT ( 'NONE',  ( 172.4831635826484444, 290.8796410925290843, -1.652085212636280609 ) ) ;
#44778=CARTESIAN_POINT ( 'NONE',  ( 153.0790963368640689, 265.5062228982576471, -17.74594954892339160 ) ) ;
#44779=ORIENTED_EDGE ( 'NONE', *, *, #53702, .F. ) ;
#44784=CARTESIAN_POINT ( 'NONE',  ( 190.5477107455830321, 300.6086790531491033, 3.126266616601216963 ) ) ;
#44785=FACE_OUTER_BOUND ( 'NONE', #97971, .T. ) ;
#44786=CARTESIAN_POINT ( 'NONE',  ( 189.1342855833499925, 297.0966903347303969, 8.133747755478912822 ) ) ;
#44788=CARTESIAN_POINT ( 'NONE',  ( 191.4852287632733123, 298.9848502134979071, -9.870565261052552941 ) ) ;
#44791=CARTESIAN_POINT ( 'NONE',  ( 204.2129321040862919, 276.9398213635460024, 14.41515352680879758 ) ) ;
#44792=CARTESIAN_POINT ( 'NONE',  ( 46.83931157395847578, 209.3967562850346837, 1.101618078115930403E-13 ) ) ;
#44794=CARTESIAN_POINT ( 'NONE',  ( 82.14994038281616895, 227.4244531367911293, -4.594050593750046652 ) ) ;
#44795=CARTESIAN_POINT ( 'NONE',  ( 203.5644143473884071, 278.0630870677574649, 15.19023846038192183 ) ) ;
#44797=CARTESIAN_POINT ( 'NONE',  ( 181.2813888893848571, 271.4291121770711470, -16.07812310781979548 ) ) ;
#44800=EDGE_CURVE ( 'NONE', #13224, #86658, #62474, .T. ) ;
#44801=ORIENTED_EDGE ( 'NONE', *, *, #29347, .T. ) ;
#44804=ORIENTED_EDGE ( 'NONE', *, *, #20350, .F. ) ;
#44807=ADVANCED_FACE ( 'NONE', ( #11127 ), #43282, .F. ) ;
#44813=EDGE_CURVE ( 'NONE', #63549, #79661, #82552, .T. ) ;
#44814=CARTESIAN_POINT ( 'NONE',  ( 165.0528804069804494, 264.4852527057752241, -17.76608744198970768 ) ) ;
#44816=CARTESIAN_POINT ( 'NONE',  ( -22.42236680055709641, 157.8615022471902591, 0.000000000000000000 ) ) ;
#44819=EDGE_CURVE ( 'NONE', #6345, #12659, #91623, .T. ) ;
#44820=CARTESIAN_POINT ( 'NONE',  ( 166.8217491802902259, 284.2403532778428712, 9.447065769108251132 ) ) ;
#44822=CARTESIAN_POINT ( 'NONE',  ( 119.8764323552255604, 240.0177522451418497, -10.00000000000009592 ) ) ;
#44825=CARTESIAN_POINT ( 'NONE',  ( 163.0171530587457767, 248.2930037274571191, 9.677214176418313940 ) ) ;
#44828=CARTESIAN_POINT ( 'NONE',  ( 185.8333456925277289, 259.2190590162801982, 2.892714555682415867 ) ) ;
#44829=CARTESIAN_POINT ( 'NONE',  ( 157.6030016657039994, 279.9469238675063139, -6.853747175795008140 ) ) ;
#44832=CARTESIAN_POINT ( 'NONE',  ( 161.1611771195837548, 251.5076483517112536, 14.17749514252127163 ) ) ;
#44833=CARTESIAN_POINT ( 'NONE',  ( 160.2158583160598653, 282.4101726736743672, 2.089109771773170365 ) ) ;
#44836=CARTESIAN_POINT ( 'NONE',  ( 194.5990735076113936, 293.5915129094234430, -15.16177817946606865 ) ) ;
#44837=CARTESIAN_POINT ( 'NONE',  ( 160.3456795905085812, 276.2092357212747515, 12.64195674795301727 ) ) ;
#44838=CARTESIAN_POINT ( 'NONE',  ( 3.829028248110833754, 163.0177522451418213, 5.000000000000051514 ) ) ;
#44839=CARTESIAN_POINT ( 'NONE',  ( 192.9426967849980485, 267.3039850408317193, -11.05276717515422114 ) ) ;
#44840=CARTESIAN_POINT ( 'NONE',  ( 172.0926279537021344, 280.4607217264099290, -15.30784906875749840 ) ) ;
#44841=CARTESIAN_POINT ( 'NONE',  ( 203.4577257922414333, 278.2478770658579492, -15.05669205718196402 ) ) ;
#44843=CARTESIAN_POINT ( 'NONE',  ( 164.6063343576543048, 274.4739709976624908, 16.17759516952312637 ) ) ;
#44844=CARTESIAN_POINT ( 'NONE',  ( -2.801652295722365071, 175.3149278399160949, -9.188101187500095079 ) ) ;
#44845=CARTESIAN_POINT ( 'NONE',  ( 33.29424590502123493, 178.4824982072973683, 3.021315404115420679E-15 ) ) ;
#44846=CARTESIAN_POINT ( 'NONE',  ( 189.0285275759924559, 297.0242660314676755, 8.140054971467193923 ) ) ;
#44847=EDGE_LOOP ( 'NONE', ( #73757, #92572, #99055 ) ) ;
#44852=CARTESIAN_POINT ( 'NONE',  ( 63.33450210234187239, 195.8262482093458061, 3.021315404115420679E-15 ) ) ;
#44854=CARTESIAN_POINT ( 'NONE',  ( 150.0982468106783472, 276.6106350970345034, 3.452134251224849404 ) ) ;
#44855=CARTESIAN_POINT ( 'NONE',  ( 21.25804982287034406, 173.8923013555409796, 4.594050593750050204 ) ) ;
#44856=CARTESIAN_POINT ( 'NONE',  ( 117.0885659928033817, 250.6589784336661637, -6.496448406907675876E-16 ) ) ;
#44859=CARTESIAN_POINT ( 'NONE',  ( 206.5228006916347852, 272.3196060122579070, -7.607667339345448809 ) ) ;
#44864=CARTESIAN_POINT ( 'NONE',  ( 154.9226727788713731, 262.3130548330639726, 18.22497199616848818 ) ) ;
#44865=CARTESIAN_POINT ( 'NONE',  ( 161.4816992964961742, 250.9524876563463067, -12.92750327687364198 ) ) ;
#44866=CARTESIAN_POINT ( 'NONE',  ( 189.7876278749425580, 284.7637188201192089, 17.36559644418266757 ) ) ;
#44868=B_SPLINE_CURVE_WITH_KNOTS ( 'NONE', 3,
 ( #85975, #46387, #47396, #77312 ),
 .UNSPECIFIED., .F., .F.,
 ( 4, 4 ),
 ( 7.858125020761361721E-17, 0.007288700693340222428 ),
 .UNSPECIFIED. ) ;
#44872=CARTESIAN_POINT ( 'NONE',  ( 55.77019854693759271, 214.5530062829863311, -4.648177544792955347E-16 ) ) ;
#44875=CARTESIAN_POINT ( 'NONE',  ( 181.6437473107036169, 268.0140057806834761, 15.00620755021360964 ) ) ;
#44876=CARTESIAN_POINT ( 'NONE',  ( 95.92559083146868204, 220.0643266524159856, -9.188101187500093303 ) ) ;
#44883=CARTESIAN_POINT ( 'NONE',  ( 150.8247211172754589, 269.4109153179094278, -14.37608026040300402 ) ) ;
#44886=CARTESIAN_POINT ( 'NONE',  ( 192.5551423381268989, 297.1317055421444024, -13.20528585388119858 ) ) ;
#44892=CARTESIAN_POINT ( 'NONE',  ( 146.7842303614460207, 276.4092505945183689, -4.491116827832889236 ) ) ;
#44893=CARTESIAN_POINT ( 'NONE',  ( 149.7109319212262051, 271.3400547943878109, -12.38605961032017433 ) ) ;
#44895=VERTEX_POINT ( 'NONE', #94624 ) ;
#44898=CARTESIAN_POINT ( 'NONE',  ( 159.5204760365350012, 254.3494259875849082, 16.90107507090185379 ) ) ;
#44899=CARTESIAN_POINT ( 'NONE',  ( 171.9881733610453978, 253.5440279410006781, -8.835078667792725327 ) ) ;
#44900=CARTESIAN_POINT ( 'NONE',  ( 136.0602820919951341, 259.3615022471902876, 5.000000000000046185 ) ) ;
#44902=ORIENTED_EDGE ( 'NONE', *, *, #96675, .F. ) ;
#44903=CARTESIAN_POINT ( 'NONE',  ( 28.09809348231459936, 175.4824982072973967, 3.021315404115420679E-15 ) ) ;
#44907=EDGE_LOOP ( 'NONE', ( #36926, #74275, #16682, #1826 ) ) ;
#44908=CARTESIAN_POINT ( 'NONE',  ( 181.9468416852762971, 290.8932940152133142, -10.89979107759946153 ) ) ;
#44911=CARTESIAN_POINT ( 'NONE',  ( 206.3088856847695922, 273.3095232714966869, 11.40914494729949880 ) ) ;
#44913=CARTESIAN_POINT ( 'NONE',  ( 153.3548908812967966, 265.0285327348495912, -17.67588370404063625 ) ) ;
#44914=CARTESIAN_POINT ( 'NONE',  ( 200.6583719735737645, 283.0965001081523269, -17.35266956530146132 ) ) ;
#44917=CARTESIAN_POINT ( 'NONE',  ( 192.1943038168404314, 277.1473907896511264, 17.36549850453357635 ) ) ;
#44919=CARTESIAN_POINT ( 'NONE',  ( 62.42776884207837895, 218.3967562850346837, -4.648177544792955347E-16 ) ) ;
#44920=VERTEX_POINT ( 'NONE', #23667 ) ;
#44921=VERTEX_POINT ( 'NONE', #25181 ) ;
#44922=CARTESIAN_POINT ( 'NONE',  ( 205.1793861064249711, 275.2658739283173759, -14.08953480709093675 ) ) ;
#44926=CARTESIAN_POINT ( 'NONE',  ( 174.5179243658558335, 257.1845942475917468, -12.14858670780875904 ) ) ;
#44927=CARTESIAN_POINT ( 'NONE',  ( 165.9766573681747559, 274.1408043494670892, -15.16394994857281020 ) ) ;
#44928=CARTESIAN_POINT ( 'NONE',  ( 206.0061733044583434, 273.8338364942757153, -9.988470584493322590 ) ) ;
#44929=CARTESIAN_POINT ( 'NONE',  ( 197.5903643141157886, 272.8324856170032149, -13.22247203134994997 ) ) ;
#44930=CARTESIAN_POINT ( 'NONE',  ( 156.3551087084618700, 261.3239775484371989, -17.56576820129662053 ) ) ;
#44933=CARTESIAN_POINT ( 'NONE',  ( 170.3352017334123047, 289.0068553437270111, -4.481107825698984470 ) ) ;
#44936=CARTESIAN_POINT ( 'NONE',  ( 184.0013592068560229, 285.0434840400766348, -15.03075733970070083 ) ) ;
#44938=CARTESIAN_POINT ( 'NONE',  ( 109.2943373587434053, 246.1589784336661069, -6.496448406907675876E-16 ) ) ;
#44939=ORIENTED_EDGE ( 'NONE', *, *, #50862, .T. ) ;
#44940=CARTESIAN_POINT ( 'NONE',  ( 183.4673376644933853, 260.0777518357641611, -9.504335236147220201 ) ) ;
#44942=DIRECTION ( 'NONE',  ( 0.8660254037844395958, 0.4999999999999985567, 0.000000000000000000 ) ) ;
#44948=EDGE_CURVE ( 'NONE', #68820, #46298, #85543, .T. ) ;
#44949=B_SPLINE_SURFACE_WITH_KNOTS ( 'NONE', 3, 1, ( 
 ( #82616, #99762 ),
 ( #35951, #37434 ),
 ( #74977, #44036 ),
 ( #97781, #60722 ),
 ( #14657, #68345 ),
 ( #36948, #98781 ),
 ( #90203, #7047 ),
 ( #98278, #74491 ),
 ( #29364, #91685 ),
 ( #60230, #52637 ),
 ( #13665, #58738 ),
 ( #66852, #83593 ),
 ( #5558, #36444 ),
 ( #14157, #5069 ),
 ( #6561, #45044 ),
 ( #20777, #75987 ),
 ( #99269, #22247 ),
 ( #67349, #28865 ),
 ( #59743, #20274 ),
 ( #53149, #90713 ),
 ( #51148, #37927 ),
 ( #21268, #84104 ),
 ( #52146, #45534 ),
 ( #82111, #83095 ),
 ( #28349, #12684 ),
 ( #43551, #59228 ),
 ( #86610, #9571 ),
 ( #7543, #955 ),
 ( #32349, #69841 ),
 ( #94191, #31832 ),
 ( #78984, #85609 ),
 ( #93691, #38434 ),
 ( #454, #77469 ),
 ( #46026, #24254 ) ),
 .UNSPECIFIED., .T., .F., .F.,
 ( 4, 2, 2, 2, 2, 2, 2, 2, 2, 2, 2, 2, 2, 2, 2, 2, 4 ),
 ( 2, 2 ),
 ( 0.000000000000000000, 0.06250000000000000000, 0.1250000000000000000, 0.1875000000000000000, 0.2500000000000000000, 0.3125000000000000000, 0.3750000000000000000, 0.4375000000000000000, 0.5000000000000000000, 0.5625000000000000000, 0.6250000000000000000, 0.6875000000000000000, 0.7500000000000000000, 0.8125000000000000000, 0.8750000000000000000, 0.9375000000000000000, 1.000000000000000000 ),
 ( 0.000000000000000000, 1.000000000000000000 ),
 .UNSPECIFIED. ) ;
#44950=CARTESIAN_POINT ( 'NONE',  ( 180.1752864420345475, 295.1175617866244920, -2.097363342680641729 ) ) ;
#44951=CARTESIAN_POINT ( 'NONE',  ( 164.6675328809421330, 249.1567145543851325, 9.967022399947358835 ) ) ;
#44952=CARTESIAN_POINT ( 'NONE',  ( 159.8946522441011382, 253.7013337850969492, -16.68230890105693121 ) ) ;
#44953=DIRECTION ( 'NONE',  ( -0.8660254037844387076, -0.4999999999999998890, -0.000000000000000000 ) ) ;
#44955=CARTESIAN_POINT ( 'NONE',  ( 148.7061709727940979, 273.0803518065333151, 9.839166884367505972 ) ) ;
#44956=AXIS2_PLACEMENT_3D ( 'NONE', #45488, #53098, #77915 ) ;
#44957=ORIENTED_EDGE ( 'NONE', *, *, #39206, .F. ) ;
#44960=CARTESIAN_POINT ( 'NONE',  ( 164.5348324038273518, 245.6643059921780718, 1.473102934610569958 ) ) ;
#44962=CARTESIAN_POINT ( 'NONE',  ( 193.4228679857477005, 263.9407716114525897, 4.448677965214572261 ) ) ;
#44963=CARTESIAN_POINT ( 'NONE',  ( 35.89232211637455094, 179.9824982072973683, 3.021315404115420679E-15 ) ) ;
#44964=CARTESIAN_POINT ( 'NONE',  ( 192.6946760137320780, 261.4813915186712165, 3.932628284434791966E-12 ) ) ;
#44965=DIRECTION ( 'NONE',  ( -0.8660254037844387076, -0.4999999999999998890, -0.000000000000000000 ) ) ;
#44966=CARTESIAN_POINT ( 'NONE',  ( 156.9403576227286976, 280.1547494552592070, 5.860362588905387859 ) ) ;
#44967=CARTESIAN_POINT ( 'NONE',  ( 201.4463813434794019, 281.7316278426353620, -17.16864527463587820 ) ) ;
#44969=CARTESIAN_POINT ( 'NONE',  ( 69.66731286396763778, 199.4824982072973967, 3.021315404115420679E-15 ) ) ;
#44970=B_SPLINE_SURFACE_WITH_KNOTS ( 'NONE', 3, 1, ( 
 ( #64254, #87634 ),
 ( #95205, #12062 ),
 ( #19676, #95714 ),
 ( #50537, #72380 ),
 ( #10565, #18162 ),
 ( #58629, #65249 ),
 ( #49062, #26262 ),
 ( #57138, #27757 ),
 ( #65738, #79996 ),
 ( #26756, #81493 ),
 ( #42431, #89603 ),
 ( #42918, #41440 ),
 ( #88119, #20167 ),
 ( #73860, #18668 ),
 ( #49548, #51034 ),
 ( #19183, #80501 ),
 ( #11075, #81991 ),
 ( #41951, #72886 ),
 ( #3478, #34353 ),
 ( #96195, #57639 ),
 ( #11573, #88615 ),
 ( #50054, #81011 ),
 ( #73365, #28241 ),
 ( #45427, #36337 ),
 ( #43931, #21649 ),
 ( #6451, #20657 ),
 ( #84479, #53032 ),
 ( #74870, #60615 ),
 ( #51546, #53528 ),
 ( #99154, #44433 ),
 ( #21166, #52532 ),
 ( #82508, #29743 ),
 ( #14048, #67239 ),
 ( #92098, #91570 ) ),
 .UNSPECIFIED., .T., .F., .F.,
 ( 4, 2, 2, 2, 2, 2, 2, 2, 2, 2, 2, 2, 2, 2, 2, 2, 4 ),
 ( 2, 2 ),
 ( 0.000000000000000000, 0.06250000000000000000, 0.1250000000000000000, 0.1875000000000000000, 0.2500000000000000000, 0.3125000000000000000, 0.3750000000000000000, 0.4375000000000000000, 0.5000000000000000000, 0.5625000000000000000, 0.6250000000000000000, 0.6875000000000000000, 0.7500000000000000000, 0.8125000000000000000, 0.8750000000000000000, 0.9375000000000000000, 1.000000000000000000 ),
 ( 0.000000000000000000, 1.000000000000000000 ),
 .UNSPECIFIED. ) ;
#44972=CARTESIAN_POINT ( 'NONE',  ( 190.4293642567297411, 263.8188777254847537, -9.661471042078789040 ) ) ;
#44973=CARTESIAN_POINT ( 'NONE',  ( 170.4554201786903889, 249.5219033123342172, -0.2601445000210800274 ) ) ;
#44974=CARTESIAN_POINT ( 'NONE',  ( 189.0767298292155942, 269.8417627541793991, -13.98674968934414409 ) ) ;
#44975=CARTESIAN_POINT ( 'NONE',  ( 153.5028723857075761, 272.7411571805866970, -13.59438242947847719 ) ) ;
#44978=CARTESIAN_POINT ( 'NONE',  ( 26.00288702772274263, 192.4865022471903160, 10.00000000000009415 ) ) ;
#44979=CARTESIAN_POINT ( 'NONE',  ( 86.31820828217628616, 211.4548013555409796, -4.594050593750042211 ) ) ;
#44980=CARTESIAN_POINT ( 'NONE',  ( 206.7893622945242385, 272.4773133715531230, -10.52881283832460291 ) ) ;
#44982=CARTESIAN_POINT ( 'NONE',  ( 163.2000388741132895, 247.9762362032568035, -11.19676374274550312 ) ) ;
#44983=EDGE_CURVE ( 'NONE', #34461, #63662, #79210, .T. ) ;
#44985=CARTESIAN_POINT ( 'NONE',  ( 207.5462191418491500, 271.1663988579299485, -5.239401497773396699 ) ) ;
#44990=FACE_OUTER_BOUND ( 'NONE', #91350, .T. ) ;
#44994=CARTESIAN_POINT ( 'NONE',  ( 196.4677418905696129, 290.3548843276421394, 17.08610552292358520 ) ) ;
#44996=ADVANCED_FACE ( 'NONE', ( #46469 ), #75709, .F. ) ;
#44998=CARTESIAN_POINT ( 'NONE',  ( 165.9251183996210557, 249.1081943271603052, -9.381642927290494427 ) ) ;
#45000=CARTESIAN_POINT ( 'NONE',  ( 48.05019010880389629, 207.7369531367911293, -4.594050593750048428 ) ) ;
#45003=CARTESIAN_POINT ( 'NONE',  ( 171.2930143073555485, 286.6872321052386496, 7.314772950087515824 ) ) ;
#45004=CARTESIAN_POINT ( 'NONE',  ( 149.3253462891332219, 272.0079086998416074, -12.99539319630191336 ) ) ;
#45006=CARTESIAN_POINT ( 'NONE',  ( 157.1002372043759010, 258.5414026113353430, -17.73553732786789539 ) ) ;
#45007=CARTESIAN_POINT ( 'NONE',  ( 202.8866346594412846, 269.9979106734580228, -6.436829395617527538 ) ) ;
#45008=CARTESIAN_POINT ( 'NONE',  ( 175.9514560434575401, 291.1772476316439793, 2.554599904375252528 ) ) ;
#45010=CARTESIAN_POINT ( 'NONE',  ( 176.1283921439560061, 274.8553815178914306, 16.96726162417416717 ) ) ;
#45012=CARTESIAN_POINT ( 'NONE',  ( 152.7176750937324812, 276.5233964160840969, 7.187293814298707062 ) ) ;
#45014=ADVANCED_FACE ( 'NONE', ( #72944 ), #42011, .F. ) ;
#45018=CARTESIAN_POINT ( 'NONE',  ( 96.65612621980322672, 226.6115022471902307, 10.00000000000009592 ) ) ;
#45019=CARTESIAN_POINT ( 'NONE',  ( 200.1103929410127762, 284.0456276340304953, 17.67835211026828901 ) ) ;
#45020=CARTESIAN_POINT ( 'NONE',  ( 194.6617293356793539, 285.5289016145630399, -17.32716204712188102 ) ) ;
#45022=CARTESIAN_POINT ( 'NONE',  ( 48.48320281069610616, 207.9869531367911009, 4.594050593750046652 ) ) ;
#45023=BREP_WITH_VOIDS ( 'NONE', #52348, ( #52172 ) );
#45025=CARTESIAN_POINT ( 'NONE',  ( 156.6812872898450735, 261.2670451491295012, 0.000000000000000000 ) ) ;
#45027=CARTESIAN_POINT ( 'NONE',  ( 170.3127733705114224, 263.9010670580030364, 17.23448983536806622 ) ) ;
#45028=ORIENTED_EDGE ( 'NONE', *, *, #93908, .F. ) ;
#45030=CARTESIAN_POINT ( 'NONE',  ( 178.6423073663378602, 290.9544255387157818, 10.03153667033594765 ) ) ;
#45033=CARTESIAN_POINT ( 'NONE',  ( 176.0559032325554085, 274.2081378810889305, -17.70795040911156804 ) ) ;
#45034=CARTESIAN_POINT ( 'NONE',  ( 206.9514768121390489, 271.8153902181765034, -5.779928228329159978 ) ) ;
#45035=CARTESIAN_POINT ( 'NONE',  ( 204.9620549308181694, 275.6423025665365572, 14.49661402992083481 ) ) ;
#45036=ORIENTED_EDGE ( 'NONE', *, *, #99722, .T. ) ;
#45044=CARTESIAN_POINT ( 'NONE',  ( 159.3237119419271437, 254.6902313965507858, -15.56765445935501191 ) ) ;
#45050=CARTESIAN_POINT ( 'NONE',  ( 53.17212233558426959, 213.0530062829863311, -4.648177544792955347E-16 ) ) ;
#45052=CARTESIAN_POINT ( 'NONE',  ( 204.7235752877335244, 276.0553614249301972, 14.82397698933823271 ) ) ;
#45056=CARTESIAN_POINT ( 'NONE',  ( 131.1618259000655371, 246.5333772461660544, 9.188101187500095079 ) ) ;
#45057=CARTESIAN_POINT ( 'NONE',  ( 175.9407212156297078, 268.6798998318777194, 16.14890207857037652 ) ) ;
#45058=CARTESIAN_POINT ( 'NONE',  ( 179.9705885308941902, 259.1087249338424954, 9.582984254543152502 ) ) ;
#45059=CARTESIAN_POINT ( 'NONE',  ( 75.49289073487081225, 205.2048013555409796, 4.594050593750051981 ) ) ;
#45061=CARTESIAN_POINT ( 'NONE',  ( 174.1167577371777782, 265.6544076377189185, 16.40429495823174832 ) ) ;
#45063=CARTESIAN_POINT ( 'NONE',  ( 149.0807665407234026, 276.4376266709116408, -5.539133476438467873 ) ) ;
#45065=ORIENTED_EDGE ( 'NONE', *, *, #47664, .T. ) ;
#45071=CARTESIAN_POINT ( 'NONE',  ( -6.130263895410292818, 177.2677522451419350, -5.000000000000047962 ) ) ;
#45073=CARTESIAN_POINT ( 'NONE',  ( 109.1931406464380530, 245.3967562850346837, -4.648177544792955347E-16 ) ) ;
#45074=CARTESIAN_POINT ( 'NONE',  ( 155.4917600441137324, 261.3273667757233056, 17.14261720787171939 ) ) ;
#45079=CARTESIAN_POINT ( 'NONE',  ( 201.0973175254986245, 282.3362241104620125, -17.32135558411286524 ) ) ;
#45081=VERTEX_POINT ( 'NONE', #50599 ) ;
#45083=CARTESIAN_POINT ( 'NONE',  ( 175.2131407122271298, 254.6897258708467007, -7.357366922857768721 ) ) ;
#45088=CARTESIAN_POINT ( 'NONE',  ( 206.5571822944673670, 272.8794609281530938, 10.95833005210827515 ) ) ;
#45089=CARTESIAN_POINT ( 'NONE',  ( 148.9831146496684084, 272.6006712873522133, -12.63706091291043343 ) ) ;
#45093=CARTESIAN_POINT ( 'NONE',  ( 143.3676317564762144, 244.3923013555409511, 4.594050593750050204 ) ) ;
#45108=CARTESIAN_POINT ( 'NONE',  ( 182.9443896863899113, 280.6423201065871353, 16.69554559524186743 ) ) ;
#45109=B_SPLINE_CURVE_WITH_KNOTS ( 'NONE', 3,
 ( #71411, #55176, #79027, #61783, #63790, #47585, #86160, #9098, #16694, #87170, #85656, #93740, #54672, #46076, #85136, #86654 ),
 .UNSPECIFIED., .F., .F.,
 ( 4, 2, 2, 2, 2, 2, 2, 4 ),
 ( 3.002691588427585642E-15, 0.0005721413298776353764, 0.0008582119948149507941, 0.001144282659752266429, 0.001430353324689581738, 0.001716423989626897264, 0.002002494654564213224, 0.002288565319501528750 ),
 .UNSPECIFIED. ) ;
#45110=VECTOR ( 'NONE', #70942, 1000.000000000000000 ) ;
#45111=CARTESIAN_POINT ( 'NONE',  ( 159.7068082092014265, 262.5164536406643379, -17.81808555889180923 ) ) ;
#45112=CARTESIAN_POINT ( 'NONE',  ( 170.6844402143995012, 263.2133925425807206, -17.01386034520750812 ) ) ;
#45117=CARTESIAN_POINT ( 'NONE',  ( 198.4264492142971221, 286.9623037257889564, 17.00126466006521397 ) ) ;
#45119=CARTESIAN_POINT ( 'NONE',  ( 145.8571944687587632, 255.0177522451418497, -10.00000000000009592 ) ) ;
#45124=CARTESIAN_POINT ( 'NONE',  ( 151.4428545556028780, 268.3402767968688067, -15.03309903163500749 ) ) ;
#45125=CARTESIAN_POINT ( 'NONE',  ( 11.59636713795893925, 171.3768266524160424, 9.188101187500096856 ) ) ;
#45128=CARTESIAN_POINT ( 'NONE',  ( 63.44840177721309971, 218.9860189848785126, -2.679491924311252493 ) ) ;
#45130=CARTESIAN_POINT ( 'NONE',  ( 122.2995471069890812, 252.9637435831425023, 2.679491924311251605 ) ) ;
#45132=CARTESIAN_POINT ( 'NONE',  ( 151.0480362197490933, 269.0241222143274626, 14.53796507407317762 ) ) ;
#45135=CARTESIAN_POINT ( 'NONE',  ( 53.78786873247351252, 201.8615022471902307, -10.00000000000009592 ) ) ;
#45136=FACE_OUTER_BOUND ( 'NONE', #55164, .T. ) ;
#45137=CARTESIAN_POINT ( 'NONE',  ( 190.0515794655415789, 301.4680036374047063, -1.296825456579539626 ) ) ;
#45139=CARTESIAN_POINT ( 'NONE',  ( 17.30628827445631401, 189.9869531367911293, 4.594050593750046652 ) ) ;
#45146=CARTESIAN_POINT ( 'NONE',  ( -22.42236680055709641, 157.8615022471902591, 0.000000000000000000 ) ) ;
#45147=CARTESIAN_POINT ( 'NONE',  ( 189.1267433986236597, 268.0052114195003128, 14.01527934077552473 ) ) ;
#45148=DIRECTION ( 'NONE',  ( -0.8660254037844387076, -0.4999999999999998890, -0.000000000000000000 ) ) ;
#45149=CARTESIAN_POINT ( 'NONE',  ( 160.3357114222172868, 280.0449195850608248, 9.200148331950654068 ) ) ;
#45152=CARTESIAN_POINT ( 'NONE',  ( 190.5674408456512765, 300.5745055173924811, -0.9151048603553563199 ) ) ;
#45154=CARTESIAN_POINT ( 'NONE',  ( 147.4771028564622100, 275.6046161191591182, 9.141179566768406735E-14 ) ) ;
#45157=CARTESIAN_POINT ( 'NONE',  ( 181.7992873095532786, 289.2334549628592981, 12.46585778909335929 ) ) ;
#45163=CARTESIAN_POINT ( 'NONE',  ( 165.3118168859175796, 246.3185293925050701, -4.432402497422931020 ) ) ;
#45164=CARTESIAN_POINT ( 'NONE',  ( 203.2732885619977026, 278.5673317194472247, -16.64305493556850024 ) ) ;
#45165=ORIENTED_EDGE ( 'NONE', *, *, #54153, .T. ) ;
#45168=CARTESIAN_POINT ( 'NONE',  ( 201.6710194064352208, 279.8704541772306129, 16.35544272301150670 ) ) ;
#45169=CARTESIAN_POINT ( 'NONE',  ( 152.8593402092683959, 275.2840601128194749, 10.96293945604634068 ) ) ;
#45170=VERTEX_POINT ( 'NONE', #1859 ) ;
#45171=CARTESIAN_POINT ( 'NONE',  ( 201.0844796915553161, 282.3584598911111812, -16.59562674965125950 ) ) ;
#45175=EDGE_LOOP ( 'NONE', ( #75695, #68838, #7557, #72645 ) ) ;
#45179=CARTESIAN_POINT ( 'NONE',  ( 205.7829192689729325, 274.2205238267313234, 11.21202327925415254 ) ) ;
#45182=CARTESIAN_POINT ( 'NONE',  ( 149.1903793729515257, 272.2416782560088677, 12.95958987445043675 ) ) ;
#45186=CARTESIAN_POINT ( 'NONE',  ( 85.75863988884901801, 226.9865022471903160, 10.00000000000009415 ) ) ;
#45187=CARTESIAN_POINT ( 'NONE',  ( 183.2707082818002107, 282.3109398786273800, 17.13350622414966296 ) ) ;
#45189=ORIENTED_EDGE ( 'NONE', *, *, #3991, .F. ) ;
#45191=CARTESIAN_POINT ( 'NONE',  ( 156.6433882741441721, 266.7315762886727271, -16.19180110469071465 ) ) ;
#45192=CARTESIAN_POINT ( 'NONE',  ( 190.7908437487391780, 300.1875603386860689, -4.317984972589949955 ) ) ;
#45193=CARTESIAN_POINT ( 'NONE',  ( 189.8314329296643450, 301.8493086226544619, -0.8085564604676659384 ) ) ;
#45194=CARTESIAN_POINT ( 'NONE',  ( 190.7705347155322499, 300.2227366160529414, 3.504769718465625239 ) ) ;
#45195=CARTESIAN_POINT ( 'NONE',  ( 192.2185419806677942, 297.7147144631093170, 12.45868041609393728 ) ) ;
#45196=CARTESIAN_POINT ( 'NONE',  ( 191.5201351928026270, 298.9243905040425489, 8.280408090104206309 ) ) ;
#45197=CARTESIAN_POINT ( 'NONE',  ( 147.2180753513904961, 275.6578090293250511, 0.4909717733184589261 ) ) ;
#45198=CARTESIAN_POINT ( 'NONE',  ( 163.7500375660153793, 257.3530331621871028, 15.54842262632091909 ) ) ;
#45199=EDGE_CURVE ( 'NONE', #15352, #12202, #16562, .T. ) ;
#45201=CARTESIAN_POINT ( 'NONE',  ( 149.5796913320911870, 271.5673701627850960, -12.80793412251569841 ) ) ;
#45202=CARTESIAN_POINT ( 'NONE',  ( 97.10949284993499475, 215.3262482093457493, 3.021315404115420679E-15 ) ) ;
#45204=CARTESIAN_POINT ( 'NONE',  ( 168.3419904543532937, 286.3602298079341040, 4.048007086931957765 ) ) ;
#45206=CARTESIAN_POINT ( 'NONE',  ( 96.62871582839601103, 238.8464784336661637, 1.353441290958777327E-15 ) ) ;
#45208=CARTESIAN_POINT ( 'NONE',  ( 149.1483424966081657, 272.3144882616274458, -12.96605911529412403 ) ) ;
#45210=CARTESIAN_POINT ( 'NONE',  ( 148.8371570812549294, 273.9697221964345886, 8.907495186123728814 ) ) ;
#45215=CARTESIAN_POINT ( 'NONE',  ( 165.4103701307380163, 283.8590981551407708, -8.431619659680563927 ) ) ;
#45217=CARTESIAN_POINT ( 'NONE',  ( 167.3001686924326918, 253.0705894573350179, -12.10497857386071985 ) ) ;
#45218=CARTESIAN_POINT ( 'NONE',  ( 206.4484807199597753, 273.0677375780628608, -9.220527398138528952 ) ) ;
#45221=CARTESIAN_POINT ( 'NONE',  ( 48.42933654300943402, 188.7677522451417929, -5.000000000000041744 ) ) ;
#45222=CARTESIAN_POINT ( 'NONE',  ( 105.2078667585768557, 240.7369531367911009, -4.594050593750048428 ) ) ;
#45223=FACE_OUTER_BOUND ( 'NONE', #77254, .T. ) ;
#45227=CARTESIAN_POINT ( 'NONE',  ( 172.2247897617710066, 250.7459979994374066, -4.062067949591432914 ) ) ;
#45228=CARTESIAN_POINT ( 'NONE',  ( 26.15589859543730000, 198.1589784336661637, -6.496448406907675876E-16 ) ) ;
#45229=CARTESIAN_POINT ( 'NONE',  ( 147.7917198021585534, 275.6304213403500398, -3.790807063116589770 ) ) ;
#45230=AXIS2_PLACEMENT_3D ( 'NONE', #65802, #81556, #34902 ) ;
#45231=ORIENTED_EDGE ( 'NONE', *, *, #72191, .F. ) ;
#45233=CARTESIAN_POINT ( 'NONE',  ( 177.9867648153962989, 265.4645870862016181, 15.84164618472818198 ) ) ;
#45239=CARTESIAN_POINT ( 'NONE',  ( 165.9669116182938353, 251.0260590123588145, 10.21599650959468519 ) ) ;
#45240=CARTESIAN_POINT ( 'NONE',  ( 113.8864233123832577, 229.8927522451418213, 10.00000000000009592 ) ) ;
#45243=B_SPLINE_CURVE_WITH_KNOTS ( 'NONE', 3,
 ( #95350, #12700, #57769, #65870, #41573, #43570, #81134, #64386, #11700, #25905, #21286, #28884, #52162, #67879, #44554, #45555 ),
 .UNSPECIFIED., .F., .F.,
 ( 4, 2, 2, 2, 2, 2, 2, 4 ),
 ( 1.040834085586084257E-17, 0.0003787177898466214700, 0.0007574355796932325316, 0.001136153369539843593, 0.001514871159386454655, 0.001893588949233065716, 0.002272306739079676778, 0.003029742318772891529 ),
 .UNSPECIFIED. ) ;
#45244=CARTESIAN_POINT ( 'NONE',  ( 154.9032082715209810, 280.6326124547101699, -2.389722542998433230 ) ) ;
#45245=CARTESIAN_POINT ( 'NONE',  ( 154.0193023235302689, 265.1638567325853728, 16.81819982589781048 ) ) ;
#45247=CARTESIAN_POINT ( 'NONE',  ( 21.25804982287034406, 173.8923013555409796, 4.594050593750050204 ) ) ;
#45249=CARTESIAN_POINT ( 'NONE',  ( 196.0356377417433862, 273.4210236615080589, 15.17726198895217493 ) ) ;
#45253=CARTESIAN_POINT ( 'NONE',  ( 194.7629524071031426, 274.9938599527168890, -15.98506956286481895 ) ) ;
#45254=CARTESIAN_POINT ( 'NONE',  ( 64.39641960523518094, 217.1744531367911293, 4.594050593750047540 ) ) ;
#45255=CARTESIAN_POINT ( 'NONE',  ( 207.6172352878830907, 271.0433952848413810, 3.316653249540578496 ) ) ;
#45260=CARTESIAN_POINT ( 'NONE',  ( 17.34263298987844237, 167.4865022471901739, 1.119607411625061291E-15 ) ) ;
#45261=B_SPLINE_CURVE_WITH_KNOTS ( 'NONE', 3,
 ( #39002, #94256, #522, #39488 ),
 .UNSPECIFIED., .F., .F.,
 ( 4, 4 ),
 ( 0.009195655101482617944, 0.01511765829135664103 ),
 .UNSPECIFIED. ) ;
#45262=CARTESIAN_POINT ( 'NONE',  ( 207.8302079587528794, 270.6745157982714431, 3.572475529330238153 ) ) ;
#45263=CARTESIAN_POINT ( 'NONE',  ( 140.7695555451228984, 242.8923013555409796, 4.594050593750050204 ) ) ;
#45268=CARTESIAN_POINT ( 'NONE',  ( 206.1585898378126274, 271.5698433145930721, 8.212139725584252758 ) ) ;
#45270=CARTESIAN_POINT ( 'NONE',  ( 189.2726224819945458, 299.8637631263580943, 4.914554397034637923 ) ) ;
#45275=CARTESIAN_POINT ( 'NONE',  ( 156.6772434156269753, 280.3381848834534935, -5.402216236100986890 ) ) ;
#45279=CARTESIAN_POINT ( 'NONE',  ( 170.1203493898869397, 283.3057450205278087, -11.00909384804022473 ) ) ;
#45281=CARTESIAN_POINT ( 'NONE',  ( 148.7749086576190791, 273.3915829829758195, -9.018907845894478470 ) ) ;
#45282=CARTESIAN_POINT ( 'NONE',  ( 196.1574275305892741, 271.0118636216350865, 12.32861447576741298 ) ) ;
#45283=CARTESIAN_POINT ( 'NONE',  ( 107.5017976953482446, 221.3262482093458061, 3.021315404115420679E-15 ) ) ;
#45285=CARTESIAN_POINT ( 'NONE',  ( 200.9521687275011175, 282.5876292032514243, -18.16013154125647944 ) ) ;
#45286=VERTEX_POINT ( 'NONE', #82407 ) ;
#45287=CARTESIAN_POINT ( 'NONE',  ( 190.5050603160280787, 281.5143243275973077, 17.11203965365400492 ) ) ;
#45289=CARTESIAN_POINT ( 'NONE',  ( 164.6077667029246925, 248.8717717204749817, 10.07792378446523607 ) ) ;
#45291=CARTESIAN_POINT ( 'NONE',  ( 149.7166446726674565, 271.3301600186404698, 12.26048591517335495 ) ) ;
#45293=CARTESIAN_POINT ( 'NONE',  ( 189.0786975680280477, 297.0699590293599499, 8.119915869620735194 ) ) ;
#45294=ORIENTED_EDGE ( 'NONE', *, *, #10391, .F. ) ;
#45296=CARTESIAN_POINT ( 'NONE',  ( 146.7373254022577100, 276.4904923669593586, -0.7242168585908188572 ) ) ;
#45297=CARTESIAN_POINT ( 'NONE',  ( 165.9013214703126948, 280.3534790633716511, 13.25418706671784541 ) ) ;
#45298=B_SPLINE_CURVE_WITH_KNOTS ( 'NONE', 3,
 ( #93881, #53168, #37451, #51683, #36462, #36962, #84606, #82632, #83107, #52656, #91204, #60245, #45061, #29868, #91701, #60739, #76958, #5570, #92221, #38450, #53650, #21765, #67363, #13193, #29377, #52159, #28366, #59242, #75485, #98291, #90222, #44551, #22773, #6068, #98796, #44049, #45551, #83608, #14176, #28880, #20791, #74990, #76002, #13678, #90726, #67875, #6579, #22264 ),
 .UNSPECIFIED., .F., .F.,
 ( 4, 2, 2, 2, 2, 2, 2, 2, 2, 2, 2, 2, 2, 2, 2, 2, 2, 2, 2, 2, 2, 2, 2, 4 ),
 ( 0.001171907001705587087, 0.001643730509668527798, 0.002115554017631468726, 0.002351465771612907749, 0.002587377525594346771, 0.002705333402585056307, 0.002823289279575765410, 0.003059201033557106420, 0.003531024541519774129, 0.004002848049482442272, 0.004946495065407923407, 0.005890142081333404542, 0.006361965589296181105, 0.006833789097258956800, 0.006951744974249671541, 0.007010722912745051896, 0.007069700851240433119, 0.007187656728231248474, 0.007305612605222063828, 0.007541524359203702343, 0.007777436113185339991, 0.008013347867166977639, 0.008249259621148617022, 0.008721083129111881910 ),
 .UNSPECIFIED. ) ;
#45299=CARTESIAN_POINT ( 'NONE',  ( 164.2297246530060875, 246.1927681183832988, 5.803160395959773510 ) ) ;
#45302=CARTESIAN_POINT ( 'NONE',  ( 101.4461556848294492, 235.5024278399160949, -9.188101187500093303 ) ) ;
#45304=CARTESIAN_POINT ( 'NONE',  ( 190.0601721553029222, 300.2863949309033842, 3.228815124723532382 ) ) ;
#45310=ORIENTED_EDGE ( 'NONE', *, *, #12922, .T. ) ;
#45314=CARTESIAN_POINT ( 'NONE',  ( 207.5230514910949182, 271.2065264061283756, 2.678931747975364708 ) ) ;
#45315=CARTESIAN_POINT ( 'NONE',  ( -22.42236680055709641, 157.8615022471902591, 0.000000000000000000 ) ) ;
#45316=CARTESIAN_POINT ( 'NONE',  ( 168.4414336168281636, 281.4392610354049680, 11.65181175857584428 ) ) ;
#45320=CARTESIAN_POINT ( 'NONE',  ( 194.3589246629463787, 272.8122030992582836, -15.48160684239839568 ) ) ;
#45323=CARTESIAN_POINT ( 'NONE',  ( 198.4820782953651133, 277.0876319724349628, -15.27341537592363707 ) ) ;
#45325=CARTESIAN_POINT ( 'NONE',  ( 182.4004271739244700, 284.1903799708203451, 16.39187655311515002 ) ) ;
#45327=CARTESIAN_POINT ( 'NONE',  ( 163.4216610345155800, 247.5923753613567442, 10.58669027323842826 ) ) ;
#45328=EDGE_CURVE ( 'NONE', #94086, #22165, #52792, .T. ) ;
#45329=CARTESIAN_POINT ( 'NONE',  ( 185.0221735844220063, 258.3581008124040181, 2.953144405170906595 ) ) ;
#45332=CARTESIAN_POINT ( 'NONE',  ( 171.4141472835499940, 255.5714509828059136, 11.16434605878179021 ) ) ;
#45333=CARTESIAN_POINT ( 'NONE',  ( 193.1345686763260971, 263.1208943439388577, -0.7594564661863862920 ) ) ;
#45335=B_SPLINE_CURVE_WITH_KNOTS ( 'NONE', 3,
 ( #21725, #53121, #93152, #69322, #60698, #85056, #22222, #54100, #68810, #38408, #84567, #99739, #92659, #47022, #22729, #45012, #91657, #100243, #91159, #52609, #69814, #31804, #99238, #15604, #84077, #46503, #6534, #14630, #424, #45996, #8037, #38910, #8528, #45510, #77440, #37409, #76914, #83567 ),
 .UNSPECIFIED., .F., .F.,
 ( 4, 2, 2, 2, 2, 2, 2, 2, 2, 2, 2, 2, 2, 2, 2, 2, 2, 2, 4 ),
 ( 0.0009380411731141725462, 0.001032228557793670462, 0.001126415942473168270, 0.001314790711832097315, 0.001691540250549881247, 0.002445039327985399670, 0.003952037482856488558, 0.004705536560292067697, 0.005082286099009856832, 0.005270660868368789130, 0.005364848253048254412, 0.005459035637727720561, 0.005506129330067452768, 0.005553223022407186710, 0.005647410407086621634, 0.005835785176445533115, 0.006212534715163351741, 0.006589284253881176438, 0.006966033792599000268 ),
 .UNSPECIFIED. ) ;
#45338=DIRECTION ( 'NONE',  ( -0.8660254037844387076, -0.4999999999999998890, -0.000000000000000000 ) ) ;
#45340=CARTESIAN_POINT ( 'NONE',  ( 9.025180670817464446, 166.0177522451418213, 5.000000000000051514 ) ) ;
#45341=CARTESIAN_POINT ( 'NONE',  ( 192.9924223820390239, 267.3565088504736877, -11.03506825955556536 ) ) ;
#45342=CARTESIAN_POINT ( 'NONE',  ( 171.2938825197189487, 279.7153930126568184, -14.88499062438163101 ) ) ;
#45343=CARTESIAN_POINT ( 'NONE',  ( 204.1768090745211452, 277.0023882860760409, -15.56867155119955015 ) ) ;
#45346=CARTESIAN_POINT ( 'NONE',  ( -4.614459115189767147, 158.9548013555409796, -4.594050593750042211 ) ) ;
#45348=CARTESIAN_POINT ( 'NONE',  ( 185.2439061181696331, 295.2756445577334716, 8.340933124425840006 ) ) ;
#45349=ORIENTED_EDGE ( 'NONE', *, *, #85701, .T. ) ;
#45352=CARTESIAN_POINT ( 'NONE',  ( 128.1703819823903245, 233.2592609112379876, 2.679491924311254714 ) ) ;
#45353=EDGE_CURVE ( 'NONE', #76711, #70599, #86319, .T. ) ;
#45356=CARTESIAN_POINT ( 'NONE',  ( 202.0712002603176813, 280.6494097331414537, -16.02287548436454045 ) ) ;
#45358=CARTESIAN_POINT ( 'NONE',  ( 150.1592538715819671, 276.5420469420121208, 3.659585770713507547 ) ) ;
#45359=CARTESIAN_POINT ( 'NONE',  ( 13.11156449881669595, 184.5024278399160949, -9.188101187500093303 ) ) ;
#45360=CARTESIAN_POINT ( 'NONE',  ( 124.3418758452630613, 242.5958772461660544, -9.188101187500095079 ) ) ;
#45361=CARTESIAN_POINT ( 'NONE',  ( 182.0298379502229693, 294.6333645221262714, -6.494620609296796410 ) ) ;
#45366=CARTESIAN_POINT ( 'NONE',  ( 194.1011995340913074, 294.4538559273262877, 13.93949783759920713 ) ) ;
#45367=CARTESIAN_POINT ( 'NONE',  ( 184.1072741032023146, 274.9104562530689009, 16.37390854714151800 ) ) ;
#45369=EDGE_CURVE ( 'NONE', #91593, #51615, #31224, .T. ) ;
#45371=CARTESIAN_POINT ( 'NONE',  ( 170.2786588980588363, 279.2388764142214086, 13.93236286921391631 ) ) ;
#45372=CARTESIAN_POINT ( 'NONE',  ( 187.2183957178467608, 298.8926474041342658, -0.5935065169117408335 ) ) ;
#45373=CARTESIAN_POINT ( 'NONE',  ( 191.4852287632733123, 298.9848502134979071, -9.870565261052552941 ) ) ;
#45374=CARTESIAN_POINT ( 'NONE',  ( 184.4900473518464139, 268.6311471613904587, -15.53052497869454207 ) ) ;
#45379=CARTESIAN_POINT ( 'NONE',  ( 185.0590661537433164, 269.5214566935702010, 15.89575827224772731 ) ) ;
#45380=CARTESIAN_POINT ( 'NONE',  ( 92.19068272976576850, 224.0333772461660544, 9.188101187500095079 ) ) ;
#45382=CARTESIAN_POINT ( 'NONE',  ( 160.4237162281696953, 273.2376347127639633, -15.66572034412998882 ) ) ;
#45383=EDGE_CURVE ( 'NONE', #62639, #15755, #74549, .T. ) ;
#45384=CARTESIAN_POINT ( 'NONE',  ( 176.0127109592394277, 252.6004560315867593, -4.768680066900455650 ) ) ;
#45386=CARTESIAN_POINT ( 'NONE',  ( 152.1253780900047161, 267.1581113579235307, 17.01065375775331745 ) ) ;
#45387=CARTESIAN_POINT ( 'NONE',  ( 152.6547697591180111, 278.7515079535921814, -4.825746761778547445 ) ) ;
#45389=CARTESIAN_POINT ( 'NONE',  ( 149.2923684163597784, 272.0650280510108701, -12.99082738998495756 ) ) ;
#45391=CARTESIAN_POINT ( 'NONE',  ( 125.0004159942834860, 249.6427522451419065, -10.00000000000009592 ) ) ;
#45395=CARTESIAN_POINT ( 'NONE',  ( 177.8324374767559846, 280.3398814767268732, 16.75142732283180180 ) ) ;
#45396=CARTESIAN_POINT ( 'NONE',  ( 146.8312060062178830, 276.3278863910550172, -4.807241325481028227 ) ) ;
#45397=CARTESIAN_POINT ( 'NONE',  ( 197.0226655822963551, 289.3937282992477549, -17.28982543158101493 ) ) ;
#45403=CARTESIAN_POINT ( 'NONE',  ( 181.1554500484497794, 263.5640902285028915, -12.87665043090944650 ) ) ;
#45404=CARTESIAN_POINT ( 'NONE',  ( 173.2694288764014345, 253.7023385635754380, -9.145525555831373055 ) ) ;
#45405=CARTESIAN_POINT ( 'NONE',  ( 192.0645969571214096, 297.9813550654635605, 11.46542907566974812 ) ) ;
#45407=CARTESIAN_POINT ( 'NONE',  ( 187.2093787057832515, 278.7783034237749007, 17.22333937481381483 ) ) ;
#45408=ORIENTED_EDGE ( 'NONE', *, *, #20368, .T. ) ;
#45409=CARTESIAN_POINT ( 'NONE',  ( 172.0728039219370658, 285.9831811572526021, 11.38650458882361427 ) ) ;
#45410=CARTESIAN_POINT ( 'NONE',  ( 184.6894110187365641, 293.7322318964822330, -10.88359728165448814 ) ) ;
#45413=CARTESIAN_POINT ( 'NONE',  ( -13.76211276271269668, 162.8615022471902591, 0.000000000000000000 ) ) ;
#45414=CARTESIAN_POINT ( 'NONE',  ( 190.4975935673924141, 278.7163863375838559, -16.50822108151892920 ) ) ;
#45415=CARTESIAN_POINT ( 'NONE',  ( 192.4990000879081720, 297.2289467719743357, -12.72483680792790750 ) ) ;
#45416=CARTESIAN_POINT ( 'NONE',  ( 153.0927037754837556, 265.4826541232073964, -16.15085267704102634 ) ) ;
#45418=CARTESIAN_POINT ( 'NONE',  ( 190.0398248856338057, 298.8169614316505545, -8.166243001185458539 ) ) ;
#45420=VERTEX_POINT ( 'NONE', #100050 ) ;
#45421=CARTESIAN_POINT ( 'NONE',  ( 195.1948488736749709, 291.0624176751974233, 16.30441594086294543 ) ) ;
#45422=EDGE_LOOP ( 'NONE', ( #72188, #14808, #65359, #17021 ) ) ;
#45423=VERTEX_POINT ( 'NONE', #69623 ) ;
#45425=CARTESIAN_POINT ( 'NONE',  ( 170.5373622343556690, 269.7751423367952270, 17.81562764448176850 ) ) ;
#45426=( BOUNDED_CURVE ( )  B_SPLINE_CURVE ( 2, ( #81633, #15040, #66882, #75007, #38340, #90742, #97320, #74009, #66391 ),
 .UNSPECIFIED., .F., .T. ) 
 B_SPLINE_CURVE_WITH_KNOTS ( ( 3, 2, 2, 2, 3 ),
 ( 0.8024193548387096309, 0.8037634408602150060, 0.8064516129032257563, 0.8091397849462365066, 0.8104838709677418818 ),
 .UNSPECIFIED. ) 
 CURVE ( )  GEOMETRIC_REPRESENTATION_ITEM ( )  RATIONAL_B_SPLINE_CURVE ( ( 0.9330127018922194093, 0.9330127018922194093, 1.000000000000000000, 0.8660254037844387076, 1.000000000000000000, 0.8660254037844387076, 1.000000000000000000, 0.9330127018922194093, 0.9330127018922194093 ) ) 
 REPRESENTATION_ITEM ( '' )  );
#45427=CARTESIAN_POINT ( 'NONE',  ( 204.7610021263893429, 275.9905362388115577, 13.36619428527026976 ) ) ;
#45428=CARTESIAN_POINT ( 'NONE',  ( 164.8817931653405253, 246.2093970608671327, 2.959562278375574618 ) ) ;
#45429=CARTESIAN_POINT ( 'NONE',  ( 206.6961830126489303, 272.6387046219738295, -10.22526498917591375 ) ) ;
#45430=CARTESIAN_POINT ( 'NONE',  ( 197.4562109845989255, 273.0769534991460432, -13.28701267068813152 ) ) ;
#45431=CARTESIAN_POINT ( 'NONE',  ( 203.5137996566828633, 276.3711131836337813, 14.38221294039407994 ) ) ;
#45433=CARTESIAN_POINT ( 'NONE',  ( 170.9667952754920748, 287.9054735324309604, -4.302708445872753806 ) ) ;
#45435=CARTESIAN_POINT ( 'NONE',  ( 183.4135640167273209, 284.6506825199782043, -15.02283699949769158 ) ) ;
#45436=CARTESIAN_POINT ( 'NONE',  ( 108.2389556718223673, 242.4869531367911009, 4.594050593750046652 ) ) ;
#45442=ADVANCED_FACE ( 'NONE', ( #5841 ), #99547, .T. ) ;
#45446=CARTESIAN_POINT ( 'NONE',  ( 180.6820162318767871, 294.0274809239796809, -2.627441245078403931 ) ) ;
#45447=CARTESIAN_POINT ( 'NONE',  ( 157.4177733328310467, 257.9914139036126812, 18.29188238796808363 ) ) ;
#45448=CARTESIAN_POINT ( 'NONE',  ( 159.8597520197352537, 253.7617827468940277, -16.74905990210778839 ) ) ;
#45450=VERTEX_POINT ( 'NONE', #67634 ) ;
#45451=CARTESIAN_POINT ( 'NONE',  ( 194.8100188241370176, 293.2261449035823375, 15.40535685002683586 ) ) ;
#45453=EDGE_LOOP ( 'NONE', ( #67664, #79244, #41177, #92320 ) ) ;
#45454=CARTESIAN_POINT ( 'NONE',  ( 198.0699909391895233, 265.2131322728000669, -4.382015913889547143 ) ) ;
#45456=CARTESIAN_POINT ( 'NONE',  ( 188.6181737819976263, 265.0236329270882152, -12.14609691747098630 ) ) ;
#45457=EDGE_CURVE ( 'NONE', #6076, #15004, #18924, .T. ) ;
#45458=CARTESIAN_POINT ( 'NONE',  ( 191.8060291873681535, 298.4292075798759925, -10.98119608837455630 ) ) ;
#45459=CARTESIAN_POINT ( 'NONE',  ( 158.3585752585947262, 263.3710999200782226, 17.79390465796247156 ) ) ;
#45460=FACE_OUTER_BOUND ( 'NONE', #74955, .T. ) ;
#45461=CARTESIAN_POINT ( 'NONE',  ( 184.3420480696962045, 288.6290895812416011, -13.42755799798725569 ) ) ;
#45462=CARTESIAN_POINT ( 'NONE',  ( 159.5496032553882628, 280.9406269996898686, 5.636233419987954463 ) ) ;
#45463=CARTESIAN_POINT ( 'NONE',  ( 153.2283961777204695, 265.2476279883323400, -17.66880461074566000 ) ) ;
#45465=CARTESIAN_POINT ( 'NONE',  ( 156.6812872898450735, 261.2670451491295012, 0.000000000000000000 ) ) ;
#45468=CARTESIAN_POINT ( 'NONE',  ( 171.0478277236890676, 250.0784670999508421, -0.2578715090061357018 ) ) ;
#45469=CARTESIAN_POINT ( 'NONE',  ( 192.5993683522255537, 271.7468063364418072, -14.60450809009411621 ) ) ;
#45474=CARTESIAN_POINT ( 'NONE',  ( 190.8679683466651227, 268.2575022531604532, 14.00021181731352016 ) ) ;
#45475=CARTESIAN_POINT ( 'NONE',  ( 191.2323848354392055, 283.4409172823887388, -16.58526465056708687 ) ) ;
#45477=CARTESIAN_POINT ( 'NONE',  ( 72.38035161819672680, 212.5958772461660544, -9.188101187500095079 ) ) ;
#45479=CARTESIAN_POINT ( 'NONE',  ( 192.9523350703175311, 296.4437475495926719, -13.35611922184540923 ) ) ;
#45481=CARTESIAN_POINT ( 'NONE',  ( 196.9477862557387766, 288.8927537360994506, -16.71206681448230924 ) ) ;
#45482=CARTESIAN_POINT ( 'NONE',  ( 161.0965315767822972, 251.6196177163260188, -13.76772246540905442 ) ) ;
#45483=CARTESIAN_POINT ( 'NONE',  ( 162.5093986457823974, 284.9610020461826139, 2.827745808343583356 ) ) ;
#45488=CARTESIAN_POINT ( 'NONE',  ( -22.42236680055709641, 157.8615022471902591, 0.000000000000000000 ) ) ;
#45491=EDGE_CURVE ( 'NONE', #4092, #79192, #90362, .T. ) ;
#45492=CARTESIAN_POINT ( 'NONE',  ( 34.68144358152915174, 181.6423013555409796, -4.594050593750043987 ) ) ;
#45493=CARTESIAN_POINT ( 'NONE',  ( 43.61180991440864574, 205.1744531367911293, 4.594050593750047540 ) ) ;
#45494=CARTESIAN_POINT ( 'NONE',  ( 157.6286460899086137, 257.6261715744221306, 18.25526781158026779 ) ) ;
#45496=ADVANCED_FACE ( 'NONE', ( #39694 ), #4470, .F. ) ;
#45498=CARTESIAN_POINT ( 'NONE',  ( -5.101858724868275630, 157.8615022471902023, 5.000000000000051514 ) ) ;
#45499=CARTESIAN_POINT ( 'NONE',  ( 47.69862761034023180, 198.3458772461660544, 9.188101187500095079 ) ) ;
#45501=CARTESIAN_POINT ( 'NONE',  ( 151.3124059063077311, 268.5662204852269497, -14.45542936000225609 ) ) ;
#45502=CARTESIAN_POINT ( 'NONE',  ( 196.6800254274587019, 289.9871984561398222, -17.90749311895638129 ) ) ;
#45505=CARTESIAN_POINT ( 'NONE',  ( 158.8666211102878947, 255.9103432951560535, -16.04241150037398711 ) ) ;
#45508=CARTESIAN_POINT ( 'NONE',  ( 176.2472916049610205, 274.9672641557643828, 17.27598799561485876 ) ) ;
#45509=CYLINDRICAL_SURFACE ( 'NONE', #57077, 17.82106496071139645 ) ;
#45510=CARTESIAN_POINT ( 'NONE',  ( 153.2981356959497816, 276.9127835245838014, 7.993427546634691794 ) ) ;
#45512=CARTESIAN_POINT ( 'NONE',  ( 153.7869224421094714, 276.6684750246370754, 9.963584371085772773 ) ) ;
#45513=CARTESIAN_POINT ( 'NONE',  ( 105.7493929595398470, 231.8615022471902591, -10.00000000000009592 ) ) ;
#45514=CARTESIAN_POINT ( 'NONE',  ( 161.7101619467568980, 250.5567787384628389, 13.05644392949610655 ) ) ;
#45515=CARTESIAN_POINT ( 'NONE',  ( 164.8188621457609031, 269.4130389654807800, -16.30850380620819351 ) ) ;
#45516=ORIENTED_EDGE ( 'NONE', *, *, #17750, .T. ) ;
#45518=ORIENTED_EDGE ( 'NONE', *, *, #51118, .T. ) ;
#45519=CARTESIAN_POINT ( 'NONE',  ( 165.6809110264175615, 265.1086644751799213, 16.57607991724843899 ) ) ;
#45520=CARTESIAN_POINT ( 'NONE',  ( 187.8107902964165135, 277.2180192601347812, -16.66606730953470716 ) ) ;
#45525=CARTESIAN_POINT ( 'NONE',  ( 194.5298665426430489, 293.7113828889860656, -16.13302716640051315 ) ) ;
#45526=CARTESIAN_POINT ( 'NONE',  ( 177.2790252787945349, 274.8473450460222125, -17.02799535311900669 ) ) ;
#45527=ORIENTED_EDGE ( 'NONE', *, *, #52370, .T. ) ;
#45533=CARTESIAN_POINT ( 'NONE',  ( 171.7154418923348942, 259.3365693118849435, -15.26938553599716641 ) ) ;
#45534=CARTESIAN_POINT ( 'NONE',  ( 159.2651917302844993, 254.7915913763855258, -16.53922207549818424 ) ) ;
#45536=EDGE_LOOP ( 'NONE', ( #68075, #45516, #5325, #69336 ) ) ;
#45537=CARTESIAN_POINT ( 'NONE',  ( 174.7605424730916468, 286.1926619560792346, 10.62116624121103037 ) ) ;
#45538=CARTESIAN_POINT ( 'NONE',  ( 159.5064483110165554, 282.2686952242540315, -3.232496309074801122 ) ) ;
#45540=CARTESIAN_POINT ( 'NONE',  ( 162.9111474110223412, 248.4766108952035211, -9.702990628959184960 ) ) ;
#45541=CARTESIAN_POINT ( 'NONE',  ( 163.7136804588959649, 247.0865828815331042, 6.783386239354816105 ) ) ;
#45542=CARTESIAN_POINT ( 'NONE',  ( 198.4772197948566372, 286.8743665007300478, 18.43646439804394532 ) ) ;
#45543=CARTESIAN_POINT ( 'NONE',  ( 164.6134528626768088, 265.2130342782942307, -16.63617519986410187 ) ) ;
#45544=B_SPLINE_CURVE_WITH_KNOTS ( 'NONE', 3,
 ( #70793, #95649, #57075, #889 ),
 .UNSPECIFIED., .F., .F.,
 ( 4, 4 ),
 ( 0.01095786972172493184, 0.01671678501755174268 ),
 .UNSPECIFIED. ) ;
#45545=ADVANCED_FACE ( 'NONE', ( #3747 ), #81764, .T. ) ;
#45546=CARTESIAN_POINT ( 'NONE',  ( 129.3218690127885964, 233.2202760586659736, -5.415160957724236172E-17 ) ) ;
#45547=CARTESIAN_POINT ( 'NONE',  ( 177.3894926443979614, 269.1231757516105176, 16.10179540431882472 ) ) ;
#45548=CARTESIAN_POINT ( 'NONE',  ( 179.7076816803278234, 257.8881168337280201, 10.24022085344165411 ) ) ;
#45549=CARTESIAN_POINT ( 'NONE',  ( 65.61435460324827318, 214.8149278399160664, 9.188101187500093303 ) ) ;
#45551=CARTESIAN_POINT ( 'NONE',  ( 170.2874585057777210, 263.9538622975835551, 15.97034119630043314 ) ) ;
#45555=CARTESIAN_POINT ( 'NONE',  ( 200.3804403721752578, 281.5778917628034606, 17.30444700233937994 ) ) ;
#45556=B_SPLINE_CURVE_WITH_KNOTS ( 'NONE', 3,
 ( #70119, #53429, #29647, #45814 ),
 .UNSPECIFIED., .F., .F.,
 ( 4, 4 ),
 ( 0.008276874795924938841, 0.01457606355628901854 ),
 .UNSPECIFIED. ) ;
#45557=VERTEX_POINT ( 'NONE', #57922 ) ;
#45563=B_SPLINE_SURFACE_WITH_KNOTS ( 'NONE', 3, 1, ( 
 ( #40450, #62242 ),
 ( #79513, #31847 ),
 ( #9586, #32860 ),
 ( #94205, #71385 ),
 ( #62750, #92702 ),
 ( #85622, #93706 ),
 ( #47064, #77978 ),
 ( #47556, #69364 ),
 ( #48574, #9071 ),
 ( #10075, #1973 ),
 ( #56144, #15649 ),
 ( #78483, #39937 ),
 ( #25261, #24269 ),
 ( #16662, #46548 ),
 ( #8574, #55639 ),
 ( #87143, #39439 ),
 ( #70358, #85102 ),
 ( #77483, #970 ),
 ( #8079, #17674 ),
 ( #55146, #86132 ),
 ( #100283, #1482 ),
 ( #23749, #48057 ),
 ( #63767, #30869 ),
 ( #32365, #93196 ),
 ( #63264, #61752 ),
 ( #38952, #24760 ),
 ( #94699, #54645 ),
 ( #54140, #86625 ),
 ( #470, #31359 ),
 ( #69857, #17159 ),
 ( #16166, #79000 ),
 ( #12073, #33892 ),
 ( #51045, #3489 ),
 ( #81505, #4459 ) ),
 .UNSPECIFIED., .T., .F., .F.,
 ( 4, 2, 2, 2, 2, 2, 2, 2, 2, 2, 2, 2, 2, 2, 2, 2, 4 ),
 ( 2, 2 ),
 ( 0.000000000000000000, 0.06250000000000000000, 0.1250000000000000000, 0.1875000000000000000, 0.2500000000000000000, 0.3125000000000000000, 0.3750000000000000000, 0.4375000000000000000, 0.5000000000000000000, 0.5625000000000000000, 0.6250000000000000000, 0.6875000000000000000, 0.7500000000000000000, 0.8125000000000000000, 0.8750000000000000000, 0.9375000000000000000, 1.000000000000000000 ),
 ( 0.000000000000000000, 1.000000000000000000 ),
 .UNSPECIFIED. ) ;
#45565=CARTESIAN_POINT ( 'NONE',  ( 155.5888570658010508, 261.1591898008976500, 17.34682632352454945 ) ) ;
#45569=CARTESIAN_POINT ( 'NONE',  ( 162.0157470128914952, 250.0274898778833688, -13.78877802034368649 ) ) ;
#45574=CARTESIAN_POINT ( 'NONE',  ( 196.2421909983451940, 290.7455499326673021, -17.31908925000307065 ) ) ;
#45575=CARTESIAN_POINT ( 'NONE',  ( 195.1551897557243933, 279.2352859451050904, 16.33844644333552054 ) ) ;
#45576=CARTESIAN_POINT ( 'NONE',  ( 162.2853105227554238, 261.2444871014557748, 16.87942141898201953 ) ) ;
#45577=CARTESIAN_POINT ( 'NONE',  ( 142.8531688511554307, 253.2833772461660544, -9.188101187500095079 ) ) ;
#45578=VERTEX_POINT ( 'NONE', #20437 ) ;
#45580=CARTESIAN_POINT ( 'NONE',  ( 183.1915443601783977, 257.6986921343423091, 6.833778512193781296 ) ) ;
#45582=CARTESIAN_POINT ( 'NONE',  ( 153.3506059258413643, 265.0359544954067132, -16.39100908615009899 ) ) ;
#45588=CARTESIAN_POINT ( 'NONE',  ( 199.7626786811085822, 266.7967628138173950, 4.643313006584093294 ) ) ;
#45589=CARTESIAN_POINT ( 'NONE',  ( 200.1133476818314705, 272.1141633677412415, 12.87458617912082914 ) ) ;
#45591=CARTESIAN_POINT ( 'NONE',  ( 184.8342610281462726, 263.5722196047579473, -12.52600749362046528 ) ) ;
#45592=CARTESIAN_POINT ( 'NONE',  ( 198.7518522379862418, 265.8040289700034577, 1.598954627491116165 ) ) ;
#45593=ORIENTED_EDGE ( 'NONE', *, *, #3991, .T. ) ;
#45594=CARTESIAN_POINT ( 'NONE',  ( 190.6218339396177441, 300.4802939150614520, -4.178005820806754755 ) ) ;
#45597=CARTESIAN_POINT ( 'NONE',  ( 155.6126298223767890, 261.1180141786725244, 18.15400560664037855 ) ) ;
#45598=CARTESIAN_POINT ( 'NONE',  ( 192.8037126019380594, 268.3597080544300297, 12.45183830779196299 ) ) ;
#45601=CARTESIAN_POINT ( 'NONE',  ( 163.1996623812120504, 283.9505196342968816, -3.834948744398505305 ) ) ;
#45605=CARTESIAN_POINT ( 'NONE',  ( -13.03140383004354241, 163.2833772461660544, -9.188101187500095079 ) ) ;
#45610=CARTESIAN_POINT ( 'NONE',  ( 202.6716764631725027, 274.3364404589790411, -12.86965901471974227 ) ) ;
#45612=CARTESIAN_POINT ( 'NONE',  ( 14.19444334931225349, 172.8768266524160140, 9.188101187500096856 ) ) ;
#45614=CARTESIAN_POINT ( 'NONE',  ( 178.7130411427290539, 273.8027002318069094, -16.86336393568773673 ) ) ;
#45617=CARTESIAN_POINT ( 'NONE',  ( 170.5589339941222136, 270.9438782765666929, -16.77442372788140901 ) ) ;
#45618=CARTESIAN_POINT ( 'NONE',  ( 133.3665344050969566, 236.2592609112379876, 2.679491924311254714 ) ) ;
#45620=CARTESIAN_POINT ( 'NONE',  ( 175.5454376425959424, 253.5828794482383159, -3.844180409976710511 ) ) ;
#45621=CARTESIAN_POINT ( 'NONE',  ( 191.3040952703574078, 261.0541660929657723, -1.520933822623211640 ) ) ;
#45622=CARTESIAN_POINT ( 'NONE',  ( 55.08690683815022027, 192.6115022471902023, -5.000000000000041744 ) ) ;
#45624=CARTESIAN_POINT ( 'NONE',  ( 190.4744901378711290, 300.7355008658671522, 0.04566709859947504224 ) ) ;
#45625=CARTESIAN_POINT ( 'NONE',  ( 16.17015057563676450, 170.9548013555409796, -4.594050593750042211 ) ) ;
#45626=CARTESIAN_POINT ( 'NONE',  ( 165.0391502558331069, 249.6778246878102436, -10.74756611015070717 ) ) ;
#45630=CARTESIAN_POINT ( 'NONE',  ( 206.9026071836525205, 272.2811674698855313, 7.240992997279449561 ) ) ;
#45631=CARTESIAN_POINT ( 'NONE',  ( 185.2935054837330711, 266.5941941465212039, 14.38430047949690049 ) ) ;
#45633=CARTESIAN_POINT ( 'NONE',  ( 179.7701192287809135, 262.8885550775633533, -12.91845977881626339 ) ) ;
#45636=CARTESIAN_POINT ( 'NONE',  ( 148.3519871123208986, 273.6938162480936398, 8.180046468253793890 ) ) ;
#45638=CARTESIAN_POINT ( 'NONE',  ( 155.4186054393023255, 261.4540742680644598, 17.05753227160644769 ) ) ;
#45640=CARTESIAN_POINT ( 'NONE',  ( -22.42236680055709641, 157.8615022471902591, 0.000000000000000000 ) ) ;
#45645=EDGE_LOOP ( 'NONE', ( #100121, #80115, #49688, #65227 ) ) ;
#45646=CARTESIAN_POINT ( 'NONE',  ( 196.1556763520775064, 289.0687990662340212, -17.19517613012386548 ) ) ;
#45649=CARTESIAN_POINT ( 'NONE',  ( 203.4696564630250464, 278.2272125378923988, -16.38980782817167636 ) ) ;
#45652=ORIENTED_EDGE ( 'NONE', *, *, #67929, .T. ) ;
#45655=ORIENTED_EDGE ( 'NONE', *, *, #11433, .T. ) ;
#45656=CARTESIAN_POINT ( 'NONE',  ( 191.5451565139252068, 298.8810523045859213, 7.782291334092181323 ) ) ;
#45662=CARTESIAN_POINT ( 'NONE',  ( 190.3144310910409445, 301.0127312671879167, -1.334877248546042949 ) ) ;
#45663=CARTESIAN_POINT ( 'NONE',  ( 149.3141802193904368, 272.0272488999566463, -11.40332369054239336 ) ) ;
#45665=CARTESIAN_POINT ( 'NONE',  ( 195.7291850945597957, 291.6341022226063160, 17.08310330964873813 ) ) ;
#45666=CARTESIAN_POINT ( 'NONE',  ( 158.1219681159314518, 265.1686937430463331, 17.54345935383751964 ) ) ;
#45668=CARTESIAN_POINT ( 'NONE',  ( 190.7705347155322499, 300.2227366160529414, 3.504769718465625239 ) ) ;
#45670=EDGE_LOOP ( 'NONE', ( #96956, #37059, #94324, #28380 ) ) ;
#45671=CARTESIAN_POINT ( 'NONE',  ( 174.8213806158123589, 292.3284732554488414, -0.08473646757267205842 ) ) ;
#45678=CARTESIAN_POINT ( 'NONE',  ( 146.8358616138309571, 276.3198226421291679, 4.054088818585255716 ) ) ;
#45679=CARTESIAN_POINT ( 'NONE',  ( 148.2267527339363369, 273.9107285543102535, 7.913369084260907016 ) ) ;
#45680=CARTESIAN_POINT ( 'NONE',  ( 149.2561433752359505, 272.1277716627430436, 12.99353668144589946 ) ) ;
#45682=CARTESIAN_POINT ( 'NONE',  ( 147.2930760453491246, 275.5279040167861240, 0.1825760380121495829 ) ) ;
#45683=CARTESIAN_POINT ( 'NONE',  ( 191.4852287632733123, 298.9848502134979071, -9.870565261052552941 ) ) ;
#45684=CARTESIAN_POINT ( 'NONE',  ( 149.0761751337341821, 272.4394858007734683, 11.56094486755886130 ) ) ;
#45687=CARTESIAN_POINT ( 'NONE',  ( 86.69683407628214411, 230.8615022471903160, 5.000000000000046185 ) ) ;
#45689=CARTESIAN_POINT ( 'NONE',  ( 168.7836086128107524, 286.6128497672082176, 4.077482129993557081 ) ) ;
#45692=CARTESIAN_POINT ( 'NONE',  ( 149.7654984860464253, 271.2455427317246404, -12.38634015387427034 ) ) ;
#45695=AXIS2_PLACEMENT_3D ( 'NONE', #68826, #30337, #67336 ) ;
#45698=B_SPLINE_CURVE_WITH_KNOTS ( 'NONE', 3,
 ( #24987, #10809, #58380, #4186 ),
 .UNSPECIFIED., .F., .F.,
 ( 4, 4 ),
 ( 0.005865586104323563567, 0.01086301216498964349 ),
 .UNSPECIFIED. ) ;
#45700=EDGE_CURVE ( 'NONE', #33613, #51377, #44202, .T. ) ;
#45701=CARTESIAN_POINT ( 'NONE',  ( -17.42236680055705023, 149.2012482093457777, 0.000000000000000000 ) ) ;
#45702=CARTESIAN_POINT ( 'NONE',  ( 165.5469076125238814, 284.0653433844562983, -8.492543197847592040 ) ) ;
#45704=CARTESIAN_POINT ( 'NONE',  ( 163.4222916751007801, 247.5912830598222172, -10.52132777929285012 ) ) ;
#45708=CARTESIAN_POINT ( 'NONE',  ( 44.46005344233068257, 203.1427522451418781, -10.00000000000009415 ) ) ;
#45709=CARTESIAN_POINT ( 'NONE',  ( 120.4447615282330588, 240.3458772461660544, 9.188101187500095079 ) ) ;
#45710=CARTESIAN_POINT ( 'NONE',  ( 198.9832789858017463, 285.9978462703757600, -18.55676541969546278 ) ) ;
#45712=CARTESIAN_POINT ( 'NONE',  ( 162.2336410148055279, 251.8862672885301492, -14.09881826716025799 ) ) ;
#45713=CARTESIAN_POINT ( 'NONE',  ( 157.7365441389748923, 257.4392866714015895, 18.13124212464487073 ) ) ;
#45714=CARTESIAN_POINT ( 'NONE',  ( 175.4373900952620886, 253.5400337193396467, -3.935082475582811323 ) ) ;
#45715=CARTESIAN_POINT ( 'NONE',  ( 31.83936385565518279, 195.3149278399160664, 9.188101187500093303 ) ) ;
#45717=EDGE_LOOP ( 'NONE', ( #46931, #26372, #29404 ) ) ;
#45718=CARTESIAN_POINT ( 'NONE',  ( 199.3868061948075194, 268.7461186553251764, -9.827356238820643242 ) ) ;
#45720=( BOUNDED_CURVE ( )  B_SPLINE_CURVE ( 2, ( #48855, #78254, #8834, #39703, #33139, #71159, #70633, #1244, #32126 ),
 .UNSPECIFIED., .F., .T. ) 
 B_SPLINE_CURVE_WITH_KNOTS ( ( 3, 2, 2, 2, 3 ),
 ( 0.7620967741935483764, 0.7634408602150537515, 0.7661290322580645018, 0.7688172043010752521, 0.7701612903225806273 ),
 .UNSPECIFIED. ) 
 CURVE ( )  GEOMETRIC_REPRESENTATION_ITEM ( )  RATIONAL_B_SPLINE_CURVE ( ( 0.9330127018922194093, 0.9330127018922194093, 1.000000000000000000, 0.8660254037844387076, 1.000000000000000000, 0.8660254037844387076, 1.000000000000000000, 0.9330127018922194093, 0.9330127018922194093 ) ) 
 REPRESENTATION_ITEM ( '' )  );
#45722=CARTESIAN_POINT ( 'NONE',  ( 190.3625087333586521, 300.9294583479858147, -4.271886578030237303 ) ) ;
#45724=CARTESIAN_POINT ( 'NONE',  ( 181.2440676231241241, 294.5520841294345473, -6.623935519155441654 ) ) ;
#45725=CARTESIAN_POINT ( 'NONE',  ( 164.1488579720687255, 250.0635283098263244, 10.33718753367986132 ) ) ;
#45727=CARTESIAN_POINT ( 'NONE',  ( 110.3501529135968013, 224.5177522451418213, 5.000000000000051514 ) ) ;
#45728=CARTESIAN_POINT ( 'NONE',  ( 175.6063544791335573, 254.0105997054014040, 8.344378697908656051 ) ) ;
#45730=CARTESIAN_POINT ( 'NONE',  ( 202.7865629936218284, 279.4103651332174536, 17.10878160033216133 ) ) ;
#45732=CARTESIAN_POINT ( 'NONE',  ( 18.65997361151702449, 172.3923013555409796, 4.594050593750050204 ) ) ;
#45738=CARTESIAN_POINT ( 'NONE',  ( 195.0059191867570405, 275.0380839613920330, -16.17140022037657943 ) ) ;
#45739=CARTESIAN_POINT ( 'NONE',  ( 75.81765026128996965, 205.3923013555409796, 4.594050593750050204 ) ) ;
#45740=CARTESIAN_POINT ( 'NONE',  ( 161.5875797534026219, 250.7690973254556468, 12.95526170413129030 ) ) ;
#45742=CARTESIAN_POINT ( 'NONE',  ( 46.26427303354824261, 207.5177522451419065, 5.000000000000046185 ) ) ;
#45743=CARTESIAN_POINT ( 'NONE',  ( 207.5338226493333025, 271.1878702128032614, 6.432541580693135863 ) ) ;
#45744=VERTEX_POINT ( 'NONE', #54800 ) ;
#45745=CARTESIAN_POINT ( 'NONE',  ( 14.88889434582250537, 172.7365022471902023, -10.00000000000009059 ) ) ;
#45746=CARTESIAN_POINT ( 'NONE',  ( 164.4414259850711915, 245.8260906552167171, -6.983224448873608381 ) ) ;
#45747=CARTESIAN_POINT ( 'NONE',  ( 139.2268610206906203, 245.0643266524160140, 9.188101187500095079 ) ) ;
#45749=CARTESIAN_POINT ( 'NONE',  ( 164.4637126465671884, 260.7786515323086860, -16.15215151101600455 ) ) ;
#45750=CARTESIAN_POINT ( 'NONE',  ( 192.7288556637334125, 292.1918731402626577, -15.52061534916644447 ) ) ;
#45751=CARTESIAN_POINT ( 'NONE',  ( -27.42236680055714260, 166.5217562850347406, 1.224646799147364892E-15 ) ) ;
#45759=CARTESIAN_POINT ( 'NONE',  ( 143.0969038086192597, 260.4263049900483225, -7.951529393128359935 ) ) ;
#45761=CARTESIAN_POINT ( 'NONE',  ( 172.9311764467664716, 268.4779053881692334, -17.72160738022306603 ) ) ;
#45764=CARTESIAN_POINT ( 'NONE',  ( 206.8804362336228166, 272.3195686817890078, 7.951031312702417253 ) ) ;
#45765=DIRECTION ( 'NONE',  ( -0.8660254037844387076, -0.4999999999999998890, -0.000000000000000000 ) ) ;
#45767=CARTESIAN_POINT ( 'NONE',  ( 149.0092716443465406, 273.2528299346296876, -9.628675884572079013 ) ) ;
#45769=CARTESIAN_POINT ( 'NONE',  ( 38.54221318313706490, 186.3927522451418213, 10.00000000000009948 ) ) ;
#45771=CARTESIAN_POINT ( 'NONE',  ( 153.4613150239306094, 264.8442007126561748, -16.86932470306368259 ) ) ;
#45772=CARTESIAN_POINT ( 'NONE',  ( 197.0571419530650701, 283.2438395117923733, -17.78737236506320940 ) ) ;
#45775=CARTESIAN_POINT ( 'NONE',  ( 149.7119746935222793, 271.3382486597900538, 12.05352563709836922 ) ) ;
#45778=VERTEX_POINT ( 'NONE', #16306 ) ;
#45779=CARTESIAN_POINT ( 'NONE',  ( 146.7434471017767521, 276.4798892723637209, 0.7354350123930684102 ) ) ;
#45786=CARTESIAN_POINT ( 'NONE',  ( 109.5926410088830920, 224.8923013555410080, 4.594050593750050204 ) ) ;
#45787=CARTESIAN_POINT ( 'NONE',  ( 200.2316334480823912, 283.8356329158505105, 17.02791935830326508 ) ) ;
#45789=CARTESIAN_POINT ( 'NONE',  ( 177.9271722668541429, 269.0421873018364067, -16.58597972526078479 ) ) ;
#45790=CARTESIAN_POINT ( 'NONE',  ( 131.2304340799682052, 258.1199935810940929, 2.679491924311251605 ) ) ;
#45794=ORIENTED_EDGE ( 'NONE', *, *, #80026, .T. ) ;
#45795=CARTESIAN_POINT ( 'NONE',  ( 155.9200296242932495, 280.3860598674420430, -5.539708607631867565 ) ) ;
#45796=VERTEX_POINT ( 'NONE', #78626 ) ;
#45798=ORIENTED_EDGE ( 'NONE', *, *, #28093, .T. ) ;
#45799=CARTESIAN_POINT ( 'NONE',  ( 164.4405316900629259, 245.8276396196081350, -6.144538123479245328 ) ) ;
#45800=DIRECTION ( 'NONE',  ( -0.8660254037844387076, -0.4999999999999998890, -0.000000000000000000 ) ) ;
#45801=CARTESIAN_POINT ( 'NONE',  ( 147.8819534105757043, 274.5079385007862811, -9.338341377131436971 ) ) ;
#45804=CARTESIAN_POINT ( 'NONE',  ( 203.0722418932742244, 271.9993247240984147, -11.15264743686702431 ) ) ;
#45806=CARTESIAN_POINT ( 'NONE',  ( 198.4552072442472195, 277.1389102503209187, -15.27480873049025334 ) ) ;
#45808=EDGE_LOOP ( 'NONE', ( #65978, #12076, #68227, #55741 ) ) ;
#45809=CARTESIAN_POINT ( 'NONE',  ( 202.3425522658138505, 280.1794142728863903, 15.86053073629060961 ) ) ;
#45814=CARTESIAN_POINT ( 'NONE',  ( 172.8951663193395234, 288.9549776225803157, 8.104654168245465584 ) ) ;
#45816=CARTESIAN_POINT ( 'NONE',  ( 193.9979983253333842, 262.2552985615510579, -0.8131695963413709816 ) ) ;
#45818=CARTESIAN_POINT ( 'NONE',  ( 155.7883366700203283, 260.8136809913161756, -17.92854480136704609 ) ) ;
#45822=CARTESIAN_POINT ( 'NONE',  ( 2.890834060677622830, 179.1427522451419350, -10.00000000000009415 ) ) ;
#45823=CARTESIAN_POINT ( 'NONE',  ( 193.4895222550737799, 267.7935039460338089, -10.92382970030925904 ) ) ;
#45825=CARTESIAN_POINT ( 'NONE',  ( 167.5469267500292574, 266.7168544022062520, -17.80679023418265672 ) ) ;
#45827=CARTESIAN_POINT ( 'NONE',  ( 162.7435819479956933, 250.7668427907593411, -13.06080741167749082 ) ) ;
#45828=CARTESIAN_POINT ( 'NONE',  ( -5.047471817081990331, 158.7048013555409796, 4.594050593750051981 ) ) ;
#45832=ORIENTED_EDGE ( 'NONE', *, *, #77318, .T. ) ;
#45836=CARTESIAN_POINT ( 'NONE',  ( 202.6121680448818836, 279.7124260450182192, -17.20265281220889619 ) ) ;
#45838=CARTESIAN_POINT ( 'NONE',  ( 152.8043993858796910, 278.1759084314348911, 3.722792219655572055 ) ) ;
#45839=CARTESIAN_POINT ( 'NONE',  ( 18.14551070619625150, 181.2833772461660544, -9.188101187500095079 ) ) ;
#45841=CARTESIAN_POINT ( 'NONE',  ( 121.5815934185826421, 234.8768266524159856, -9.188101187500091527 ) ) ;
#45842=CARTESIAN_POINT ( 'NONE',  ( 181.4801324847757371, 293.6536699639055996, -6.265443341854637360 ) ) ;
#45844=CARTESIAN_POINT ( 'NONE',  ( 150.0125358617781046, 271.5677179990414629, -11.81783918238916975 ) ) ;
#45846=CARTESIAN_POINT ( 'NONE',  ( 177.9706801847183044, 283.7805232136731206, -15.20094465328249100 ) ) ;
#45847=CARTESIAN_POINT ( 'NONE',  ( 190.7809735039951420, 299.8080322731761953, -4.803559423902265202 ) ) ;
#45848=CARTESIAN_POINT ( 'NONE',  ( 157.1338510812060747, 258.4831816688264325, 17.88958125218800888 ) ) ;
#45850=CARTESIAN_POINT ( 'NONE',  ( 207.6129110656513035, 271.0508850574501025, -5.265106572941297358 ) ) ;
#45851=CARTESIAN_POINT ( 'NONE',  ( 190.0457908948199304, 284.8755663360458925, 17.21853735360699034 ) ) ;
#45853=CARTESIAN_POINT ( 'NONE',  ( 189.2525414291476693, 262.7352831944227773, 8.031418296191455752 ) ) ;
#45854=CARTESIAN_POINT ( 'NONE',  ( 168.4817192172301930, 278.3851404970916406, 14.18369869134152950 ) ) ;
#45855=DIRECTION ( 'NONE',  ( -0.8660254037844387076, -0.4999999999999998890, -0.000000000000000000 ) ) ;
#45856=CARTESIAN_POINT ( 'NONE',  ( 191.2111338740054975, 299.4595964878050154, -9.718193530796334301 ) ) ;
#45857=DIRECTION ( 'NONE',  ( -0.4999999999999998890, 0.8660254037844387076, 0.000000000000000000 ) ) ;
#45860=CARTESIAN_POINT ( 'NONE',  ( 184.6987793500286159, 269.2149976013500918, 16.08913214107394651 ) ) ;
#45861=CARTESIAN_POINT ( 'NONE',  ( 95.54687826519547400, 213.7202760586659167, -5.415160957724236172E-17 ) ) ;
#45863=CARTESIAN_POINT ( 'NONE',  ( 151.4327733764141612, 268.3577379114237829, 14.90862905801242100 ) ) ;
#45864=CARTESIAN_POINT ( 'NONE',  ( 158.5750977676651132, 259.0605719887398095, -17.09334224669940028 ) ) ;
#45866=CARTESIAN_POINT ( 'NONE',  ( 192.0134456341967564, 277.2561770618384003, 16.56410798670358631 ) ) ;
#45867=CARTESIAN_POINT ( 'NONE',  ( 196.6029714102277808, 290.1206599289108112, 17.93210582400232767 ) ) ;
#45868=CARTESIAN_POINT ( 'NONE',  ( 198.5511052797322975, 286.7463930869835167, -17.24711022262289006 ) ) ;
#45869=CARTESIAN_POINT ( 'NONE',  ( 149.7247407264208618, 272.0633196944937140, -11.44969454563192279 ) ) ;
#45870=ADVANCED_FACE ( 'NONE', ( #34029 ), #12726, .T. ) ;
#45872=CARTESIAN_POINT ( 'NONE',  ( 146.8312060062178830, 276.3278863910550172, -4.807241325481028227 ) ) ;
#45873=CARTESIAN_POINT ( 'NONE',  ( 196.3956310503436953, 264.1850728776087180, 4.154333235580330630 ) ) ;
#45874=VERTEX_POINT ( 'NONE', #50204 ) ;
#45876=CARTESIAN_POINT ( 'NONE',  ( 178.7883952590142940, 280.5407180839665102, 15.89476656820465728 ) ) ;
#45877=DIRECTION ( 'NONE',  ( -0.8660254037844387076, -0.4999999999999998890, -0.000000000000000000 ) ) ;
#45878=CARTESIAN_POINT ( 'NONE',  ( 149.0164813726494799, 272.5428784278667536, -11.67305721329070423 ) ) ;
#45879=ORIENTED_EDGE ( 'NONE', *, *, #14840, .T. ) ;
#45881=CARTESIAN_POINT ( 'NONE',  ( 159.9671766634011192, 253.5757178060795809, 16.49140845334465411 ) ) ;
#45882=CARTESIAN_POINT ( 'NONE',  ( 178.5747556458698853, 290.2456356026511344, -10.84108072231283515 ) ) ;
#45884=CARTESIAN_POINT ( 'NONE',  ( 188.1799812681836102, 277.7687690950278920, 17.76449826988982394 ) ) ;
#45885=CARTESIAN_POINT ( 'NONE',  ( -17.42236680055705023, 149.2012482093457777, 0.000000000000000000 ) ) ;
#45887=CARTESIAN_POINT ( 'NONE',  ( 188.0035612729766115, 279.2325960380115362, 17.82077010991123700 ) ) ;
#45889=ORIENTED_EDGE ( 'NONE', *, *, #54999, .T. ) ;
#45890=CYLINDRICAL_SURFACE ( 'NONE', #85419, 10.00000000000010658 ) ;
#45892=CARTESIAN_POINT ( 'NONE',  ( 181.6041183721993946, 291.2867937091023123, -11.32870443584723930 ) ) ;
#45893=VERTEX_POINT ( 'NONE', #72538 ) ;
#45895=CARTESIAN_POINT ( 'NONE',  ( 159.0925993676364953, 255.0905301174903457, 16.49470061235192020 ) ) ;
#45897=CARTESIAN_POINT ( 'NONE',  ( 193.2875054959514785, 295.8632153432003520, -12.54951740302059982 ) ) ;
#45898=B_SPLINE_CURVE_WITH_KNOTS ( 'NONE', 3,
 ( #39743, #70672, #46875, #15457 ),
 .UNSPECIFIED., .F., .F.,
 ( 4, 4 ),
 ( 1.260064970365687123E-16, 0.005076538409987941397 ),
 .UNSPECIFIED. ) ;
#45899=CARTESIAN_POINT ( 'NONE',  ( 153.0444155045374544, 265.5662918618958201, -16.15173036748435109 ) ) ;
#45906=CARTESIAN_POINT ( 'NONE',  ( 171.1295603993285965, 249.6517061031812545, 4.344809613321301889 ) ) ;
#45910=CARTESIAN_POINT ( 'NONE',  ( 198.0529239074794532, 286.9055631288374570, 16.94304631173295306 ) ) ;
#45911=CARTESIAN_POINT ( 'NONE',  ( 171.5095832474949304, 270.2981375784696638, 16.50875514196534155 ) ) ;
#45913=CARTESIAN_POINT ( 'NONE',  ( 165.5170328988546373, 275.0156723620771686, -15.58398378318264754 ) ) ;
#45914=CARTESIAN_POINT ( 'NONE',  ( 206.3528985702396596, 273.2332907176744925, -9.687807306503337657 ) ) ;
#45915=CARTESIAN_POINT ( 'NONE',  ( 197.6236242130358676, 272.7773651221880300, -13.22260735042824287 ) ) ;
#45916=AXIS2_PLACEMENT_3D ( 'NONE', #95540, #87948, #17476 ) ;
#45918=CARTESIAN_POINT ( 'NONE',  ( 146.9700173529739970, 276.0874580858064746, -5.099093031535578469 ) ) ;
#45919=CARTESIAN_POINT ( 'NONE',  ( 169.7010302950471612, 250.3720810868360047, -5.484198761109861486 ) ) ;
#45922=CARTESIAN_POINT ( 'NONE',  ( 183.4601068508181640, 284.4945872344713962, -15.13106351166021213 ) ) ;
#45923=CARTESIAN_POINT ( 'NONE',  ( 123.8009570636627785, 230.0327760586659736, 1.948934522072303157E-15 ) ) ;
#45924=ORIENTED_EDGE ( 'NONE', *, *, #44375, .F. ) ;
#45925=CARTESIAN_POINT ( 'NONE',  ( 183.7739455050309232, 260.7523580455279557, -9.220920309613330090 ) ) ;
#45927=CARTESIAN_POINT ( 'NONE',  ( 188.2554578474332914, 273.5037763784579852, 15.65903759604143985 ) ) ;
#45929=B_SPLINE_CURVE_WITH_KNOTS ( 'NONE', 3,
 ( #9592, #63772, #79520, #89141 ),
 .UNSPECIFIED., .F., .F.,
 ( 4, 4 ),
 ( 0.008366579159829847998, 0.01473107717590894927 ),
 .UNSPECIFIED. ) ;
#45930=CARTESIAN_POINT ( 'NONE',  ( 162.8931802014337791, 249.0911889412991229, -10.32038157250286048 ) ) ;
#45931=EDGE_CURVE ( 'NONE', #96482, #76355, #24718, .T. ) ;
#45933=CARTESIAN_POINT ( 'NONE',  ( 180.7483976610911611, 294.0911617732556351, -2.543390022621885294 ) ) ;
#45934=CARTESIAN_POINT ( 'NONE',  ( 206.7927593038066618, 270.4714295788825780, 5.070506503021109168 ) ) ;
#45937=ORIENTED_EDGE ( 'NONE', *, *, #55395, .T. ) ;
#45938=CARTESIAN_POINT ( 'NONE',  ( 148.4581628440222971, 273.5099144862561502, 10.38959067216531373 ) ) ;
#45939=ORIENTED_EDGE ( 'NONE', *, *, #99346, .T. ) ;
#45940=CARTESIAN_POINT ( 'NONE',  ( 56.22356517706933943, 203.2677522451418781, 10.00000000000009592 ) ) ;
#45943=CARTESIAN_POINT ( 'NONE',  ( 191.8443339775285494, 267.7755496645525000, -12.38404032343068373 ) ) ;
#45945=CARTESIAN_POINT ( 'NONE',  ( 195.5588106879092152, 265.2999770288793684, 4.407320425118734342 ) ) ;
#45946=CARTESIAN_POINT ( 'NONE',  ( 158.2848466404973919, 263.3015549465852700, 17.37201711831807316 ) ) ;
#45947=CARTESIAN_POINT ( 'NONE',  ( 10.75723147838630034, 177.0177522451418497, -10.00000000000009592 ) ) ;
#45948=CARTESIAN_POINT ( 'NONE',  ( 186.0921632850933065, 290.0109707162887958, -13.31660835586359681 ) ) ;
#45949=CARTESIAN_POINT ( 'NONE',  ( 156.8470823004346641, 280.2066661834281831, 5.893157905567727006 ) ) ;
#45951=VERTEX_POINT ( 'NONE', #66402 ) ;
#45952=CARTESIAN_POINT ( 'NONE',  ( 204.7552454032017408, 272.8428230285074960, -9.594377649449842949 ) ) ;
#45956=CARTESIAN_POINT ( 'NONE',  ( 189.6692937066967488, 270.4073510551538106, -14.09879195927397788 ) ) ;
#45957=CARTESIAN_POINT ( 'NONE',  ( 176.0535401773562683, 259.9697838701345631, -14.17309044617966407 ) ) ;
#45959=CARTESIAN_POINT ( 'NONE',  ( 169.3928097498865668, 252.4249310383071645, 11.01504250006889229 ) ) ;
#45960=CARTESIAN_POINT ( 'NONE',  ( 194.5047661587782386, 293.7548580291293092, 14.86680123054176583 ) ) ;
#45961=CARTESIAN_POINT ( 'NONE',  ( 191.3906598757142490, 282.8513481914541217, -16.97112179597618820 ) ) ;
#45963=CARTESIAN_POINT ( 'NONE',  ( 77.03558525930309031, 203.0327760586659451, 1.948934522072303157E-15 ) ) ;
#45964=CARTESIAN_POINT ( 'NONE',  ( 206.2041691044954348, 273.4908977089264113, -9.455375957961031474 ) ) ;
#45965=CARTESIAN_POINT ( 'NONE',  ( 147.2089949622447875, 275.6735367246781720, -3.633014386235353221 ) ) ;
#45968=B_SPLINE_CURVE_WITH_KNOTS ( 'NONE', 3,
 ( #80349, #40777, #33720, #42283, #88978, #10918, #95566, #57484, #34209, #9919, #4291, #3329, #19028, #72225, #41792, #87972, #2831, #96052, #50393, #26112, #64610, #34693, #11919, #65101, #95049, #25611, #35191, #2321, #49901, #56498, #80859, #71728, #18020, #3812, #49402, #11431, #73218, #42775, #65594, #33201, #64102, #27114, #19533, #72738, #56988, #73709, #94537, #48913, #25090, #55971 ),
 .UNSPECIFIED., .F., .F.,
 ( 4, 2, 2, 2, 2, 2, 2, 2, 2, 2, 2, 2, 2, 2, 2, 2, 2, 2, 2, 2, 2, 2, 2, 2, 4 ),
 ( 0.001408021394296337303, 0.001871204839914372654, 0.002334388285532408222, 0.002565980008341460158, 0.002681775869745926712, 0.002797571731150393700, 0.002913367592554860688, 0.003029163453959327242, 0.003260755176768255145, 0.003723938622386087534, 0.004187122068003919055, 0.005113488959239669701, 0.006039855850475420347, 0.006503039296093259675, 0.006966222741711099002, 0.007082018603115559051, 0.007139916533817849791, 0.007197814464520141398, 0.007313610325924579762, 0.007429406187329018127, 0.007660997910138013685, 0.007892589632947010977, 0.008124181355756005668, 0.008355773078565002093, 0.008818956524182994944 ),
 .UNSPECIFIED. ) ;
#45969=CARTESIAN_POINT ( 'NONE',  ( 161.1750406344237661, 251.4836360396366501, -14.21198410781773802 ) ) ;
#45974=CARTESIAN_POINT ( 'NONE',  ( 164.0407096501202204, 246.5201517067746977, -4.555688043559123379 ) ) ;
#45975=CARTESIAN_POINT ( 'NONE',  ( 157.3988263959001870, 258.0242309610243865, 16.72376558639979294 ) ) ;
#45977=AXIS2_PLACEMENT_3D ( 'NONE', #528, #31415, #16227 ) ;
#45978=CARTESIAN_POINT ( 'NONE',  ( 29.56604717072103483, 194.0024278399160949, 9.188101187500095079 ) ) ;
#45979=CARTESIAN_POINT ( 'NONE',  ( 55.81761577081934433, 203.0333772461660544, 9.188101187500095079 ) ) ;
#45982=CARTESIAN_POINT ( 'NONE',  ( 199.5166962049540018, 277.5858014024767613, 15.20220047213190995 ) ) ;
#45983=CARTESIAN_POINT ( 'NONE',  ( -22.42236680055709641, 157.8615022471902591, 0.000000000000000000 ) ) ;
#45984=CARTESIAN_POINT ( 'NONE',  ( -7.266922234329411978, 166.6115022471902591, 10.00000000000009592 ) ) ;
#45988=CARTESIAN_POINT ( 'NONE',  ( 150.6438662863770332, 269.7241650738195631, -14.92510732909997628 ) ) ;
#45991=CARTESIAN_POINT ( 'NONE',  ( 58.87550765610937731, 213.9869531367911009, 4.594050593750046652 ) ) ;
#45994=CARTESIAN_POINT ( 'NONE',  ( 159.7608930362198407, 253.9330115291272421, 15.38895778945778581 ) ) ;
#45995=CARTESIAN_POINT ( 'NONE',  ( 156.1095879582928774, 264.4631574034182222, 17.55859510772456389 ) ) ;
#45996=CARTESIAN_POINT ( 'NONE',  ( 153.3697773540452545, 276.7804196118793243, 7.402161975777190150 ) ) ;
#45999=CARTESIAN_POINT ( 'NONE',  ( 108.2753003872444140, 239.9865022471903444, -10.00000000000009415 ) ) ;
#46000=( BOUNDED_CURVE ( )  B_SPLINE_CURVE ( 2, ( #3858, #66644, #57538, #97574, #72791, #82409, #59016, #19078, #27163 ),
 .UNSPECIFIED., .F., .T. ) 
 B_SPLINE_CURVE_WITH_KNOTS ( ( 3, 2, 2, 2, 3 ),
 ( 0.07661290322580645296, 0.07795698924731182811, 0.08064516129032257841, 0.08333333333333332871, 0.08467741935483871774 ),
 .UNSPECIFIED. ) 
 CURVE ( )  GEOMETRIC_REPRESENTATION_ITEM ( )  RATIONAL_B_SPLINE_CURVE ( ( 0.9330127018922194093, 0.9330127018922194093, 1.000000000000000000, 0.8660254037844387076, 1.000000000000000000, 0.8660254037844387076, 1.000000000000000000, 0.9330127018922189652, 0.9330127018922192983 ) ) 
 REPRESENTATION_ITEM ( '' )  );
#46001=CARTESIAN_POINT ( 'NONE',  ( 161.3227470381586102, 251.2278010437646856, 14.45097375514160731 ) ) ;
#46002=CARTESIAN_POINT ( 'NONE',  ( 207.5338226493333025, 271.1878702128032614, 6.432541580693135863 ) ) ;
#46006=VERTEX_POINT ( 'NONE', #13220 ) ;
#46007=CARTESIAN_POINT ( 'NONE',  ( 206.7408728089182546, 272.5612996242556960, -10.63134519248043475 ) ) ;
#46008=CARTESIAN_POINT ( 'NONE',  ( 187.7710022618638277, 277.0665775429750397, -17.72351784843695555 ) ) ;
#46012=ORIENTED_EDGE ( 'NONE', *, *, #35961, .F. ) ;
#46014=CARTESIAN_POINT ( 'NONE',  ( 148.3874010092782498, 273.6324775792697892, -8.328854486678444857 ) ) ;
#46021=CARTESIAN_POINT ( 'NONE',  ( 178.0191268533054938, 276.9262132288450857, 17.58692550855656123 ) ) ;
#46022=EDGE_CURVE ( 'NONE', #104, #30236, #80486, .T. ) ;
#46024=CARTESIAN_POINT ( 'NONE',  ( 152.6977370281523179, 272.7175316449822731, 13.26472897831007458 ) ) ;
#46025=EDGE_CURVE ( 'NONE', #82781, #10047, #58445, .T. ) ;
#46026=CARTESIAN_POINT ( 'NONE',  ( 206.7893622945242385, 272.4773133715531230, -10.52881283832460291 ) ) ;
#46029=CARTESIAN_POINT ( 'NONE',  ( 161.8718470072856803, 283.0133716661769654, -3.127779434105778744 ) ) ;
#46031=CARTESIAN_POINT ( 'NONE',  ( 207.9328781051891042, 270.4966858882232259, -0.8820402142964423042 ) ) ;
#46032=CARTESIAN_POINT ( 'NONE',  ( 204.1780753366177237, 277.0001950557890495, 14.05599973203924158 ) ) ;
#46033=CARTESIAN_POINT ( 'NONE',  ( 198.6012358295098750, 286.6595644277572887, 18.21911298807435386 ) ) ;
#46034=CARTESIAN_POINT ( 'NONE',  ( 164.5827125224535905, 265.0803347849686702, -16.62742669594850753 ) ) ;
#46035=B_SPLINE_CURVE_WITH_KNOTS ( 'NONE', 3,
 ( #98711, #29296, #21201, #97709, #13107, #28787, #44972, #37860, #75910, #29782, #84519, #6490, #68769, #90640, #20699, #60654, #99693, #43967, #91610, #22183, #52080, #30277, #53076, #84030, #874, #38362, #87044, #24670, #379, #78393, #1887, #55554, #92616, #86537, #54054, #15555, #31268, #85011, #62154, #23657, #16074, #17068, #47959, #94613, #17577, #77388, #69771, #32769, #40357, #39844, #77895, #85532, #78901, #63675 ),
 .UNSPECIFIED., .F., .F.,
 ( 4, 2, 2, 2, 2, 2, 2, 2, 2, 2, 2, 2, 2, 2, 2, 2, 2, 2, 2, 2, 2, 2, 2, 2, 2, 2, 4 ),
 ( 0.0001092562925467074387, 0.0006072969982681204098, 0.001105337703989533408, 0.001354358056850239961, 0.001603378409710946298, 0.001727888586141281685, 0.001852398762571617072, 0.001976908939001952459, 0.002101419115432288064, 0.002350439468292954935, 0.002599459821153621373, 0.003097500526874954682, 0.004093581938317621301, 0.005089663349760287919, 0.005587704055481584366, 0.005836724408342232155, 0.005961234584772556050, 0.006085744761202879077, 0.006147999849418073551, 0.006210254937633268024, 0.006334765114063651767, 0.006583785466924451345, 0.006832805819785250923, 0.007081826172646049633, 0.007330846525506850078, 0.007579866878367648789, 0.008077907584089218454 ),
 .UNSPECIFIED. ) ;
#46036=CARTESIAN_POINT ( 'NONE',  ( 134.5444773117747275, 257.6744531367911577, 4.594050593750047540 ) ) ;
#46037=CARTESIAN_POINT ( 'NONE',  ( 159.6585898550698630, 255.0347362821099750, -15.85242424285993401 ) ) ;
#46038=CARTESIAN_POINT ( 'NONE',  ( 181.9960526061360326, 260.3811653260469825, 9.445214464232433826 ) ) ;
#46039=CARTESIAN_POINT ( 'NONE',  ( 71.35211999908521818, 205.8768266524160140, 9.188101187500098632 ) ) ;
#46041=B_SPLINE_CURVE_WITH_KNOTS ( 'NONE', 3,
 ( #78798, #92520, #31170, #39256 ),
 .UNSPECIFIED., .F., .F.,
 ( 4, 4 ),
 ( 0.04113468878722496835, 0.04887066958154939050 ),
 .UNSPECIFIED. ) ;
#46043=DIRECTION ( 'NONE',  ( 0.4999999999999998890, -0.8660254037844385966, 0.000000000000000000 ) ) ;
#46044=CARTESIAN_POINT ( 'NONE',  ( -27.42236680055714260, 166.5217562850347406, 1.224646799147364892E-15 ) ) ;
#46045=EDGE_LOOP ( 'NONE', ( #6564, #9439, #12717, #31026 ) ) ;
#46052=CARTESIAN_POINT ( 'NONE',  ( 2.233356772565878057, 160.5494855054051584, -2.679491924311248496 ) ) ;
#46053=CARTESIAN_POINT ( 'NONE',  ( 146.6647111637776106, 276.6162639173599587, -0.6373001129109082674 ) ) ;
#46055=CARTESIAN_POINT ( 'NONE',  ( 155.0303156110108489, 262.1266119787277944, 17.11986653161320859 ) ) ;
#46057=CARTESIAN_POINT ( 'NONE',  ( 76.95378796010953693, 224.4244531367911293, -4.594050593750046652 ) ) ;
#46058=VERTEX_POINT ( 'NONE', #31873 ) ;
#46060=EDGE_CURVE ( 'NONE', #52312, #43398, #90158, .T. ) ;
#46061=CARTESIAN_POINT ( 'NONE',  ( 200.5982530106205388, 283.2006292064855870, -16.76555514870729624 ) ) ;
#46066=CARTESIAN_POINT ( 'NONE',  ( 183.6775799446257622, 275.6805839496243493, 16.80015316766806421 ) ) ;
#46067=EDGE_CURVE ( 'NONE', #39162, #78092, #30647, .T. ) ;
#46068=CARTESIAN_POINT ( 'NONE',  ( 162.6897041064822247, 284.0413850360118317, 0.5105129000292804031 ) ) ;
#46069=DIRECTION ( 'NONE',  ( -0.8660254037844387076, -0.4999999999999998890, -0.000000000000000000 ) ) ;
#46070=CARTESIAN_POINT ( 'NONE',  ( 162.1730311952291572, 261.1847194969478210, 16.85311962717550571 ) ) ;
#46071=ORIENTED_EDGE ( 'NONE', *, *, #737, .T. ) ;
#46074=CARTESIAN_POINT ( 'NONE',  ( 156.6719645457748982, 274.0816551557289245, 13.52539259823061357 ) ) ;
#46076=CARTESIAN_POINT ( 'NONE',  ( 147.7561322771605319, 275.4500581284187888, -3.854405246717441447 ) ) ;
#46077=CARTESIAN_POINT ( 'NONE',  ( 153.2513309553138470, 265.2079037882803618, -16.24091495603130397 ) ) ;
#46081=CARTESIAN_POINT ( 'NONE',  ( 199.6331895497083337, 266.8549210871742048, 4.611541600118369111 ) ) ;
#46082=CARTESIAN_POINT ( 'NONE',  ( 152.5423653171682474, 268.4358682943698682, -15.78187745328793490 ) ) ;
#46083=CARTESIAN_POINT ( 'NONE',  ( 193.8477229354528220, 262.3541544976313844, 2.578193913946859706 ) ) ;
#46084=CARTESIAN_POINT ( 'NONE',  ( 184.8052499677449134, 263.9936221479479173, -12.13309983589799046 ) ) ;
#46086=CARTESIAN_POINT ( 'NONE',  ( 156.9199168296383391, 272.6955506662872608, 14.53585852203788598 ) ) ;
#46088=CARTESIAN_POINT ( 'NONE',  ( 146.8881680668833951, 276.2292252078784145, 4.973452195244782104 ) ) ;
#46089=CARTESIAN_POINT ( 'NONE',  ( 186.8476719251497968, 282.1398254177984768, 17.29477932248579819 ) ) ;
#46091=CARTESIAN_POINT ( 'NONE',  ( 207.0548180518391916, 272.0175305127218053, 7.721676452263806389 ) ) ;
#46096=CARTESIAN_POINT ( 'NONE',  ( 163.3401707525704296, 283.7542478731094207, -3.207333608244951062 ) ) ;
#46098=CARTESIAN_POINT ( 'NONE',  ( 198.5558597050348908, 286.7381581807989051, 17.16554469393394200 ) ) ;
#46099=CARTESIAN_POINT ( 'NONE',  ( -9.134289513013563067, 165.5333772461660828, 9.188101187500095079 ) ) ;
#46101=ORIENTED_EDGE ( 'NONE', *, *, #75275, .T. ) ;
#46102=CARTESIAN_POINT ( 'NONE',  ( 178.8506441891429120, 256.6935935793209751, 8.649200206363696353 ) ) ;
#46105=DIRECTION ( 'NONE',  ( 0.4999999999999998890, -0.8660254037844385966, 0.000000000000000000 ) ) ;
#46106=CARTESIAN_POINT ( 'NONE',  ( 11.05475416482865114, 183.3149278399161233, 9.188101187500093303 ) ) ;
#46109=CARTESIAN_POINT ( 'NONE',  ( 119.7014708956357794, 251.4637435831425023, 2.679491924311251605 ) ) ;
#46110=CARTESIAN_POINT ( 'NONE',  ( 157.4893260420801653, 257.8674809757739013, -18.30842125257398223 ) ) ;
#46112=CARTESIAN_POINT ( 'NONE',  ( 175.5045987706217829, 253.5154819701446058, -3.738308729259062435 ) ) ;
#46115=CARTESIAN_POINT ( 'NONE',  ( 75.43850382708453139, 204.3615022471901739, 5.000000000000051514 ) ) ;
#46117=CARTESIAN_POINT ( 'NONE',  ( 148.3190727836317535, 273.7508255376806119, 8.080277324579027365 ) ) ;
#46118=CARTESIAN_POINT ( 'NONE',  ( 32.11017034222032862, 189.3458772461660544, 9.188101187500095079 ) ) ;
#46122=CARTESIAN_POINT ( 'NONE',  ( 199.0363797504450929, 285.9058730480928716, -17.12190301149298222 ) ) ;
#46124=EDGE_CURVE ( 'NONE', #77820, #63549, #96239, .T. ) ;
#46125=CARTESIAN_POINT ( 'NONE',  ( 207.6727254509676186, 270.9472835030587703, 7.315149605389819953 ) ) ;
#46126=CARTESIAN_POINT ( 'NONE',  ( 185.1787217285512384, 266.7930642242706654, 13.70357059227357688 ) ) ;
#46127=CARTESIAN_POINT ( 'NONE',  ( 162.0955723731790101, 279.9228038994015719, -9.850904930694312611 ) ) ;
#46128=CARTESIAN_POINT ( 'NONE',  ( 164.0322825057177170, 281.5311351839372946, 8.862866254731592619 ) ) ;
#46133=CARTESIAN_POINT ( 'NONE',  ( 188.8338017993633571, 269.9617145311643185, -14.08363440685359791 ) ) ;
#46134=ORIENTED_EDGE ( 'NONE', *, *, #18760, .T. ) ;
#46138=ADVANCED_FACE ( 'NONE', ( #54667 ), #7586, .T. ) ;
#46139=ORIENTED_EDGE ( 'NONE', *, *, #41602, .F. ) ;
#46140=CARTESIAN_POINT ( 'NONE',  ( 23.90999230191033575, 194.6115022471903160, -5.000000000000047962 ) ) ;
#46144=CARTESIAN_POINT ( 'NONE',  ( 170.6538086303071111, 280.9384219949420185, -14.72317928558904754 ) ) ;
#46147=CARTESIAN_POINT ( 'NONE',  ( 187.1893300299016687, 272.3238949448195285, -16.82286396092820979 ) ) ;
#46150=CARTESIAN_POINT ( 'NONE',  ( 150.6790040019602088, 269.6633047651677089, 15.38315204620803378 ) ) ;
#46153=CARTESIAN_POINT ( 'NONE',  ( 52.39861964368810732, 194.3927522451417929, -10.00000000000009237 ) ) ;
#46154=ORIENTED_EDGE ( 'NONE', *, *, #82211, .T. ) ;
#46155=CARTESIAN_POINT ( 'NONE',  ( 148.0427192501136062, 274.2294838985851015, 9.385226820296049155 ) ) ;
#46156=CARTESIAN_POINT ( 'NONE',  ( 149.1939152435731728, 272.2355539484436235, -11.44223522189843933 ) ) ;
#46157=ORIENTED_EDGE ( 'NONE', *, *, #16678, .F. ) ;
#46158=CARTESIAN_POINT ( 'NONE',  ( 195.8947060313465443, 291.3474115503753410, 16.07878593000791767 ) ) ;
#46159=CARTESIAN_POINT ( 'NONE',  ( 158.5477485432647313, 265.3246957002631916, 17.03042601231237896 ) ) ;
#46161=CARTESIAN_POINT ( 'NONE',  ( 149.2561433752359505, 272.1277716627430436, 12.99353668144589946 ) ) ;
#46163=ORIENTED_EDGE ( 'NONE', *, *, #59614, .T. ) ;
#46165=CARTESIAN_POINT ( 'NONE',  ( 150.6487462746963502, 269.7157126861102370, 15.18501655901553704 ) ) ;
#46170=ORIENTED_EDGE ( 'NONE', *, *, #16976, .F. ) ;
#46174=CARTESIAN_POINT ( 'NONE',  ( 77.46154149802761424, 203.9824982072973967, 3.021315404115420679E-15 ) ) ;
#46175=CARTESIAN_POINT ( 'NONE',  ( 147.8465295590381743, 274.5692944114487091, 9.322947948439978205 ) ) ;
#46176=CARTESIAN_POINT ( 'NONE',  ( 190.1190668544949460, 301.3511120508678118, 4.410340539513557090 ) ) ;
#46177=CARTESIAN_POINT ( 'NONE',  ( 172.1606859485697498, 275.9764482197007851, -15.78976850212529826 ) ) ;
#46178=CARTESIAN_POINT ( 'NONE',  ( 164.1654149204426858, 248.3041558426086226, -9.671695341034215687 ) ) ;
#46179=CARTESIAN_POINT ( 'NONE',  ( 147.2658550951450422, 275.5750520855697800, -5.215660180131691526 ) ) ;
#46180=EDGE_CURVE ( 'NONE', #87041, #18408, #78507, .T. ) ;
#46181=CARTESIAN_POINT ( 'NONE',  ( 163.9020937770961552, 257.0909063598783746, 15.75990737960287369 ) ) ;
#46182=CARTESIAN_POINT ( 'NONE',  ( -22.42236680055709641, 157.8615022471902591, 0.000000000000000000 ) ) ;
#46187=CARTESIAN_POINT ( 'NONE',  ( 107.4275774994220001, 223.6423013555409796, -4.594050593750043987 ) ) ;
#46188=ORIENTED_EDGE ( 'NONE', *, *, #95834, .F. ) ;
#46190=CARTESIAN_POINT ( 'NONE',  ( 149.2237128415488598, 272.1839429948059319, -13.04302063563883607 ) ) ;
#46192=EDGE_CURVE ( 'NONE', #64644, #31200, #79222, .T. ) ;
#46195=CARTESIAN_POINT ( 'NONE',  ( 179.9795673731253487, 282.8863147452317435, -15.33225209653127585 ) ) ;
#46196=CARTESIAN_POINT ( 'NONE',  ( 189.9366275249276157, 301.6671062389771691, -0.07615766263248391343 ) ) ;
#46197=CARTESIAN_POINT ( 'NONE',  ( 168.6230640848619373, 286.4021248756633895, -8.144242964583304101 ) ) ;
#46199=CARTESIAN_POINT ( 'NONE',  ( 207.6067494229581314, 271.0615573356529353, -1.924113146155245868 ) ) ;
#46201=CARTESIAN_POINT ( 'NONE',  ( 49.80054343233477709, 192.8927522451417929, -10.00000000000009059 ) ) ;
#46202=CARTESIAN_POINT ( 'NONE',  ( 122.2847184155099995, 253.6589784336661069, -6.496448406907676862E-16 ) ) ;
#46203=CARTESIAN_POINT ( 'NONE',  ( 180.4966966598214242, 294.5715408904403603, -3.526636318079005239 ) ) ;
#46205=CARTESIAN_POINT ( 'NONE',  ( 157.7861133721078772, 257.3534302411229646, 18.03837896619386783 ) ) ;
#46206=CARTESIAN_POINT ( 'NONE',  ( 175.1236258135627679, 253.3313582753198716, -3.877381073628868524 ) ) ;
#46207=CARTESIAN_POINT ( 'NONE',  ( 48.99766571601688270, 199.0958772461660544, -9.188101187500095079 ) ) ;
#46208=CARTESIAN_POINT ( 'NONE',  ( 113.5436215935997808, 236.3615022471902307, -10.00000000000009592 ) ) ;
#46209=CARTESIAN_POINT ( 'NONE',  ( 189.4199209167946663, 300.3895034224956930, 3.306026617473488027 ) ) ;
#46217=CARTESIAN_POINT ( 'NONE',  ( 108.1850894041355957, 243.2677522451419065, -5.000000000000047962 ) ) ;
#46218=CARTESIAN_POINT ( 'NONE',  ( 172.9311764467664716, 268.4779053881692334, -17.72160738022306603 ) ) ;
#46219=ORIENTED_EDGE ( 'NONE', *, *, #8287, .T. ) ;
#46220=EDGE_CURVE ( 'NONE', #57499, #41965, #26080, .T. ) ;
#46221=B_SPLINE_CURVE_WITH_KNOTS ( 'NONE', 3,
 ( #36489, #6601, #67392, #83637 ),
 .UNSPECIFIED., .F., .F.,
 ( 4, 4 ),
 ( 0.01296617310113466065, 0.01931249317442805188 ),
 .UNSPECIFIED. ) ;
#46222=CARTESIAN_POINT ( 'NONE',  ( 189.8123550829396891, 301.8823524224806647, -0.5679054518196169354 ) ) ;
#46225=CARTESIAN_POINT ( 'NONE',  ( 31.65035466828360100, 179.8923013555409796, 4.594050593750050204 ) ) ;
#46228=CARTESIAN_POINT ( 'NONE',  ( 146.8729474948188454, 276.2555880120147549, 3.934020695290606273 ) ) ;
#46230=CARTESIAN_POINT ( 'NONE',  ( 174.6162333118450931, 286.4903673861072662, 10.29252846444475722 ) ) ;
#46231=CARTESIAN_POINT ( 'NONE',  ( 73.21957404993666785, 203.8923013555409796, 4.594050593750050204 ) ) ;
#46232=CARTESIAN_POINT ( 'NONE',  ( 161.3644539559160478, 251.1555625431813894, 12.97746593258196413 ) ) ;
#46237=AXIS2_PLACEMENT_3D ( 'NONE', #28625, #98555, #29142 ) ;
#46238=CARTESIAN_POINT ( 'NONE',  ( 27.87927540258900549, 200.2365022471903160, 2.944929066748280225E-16 ) ) ;
#46239=CARTESIAN_POINT ( 'NONE',  ( 207.9622466093905189, 270.4458181468041289, 3.586592550214158681 ) ) ;
#46240=CARTESIAN_POINT ( 'NONE',  ( 148.5637841791828464, 247.3923013555409796, 4.594050593750050204 ) ) ;
#46242=CARTESIAN_POINT ( 'NONE',  ( 164.5139018292655919, 259.6662038739244736, -17.01387605652571366 ) ) ;
#46243=CARTESIAN_POINT ( 'NONE',  ( 185.4827390772690876, 260.4226536598483790, 6.340749577449164676 ) ) ;
#46244=CARTESIAN_POINT ( 'NONE',  ( 164.4573439719129340, 245.7985198932525748, 1.541132361166968501 ) ) ;
#46247=CARTESIAN_POINT ( 'NONE',  ( 189.0720805967732758, 299.7343203868808246, 4.955419684386629164 ) ) ;
#46249=VERTEX_POINT ( 'NONE', #87666 ) ;
#46250=CARTESIAN_POINT ( 'NONE',  ( 190.8443993347725325, 300.0947993426467519, 8.522468760355437212 ) ) ;
#46251=CARTESIAN_POINT ( 'NONE',  ( 178.4979445755931806, 285.4942094443755991, 13.01262888890980385 ) ) ;
#46252=CARTESIAN_POINT ( 'NONE',  ( 156.3390064593949944, 279.7328267885979471, -5.286091551933326471 ) ) ;
#46256=CARTESIAN_POINT ( 'NONE',  ( 168.0457992865198662, 281.9604434737263432, -10.94842533682070140 ) ) ;
#46258=CARTESIAN_POINT ( 'NONE',  ( 157.5487431480040925, 257.7645675294749594, -18.29554785922338311 ) ) ;
#46260=DIRECTION ( 'NONE',  ( 0.4999999999999992784, -0.8660254037844390407, 0.000000000000000000 ) ) ;
#46261=CARTESIAN_POINT ( 'NONE',  ( 190.7144704529493140, 295.3703424786987739, 12.68450966750776843 ) ) ;
#46264=CARTESIAN_POINT ( 'NONE',  ( 207.6163508138795635, 271.0449272387537576, -1.385071889578343152 ) ) ;
#46265=CARTESIAN_POINT ( 'NONE',  ( 200.8251833487811666, 282.8075743310126882, -16.74393672780000131 ) ) ;
#46267=CARTESIAN_POINT ( 'NONE',  ( 190.6261097325742355, 281.3049748184752161, 16.80476181508462474 ) ) ;
#46269=VERTEX_POINT ( 'NONE', #26297 ) ;
#46270=CARTESIAN_POINT ( 'NONE',  ( 190.7862358025146534, 300.1955415356651429, 3.573119809004446257 ) ) ;
#46274=CARTESIAN_POINT ( 'NONE',  ( 191.3413020738616410, 299.2341385521244774, -8.295023558158421295 ) ) ;
#46276=CARTESIAN_POINT ( 'NONE',  ( 149.4456112649506281, 271.7996036513546869, -12.95648166494593667 ) ) ;
#46279=CARTESIAN_POINT ( 'NONE',  ( 96.25000326212280299, 232.5024278399160664, -9.188101187500093303 ) ) ;
#46280=CARTESIAN_POINT ( 'NONE',  ( 200.4116241316243645, 283.5238799070667142, 18.37703770054986663 ) ) ;
#46281=CARTESIAN_POINT ( 'NONE',  ( 190.9061255863007318, 299.9878863388391892, 7.497146773253707153 ) ) ;
#46290=CARTESIAN_POINT ( 'NONE',  ( 207.5583741822599393, 271.1453457103705205, 3.140867606700001424 ) ) ;
#46293=CARTESIAN_POINT ( 'NONE',  ( 167.7567270317426846, 281.0680522135961610, 11.62081748593863395 ) ) ;
#46294=ADVANCED_FACE ( 'NONE', ( #34872 ), #68793, .T. ) ;
#46295=CARTESIAN_POINT ( 'NONE',  ( 147.6095889327917803, 274.9796876144846465, -8.460961150142429332 ) ) ;
#46298=VERTEX_POINT ( 'NONE', #89114 ) ;
#46301=AXIS2_PLACEMENT_3D ( 'NONE', #94478, #25033, #50334 ) ;
#46302=CARTESIAN_POINT ( 'NONE',  ( -27.42236680055714260, 166.5217562850347406, 1.224646799147364892E-15 ) ) ;
#46307=CARTESIAN_POINT ( 'NONE',  ( 170.3868164922740505, 258.7065172848251677, -13.94078176683852810 ) ) ;
#46312=CARTESIAN_POINT ( 'NONE',  ( 178.6026051973306323, 254.4708812555809345, 5.813106864979912913 ) ) ;
#46313=CARTESIAN_POINT ( 'NONE',  ( 171.2382477466557305, 255.5321334004109133, 11.22453428535387943 ) ) ;
#46314=CARTESIAN_POINT ( 'NONE',  ( 194.4417037765285841, 263.4645709469522785, -0.7758984588134626437 ) ) ;
#46315=ORIENTED_EDGE ( 'NONE', *, *, #74265, .F. ) ;
#46316=DIRECTION ( 'NONE',  ( -0.8660254037844387076, -0.4999999999999998890, -0.000000000000000000 ) ) ;
#46317=CARTESIAN_POINT ( 'NONE',  ( 139.6993451667227646, 239.9155109091896065, 2.679491924311254714 ) ) ;
#46318=CARTESIAN_POINT ( 'NONE',  ( 161.1710432324487954, 255.5389764900634191, -16.30050909083865207 ) ) ;
#46319=CARTESIAN_POINT ( 'NONE',  ( 12.05626958406300098, 167.7677522451417929, -5.000000000000041744 ) ) ;
#46320=CARTESIAN_POINT ( 'NONE',  ( 95.60083130504949622, 219.8768266524159856, -9.188101187500093303 ) ) ;
#46321=CARTESIAN_POINT ( 'NONE',  ( 193.7449971229907533, 267.0691033174243785, -11.57060755736609003 ) ) ;
#46322=CARTESIAN_POINT ( 'NONE',  ( 174.5292714763907895, 282.4389550827968378, -15.07491654093877287 ) ) ;
#46323=CARTESIAN_POINT ( 'NONE',  ( 170.1035794950240359, 280.7289576921961611, -14.13142533609434004 ) ) ;
#46326=CARTESIAN_POINT ( 'NONE',  ( -0.8802452050168975139, 179.4869531367911293, 4.594050593750046652 ) ) ;
#46327=CARTESIAN_POINT ( 'NONE',  ( 106.5950644350847369, 243.8967562850346837, -4.648177544792955347E-16 ) ) ;
#46328=CARTESIAN_POINT ( 'NONE',  ( 187.0158281458424767, 295.8913910117000796, 8.146972701975970566 ) ) ;
#46329=ORIENTED_EDGE ( 'NONE', *, *, #15389, .T. ) ;
#46331=ORIENTED_EDGE ( 'NONE', *, *, #92946, .T. ) ;
#46332=CARTESIAN_POINT ( 'NONE',  ( 149.8800565769795696, 277.8602840446432083, 1.406115164305642651 ) ) ;
#46333=CARTESIAN_POINT ( 'NONE',  ( 198.4097421844162170, 265.0824675037606539, -3.039349057205883664 ) ) ;
#46339=CARTESIAN_POINT ( 'NONE',  ( 150.2560907947555791, 276.5831698823408829, 3.693008398856615138 ) ) ;
#46340=CARTESIAN_POINT ( 'NONE',  ( 25.39882055865594168, 173.2202760586659736, -5.415160957724236172E-17 ) ) ;
#46341=CARTESIAN_POINT ( 'NONE',  ( 121.2028808523094767, 228.5327760586659451, 1.948934522072303157E-15 ) ) ;
#46343=CARTESIAN_POINT ( 'NONE',  ( 182.9759581861415825, 257.6832614031042112, -2.318740451596759566 ) ) ;
#46345=DIRECTION ( 'NONE',  ( -0.8660254037844387076, -0.4999999999999998890, -0.000000000000000000 ) ) ;
#46346=CARTESIAN_POINT ( 'NONE',  ( 175.2394285866089092, 281.2249514087385478, -15.30553675368379274 ) ) ;
#46348=CARTESIAN_POINT ( 'NONE',  ( 195.8947060313465443, 291.3474115503753410, 16.07878593000791767 ) ) ;
#46349=CARTESIAN_POINT ( 'NONE',  ( 194.0672051292551430, 294.5127359636757660, 15.53337744471869364 ) ) ;
#46350=CARTESIAN_POINT ( 'NONE',  ( 207.1285138014047504, 271.8898857301724661, -5.752177443817618752 ) ) ;
#46352=CARTESIAN_POINT ( 'NONE',  ( 148.2352135776142177, 273.8960739431854563, -9.245976304249309052 ) ) ;
#46353=CARTESIAN_POINT ( 'NONE',  ( 189.5408823802965230, 263.1112053540622355, 7.934038689971461444 ) ) ;
#46354=CARTESIAN_POINT ( 'NONE',  ( 164.9640897230306962, 249.8568093354230371, -10.60187880726004650 ) ) ;
#46355=CARTESIAN_POINT ( 'NONE',  ( 18.14444784528756216, 192.8297689869269504, -2.679491924311252493 ) ) ;
#46357=CARTESIAN_POINT ( 'NONE',  ( 189.9457600613112902, 301.6512882219586800, 0.04117870562599101891 ) ) ;
#46358=CARTESIAN_POINT ( 'NONE',  ( 181.1288997990943699, 267.1128527043363192, -14.76543443481348206 ) ) ;
#46359=VERTEX_POINT ( 'NONE', #42420 ) ;
#46361=CARTESIAN_POINT ( 'NONE',  ( 179.4583960273904211, 270.4090523040318885, 17.47970616590194837 ) ) ;
#46362=CARTESIAN_POINT ( 'NONE',  ( 98.14495447654879001, 215.2202760586659167, -5.415160957724236172E-17 ) ) ;
#46364=CARTESIAN_POINT ( 'NONE',  ( 150.6790040019602088, 269.6633047651677089, 15.38315204620803378 ) ) ;
#46367=CARTESIAN_POINT ( 'NONE',  ( 193.0705714787908960, 277.9200196554784839, 16.36204623017445314 ) ) ;
#46374=EDGE_LOOP ( 'NONE', ( #14920, #82732, #17390, #29764 ) ) ;
#46375=FACE_OUTER_BOUND ( 'NONE', #15788, .T. ) ;
#46379=CARTESIAN_POINT ( 'NONE',  ( -27.42236680055714260, 166.5217562850347406, 1.224646799147364892E-15 ) ) ;
#46380=CARTESIAN_POINT ( 'NONE',  ( 196.4808189786114951, 290.3322341467384717, -17.84817245450773271 ) ) ;
#46381=ORIENTED_EDGE ( 'NONE', *, *, #54575, .F. ) ;
#46382=B_SPLINE_SURFACE_WITH_KNOTS ( 'NONE', 3, 1, ( 
 ( #9112, #32409 ),
 ( #77000, #85150 ),
 ( #7608, #34285 ),
 ( #77528, #38495 ),
 ( #3411, #63306 ),
 ( #513, #57070 ),
 ( #70405, #1013 ),
 ( #78023, #96130 ),
 ( #88051, #31400 ),
 ( #23, #46593 ),
 ( #18599, #86173 ),
 ( #49478, #69412 ),
 ( #23799, #54685 ),
 ( #61796, #92742 ),
 ( #38994, #85671 ),
 ( #16209, #11008 ),
 ( #16706, #47102 ),
 ( #47599, #8613 ),
 ( #41881, #72819 ),
 ( #65182, #26684 ),
 ( #32612, #63508 ),
 ( #18427, #50301 ),
 ( #72643, #69730 ),
 ( #96453, #88377 ),
 ( #81253, #95474 ),
 ( #65017, #11341 ),
 ( #26523, #1732 ),
 ( #64517, #73133 ),
 ( #57903, #26027 ),
 ( #33110, #56897 ),
 ( #9833, #94447 ),
 ( #49316, #40694 ),
 ( #41698, #18932 ),
 ( #80255, #86874 ) ),
 .UNSPECIFIED., .T., .F., .F.,
 ( 4, 2, 2, 2, 2, 2, 2, 2, 2, 2, 2, 2, 2, 2, 2, 2, 4 ),
 ( 2, 2 ),
 ( 0.000000000000000000, 0.06250000000000000000, 0.1250000000000000000, 0.1875000000000000000, 0.2500000000000000000, 0.3125000000000000000, 0.3750000000000000000, 0.4375000000000000000, 0.5000000000000000000, 0.5625000000000000000, 0.6250000000000000000, 0.6875000000000000000, 0.7500000000000000000, 0.8125000000000000000, 0.8750000000000000000, 0.9375000000000000000, 1.000000000000000000 ),
 ( 0.000000000000000000, 1.000000000000000000 ),
 .UNSPECIFIED. ) ;
#46385=CARTESIAN_POINT ( 'NONE',  ( 152.8230551641381396, 275.2333800586559391, 10.94291057119876420 ) ) ;
#46387=CARTESIAN_POINT ( 'NONE',  ( 194.3209714950976945, 287.2951553348708558, -17.43383849888540027 ) ) ;
#46390=CARTESIAN_POINT ( 'NONE',  ( 153.1164404339926080, 265.4415410246681972, 16.15325778160653414 ) ) ;
#46391=B_SPLINE_CURVE_WITH_KNOTS ( 'NONE', 3,
 ( #99000, #30580, #16376, #52872 ),
 .UNSPECIFIED., .F., .F.,
 ( 4, 4 ),
 ( 0.01049495788375092234, 0.01588891246743844368 ),
 .UNSPECIFIED. ) ;
#46393=CARTESIAN_POINT ( 'NONE',  ( 188.0737869051473012, 299.5124861214166572, -3.734995909225475863 ) ) ;
#46394=EDGE_CURVE ( 'NONE', #3492, #42198, #19978, .T. ) ;
#46397=DIRECTION ( 'NONE',  ( -0.8660254037844387076, -0.4999999999999998890, -0.000000000000000000 ) ) ;
#46404=CARTESIAN_POINT ( 'NONE',  ( 154.1166010273282438, 263.7092120612824147, -17.33440268030034304 ) ) ;
#46405=CARTESIAN_POINT ( 'NONE',  ( 167.5861325596884797, 256.5095974891418109, 15.03189046419509367 ) ) ;
#46409=CARTESIAN_POINT ( 'NONE',  ( 197.3327212804159103, 267.5970440452412049, 9.861675131224707513 ) ) ;
#46411=CARTESIAN_POINT ( 'NONE',  ( 202.5650245025327081, 277.7940810556053179, -15.59262966521933791 ) ) ;
#46413=ORIENTED_EDGE ( 'NONE', *, *, #67437, .F. ) ;
#46414=ORIENTED_EDGE ( 'NONE', *, *, #74352, .T. ) ;
#46415=CARTESIAN_POINT ( 'NONE',  ( 172.3434955255090699, 270.7759313641087715, 16.44516896573899345 ) ) ;
#46416=ORIENTED_EDGE ( 'NONE', *, *, #3450, .T. ) ;
#46417=CARTESIAN_POINT ( 'NONE',  ( 164.7580746839756785, 246.2315630300633131, 2.864679634845263223 ) ) ;
#46418=CARTESIAN_POINT ( 'NONE',  ( 205.9226911964632052, 273.9784317468465815, -10.54881836492553404 ) ) ;
#46419=CARTESIAN_POINT ( 'NONE',  ( 197.4711460630325632, 273.2607306827283651, -13.37816035555838035 ) ) ;
#46421=CARTESIAN_POINT ( 'NONE',  ( 147.1125781744767949, 275.8405354997948962, -5.216646253929903665 ) ) ;
#46422=CARTESIAN_POINT ( 'NONE',  ( 167.7614935370554008, 249.2934080693781027, -5.466447205817170030 ) ) ;
#46423=CARTESIAN_POINT ( 'NONE',  ( 52.99401211233780629, 194.7365022471902307, 10.00000000000009948 ) ) ;
#46424=CARTESIAN_POINT ( 'NONE',  ( 186.5050373472817284, 286.7230076623727086, -15.46505519963496589 ) ) ;
#46425=CARTESIAN_POINT ( 'NONE',  ( 116.0067284296028589, 225.5327760586659451, 1.948934522072303157E-15 ) ) ;
#46426=CARTESIAN_POINT ( 'NONE',  ( 185.3936501019832406, 261.9788283115297531, -9.055590929688063895 ) ) ;
#46428=CARTESIAN_POINT ( 'NONE',  ( 177.3729564342710034, 288.8709971325815786, -9.341937108417035063 ) ) ;
#46429=ORIENTED_EDGE ( 'NONE', *, *, #40480, .F. ) ;
#46433=CARTESIAN_POINT ( 'NONE',  ( 196.3021893095863959, 290.6416298092292436, 17.45656988653421138 ) ) ;
#46436=CARTESIAN_POINT ( 'NONE',  ( 177.1640229826661823, 288.7756000595433079, -9.303873556051240001 ) ) ;
#46440=CARTESIAN_POINT ( 'NONE',  ( 148.4042165687623083, 273.6033521758856750, -8.709765892313745539 ) ) ;
#46441=CARTESIAN_POINT ( 'NONE',  ( 46.40065236557224893, 186.0494855054051868, -2.679491924311248496 ) ) ;
#46442=ORIENTED_EDGE ( 'NONE', *, *, #86538, .T. ) ;
#46443=CARTESIAN_POINT ( 'NONE',  ( 188.0248464885530666, 266.0881402788382388, -11.75859168027853840 ) ) ;
#46444=CARTESIAN_POINT ( 'NONE',  ( 157.5254383281065600, 276.9205291671078157, 10.24548677782836670 ) ) ;
#46445=CARTESIAN_POINT ( 'NONE',  ( 192.5542622421363603, 262.6158310691380962, 4.646693819196449304 ) ) ;
#46446=CARTESIAN_POINT ( 'NONE',  ( 187.8362272217282509, 287.5474138042418417, -16.31275406728138933 ) ) ;
#46449=CARTESIAN_POINT ( 'NONE',  ( 15.10771242554802463, 167.9824982072973967, -5.229199737892075682E-14 ) ) ;
#46450=CARTESIAN_POINT ( 'NONE',  ( 185.4082111984200765, 289.5490485375350431, -13.24228234091079592 ) ) ;
#46452=CARTESIAN_POINT ( 'NONE',  ( 200.8665851640556070, 282.7358642834317948, -16.69422397739980823 ) ) ;
#46455=CARTESIAN_POINT ( 'NONE',  ( 190.9559560067148425, 299.9015775189195665, -4.895152914295826108 ) ) ;
#46457=CARTESIAN_POINT ( 'NONE',  ( 190.5138415335236743, 260.7340691433176971, 3.969352497929276691 ) ) ;
#46458=CARTESIAN_POINT ( 'NONE',  ( 183.2115438791051645, 276.4014300552622672, -16.48630945905322776 ) ) ;
#46459=CARTESIAN_POINT ( 'NONE',  ( 9.004826742577897392, 187.5530062829863027, -4.648177544792955347E-16 ) ) ;
#46461=CARTESIAN_POINT ( 'NONE',  ( 185.3661735032551974, 296.9378314866745541, -4.315971704415366261 ) ) ;
#46468=CARTESIAN_POINT ( 'NONE',  ( 70.81050702595493362, 217.8149278399160664, 9.188101187500093303 ) ) ;
#46469=FACE_OUTER_BOUND ( 'NONE', #9436, .T. ) ;
#46470=CARTESIAN_POINT ( 'NONE',  ( 192.5551423381268989, 297.1317055421444024, -13.20528585388119858 ) ) ;
#46471=CARTESIAN_POINT ( 'NONE',  ( 51.98364914125591696, 207.4865022471903160, 10.00000000000009415 ) ) ;
#46472=EDGE_CURVE ( 'NONE', #55984, #58170, #84061, .T. ) ;
#46473=CARTESIAN_POINT ( 'NONE',  ( 155.4810912439522212, 261.3458456796594760, -18.44218279064527266 ) ) ;
#46474=CARTESIAN_POINT ( 'NONE',  ( 161.4816992964961742, 250.9524876563463067, -12.92750327687364198 ) ) ;
#46477=CYLINDRICAL_SURFACE ( 'NONE', #59784, 17.82106496071139645 ) ;
#46478=CARTESIAN_POINT ( 'NONE',  ( 104.2879750871056928, 231.0177522451418781, -10.00000000000009592 ) ) ;
#46482=CARTESIAN_POINT ( 'NONE',  ( 164.2035862026529287, 246.2380412424262204, -4.285327505657965830 ) ) ;
#46483=CARTESIAN_POINT ( 'NONE',  ( 195.8449251089225811, 291.4336346372613775, 16.14492769602857081 ) ) ;
#46486=CARTESIAN_POINT ( 'NONE',  ( 41.01373370305532973, 203.6744531367911293, 4.594050593750047540 ) ) ;
#46487=VECTOR ( 'NONE', #3888, 1000.000000000000000 ) ;
#46488=CARTESIAN_POINT ( 'NONE',  ( 49.86334402403631572, 211.8464784336661637, 1.353441290958777327E-15 ) ) ;
#46491=CARTESIAN_POINT ( 'NONE',  ( 166.8965953329662568, 259.4083194189263963, 16.50658842888446642 ) ) ;
#46492=CARTESIAN_POINT ( 'NONE',  ( 148.6720373546558847, 247.4548013555409796, -4.594050593750042211 ) ) ;
#46493=CARTESIAN_POINT ( 'NONE',  ( 200.0612311737130540, 271.1040812139211198, -11.28087083430611592 ) ) ;
#46498=CARTESIAN_POINT ( 'NONE',  ( 67.02199298016300588, 203.3768266524159856, -9.188101187500093303 ) ) ;
#46501=CARTESIAN_POINT ( 'NONE',  ( 198.2414483977475754, 287.2827345394944700, 16.94931984969033678 ) ) ;
#46503=CARTESIAN_POINT ( 'NONE',  ( 153.3323608220152607, 276.8159399788930273, 7.221710064476104307 ) ) ;
#46506=CARTESIAN_POINT ( 'NONE',  ( 118.8119427999551760, 232.7365022471901739, -10.00000000000009059 ) ) ;
#46507=CARTESIAN_POINT ( 'NONE',  ( 161.7587802986029999, 250.4725692828850754, 14.33336164792646450 ) ) ;
#46508=CARTESIAN_POINT ( 'NONE',  ( 206.8968397926183229, 272.2911568841838061, 7.145103750817420440 ) ) ;
#46513=CARTESIAN_POINT ( 'NONE',  ( 159.2122473525774069, 254.8832937285494609, -16.22689353966294590 ) ) ;
#46514=CARTESIAN_POINT ( 'NONE',  ( 194.2437465966334571, 293.7439872100536036, 14.26449127607053313 ) ) ;
#46518=CARTESIAN_POINT ( 'NONE',  ( 173.3536786335043587, 251.5408331122485208, 0.1975630382450959399 ) ) ;
#46519=ORIENTED_EDGE ( 'NONE', *, *, #32298, .T. ) ;
#46521=CARTESIAN_POINT ( 'NONE',  ( 194.7900911235093133, 293.2606606935473792, -14.66228443412922999 ) ) ;
#46526=CARTESIAN_POINT ( 'NONE',  ( 153.8774496355958661, 270.8400042090240163, -14.95803277361719097 ) ) ;
#46531=VERTEX_POINT ( 'NONE', #95596 ) ;
#46536=CARTESIAN_POINT ( 'NONE',  ( 162.8480293090835005, 248.5859346546387769, -9.753154585358942086 ) ) ;
#46537=CARTESIAN_POINT ( 'NONE',  ( 164.0777181605478745, 246.4560510864015441, 5.763760713451748785 ) ) ;
#46538=CARTESIAN_POINT ( 'NONE',  ( 198.2819808855875863, 287.2125302111982705, 18.53535247371401695 ) ) ;
#46539=CARTESIAN_POINT ( 'NONE',  ( 157.8159121039657293, 257.3018173235443555, -17.05074702406642118 ) ) ;
#46540=CARTESIAN_POINT ( 'NONE',  ( 147.0210896547505399, 249.5643266524160140, 9.188101187500095079 ) ) ;
#46541=CARTESIAN_POINT ( 'NONE',  ( 163.9868517627649283, 262.4765967983332757, 17.63283070717088208 ) ) ;
#46543=CARTESIAN_POINT ( 'NONE',  ( 195.5194402673059528, 290.4564941404553338, -16.58695021901899125 ) ) ;
#46544=B_SPLINE_CURVE_WITH_KNOTS ( 'NONE', 3,
 ( #14673, #76484, #7061, #37943 ),
 .UNSPECIFIED., .F., .F.,
 ( 4, 4 ),
 ( 0.03315600111831654845, 0.04206725051739886034 ),
 .UNSPECIFIED. ) ;
#46545=CARTESIAN_POINT ( 'NONE',  ( 72.54255783352381570, 218.8149278399160664, -9.188101187500095079 ) ) ;
#46546=B_SPLINE_CURVE_WITH_KNOTS ( 'NONE', 3,
 ( #59721, #92183, #53127, #90687 ),
 .UNSPECIFIED., .F., .F.,
 ( 4, 4 ),
 ( 0.008574140209404586613, 0.01493074025973913956 ),
 .UNSPECIFIED. ) ;
#46548=CARTESIAN_POINT ( 'NONE',  ( 151.3284628043366524, 268.5384091220288383, 14.49047510809488237 ) ) ;
#46549=CARTESIAN_POINT ( 'NONE',  ( 183.8301289239822722, 272.2411597453489662, -17.34995410509954183 ) ) ;
#46551=AXIS2_PLACEMENT_3D ( 'NONE', #44060, #74512, #35971 ) ;
#46552=CARTESIAN_POINT ( 'NONE',  ( 189.6666044902458168, 284.7049877867155487, 17.41007887138588117 ) ) ;
#46556=CARTESIAN_POINT ( 'NONE',  ( 197.9002110616137884, 286.8208446428124034, 16.93415638934909495 ) ) ;
#46557=CARTESIAN_POINT ( 'NONE',  ( 191.7247331938518187, 298.5700163710982338, -9.650650827884682315 ) ) ;
#46561=CARTESIAN_POINT ( 'NONE',  ( 84.66726058227095564, 213.5643266524160140, 9.188101187500095079 ) ) ;
#46562=ORIENTED_EDGE ( 'NONE', *, *, #93239, .F. ) ;
#46564=ORIENTED_EDGE ( 'NONE', *, *, #2405, .T. ) ;
#46569=CARTESIAN_POINT ( 'NONE',  ( 164.5813345449211624, 245.5837619211427523, 1.447064457712487373 ) ) ;
#46572=CARTESIAN_POINT ( 'NONE',  ( 98.80083580102481733, 239.3967562850347122, -4.648177544792955347E-16 ) ) ;
#46576=CARTESIAN_POINT ( 'NONE',  ( 185.9340259846279650, 259.2058230038674083, 6.068042760456333617 ) ) ;
#46579=CARTESIAN_POINT ( 'NONE',  ( 200.9445292274600092, 282.6008612054670266, -16.62830946367346741 ) ) ;
#46582=VERTEX_POINT ( 'NONE', #78351 ) ;
#46583=CARTESIAN_POINT ( 'NONE',  ( 199.8090841209456698, 266.6002589468719748, 4.696852429360418135 ) ) ;
#46584=CARTESIAN_POINT ( 'NONE',  ( 181.8671909181005333, 291.4740761920108412, 9.945688837270767024 ) ) ;
#46587=CARTESIAN_POINT ( 'NONE',  ( 185.1689866119487249, 264.3216279136979665, -12.02713122612823504 ) ) ;
#46589=ADVANCED_FACE ( 'NONE', ( #72259 ), #19030, .F. ) ;
#46593=CARTESIAN_POINT ( 'NONE',  ( 162.6220573360242270, 248.9773295930640131, 10.49878733418918486 ) ) ;
#46597=CARTESIAN_POINT ( 'NONE',  ( 155.5770330754656072, 261.1796695529068302, 18.26969263326161297 ) ) ;
#46599=CARTESIAN_POINT ( 'NONE',  ( 178.7764833861777163, 287.8890986131111731, -12.93556640157745719 ) ) ;
#46603=CARTESIAN_POINT ( 'NONE',  ( 168.6924467145065307, 273.0555373943842028, 15.94676933137322372 ) ) ;
#46604=CARTESIAN_POINT ( 'NONE',  ( 163.3442030120103823, 283.7586793589214267, -3.186042431646216588 ) ) ;
#46606=CARTESIAN_POINT ( 'NONE',  ( 189.7858391559284428, 261.6244128272988974, 2.876109323323718492 ) ) ;
#46608=( BOUNDED_CURVE ( )  B_SPLINE_CURVE ( 2, ( #16796, #56792, #72529, #94339, #41078, #24894, #86762, #17296, #72015 ),
 .UNSPECIFIED., .F., .T. ) 
 B_SPLINE_CURVE_WITH_KNOTS ( ( 3, 2, 2, 2, 3 ),
 ( 0.7379032258064516236, 0.7392473118279569988, 0.7419354838709677491, 0.7446236559139784994, 0.7459677419354838745 ),
 .UNSPECIFIED. ) 
 CURVE ( )  GEOMETRIC_REPRESENTATION_ITEM ( )  RATIONAL_B_SPLINE_CURVE ( ( 0.9330127018922194093, 0.9330127018922194093, 1.000000000000000000, 0.8660254037844387076, 1.000000000000000000, 0.8660254037844387076, 1.000000000000000000, 0.9330127018922194093, 0.9330127018922194093 ) ) 
 REPRESENTATION_ITEM ( '' )  );
#46609=CARTESIAN_POINT ( 'NONE',  ( -9.405095999578703569, 171.5024278399160949, 9.188101187500095079 ) ) ;
#46610=CARTESIAN_POINT ( 'NONE',  ( 190.7050128886200753, 296.3700851971329939, -11.76232993392748583 ) ) ;
#46611=VERTEX_POINT ( 'NONE', #57522 ) ;
#46612=CARTESIAN_POINT ( 'NONE',  ( 174.9397293896797976, 255.2796731743772796, 8.271871831370619432 ) ) ;
#46614=CARTESIAN_POINT ( 'NONE',  ( 202.4695312440243526, 274.0310513324629937, -13.04997687495370684 ) ) ;
#46615=FACE_OUTER_BOUND ( 'NONE', #28646, .T. ) ;
#46616=CARTESIAN_POINT ( 'NONE',  ( 25.77718602916411328, 191.8149278399160949, -9.188101187500095079 ) ) ;
#46618=CARTESIAN_POINT ( 'NONE',  ( 178.9869515928023986, 273.9622273161898534, -16.75238912495000676 ) ) ;
#46621=CARTESIAN_POINT ( 'NONE',  ( 170.4904982756437732, 270.9068794242204490, -16.80084387905754895 ) ) ;
#46623=B_SPLINE_SURFACE_WITH_KNOTS ( 'NONE', 3, 1, ( 
 ( #94331, #77612 ),
 ( #30492, #46165 ),
 ( #31978, #1614 ),
 ( #8196, #61381 ),
 ( #53769, #61871 ),
 ( #92823, #46685 ),
 ( #9718, #87275 ),
 ( #26402, #19325 ),
 ( #25389, #11217 ),
 ( #42084, #65387 ),
 ( #41580, #50188 ),
 ( #56277, #4085 ),
 ( #64394, #72521 ),
 ( #3130, #41068 ),
 ( #79137, #95357 ),
 ( #49205, #89256 ),
 ( #72006, #25912 ),
 ( #95846, #2610 ),
 ( #17805, #81141 ),
 ( #34976, #26899 ),
 ( #34015, #57279 ),
 ( #32985, #71514 ),
 ( #63889, #48705 ),
 ( #11707, #64900 ),
 ( #58280, #88255 ),
 ( #10205, #48190 ),
 ( #88753, #49685 ),
 ( #40573, #96834 ),
 ( #96329, #18802 ),
 ( #10702, #33498 ),
 ( #65880, #2104 ),
 ( #80640, #73016 ),
 ( #56784, #79638 ),
 ( #3608, #27399 ) ),
 .UNSPECIFIED., .T., .F., .F.,
 ( 4, 2, 2, 2, 2, 2, 2, 2, 2, 2, 2, 2, 2, 2, 2, 2, 4 ),
 ( 2, 2 ),
 ( 0.000000000000000000, 0.06250000000000000000, 0.1250000000000000000, 0.1875000000000000000, 0.2500000000000000000, 0.3125000000000000000, 0.3750000000000000000, 0.4375000000000000000, 0.5000000000000000000, 0.5625000000000000000, 0.6250000000000000000, 0.6875000000000000000, 0.7500000000000000000, 0.8125000000000000000, 0.8750000000000000000, 0.9375000000000000000, 1.000000000000000000 ),
 ( 0.000000000000000000, 1.000000000000000000 ),
 .UNSPECIFIED. ) ;
#46625=EDGE_CURVE ( 'NONE', #42203, #6702, #2496, .T. ) ;
#46629=CARTESIAN_POINT ( 'NONE',  ( 183.1016766898827939, 295.7534076944302228, 1.248025944548516675 ) ) ;
#46630=CARTESIAN_POINT ( 'NONE',  ( 75.87151652897671283, 214.6115022471902591, 10.00000000000009592 ) ) ;
#46633=CARTESIAN_POINT ( 'NONE',  ( -22.42236680055709641, 157.8615022471902591, 0.000000000000000000 ) ) ;
#46634=CARTESIAN_POINT ( 'NONE',  ( 30.81113223654366706, 188.5958772461660544, -9.188101187500095079 ) ) ;
#46637=CARTESIAN_POINT ( 'NONE',  ( 203.2055155232897619, 269.6379347368149411, -5.981236179145930976 ) ) ;
#46638=CARTESIAN_POINT ( 'NONE',  ( 199.2383506163646132, 285.5560492466715345, -17.78808061564097898 ) ) ;
#46641=CARTESIAN_POINT ( 'NONE',  ( 5.290446120544989306, 163.8615022471902023, 5.000000000000051514 ) ) ;
#46642=CARTESIAN_POINT ( 'NONE',  ( 161.9461893331167914, 280.9078031139047198, -10.53061385661272276 ) ) ;
#46646=CARTESIAN_POINT ( 'NONE',  ( 148.0389988358468827, 274.2359278451201590, 7.783622668412842671 ) ) ;
#46648=CARTESIAN_POINT ( 'NONE',  ( 188.0957521190605348, 269.5173058182602404, -14.08221027142250925 ) ) ;
#46655=ORIENTED_EDGE ( 'NONE', *, *, #52909, .F. ) ;
#46657=CARTESIAN_POINT ( 'NONE',  ( -17.42236680055705023, 149.2012482093457777, 0.000000000000000000 ) ) ;
#46660=B_SPLINE_CURVE_WITH_KNOTS ( 'NONE', 3,
 ( #66138, #81878, #26648, #11956 ),
 .UNSPECIFIED., .F., .F.,
 ( 4, 4 ),
 ( 0.02488339598696336433, 0.03413011071240022731 ),
 .UNSPECIFIED. ) ;
#46662=ORIENTED_EDGE ( 'NONE', *, *, #96431, .F. ) ;
#46665=ORIENTED_EDGE ( 'NONE', *, *, #5426, .T. ) ;
#46666=CARTESIAN_POINT ( 'NONE',  ( 151.4384131719918685, 268.3479694989391078, 14.98299707687648841 ) ) ;
#46667=AXIS2_PLACEMENT_3D ( 'NONE', #24523, #25018, #10841 ) ;
#46668=LINE ( 'NONE', #77594, #96636 ) ;
#46671=CARTESIAN_POINT ( 'NONE',  ( 147.6140518775699491, 274.9719575673779559, 8.457032797753797126 ) ) ;
#46672=CARTESIAN_POINT ( 'NONE',  ( 196.8104339078508076, 289.7613243423628546, -16.40335862274955403 ) ) ;
#46675=EDGE_LOOP ( 'NONE', ( #41173, #9457, #1373, #18357 ) ) ;
#46676=CARTESIAN_POINT ( 'NONE',  ( 157.1338510812060747, 258.4831816688264325, 17.88958125218800888 ) ) ;
#46678=CARTESIAN_POINT ( 'NONE',  ( 161.9072444017735677, 267.0357427074497423, 16.52068954757439556 ) ) ;
#46679=ORIENTED_EDGE ( 'NONE', *, *, #23169, .F. ) ;
#46681=CARTESIAN_POINT ( 'NONE',  ( 149.7128599965862463, 271.3367152699035501, 12.33532264622322394 ) ) ;
#46682=CARTESIAN_POINT ( 'NONE',  ( 155.3598242554943454, 267.1614050273207113, -16.86360361314166667 ) ) ;
#46685=CARTESIAN_POINT ( 'NONE',  ( 150.6931560952953646, 269.6387926204777727, 14.65021044537114037 ) ) ;
#46688=B_SPLINE_CURVE_WITH_KNOTS ( 'NONE', 3,
 ( #90438, #6281, #52869, #21976 ),
 .UNSPECIFIED., .F., .F.,
 ( 4, 4 ),
 ( 0.009394083817439216264, 0.01463245930893269410 ),
 .UNSPECIFIED. ) ;
#46689=ORIENTED_EDGE ( 'NONE', *, *, #97722, .T. ) ;
#46690=ORIENTED_EDGE ( 'NONE', *, *, #87389, .T. ) ;
#46692=CARTESIAN_POINT ( 'NONE',  ( 193.8652130780152731, 280.5836658925297229, -17.72338988841175933 ) ) ;
#46694=CARTESIAN_POINT ( 'NONE',  ( 147.9710862514405960, 274.3535558917855042, 7.785500222159708272 ) ) ;
#46695=ORIENTED_EDGE ( 'NONE', *, *, #334, .F. ) ;
#46696=CARTESIAN_POINT ( 'NONE',  ( 149.5593209768671841, 271.6026526530012575, 11.55487339793564949 ) ) ;
#46697=CARTESIAN_POINT ( 'NONE',  ( 161.8668411317136986, 250.2854024296290447, -13.43522912998426655 ) ) ;
#46698=CARTESIAN_POINT ( 'NONE',  ( 192.6170194583582429, 297.0245312260774995, -11.90166228306590490 ) ) ;
#46699=CARTESIAN_POINT ( 'NONE',  ( 163.9688125216115679, 256.9763212860731301, 15.96522343182667569 ) ) ;
#46706=CARTESIAN_POINT ( 'NONE',  ( 112.9752924205922824, 236.0333772461660544, 9.188101187500095079 ) ) ;
#46708=CARTESIAN_POINT ( 'NONE',  ( 149.0029452494615327, 272.5663236809658088, -12.62683636271733079 ) ) ;
#46711=CARTESIAN_POINT ( 'NONE',  ( 154.8579861482817535, 262.4250953638155011, -17.69813260923097786 ) ) ;
#46712=CARTESIAN_POINT ( 'NONE',  ( 180.1020640141543652, 283.3390819473285092, -16.04965679842496229 ) ) ;
#46714=CARTESIAN_POINT ( 'NONE',  ( 168.6545886844981794, 284.7638151564323721, -7.963406596605243415 ) ) ;
#46719=CARTESIAN_POINT ( 'NONE',  ( 130.0524911732904343, 236.7048013555409796, 4.594050593750051981 ) ) ;
#46720=EDGE_CURVE ( 'NONE', #94946, #19691, #69477, .T. ) ;
#46721=CARTESIAN_POINT ( 'NONE',  ( 192.9518127100452034, 296.0217619941561793, -12.12386602825073645 ) ) ;
#46722=CARTESIAN_POINT ( 'NONE',  ( 185.2824853868734181, 297.7695098558858149, 4.231266468330407093 ) ) ;
#46723=CARTESIAN_POINT ( 'NONE',  ( 195.8947060313465443, 291.3474115503753410, 16.07878593000791767 ) ) ;
#46725=CARTESIAN_POINT ( 'NONE',  ( 47.34706511187656020, 188.9548013555409796, -4.594050593750042211 ) ) ;
#46730=ADVANCED_FACE ( 'NONE', ( #73240 ), #67110, .T. ) ;
#46734=CARTESIAN_POINT ( 'NONE',  ( 151.2656506589457592, 278.4592319541795291, -1.679994777838232922 ) ) ;
#46735=FACE_OUTER_BOUND ( 'NONE', #11988, .T. ) ;
#46736=CARTESIAN_POINT ( 'NONE',  ( 178.3983311753540306, 261.1767784504364727, 12.27131754663537500 ) ) ;
#46737=CARTESIAN_POINT ( 'NONE',  ( 109.4119587261635758, 240.6427522451419065, -10.00000000000009415 ) ) ;
#46742=B_SPLINE_CURVE_WITH_KNOTS ( 'NONE', 3,
 ( #26927, #57806, #48221, #40607 ),
 .UNSPECIFIED., .F., .F.,
 ( 4, 4 ),
 ( 0.02452775330616315669, 0.03377330297669509096 ),
 .UNSPECIFIED. ) ;
#46743=CARTESIAN_POINT ( 'NONE',  ( 162.6937333994314656, 248.8531830095558632, 10.02305144031113926 ) ) ;
#46745=B_SPLINE_CURVE_WITH_KNOTS ( 'NONE', 3,
 ( #41799, #64108, #48414, #95574 ),
 .UNSPECIFIED., .F., .F.,
 ( 4, 4 ),
 ( 0.03913036675905790657, 0.04762113371402499490 ),
 .UNSPECIFIED. ) ;
#46747=CARTESIAN_POINT ( 'NONE',  ( 17.19803509898326510, 189.9244531367911293, -4.594050593750046652 ) ) ;
#46750=LINE ( 'NONE', #16351, #50082 ) ;
#46753=CARTESIAN_POINT ( 'NONE',  ( 194.7888003072046104, 275.1355240377584437, -15.74026182316778666 ) ) ;
#46754=CARTESIAN_POINT ( 'NONE',  ( 66.20992061623260838, 209.0333772461660544, 9.188101187500095079 ) ) ;
#46755=CARTESIAN_POINT ( 'NONE',  ( 200.5810378487751393, 283.2304467414622877, 18.38516374632547112 ) ) ;
#46761=EDGE_CURVE ( 'NONE', #55485, #74117, #7255, .T. ) ;
#46762=CARTESIAN_POINT ( 'NONE',  ( 35.67350403664903524, 184.7365022471902023, -10.00000000000009059 ) ) ;
#46763=CARTESIAN_POINT ( 'NONE',  ( 164.4915767550571957, 245.7392269735623529, -6.407198159945809657 ) ) ;
#46764=CARTESIAN_POINT ( 'NONE',  ( -13.35616335646270691, 163.0958772461660544, -9.188101187500095079 ) ) ;
#46766=CARTESIAN_POINT ( 'NONE',  ( 164.2882805638152774, 260.0608980275483759, -16.19707932525749072 ) ) ;
#46767=CARTESIAN_POINT ( 'NONE',  ( 188.4741096679671841, 261.7728559205870624, 6.464328172697664243 ) ) ;
#46768=EDGE_CURVE ( 'NONE', #38420, #24993, #86404, .T. ) ;
#46769=CARTESIAN_POINT ( 'NONE',  ( 206.1932826529868805, 273.5097535960530877, 11.72208607728249241 ) ) ;
#46775=CARTESIAN_POINT ( 'NONE',  ( 164.0776496603550925, 246.4561697322156419, 8.566708626497000267 ) ) ;
#46776=CARTESIAN_POINT ( 'NONE',  ( 179.0267790344579453, 285.7867660831970511, 13.04357193698000295 ) ) ;
#46777=CARTESIAN_POINT ( 'NONE',  ( 196.2629180738001082, 288.9574505909730533, 17.19408331658577183 ) ) ;
#46780=VERTEX_POINT ( 'NONE', #15899 ) ;
#46781=CARTESIAN_POINT ( 'NONE',  ( 206.8783240872470230, 272.3232270266246928, 9.546753091190767648 ) ) ;
#46784=CARTESIAN_POINT ( 'NONE',  ( 205.1793861064249711, 275.2658739283173759, -14.08953480709093675 ) ) ;
#46785=EDGE_CURVE ( 'NONE', #56036, #7074, #73094, .T. ) ;
#46786=CARTESIAN_POINT ( 'NONE',  ( 192.1859061758433143, 297.7712413352111298, 11.15082371775444336 ) ) ;
#46787=CARTESIAN_POINT ( 'NONE',  ( 207.6727254509676186, 270.9472835030587703, 7.315149605389819953 ) ) ;
#46788=CARTESIAN_POINT ( 'NONE',  ( 188.0035612729766115, 279.2325960380115362, 17.82077010991123700 ) ) ;
#46789=CARTESIAN_POINT ( 'NONE',  ( 207.6837091943624785, 270.9282591014416539, -1.156610046911421552 ) ) ;
#46790=CARTESIAN_POINT ( 'NONE',  ( 200.6985908945154335, 283.0268388936558495, -17.74173253065502820 ) ) ;
#46794=CARTESIAN_POINT ( 'NONE',  ( 190.4775783470208523, 281.5643400410450568, 17.30152405614960287 ) ) ;
#46800=CARTESIAN_POINT ( 'NONE',  ( 193.2752197284765998, 263.9480352582601768, 7.898392093415175452 ) ) ;
#46802=FACE_OUTER_BOUND ( 'NONE', #28866, .T. ) ;
#46804=CARTESIAN_POINT ( 'NONE',  ( 155.7347251133665225, 260.9065389313133778, 17.38482804120033975 ) ) ;
#46805=CARTESIAN_POINT ( 'NONE',  ( 151.3560786774222322, 268.4905770267490652, 15.54402364351346932 ) ) ;
#46806=CARTESIAN_POINT ( 'NONE',  ( 173.4606779374792325, 267.5814416807811540, -17.58000433512257032 ) ) ;
#46811=ORIENTED_EDGE ( 'NONE', *, *, #8906, .F. ) ;
#46813=EDGE_LOOP ( 'NONE', ( #77713, #13809, #18026, #57481 ) ) ;
#46814=CARTESIAN_POINT ( 'NONE',  ( 207.5408646414791178, 271.1756731246201753, 3.050859480894625886 ) ) ;
#46816=CARTESIAN_POINT ( 'NONE',  ( 165.1439403752926864, 271.0709351213488389, 16.99278240859458933 ) ) ;
#46817=CARTESIAN_POINT ( 'NONE',  ( 168.5857730741145986, 281.5268171081109472, 11.65604101945246995 ) ) ;
#46819=CARTESIAN_POINT ( 'NONE',  ( 147.6508870500795467, 274.9081571770856272, -8.950912509993816712 ) ) ;
#46821=CARTESIAN_POINT ( 'NONE',  ( 174.7916223044742026, 289.9785585703071433, 6.260260462112181123 ) ) ;
#46822=DIRECTION ( 'NONE',  ( -0.8660254037844387076, -0.4999999999999998890, -0.000000000000000000 ) ) ;
#46825=CARTESIAN_POINT ( 'NONE',  ( 198.5400493072713459, 276.9865022881721188, -15.28351296223202382 ) ) ;
#46830=CARTESIAN_POINT ( 'NONE',  ( 146.9087229868707425, 276.1936230421149503, -4.111764399247472390 ) ) ;
#46831=CARTESIAN_POINT ( 'NONE',  ( 178.0495033679298160, 294.1167481546831368, 1.468944331028391614 ) ) ;
#46832=CARTESIAN_POINT ( 'NONE',  ( 159.5895502557670795, 254.2297859303815244, -16.92708575547316485 ) ) ;
#46835=CARTESIAN_POINT ( 'NONE',  ( 171.9867212485171990, 254.6089363721731900, 11.25268575585596409 ) ) ;
#46836=CARTESIAN_POINT ( 'NONE',  ( 161.2739978509602565, 283.4540655898655928, 2.136591234652173377 ) ) ;
#46838=CARTESIAN_POINT ( 'NONE',  ( 194.1350435649782185, 294.3952363462973949, -14.11333646480683512 ) ) ;
#46841=CARTESIAN_POINT ( 'NONE',  ( 4.695053651895191749, 183.5177522451419350, 5.000000000000046185 ) ) ;
#46842=CARTESIAN_POINT ( 'NONE',  ( 88.91628449352961638, 212.9548013555409796, -4.594050593750042211 ) ) ;
#46846=CARTESIAN_POINT ( 'NONE',  ( 166.9710079792242539, 278.1405409321207003, -13.47372957072173172 ) ) ;
#46848=CARTESIAN_POINT ( 'NONE',  ( 15.06046875309669630, 173.3768266524159856, -9.188101187500091527 ) ) ;
#46851=CARTESIAN_POINT ( 'NONE',  ( 200.3134965941964651, 283.6938417875134064, 18.29802468362849766 ) ) ;
#46854=CARTESIAN_POINT ( 'NONE',  ( 188.1720092016451247, 260.2520035817423150, -6.289840127462773545 ) ) ;
#46859=CARTESIAN_POINT ( 'NONE',  ( 109.4841275098123248, 234.0177522451418781, -10.00000000000009592 ) ) ;
#46861=CARTESIAN_POINT ( 'NONE',  ( 38.93012039702277605, 193.2833772461660544, -9.188101187500095079 ) ) ;
#46862=CARTESIAN_POINT ( 'NONE',  ( 120.7963240266967375, 249.7369531367911293, -4.594050593750048428 ) ) ;
#46863=CARTESIAN_POINT ( 'NONE',  ( 195.9325654604906788, 275.2851410020765570, 15.59701231568197066 ) ) ;
#46864=EDGE_LOOP ( 'NONE', ( #82631, #92727, #38485, #42943 ) ) ;
#46865=DIRECTION ( 'NONE',  ( 0.4999999999999998890, -0.8660254037844385966, 0.000000000000000000 ) ) ;
#46866=CARTESIAN_POINT ( 'NONE',  ( 181.4204268205617154, 259.5203828285251006, -11.17471347674236348 ) ) ;
#46867=CARTESIAN_POINT ( 'NONE',  ( 152.7730629122270898, 271.2363297891400293, 14.33490734661111610 ) ) ;
#46869=CARTESIAN_POINT ( 'NONE',  ( 193.9204722154232741, 294.7668848255750049, 15.43855698596013859 ) ) ;
#46870=CARTESIAN_POINT ( 'NONE',  ( 175.0286707332103902, 254.6843269425917526, -9.831770975638562504 ) ) ;
#46871=CARTESIAN_POINT ( 'NONE',  ( 194.3177355571849318, 294.0788045336591381, -15.93712594727561616 ) ) ;
#46872=CARTESIAN_POINT ( 'NONE',  ( 148.3629184514745987, 273.6748826132846375, -8.219814532462343948 ) ) ;
#46873=CARTESIAN_POINT ( 'NONE',  ( 191.2696313288225838, 264.4260228325948674, 7.786588993488871679 ) ) ;
#46874=CARTESIAN_POINT ( 'NONE',  ( 171.3086152948395693, 279.7961921927451954, 13.89506224002436419 ) ) ;
#46875=CARTESIAN_POINT ( 'NONE',  ( 186.9764723332892231, 298.1440520839146870, 5.986317207956076913 ) ) ;
#46877=CARTESIAN_POINT ( 'NONE',  ( 148.3837145175834280, 273.6388627701866767, 8.841971351370922605 ) ) ;
#46878=CARTESIAN_POINT ( 'NONE',  ( 181.1787732913807076, 266.0605537588476750, -14.95906821892703320 ) ) ;
#46881=EDGE_CURVE ( 'NONE', #13304, #61069, #96090, .T. ) ;
#46882=CARTESIAN_POINT ( 'NONE',  ( 160.6734846709049691, 282.6943762970620924, -6.583290857611773461 ) ) ;
#46883=CARTESIAN_POINT ( 'NONE',  ( 107.0210206738092609, 244.8464784336661353, 1.353441290958777327E-15 ) ) ;
#46885=CARTESIAN_POINT ( 'NONE',  ( 151.4281781455628675, 268.3656970847310390, 15.24742929158552585 ) ) ;
#46890=CARTESIAN_POINT ( 'NONE',  ( 150.5770346625965601, 269.8399208417597492, -15.30223397899647964 ) ) ;
#46891=CARTESIAN_POINT ( 'NONE',  ( 150.7850480413316632, 269.4796311011364764, -14.43114374163211089 ) ) ;
#46892=CARTESIAN_POINT ( 'NONE',  ( 149.3253462891332219, 272.0079086998416074, -12.99539319630191336 ) ) ;
#46897=CARTESIAN_POINT ( 'NONE',  ( 163.3822952242776125, 256.1223835475196324, -14.91910106040644024 ) ) ;
#46898=CARTESIAN_POINT ( 'NONE',  ( 159.3056354669941470, 256.7215407695565546, 17.03060606420897471 ) ) ;
#46903=CARTESIAN_POINT ( 'NONE',  ( 179.9551071249317715, 262.8846855073763891, -12.83320019091600983 ) ) ;
#46906=CARTESIAN_POINT ( 'NONE',  ( 146.0195742355162452, 255.1115022471902591, 10.00000000000009592 ) ) ;
#46909=B_SPLINE_SURFACE_WITH_KNOTS ( 'NONE', 3, 1, ( 
 ( #30957, #61847 ),
 ( #91629, #22196 ),
 ( #60669, #37383 ),
 ( #85026, #54071 ),
 ( #52093, #90657 ),
 ( #67293, #69290 ),
 ( #61183, #98220 ),
 ( #92630, #67803 ),
 ( #75415, #15080 ),
 ( #13611, #46474 ),
 ( #44985, #99211 ),
 ( #59687, #5999 ),
 ( #44484, #28802 ),
 ( #15572, #98729 ),
 ( #21214, #83039 ),
 ( #22704, #29309 ),
 ( #83540, #84047 ),
 ( #14103, #77405 ),
 ( #14604, #45482 ),
 ( #76417, #6989 ),
 ( #36892, #37874 ),
 ( #91138, #45969 ),
 ( #75928, #60173 ),
 ( #68289, #36388 ),
 ( #21700, #30296 ),
 ( #6507, #52585 ),
 ( #53091, #29797 ),
 ( #68785, #99708 ),
 ( #92152, #53581 ),
 ( #84535, #76886 ),
 ( #7484, #23179 ),
 ( #38376, #100215 ),
 ( #30800, #61680 ),
 ( #39860, #16589 ) ),
 .UNSPECIFIED., .T., .F., .F.,
 ( 4, 2, 2, 2, 2, 2, 2, 2, 2, 2, 2, 2, 2, 2, 2, 2, 4 ),
 ( 2, 2 ),
 ( 0.000000000000000000, 0.06250000000000000000, 0.1250000000000000000, 0.1875000000000000000, 0.2500000000000000000, 0.3125000000000000000, 0.3750000000000000000, 0.4375000000000000000, 0.5000000000000000000, 0.5625000000000000000, 0.6250000000000000000, 0.6875000000000000000, 0.7500000000000000000, 0.8125000000000000000, 0.8750000000000000000, 0.9375000000000000000, 1.000000000000000000 ),
 ( 0.000000000000000000, 1.000000000000000000 ),
 .UNSPECIFIED. ) ;
#46912=CARTESIAN_POINT ( 'NONE',  ( 166.4874640644562476, 283.5895171948562279, 10.47325102323563861 ) ) ;
#46914=CARTESIAN_POINT ( 'NONE',  ( 157.3094609834150788, 258.1790163958882545, 18.30007615310968916 ) ) ;
#46918=CARTESIAN_POINT ( 'NONE',  ( 192.5903950300756264, 297.0706460885853062, -12.26281696942424482 ) ) ;
#46923=B_SPLINE_CURVE_WITH_KNOTS ( 'NONE', 3,
 ( #28232, #34343, #58134, #97664 ),
 .UNSPECIFIED., .F., .F.,
 ( 4, 4 ),
 ( 0.01035187532749593138, 0.01557239096276301533 ),
 .UNSPECIFIED. ) ;
#46926=( BOUNDED_CURVE ( )  B_SPLINE_CURVE ( 2, ( #51757, #85044, #70304, #59831, #44127, #23199, #15593, #62694, #8518 ),
 .UNSPECIFIED., .F., .T. ) 
 B_SPLINE_CURVE_WITH_KNOTS ( ( 3, 2, 2, 2, 3 ),
 ( 0.1895161290322580627, 0.1908602150537634379, 0.1935483870967741882, 0.1962365591397849385, 0.1975806451612903136 ),
 .UNSPECIFIED. ) 
 CURVE ( )  GEOMETRIC_REPRESENTATION_ITEM ( )  RATIONAL_B_SPLINE_CURVE ( ( 0.9330127018922194093, 0.9330127018922194093, 1.000000000000000000, 0.8660254037844387076, 1.000000000000000000, 0.8660254037844387076, 1.000000000000000000, 0.9330127018922194093, 0.9330127018922194093 ) ) 
 REPRESENTATION_ITEM ( '' )  );
#46927=EDGE_LOOP ( 'NONE', ( #71987, #67093, #100154, #42445, #44902 ) ) ;
#46928=CARTESIAN_POINT ( 'NONE',  ( 195.6440376929661511, 290.9937640891101296, 16.03543930387630922 ) ) ;
#46929=ORIENTED_EDGE ( 'NONE', *, *, #29907, .F. ) ;
#46931=ORIENTED_EDGE ( 'NONE', *, *, #73436, .T. ) ;
#46932=CARTESIAN_POINT ( 'NONE',  ( 169.6661456060803062, 269.2651292227166095, 17.56127676152747341 ) ) ;
#46935=CARTESIAN_POINT ( 'NONE',  ( 189.8111788993726918, 300.3393367352153973, -3.345254087122194075 ) ) ;
#46936=CARTESIAN_POINT ( 'NONE',  ( 164.3104563928357322, 246.0529366432151051, -1.966241142131954334 ) ) ;
#46937=CARTESIAN_POINT ( 'NONE',  ( 190.6614556884314311, 300.4116670330316765, 2.330378985950405824 ) ) ;
#46938=CARTESIAN_POINT ( 'NONE',  ( 148.9228818358559749, 272.7049975811580680, 12.13823097167056275 ) ) ;
#46939=CARTESIAN_POINT ( 'NONE',  ( 193.8987971561367090, 262.1765911843755248, 0.2925312025757377254 ) ) ;
#46940=CARTESIAN_POINT ( 'NONE',  ( 168.1437700021587318, 248.2856729686970993, -4.993057267767092355 ) ) ;
#46941=EDGE_CURVE ( 'NONE', #58155, #42571, #57266, .T. ) ;
#46943=CARTESIAN_POINT ( 'NONE',  ( 183.5690767159531731, 284.2936931788220818, -15.45078497124822725 ) ) ;
#46944=CARTESIAN_POINT ( 'NONE',  ( 120.4447615282330588, 240.3458772461660544, 9.188101187500095079 ) ) ;
#46946=CARTESIAN_POINT ( 'NONE',  ( 185.9689676041826658, 262.3423500751161441, -9.039159276176199853 ) ) ;
#46947=CARTESIAN_POINT ( 'NONE',  ( 161.2880211751412958, 283.7149074318706994, 2.164506641643817009 ) ) ;
#46948=CARTESIAN_POINT ( 'NONE',  ( 180.3605947894885730, 291.0927862716739014, -9.605956182346858441 ) ) ;
#46951=CARTESIAN_POINT ( 'NONE',  ( 200.0930818951990489, 273.8593626791692373, 13.67973991811845558 ) ) ;
#46952=CARTESIAN_POINT ( 'NONE',  ( 180.6189675032831303, 256.1636222267840139, 1.305556376142541275 ) ) ;
#46953=CARTESIAN_POINT ( 'NONE',  ( 174.3074440017029190, 290.4856170877609429, -4.843019479348414258 ) ) ;
#46954=CARTESIAN_POINT ( 'NONE',  ( 146.6932111911164327, 276.5669004219916474, 3.080321240977672126 ) ) ;
#46956=CARTESIAN_POINT ( 'NONE',  ( 200.7134601498536028, 283.0010845879393742, -16.98649239173277792 ) ) ;
#46959=CARTESIAN_POINT ( 'NONE',  ( 174.0357770199878473, 253.2726379897468689, -7.670654613122240839 ) ) ;
#46961=CARTESIAN_POINT ( 'NONE',  ( 200.4981329224417550, 282.9858865130267986, -16.73064699428216784 ) ) ;
#46963=ORIENTED_EDGE ( 'NONE', *, *, #78442, .F. ) ;
#46964=CARTESIAN_POINT ( 'NONE',  ( 191.2010045876914432, 266.9569875230786806, -12.78557827834137761 ) ) ;
#46968=CARTESIAN_POINT ( 'NONE',  ( 149.2511585606875428, 272.1364056148075292, 11.40684181024752242 ) ) ;
#46969=CARTESIAN_POINT ( 'NONE',  ( 204.6797164308104584, 272.9778086334555951, -9.766007597308432153 ) ) ;
#46970=CARTESIAN_POINT ( 'NONE',  ( 164.6595611665577508, 284.1616173530609331, -6.908293781447585324 ) ) ;
#46971=CARTESIAN_POINT ( 'NONE',  ( 151.3919346942391257, 275.1019727134247432, -9.604374707620896956 ) ) ;
#46972=CARTESIAN_POINT ( 'NONE',  ( 200.6737073311291795, 283.0699384897140476, -17.61533935526990291 ) ) ;
#46974=CARTESIAN_POINT ( 'NONE',  ( 205.0608245822267293, 272.3115459547129262, -9.418476286974653888 ) ) ;
#46976=CARTESIAN_POINT ( 'NONE',  ( 163.6234338235976224, 247.9473133546832457, -8.351226439232171117 ) ) ;
#46977=CARTESIAN_POINT ( 'NONE',  ( 129.4230657250939203, 233.9824982072973683, 3.021315404115420679E-15 ) ) ;
#46978=CARTESIAN_POINT ( 'NONE',  ( 191.9824032073976241, 287.6194387751458521, -17.05427143794285882 ) ) ;
#46980=CARTESIAN_POINT ( 'NONE',  ( 188.1364496919973703, 299.4054452434185691, -3.692017684402327138 ) ) ;
#46981=CARTESIAN_POINT ( 'NONE',  ( 192.1149248854976861, 297.8941845364767005, 12.26771790733441314 ) ) ;
#46984=AXIS2_PLACEMENT_3D ( 'NONE', #16210, #514, #22813 ) ;
#46986=CARTESIAN_POINT ( 'NONE',  ( 165.3118168859175796, 246.3185293925050701, -4.432402497422931020 ) ) ;
#46989=CARTESIAN_POINT ( 'NONE',  ( 94.11243691623624841, 215.9548013555409796, -4.594050593750042211 ) ) ;
#46991=CARTESIAN_POINT ( 'NONE',  ( 147.3379027498079381, 275.4502618871274535, -3.695260257281167249 ) ) ;
#46992=CARTESIAN_POINT ( 'NONE',  ( 59.85004655896462111, 195.3615022471901739, 5.000000000000051514 ) ) ;
#46994=CARTESIAN_POINT ( 'NONE',  ( 203.2732885619977026, 278.5673317194472247, -16.64305493556850024 ) ) ;
#46999=CARTESIAN_POINT ( 'NONE',  ( 207.2200715578708810, 271.7313030441461024, 6.059433301868463850 ) ) ;
#47000=CARTESIAN_POINT ( 'NONE',  ( -8.728340106763610606, 175.7677522451419350, -5.000000000000047962 ) ) ;
#47001=CARTESIAN_POINT ( 'NONE',  ( 205.5564942343509927, 274.6127034908020050, -12.67609813140607677 ) ) ;
#47002=CARTESIAN_POINT ( 'NONE',  ( 196.4677418905696129, 290.3548843276421394, 17.08610552292358520 ) ) ;
#47003=CARTESIAN_POINT ( 'NONE',  ( 190.3167824967908643, 299.0086585129598689, -8.112609889089975823 ) ) ;
#47004=CARTESIAN_POINT ( 'NONE',  ( 32.16412338207434374, 195.5024278399160949, 9.188101187500095079 ) ) ;
#47005=CARTESIAN_POINT ( 'NONE',  ( 78.41572647264329987, 206.8923013555409796, 4.594050593750050204 ) ) ;
#47008=CARTESIAN_POINT ( 'NONE',  ( 159.1311797733062861, 257.0237068946943282, -17.13424826516079946 ) ) ;
#47009=CARTESIAN_POINT ( 'NONE',  ( -15.06115086838940442, 172.1115022471903160, -5.000000000000047962 ) ) ;
#47011=FACE_OUTER_BOUND ( 'NONE', #63116, .T. ) ;
#47012=CARTESIAN_POINT ( 'NONE',  ( 196.7097633948733915, 269.7859973795743826, -10.82099196770793803 ) ) ;
#47014=CARTESIAN_POINT ( 'NONE',  ( 128.9696990949621522, 255.2677522451419350, -5.000000000000047962 ) ) ;
#47017=CARTESIAN_POINT ( 'NONE',  ( 53.24634253151052832, 210.7369531367911293, -4.594050593750048428 ) ) ;
#47018=CARTESIAN_POINT ( 'NONE',  ( 158.6964626966795322, 256.6164276897989112, -16.48947266769615538 ) ) ;
#47020=CARTESIAN_POINT ( 'NONE',  ( 198.4706398937704819, 286.8857632237200619, 17.04020736381253798 ) ) ;
#47022=CARTESIAN_POINT ( 'NONE',  ( 152.1494898648788876, 276.2488230399721374, 7.208019174511549387 ) ) ;
#47023=B_SPLINE_CURVE_WITH_KNOTS ( 'NONE', 3,
 ( #47459, #864, #63163, #56042, #54043, #24660, #39835, #86528, #77885, #8965, #55052, #70256, #1381, #87034, #31743, #62647, #48474, #7979, #61656, #23152, #79416, #85001, #69761, #15545, #17058, #9982, #46444, #32261, #47949, #369, #31257, #16064, #62144, #93090, #54537, #96115, #73775, #27177, #10990, #12483, #48976, #11497, #81904, #56562, #34269, #73280, #97113, #49971 ),
 .UNSPECIFIED., .F., .F.,
 ( 4, 2, 2, 2, 2, 2, 2, 2, 2, 2, 2, 2, 2, 2, 2, 2, 2, 2, 2, 2, 2, 2, 2, 4 ),
 ( 0.002066062993612058103, 0.002506753530674276243, 0.002727098799205442126, 0.002947444067736608442, 0.003057616702002205478, 0.003167789336267802947, 0.003277961970533399983, 0.003388134604798997019, 0.003608479873330146422, 0.003828825141861295391, 0.004710206215986056932, 0.005591587290110819342, 0.006472968364235581751, 0.006913658901297997650, 0.007354349438360415284, 0.007464522072626019258, 0.007519608389758753592, 0.007574694706891489659, 0.007684867341156831691, 0.007795039975422173723, 0.008015385243952859520, 0.008235730512483545318, 0.008676421049544958547, 0.009117111586606371776 ),
 .UNSPECIFIED. ) ;
#47024=CARTESIAN_POINT ( 'NONE',  ( 110.8733765985978295, 221.4865022471901455, 1.119607411625061291E-15 ) ) ;
#47026=CARTESIAN_POINT ( 'NONE',  ( 164.3274319858398087, 246.0235340536434592, -1.770631424362269168 ) ) ;
#47029=CARTESIAN_POINT ( 'NONE',  ( 185.0467156058686271, 271.2432507303810780, 16.62608513826324241 ) ) ;
#47031=CARTESIAN_POINT ( 'NONE',  ( 206.1062572280473546, 273.6604860535989587, -9.773577984388410300 ) ) ;
#47032=CARTESIAN_POINT ( 'NONE',  ( 190.1052544924596361, 279.3404689574773556, -17.51920321573983230 ) ) ;
#47035=CARTESIAN_POINT ( 'NONE',  ( 173.4904780533158259, 251.2976502526514935, 0.4376931724216052144 ) ) ;
#47038=CARTESIAN_POINT ( 'NONE',  ( 147.7785919239399846, 274.6869658471848652, -7.924750738206837397 ) ) ;
#47040=EDGE_CURVE ( 'NONE', #42087, #96482, #50296, .T. ) ;
#47041=ORIENTED_EDGE ( 'NONE', *, *, #32298, .F. ) ;
#47046=EDGE_LOOP ( 'NONE', ( #80815, #58408, #39302, #40628 ) ) ;
#47048=CARTESIAN_POINT ( 'NONE',  ( 192.1109889407927369, 285.6170536346646145, 17.50456793668967848 ) ) ;
#47050=CIRCLE ( 'NONE', #22759, 14.82106496071134671 ) ;
#47051=CARTESIAN_POINT ( 'NONE',  ( 172.0728039219370658, 285.9831811572526021, 11.38650458882361427 ) ) ;
#47055=CARTESIAN_POINT ( 'NONE',  ( 154.9455285025717615, 262.2734675583710100, 18.28470720339922551 ) ) ;
#47056=CARTESIAN_POINT ( 'NONE',  ( 186.4817412336421114, 293.3135959024839963, -10.75848554020329928 ) ) ;
#47057=CARTESIAN_POINT ( 'NONE',  ( 204.6235849755581455, 276.2285497258825444, -13.59355699282649432 ) ) ;
#47058=ADVANCED_FACE ( 'NONE', ( #11824 ), #81250, .T. ) ;
#47059=CARTESIAN_POINT ( 'NONE',  ( 136.7095408212358052, 258.9244531367911577, -4.594050593750046652 ) ) ;
#47060=CARTESIAN_POINT ( 'NONE',  ( -17.42236680055705023, 149.2012482093457777, 0.000000000000000000 ) ) ;
#47061=CARTESIAN_POINT ( 'NONE',  ( 182.1519740190898915, 260.1784896748602023, 9.240519323136620500 ) ) ;
#47062=CARTESIAN_POINT ( 'NONE',  ( 94.73480590126506229, 219.3768266524160140, 9.188101187500098632 ) ) ;
#47064=CARTESIAN_POINT ( 'NONE',  ( 190.8001679306945277, 300.1714103817999444, 7.815449226872675403 ) ) ;
#47067=CARTESIAN_POINT ( 'NONE',  ( 195.7264009744229725, 291.6389244601378437, -15.67420937712721241 ) ) ;
#47068=ORIENTED_EDGE ( 'NONE', *, *, #26480, .T. ) ;
#47071=CARTESIAN_POINT ( 'NONE',  ( 146.5502055023624735, 276.8145935406849389, 0.3770461397900869427 ) ) ;
#47073=CARTESIAN_POINT ( 'NONE',  ( 49.65620586503731460, 206.1427522451419350, -10.00000000000009592 ) ) ;
#47074=CARTESIAN_POINT ( 'NONE',  ( 208.0964157306580375, 270.2134304119617809, 3.093366075300640894 ) ) ;
#47075=CARTESIAN_POINT ( 'NONE',  ( 72.86731735994297310, 219.0024278399160664, -9.188101187500093303 ) ) ;
#47078=CARTESIAN_POINT ( 'NONE',  ( 201.0418987006243015, 282.4322123308404571, -17.97701256704421624 ) ) ;
#47081=CARTESIAN_POINT ( 'NONE',  ( 184.1252449710846690, 275.2156845598054247, 16.36999343884330571 ) ) ;
#47083=CARTESIAN_POINT ( 'NONE',  ( 207.4148176945302851, 271.0058409609101204, -1.674630231550592763 ) ) ;
#47086=CARTESIAN_POINT ( 'NONE',  ( 189.1055522710370838, 294.9567770444353982, 11.45155291829760635 ) ) ;
#47087=CARTESIAN_POINT ( 'NONE',  ( 185.2880202283114386, 260.2658527302596667, 6.255690438817225640 ) ) ;
#47088=CARTESIAN_POINT ( 'NONE',  ( 155.8843544236747221, 262.1387722156669611, -16.98283378502294738 ) ) ;
#47089=CARTESIAN_POINT ( 'NONE',  ( 200.9061540366740246, 282.6673289856585143, -18.13083321883407351 ) ) ;
#47093=CARTESIAN_POINT ( 'NONE',  ( 195.7593054227485823, 265.4221328166344165, 4.448014571397773231 ) ) ;
#47094=CARTESIAN_POINT ( 'NONE',  ( 148.3402371503543122, 276.4804746445443016, -3.894670276620923133 ) ) ;
#47096=CARTESIAN_POINT ( 'NONE',  ( 171.5709521921977228, 251.6229358086910395, 7.178360255118172439 ) ) ;
#47097=CARTESIAN_POINT ( 'NONE',  ( 198.7195985473925646, 265.8573709945092105, 1.571795761342086761 ) ) ;
#47098=CARTESIAN_POINT ( 'NONE',  ( 154.0195336324254640, 270.6124772311886773, 14.00887731801343783 ) ) ;
#47101=CYLINDRICAL_SURFACE ( 'NONE', #25503, 17.82106496071139645 ) ;
#47102=CARTESIAN_POINT ( 'NONE',  ( 162.9148248802443106, 248.4702413316674381, 9.709394404200100581 ) ) ;
#47104=CARTESIAN_POINT ( 'NONE',  ( 194.1153812227096864, 294.4292925221022870, 15.54001482840963710 ) ) ;
#47108=CARTESIAN_POINT ( 'NONE',  ( 168.4528758249346936, 273.4544194249853035, 16.10234030937003169 ) ) ;
#47109=CARTESIAN_POINT ( 'NONE',  ( 163.4695553787563256, 283.8388210698513490, -3.127313904983202608 ) ) ;
#47110=CARTESIAN_POINT ( 'NONE',  ( 133.0291931787496935, 237.6115022471901739, -5.000000000000041744 ) ) ;
#47111=CARTESIAN_POINT ( 'NONE',  ( 188.3505816287238872, 260.6072362739506616, 3.597359921573489494 ) ) ;
#47113=CARTESIAN_POINT ( 'NONE',  ( 161.2488013048736377, 251.3558788108169040, -13.10044423494716170 ) ) ;
#47114=CARTESIAN_POINT ( 'NONE',  ( 9.810363290536042058, 164.2202760586659736, -5.415160957724236172E-17 ) ) ;
#47115=CARTESIAN_POINT ( 'NONE',  ( 151.9175917390909376, 272.5014707736564219, -13.07602542188641159 ) ) ;
#47117=CARTESIAN_POINT ( 'NONE',  ( 160.5864543089798246, 253.1986605448440173, -14.65770029701640631 ) ) ;
#47119=CARTESIAN_POINT ( 'NONE',  ( 151.1126408083691501, 268.9122237844355254, -15.82705194100464396 ) ) ;
#47120=CARTESIAN_POINT ( 'NONE',  ( 26.56245542105003210, 176.9548013555409796, -4.594050593750042211 ) ) ;
#47121=CARTESIAN_POINT ( 'NONE',  ( 181.6638189564591528, 276.3585937635120331, -17.48262025715165890 ) ) ;
#47123=CARTESIAN_POINT ( 'NONE',  ( 165.0528804069804494, 264.4852527057752241, -17.76608744198970768 ) ) ;
#47124=CARTESIAN_POINT ( 'NONE',  ( 173.6403832423602864, 272.8088530217519860, -16.35538478938354956 ) ) ;
#47126=CARTESIAN_POINT ( 'NONE',  ( 190.0778721158842473, 298.5574750956744765, -8.040639183429819425 ) ) ;
#47127=CARTESIAN_POINT ( 'NONE',  ( 190.7186658257535044, 261.9562542827834477, -0.7910153147876757274 ) ) ;
#47128=CARTESIAN_POINT ( 'NONE',  ( 192.9932412455602559, 295.9775479609656372, -12.16274212864271753 ) ) ;
#47129=CARTESIAN_POINT ( 'NONE',  ( 66.85041857288881317, 202.7365022471902023, -10.00000000000009059 ) ) ;
#47131=CARTESIAN_POINT ( 'NONE',  ( 203.6409074000794703, 269.6153886175684420, 7.070074589036742907 ) ) ;
#47132=CARTESIAN_POINT ( 'NONE',  ( 30.97333845187074886, 194.8149278399160949, -9.188101187500095079 ) ) ;
#47134=CARTESIAN_POINT ( 'NONE',  ( 133.5343746642906240, 241.2365022471902307, 10.00000000000009948 ) ) ;
#47135=CARTESIAN_POINT ( 'NONE',  ( 203.5276888907893635, 269.0805626209144634, -6.031028571504151614 ) ) ;
#47136=CARTESIAN_POINT ( 'NONE',  ( 198.7357616895271804, 286.4265588032756114, -17.04018524297827497 ) ) ;
#47138=CARTESIAN_POINT ( 'NONE',  ( 194.2321518193436987, 294.2270399159019121, 13.98132384850917020 ) ) ;
#47139=CARTESIAN_POINT ( 'NONE',  ( 159.8837875743465986, 278.5245631928274292, -9.817169623836209169 ) ) ;
#47142=CARTESIAN_POINT ( 'NONE',  ( 202.7865629936218284, 279.4103651332174536, 17.10878160033216133 ) ) ;
#47143=CARTESIAN_POINT ( 'NONE',  ( 181.8774662184618194, 285.1120569720015965, 15.89814067624403116 ) ) ;
#47145=CARTESIAN_POINT ( 'NONE',  ( 174.8146681715918476, 256.6396774605312316, 12.00018018173206613 ) ) ;
#47146=ORIENTED_EDGE ( 'NONE', *, *, #75864, .T. ) ;
#47155=CARTESIAN_POINT ( 'NONE',  ( 155.4810912439522212, 261.3458456796594760, -18.44218279064527266 ) ) ;
#47159=FACE_OUTER_BOUND ( 'NONE', #45717, .T. ) ;
#47161=VERTEX_POINT ( 'NONE', #52771 ) ;
#47162=CARTESIAN_POINT ( 'NONE',  ( 153.3506059258413643, 265.0359544954067132, -16.39100908615009899 ) ) ;
#47166=EDGE_CURVE ( 'NONE', #42571, #32950, #21062, .T. ) ;
#47167=CARTESIAN_POINT ( 'NONE',  ( 190.1158090214649405, 301.3567547831981983, -1.340987185199551845 ) ) ;
#47168=B_SPLINE_CURVE_WITH_KNOTS ( 'NONE', 3,
 ( #54707, #24330, #55206, #86187 ),
 .UNSPECIFIED., .F., .F.,
 ( 4, 4 ),
 ( 0.01606534115735265555, 0.02489855931191051891 ),
 .UNSPECIFIED. ) ;
#47169=CARTESIAN_POINT ( 'NONE',  ( 196.4808189786114951, 290.3322341467384717, -17.84817245450773271 ) ) ;
#47170=CARTESIAN_POINT ( 'NONE',  ( 180.5405277538137625, 287.0200771715591372, -13.55746091599727521 ) ) ;
#47172=CARTESIAN_POINT ( 'NONE',  ( 195.6986305151803549, 291.6870243064952888, 16.84182339398051909 ) ) ;
#47173=CARTESIAN_POINT ( 'NONE',  ( 176.3152674796077974, 277.8542160414133946, -17.23542792216073138 ) ) ;
#47176=CARTESIAN_POINT ( 'NONE',  ( 198.0792648159935538, 287.5636447432459022, 17.04758482866669667 ) ) ;
#47177=CARTESIAN_POINT ( 'NONE',  ( 173.8805019302338621, 250.6242863632701585, 0.4030408839048176262 ) ) ;
#47178=CARTESIAN_POINT ( 'NONE',  ( 60.22919299317007358, 196.3923013555409796, 4.594050593750050204 ) ) ;
#47180=B_SPLINE_CURVE_WITH_KNOTS ( 'NONE', 3,
 ( #51639, #76445, #99743, #52120 ),
 .UNSPECIFIED., .F., .F.,
 ( 4, 4 ),
 ( 0.01234167213556876079, 0.01858179642034042678 ),
 .UNSPECIFIED. ) ;
#47182=CARTESIAN_POINT ( 'NONE',  ( 160.6673679105988697, 254.1955030722899380, 15.77102516331386362 ) ) ;
#47183=CYLINDRICAL_SURFACE ( 'NONE', #30497, 17.82106496071139645 ) ;
#47184=CARTESIAN_POINT ( 'NONE',  ( 175.1271263694729328, 272.4273639404348728, 17.81557788710851042 ) ) ;
#47185=ORIENTED_EDGE ( 'NONE', *, *, #50620, .T. ) ;
#47189=CARTESIAN_POINT ( 'NONE',  ( 69.21394623383588396, 220.7677522451419065, -5.000000000000047962 ) ) ;
#47190=CARTESIAN_POINT ( 'NONE',  ( 148.3280470635002928, 273.7352816289870248, 9.058704604771318003 ) ) ;
#47191=VERTEX_POINT ( 'NONE', #14294 ) ;
#47194=CARTESIAN_POINT ( 'NONE',  ( 207.8718670335145475, 270.6023601641878713, -6.322166851501095586 ) ) ;
#47195=CARTESIAN_POINT ( 'NONE',  ( 146.9978162861947908, 276.0393089210717790, -5.134868500856280882 ) ) ;
#47196=CARTESIAN_POINT ( 'NONE',  ( 163.3751545559699707, 257.8073145213600128, 15.56062503124628726 ) ) ;
#47197=CARTESIAN_POINT ( 'NONE',  ( 155.5207183646172950, 261.6826666266933898, -16.99780945766855922 ) ) ;
#47198=CARTESIAN_POINT ( 'NONE',  ( 164.7297297678022403, 245.3267338555121455, 3.020078936458732599 ) ) ;
#47202=CARTESIAN_POINT ( 'NONE',  ( 109.5926410088830920, 224.8923013555410080, 4.594050593750050204 ) ) ;
#47203=ORIENTED_EDGE ( 'NONE', *, *, #11288, .T. ) ;
#47204=CARTESIAN_POINT ( 'NONE',  ( 147.0660117096331874, 275.9211909828330249, -0.7354350123930680772 ) ) ;
#47209=CARTESIAN_POINT ( 'NONE',  ( 155.6066474290145720, 261.1283759879266881, -18.16552045242181279 ) ) ;
#47210=CARTESIAN_POINT ( 'NONE',  ( 183.0265560501797495, 285.2188940410537725, -14.98214014822414164 ) ) ;
#47212=CARTESIAN_POINT ( 'NONE',  ( 165.6338766894626531, 283.5762763500268306, -8.233634190165624034 ) ) ;
#47214=CARTESIAN_POINT ( 'NONE',  ( 163.3020905273760093, 247.7994775548095845, -11.05431316445765155 ) ) ;
#47217=CARTESIAN_POINT ( 'NONE',  ( 165.0807124393095364, 244.7188140358855151, -1.586079993046279446 ) ) ;
#47218=CARTESIAN_POINT ( 'NONE',  ( 123.3944002380500677, 251.2369531367911293, -4.594050593750048428 ) ) ;
#47219=CARTESIAN_POINT ( 'NONE',  ( 150.9363692955544991, 269.2175350005573478, -14.27857383982596140 ) ) ;
#47221=CARTESIAN_POINT ( 'NONE',  ( 188.9842081906053295, 299.1938366728135748, 4.832788090775505196 ) ) ;
#47222=CARTESIAN_POINT ( 'NONE',  ( 187.5788460363194758, 281.4634433164364964, -17.49678885218273550 ) ) ;
#47224=CARTESIAN_POINT ( 'NONE',  ( 49.53858449761714411, 211.6589784336661637, -6.496448406907675876E-16 ) ) ;
#47227=ORIENTED_EDGE ( 'NONE', *, *, #81869, .T. ) ;
#47234=CARTESIAN_POINT ( 'NONE',  ( 175.0574341850002895, 261.2992596373129572, 14.66236234505684877 ) ) ;
#47235=CARTESIAN_POINT ( 'NONE',  ( 152.6547697591180111, 278.7515079535921814, -4.825746761778547445 ) ) ;
#47236=CARTESIAN_POINT ( 'NONE',  ( 202.7754741559590173, 279.4295715634463022, -15.65855077192107636 ) ) ;
#47237=CARTESIAN_POINT ( 'NONE',  ( 178.3679663846656354, 261.2045661951830198, 12.31888526918040583 ) ) ;
#47238=CARTESIAN_POINT ( 'NONE',  ( 119.8042635715768540, 246.6427522451419065, -10.00000000000009415 ) ) ;
#47240=EDGE_LOOP ( 'NONE', ( #78568, #2222, #59181 ) ) ;
#47241=CARTESIAN_POINT ( 'NONE',  ( 202.6551236945213361, 279.6380246773706517, 15.55476940527561425 ) ) ;
#47243=CARTESIAN_POINT ( 'NONE',  ( 30.59497298136257726, 176.2202760586660020, -5.415160957724236172E-17 ) ) ;
#47245=CARTESIAN_POINT ( 'NONE',  ( 192.3713340522295709, 271.8780416168410170, 15.57788208939756380 ) ) ;
#47248=CARTESIAN_POINT ( 'NONE',  ( 191.2126589609105736, 267.4645585149979752, 13.28012995173027733 ) ) ;
#47249=CARTESIAN_POINT ( 'NONE',  ( 64.74867629522887569, 202.0643266524159856, -9.188101187500093303 ) ) ;
#47251=CARTESIAN_POINT ( 'NONE',  ( 163.1976272564393184, 256.1029571228265809, -14.97062603987144058 ) ) ;
#47255=CARTESIAN_POINT ( 'NONE',  ( 27.87927540258908365, 180.2365022471902023, -10.00000000000009059 ) ) ;
#47257=CARTESIAN_POINT ( 'NONE',  ( 162.6476498368881494, 248.9330020812748785, 10.75824100428386743 ) ) ;
#47258=CARTESIAN_POINT ( 'NONE',  ( -9.459049039432731121, 165.3458772461660544, 9.188101187500095079 ) ) ;
#47260=CARTESIAN_POINT ( 'NONE',  ( 167.2771105491443677, 262.3221479689785269, -16.42317405296926935 ) ) ;
#47261=CARTESIAN_POINT ( 'NONE',  ( 170.4370497408796723, 263.6275113357616533, 15.80834233833078351 ) ) ;
#47262=CARTESIAN_POINT ( 'NONE',  ( 189.2125443449212696, 261.8290248071659221, 6.598221272828422634 ) ) ;
#47263=CARTESIAN_POINT ( 'NONE',  ( 164.8616299252405213, 245.0982760813026857, 1.544363874765093625 ) ) ;
#47264=CARTESIAN_POINT ( 'NONE',  ( 187.0048093878013731, 259.3019680120904695, -2.391362674332986771 ) ) ;
#47268=CARTESIAN_POINT ( 'NONE',  ( 181.7502613149374326, 287.7871512160830889, 13.52857313414122054 ) ) ;
#47269=CARTESIAN_POINT ( 'NONE',  ( 196.2865739685663300, 290.0389735281796675, 16.35500968239857755 ) ) ;
#47271=CARTESIAN_POINT ( 'NONE',  ( 206.5215086902351516, 272.9412494231720530, 8.384715559417665887 ) ) ;
#47274=EDGE_CURVE ( 'NONE', #86364, #38315, #9006, .T. ) ;
#47276=CARTESIAN_POINT ( 'NONE',  ( 89.31526421587503251, 210.8262482093457777, 3.021315404115420679E-15 ) ) ;
#47277=CARTESIAN_POINT ( 'NONE',  ( 94.49106271034210636, 235.3615022471903160, 5.000000000000046185 ) ) ;
#47278=CARTESIAN_POINT ( 'NONE',  ( 207.5920568422024814, 271.0870056320159165, -1.586464549033245186 ) ) ;
#47279=CARTESIAN_POINT ( 'NONE',  ( 193.8913555215501390, 294.8173164187117550, 15.40725395879721837 ) ) ;
#47281=CARTESIAN_POINT ( 'NONE',  ( 156.4864942492372677, 277.0302591896826812, -10.06882784799783437 ) ) ;
#47285=CARTESIAN_POINT ( 'NONE',  ( 155.4185480231587064, 262.3956844143579588, -17.21684874643274554 ) ) ;
#47288=CARTESIAN_POINT ( 'NONE',  ( 191.1687199697037443, 299.5330595250031820, -8.491751560014430211 ) ) ;
#47294=CARTESIAN_POINT ( 'NONE',  ( 200.2631011806900005, 283.7811292041749311, 18.23377125296567058 ) ) ;
#47295=CARTESIAN_POINT ( 'NONE',  ( 133.0291931787496651, 247.6115022471902591, 10.00000000000009592 ) ) ;
#47296=CARTESIAN_POINT ( 'NONE',  ( 191.2056514706806070, 299.4690922889112699, 7.290007621276087590 ) ) ;
#47297=CARTESIAN_POINT ( 'NONE',  ( 177.4640749235418866, 269.0261679207779935, -17.44345675124527517 ) ) ;
#47299=EDGE_CURVE ( 'NONE', #69624, #19580, #36820, .T. ) ;
#47305=CARTESIAN_POINT ( 'NONE',  ( 163.8111981134063342, 274.4328725233862087, -16.00973502687279648 ) ) ;
#47309=CARTESIAN_POINT ( 'NONE',  ( 165.1854192917994624, 270.9806551308440703, 16.59870098112833148 ) ) ;
#47310=CARTESIAN_POINT ( 'NONE',  ( 171.0782956557647196, 283.4844436738434865, 12.11060603767918131 ) ) ;
#47311=CARTESIAN_POINT ( 'NONE',  ( 147.6264044922760377, 274.9505622111005323, -8.841872555777701592 ) ) ;
#47313=CARTESIAN_POINT ( 'NONE',  ( 159.0969231069750549, 255.0830411812770535, -17.15863751354124034 ) ) ;
#47319=CARTESIAN_POINT ( 'NONE',  ( 206.9182786203111277, 271.7016349257525576, 5.804932932542666180 ) ) ;
#47320=VERTEX_POINT ( 'NONE', #47669 ) ;
#47323=CARTESIAN_POINT ( 'NONE',  ( 174.9358745049650565, 292.2217799751211942, 2.235529367806339263 ) ) ;
#47324=CARTESIAN_POINT ( 'NONE',  ( 206.1062572280473546, 273.6604860535989587, -9.773577984388410300 ) ) ;
#47325=DIRECTION ( 'NONE',  ( -0.8660254037844387076, -0.4999999999999998890, -0.000000000000000000 ) ) ;
#47327=CARTESIAN_POINT ( 'NONE',  ( 199.3695014196146644, 285.3288893919889802, -18.21719466810020549 ) ) ;
#47330=CARTESIAN_POINT ( 'NONE',  ( 194.4557758866845916, 293.8397116694720808, -14.23894577158402086 ) ) ;
#47333=DIRECTION ( 'NONE',  ( -0.8660254037844387076, -0.4999999999999998890, -0.000000000000000000 ) ) ;
#47334=CARTESIAN_POINT ( 'NONE',  ( 17.25242200676963833, 170.7677522451417929, -5.000000000000041744 ) ) ;
#47335=CARTESIAN_POINT ( 'NONE',  ( 78.11742282250361313, 228.1589784336661353, -6.496448406907676862E-16 ) ) ;
#47337=ADVANCED_FACE ( 'NONE', ( #17798 ), #10920, .F. ) ;
#47339=CARTESIAN_POINT ( 'NONE',  ( 170.0185468137966609, 280.2994163020263727, -13.67235037299359668 ) ) ;
#47340=CARTESIAN_POINT ( 'NONE',  ( 14.19444334931225349, 172.8768266524160140, 9.188101187500098632 ) ) ;
#47342=EDGE_CURVE ( 'NONE', #61372, #45744, #45243, .T. ) ;
#47343=CARTESIAN_POINT ( 'NONE',  ( 200.5810378487751393, 283.2304467414622877, 18.38516374632547112 ) ) ;
#47348=PLANE ( 'NONE',  #85294 ) ;
#47352=CARTESIAN_POINT ( 'NONE',  ( 94.05805000844996755, 215.1115022471902023, -5.000000000000041744 ) ) ;
#47354=CARTESIAN_POINT ( 'NONE',  ( 32.08336737017582152, 180.1423013555409796, -4.594050593750043987 ) ) ;
#47357=CARTESIAN_POINT ( 'NONE',  ( 30.40518283029366842, 188.3615022471902591, -10.00000000000009592 ) ) ;
#47358=CARTESIAN_POINT ( 'NONE',  ( 182.6002590226659663, 260.6490965261490373, -10.86303761599557660 ) ) ;
#47363=CARTESIAN_POINT ( 'NONE',  ( 68.41462912126404206, 198.7592609112380728, 2.679491924311254714 ) ) ;
#47364=CARTESIAN_POINT ( 'NONE',  ( 186.2368818158729198, 283.2115614060767825, 16.35907209874016388 ) ) ;
#47365=CARTESIAN_POINT ( 'NONE',  ( 194.9757425430702824, 292.9391030023704161, -15.21392314336593365 ) ) ;
#47367=CARTESIAN_POINT ( 'NONE',  ( 192.2383246029743873, 265.0112368890651169, 7.772948199626619648 ) ) ;
#47368=CARTESIAN_POINT ( 'NONE',  ( 168.0937730764468370, 278.6755643525841606, 14.89096657633803744 ) ) ;
#47371=CARTESIAN_POINT ( 'NONE',  ( 148.3519871123208986, 273.6938162480936398, 8.180046468253793890 ) ) ;
#47375=CARTESIAN_POINT ( 'NONE',  ( 16.56913029798217352, 168.8262482093458061, 3.021315404115420679E-15 ) ) ;
#47376=CARTESIAN_POINT ( 'NONE',  ( 109.5926410088830920, 224.8923013555410080, 4.594050593750050204 ) ) ;
#47378=B_SPLINE_CURVE_WITH_KNOTS ( 'NONE', 3,
 ( #20607, #43880, #60562, #52981, #83930, #74821, #60069, #45374, #5401, #36285, #30180, #61068, #67184, #82934, #98108, #13509, #5892, #75311, #50981, #21597, #81934, #43382, #84917, #24077, #46358, #61569, #78295, #62056, #70675, #92517, #100105, #15460, #31660, #72581, #31167, #30689, #38260, #64454, #7374, #77803, #7893, #46878, #23065, #85949, #95414, #69173, #70165, #54971 ),
 .UNSPECIFIED., .F., .F.,
 ( 4, 2, 2, 2, 2, 2, 2, 2, 2, 2, 2, 2, 2, 2, 2, 2, 2, 2, 2, 2, 2, 2, 2, 4 ),
 ( 0.0001223504472693309937, 0.001139333269370160261, 0.001647824680420526336, 0.001902070385945734635, 0.002029193238708323823, 0.002156316091470912577, 0.002410561796996093121, 0.002664807502521273665, 0.003173298913571691564, 0.004190281735672526063, 0.005207264557773360995, 0.005715755968823742900, 0.005970001674348896122, 0.006224247379874050211, 0.006287808806255272380, 0.006351370232636494549, 0.006414931659017716718, 0.006478493085398939755, 0.006732738790923782461, 0.006986984496448626035, 0.007241230201973469609, 0.007495475907498313183, 0.007749721613023156756, 0.008258213024072825689 ),
 .UNSPECIFIED. ) ;
#47379=CARTESIAN_POINT ( 'NONE',  ( 150.7530568467738590, 269.5350414755053521, 15.60317050893315916 ) ) ;
#47381=CIRCLE ( 'NONE', #49071, 17.82106496071138224 ) ;
#47382=CARTESIAN_POINT ( 'NONE',  ( 195.9920715006079490, 291.1787696107118677, 15.99608784761372071 ) ) ;
#47383=CARTESIAN_POINT ( 'NONE',  ( 194.5245920682378369, 278.7753957560683489, 16.29798302962802126 ) ) ;
#47384=DIRECTION ( 'NONE',  ( -0.8660254037844387076, -0.4999999999999998890, -0.000000000000000000 ) ) ;
#47385=CARTESIAN_POINT ( 'NONE',  ( 193.1052853069701882, 263.5410494637605439, -5.234861273610968091 ) ) ;
#47390=ORIENTED_EDGE ( 'NONE', *, *, #17228, .T. ) ;
#47391=CARTESIAN_POINT ( 'NONE',  ( 191.1348134016154745, 266.6500986785706573, 10.84710269163073271 ) ) ;
#47392=CARTESIAN_POINT ( 'NONE',  ( 179.0380341696543383, 280.7593727008336373, 16.07746832305279128 ) ) ;
#47393=CARTESIAN_POINT ( 'NONE',  ( 196.6211565541474613, 267.8594331423399808, 9.474020388104994694 ) ) ;
#47395=CARTESIAN_POINT ( 'NONE',  ( 188.8639537394926720, 283.4252602687708986, -17.55272065613104715 ) ) ;
#47396=CARTESIAN_POINT ( 'NONE',  ( 192.4888807200563292, 285.7021917670288644, -17.52758604510307450 ) ) ;
#47397=CARTESIAN_POINT ( 'NONE',  ( 167.9549855348998335, 286.6226398335882095, 7.176453026111839328 ) ) ;
#47399=CARTESIAN_POINT ( 'NONE',  ( 192.1149248854976861, 297.8941845364767005, 12.26771790733441314 ) ) ;
#47401=CARTESIAN_POINT ( 'NONE',  ( 191.2550863981256271, 280.2068698123553645, 17.52853399581771399 ) ) ;
#47405=CARTESIAN_POINT ( 'NONE',  ( -13.51183432020139819, 142.4280072687214442, 0.000000000000000000 ) ) ;
#47406=CARTESIAN_POINT ( 'NONE',  ( 107.6156973702194648, 244.4860189848785126, -2.679491924311252493 ) ) ;
#47407=ORIENTED_EDGE ( 'NONE', *, *, #14912, .T. ) ;
#47408=EDGE_CURVE ( 'NONE', #7177, #84862, #6505, .T. ) ;
#47410=CARTESIAN_POINT ( 'NONE',  ( -22.42236680055709641, 157.8615022471902591, 0.000000000000000000 ) ) ;
#47411=CARTESIAN_POINT ( 'NONE',  ( 163.7239493340838123, 247.0687966679708438, 6.286946239157660266 ) ) ;
#47416=VERTEX_POINT ( 'NONE', #30372 ) ;
#47417=EDGE_CURVE ( 'NONE', #18290, #75148, #53670, .T. ) ;
#47419=CARTESIAN_POINT ( 'NONE',  ( 200.1038300618348273, 276.8705922012964606, -15.82546249815781181 ) ) ;
#47423=ORIENTED_EDGE ( 'NONE', *, *, #41241, .T. ) ;
#47425=CARTESIAN_POINT ( 'NONE',  ( 203.4357368910538355, 278.2859629599173559, -16.45855118664066197 ) ) ;
#47427=CARTESIAN_POINT ( 'NONE',  ( 190.5325656458726087, 300.1042792322296009, -3.574822255195763798 ) ) ;
#47428=CARTESIAN_POINT ( 'NONE',  ( 206.5431607373320730, 272.9037469775124691, -11.15649369879132102 ) ) ;
#47429=CARTESIAN_POINT ( 'NONE',  ( 147.4587540121967209, 275.2409413605112718, -7.408606599236415846 ) ) ;
#47430=CARTESIAN_POINT ( 'NONE',  ( 196.0380285978610289, 284.4171904029984717, -17.66719457817500682 ) ) ;
#47432=CARTESIAN_POINT ( 'NONE',  ( 167.6414094296473820, 249.1822265415601123, -5.393406076269569027 ) ) ;
#47434=CARTESIAN_POINT ( 'NONE',  ( 155.4191430981459519, 279.8345045701359481, 2.111987297901974703 ) ) ;
#47435=CARTESIAN_POINT ( 'NONE',  ( 133.7059490715648167, 241.8768266524159856, 9.188101187500098632 ) ) ;
#47436=CARTESIAN_POINT ( 'NONE',  ( 183.4116579307454913, 260.3025310349262327, -9.357811455373186149 ) ) ;
#47442=CARTESIAN_POINT ( 'NONE',  ( 180.8220585722234830, 256.2043429177185772, 1.036815351425113052 ) ) ;
#47443=CARTESIAN_POINT ( 'NONE',  ( 165.2023837071825483, 246.1063600852122875, -2.838470414776972817 ) ) ;
#47444=CARTESIAN_POINT ( 'NONE',  ( 192.3733747235286557, 297.4465362857985724, 11.01966089874153631 ) ) ;
#47447=CARTESIAN_POINT ( 'NONE',  ( 173.4984831628007953, 287.1903257367396805, -9.639986186396646062 ) ) ;
#47449=CARTESIAN_POINT ( 'NONE',  ( 181.1060688601531297, 255.8911062559022298, -5.777534809724734544 ) ) ;
#47451=CARTESIAN_POINT ( 'NONE',  ( 194.4826705584825390, 293.7931287314651740, -16.11258321617245315 ) ) ;
#47452=EDGE_CURVE ( 'NONE', #7762, #21258, #30724, .T. ) ;
#47453=CARTESIAN_POINT ( 'NONE',  ( 151.3107971817505586, 272.4644232592236790, 11.71674968251862836 ) ) ;
#47456=CARTESIAN_POINT ( 'NONE',  ( 191.7826753266332673, 267.7942839150106238, -12.33540156790041742 ) ) ;
#47459=CARTESIAN_POINT ( 'NONE',  ( 159.3291946290163992, 279.0199804063916531, 10.96233109238993109 ) ) ;
#47460=CARTESIAN_POINT ( 'NONE',  ( 151.8373860759844831, 267.6569281583805946, -16.78611463437632167 ) ) ;
#47461=CARTESIAN_POINT ( 'NONE',  ( 148.9498507103374152, 272.6582861203333437, 11.90061892622094852 ) ) ;
#47462=CARTESIAN_POINT ( 'NONE',  ( 6.860117161356284576, 184.7677522451419065, -5.000000000000047962 ) ) ;
#47463=CARTESIAN_POINT ( 'NONE',  ( 161.6287415102018770, 281.5831586784601654, -6.602482105918118904 ) ) ;
#47464=CARTESIAN_POINT ( 'NONE',  ( 154.9357316289406015, 277.4855806559950224, -8.880802751379739846 ) ) ;
#47465=DIRECTION ( 'NONE',  ( -0.8660254037844387076, -0.4999999999999998890, -0.000000000000000000 ) ) ;
#47467=CARTESIAN_POINT ( 'NONE',  ( 204.6849407614616041, 272.9629571217342914, -9.743767658441230495 ) ) ;
#47468=B_SPLINE_SURFACE_WITH_KNOTS ( 'NONE', 3, 1, ( 
 ( #88754, #4086 ),
 ( #96835, #89257 ),
 ( #27400, #19807 ),
 ( #50674, #81627 ),
 ( #7573, #68865 ),
 ( #15158, #52170 ),
 ( #22784, #38461 ),
 ( #92712, #84135 ),
 ( #22276, #82646 ),
 ( #30878, #46055 ),
 ( #68374, #92233 ),
 ( #13204, #76971 ),
 ( #60259, #61765 ),
 ( #44062, #21296 ),
 ( #98809, #53180 ),
 ( #67377, #45074 ),
 ( #13689, #91215 ),
 ( #44562, #100294 ),
 ( #14684, #45565 ),
 ( #29879, #23262 ),
 ( #21778, #75002 ),
 ( #52667, #61263 ),
 ( #83622, #83119 ),
 ( #76494, #5581 ),
 ( #76013, #69375 ),
 ( #37957, #99791 ),
 ( #7072, #30380 ),
 ( #84617, #36473 ),
 ( #98303, #53661 ),
 ( #59770, #28893 ),
 ( #90738, #14189 ),
 ( #75497, #6082 ),
 ( #36975, #60751 ),
 ( #67887, #29390 ) ),
 .UNSPECIFIED., .T., .F., .F.,
 ( 4, 2, 2, 2, 2, 2, 2, 2, 2, 2, 2, 2, 2, 2, 2, 2, 4 ),
 ( 2, 2 ),
 ( 0.000000000000000000, 0.06250000000000000000, 0.1250000000000000000, 0.1875000000000000000, 0.2500000000000000000, 0.3125000000000000000, 0.3750000000000000000, 0.4375000000000000000, 0.5000000000000000000, 0.5625000000000000000, 0.6250000000000000000, 0.6875000000000000000, 0.7500000000000000000, 0.8125000000000000000, 0.8750000000000000000, 0.9375000000000000000, 1.000000000000000000 ),
 ( 0.000000000000000000, 1.000000000000000000 ),
 .UNSPECIFIED. ) ;
#47471=CARTESIAN_POINT ( 'NONE',  ( 192.5737543603648589, 275.7597456448726234, -15.97875861998497626 ) ) ;
#47472=CARTESIAN_POINT ( 'NONE',  ( 144.7205361298395871, 254.3615022471902307, -10.00000000000009592 ) ) ;
#47473=CARTESIAN_POINT ( 'NONE',  ( 197.2328925967401858, 274.3547493420543333, 15.41857190266785871 ) ) ;
#47474=CARTESIAN_POINT ( 'NONE',  ( 192.5712965840290849, 297.1037255674836501, 11.03742858512898906 ) ) ;
#47478=CARTESIAN_POINT ( 'NONE',  ( -8.349714312657674498, 175.1744531367911293, 4.594050593750047540 ) ) ;
#47479=CARTESIAN_POINT ( 'NONE',  ( 98.19890751640281223, 221.3768266524159856, -9.188101187500091527 ) ) ;
#47480=CARTESIAN_POINT ( 'NONE',  ( 155.5587153255869453, 261.2113968263770971, -18.30500480654006878 ) ) ;
#47481=CARTESIAN_POINT ( 'NONE',  ( 192.6170194583582429, 297.0245312260774995, -11.90166228306590490 ) ) ;
#47483=CARTESIAN_POINT ( 'NONE',  ( 202.7602807045765019, 279.4558873931827065, -15.90558713185497020 ) ) ;
#47489=CARTESIAN_POINT ( 'NONE',  ( 180.5623436295364854, 290.8789022247497087, 9.334073381727758800 ) ) ;
#47490=CARTESIAN_POINT ( 'NONE',  ( 169.2406489442459190, 252.1939778885328849, -9.400937777832105269 ) ) ;
#47491=CARTESIAN_POINT ( 'NONE',  ( 204.7998534689117491, 275.9232437396207729, -13.00948150499847067 ) ) ;
#47492=CARTESIAN_POINT ( 'NONE',  ( 196.0034224882197975, 291.1591091234520263, 17.53794140922627776 ) ) ;
#47495=CARTESIAN_POINT ( 'NONE',  ( 207.4541616930702617, 271.3258470364304458, -6.834942797545373594 ) ) ;
#47496=CARTESIAN_POINT ( 'NONE',  ( 46.18343024948246978, 185.2202760586659736, -5.415160957724236172E-17 ) ) ;
#47497=EDGE_CURVE ( 'NONE', #31208, #32891, #89973, .T. ) ;
#47498=CARTESIAN_POINT ( 'NONE',  ( 67.34675250658217749, 203.5643266524159856, -9.188101187500093303 ) ) ;
#47499=CARTESIAN_POINT ( 'NONE',  ( 61.58209736653347477, 206.3615022471902307, -10.00000000000009592 ) ) ;
#47502=CARTESIAN_POINT ( 'NONE',  ( 166.7607585703058817, 259.6620056817021123, 15.79927695026398382 ) ) ;
#47504=CARTESIAN_POINT ( 'NONE',  ( 196.2630425146829225, 269.4134538897955622, -10.69405362647414925 ) ) ;
#47506=CARTESIAN_POINT ( 'NONE',  ( 150.6815632051821581, 269.6588720951601772, -14.68790257316217307 ) ) ;
#47509=CARTESIAN_POINT ( 'NONE',  ( 74.43750904794978851, 201.5327760586659167, 1.948934522072302763E-15 ) ) ;
#47511=CARTESIAN_POINT ( 'NONE',  ( 155.3716771045260714, 261.5353565282119348, -18.54934131471355840 ) ) ;
#47512=CARTESIAN_POINT ( 'NONE',  ( 198.6562788533279615, 286.5642271139020636, 17.47134757795404525 ) ) ;
#47513=CARTESIAN_POINT ( 'NONE',  ( 48.86234924490155862, 209.0177522451419065, 5.000000000000046185 ) ) ;
#47514=CARTESIAN_POINT ( 'NONE',  ( 198.9730007453206042, 281.0620181772907245, 17.36568714939058822 ) ) ;
#47515=( BOUNDED_CURVE ( )  B_SPLINE_CURVE ( 2, ( #65314, #79051, #9640, #87193, #25309, #19248, #49122, #26817, #87694 ),
 .UNSPECIFIED., .F., .T. ) 
 B_SPLINE_CURVE_WITH_KNOTS ( ( 3, 2, 2, 2, 3 ),
 ( 0.6733870967741935054, 0.6747311827956988806, 0.6774193548387096309, 0.6801075268817203812, 0.6814516129032257563 ),
 .UNSPECIFIED. ) 
 CURVE ( )  GEOMETRIC_REPRESENTATION_ITEM ( )  RATIONAL_B_SPLINE_CURVE ( ( 0.9330127018922194093, 0.9330127018922194093, 1.000000000000000000, 0.8660254037844387076, 1.000000000000000000, 0.8660254037844387076, 1.000000000000000000, 0.9330127018922194093, 0.9330127018922194093 ) ) 
 REPRESENTATION_ITEM ( '' )  );
#47518=CARTESIAN_POINT ( 'NONE',  ( 114.4096469973842858, 226.8615022471902023, 5.000000000000051514 ) ) ;
#47519=LINE ( 'NONE', #23215, #24121 ) ;
#47520=ORIENTED_EDGE ( 'NONE', *, *, #39834, .F. ) ;
#47522=CARTESIAN_POINT ( 'NONE',  ( 186.6564022441646671, 272.5344008312805499, 15.68346972453315402 ) ) ;
#47524=CARTESIAN_POINT ( 'NONE',  ( 159.2394649670193303, 254.8361514374751664, -16.43133403737800791 ) ) ;
#47525=CARTESIAN_POINT ( 'NONE',  ( 193.7402390244666606, 294.2808330005247512, 13.97520787983859236 ) ) ;
#47527=VERTEX_POINT ( 'NONE', #74994 ) ;
#47528=CARTESIAN_POINT ( 'NONE',  ( 168.1726423428391399, 255.4859975196775963, 14.21197738914692366 ) ) ;
#47531=CARTESIAN_POINT ( 'NONE',  ( 148.3629184514745987, 273.6748826132846375, -8.219814532462343948 ) ) ;
#47532=CARTESIAN_POINT ( 'NONE',  ( 148.4666013490241596, 274.0772673839664435, 7.858165846707668045 ) ) ;
#47533=ORIENTED_EDGE ( 'NONE', *, *, #69640, .F. ) ;
#47541=CARTESIAN_POINT ( 'NONE',  ( 173.6836341738550971, 260.0703094413875647, 15.05886286463676349 ) ) ;
#47542=EDGE_CURVE ( 'NONE', #7044, #21557, #66948, .T. ) ;
#47543=VERTEX_POINT ( 'NONE', #46552 ) ;
#47544=CARTESIAN_POINT ( 'NONE',  ( 170.9926132455484264, 284.6176199787537939, 10.85232337705370576 ) ) ;
#47548=CARTESIAN_POINT ( 'NONE',  ( 155.6518451030846961, 261.0500913200531841, 17.91778754207898317 ) ) ;
#47549=CARTESIAN_POINT ( 'NONE',  ( 185.6025440602765002, 292.7411672476788453, -10.71517798447736425 ) ) ;
#47550=CARTESIAN_POINT ( 'NONE',  ( 157.2104826425669728, 258.3504519110855995, -16.92635148710569482 ) ) ;
#47551=CARTESIAN_POINT ( 'NONE',  ( 148.5637841791828464, 247.3923013555409796, 4.594050593750050204 ) ) ;
#47554=CARTESIAN_POINT ( 'NONE',  ( 96.71051312758956442, 217.4548013555409511, -4.594050593750042211 ) ) ;
#47556=CARTESIAN_POINT ( 'NONE',  ( 190.8604783348975502, 300.0669496974951471, 7.597731640149610222 ) ) ;
#47560=CARTESIAN_POINT ( 'NONE',  ( 156.7527532867754019, 259.1432624114326586, -17.18866891080081416 ) ) ;
#47561=ORIENTED_EDGE ( 'NONE', *, *, #7635, .T. ) ;
#47562=ORIENTED_EDGE ( 'NONE', *, *, #38263, .F. ) ;
#47566=CYLINDRICAL_SURFACE ( 'NONE', #59543, 17.82106496071139645 ) ;
#47568=CARTESIAN_POINT ( 'NONE',  ( 207.6470076888861342, 270.9918279736407385, 2.882721586646819212 ) ) ;
#47569=CARTESIAN_POINT ( 'NONE',  ( 83.25962220535622293, 225.0024278399160664, -9.188101187500093303 ) ) ;
#47571=ORIENTED_EDGE ( 'NONE', *, *, #28876, .T. ) ;
#47572=ADVANCED_FACE ( 'NONE', ( #54648 ), #56990, .F. ) ;
#47573=CARTESIAN_POINT ( 'NONE',  ( 200.5761841437080193, 283.2388536052437757, -18.29075185947827364 ) ) ;
#47574=ORIENTED_EDGE ( 'NONE', *, *, #71251, .F. ) ;
#47576=CARTESIAN_POINT ( 'NONE',  ( 204.8008807586744524, 272.7600038595665524, -10.89009281376315741 ) ) ;
#47578=CARTESIAN_POINT ( 'NONE',  ( 161.6188153416260604, 283.9408672562620950, 0.5238794243677475926 ) ) ;
#47582=CARTESIAN_POINT ( 'NONE',  ( 190.1843253477620408, 295.3820500736599115, 11.30047355920397223 ) ) ;
#47583=LINE ( 'NONE', #31385, #75577 ) ;
#47584=CARTESIAN_POINT ( 'NONE',  ( 159.5221561062548972, 254.3465160214695118, -16.91023001054109542 ) ) ;
#47585=CARTESIAN_POINT ( 'NONE',  ( 147.8939059469516621, 275.2579607316754959, -4.845476154560380166 ) ) ;
#47586=DIRECTION ( 'NONE',  ( -0.8660254037844387076, -0.4999999999999998890, -0.000000000000000000 ) ) ;
#47587=CARTESIAN_POINT ( 'NONE',  ( 110.7831656154890254, 224.7677522451417929, -5.000000000000041744 ) ) ;
#47589=CARTESIAN_POINT ( 'NONE',  ( 195.6387348270936002, 279.6800705220005057, -17.43641212817176722 ) ) ;
#47591=CARTESIAN_POINT ( 'NONE',  ( -2.524136441754524451, 180.8967562850347406, 2.649461200531984646E-14 ) ) ;
#47592=CARTESIAN_POINT ( 'NONE',  ( 161.3227470381586102, 251.2278010437646856, 14.45097375514160731 ) ) ;
#47594=CARTESIAN_POINT ( 'NONE',  ( 187.8464235218109195, 266.1023814865406507, -11.84412950951504229 ) ) ;
#47595=DIRECTION ( 'NONE',  ( -0.8660254037844387076, -0.4999999999999998890, -0.000000000000000000 ) ) ;
#47597=EDGE_LOOP ( 'NONE', ( #80511, #56434, #78783, #62880 ) ) ;
#47599=CARTESIAN_POINT ( 'NONE',  ( 202.4900219881211854, 279.9239892212719383, 15.63116161057562259 ) ) ;
#47600=ADVANCED_FACE ( 'NONE', ( #59008 ), #33368, .T. ) ;
#47601=CARTESIAN_POINT ( 'NONE',  ( 207.4764081617721843, 271.2873150223495600, 6.359972247200924578 ) ) ;
#47602=CARTESIAN_POINT ( 'NONE',  ( 194.5047661587782386, 293.7548580291293092, 14.86680123054176583 ) ) ;
#47606=CARTESIAN_POINT ( 'NONE',  ( 172.1884445069138678, 275.0993914995688669, 16.85348085832728060 ) ) ;
#47607=CARTESIAN_POINT ( 'NONE',  ( 163.2958758767942697, 283.7880877081312292, -3.557553060821605939 ) ) ;
#47609=B_SPLINE_CURVE_WITH_KNOTS ( 'NONE', 3,
 ( #77361, #44448, #75381, #60140, #21668, #52548, #83500, #47443, #9463, #850 ),
 .UNSPECIFIED., .F., .F.,
 ( 4, 2, 2, 2, 4 ),
 ( 0.001342876365094863422, 0.001763185234570876624, 0.002183494104046890261, 0.002603802973522903463, 0.003024111842998916666 ),
 .UNSPECIFIED. ) ;
#47610=CARTESIAN_POINT ( 'NONE',  ( 191.1700880229242614, 262.1676510039363279, 2.914548928543342576 ) ) ;
#47611=CARTESIAN_POINT ( 'NONE',  ( 161.8935665241663457, 250.2391126920490194, -13.69501063978231770 ) ) ;
#47612=CARTESIAN_POINT ( 'NONE',  ( 2.394847222749281190, 166.0643266524160140, -9.188101187500093303 ) ) ;
#47615=CARTESIAN_POINT ( 'NONE',  ( 175.6243877072629402, 255.6581301832358122, 8.239597966241703375 ) ) ;
#47618=CARTESIAN_POINT ( 'NONE',  ( 16.87327557256410060, 189.7369531367911293, -4.594050593750048428 ) ) ;
#47619=CARTESIAN_POINT ( 'NONE',  ( 181.7508493730100554, 276.2066116400742999, -17.76433735679825432 ) ) ;
#47621=CARTESIAN_POINT ( 'NONE',  ( 128.3382222415839635, 238.2365022471902307, 10.00000000000009948 ) ) ;
#47622=CARTESIAN_POINT ( 'NONE',  ( 173.4424205204250882, 272.5764413300324804, -16.36125399428295779 ) ) ;
#47624=DIRECTION ( 'NONE',  ( 0.4999999999999998890, -0.8660254037844385966, 0.000000000000000000 ) ) ;
#47625=CARTESIAN_POINT ( 'NONE',  ( 186.8357342210453851, 295.8110015290263277, -7.913238257363107486 ) ) ;
#47626=CARTESIAN_POINT ( 'NONE',  ( 190.3064699681596608, 261.7168245545821037, -0.7557934191962326631 ) ) ;
#47627=CARTESIAN_POINT ( 'NONE',  ( 74.50030963965139108, 200.4865022471901739, 1.119607411625061291E-15 ) ) ;
#47629=CARTESIAN_POINT ( 'NONE',  ( 203.5904874318909492, 269.7020407831449802, 7.034387229931597929 ) ) ;
#47630=CARTESIAN_POINT ( 'NONE',  ( 31.75860784375665702, 179.9548013555409796, -4.594050593750042211 ) ) ;
#47631=FACE_OUTER_BOUND ( 'NONE', #8318, .T. ) ;
#47632=CARTESIAN_POINT ( 'NONE',  ( 202.9930240272727815, 270.0243998824601590, -6.379419799043575701 ) ) ;
#47633=CARTESIAN_POINT ( 'NONE',  ( 198.8533049117289977, 286.2229679703367538, -18.60939981449148561 ) ) ;
#47639=CARTESIAN_POINT ( 'NONE',  ( 202.4943568615953779, 279.9164810001701085, 17.09064351659286984 ) ) ;
#47640=CARTESIAN_POINT ( 'NONE',  ( 149.4456112649506281, 271.7996036513546869, -12.95648166494593667 ) ) ;
#47641=CARTESIAN_POINT ( 'NONE',  ( 185.6350556674202892, 267.8156451814128332, -14.47898365169702828 ) ) ;
#47643=CARTESIAN_POINT ( 'NONE',  ( 185.5630754609182986, 290.7785217972672172, 12.70007870419082430 ) ) ;
#47644=CARTESIAN_POINT ( 'NONE',  ( 195.2466578971736908, 263.4181923903869915, -3.779627582060766322 ) ) ;
#47646=CARTESIAN_POINT ( 'NONE',  ( 25.13686162393831225, 191.9865022471903160, -10.00000000000009592 ) ) ;
#47649=CARTESIAN_POINT ( 'NONE',  ( 191.3638605175971747, 299.1950661814348678, 7.382965314423603154 ) ) ;
#47650=CARTESIAN_POINT ( 'NONE',  ( 178.5653124836910877, 256.7979852036974080, -7.281116805671778991 ) ) ;
#47652=EDGE_CURVE ( 'NONE', #33225, #62454, #2941, .T. ) ;
#47653=EDGE_LOOP ( 'NONE', ( #72524, #83462, #46315 ) ) ;
#47654=ORIENTED_EDGE ( 'NONE', *, *, #10351, .F. ) ;
#47657=VERTEX_POINT ( 'NONE', #75750 ) ;
#47663=CARTESIAN_POINT ( 'NONE',  ( 148.3190727836317535, 273.7508255376806119, 8.080277324579027365 ) ) ;
#47664=EDGE_CURVE ( 'NONE', #88081, #3978, #65242, .T. ) ;
#47665=AXIS2_PLACEMENT_3D ( 'NONE', #48666, #17766, #18267 ) ;
#47666=CARTESIAN_POINT ( 'NONE',  ( 180.7465490385022520, 287.0650312162388786, -13.47353663417578673 ) ) ;
#47669=CARTESIAN_POINT ( 'NONE',  ( 172.4419760422836134, 290.9306500000749907, -0.6531725299933459628 ) ) ;
#47672=CARTESIAN_POINT ( 'NONE',  ( 159.6610344727618269, 254.1059716346071866, 15.33388637456589620 ) ) ;
#47673=CARTESIAN_POINT ( 'NONE',  ( 50.35065686154756293, 206.0024278399161233, 9.188101187500095079 ) ) ;
#47675=CARTESIAN_POINT ( 'NONE',  ( 159.5503045904109740, 254.6834971896836919, 15.44555384949675236 ) ) ;
#47676=CARTESIAN_POINT ( 'NONE',  ( 86.94711308317737064, 232.5530062829863027, -4.648177544792955347E-16 ) ) ;
#47677=CARTESIAN_POINT ( 'NONE',  ( -17.42236680055705023, 149.2012482093457777, 0.000000000000000000 ) ) ;
#47679=CARTESIAN_POINT ( 'NONE',  ( 189.7094295309238419, 300.0606247079692253, 5.078421157105148076 ) ) ;
#47681=CARTESIAN_POINT ( 'NONE',  ( 168.2925188335944711, 279.9374692537770102, 14.50896303939727261 ) ) ;
#47683=CARTESIAN_POINT ( 'NONE',  ( 175.1988943574488644, 261.2637229863152015, -14.23086624307204850 ) ) ;
#47685=DIRECTION ( 'NONE',  ( 0.4999999999999998890, -0.8660254037844385966, 0.000000000000000000 ) ) ;
#47686=CARTESIAN_POINT ( 'NONE',  ( 147.5851099763508216, 275.0220864107570264, -4.372720440640867956 ) ) ;
#47687=CARTESIAN_POINT ( 'NONE',  ( 149.7119746935222793, 271.3382486597900538, 12.05352563709836922 ) ) ;
#47688=CARTESIAN_POINT ( 'NONE',  ( 177.2704016510258782, 269.4991140589317524, 16.10227469079067220 ) ) ;
#47690=CARTESIAN_POINT ( 'NONE',  ( 164.9103019330012216, 245.0139736909548560, 2.841678961959298810 ) ) ;
#47693=CARTESIAN_POINT ( 'NONE',  ( -22.42236680055709641, 157.8615022471902591, 0.000000000000000000 ) ) ;
#47694=CARTESIAN_POINT ( 'NONE',  ( 101.8248682511026573, 241.8464784336661353, 1.353441290958777327E-15 ) ) ;
#47695=EDGE_LOOP ( 'NONE', ( #22423, #25473, #95941, #62358 ) ) ;
#47696=CARTESIAN_POINT ( 'NONE',  ( 191.7247331938518187, 298.5700163710982338, -9.650650827884682315 ) ) ;
#47697=CARTESIAN_POINT ( 'NONE',  ( 22.90194105960797089, 172.4824982072973967, 3.021315404115420679E-15 ) ) ;
#47698=CARTESIAN_POINT ( 'NONE',  ( 154.9903553346911735, 262.1958252075976361, -18.39016733948542637 ) ) ;
#47699=CARTESIAN_POINT ( 'NONE',  ( 182.8460422257451512, 285.5338780432256272, -15.29722646433579492 ) ) ;
#47701=CARTESIAN_POINT ( 'NONE',  ( 174.9976167624121501, 253.1009688407763178, 5.034851627924513018 ) ) ;
#47703=CARTESIAN_POINT ( 'NONE',  ( 162.8223739550644211, 248.6303710312858186, -11.16939803179192658 ) ) ;
#47705=CARTESIAN_POINT ( 'NONE',  ( 185.2286309111798914, 261.0640975966447286, 10.24933178681469137 ) ) ;
#47706=CARTESIAN_POINT ( 'NONE',  ( 206.3426153068844542, 272.1430791857031295, 8.023365743556523100 ) ) ;
#47707=CARTESIAN_POINT ( 'NONE',  ( 137.8467198073504107, 241.2048013555409796, 4.594050593750051981 ) ) ;
#47708=CARTESIAN_POINT ( 'NONE',  ( 150.6916211261701619, 269.6414512649903941, -15.44346024757110847 ) ) ;
#47709=FACE_OUTER_BOUND ( 'NONE', #84340, .T. ) ;
#47710=CARTESIAN_POINT ( 'NONE',  ( 187.6813309808503050, 281.4444333665542217, -16.91448409808978326 ) ) ;
#47712=CARTESIAN_POINT ( 'NONE',  ( 43.28705038798948124, 204.9869531367911293, 4.594050593750046652 ) ) ;
#47719=CARTESIAN_POINT ( 'NONE',  ( 171.9522100717342710, 260.0157765023859042, 15.50740241267492969 ) ) ;
#47720=CARTESIAN_POINT ( 'NONE',  ( 151.3906727466529389, 278.2750905898312794, -1.659020316575751330 ) ) ;
#47723=CARTESIAN_POINT ( 'NONE',  ( 203.5555343017997529, 278.0784677578903370, -15.71723084798551362 ) ) ;
#47724=CARTESIAN_POINT ( 'NONE',  ( 181.7766938514437243, 262.7534622773716819, 12.50707551241419324 ) ) ;
#47725=CARTESIAN_POINT ( 'NONE',  ( 125.9386101817166974, 233.5177522451417929, 5.000000000000051514 ) ) ;
#47726=B_SPLINE_SURFACE_WITH_KNOTS ( 'NONE', 3, 1, ( 
 ( #68172, #37764 ),
 ( #21111, #29195 ),
 ( #82928, #84909 ),
 ( #83925, #60063 ),
 ( #59565, #51989 ),
 ( #76301, #13988 ),
 ( #30682, #68666 ),
 ( #99590, #30174 ),
 ( #91026, #99099 ),
 ( #45850, #44865 ),
 ( #61061, #6389 ),
 ( #60556, #29683 ),
 ( #53464, #84414 ),
 ( #44373, #76773 ),
 ( #7366, #15451 ),
 ( #69166, #61562 ),
 ( #92509, #53953 ),
 ( #46350, #77274 ),
 ( #7885, #28681 ),
 ( #31651, #86940 ),
 ( #38762, #79326 ),
 ( #17472, #17991 ),
 ( #33175, #93512 ),
 ( #31157, #24565 ),
 ( #63070, #39735 ),
 ( #87459, #56469 ),
 ( #54444, #92999 ),
 ( #69666, #25066 ),
 ( #55448, #9377 ),
 ( #95020, #70155 ),
 ( #77794, #48382 ),
 ( #15968, #94512 ),
 ( #40752, #62549 ),
 ( #62046, #8379 ) ),
 .UNSPECIFIED., .T., .F., .F.,
 ( 4, 2, 2, 2, 2, 2, 2, 2, 2, 2, 2, 2, 2, 2, 2, 2, 4 ),
 ( 2, 2 ),
 ( 0.000000000000000000, 0.06250000000000000000, 0.1250000000000000000, 0.1875000000000000000, 0.2500000000000000000, 0.3125000000000000000, 0.3750000000000000000, 0.4375000000000000000, 0.5000000000000000000, 0.5625000000000000000, 0.6250000000000000000, 0.6875000000000000000, 0.7500000000000000000, 0.8125000000000000000, 0.8750000000000000000, 0.9375000000000000000, 1.000000000000000000 ),
 ( 0.000000000000000000, 1.000000000000000000 ),
 .UNSPECIFIED. ) ;
#47727=CARTESIAN_POINT ( 'NONE',  ( 55.77019854693759271, 214.5530062829863311, -4.648177544792955347E-16 ) ) ;
#47730=CARTESIAN_POINT ( 'NONE',  ( 203.0337691736598629, 278.9821914694464340, 16.08167820133810011 ) ) ;
#47731=FACE_OUTER_BOUND ( 'NONE', #75, .T. ) ;
#47732=CARTESIAN_POINT ( 'NONE',  ( 23.17945691357580529, 178.0643266524160424, -9.188101187500093303 ) ) ;
#47734=CARTESIAN_POINT ( 'NONE',  ( 188.8691947583266426, 290.7266936548607532, -15.09369555602670587 ) ) ;
#47736=CARTESIAN_POINT ( 'NONE',  ( 198.0902711536284357, 277.7603059513703556, -15.87033955601944690 ) ) ;
#47737=CARTESIAN_POINT ( 'NONE',  ( 57.52260328274599033, 204.0177522451418497, -10.00000000000009592 ) ) ;
#47738=CARTESIAN_POINT ( 'NONE',  ( 174.4148835039708274, 289.3800151988198195, 7.905235673531343821 ) ) ;
#47740=CARTESIAN_POINT ( 'NONE',  ( 157.8811243250769110, 257.1888664433053009, -17.39256699147873064 ) ) ;
#47741=CARTESIAN_POINT ( 'NONE',  ( 162.2469855708762054, 251.8525454486305648, -12.98361378634216123 ) ) ;
#47743=B_SPLINE_CURVE_WITH_KNOTS ( 'NONE', 3,
 ( #66310, #82561, #13125, #26814, #34410, #80558 ),
 .UNSPECIFIED., .F., .F.,
 ( 4, 2, 4 ),
 ( 0.02004572608914358123, 0.02459847040748617750, 0.02915121472582877377 ),
 .UNSPECIFIED. ) ;
#47744=CARTESIAN_POINT ( 'NONE',  ( 31.27120823407814854, 178.8615022471902023, 5.000000000000051514 ) ) ;
#47745=CARTESIAN_POINT ( 'NONE',  ( 140.4712518949831974, 264.1589784336661637, -6.496448406907675876E-16 ) ) ;
#47746=CARTESIAN_POINT ( 'NONE',  ( 202.2576150004249200, 280.3265299319959354, 16.24828394350762295 ) ) ;
#47747=CARTESIAN_POINT ( 'NONE',  ( -11.70556275232237908, 173.2369531367911293, -4.594050593750048428 ) ) ;
#47751=CARTESIAN_POINT ( 'NONE',  ( 186.1518260931114526, 260.7827538074319023, 6.339317543960328649 ) ) ;
#47752=CARTESIAN_POINT ( 'NONE',  ( 164.7762319088960794, 245.2461897844768828, 2.994040459560653122 ) ) ;
#47756=CARTESIAN_POINT ( 'NONE',  ( 150.5287101026835330, 271.9236214347867531, -12.89083132144543775 ) ) ;
#47757=CARTESIAN_POINT ( 'NONE',  ( 178.6565837683001519, 285.5687190954733410, 13.02810775182850911 ) ) ;
#47758=CARTESIAN_POINT ( 'NONE',  ( 168.7068454911210438, 288.1994200320167465, 0.5267417468238662082 ) ) ;
#47760=CARTESIAN_POINT ( 'NONE',  ( 160.5489464122825325, 252.5680630427104063, 14.85483651643795788 ) ) ;
#47762=CARTESIAN_POINT ( 'NONE',  ( 159.2394649670193303, 254.8361514374751664, -16.43133403737800791 ) ) ;
#47764=CARTESIAN_POINT ( 'NONE',  ( 192.0331311261993790, 298.0358554833232461, 11.82583305898340953 ) ) ;
#47769=ORIENTED_EDGE ( 'NONE', *, *, #26141, .F. ) ;
#47770=ORIENTED_EDGE ( 'NONE', *, *, #33012, .F. ) ;
#47775=CARTESIAN_POINT ( 'NONE',  ( 6.522775935009023307, 186.1199935810940644, 2.679491924311251605 ) ) ;
#47776=ADVANCED_FACE ( 'NONE', ( #51028 ), #11565, .T. ) ;
#47785=CARTESIAN_POINT ( 'NONE',  ( 200.1444820856229967, 283.9865835035790269, 17.93386694781497326 ) ) ;
#47787=CARTESIAN_POINT ( 'NONE',  ( 161.0515428782683500, 277.3244187559503189, -13.42420650014866368 ) ) ;
#47790=CARTESIAN_POINT ( 'NONE',  ( 170.8211178702818529, 255.2134001104743390, -11.38359876985272301 ) ) ;
#47792=ORIENTED_EDGE ( 'NONE', *, *, #73326, .T. ) ;
#47795=ORIENTED_EDGE ( 'NONE', *, *, #23524, .F. ) ;
#47796=CARTESIAN_POINT ( 'NONE',  ( 186.0400780920065529, 271.7087950812899066, 16.90619359840448510 ) ) ;
#47798=( BOUNDED_CURVE ( )  B_SPLINE_CURVE ( 2, ( #41161, #80735, #72098, #18392, #49287, #86338, #80223, #3213, #34097 ),
 .UNSPECIFIED., .F., .T. ) 
 B_SPLINE_CURVE_WITH_KNOTS ( ( 3, 2, 2, 2, 3 ),
 ( 0.5282258064516128782, 0.5295698924731182533, 0.5322580645161290036, 0.5349462365591397539, 0.5362903225806451291 ),
 .UNSPECIFIED. ) 
 CURVE ( )  GEOMETRIC_REPRESENTATION_ITEM ( )  RATIONAL_B_SPLINE_CURVE ( ( 0.9330127018922194093, 0.9330127018922194093, 1.000000000000000000, 0.8660254037844387076, 1.000000000000000000, 0.8660254037844387076, 1.000000000000000000, 0.9330127018922194093, 0.9330127018922194093 ) ) 
 REPRESENTATION_ITEM ( '' )  );
#47799=DIRECTION ( 'NONE',  ( -0.8660254037844387076, -0.4999999999999998890, -0.000000000000000000 ) ) ;
#47800=CARTESIAN_POINT ( 'NONE',  ( 162.9148809972199672, 269.1323162226891554, 17.43693885807998001 ) ) ;
#47801=CARTESIAN_POINT ( 'NONE',  ( 147.8308140999695866, 274.5965143850199865, -7.866624397492971710 ) ) ;
#47803=DIRECTION ( 'NONE',  ( 0.4999999999999998890, -0.8660254037844385966, 0.000000000000000000 ) ) ;
#47805=B_SPLINE_CURVE_WITH_KNOTS ( 'NONE', 3,
 ( #23172, #60661, #29789, #68281 ),
 .UNSPECIFIED., .F., .F.,
 ( 4, 4 ),
 ( 0.002207507469835296148, 0.004300347803759868928 ),
 .UNSPECIFIED. ) ;
#47807=CARTESIAN_POINT ( 'NONE',  ( 205.7829192689729325, 274.2205238267313234, 11.21202327925415254 ) ) ;
#47808=CARTESIAN_POINT ( 'NONE',  ( 206.0691053506789387, 273.7248349927971844, 11.70564474658248422 ) ) ;
#47809=CARTESIAN_POINT ( 'NONE',  ( 197.9552487813401456, 287.7784468162186613, 17.26493623863614602 ) ) ;
#47810=ORIENTED_EDGE ( 'NONE', *, *, #87678, .F. ) ;
#47812=CARTESIAN_POINT ( 'NONE',  ( 64.35513503747660025, 196.4155109091896350, 2.679491924311254714 ) ) ;
#47813=CARTESIAN_POINT ( 'NONE',  ( 159.9647205790309101, 253.5799718689968927, -16.48298384325780219 ) ) ;
#47814=CARTESIAN_POINT ( 'NONE',  ( 159.3773945546513460, 271.5416235043197162, -16.14591210334819849 ) ) ;
#47815=CARTESIAN_POINT ( 'NONE',  ( 161.6673510627899191, 250.6309293646106653, 13.01175935005004192 ) ) ;
#47816=CARTESIAN_POINT ( 'NONE',  ( 190.7952227603998665, 261.9688979877246311, -0.5812294033076593758 ) ) ;
#47818=CARTESIAN_POINT ( 'NONE',  ( 185.8626946602280441, 259.3471889805154547, 7.308832903665572367 ) ) ;
#47819=CARTESIAN_POINT ( 'NONE',  ( 131.5677753063155251, 246.7677522451418497, 10.00000000000009592 ) ) ;
#47820=CARTESIAN_POINT ( 'NONE',  ( 194.9499559406243918, 279.5747724307917679, 17.51673600049429780 ) ) ;
#47821=CARTESIAN_POINT ( 'NONE',  ( 8.953011887168695893, 182.6427522451419350, 10.00000000000009237 ) ) ;
#47822=CARTESIAN_POINT ( 'NONE',  ( 91.08134800299070832, 214.2048013555409796, 4.594050593750051981 ) ) ;
#47825=CARTESIAN_POINT ( 'NONE',  ( 169.7087038524299771, 280.0432160542959537, -13.57890784763611336 ) ) ;
#47826=CARTESIAN_POINT ( 'NONE',  ( 3.531332017333847606, 172.8458772461660828, 9.188101187500095079 ) ) ;
#47830=CARTESIAN_POINT ( 'NONE',  ( 200.4775477985258760, 283.4096967665721536, 16.80647240730505487 ) ) ;
#47831=ORIENTED_EDGE ( 'NONE', *, *, #100099, .F. ) ;
#47832=VERTEX_POINT ( 'NONE', #50530 ) ;
#47833=CARTESIAN_POINT ( 'NONE',  ( 200.6160348301466456, 267.6256034195902203, -2.850748744823686565 ) ) ;
#47838=CARTESIAN_POINT ( 'NONE',  ( 185.5962948356213360, 286.5636094107885015, 15.98812411951390544 ) ) ;
#47839=CARTESIAN_POINT ( 'NONE',  ( 164.7647380297938184, 248.9862001899016946, 10.10785415616959071 ) ) ;
#47840=CARTESIAN_POINT ( 'NONE',  ( 39.87759600423577666, 184.6423013555410080, -4.594050593750043987 ) ) ;
#47841=CARTESIAN_POINT ( 'NONE',  ( 78.30721297357251842, 216.0177522451418497, -10.00000000000009592 ) ) ;
#47842=CARTESIAN_POINT ( 'NONE',  ( 195.8878223364301050, 275.2230923960996165, 15.66255634890894832 ) ) ;
#47845=FACE_OUTER_BOUND ( 'NONE', #42210, .T. ) ;
#47846=CARTESIAN_POINT ( 'NONE',  ( 175.1702272577395263, 281.4177487094669345, -14.21329840767373121 ) ) ;
#47847=CARTESIAN_POINT ( 'NONE',  ( -14.60124842228533915, 168.5024278399160949, 9.188101187500095079 ) ) ;
#47848=CARTESIAN_POINT ( 'NONE',  ( 157.0935036675524827, 258.5530654392286465, 17.32636058289560665 ) ) ;
#47850=CARTESIAN_POINT ( 'NONE',  ( 198.8157103782086210, 286.2880836124806478, -18.60729372713428020 ) ) ;
#47854=CARTESIAN_POINT ( 'NONE',  ( 194.8708600166808651, 293.1207648669033006, -14.79199694356877970 ) ) ;
#47855=CARTESIAN_POINT ( 'NONE',  ( 192.5555981258711995, 265.1457337795512785, 7.710077344952797063 ) ) ;
#47856=CARTESIAN_POINT ( 'NONE',  ( 204.5730103890532519, 276.3161474792809145, 14.88139715235883109 ) ) ;
#47857=CARTESIAN_POINT ( 'NONE',  ( 70.17018262072913615, 217.9865022471902876, 10.00000000000009415 ) ) ;
#47858=CARTESIAN_POINT ( 'NONE',  ( 148.3930300673291640, 273.6227277647267897, 8.375036249079425232 ) ) ;
#47859=EDGE_CURVE ( 'NONE', #38166, #53063, #8818, .T. ) ;
#47861=AXIS2_PLACEMENT_3D ( 'NONE', #8367, #92496, #91014 ) ;
#47862=CARTESIAN_POINT ( 'NONE',  ( 152.9502192050138660, 266.8376656511403553, -16.03576590126549561 ) ) ;
#47864=CARTESIAN_POINT ( 'NONE',  ( 117.3868696429430258, 229.3923013555409796, 4.594050593750050204 ) ) ;
#47869=DIRECTION ( 'NONE',  ( 0.5000000000000001110, -0.8660254037844385966, 0.000000000000000000 ) ) ;
#47871=CARTESIAN_POINT ( 'NONE',  ( 190.8775532225699862, 300.0373751245133462, -6.456187174708069243 ) ) ;
#47873=CARTESIAN_POINT ( 'NONE',  ( 149.6890529486499872, 271.3779502865075983, -12.51465682618088593 ) ) ;
#47874=CARTESIAN_POINT ( 'NONE',  ( 91.79731502344390037, 212.2592609112380444, 2.679491924311254714 ) ) ;
#47875=CARTESIAN_POINT ( 'NONE',  ( 173.1586067699058162, 289.7215660399545527, -1.264861486351297248 ) ) ;
#47879=CARTESIAN_POINT ( 'NONE',  ( 175.1138237960793447, 279.3531053840294476, 15.84073920059228158 ) ) ;
#47880=CARTESIAN_POINT ( 'NONE',  ( 199.6627426296996930, 270.0018726912092006, 9.250069944390398646 ) ) ;
#47884=CARTESIAN_POINT ( 'NONE',  ( 185.1790142135946837, 260.5378326486920741, -9.806357480331048038 ) ) ;
#47885=CARTESIAN_POINT ( 'NONE',  ( 191.7967966825411850, 283.9693557995756805, 17.70397221340040161 ) ) ;
#47886=CARTESIAN_POINT ( 'NONE',  ( 192.7944000592152634, 296.7172990131160759, 11.44860011299869740 ) ) ;
#47888=VERTEX_POINT ( 'NONE', #44917 ) ;
#47889=CARTESIAN_POINT ( 'NONE',  ( 190.7357586861858749, 280.8065426626702106, 16.64018919219373061 ) ) ;
#47891=LINE ( 'NONE', #7037, #11004 ) ;
#47893=CARTESIAN_POINT ( 'NONE',  ( 167.5344527987841730, 280.9027864911226402, 11.65609303130555574 ) ) ;
#47894=CYLINDRICAL_SURFACE ( 'NONE', #14361, 17.82106496071139645 ) ;
#47895=CARTESIAN_POINT ( 'NONE',  ( 164.4854433269806577, 246.2060377238486808, -1.879056492287135116 ) ) ;
#47899=CARTESIAN_POINT ( 'NONE',  ( 162.8756881843043516, 250.5380280774768949, 12.81046238701583029 ) ) ;
#47900=CARTESIAN_POINT ( 'NONE',  ( 192.4380962356868281, 295.3344353383980661, 13.50754959408193656 ) ) ;
#47906=CARTESIAN_POINT ( 'NONE',  ( 203.4696564630250464, 278.2272125378923988, -16.38980782817167636 ) ) ;
#47907=EDGE_CURVE ( 'NONE', #98060, #75682, #86206, .T. ) ;
#47909=ORIENTED_EDGE ( 'NONE', *, *, #26316, .F. ) ;
#47910=CARTESIAN_POINT ( 'NONE',  ( 177.9882410936357928, 260.8588164829307630, 12.21663056129005120 ) ) ;
#47914=B_SPLINE_CURVE_WITH_KNOTS ( 'NONE', 3,
 ( #8075, #465, #46541, #62745 ),
 .UNSPECIFIED., .F., .F.,
 ( 4, 4 ),
 ( 0.008817850388587639837, 0.01395074355647914210 ),
 .UNSPECIFIED. ) ;
#47919=CARTESIAN_POINT ( 'NONE',  ( 182.7138520656610012, 280.2226620527670775, -16.11794820187313704 ) ) ;
#47920=CARTESIAN_POINT ( 'NONE',  ( 165.0477436618537865, 244.7759176335020186, -2.027991469056170448 ) ) ;
#47921=CARTESIAN_POINT ( 'NONE',  ( 190.0146931831988013, 301.5318925525250506, 2.191471318341308372 ) ) ;
#47922=CARTESIAN_POINT ( 'NONE',  ( 179.4722142099873565, 269.7276464518548096, -17.35046799866735157 ) ) ;
#47924=CARTESIAN_POINT ( 'NONE',  ( 170.9484186264854770, 250.8673865788455544, -5.551388615809983662 ) ) ;
#47925=CARTESIAN_POINT ( 'NONE',  ( 196.8708119716154954, 268.3476497963631573, -11.07389558091716708 ) ) ;
#47926=CARTESIAN_POINT ( 'NONE',  ( 153.8479027513132280, 279.7076740674982034, 2.196726205667342668 ) ) ;
#47927=CARTESIAN_POINT ( 'NONE',  ( 127.4808708382166316, 256.6589784336661637, -6.496448406907675876E-16 ) ) ;
#47928=VERTEX_POINT ( 'NONE', #53023 ) ;
#47929=CARTESIAN_POINT ( 'NONE',  ( 186.6466788774901602, 262.7990401948939621, -9.116086771617830209 ) ) ;
#47930=VERTEX_POINT ( 'NONE', #45418 ) ;
#47932=ORIENTED_EDGE ( 'NONE', *, *, #96726, .F. ) ;
#47934=CARTESIAN_POINT ( 'NONE',  ( 201.8235137129046279, 275.1765603161098284, 13.33099703020108073 ) ) ;
#47935=CARTESIAN_POINT ( 'NONE',  ( 180.9179439205437916, 256.0455442330405731, 0.7724379216420866889 ) ) ;
#47937=CARTESIAN_POINT ( 'NONE',  ( 192.0467657490588351, 298.0122396237888438, 11.75052100010666045 ) ) ;
#47940=CARTESIAN_POINT ( 'NONE',  ( 173.4000888393750017, 287.4655024987716843, -9.837467039034411442 ) ) ;
#47942=CARTESIAN_POINT ( 'NONE',  ( 174.9461632972169696, 282.2965899055037085, 14.42753729772996252 ) ) ;
#47943=CARTESIAN_POINT ( 'NONE',  ( 177.2261086063719517, 256.1163090582663244, -7.433373391858083323 ) ) ;
#47944=VERTEX_POINT ( 'NONE', #38814 ) ;
#47945=CARTESIAN_POINT ( 'NONE',  ( 147.6884207308302450, 274.8431469350302336, -8.096293592099874203 ) ) ;
#47949=CARTESIAN_POINT ( 'NONE',  ( 157.1454194340104209, 276.7041856997979039, 10.24769222078917608 ) ) ;
#47950=CARTESIAN_POINT ( 'NONE',  ( 192.1068185053286754, 297.9082251987945824, -9.660304852024209410 ) ) ;
#47952=CARTESIAN_POINT ( 'NONE',  ( 162.8996025780091941, 248.4966071325470125, 11.23567065566008516 ) ) ;
#47953=CARTESIAN_POINT ( 'NONE',  ( 153.1401327494902773, 270.1234001006548624, 14.03976522339925381 ) ) ;
#47954=CARTESIAN_POINT ( 'NONE',  ( 151.5066875197445597, 274.9073607968387023, -8.887479126886400849 ) ) ;
#47955=CARTESIAN_POINT ( 'NONE',  ( 200.7694952279801157, 282.9040289856181403, -17.94628235092568502 ) ) ;
#47958=CARTESIAN_POINT ( 'NONE',  ( 147.1199024702499969, 275.8278494473859723, 5.224467159276165340 ) ) ;
#47959=CARTESIAN_POINT ( 'NONE',  ( 186.8442235758623156, 262.5257503668073582, -8.765433223893147385 ) ) ;
#47960=CARTESIAN_POINT ( 'NONE',  ( 193.5216815486326425, 276.1393389031752577, -16.40952103877357970 ) ) ;
#47961=DIRECTION ( 'NONE',  ( 0.5000000000000048850, -0.8660254037844358210, 0.000000000000000000 ) ) ;
#47962=CARTESIAN_POINT ( 'NONE',  ( 184.5612557885503975, 296.9796338933509219, -4.430542032517011286 ) ) ;
#47963=CARTESIAN_POINT ( 'NONE',  ( 192.0645969571214096, 297.9813550654635605, 11.46542907566974812 ) ) ;
#47967=CARTESIAN_POINT ( 'NONE',  ( -6.807019788225388446, 173.0024278399160949, 9.188101187500095079 ) ) ;
#47968=CARTESIAN_POINT ( 'NONE',  ( 92.65049840370248546, 233.4869531367911293, 4.594050593750046652 ) ) ;
#47969=CARTESIAN_POINT ( 'NONE',  ( 34.80747863286459420, 184.2365022471901739, 10.00000000000009948 ) ) ;
#47970=CARTESIAN_POINT ( 'NONE',  ( 180.2468139727683649, 280.2236653090821505, -17.21193327238699666 ) ) ;
#47973=CARTESIAN_POINT ( 'NONE',  ( 202.8151641853381477, 279.3608264160075692, -16.28741359973609448 ) ) ;
#47979=CARTESIAN_POINT ( 'NONE',  ( 190.4469008128301653, 300.3948906649509922, -0.6521089053012534276 ) ) ;
#47980=CARTESIAN_POINT ( 'NONE',  ( 162.7070706717508699, 248.8300821762643693, -9.986337079333621247 ) ) ;
#47981=CARTESIAN_POINT ( 'NONE',  ( 207.6250539976609275, 271.0298528822568187, 4.860623598087060238 ) ) ;
#47983=CARTESIAN_POINT ( 'NONE',  ( -9.181706736895311138, 177.0530062829863027, -4.648177544792955347E-16 ) ) ;
#47984=DIRECTION ( 'NONE',  ( 0.4999999999999998890, -0.8660254037844385966, 0.000000000000000000 ) ) ;
#47985=CARTESIAN_POINT ( 'NONE',  ( 157.0957870390718369, 258.5491105237443321, 17.69218919045495397 ) ) ;
#47987=CARTESIAN_POINT ( 'NONE',  ( -7.357133217438179607, 159.8927522451417929, -10.00000000000009237 ) ) ;
#47989=B_SPLINE_CURVE_WITH_KNOTS ( 'NONE', 3,
 ( #92726, #76983, #22292, #38976, #21795, #37969, #76026, #7085, #495, #6603, #53192, #23276, #14693, #45576, #46070, #76504, #92246, #22796, #16192, #84629, #69881, #85130, #85649, #6096, #36991, #10331, #34611, #27026, #25522, #58400, #79767, #33630, #57910, #19929, #95967, #17936, #81259, #88889, #42692, #73623 ),
 .UNSPECIFIED., .F., .F.,
 ( 4, 2, 2, 2, 2, 2, 2, 2, 2, 2, 2, 2, 2, 2, 2, 2, 2, 2, 2, 4 ),
 ( 0.003159330915503282683, 0.003354433587230957418, 0.003549536258958632586, 0.003647087594822461497, 0.003744638930686289974, 0.003939741602413947795, 0.004329946945869263437, 0.004720152289324578213, 0.005500562976235209497, 0.006280973663145839915, 0.007061384350056471200, 0.007841795036967101618, 0.007939346372830951779, 0.008036897708694801939, 0.008085673376626687989, 0.008134449044558574038, 0.008232000380422342667, 0.008622205723877195138, 0.009012411067332047609, 0.009402616410786900081 ),
 .UNSPECIFIED. ) ;
#47990=CARTESIAN_POINT ( 'NONE',  ( 207.8575108622103755, 270.6272257822888037, -6.381720258959569847 ) ) ;
#47991=CARTESIAN_POINT ( 'NONE',  ( 36.87296296726972855, 204.3464784336661637, 1.353441290958777327E-15 ) ) ;
#47992=B_SPLINE_CURVE_WITH_KNOTS ( 'NONE', 3,
 ( #26201, #47979, #71816, #33816, #10497, #86555, #55571, #78924, #79938, #49488, #72828, #32291 ),
 .UNSPECIFIED., .F., .F.,
 ( 4, 2, 2, 2, 2, 4 ),
 ( 0.001378329982659087533, 0.001584756524673330271, 0.001791183066687573010, 0.002204036150716021623, 0.002616889234744470237, 0.003029742318772918417 ),
 .UNSPECIFIED. ) ;
#47993=CARTESIAN_POINT ( 'NONE',  ( 62.85372508080289577, 219.3464784336661637, 1.353441290958777327E-15 ) ) ;
#47994=CARTESIAN_POINT ( 'NONE',  ( 164.4708158012598460, 246.8356330233726794, -5.687495631043780087 ) ) ;
#47996=CARTESIAN_POINT ( 'NONE',  ( 166.9993039719644230, 259.7585743740527278, 15.88680828586103821 ) ) ;
#47999=B_SPLINE_CURVE_WITH_KNOTS ( 'NONE', 3,
 ( #5465, #35857, #53044, #43942, #52058, #59127, #14563, #66751, #14059, #68742, #20668, #44443, #21178, #5959, #36850, #90611 ),
 .UNSPECIFIED., .F., .F.,
 ( 4, 2, 2, 2, 2, 2, 2, 4 ),
 ( 8.673617379884035472E-19, 0.0003786681000627550929, 0.0007573362001255093184, 0.001136004300188263490, 0.001514672400251017769, 0.001893340500313771832, 0.002272008600376526112, 0.003029344800502178654 ),
 .UNSPECIFIED. ) ;
#48002=CARTESIAN_POINT ( 'NONE',  ( 198.4782858197754649, 286.8725200914082620, -17.44895083299520522 ) ) ;
#48003=CARTESIAN_POINT ( 'NONE',  ( 196.3507576896697344, 290.5575069072837664, -17.68249398312240928 ) ) ;
#48004=ORIENTED_EDGE ( 'NONE', *, *, #57294, .F. ) ;
#48006=CARTESIAN_POINT ( 'NONE',  ( 63.28708487846012076, 207.3458772461660544, 9.188101187500095079 ) ) ;
#48008=CARTESIAN_POINT ( 'NONE',  ( 94.51141663858166453, 213.8262482093457493, 3.021315404115420679E-15 ) ) ;
#48010=CARTESIAN_POINT ( 'NONE',  ( 159.9307118030769175, 253.6388767968520881, 16.60600887889890487 ) ) ;
#48012=CARTESIAN_POINT ( 'NONE',  ( 153.5280555550942267, 264.7286027217564879, 16.61052749018010388 ) ) ;
#48015=CARTESIAN_POINT ( 'NONE',  ( 125.7401460302306759, 236.7365022471902023, 10.00000000000009592 ) ) ;
#48018=CARTESIAN_POINT ( 'NONE',  ( 207.6508796976096107, 270.9851214578045528, 6.713685698622268383 ) ) ;
#48023=CARTESIAN_POINT ( 'NONE',  ( 159.9997000813754084, 253.5193855937126841, -16.28798248637880519 ) ) ;
#48024=CARTESIAN_POINT ( 'NONE',  ( 207.3206384775119488, 270.4334275325076646, -0.2364287663163220921 ) ) ;
#48031=EDGE_CURVE ( 'NONE', #40710, #21425, #96666, .T. ) ;
#48032=CARTESIAN_POINT ( 'NONE',  ( 170.3389527966260175, 250.2486659550142178, 3.410583519328374003 ) ) ;
#48033=CARTESIAN_POINT ( 'NONE',  ( 148.4796866745341219, 273.9119512061620298, 7.990242866642934594 ) ) ;
#48038=ADVANCED_FACE ( 'NONE', ( #1335 ), #3647, .F. ) ;
#48039=ADVANCED_FACE ( 'NONE', ( #85053 ), #39891, .T. ) ;
#48040=VERTEX_POINT ( 'NONE', #48008 ) ;
#48045=CARTESIAN_POINT ( 'NONE',  ( 192.1943038168404314, 277.1473907896511264, 17.36549850453357635 ) ) ;
#48047=CARTESIAN_POINT ( 'NONE',  ( 194.8598199529639317, 293.1398868181796615, -15.91766051364927570 ) ) ;
#48049=CARTESIAN_POINT ( 'NONE',  ( 155.6276701977099890, 261.0919634844306643, 17.49722577287685255 ) ) ;
#48050=CARTESIAN_POINT ( 'NONE',  ( 186.2639079497381545, 293.1677061230143977, -10.74393367941972244 ) ) ;
#48051=CARTESIAN_POINT ( 'NONE',  ( 157.1850763439666139, 258.3944569110938687, -16.98181238659443437 ) ) ;
#48052=CARTESIAN_POINT ( 'NONE',  ( 142.9371257517045137, 259.7655487066560340, -7.305945665944389766 ) ) ;
#48055=CARTESIAN_POINT ( 'NONE',  ( 84.85626976964255164, 228.9869531367911293, 4.594050593750046652 ) ) ;
#48057=CARTESIAN_POINT ( 'NONE',  ( 151.3883635558152321, 268.4346579770563608, 15.44343517165679103 ) ) ;
#48061=CARTESIAN_POINT ( 'NONE',  ( 195.9660570498024299, 291.2238279612380438, -17.10029777481811308 ) ) ;
#48063=ORIENTED_EDGE ( 'NONE', *, *, #3118, .T. ) ;
#48067=B_SPLINE_SURFACE_WITH_KNOTS ( 'NONE', 3, 1, ( 
 ( #16366, #665 ),
 ( #17360, #48779 ),
 ( #62439, #15856 ),
 ( #23954, #93406 ),
 ( #40648, #1685 ),
 ( #40144, #41144 ),
 ( #79711, #33064 ),
 ( #70558, #10274 ),
 ( #71586, #47257 ),
 ( #24465, #94900 ),
 ( #16859, #32048 ),
 ( #47746, #71086 ),
 ( #63958, #77689 ),
 ( #78178, #1175 ),
 ( #78683, #32570 ),
 ( #94402, #24956 ),
 ( #2181, #25463 ),
 ( #56351, #87352 ),
 ( #72082, #2683 ),
 ( #64468, #25982 ),
 ( #74582, #65459 ),
 ( #49272, #43132 ),
 ( #95916, #42640 ),
 ( #5161, #36040 ),
 ( #27478, #41652 ),
 ( #26970, #12778 ),
 ( #11292, #58346 ),
 ( #50255, #35049 ),
 ( #73086, #57852 ),
 ( #80209, #81208 ),
 ( #35555, #19876 ),
 ( #72593, #19396 ),
 ( #18377, #10777 ),
 ( #26476, #3199 ) ),
 .UNSPECIFIED., .T., .F., .F.,
 ( 4, 2, 2, 2, 2, 2, 2, 2, 2, 2, 2, 2, 2, 2, 2, 2, 4 ),
 ( 2, 2 ),
 ( 0.000000000000000000, 0.06250000000000000000, 0.1250000000000000000, 0.1875000000000000000, 0.2500000000000000000, 0.3125000000000000000, 0.3750000000000000000, 0.4375000000000000000, 0.5000000000000000000, 0.5625000000000000000, 0.6250000000000000000, 0.6875000000000000000, 0.7500000000000000000, 0.8125000000000000000, 0.8750000000000000000, 0.9375000000000000000, 1.000000000000000000 ),
 ( 0.000000000000000000, 1.000000000000000000 ),
 .UNSPECIFIED. ) ;
#48068=CARTESIAN_POINT ( 'NONE',  ( 164.0723032761492846, 249.9223654822971241, 10.21660028793007058 ) ) ;
#48070=CARTESIAN_POINT ( 'NONE',  ( 207.8018416422513894, 270.7236476996756664, 1.610379135119299754 ) ) ;
#48071=CARTESIAN_POINT ( 'NONE',  ( 86.99453030705913648, 221.0333772461660544, 9.188101187500095079 ) ) ;
#48073=AXIS2_PLACEMENT_3D ( 'NONE', #97578, #80916, #65647 ) ;
#48074=EDGE_LOOP ( 'NONE', ( #51583, #96177, #10935, #57918 ) ) ;
#48075=CARTESIAN_POINT ( 'NONE',  ( 163.3723087697842971, 247.6778559913402091, -10.08585062664141319 ) ) ;
#48078=CYLINDRICAL_SURFACE ( 'NONE', #75698, 17.82106496071139645 ) ;
#48079=CARTESIAN_POINT ( 'NONE',  ( 164.7750468393942072, 284.9269967741507799, 0.5039332410673107443 ) ) ;
#48080=DIRECTION ( 'NONE',  ( -0.5000000000000006661, 0.8660254037844382635, -1.877843081442120958E-16 ) ) ;
#48085=CARTESIAN_POINT ( 'NONE',  ( 160.7116691410181204, 275.5603374970829691, 13.86191725030325905 ) ) ;
#48086=CARTESIAN_POINT ( 'NONE',  ( 159.2651917302844993, 254.7915913763855258, -16.53922207549818424 ) ) ;
#48087=CARTESIAN_POINT ( 'NONE',  ( 155.9304167309410616, 262.0567994629158193, -16.96786909722664660 ) ) ;
#48088=CARTESIAN_POINT ( 'NONE',  ( 174.7346703842556224, 283.9960318526788114, 13.82134370946545943 ) ) ;
#48089=CARTESIAN_POINT ( 'NONE',  ( 198.6444633007815810, 284.5846922512318997, -17.80363864581810418 ) ) ;
#48090=CARTESIAN_POINT ( 'NONE',  ( 195.5147172610062967, 279.6304477706623857, -17.34193691489010902 ) ) ;
#48092=CARTESIAN_POINT ( 'NONE',  ( 8.658876260137789771, 164.2592609112380160, 2.679491924311254714 ) ) ;
#48093=( BOUNDED_CURVE ( )  B_SPLINE_CURVE ( 2, ( #11503, #95634, #27184, #64684, #42356, #26182, #52954, #61544, #61037 ),
 .UNSPECIFIED., .F., .F. ) 
 B_SPLINE_CURVE_WITH_KNOTS ( ( 3, 2, 2, 2, 3 ),
 ( 0.4637096774193548154, 0.4650537634408601906, 0.4677419354838709409, 0.4704301075268817467, 0.4717741935483871218 ),
 .UNSPECIFIED. ) 
 CURVE ( )  GEOMETRIC_REPRESENTATION_ITEM ( )  RATIONAL_B_SPLINE_CURVE ( ( 0.9330127018922194093, 0.9330127018922194093, 1.000000000000000000, 0.8660254037844387076, 1.000000000000000000, 0.8660254037844387076, 1.000000000000000000, 0.9330127018922194093, 0.9330127018922194093 ) ) 
 REPRESENTATION_ITEM ( '' )  );
#48094=CARTESIAN_POINT ( 'NONE',  ( 200.1444820856229967, 283.9865835035790269, 17.93386694781497326 ) ) ;
#48097=CARTESIAN_POINT ( 'NONE',  ( 187.9089654282127526, 266.1749911718636099, -11.87902348831128485 ) ) ;
#48099=CARTESIAN_POINT ( 'NONE',  ( 175.1301202802792432, 290.1368936646978227, -6.315612267206111241 ) ) ;
#48100=CARTESIAN_POINT ( 'NONE',  ( 156.9309300460126906, 272.6596396618500080, 14.48126528928379031 ) ) ;
#48103=CARTESIAN_POINT ( 'NONE',  ( 207.1059763530604698, 271.9289217357780899, 6.370907250589925575 ) ) ;
#48104=CARTESIAN_POINT ( 'NONE',  ( 180.6081384992149594, 267.0382346236909825, -16.05224082202179403 ) ) ;
#48106=CARTESIAN_POINT ( 'NONE',  ( 199.4400349757259789, 281.3072289442092142, -16.75105224125054448 ) ) ;
#48110=CARTESIAN_POINT ( 'NONE',  ( 169.2488921996751401, 273.1503855280286643, 15.96805902338648409 ) ) ;
#48111=( BOUNDED_CURVE ( )  B_SPLINE_CURVE ( 2, ( #40924, #94685, #48557, #80497, #34832, #96191, #2984, #1957, #71871 ),
 .UNSPECIFIED., .F., .T. ) 
 B_SPLINE_CURVE_WITH_KNOTS ( ( 3, 2, 2, 2, 3 ),
 ( 0.5846774193548387455, 0.5860215053763441206, 0.5887096774193548709, 0.5913978494623656212, 0.5927419354838709964 ),
 .UNSPECIFIED. ) 
 CURVE ( )  GEOMETRIC_REPRESENTATION_ITEM ( )  RATIONAL_B_SPLINE_CURVE ( ( 0.9330127018922194093, 0.9330127018922194093, 1.000000000000000000, 0.8660254037844387076, 1.000000000000000000, 0.8660254037844387076, 1.000000000000000000, 0.9330127018922194093, 0.9330127018922194093 ) ) 
 REPRESENTATION_ITEM ( '' )  );
#48112=CARTESIAN_POINT ( 'NONE',  ( 181.2820369676599910, 273.4109893422450455, 17.60600081488427193 ) ) ;
#48113=CARTESIAN_POINT ( 'NONE',  ( 196.4164021072083983, 270.5621661862001019, 13.33908636140236936 ) ) ;
#48114=CARTESIAN_POINT ( 'NONE',  ( 205.8889072768004951, 273.5716727396786041, -9.812782715980612025 ) ) ;
#48116=CARTESIAN_POINT ( 'NONE',  ( 190.5526305594705434, 299.9695577504274979, -4.324655322867677398 ) ) ;
#48117=CARTESIAN_POINT ( 'NONE',  ( -1.610867365518755978, 176.0024278399160949, 9.188101187500095079 ) ) ;
#48120=CARTESIAN_POINT ( 'NONE',  ( 175.0080295257186265, 255.0607892082682895, 9.260279940284284805 ) ) ;
#48123=CARTESIAN_POINT ( 'NONE',  ( 15.76359375002403596, 192.1589784336661637, -6.496448406907676862E-16 ) ) ;
#48125=CARTESIAN_POINT ( 'NONE',  ( 181.7217459927706216, 276.2532386564253670, -17.70126685545563916 ) ) ;
#48128=CARTESIAN_POINT ( 'NONE',  ( 147.2405539530007559, 275.6188749492528132, 0.4306668706573002492 ) ) ;
#48130=CARTESIAN_POINT ( 'NONE',  ( 196.3189437186685211, 290.6126103214480167, 17.40845986800375300 ) ) ;
#48132=CARTESIAN_POINT ( 'NONE',  ( -22.42236680055709641, 157.8615022471902591, 0.000000000000000000 ) ) ;
#48133=CARTESIAN_POINT ( 'NONE',  ( 156.6812872898450735, 261.2670451491295012, 0.000000000000000000 ) ) ;
#48136=CARTESIAN_POINT ( 'NONE',  ( 77.09838585100470709, 201.9865022471901739, 1.119607411625061291E-15 ) ) ;
#48140=CARTESIAN_POINT ( 'NONE',  ( -22.42236680055709641, 157.8615022471902591, 0.000000000000000000 ) ) ;
#48141=CARTESIAN_POINT ( 'NONE',  ( 34.35668405510998724, 181.4548013555409796, -4.594050593750042211 ) ) ;
#48142=CARTESIAN_POINT ( 'NONE',  ( 197.9552487813401456, 287.7784468162186613, 17.26493623863614602 ) ) ;
#48143=CARTESIAN_POINT ( 'NONE',  ( 69.37632600059342280, 210.8615022471902591, -10.00000000000009592 ) ) ;
#48144=CARTESIAN_POINT ( 'NONE',  ( 171.3928239984006723, 250.3015599828365509, -5.796133048607560845 ) ) ;
#48149=DIRECTION ( 'NONE',  ( -0.8660254037844387076, -0.4999999999999998890, -0.000000000000000000 ) ) ;
#48152=CARTESIAN_POINT ( 'NONE',  ( 163.1014434023538513, 248.1470085697407058, 9.692260209037655727 ) ) ;
#48153=CARTESIAN_POINT ( 'NONE',  ( 196.8363552541316324, 289.7164272536036265, -17.80258609350122967 ) ) ;
#48154=CARTESIAN_POINT ( 'NONE',  ( 185.8051906529039172, 267.9722644852660096, -14.39617185440305747 ) ) ;
#48157=CARTESIAN_POINT ( 'NONE',  ( 185.4481162553822173, 290.9827097585334741, 13.29153407209991755 ) ) ;
#48162=ORIENTED_EDGE ( 'NONE', *, *, #28815, .F. ) ;
#48163=CARTESIAN_POINT ( 'NONE',  ( 182.0338464029501040, 278.3680066549227945, 17.69288446120480174 ) ) ;
#48167=CARTESIAN_POINT ( 'NONE',  ( 149.7128599965862463, 271.3367152699035501, 12.33532264622322394 ) ) ;
#48170=CARTESIAN_POINT ( 'NONE',  ( 189.5591655548766425, 274.6138781789617838, -16.86315132615974832 ) ) ;
#48172=ORIENTED_EDGE ( 'NONE', *, *, #52238, .T. ) ;
#48173=CARTESIAN_POINT ( 'NONE',  ( 152.6621968174709991, 266.2283140474973493, -17.02835521334403168 ) ) ;
#48174=CARTESIAN_POINT ( 'NONE',  ( -13.76211276271269668, 162.8615022471902591, 0.000000000000000000 ) ) ;
#48177=FACE_OUTER_BOUND ( 'NONE', #60044, .T. ) ;
#48178=CARTESIAN_POINT ( 'NONE',  ( 100.3364738622893810, 237.9244531367911009, -4.594050593750046652 ) ) ;
#48179=CARTESIAN_POINT ( 'NONE',  ( 196.3174919959537306, 290.6151247789487684, -17.61248417473235151 ) ) ;
#48180=EDGE_CURVE ( 'NONE', #33184, #40534, #79017, .T. ) ;
#48181=CARTESIAN_POINT ( 'NONE',  ( 184.1766470405371194, 288.8506743398048684, -13.13675576434501835 ) ) ;
#48183=CARTESIAN_POINT ( 'NONE',  ( 208.1876422586379647, 270.0554214305024630, 3.377638779759113863 ) ) ;
#48184=VERTEX_POINT ( 'NONE', #79303 ) ;
#48186=CARTESIAN_POINT ( 'NONE',  ( 198.2819808855875863, 287.2125302111982705, 18.53535247371401695 ) ) ;
#48188=CARTESIAN_POINT ( 'NONE',  ( 53.21953955946602122, 201.5333772461660544, 9.188101187500095079 ) ) ;
#48190=CARTESIAN_POINT ( 'NONE',  ( 151.0778907302193943, 268.9724126853576536, 15.84769371787143832 ) ) ;
#48191=CARTESIAN_POINT ( 'NONE',  ( 150.2950809960438221, 270.3282789176094525, 14.12607625385173193 ) ) ;
#48192=CARTESIAN_POINT ( 'NONE',  ( 173.0661364776218818, 271.2294764343828319, 16.42400051025034458 ) ) ;
#48195=CARTESIAN_POINT ( 'NONE',  ( 177.5535686395006962, 288.9327453076302277, 11.22957305193713928 ) ) ;
#48198=ORIENTED_EDGE ( 'NONE', *, *, #46124, .F. ) ;
#48201=B_SPLINE_CURVE_WITH_KNOTS ( 'NONE', 3,
 ( #81677, #90284, #83670, #14233, #5140, #96885, #89774, #89301, #19854, #50722, #43108, #74052, #26977, #3206, #80726, #89803, #19883, #12787, #27955, #18890, #42159, #73095, #90310, #58836, #97878, #35056, #43650, #3687, #41659, #34566, #82215, #43139, #74589, #82712, #20882, #51247, #65468, #81215, #26484, #4160, #96409, #72603, #57859, #88840, #19403, #96914, #89330, #50262, #11789, #11301, #5167, #59330 ),
 .UNSPECIFIED., .F., .F.,
 ( 4, 2, 2, 2, 2, 2, 2, 2, 2, 2, 2, 2, 2, 2, 2, 2, 2, 2, 2, 2, 2, 2, 2, 2, 2, 4 ),
 ( 0.0001359809603122414388, 0.0006282668108888124145, 0.001120552661465383255, 0.001366695586753668675, 0.001612838512041954312, 0.001735909974686074362, 0.001858981437330194629, 0.001982052899974314896, 0.002105124362618435163, 0.002597410213194750132, 0.003089696063771064666, 0.004074267764923540647, 0.005058839466076017928, 0.005551125316652261339, 0.005797268241940383912, 0.005920339704584443898, 0.006043411167228504750, 0.006104946898550515227, 0.006166482629872525704, 0.006289554092516613445, 0.006535697017804746427, 0.006781839943092880275, 0.007027982868381014124, 0.007274125793669147105, 0.007520268718957280087, 0.008012554569533536508 ),
 .UNSPECIFIED. ) ;
#48202=CARTESIAN_POINT ( 'NONE',  ( -22.42236680055709641, 157.8615022471902591, 0.000000000000000000 ) ) ;
#48203=CARTESIAN_POINT ( 'NONE',  ( 192.4743214706506365, 297.2716913909250707, -12.17804856100553046 ) ) ;
#48204=CARTESIAN_POINT ( 'NONE',  ( 149.2511585606875428, 272.1364056148075292, 11.40684181024752242 ) ) ;
#48205=B_SPLINE_CURVE_WITH_KNOTS ( 'NONE', 3,
 ( #855, #62637, #93593, #24160, #1868, #94100, #55045, #86026, #70758, #24652, #86519, #47942, #32752, #34747, #66157, #89039, #49454, #42830, #2379, #48968, #48466, #96103, #41344, #11970, #80409, #19586, #3387, #33258, #34259, #95619, #42340, #79902, #73765, #26167, #71780, #57045, #64159, #33785, #95109, #88026, #4356, #58056, #10467, #72797, #50450, #2889, #72285, #64670, #18576, #10979 ),
 .UNSPECIFIED., .F., .F.,
 ( 4, 2, 2, 2, 2, 2, 2, 2, 2, 2, 2, 2, 2, 2, 2, 2, 2, 2, 2, 2, 2, 2, 2, 2, 4 ),
 ( 0.0001777596983279888224, 0.001185089187328521899, 0.001688753931828796068, 0.001940586304078896181, 0.002066502490203914362, 0.002192418676328932326, 0.002318334862453950290, 0.002444251048578967821, 0.002696083420829005917, 0.003199748165329127213, 0.004207077654329402332, 0.005214407143329677016, 0.005718071887829815660, 0.005969904260079806485, 0.006221736632329797310, 0.006284694725392295234, 0.006347652818454793157, 0.006410610911517290213, 0.006473569004579788136, 0.006725401376829856157, 0.006977233749079924177, 0.007229066121329991330, 0.007480898493580059351, 0.007732730865830127372, 0.008236395610330311118 ),
 .UNSPECIFIED. ) ;
#48207=CARTESIAN_POINT ( 'NONE',  ( 180.8410963975274228, 271.3820433072099263, 16.71430284973371627 ) ) ;
#48213=CARTESIAN_POINT ( 'NONE',  ( 116.7102005222951817, 232.0643266524159856, -9.188101187500093303 ) ) ;
#48214=ORIENTED_EDGE ( 'NONE', *, *, #97235, .T. ) ;
#48215=CARTESIAN_POINT ( 'NONE',  ( 146.8637854207107409, 276.2714571898724216, 0.7988785540157756770 ) ) ;
#48217=CARTESIAN_POINT ( 'NONE',  ( 204.1780753366177237, 277.0001950557890495, 14.05599973203924158 ) ) ;
#48219=CARTESIAN_POINT ( 'NONE',  ( 175.3791991197070672, 252.5596894157395980, 5.239567693004966387 ) ) ;
#48221=CARTESIAN_POINT ( 'NONE',  ( 174.7762878479638857, 265.7456530501560792, -17.06323711782486541 ) ) ;
#48223=CARTESIAN_POINT ( 'NONE',  ( 155.9194312736545385, 273.7031741143842964, -12.76921509093127050 ) ) ;
#48224=CARTESIAN_POINT ( 'NONE',  ( 181.9855612025720575, 260.5135956200978740, 9.640126796794145747 ) ) ;
#48225=CARTESIAN_POINT ( 'NONE',  ( 164.9825360643182535, 244.8888605054729624, -1.157747536866345461 ) ) ;
#48226=CARTESIAN_POINT ( 'NONE',  ( 123.8274129399422918, 251.4869531367911577, 4.594050593750046652 ) ) ;
#48227=CARTESIAN_POINT ( 'NONE',  ( 190.5153763745130675, 294.7680481657044993, -12.25754067625421229 ) ) ;
#48229=CYLINDRICAL_SURFACE ( 'NONE', #33611, 10.00000000000010658 ) ;
#48230=CARTESIAN_POINT ( 'NONE',  ( 133.7124848875370731, 259.5530062829863596, -4.648177544792955347E-16 ) ) ;
#48231=CARTESIAN_POINT ( 'NONE',  ( 53.65289935712325331, 189.5327760586659451, 1.948934522072303157E-15 ) ) ;
#48232=B_SPLINE_CURVE_WITH_KNOTS ( 'NONE', 3,
 ( #56727, #10644, #94764, #57713, #87710, #25327, #49139, #88192, #50130, #2039, #80073, #81082, #11648, #72462, #42508, #82076, #82580, #4523, #67827, #20239, #35424, #98242, #13632, #50612, #89199, #91155, #44506, #75953, #43516, #45007, #6529, #81566, #52112, #65812, #5526, #75435, #60195, #28828, #73937, #51628, #5035, #36410, #74942, #12137, #74455, #42999, #6019, #89678, #13143, #44000 ),
 .UNSPECIFIED., .F., .F.,
 ( 4, 2, 2, 2, 2, 2, 2, 2, 2, 2, 2, 2, 2, 2, 2, 2, 2, 2, 2, 2, 2, 2, 2, 2, 4 ),
 ( 0.002843746976746490841, 0.003047737582608842262, 0.003251728188471194117, 0.003353723491402369611, 0.003455718794333545105, 0.003557714097264720165, 0.003659709400195895659, 0.003863700006058367210, 0.004067690611920839194, 0.004475671823645782296, 0.005291634247095621663, 0.006107596670545461029, 0.006923559093995300395, 0.007739521517445139762, 0.007841516820376355154, 0.007892514471841962850, 0.007943512123307570547, 0.007994509774773178243, 0.008045507426238784204, 0.008147502729170008270, 0.008555483940894892392, 0.008759474546757333585, 0.008963465152619774778, 0.009167455758482215972, 0.009371446364344657165 ),
 .UNSPECIFIED. ) ;
#48234=CARTESIAN_POINT ( 'NONE',  ( 205.2941531242069857, 275.0670916224857478, -13.92605142593109058 ) ) ;
#48235=CARTESIAN_POINT ( 'NONE',  ( 185.9427433571077586, 257.7868782628476083, -2.501399907045548598 ) ) ;
#48237=CARTESIAN_POINT ( 'NONE',  ( 171.6037788498051953, 259.8733260417915290, 15.41710503213636763 ) ) ;
#48239=CARTESIAN_POINT ( 'NONE',  ( 178.8732274734658745, 291.7255955964181453, -6.546936884515894839 ) ) ;
#48240=CARTESIAN_POINT ( 'NONE',  ( 155.5211745099813356, 261.2764194263634749, -17.18163098020766810 ) ) ;
#48242=CARTESIAN_POINT ( 'NONE',  ( 178.9139577745172858, 261.4084931650070871, 12.21660760478297370 ) ) ;
#48244=CARTESIAN_POINT ( 'NONE',  ( 120.6702889753613022, 247.1427522451419065, 10.00000000000009237 ) ) ;
#48245=EDGE_CURVE ( 'NONE', #7074, #18151, #99448, .T. ) ;
#48247=VERTEX_POINT ( 'NONE', #81291 ) ;
#48249=CARTESIAN_POINT ( 'NONE',  ( 147.7978300115112233, 274.6536445020713018, 7.902890709649431855 ) ) ;
#48251=CARTESIAN_POINT ( 'NONE',  ( 24.99226373304320958, 194.4244531367911293, -4.594050593750046652 ) ) ;
#48254=CARTESIAN_POINT ( 'NONE',  ( 31.25085430583858681, 200.3967562850347122, -4.648177544792955347E-16 ) ) ;
#48257=CARTESIAN_POINT ( 'NONE',  ( 57.45043449909725553, 210.6427522451419634, -10.00000000000009415 ) ) ;
#48263=CARTESIAN_POINT ( 'NONE',  ( 161.9103913065419249, 267.1972571684306104, 16.48826679605286216 ) ) ;
#48264=CARTESIAN_POINT ( 'NONE',  ( 29.61132621015795863, 181.2365022471902307, 10.00000000000009592 ) ) ;
#48268=CARTESIAN_POINT ( 'NONE',  ( -12.81524457486244550, 175.6589784336661353, -6.496448406907675876E-16 ) ) ;
#48270=B_SPLINE_CURVE_WITH_KNOTS ( 'NONE', 3,
 ( #62480, #1213, #71124, #55872 ),
 .UNSPECIFIED., .F., .F.,
 ( 4, 4 ),
 ( 0.008820457929765233851, 0.01706750817050696478 ),
 .UNSPECIFIED. ) ;
#48273=CARTESIAN_POINT ( 'NONE',  ( 153.4619471835925708, 264.8431057800031567, 16.95044998314351758 ) ) ;
#48276=CARTESIAN_POINT ( 'NONE',  ( 184.4794126637048066, 258.5029335018122083, -2.309405192791472938 ) ) ;
#48280=CARTESIAN_POINT ( 'NONE',  ( 149.6230451358742926, 271.4922791719315001, -12.72565967355361671 ) ) ;
#48281=CARTESIAN_POINT ( 'NONE',  ( 160.1795347027651815, 282.8633239002924711, 5.491715875156680582 ) ) ;
#48293=CARTESIAN_POINT ( 'NONE',  ( 164.8329445879545290, 245.1479605429143760, -2.955380775890217304 ) ) ;
#48297=VERTEX_POINT ( 'NONE', #12358 ) ;
#48299=VERTEX_POINT ( 'NONE', #88413 ) ;
#48300=CARTESIAN_POINT ( 'NONE',  ( 156.0847645221770392, 276.9562993373755830, -10.16876128128424561 ) ) ;
#48302=ORIENTED_EDGE ( 'NONE', *, *, #23596, .T. ) ;
#48308=EDGE_CURVE ( 'NONE', #42896, #55151, #30528, .T. ) ;
#48309=EDGE_CURVE ( 'NONE', #34164, #71353, #76476, .T. ) ;
#48311=CARTESIAN_POINT ( 'NONE',  ( 173.6791921498279692, 267.2095749298062515, 16.87208145038420781 ) ) ;
#48313=CARTESIAN_POINT ( 'NONE',  ( 151.2057546125658973, 268.7509459446807227, 15.78031848731319187 ) ) ;
#48314=B_SPLINE_SURFACE_WITH_KNOTS ( 'NONE', 3, 1, ( 
 ( #85075, #70333 ),
 ( #24245, #15622 ),
 ( #8054, #69338 ),
 ( #76456, #29842 ),
 ( #45525, #23228 ),
 ( #38927, #22236 ),
 ( #86108, #54616 ),
 ( #7036, #62219 ),
 ( #93171, #85600 ),
 ( #16635, #38423 ),
 ( #8544, #93680 ),
 ( #55122, #46014 ),
 ( #69832, #47531 ),
 ( #78459, #39416 ),
 ( #37424, #62723 ),
 ( #61228, #84094 ),
 ( #53137, #31334 ),
 ( #46521, #37917 ),
 ( #16140, #53626 ),
 ( #100259, #77458 ),
 ( #92193, #7532 ),
 ( #68828, #443 ),
 ( #99257, #47038 ),
 ( #77955, #68332 ),
 ( #945, #60712 ),
 ( #14646, #31821 ),
 ( #91674, #99754 ),
 ( #76930, #30339 ),
 ( #22746, #84581 ),
 ( #15120, #30842 ),
 ( #61727, #92675 ),
 ( #54116, #23722 ),
 ( #24732, #18149 ),
 ( #64239, #71357 ) ),
 .UNSPECIFIED., .T., .F., .F.,
 ( 4, 2, 2, 2, 2, 2, 2, 2, 2, 2, 2, 2, 2, 2, 2, 2, 4 ),
 ( 2, 2 ),
 ( 0.000000000000000000, 0.06250000000000000000, 0.1250000000000000000, 0.1875000000000000000, 0.2500000000000000000, 0.3125000000000000000, 0.3750000000000000000, 0.4375000000000000000, 0.5000000000000000000, 0.5625000000000000000, 0.6250000000000000000, 0.6875000000000000000, 0.7500000000000000000, 0.8125000000000000000, 0.8750000000000000000, 0.9375000000000000000, 1.000000000000000000 ),
 ( 0.000000000000000000, 1.000000000000000000 ),
 .UNSPECIFIED. ) ;
#48315=ORIENTED_EDGE ( 'NONE', *, *, #5426, .F. ) ;
#48316=CARTESIAN_POINT ( 'NONE',  ( 170.6575497776124166, 255.5351817509920522, -11.56051450327723451 ) ) ;
#48318=VERTEX_POINT ( 'NONE', #75644 ) ;
#48325=CARTESIAN_POINT ( 'NONE',  ( -13.35616335646270691, 163.0958772461660544, -9.188101187500095079 ) ) ;
#48327=CARTESIAN_POINT ( 'NONE',  ( 152.6757560589063303, 266.2048287524194166, 16.73757896668104195 ) ) ;
#48334=CARTESIAN_POINT ( 'NONE',  ( 205.7576124508049418, 274.2643565215761328, 10.88614016733041545 ) ) ;
#48336=CARTESIAN_POINT ( 'NONE',  ( 198.2489255580726422, 287.2697837179150042, 18.53597557040773225 ) ) ;
#48339=CARTESIAN_POINT ( 'NONE',  ( 191.0989310468112308, 299.6539374852582114, 5.701794864544876162 ) ) ;
#48341=CARTESIAN_POINT ( 'NONE',  ( 206.1615484827472358, 273.5647187912443314, -9.556459874778100883 ) ) ;
#48343=CARTESIAN_POINT ( 'NONE',  ( 161.4469036912142599, 251.0127554125742222, 12.93933463576739307 ) ) ;
#48344=CARTESIAN_POINT ( 'NONE',  ( 190.8693101975414947, 262.0387244596780079, -0.7334896453799415461 ) ) ;
#48346=CARTESIAN_POINT ( 'NONE',  ( 175.3932935011599170, 269.2958584618301643, -17.65833184418574930 ) ) ;
#48350=CARTESIAN_POINT ( 'NONE',  ( 164.6649740431187183, 245.4388940607451843, -1.430729255012818557 ) ) ;
#48351=CARTESIAN_POINT ( 'NONE',  ( 21.22170510744829741, 176.3927522451418213, -10.00000000000009059 ) ) ;
#48352=CARTESIAN_POINT ( 'NONE',  ( 86.39896429407481548, 226.8149278399160664, 9.188101187500093303 ) ) ;
#48356=CARTESIAN_POINT ( 'NONE',  ( 163.0682440866927720, 248.2045114712421423, 11.63988583931958942 ) ) ;
#48358=CARTESIAN_POINT ( 'NONE',  ( 4.830370123010505168, 173.5958772461660828, -9.188101187500095079 ) ) ;
#48360=CARTESIAN_POINT ( 'NONE',  ( 200.2631011806900005, 283.7811292041749311, 18.23377125296567058 ) ) ;
#48365=CARTESIAN_POINT ( 'NONE',  ( 197.7405121978164289, 265.0121665675080749, -2.992171231212423343 ) ) ;
#48369=CARTESIAN_POINT ( 'NONE',  ( 94.51141663858166453, 213.8262482093457493, 3.021315404115420679E-15 ) ) ;
#48371=CARTESIAN_POINT ( 'NONE',  ( 24.99226373304320958, 194.4244531367911293, -4.594050593750046652 ) ) ;
#48372=CARTESIAN_POINT ( 'NONE',  ( 82.20432729060253507, 208.2677522451417929, -5.000000000000041744 ) ) ;
#48378=CARTESIAN_POINT ( 'NONE',  ( 173.9008529106967558, 272.4049662731551962, -17.79092985220220058 ) ) ;
#48380=CARTESIAN_POINT ( 'NONE',  ( -3.180017766230537557, 156.7202760586659736, -5.415160957724236172E-17 ) ) ;
#48382=CARTESIAN_POINT ( 'NONE',  ( 161.8408514536557163, 250.3304178724980318, -14.12919723462510646 ) ) ;
#48384=CARTESIAN_POINT ( 'NONE',  ( 148.3625667886952044, 273.6754917110858401, -8.960758510948144462 ) ) ;
#48386=CARTESIAN_POINT ( 'NONE',  ( 204.2457645315488719, 276.8829539310449945, 14.53406579917280261 ) ) ;
#48387=CARTESIAN_POINT ( 'NONE',  ( 191.8232488616404225, 298.3993822291468518, -9.342381338555176384 ) ) ;
#48388=CARTESIAN_POINT ( 'NONE',  ( 147.6857584380539095, 274.8477581613835810, 8.112022437684441201 ) ) ;
#48389=VERTEX_POINT ( 'NONE', #68032 ) ;
#48390=CARTESIAN_POINT ( 'NONE',  ( 143.8748646542946972, 242.3262482093457777, 3.021315404115420679E-15 ) ) ;
#48391=CARTESIAN_POINT ( 'NONE',  ( 115.5733686319456126, 237.5333772461660544, 9.188101187500095079 ) ) ;
#48395=CARTESIAN_POINT ( 'NONE',  ( 157.3412122618683497, 258.1240215684019290, 16.75554199904894048 ) ) ;
#48397=CARTESIAN_POINT ( 'NONE',  ( 204.6823371430232896, 272.9704135290961062, -9.754921121218281144 ) ) ;
#48398=CARTESIAN_POINT ( 'NONE',  ( 189.7180314725545713, 261.4674912868679257, -4.463871536367752135 ) ) ;
#48399=CARTESIAN_POINT ( 'NONE',  ( 196.2421909983451940, 290.7455499326673021, -17.31908925000307065 ) ) ;
#48401=CARTESIAN_POINT ( 'NONE',  ( 172.5371125453617935, 290.7831369524994329, -1.769056789171790101 ) ) ;
#48405=CARTESIAN_POINT ( 'NONE',  ( 194.4390729088694627, 266.5749947481197069, -10.67130533956043692 ) ) ;
#48406=VERTEX_POINT ( 'NONE', #99945 ) ;
#48410=CARTESIAN_POINT ( 'NONE',  ( 166.8083734521890449, 257.5796782931630560, -15.79284703031436798 ) ) ;
#48412=CARTESIAN_POINT ( 'NONE',  ( 192.1640094933931096, 297.8091675017319062, 12.36911124822534447 ) ) ;
#48413=EDGE_LOOP ( 'NONE', ( #9831, #1736, #37212, #62057 ) ) ;
#48414=CARTESIAN_POINT ( 'NONE',  ( 162.2577960498091443, 259.6413045848935894, 17.32708210747303212 ) ) ;
#48416=CARTESIAN_POINT ( 'NONE',  ( 173.7814884173456846, 272.7086687150770103, -16.36263896858758926 ) ) ;
#48418=CARTESIAN_POINT ( 'NONE',  ( 167.7924589794888561, 280.8658978846934247, 11.87785029710499707 ) ) ;
#48420=CARTESIAN_POINT ( 'NONE',  ( 112.0822037211656266, 235.5177522451418781, -10.00000000000009592 ) ) ;
#48421=EDGE_LOOP ( 'NONE', ( #21150, #10706, #43897 ) ) ;
#48424=CARTESIAN_POINT ( 'NONE',  ( 188.5582800777447687, 293.2501195853826061, 12.57055310508630441 ) ) ;
#48425=ADVANCED_FACE ( 'NONE', ( #45223 ), #6117, .F. ) ;
#48429=CARTESIAN_POINT ( 'NONE',  ( 154.9792334219179679, 262.2150889255981951, -17.21325849938693153 ) ) ;
#48431=B_SPLINE_CURVE_WITH_KNOTS ( 'NONE', 3,
 ( #33254, #49451, #50448, #97102, #34745, #58537, #48965, #11968, #64155, #27669, #3861, #19584, #89512, #56551, #41340, #25670, #35249, #79899, #72280, #58054, #2885, #66155, #27166, #64667, #33782, #50943, #18572, #73762, #10464, #81892, #40831, #95616, #4354, #42338, #26164, #65646, #57041, #96603, #73268, #88023, #80405, #19081, #10975, #71777 ),
 .UNSPECIFIED., .F., .F.,
 ( 4, 2, 2, 2, 2, 2, 2, 2, 2, 2, 2, 2, 2, 2, 2, 2, 2, 2, 2, 2, 2, 4 ),
 ( 0.002539959018451169899, 0.002952063888789773112, 0.003158116323959076887, 0.003261142541543766288, 0.003364168759128455689, 0.003467194976713144656, 0.003570221194297834057, 0.003776273629467117449, 0.004188378499805755356, 0.005012588240482921884, 0.005836797981160088411, 0.006661007721837254938, 0.007485217462514421466, 0.007588243680099037575, 0.007639756788891345629, 0.007691269897683653683, 0.007742783006475961738, 0.007794296115268268925, 0.007897322332852958759, 0.008309427203191686873, 0.008721532073530414986, 0.009133636943869143099 ),
 .UNSPECIFIED. ) ;
#48432=CARTESIAN_POINT ( 'NONE',  ( 178.2670323550805449, 261.0171416467691756, 12.20401725416360250 ) ) ;
#48433=ORIENTED_EDGE ( 'NONE', *, *, #9358, .F. ) ;
#48438=CARTESIAN_POINT ( 'NONE',  ( 155.6535436963908694, 261.0471492701456668, -17.87366571046205976 ) ) ;
#48440=CARTESIAN_POINT ( 'NONE',  ( 186.0992327883404300, 282.4869563496903311, -17.09887767567498074 ) ) ;
#48442=CARTESIAN_POINT ( 'NONE',  ( 190.7010893771977464, 300.3430194703970528, 2.893802326194260033 ) ) ;
#48444=CARTESIAN_POINT ( 'NONE',  ( 192.5143468344189728, 297.2023654272867361, -12.06830393602581530 ) ) ;
#48445=CARTESIAN_POINT ( 'NONE',  ( 201.2139346379346705, 282.1342373466909521, -16.65315141107179286 ) ) ;
#48446=EDGE_CURVE ( 'NONE', #50800, #69971, #81363, .T. ) ;
#48447=CARTESIAN_POINT ( 'NONE',  ( 55.42424806449747621, 191.2592609112379876, 2.679491924311254714 ) ) ;
#48448=CARTESIAN_POINT ( 'NONE',  ( 157.9540493922656879, 280.9862137877769328, 2.136681455221008274 ) ) ;
#48449=CARTESIAN_POINT ( 'NONE',  ( 118.1982478153434357, 248.2369531367911293, -4.594050593750048428 ) ) ;
#48452=B_SPLINE_CURVE_WITH_KNOTS ( 'NONE', 3,
 ( #89462, #3815, #10923, #3334 ),
 .UNSPECIFIED., .F., .F.,
 ( 4, 4 ),
 ( 0.02347114592376520203, 0.03270413735196970456 ),
 .UNSPECIFIED. ) ;
#48455=AXIS2_PLACEMENT_3D ( 'NONE', #85959, #70174, #70683 ) ;
#48457=VERTEX_POINT ( 'NONE', #41108 ) ;
#48458=CARTESIAN_POINT ( 'NONE',  ( 203.5976937514409428, 276.3333535462982695, 13.44459927773758423 ) ) ;
#48459=CARTESIAN_POINT ( 'NONE',  ( 177.6622601390721172, 253.8114938525349942, 1.357533546181270534 ) ) ;
#48460=CARTESIAN_POINT ( 'NONE',  ( 171.4551282591434926, 287.9808904575950237, -4.629812407206613578 ) ) ;
#48461=CARTESIAN_POINT ( 'NONE',  ( 192.7841353343293065, 296.7350780381442519, 12.22624134270118290 ) ) ;
#48463=CARTESIAN_POINT ( 'NONE',  ( 200.9061540366740246, 282.6673289856585143, -18.13083321883407351 ) ) ;
#48464=CARTESIAN_POINT ( 'NONE',  ( 173.9627241292350277, 288.0875699508326875, -10.01394112541635728 ) ) ;
#48466=CARTESIAN_POINT ( 'NONE',  ( 173.7260703337255734, 281.2931294367136843, 14.01478156921193552 ) ) ;
#48469=CARTESIAN_POINT ( 'NONE',  ( 194.9819925439454664, 292.9282776833073285, -15.33279721168237586 ) ) ;
#48470=CARTESIAN_POINT ( 'NONE',  ( 152.8781682389868877, 273.7668382822124045, 12.04242711029878876 ) ) ;
#48473=CARTESIAN_POINT ( 'NONE',  ( 164.0056900153536503, 278.2207161265373543, 13.42382243837776912 ) ) ;
#48474=CARTESIAN_POINT ( 'NONE',  ( 160.1198091476357206, 278.7610481921645942, 10.47921716862936670 ) ) ;
#48475=CARTESIAN_POINT ( 'NONE',  ( 191.8691792395926825, 298.3198284809228085, -9.399504496626216010 ) ) ;
#48476=CARTESIAN_POINT ( 'NONE',  ( 190.0445576990143195, 301.4801656937889902, 4.140328216824785912 ) ) ;
#48477=CARTESIAN_POINT ( 'NONE',  ( 202.3425522658138505, 280.1794142728863903, 15.86053073629060961 ) ) ;
#48478=CARTESIAN_POINT ( 'NONE',  ( 153.4232513496498598, 270.1086993216917449, 15.21047082690287588 ) ) ;
#48479=CARTESIAN_POINT ( 'NONE',  ( 160.8888607722415998, 281.5892145363297914, 5.729030087643299574 ) ) ;
#48480=CARTESIAN_POINT ( 'NONE',  ( 200.0474988174100872, 267.3471589286638164, 6.283709695813487706 ) ) ;
#48482=CARTESIAN_POINT ( 'NONE',  ( 164.2922989826749358, 280.8236579903888241, -11.68724490838191699 ) ) ;
#48483=EDGE_CURVE ( 'NONE', #81472, #83009, #54291, .T. ) ;
#48484=CARTESIAN_POINT ( 'NONE',  ( 164.1447795365461957, 247.4481183885314692, -7.445268063671048431 ) ) ;
#48486=CARTESIAN_POINT ( 'NONE',  ( 79.60625107924917643, 216.7677522451418497, 10.00000000000009592 ) ) ;
#48487=CARTESIAN_POINT ( 'NONE',  ( 165.1645208897747352, 286.5721895103531551, -2.307774008256134657 ) ) ;
#48488=CARTESIAN_POINT ( 'NONE',  ( 192.0332533962074706, 298.0356437054567778, 11.70630383928353346 ) ) ;
#48492=DIRECTION ( 'NONE',  ( 0.4999999999999998890, -0.8660254037844385966, 0.000000000000000000 ) ) ;
#48493=CARTESIAN_POINT ( 'NONE',  ( -2.124636079309504488, 160.3923013555410080, 4.594050593750050204 ) ) ;
#48494=CARTESIAN_POINT ( 'NONE',  ( 88.91628449352961638, 212.9548013555409796, -4.594050593750042211 ) ) ;
#48495=CARTESIAN_POINT ( 'NONE',  ( 154.8833801513861772, 262.3811116602312268, -17.49275566389638215 ) ) ;
#48496=CARTESIAN_POINT ( 'NONE',  ( 146.9422184197532317, 276.1356072505412840, -5.063317562214876943 ) ) ;
#48498=EDGE_CURVE ( 'NONE', #11106, #41237, #60823, .T. ) ;
#48505=CARTESIAN_POINT ( 'NONE',  ( 163.3473224498206093, 247.7211335670114352, -10.00320358166632850 ) ) ;
#48506=EDGE_CURVE ( 'NONE', #24288, #17132, #95897, .T. ) ;
#48507=CARTESIAN_POINT ( 'NONE',  ( 177.9544788665398869, 290.2550896080946359, 9.853009586926770424 ) ) ;
#48508=EDGE_CURVE ( 'NONE', #89517, #22170, #77742, .T. ) ;
#48509=CARTESIAN_POINT ( 'NONE',  ( 156.6168467568483891, 276.9391697405689001, 11.51099842983860633 ) ) ;
#48511=LINE ( 'NONE', #7493, #99740 ) ;
#48512=CARTESIAN_POINT ( 'NONE',  ( 207.8232941427535536, 270.6864908788566026, -6.505149060073906142 ) ) ;
#48514=CIRCLE ( 'NONE', #21054, 17.82106496071138935 ) ;
#48515=CARTESIAN_POINT ( 'NONE',  ( 44.12627281972940807, 196.2833772461660828, -9.188101187500095079 ) ) ;
#48516=CARTESIAN_POINT ( 'NONE',  ( 175.2923730233647177, 264.8622459507627127, -16.64663378418118356 ) ) ;
#48517=CARTESIAN_POINT ( 'NONE',  ( 73.65258675182887771, 204.1423013555409796, -4.594050593750043987 ) ) ;
#48520=CARTESIAN_POINT ( 'NONE',  ( 166.0372674191381179, 259.3140289393645617, 15.65118634594625568 ) ) ;
#48521=CARTESIAN_POINT ( 'NONE',  ( 197.6960670654980561, 286.6464179233946652, -17.55001329891280548 ) ) ;
#48522=CARTESIAN_POINT ( 'NONE',  ( -22.42236680055709641, 157.8615022471902591, 0.000000000000000000 ) ) ;
#48523=CARTESIAN_POINT ( 'NONE',  ( 176.7533145580467249, 270.1659372832907593, -17.11952259541214261 ) ) ;
#48529=CARTESIAN_POINT ( 'NONE',  ( 78.87554214658000262, 216.3458772461660544, 9.188101187500095079 ) ) ;
#48531=CARTESIAN_POINT ( 'NONE',  ( 169.1442752176298256, 288.3456522438739285, -1.115561018949916328 ) ) ;
#48533=CARTESIAN_POINT ( 'NONE',  ( 154.0399853174704958, 263.8419143634142756, 17.78904985960463847 ) ) ;
#48535=CARTESIAN_POINT ( 'NONE',  ( 123.8637576553643953, 228.9865022471901455, 1.119607411625061291E-15 ) ) ;
#48536=CARTESIAN_POINT ( 'NONE',  ( 13.28313890609088865, 185.1427522451419350, -10.00000000000009592 ) ) ;
#48541=CARTESIAN_POINT ( 'NONE',  ( 163.4260108471723640, 247.5848412648317662, 10.45113099391573108 ) ) ;
#48544=ORIENTED_EDGE ( 'NONE', *, *, #457, .F. ) ;
#48545=CARTESIAN_POINT ( 'NONE',  ( 173.3736115051062256, 251.7241798402721713, -0.2400946007419621497 ) ) ;
#48548=CARTESIAN_POINT ( 'NONE',  ( 170.9648869844012893, 249.9305383690098097, 2.790804180076797092 ) ) ;
#48555=ADVANCED_FACE ( 'NONE', ( #40492 ), #63805, .T. ) ;
#48557=CARTESIAN_POINT ( 'NONE',  ( 76.30452923086889427, 224.8615022471903160, 5.000000000000046185 ) ) ;
#48558=ORIENTED_EDGE ( 'NONE', *, *, #45383, .T. ) ;
#48560=CARTESIAN_POINT ( 'NONE',  ( 183.2720146765236677, 295.8373939426455763, 1.008183942803973832 ) ) ;
#48561=CARTESIAN_POINT ( 'NONE',  ( 163.2164407651493150, 283.9037165268248941, -2.742087382082966318 ) ) ;
#48562=CARTESIAN_POINT ( 'NONE',  ( 148.3625667886952044, 273.6754917110858401, -8.960758510948144462 ) ) ;
#48563=CARTESIAN_POINT ( 'NONE',  ( 163.3939361803663246, 247.6403962173759226, -10.78041711314006790 ) ) ;
#48564=CARTESIAN_POINT ( 'NONE',  ( 193.7706395672514645, 295.0264025848412075, 15.16938698680137065 ) ) ;
#48565=CARTESIAN_POINT ( 'NONE',  ( 186.9117901887487960, 293.6123360585760906, -10.79420932501841790 ) ) ;
#48566=CARTESIAN_POINT ( 'NONE',  ( 204.6149525604204769, 276.2435015074934199, -13.22810747389629960 ) ) ;
#48567=CARTESIAN_POINT ( 'NONE',  ( 164.7274214590310351, 245.3307319635834176, 4.681956269261704051 ) ) ;
#48572=CARTESIAN_POINT ( 'NONE',  ( 79.22710464504368133, 225.7369531367911293, -4.594050593750048428 ) ) ;
#48574=CARTESIAN_POINT ( 'NONE',  ( 190.9061255863007318, 299.9878863388391892, 7.497146773253707153 ) ) ;
#48578=CARTESIAN_POINT ( 'NONE',  ( 164.8309217477579409, 264.8793071284783878, -16.66214786874606446 ) ) ;
#48582=CARTESIAN_POINT ( 'NONE',  ( 146.5157004908022031, 276.8743579738231233, -0.1877253132609108255 ) ) ;
#48585=CARTESIAN_POINT ( 'NONE',  ( 162.7894281526998839, 248.6874348348773651, 10.21811719309735622 ) ) ;
#48586=EDGE_CURVE ( 'NONE', #99538, #80312, #74165, .T. ) ;
#48587=CARTESIAN_POINT ( 'NONE',  ( 103.3411068992554362, 218.2202760586659736, -5.415160957724236172E-17 ) ) ;
#48591=CARTESIAN_POINT ( 'NONE',  ( 113.8142545287344802, 246.5177522451419065, 5.000000000000046185 ) ) ;
#48592=B_SPLINE_SURFACE_WITH_KNOTS ( 'NONE', 3, 1, ( 
 ( #14487, #99589 ),
 ( #29194, #92030 ),
 ( #5394, #44864 ),
 ( #67177, #36774 ),
 ( #82927, #67682 ),
 ( #28183, #43377 ),
 ( #28680, #13503 ),
 ( #30173, #91025 ),
 ( #98101, #44372 ),
 ( #35787, #75804 ),
 ( #6388, #4904 ),
 ( #68171, #99098 ),
 ( #66682, #59055 ),
 ( #45366, #29682 ),
 ( #60555, #39244 ),
 ( #30681, #55447 ),
 ( #31650, #69165 ),
 ( #32669, #94511 ),
 ( #23550, #84413 ),
 ( #31156, #61561 ),
 ( #92508, #62045 ),
 ( #100096, #23054 ),
 ( #54443, #53952 ),
 ( #271, #84908 ),
 ( #24564, #86434 ),
 ( #76772, #62548 ),
 ( #8869, #39734 ),
 ( #15450, #8378 ),
 ( #93511, #7884 ),
 ( #24068, #85940 ),
 ( #46349, #85420 ),
 ( #15967, #77273 ),
 ( #9376, #92998 ),
 ( #46869, #16960 ) ),
 .UNSPECIFIED., .T., .F., .F.,
 ( 4, 2, 2, 2, 2, 2, 2, 2, 2, 2, 2, 2, 2, 2, 2, 2, 4 ),
 ( 2, 2 ),
 ( 0.000000000000000000, 0.06250000000000000000, 0.1250000000000000000, 0.1875000000000000000, 0.2500000000000000000, 0.3125000000000000000, 0.3750000000000000000, 0.4375000000000000000, 0.5000000000000000000, 0.5625000000000000000, 0.6250000000000000000, 0.6875000000000000000, 0.7500000000000000000, 0.8125000000000000000, 0.8750000000000000000, 0.9375000000000000000, 1.000000000000000000 ),
 ( 0.000000000000000000, 1.000000000000000000 ),
 .UNSPECIFIED. ) ;
#48593=CARTESIAN_POINT ( 'NONE',  ( 208.1303168694798273, 270.1547119170880364, -0.9257663487928086132 ) ) ;
#48599=CARTESIAN_POINT ( 'NONE',  ( -6.635445380951201955, 173.6427522451419065, 10.00000000000009237 ) ) ;
#48602=CARTESIAN_POINT ( 'NONE',  ( 157.2470923712064348, 258.2870420010311250, 16.90933983342926439 ) ) ;
#48603=CARTESIAN_POINT ( 'NONE',  ( 158.9004676769321236, 274.8003366604523876, 12.92727430671328470 ) ) ;
#48605=CARTESIAN_POINT ( 'NONE',  ( 159.6288139302610887, 254.1617792512662675, -15.32287760493869477 ) ) ;
#48607=CARTESIAN_POINT ( 'NONE',  ( 174.9634400046559790, 284.2171181662870367, 13.92180131362537310 ) ) ;
#48608=CARTESIAN_POINT ( 'NONE',  ( 198.9875272090999374, 285.4391185361790804, -17.09544516096110911 ) ) ;
#48610=ORIENTED_EDGE ( 'NONE', *, *, #28692, .F. ) ;
#48611=CARTESIAN_POINT ( 'NONE',  ( 203.5838568433318301, 277.5370308791458456, -14.27138230751178050 ) ) ;
#48613=CARTESIAN_POINT ( 'NONE',  ( 161.5504728662519369, 250.8333683393111926, 12.94300825113363373 ) ) ;
#48615=CARTESIAN_POINT ( 'NONE',  ( 169.0039380441634478, 250.7158015086602347, 6.952515250780078482 ) ) ;
#48617=CARTESIAN_POINT ( 'NONE',  ( 176.4148488556422762, 290.5001664222085651, -6.184015662434656946 ) ) ;
#48619=EDGE_LOOP ( 'NONE', ( #5203, #8095, #47407, #21770 ) ) ;
#48623=CARTESIAN_POINT ( 'NONE',  ( 164.5867587387928950, 245.5743669417666126, -3.022048486790635202 ) ) ;
#48624=CARTESIAN_POINT ( 'NONE',  ( 180.6308739683319402, 266.9664207081152085, -14.83175007465150408 ) ) ;
#48628=CARTESIAN_POINT ( 'NONE',  ( 189.3423859142968695, 300.6963629005612120, 0.4146017780601669589 ) ) ;
#48629=CARTESIAN_POINT ( 'NONE',  ( 168.7143801906630358, 273.0201647186528362, 15.94736956477383139 ) ) ;
#48631=B_SPLINE_CURVE_WITH_KNOTS ( 'NONE', 3,
 ( #6996, #901, #92157, #1414, #99715, #77411, #55083, #62177, #76424, #32295, #39869, #8504 ),
 .UNSPECIFIED., .F., .F.,
 ( 4, 2, 2, 2, 2, 4 ),
 ( 0.000000000000000000, 0.0004508590478066377321, 0.0009017180956132754641, 0.001352577143419913088, 0.001578006667323285242, 0.001803436191226657397 ),
 .UNSPECIFIED. ) ;
#48633=CARTESIAN_POINT ( 'NONE',  ( 188.2908577371792092, 260.7054629446816421, 3.471952975698951338 ) ) ;
#48634=CARTESIAN_POINT ( 'NONE',  ( 161.4143265314674522, 251.0691807084224365, -12.94469757303959234 ) ) ;
#48635=CARTESIAN_POINT ( 'NONE',  ( 0.4734401320438119676, 161.8923013555410080, 4.594050593750050204 ) ) ;
#48637=ORIENTED_EDGE ( 'NONE', *, *, #50435, .T. ) ;
#48638=CARTESIAN_POINT ( 'NONE',  ( 178.8556401556461140, 256.8010837051114663, 8.596802396966896964 ) ) ;
#48641=CARTESIAN_POINT ( 'NONE',  ( 17.30628827445631401, 189.9869531367911293, 4.594050593750046652 ) ) ;
#48642=CARTESIAN_POINT ( 'NONE',  ( 161.1990332043106946, 251.4420796895884394, 14.26998817770995487 ) ) ;
#48645=CARTESIAN_POINT ( 'NONE',  ( 181.4912298780635922, 293.8245865419322627, 6.251483007042555329 ) ) ;
#48646=CARTESIAN_POINT ( 'NONE',  ( 173.6199058471797230, 272.8469020441871180, -16.35875967547425347 ) ) ;
#48647=CARTESIAN_POINT ( 'NONE',  ( 149.7585222076137654, 271.2576260004179289, 12.47083832704270989 ) ) ;
#48654=CARTESIAN_POINT ( 'NONE',  ( 85.75863988884901801, 226.9865022471902876, 10.00000000000009237 ) ) ;
#48656=CARTESIAN_POINT ( 'NONE',  ( 203.4484836655096274, 270.1063680826336508, 6.027198966828741789 ) ) ;
#48657=CARTESIAN_POINT ( 'NONE',  ( 51.05482314576993730, 188.0327760586659451, 1.948934522072303157E-15 ) ) ;
#48658=CARTESIAN_POINT ( 'NONE',  ( 198.2819808855875863, 287.2125302111982705, 18.53535247371401695 ) ) ;
#48659=EDGE_LOOP ( 'NONE', ( #58390, #40890, #18534 ) ) ;
#48660=CARTESIAN_POINT ( 'NONE',  ( 162.8796071693688532, 263.4516756011302618, 17.10221866870684337 ) ) ;
#48666=CARTESIAN_POINT ( 'NONE',  ( -22.42236680055709641, 157.8615022471902591, 0.000000000000000000 ) ) ;
#48670=CARTESIAN_POINT ( 'NONE',  ( 163.2919429874875448, 247.8170536094679903, 9.876785378511263147 ) ) ;
#48671=CARTESIAN_POINT ( 'NONE',  ( 196.4242782546697015, 290.4301655533025155, -16.42402868779123537 ) ) ;
#48676=CARTESIAN_POINT ( 'NONE',  ( 23.90999230191042102, 174.6115022471901739, -5.000000000000041744 ) ) ;
#48677=DIRECTION ( 'NONE',  ( -0.2588190451024967587, -0.9659258262890746405, 0.000000000000000000 ) ) ;
#48680=CARTESIAN_POINT ( 'NONE',  ( 190.7851866479434761, 300.1973587246873194, 7.931162401707728016 ) ) ;
#48681=CARTESIAN_POINT ( 'NONE',  ( 177.9642817169934688, 254.8723555480702601, -7.199370876740468717 ) ) ;
#48682=CARTESIAN_POINT ( 'NONE',  ( 190.0601721553029222, 300.2863949309033842, 3.228815124723532382 ) ) ;
#48684=ORIENTED_EDGE ( 'NONE', *, *, #46220, .T. ) ;
#48687=ORIENTED_EDGE ( 'NONE', *, *, #99963, .T. ) ;
#48688=CARTESIAN_POINT ( 'NONE',  ( 153.1983976505312626, 265.2995869615763809, -17.69657798691567763 ) ) ;
#48689=CARTESIAN_POINT ( 'NONE',  ( 170.4745685060332221, 252.4510253584002442, 10.32956013645375570 ) ) ;
#48693=CARTESIAN_POINT ( 'NONE',  ( 88.83448719433606300, 234.3464784336661637, 1.353441290958777525E-15 ) ) ;
#48694=ADVANCED_FACE ( 'NONE', ( #11130 ), #95262, .T. ) ;
#48695=CARTESIAN_POINT ( 'NONE',  ( 200.4958402305064737, 266.0993451409080421, 1.904533336957719536 ) ) ;
#48696=ORIENTED_EDGE ( 'NONE', *, *, #97601, .T. ) ;
#48697=CARTESIAN_POINT ( 'NONE',  ( 208.3135187673106543, 269.8373969220020285, 2.829653198597726682 ) ) ;
#48698=ORIENTED_EDGE ( 'NONE', *, *, #32566, .F. ) ;
#48700=CARTESIAN_POINT ( 'NONE',  ( 198.1300353965528984, 287.4757075181870505, 18.48278456664528946 ) ) ;
#48702=CARTESIAN_POINT ( 'NONE',  ( 59.20026718252854891, 214.1744531367911293, 4.594050593750047540 ) ) ;
#48703=EDGE_CURVE ( 'NONE', #19180, #57417, #56704, .T. ) ;
#48705=CARTESIAN_POINT ( 'NONE',  ( 151.3560786774222322, 268.4905770267490652, 15.54402364351346932 ) ) ;
#48706=CARTESIAN_POINT ( 'NONE',  ( 182.4179874479192165, 295.3930394561857042, 6.267308984944027550 ) ) ;
#48707=CARTESIAN_POINT ( 'NONE',  ( 173.0033714575370425, 271.2342936761517649, 16.42547438483588351 ) ) ;
#48713=CARTESIAN_POINT ( 'NONE',  ( 178.0374733479650615, 288.7981423944819994, 10.93213786509874907 ) ) ;
#48715=EDGE_LOOP ( 'NONE', ( #30871, #30567, #46562, #29530 ) ) ;
#48716=CARTESIAN_POINT ( 'NONE',  ( 172.1715872173708135, 258.5563651535738927, -14.06291902901496371 ) ) ;
#48717=CARTESIAN_POINT ( 'NONE',  ( 173.8466962506738867, 278.0501108023409529, -16.19608603001420732 ) ) ;
#48718=CARTESIAN_POINT ( 'NONE',  ( 207.2337123599961899, 271.7076764818092443, -5.443417788256701861 ) ) ;
#48719=CARTESIAN_POINT ( 'NONE',  ( 206.4767859350078254, 270.5991797036530784, 2.338462165877995158 ) ) ;
#48721=CARTESIAN_POINT ( 'NONE',  ( 190.3572031550745294, 300.9386478791372497, 3.093832330100951378 ) ) ;
#48722=CARTESIAN_POINT ( 'NONE',  ( 180.9066661141190764, 271.3944185450963573, 16.82689088922535348 ) ) ;
#48723=CARTESIAN_POINT ( 'NONE',  ( 164.8849641302980444, 245.0578600525887794, 2.884140591399200648 ) ) ;
#48725=CARTESIAN_POINT ( 'NONE',  ( 164.7391251265351571, 254.6380307246101040, 14.05658276553760722 ) ) ;
#48726=DIRECTION ( 'NONE',  ( 0.4999999999999998890, -0.8660254037844385966, 0.000000000000000000 ) ) ;
#48727=CARTESIAN_POINT ( 'NONE',  ( 112.7044859340271472, 242.0024278399160949, 9.188101187500095079 ) ) ;
#48729=CARTESIAN_POINT ( 'NONE',  ( 149.0000156265528517, 272.5713979366907438, -11.96939414408693025 ) ) ;
#48731=CARTESIAN_POINT ( 'NONE',  ( 155.0619429961492983, 262.0718317407570339, -17.08853361476647592 ) ) ;
#48732=CARTESIAN_POINT ( 'NONE',  ( 183.2273280905530441, 284.5979244485508843, -14.99588714064362094 ) ) ;
#48734=AXIS2_PLACEMENT_3D ( 'NONE', #52490, #61581, #31180 ) ;
#48735=CARTESIAN_POINT ( 'NONE',  ( 176.9774428127479950, 254.7512675880996369, 4.897130350530210841 ) ) ;
#48739=CARTESIAN_POINT ( 'NONE',  ( 154.8737640171889609, 273.3615094271205521, -13.02948580469064943 ) ) ;
#48742=CARTESIAN_POINT ( 'NONE',  ( 205.9736828131439097, 273.8901116759951719, -10.08879389214638778 ) ) ;
#48743=CARTESIAN_POINT ( 'NONE',  ( 143.0428722300570143, 244.2048013555409511, 4.594050593750051981 ) ) ;
#48744=CARTESIAN_POINT ( 'NONE',  ( 192.3947792546893254, 295.6933971515595090, -12.11733834305915103 ) ) ;
#48745=CARTESIAN_POINT ( 'NONE',  ( 185.6688052473205630, 297.0996414484710044, 4.161359448325653965 ) ) ;
#48746=EDGE_CURVE ( 'NONE', #36428, #90703, #73418, .T. ) ;
#48748=CARTESIAN_POINT ( 'NONE',  ( 58.87550765610937731, 213.9869531367911009, 4.594050593750046652 ) ) ;
#48750=CARTESIAN_POINT ( 'NONE',  ( 171.1295603993285965, 249.6517061031812545, 4.344809613321301889 ) ) ;
#48751=ADVANCED_FACE ( 'NONE', ( #80049 ), #26282, .F. ) ;
#48753=CARTESIAN_POINT ( 'NONE',  ( 171.1201963583744146, 259.8845004021682712, 14.96928189076699844 ) ) ;
#48754=CARTESIAN_POINT ( 'NONE',  ( 152.3741921479031589, 278.3847345969097660, -1.620820812214976758 ) ) ;
#48756=CARTESIAN_POINT ( 'NONE',  ( 155.5322964227545413, 261.2571557083629159, -18.35853982030605280 ) ) ;
#48758=CARTESIAN_POINT ( 'NONE',  ( 126.3716228836088646, 243.7677522451418497, 10.00000000000009592 ) ) ;
#48760=ORIENTED_EDGE ( 'NONE', *, *, #56597, .T. ) ;
#48761=CARTESIAN_POINT ( 'NONE',  ( 190.1063449786324213, 301.3731469862293011, 0.2163967485516588019 ) ) ;
#48763=CARTESIAN_POINT ( 'NONE',  ( 48.29419362332453858, 192.5643266524160140, 9.188101187500095079 ) ) ;
#48767=CARTESIAN_POINT ( 'NONE',  ( 147.5177358149801421, 275.1387818813681179, 4.867883209065928085 ) ) ;
#48769=CARTESIAN_POINT ( 'NONE',  ( 198.1468175574237591, 277.6623963789502909, -16.51117061083609983 ) ) ;
#48770=CARTESIAN_POINT ( 'NONE',  ( 58.82164138842265544, 204.7677522451418781, 10.00000000000009592 ) ) ;
#48772=CARTESIAN_POINT ( 'NONE',  ( 180.9078741482798307, 256.3374541303720662, 1.332084592654648070 ) ) ;
#48773=CARTESIAN_POINT ( 'NONE',  ( 205.3943609285979051, 274.8935266139653777, -13.14270440534009943 ) ) ;
#48776=EDGE_CURVE ( 'NONE', #43534, #75541, #7552, .T. ) ;
#48777=CARTESIAN_POINT ( 'NONE',  ( 38.27158024800235836, 186.2365022471901739, -10.00000000000009059 ) ) ;
#48778=CARTESIAN_POINT ( 'NONE',  ( 184.8129517241381734, 294.4172780608702737, 9.971149335153635107 ) ) ;
#48779=CARTESIAN_POINT ( 'NONE',  ( 163.0683798854284703, 248.2042762609320903, 11.26611642476872710 ) ) ;
#48780=CARTESIAN_POINT ( 'NONE',  ( 9.864316330390064280, 170.3768266524160140, -9.188101187500091527 ) ) ;
#48784=ADVANCED_FACE ( 'NONE', ( #30670 ), #61550, .F. ) ;
#48785=CARTESIAN_POINT ( 'NONE',  ( 192.6773196027083372, 296.9200883123592689, 11.15745042875121484 ) ) ;
#48787=CARTESIAN_POINT ( 'NONE',  ( 155.6179570493757183, 261.5041650582481338, -17.00304691045595362 ) ) ;
#48791=CARTESIAN_POINT ( 'NONE',  ( 75.43850382708453139, 204.3615022471901739, 5.000000000000051514 ) ) ;
#48792=CARTESIAN_POINT ( 'NONE',  ( 88.40853095561152486, 233.3967562850347122, -4.648177544792955347E-16 ) ) ;
#48794=CARTESIAN_POINT ( 'NONE',  ( 168.4882224088831890, 287.4185086114543424, 0.5096248658197195525 ) ) ;
#48797=CARTESIAN_POINT ( 'NONE',  ( 152.8006295377938386, 275.0191557585933424, 10.80676033415724646 ) ) ;
#48799=ORIENTED_EDGE ( 'NONE', *, *, #4660, .T. ) ;
#48801=CARTESIAN_POINT ( 'NONE',  ( 207.6900289502458179, 270.9173129631602706, 7.178327969100043227 ) ) ;
#48802=CARTESIAN_POINT ( 'NONE',  ( 102.3574601280508176, 223.2365022471902023, 10.00000000000009948 ) ) ;
#48805=CARTESIAN_POINT ( 'NONE',  ( 155.0303156110108489, 262.1266119787277944, 17.11986653161320859 ) ) ;
#48808=CARTESIAN_POINT ( 'NONE',  ( 198.2505066714982149, 285.2670451491296149, 0.000000000000000000 ) ) ;
#48811=CARTESIAN_POINT ( 'NONE',  ( 192.7874605187217014, 292.5376213369709149, 15.36506066506490598 ) ) ;
#48812=CARTESIAN_POINT ( 'NONE',  ( 155.3625719195318027, 262.1439356272904888, -17.05869219998719899 ) ) ;
#48818=ORIENTED_EDGE ( 'NONE', *, *, #60201, .F. ) ;
#48819=CARTESIAN_POINT ( 'NONE',  ( 200.8769374536528858, 282.7179335918746688, 17.26928237494566787 ) ) ;
#48820=CARTESIAN_POINT ( 'NONE',  ( 169.0831179322903495, 276.3545926343148267, -16.16093963830661551 ) ) ;
#48821=CARTESIAN_POINT ( 'NONE',  ( 111.7912168577913974, 246.8967562850347122, -4.648177544792955347E-16 ) ) ;
#48824=CARTESIAN_POINT ( 'NONE',  ( 171.8094870316595291, 256.2585101260063993, -11.60869940165414427 ) ) ;
#48829=CARTESIAN_POINT ( 'NONE',  ( 160.2388368888874197, 268.7474976419025552, -16.58833657477884671 ) ) ;
#48833=VERTEX_POINT ( 'NONE', #44852 ) ;
#48835=CARTESIAN_POINT ( 'NONE',  ( 194.0772601196179039, 294.4953202094977769, 14.03104165446852214 ) ) ;
#48836=CARTESIAN_POINT ( 'NONE',  ( 190.8422792407884003, 275.9516057710682162, 17.28259784732214399 ) ) ;
#48838=EDGE_CURVE ( 'NONE', #16838, #35245, #6678, .T. ) ;
#48841=LINE ( 'NONE', #63521, #98210 ) ;
#48843=CARTESIAN_POINT ( 'NONE',  ( 185.4203654054929871, 257.3861754496879257, 1.843076797948306034 ) ) ;
#48845=CARTESIAN_POINT ( 'NONE',  ( 164.4261001824251878, 245.8526357240660900, 1.583002802772015549 ) ) ;
#48847=CARTESIAN_POINT ( 'NONE',  ( 197.8822014719394531, 287.9049684674569676, 17.88172308374019792 ) ) ;
#48850=CARTESIAN_POINT ( 'NONE',  ( 171.4323342072972025, 259.3649984363102021, -13.88167851551672349 ) ) ;
#48854=CARTESIAN_POINT ( 'NONE',  ( 161.7587802986029999, 250.4725692828850754, 14.33336164792646450 ) ) ;
#48855=CARTESIAN_POINT ( 'NONE',  ( 103.9969882237314351, 242.3967562850347122, -4.648177544792955347E-16 ) ) ;
#48860=CARTESIAN_POINT ( 'NONE',  ( 52.03546399666511491, 212.3967562850347122, -4.648177544792955347E-16 ) ) ;
#48861=CARTESIAN_POINT ( 'NONE',  ( -1.617403181491035902, 158.3262482093458061, 3.021315404115420679E-15 ) ) ;
#48862=CARTESIAN_POINT ( 'NONE',  ( 21.14953632379956616, 183.0177522451418497, -10.00000000000009592 ) ) ;
#48863=CARTESIAN_POINT ( 'NONE',  ( 100.4447270377624477, 237.9869531367911293, 4.594050593750046652 ) ) ;
#48865=CARTESIAN_POINT ( 'NONE',  ( 95.19470834736908671, 225.7677522451418497, 10.00000000000009592 ) ) ;
#48866=CARTESIAN_POINT ( 'NONE',  ( 167.3689703329816325, 278.5095797815824312, -13.36534151890726285 ) ) ;
#48867=CARTESIAN_POINT ( 'NONE',  ( 23.53136650780448491, 175.2048013555409796, 4.594050593750051981 ) ) ;
#48868=CARTESIAN_POINT ( 'NONE',  ( 200.6800100461949228, 283.0590218669948399, 18.32402613046234308 ) ) ;
#48869=VERTEX_POINT ( 'NONE', #25568 ) ;
#48870=ORIENTED_EDGE ( 'NONE', *, *, #59504, .F. ) ;
#48871=CARTESIAN_POINT ( 'NONE',  ( 201.0556664636881408, 267.5442616503679005, -3.613160940470883098 ) ) ;
#48874=CYLINDRICAL_SURFACE ( 'NONE', #33727, 14.82106496071141066 ) ;
#48875=CARTESIAN_POINT ( 'NONE',  ( 161.8882824960653579, 250.2482648971885340, -13.83574485983625557 ) ) ;
#48876=CARTESIAN_POINT ( 'NONE',  ( 184.9465927238675818, 285.7743050737326485, 15.21868303762837016 ) ) ;
#48878=CARTESIAN_POINT ( 'NONE',  ( 38.76791418169571557, 187.0643266524159856, -9.188101187500093303 ) ) ;
#48881=CARTESIAN_POINT ( 'NONE',  ( -6.833909532437232315, 176.8615022471903160, 5.000000000000046185 ) ) ;
#48883=CARTESIAN_POINT ( 'NONE',  ( -2.801305199957352166, 163.0643266524159571, -9.188101187500093303 ) ) ;
#48885=CARTESIAN_POINT ( 'NONE',  ( 198.8533049117289977, 286.2229679703367538, -18.60939981449148561 ) ) ;
#48886=CARTESIAN_POINT ( 'NONE',  ( 186.6343157368956156, 282.6707309082632378, 16.18028840507778199 ) ) ;
#48887=CARTESIAN_POINT ( 'NONE',  ( 193.1569697810063531, 296.0893098336876506, -13.02398914535779539 ) ) ;
#48889=CARTESIAN_POINT ( 'NONE',  ( 204.1780753366177237, 277.0001950557890495, 14.05599973203924158 ) ) ;
#48890=CARTESIAN_POINT ( 'NONE',  ( 191.8210230231139803, 298.4032374945642232, -8.800268167321144475 ) ) ;
#48891=CARTESIAN_POINT ( 'NONE',  ( 164.2578067403839555, 246.1441285162624126, -2.322300236470859591 ) ) ;
#48892=ORIENTED_EDGE ( 'NONE', *, *, #11399, .F. ) ;
#48893=CARTESIAN_POINT ( 'NONE',  ( -8.565960340006073537, 165.8615022471902591, -10.00000000000009592 ) ) ;
#48894=CARTESIAN_POINT ( 'NONE',  ( 142.1946287021350201, 246.2365022471901739, -10.00000000000009237 ) ) ;
#48895=CARTESIAN_POINT ( 'NONE',  ( 112.9752924205922824, 236.0333772461660544, 9.188101187500095079 ) ) ;
#48898=CARTESIAN_POINT ( 'NONE',  ( 151.3011447763744570, 269.1990464485573966, 14.21186556778774168 ) ) ;
#48899=CARTESIAN_POINT ( 'NONE',  ( 195.7291850945597957, 291.6341022226063160, 17.08310330964873813 ) ) ;
#48900=CARTESIAN_POINT ( 'NONE',  ( 150.2076754159204484, 245.9824982072973683, 3.021315404115420679E-15 ) ) ;
#48901=CARTESIAN_POINT ( 'NONE',  ( 150.7880176790500855, 269.4744875377281232, -15.26825497096394280 ) ) ;
#48902=B_SPLINE_CURVE_WITH_KNOTS ( 'NONE', 3,
 ( #27926, #49737, #11265, #27449 ),
 .UNSPECIFIED., .F., .F.,
 ( 4, 4 ),
 ( 0.003021277710772510023, 0.003024111843000437151 ),
 .UNSPECIFIED. ) ;
#48904=CARTESIAN_POINT ( 'NONE',  ( 192.9053747558651821, 263.8457269808281467, -4.439418679438619009 ) ) ;
#48905=CARTESIAN_POINT ( 'NONE',  ( 148.9322735291567597, 272.6887306911919495, -12.40988026045598858 ) ) ;
#48906=CARTESIAN_POINT ( 'NONE',  ( 184.6885808911535207, 260.6528513612950064, 10.31057805081157852 ) ) ;
#48907=CARTESIAN_POINT ( 'NONE',  ( 173.9194055806650283, 290.1763249296482172, -1.066906480392311174 ) ) ;
#48912=CARTESIAN_POINT ( 'NONE',  ( 175.7290542241515539, 278.6131925542825343, 15.45880334531811151 ) ) ;
#48913=CARTESIAN_POINT ( 'NONE',  ( 165.6255258425915429, 269.1894970381998178, -17.38843227986124518 ) ) ;
#48914=B_SPLINE_SURFACE_WITH_KNOTS ( 'NONE', 3, 1, ( 
 ( #40726, #24535 ),
 ( #94479, #86401 ),
 ( #2771, #65047 ),
 ( #16933, #73167 ),
 ( #55913, #78758 ),
 ( #95510, #41225 ),
 ( #72166, #48350 ),
 ( #95996, #41734 ),
 ( #79299, #26557 ),
 ( #71671, #33144 ),
 ( #26057, #87918 ),
 ( #18461, #72678 ),
 ( #43220, #28032 ),
 ( #20962, #59408 ),
 ( #67025, #11860 ),
 ( #96990, #89877 ),
 ( #44708, #19953 ),
 ( #97952, #43722 ),
 ( #36122, #58426 ),
 ( #51845, #90887 ),
 ( #27561, #65537 ),
 ( #88919, #12863 ),
 ( #28524, #5729 ),
 ( #50829, #21435 ),
 ( #52322, #82785 ),
 ( #74665, #57936 ),
 ( #74162, #29048 ),
 ( #4753, #81779 ),
 ( #35133, #42717 ),
 ( #20452, #5242 ),
 ( #51325, #19479 ),
 ( #83264, #97465 ),
 ( #50336, #82292 ),
 ( #90387, #13350 ) ),
 .UNSPECIFIED., .T., .F., .F.,
 ( 4, 2, 2, 2, 2, 2, 2, 2, 2, 2, 2, 2, 2, 2, 2, 2, 4 ),
 ( 2, 2 ),
 ( 0.000000000000000000, 0.06250000000000000000, 0.1250000000000000000, 0.1875000000000000000, 0.2500000000000000000, 0.3125000000000000000, 0.3750000000000000000, 0.4375000000000000000, 0.5000000000000000000, 0.5625000000000000000, 0.6250000000000000000, 0.6875000000000000000, 0.7500000000000000000, 0.8125000000000000000, 0.8750000000000000000, 0.9375000000000000000, 1.000000000000000000 ),
 ( 0.000000000000000000, 1.000000000000000000 ),
 .UNSPECIFIED. ) ;
#48916=CARTESIAN_POINT ( 'NONE',  ( 156.6493444904068895, 261.1156140128878178, 17.71731464056091454 ) ) ;
#48918=CARTESIAN_POINT ( 'NONE',  ( 153.4619471835925708, 264.8431057800031567, 16.95044998314351758 ) ) ;
#48922=CARTESIAN_POINT ( 'NONE',  ( 195.2858898497755433, 290.2585894125917321, -16.56900025010267896 ) ) ;
#48923=ORIENTED_EDGE ( 'NONE', *, *, #87995, .F. ) ;
#48925=CARTESIAN_POINT ( 'NONE',  ( 147.8505793332463725, 274.5622799967613332, -9.317516487097901035 ) ) ;
#48928=CYLINDRICAL_SURFACE ( 'NONE', #11907, 17.82106496071139645 ) ;
#48929=CARTESIAN_POINT ( 'NONE',  ( 188.5410240070633563, 293.7196559869043426, 13.01390607220156248 ) ) ;
#48930=CARTESIAN_POINT ( 'NONE',  ( 150.7254409736883645, 269.5828735707850683, 14.54962197351449049 ) ) ;
#48934=CARTESIAN_POINT ( 'NONE',  ( 155.6048174803203210, 261.1315455520403361, -17.38645169541727498 ) ) ;
#48936=ORIENTED_EDGE ( 'NONE', *, *, #53380, .T. ) ;
#48942=ADVANCED_FACE ( 'NONE', ( #39725 ), #73219, .F. ) ;
#48943=DIRECTION ( 'NONE',  ( 0.4999999999999992784, -0.8660254037844390407, 0.000000000000000000 ) ) ;
#48946=CARTESIAN_POINT ( 'NONE',  ( 186.1983351278354633, 282.4945498714998280, -16.89931508121779657 ) ) ;
#48948=CARTESIAN_POINT ( 'NONE',  ( 147.8889855101223532, 274.4957585470872914, -6.229723215998690833 ) ) ;
#48949=CARTESIAN_POINT ( 'NONE',  ( 161.7379161894558024, 277.5265442474504312, -13.23162672871571033 ) ) ;
#48950=CARTESIAN_POINT ( 'NONE',  ( 193.0142717932987182, 296.3364699985351081, -13.30037542329744937 ) ) ;
#48952=ADVANCED_FACE ( 'NONE', ( #89894 ), #3773, .T. ) ;
#48954=CARTESIAN_POINT ( 'NONE',  ( 157.9162940790990604, 280.9685295036878756, 2.104535951830800222 ) ) ;
#48955=CARTESIAN_POINT ( 'NONE',  ( 128.9971094863694532, 233.0327760586659451, 1.948934522072303157E-15 ) ) ;
#48956=ORIENTED_EDGE ( 'NONE', *, *, #23587, .T. ) ;
#48961=CARTESIAN_POINT ( 'NONE',  ( 203.5231681107415511, 276.4626886777189156, 14.22114972371920416 ) ) ;
#48962=CARTESIAN_POINT ( 'NONE',  ( 180.1475770660277647, 255.8711682511834340, 1.311453321043420051 ) ) ;
#48963=CARTESIAN_POINT ( 'NONE',  ( 171.1366801964148578, 287.7825823751429652, -4.654478872985349014 ) ) ;
#48965=CARTESIAN_POINT ( 'NONE',  ( 156.7136391252028602, 279.5216684332963837, 7.468001664478725488 ) ) ;
#48968=CARTESIAN_POINT ( 'NONE',  ( 174.0035762054535269, 281.4834410953270094, 14.05709486446668244 ) ) ;
#48969=CARTESIAN_POINT ( 'NONE',  ( 177.2141887958173072, 256.0616080229310114, -7.313315655081018996 ) ) ;
#48975=B_SPLINE_CURVE_WITH_KNOTS ( 'NONE', 3,
 ( #58029, #19563, #50422, #42802 ),
 .UNSPECIFIED., .F., .F.,
 ( 4, 4 ),
 ( 0.01114209618785225175, 0.01956799148668745755 ),
 .UNSPECIFIED. ) ;
#48976=CARTESIAN_POINT ( 'NONE',  ( 156.6716504413620896, 276.8562130845049296, 9.991782109645525267 ) ) ;
#48977=CARTESIAN_POINT ( 'NONE',  ( 192.2053377076082086, 297.7375849349253940, -10.11643020772709534 ) ) ;
#48978=CARTESIAN_POINT ( 'NONE',  ( 190.8153366230912411, 300.1451374358846920, 3.771947273125533684 ) ) ;
#48979=CARTESIAN_POINT ( 'NONE',  ( 202.6560281492536717, 279.6364581158209717, 17.15553667345918853 ) ) ;
#48981=CARTESIAN_POINT ( 'NONE',  ( 164.0880046841931517, 283.2396324619593884, -6.684692064823180679 ) ) ;
#48982=CARTESIAN_POINT ( 'NONE',  ( 151.5115963269173562, 274.8992243283395283, -8.951992038018516951 ) ) ;
#48984=CARTESIAN_POINT ( 'NONE',  ( 157.7632566947985708, 282.3764601569879460, -1.694678876849560645 ) ) ;
#48985=ORIENTED_EDGE ( 'NONE', *, *, #62049, .T. ) ;
#48990=CARTESIAN_POINT ( 'NONE',  ( 187.0645750985391373, 267.3865546210132038, 14.82880848505713800 ) ) ;
#48993=CARTESIAN_POINT ( 'NONE',  ( -1.069254392388470976, 164.0643266524160140, 9.188101187500095079 ) ) ;
#48994=CARTESIAN_POINT ( 'NONE',  ( 90.05242219234915524, 231.9869531367911293, 4.594050593750046652 ) ) ;
#48995=CARTESIAN_POINT ( 'NONE',  ( 155.4661767250933622, 261.3716783840932294, -17.10192542004562810 ) ) ;
#49003=CARTESIAN_POINT ( 'NONE',  ( 163.6926455977765897, 284.3758010234985818, 5.960030555855258427 ) ) ;
#49005=CARTESIAN_POINT ( 'NONE',  ( 207.6837091943624785, 270.9282591014416539, -1.156610046911421552 ) ) ;
#49006=CARTESIAN_POINT ( 'NONE',  ( 178.6423073663378602, 290.9544255387157818, 10.03153667033594765 ) ) ;
#49007=CARTESIAN_POINT ( 'NONE',  ( 164.1493212971148807, 246.3320308158860144, -5.698338322471421691 ) ) ;
#49012=CARTESIAN_POINT ( 'NONE',  ( 52.08270766911643079, 207.0024278399160664, -9.188101187500093303 ) ) ;
#49015=CARTESIAN_POINT ( 'NONE',  ( 70.26924114858965709, 217.5024278399160664, -9.188101187500093303 ) ) ;
#49016=CARTESIAN_POINT ( 'NONE',  ( 161.6127771116929921, 250.7254542206800352, -12.96229604595372464 ) ) ;
#49018=CARTESIAN_POINT ( 'NONE',  ( -22.42236680055709641, 157.8615022471902591, 0.000000000000000000 ) ) ;
#49021=CARTESIAN_POINT ( 'NONE',  ( 175.9592805506638626, 269.6404646308017163, -17.54410699522518868 ) ) ;
#49026=CARTESIAN_POINT ( 'NONE',  ( 82.61045024828291616, 212.3768266524159856, -9.188101187500093303 ) ) ;
#49028=CARTESIAN_POINT ( 'NONE',  ( 170.3290958195750022, 289.6815776661216546, -1.151831906498994140 ) ) ;
#49030=CARTESIAN_POINT ( 'NONE',  ( 202.0097953763375358, 280.7557661120279136, 17.59517121574885579 ) ) ;
#49031=ORIENTED_EDGE ( 'NONE', *, *, #81679, .T. ) ;
#49036=CARTESIAN_POINT ( 'NONE',  ( 116.0695290213043620, 244.4865022471903444, -10.00000000000009415 ) ) ;
#49041=CARTESIAN_POINT ( 'NONE',  ( 202.9685995779611858, 279.0950685203052899, 16.84977534244423580 ) ) ;
#49046=VERTEX_POINT ( 'NONE', #26572 ) ;
#49047=CARTESIAN_POINT ( 'NONE',  ( 189.1676533816863071, 290.3111667206173365, 14.33508402202939891 ) ) ;
#49048=CARTESIAN_POINT ( 'NONE',  ( 170.5023504269580030, 250.3523026268861713, 3.405075941885475022 ) ) ;
#49049=CARTESIAN_POINT ( 'NONE',  ( 180.8673497570526933, 284.8464743004457773, -15.75982562109706819 ) ) ;
#49061=CARTESIAN_POINT ( 'NONE',  ( 183.1375400018946777, 295.7571731117037643, 0.9692433187012515772 ) ) ;
#49062=CARTESIAN_POINT ( 'NONE',  ( 204.5133713884061706, 276.4194452585140311, 14.87364779308245843 ) ) ;
#49063=FACE_OUTER_BOUND ( 'NONE', #30214, .T. ) ;
#49065=CARTESIAN_POINT ( 'NONE',  ( 155.5660013421004919, 261.1987770755905558, 17.28709111629370199 ) ) ;
#49066=CARTESIAN_POINT ( 'NONE',  ( 121.6084831627943998, 251.0177522451418781, 5.000000000000046185 ) ) ;
#49068=CARTESIAN_POINT ( 'NONE',  ( 207.5461847957217003, 271.1664583471679748, -5.063772443593253847 ) ) ;
#49070=CARTESIAN_POINT ( 'NONE',  ( 166.2346546936187508, 265.4583583427066742, 16.55353420763369954 ) ) ;
#49071=AXIS2_PLACEMENT_3D ( 'NONE', #32336, #8543, #31820 ) ;
#49073=CARTESIAN_POINT ( 'NONE',  ( 75.51934661115029712, 226.6589784336661637, -6.496448406907675876E-16 ) ) ;
#49074=VERTEX_POINT ( 'NONE', #77137 ) ;
#49075=CARTESIAN_POINT ( 'NONE',  ( 150.5780525126727980, 271.8381578737140103, 12.98431582152410968 ) ) ;
#49078=CARTESIAN_POINT ( 'NONE',  ( 157.0907897361001631, 258.5577661063921937, -18.43739762333529342 ) ) ;
#49084=CARTESIAN_POINT ( 'NONE',  ( 159.3237119419271437, 254.6902313965507858, -15.56765445935501191 ) ) ;
#49086=CARTESIAN_POINT ( 'NONE',  ( 94.43719644265542001, 216.1423013555410080, -4.594050593750043987 ) ) ;
#49088=FACE_OUTER_BOUND ( 'NONE', #48715, .T. ) ;
#49090=B_SPLINE_CURVE_WITH_KNOTS ( 'NONE', 3,
 ( #83351, #59493, #98539, #90472 ),
 .UNSPECIFIED., .F., .F.,
 ( 4, 4 ),
 ( 0.03354936294194791474, 0.04243329031352276182 ),
 .UNSPECIFIED. ) ;
#49094=CARTESIAN_POINT ( 'NONE',  ( -7.357133217438179607, 159.8927522451417929, -10.00000000000009059 ) ) ;
#49097=CARTESIAN_POINT ( 'NONE',  ( 157.1187995864133882, 258.5092516225370218, 18.42986330599266509 ) ) ;
#49098=CARTESIAN_POINT ( 'NONE',  ( 160.6939490957829264, 275.5766803063729640, 12.96402070036174337 ) ) ;
#49100=CARTESIAN_POINT ( 'NONE',  ( 188.9422029048082834, 269.7498099985592148, 14.56541238386251891 ) ) ;
#49101=CYLINDRICAL_SURFACE ( 'NONE', #60833, 10.00000000000010658 ) ;
#49104=VERTEX_POINT ( 'NONE', #68044 ) ;
#49105=CARTESIAN_POINT ( 'NONE',  ( 148.9908051373835463, 274.2115824367425603, 8.962154046299646737 ) ) ;
#49106=CARTESIAN_POINT ( 'NONE',  ( 175.6264801365410051, 290.2407708024952626, 8.598400420672549060 ) ) ;
#49110=CARTESIAN_POINT ( 'NONE',  ( 117.4407359106297974, 228.6115022471901739, -5.000000000000041744 ) ) ;
#49111=CARTESIAN_POINT ( 'NONE',  ( 202.7288423927450651, 279.5103401465790398, -16.79777765389096800 ) ) ;
#49114=ADVANCED_FACE ( 'NONE', ( #46735 ), #54315, .T. ) ;
#49115=CARTESIAN_POINT ( 'NONE',  ( 164.6460902696047128, 245.4716017159096566, -3.036414139157908476 ) ) ;
#49116=CARTESIAN_POINT ( 'NONE',  ( 180.5854428321844978, 266.8285079129313999, -14.77326707302557196 ) ) ;
#49117=CARTESIAN_POINT ( 'NONE',  ( 184.8290635382854248, 266.2232361729078889, 13.18960270750180008 ) ) ;
#49118=CARTESIAN_POINT ( 'NONE',  ( 199.1207061629229429, 281.8795345183781365, -16.59791185551577186 ) ) ;
#49120=B_SPLINE_CURVE_WITH_KNOTS ( 'NONE', 3,
 ( #17583, #55065, #1394, #93615 ),
 .UNSPECIFIED., .F., .F.,
 ( 4, 4 ),
 ( 2.797157557069881010E-17, 0.003963014350466228901 ),
 .UNSPECIFIED. ) ;
#49122=CARTESIAN_POINT ( 'NONE',  ( 91.45997379709655206, 233.6115022471902876, -5.000000000000047962 ) ) ;
#49123=CARTESIAN_POINT ( 'NONE',  ( 180.9931686530488548, 273.3540426091562381, 16.66408796176733276 ) ) ;
#49124=CARTESIAN_POINT ( 'NONE',  ( 160.1418619798153600, 272.5460874529753710, -14.82127459029824124 ) ) ;
#49126=B_SPLINE_CURVE_WITH_KNOTS ( 'NONE', 3,
 ( #66627, #89966, #44312, #20546, #51424, #90973, #21533 ),
 .UNSPECIFIED., .F., .F.,
 ( 4, 3, 4 ),
 ( 0.001252835390139021452, 0.001498048275941827635, 0.002504222586275619590 ),
 .UNSPECIFIED. ) ;
#49127=CARTESIAN_POINT ( 'NONE',  ( -5.074968980656518802, 174.0024278399160664, -9.188101187500093303 ) ) ;
#49135=CARTESIAN_POINT ( 'NONE',  ( 33.24700223256990483, 183.8768266524160140, -9.188101187500093303 ) ) ;
#49136=FACE_OUTER_BOUND ( 'NONE', #60416, .T. ) ;
#49137=CARTESIAN_POINT ( 'NONE',  ( 70.67536410627012344, 201.6115022471901739, -5.000000000000041744 ) ) ;
#49139=CARTESIAN_POINT ( 'NONE',  ( 199.6646305490404814, 267.3205410694829425, -6.722116363147288887 ) ) ;
#49140=CARTESIAN_POINT ( 'NONE',  ( 191.1747001918821525, 299.5227014763493116, -9.654804683100723040 ) ) ;
#49141=CARTESIAN_POINT ( 'NONE',  ( 196.2972863317696692, 290.6501220159163381, 17.07231422512514740 ) ) ;
#49142=CARTESIAN_POINT ( 'NONE',  ( 182.5462621144656907, 280.4176611228211300, -16.08232872008645487 ) ) ;
#49144=B_SPLINE_SURFACE_WITH_KNOTS ( 'NONE', 3, 1, ( 
 ( #85772, #94343 ),
 ( #62896, #47195 ),
 ( #86260, #61882 ),
 ( #55281, #9208 ),
 ( #55773, #16800 ),
 ( #85247, #46179 ),
 ( #78621, #40081 ),
 ( #1626, #605 ),
 ( #2116, #71026 ),
 ( #1112, #7701 ),
 ( #32999, #31489 ),
 ( #63900, #47686 ),
 ( #32512, #15792 ),
 ( #8209, #16301 ),
 ( #63404, #94839 ),
 ( #24897, #69499 ),
 ( #25401, #78117 ),
 ( #23388, #24405 ),
 ( #87287, #8706 ),
 ( #54793, #54278 ),
 ( #93851, #79149 ),
 ( #86765, #77099 ),
 ( #113, #38594 ),
 ( #39574, #30997 ),
 ( #46698, #70497 ),
 ( #40585, #17299 ),
 ( #48203, #9732 ),
 ( #77625, #39079 ),
 ( #23892, #69991 ),
 ( #31990, #62381 ),
 ( #93338, #95856 ),
 ( #74015, #57788 ),
 ( #49217, #58775 ),
 ( #27896, #50200 ) ),
 .UNSPECIFIED., .T., .F., .F.,
 ( 4, 2, 2, 2, 2, 2, 2, 2, 2, 2, 2, 2, 2, 2, 2, 2, 4 ),
 ( 2, 2 ),
 ( 0.000000000000000000, 0.06250000000000000000, 0.1250000000000000000, 0.1875000000000000000, 0.2500000000000000000, 0.3125000000000000000, 0.3750000000000000000, 0.4375000000000000000, 0.5000000000000000000, 0.5625000000000000000, 0.6250000000000000000, 0.6875000000000000000, 0.7500000000000000000, 0.8125000000000000000, 0.8750000000000000000, 0.9375000000000000000, 1.000000000000000000 ),
 ( 0.000000000000000000, 1.000000000000000000 ),
 .UNSPECIFIED. ) ;
#49145=CARTESIAN_POINT ( 'NONE',  ( 187.3763302972169242, 296.2500356619865443, -7.707757652183316210 ) ) ;
#49146=ADVANCED_FACE ( 'NONE', ( #91890 ), #22442, .T. ) ;
#49149=CARTESIAN_POINT ( 'NONE',  ( 87.56285948006663489, 221.3615022471902591, -10.00000000000009592 ) ) ;
#49150=CARTESIAN_POINT ( 'NONE',  ( 164.8620696960021519, 246.0477266191988406, 0.9441760987540538386 ) ) ;
#49152=CARTESIAN_POINT ( 'NONE',  ( 50.29670382169353360, 199.8458772461660260, 9.188101187500095079 ) ) ;
#49153=CARTESIAN_POINT ( 'NONE',  ( 197.8822014719394531, 287.9049684674569676, 17.88172308374019792 ) ) ;
#49154=ORIENTED_EDGE ( 'NONE', *, *, #42120, .F. ) ;
#49156=CARTESIAN_POINT ( 'NONE',  ( 150.9115585710837877, 269.2605084359132093, -15.80434701481532578 ) ) ;
#49159=CARTESIAN_POINT ( 'NONE',  ( 169.7025245114118945, 285.7301650108328772, 7.496735491984821920 ) ) ;
#49160=CARTESIAN_POINT ( 'NONE',  ( 168.0788774586240493, 281.7893607645295333, -11.63581643431726320 ) ) ;
#49164=CARTESIAN_POINT ( 'NONE',  ( 202.9685995779611858, 279.0950685203052899, 16.84977534244423580 ) ) ;
#49165=CARTESIAN_POINT ( 'NONE',  ( 196.5806080813426888, 290.1593943507663766, -16.31912166233602690 ) ) ;
#49166=CARTESIAN_POINT ( 'NONE',  ( 175.0827542836768771, 257.3802440988434910, 11.53455802463486712 ) ) ;
#49167=ORIENTED_EDGE ( 'NONE', *, *, #77601, .T. ) ;
#49171=CARTESIAN_POINT ( 'NONE',  ( 171.6344159911060387, 252.4546017485605489, 8.684224258240840655 ) ) ;
#49174=VERTEX_POINT ( 'NONE', #7743 ) ;
#49175=CARTESIAN_POINT ( 'NONE',  ( 179.4321505992908214, 282.5710338533123718, 15.18541787117502118 ) ) ;
#49176=CARTESIAN_POINT ( 'NONE',  ( 190.8264243556038195, 300.1259329198319961, 8.466983560044813117 ) ) ;
#49177=CARTESIAN_POINT ( 'NONE',  ( 177.3128891232254318, 256.0384362114311898, -7.181690309295756691 ) ) ;
#49179=ORIENTED_EDGE ( 'NONE', *, *, #11543, .F. ) ;
#49181=CARTESIAN_POINT ( 'NONE',  ( 161.1747502674735415, 251.4841389699472529, -13.25152330924089839 ) ) ;
#49182=CARTESIAN_POINT ( 'NONE',  ( 171.7624276866505113, 273.7583704609413076, 17.52529772748773595 ) ) ;
#49183=CARTESIAN_POINT ( 'NONE',  ( 196.7823306783968746, 289.8100005636337073, -17.85370042640856170 ) ) ;
#49184=ORIENTED_EDGE ( 'NONE', *, *, #5261, .F. ) ;
#49189=CARTESIAN_POINT ( 'NONE',  ( 166.8729799300310219, 285.2663129487913238, 8.463664631012395745 ) ) ;
#49190=CARTESIAN_POINT ( 'NONE',  ( 115.8441751185107336, 231.5643266524159856, 9.188101187500095079 ) ) ;
#49192=CARTESIAN_POINT ( 'NONE',  ( 196.2293283710122012, 290.7678286567270902, -17.07152402978540096 ) ) ;
#49193=CARTESIAN_POINT ( 'NONE',  ( 183.3879987404869496, 288.3258381666292394, -13.17223454804403993 ) ) ;
#49196=CARTESIAN_POINT ( 'NONE',  ( 208.0045976720423084, 270.3724639545367836, 2.002128742561712471 ) ) ;
#49197=ORIENTED_EDGE ( 'NONE', *, *, #35698, .T. ) ;
#49198=ADVANCED_FACE ( 'NONE', ( #15319 ), #86778, .T. ) ;
#49200=CARTESIAN_POINT ( 'NONE',  ( 157.2590776934911787, 259.4042227141288208, 17.28571348683609088 ) ) ;
#49201=CARTESIAN_POINT ( 'NONE',  ( 204.8682506193380561, 275.1723083338505376, -12.18470981274732701 ) ) ;
#49202=EDGE_CURVE ( 'NONE', #59884, #55652, #29282, .T. ) ;
#49203=CARTESIAN_POINT ( 'NONE',  ( 61.36533069198963375, 215.4244531367911293, -4.594050593750046652 ) ) ;
#49205=CARTESIAN_POINT ( 'NONE',  ( 191.4685399627163633, 299.0137560639802814, 7.545791216288330716 ) ) ;
#49208=ORIENTED_EDGE ( 'NONE', *, *, #9625, .T. ) ;
#49211=CARTESIAN_POINT ( 'NONE',  ( 199.6683510264480788, 265.5076446645038573, 0.06738290090010203015 ) ) ;
#49212=CARTESIAN_POINT ( 'NONE',  ( 186.7782727736096433, 295.3793828959698544, 10.37790068846201841 ) ) ;
#49214=CARTESIAN_POINT ( 'NONE',  ( 152.7607425496961184, 268.9805552238780137, -15.58657372067007074 ) ) ;
#49216=CARTESIAN_POINT ( 'NONE',  ( 207.2683629543511756, 271.6476598918739001, -6.694388351944108528 ) ) ;
#49217=CARTESIAN_POINT ( 'NONE',  ( 192.4867975473904949, 297.2500821921321972, -13.04960750009181325 ) ) ;
#49219=CARTESIAN_POINT ( 'NONE',  ( 149.7162292714551199, 271.3308795146458010, 12.12826134257344357 ) ) ;
#49220=CARTESIAN_POINT ( 'NONE',  ( 164.4494343874829099, 245.8122196953522121, 2.922779519406129456 ) ) ;
#49223=CARTESIAN_POINT ( 'NONE',  ( 164.3545367017254364, 245.9765873086048487, -5.942639963102972267 ) ) ;
#49224=CARTESIAN_POINT ( 'NONE',  ( 123.3675972660055749, 242.0333772461660544, 9.188101187500095079 ) ) ;
#49225=ORIENTED_EDGE ( 'NONE', *, *, #54762, .F. ) ;
#49226=CARTESIAN_POINT ( 'NONE',  ( 191.0478321355427624, 299.7424433957868928, -9.006798842970001218 ) ) ;
#49228=CARTESIAN_POINT ( 'NONE',  ( 167.4785370940337543, 280.2404111755776057, -13.99786577961182665 ) ) ;
#49231=CARTESIAN_POINT ( 'NONE',  ( 174.9088318666119619, 252.9790288038798565, 5.053753844769934389 ) ) ;
#49234=CARTESIAN_POINT ( 'NONE',  ( 154.6388284336715628, 273.3529371992580081, -13.15606555357048713 ) ) ;
#49235=CARTESIAN_POINT ( 'NONE',  ( 183.3396530472832637, 261.1613252051864720, 9.520234298542119333 ) ) ;
#49236=CARTESIAN_POINT ( 'NONE',  ( 165.0817809681736037, 244.7169632896033136, -1.727194264083430131 ) ) ;
#49238=CARTESIAN_POINT ( 'NONE',  ( 195.2593017302202156, 263.4723950921689379, 0.8603167340095838611 ) ) ;
#49241=CARTESIAN_POINT ( 'NONE',  ( 69.62006919151632189, 204.8768266524160140, -9.188101187500091527 ) ) ;
#49242=CARTESIAN_POINT ( 'NONE',  ( 170.7270849433730007, 250.4993316485856099, 3.429389635961456406 ) ) ;
#49243=CARTESIAN_POINT ( 'NONE',  ( 171.3857937658397645, 260.1551371363238445, 14.78898683988441753 ) ) ;
#49244=CARTESIAN_POINT ( 'NONE',  ( 155.1480735223870226, 280.2009427251024363, -0.8861822022151647493 ) ) ;
#49245=CARTESIAN_POINT ( 'NONE',  ( 170.9511032993452204, 286.1488562452602764, -7.996916569637939176 ) ) ;
#49246=CARTESIAN_POINT ( 'NONE',  ( 159.2111180226792726, 254.8852497853115722, 16.01057445397460910 ) ) ;
#49247=CARTESIAN_POINT ( 'NONE',  ( 157.1316430727322881, 271.7231682581081600, -14.76758205110185074 ) ) ;
#49248=CARTESIAN_POINT ( 'NONE',  ( 114.6081111488702078, 243.6427522451419065, -10.00000000000009415 ) ) ;
#49251=EDGE_CURVE ( 'NONE', #13449, #95124, #14726, .T. ) ;
#49252=CARTESIAN_POINT ( 'NONE',  ( 147.6947327179224487, 274.8322142526899370, 9.090449717876689206 ) ) ;
#49253=CARTESIAN_POINT ( 'NONE',  ( -9.459049039432731121, 165.3458772461660544, 9.188101187500095079 ) ) ;
#49254=CARTESIAN_POINT ( 'NONE',  ( 37.98264478980979675, 201.9244531367911293, -4.594050593750046652 ) ) ;
#49255=B_SPLINE_CURVE_WITH_KNOTS ( 'NONE', 3,
 ( #23551, #8870, #54962, #1788 ),
 .UNSPECIFIED., .F., .F.,
 ( 4, 4 ),
 ( 0.03266906780946862709, 0.04161376246641813881 ),
 .UNSPECIFIED. ) ;
#49256=FACE_OUTER_BOUND ( 'NONE', #11387, .T. ) ;
#49260=CARTESIAN_POINT ( 'NONE',  ( 192.4852853123542786, 292.2780683445978980, -14.34739779062837783 ) ) ;
#49261=CARTESIAN_POINT ( 'NONE',  ( 147.1199024702499969, 275.8278494473859723, 5.224467159276165340 ) ) ;
#49263=CARTESIAN_POINT ( 'NONE',  ( 198.1023735320433445, 277.7417427054917312, -16.33290366355920398 ) ) ;
#49264=CARTESIAN_POINT ( 'NONE',  ( 60.91453611423501968, 212.6427522451419065, 10.00000000000009237 ) ) ;
#49266=CARTESIAN_POINT ( 'NONE',  ( 180.8189091534864588, 256.2865937343618157, 1.394926522994340612 ) ) ;
#49267=EDGE_CURVE ( 'NONE', #41296, #31700, #55795, .T. ) ;
#49268=CARTESIAN_POINT ( 'NONE',  ( 157.2777284163744582, 258.2339788142568864, -16.82360006463426316 ) ) ;
#49271=CARTESIAN_POINT ( 'NONE',  ( 46.85966550219804816, 187.8615022471902023, 5.000000000000051514 ) ) ;
#49272=CARTESIAN_POINT ( 'NONE',  ( 202.7599932440484451, 279.4563852894229967, 15.58249343055423353 ) ) ;
#49273=CARTESIAN_POINT ( 'NONE',  ( 4.992576338337581632, 179.8149278399160949, -9.188101187500095079 ) ) ;
#49275=CARTESIAN_POINT ( 'NONE',  ( 164.3408556225676875, 252.5018482456856646, 13.48875141561916635 ) ) ;
#49278=CARTESIAN_POINT ( 'NONE',  ( 206.5571822944673670, 272.8794609281530938, 10.95833005210827515 ) ) ;
#49282=CARTESIAN_POINT ( 'NONE',  ( 148.9194629746633893, 272.7109192224475009, -12.27648025871169679 ) ) ;
#49285=CARTESIAN_POINT ( 'NONE',  ( 167.6610723016181623, 288.0491441363175227, 0.5383436845847213714 ) ) ;
#49287=CARTESIAN_POINT ( 'NONE',  ( 71.97440221194672461, 212.3615022471902591, -10.00000000000009592 ) ) ;
#49290=CARTESIAN_POINT ( 'NONE',  ( -22.42236680055709641, 157.8615022471902591, 0.000000000000000000 ) ) ;
#49292=CARTESIAN_POINT ( 'NONE',  ( 152.8036029408733043, 266.6878101728642037, 15.84078619445996416 ) ) ;
#49293=CARTESIAN_POINT ( 'NONE',  ( 165.0387478276132072, 244.7914988754632191, -2.473354058663827626 ) ) ;
#49295=CARTESIAN_POINT ( 'NONE',  ( 121.3378502276597288, 240.8615022471902591, -10.00000000000009592 ) ) ;
#49296=CARTESIAN_POINT ( 'NONE',  ( 154.8989000222956349, 262.3542304552891551, 17.41779271305265908 ) ) ;
#49298=( BOUNDED_CURVE ( )  B_SPLINE_CURVE ( 2, ( #54177, #8607, #93235, #23794, #76518, #38488, #54678, #76994, #69404 ),
 .UNSPECIFIED., .F., .T. ) 
 B_SPLINE_CURVE_WITH_KNOTS ( ( 3, 2, 2, 2, 3 ),
 ( 0.2379032258064516236, 0.2392473118279569988, 0.2419354838709677491, 0.2446236559139784994, 0.2459677419354838745 ),
 .UNSPECIFIED. ) 
 CURVE ( )  GEOMETRIC_REPRESENTATION_ITEM ( )  RATIONAL_B_SPLINE_CURVE ( ( 0.9330127018922194093, 0.9330127018922194093, 1.000000000000000000, 0.8660254037844387076, 1.000000000000000000, 0.8660254037844387076, 1.000000000000000000, 0.9330127018922194093, 0.9330127018922194093 ) ) 
 REPRESENTATION_ITEM ( '' )  );
#49301=CARTESIAN_POINT ( 'NONE',  ( 156.0175100402996407, 276.9512441243991248, -10.19015957619274459 ) ) ;
#49303=EDGE_LOOP ( 'NONE', ( #2302, #23772, #82368, #98425 ) ) ;
#49311=CARTESIAN_POINT ( 'NONE',  ( 173.8168395337300467, 267.3393752366870331, 16.65285229048275184 ) ) ;
#49312=CARTESIAN_POINT ( 'NONE',  ( 166.2812625422909889, 273.7011810638111342, -15.92596022500507580 ) ) ;
#49316=CARTESIAN_POINT ( 'NONE',  ( 202.9093905060991005, 279.1976216410395182, 16.97070083370504179 ) ) ;
#49317=ORIENTED_EDGE ( 'NONE', *, *, #10255, .T. ) ;
#49319=CARTESIAN_POINT ( 'NONE',  ( 160.3677668160452470, 268.8712655723239777, -16.73982956207869677 ) ) ;
#49320=ORIENTED_EDGE ( 'NONE', *, *, #27017, .T. ) ;
#49321=CARTESIAN_POINT ( 'NONE',  ( 161.0570922196022536, 271.1543799210750763, 16.37266413406176824 ) ) ;
#49322=ORIENTED_EDGE ( 'NONE', *, *, #87113, .T. ) ;
#49323=B_SPLINE_CURVE_WITH_KNOTS ( 'NONE', 3,
 ( #42675, #72630, #3232, #58866 ),
 .UNSPECIFIED., .F., .F.,
 ( 4, 4 ),
 ( 0.000000000000000000, 0.006095114798927191331 ),
 .UNSPECIFIED. ) ;
#49325=CARTESIAN_POINT ( 'NONE',  ( 166.1760138177199622, 271.4483423397350066, 16.23974600030056337 ) ) ;
#49326=CARTESIAN_POINT ( 'NONE',  ( 147.2962480419287772, 275.5224099575481773, 5.989900301663943161 ) ) ;
#49327=CARTESIAN_POINT ( 'NONE',  ( 180.2055717995544910, 290.9255621863335932, -9.559994083472554749 ) ) ;
#49331=CARTESIAN_POINT ( 'NONE',  ( 191.0862225170008628, 299.6759493045793192, -9.402218231374108726 ) ) ;
#49334=CARTESIAN_POINT ( 'NONE',  ( 164.5648480107187197, 245.6123174360222094, 3.015887571020871238 ) ) ;
#49336=CARTESIAN_POINT ( 'NONE',  ( 164.2801755739368446, 246.1053845600426087, 2.518777461081745717 ) ) ;
#49338=VERTEX_POINT ( 'NONE', #1661 ) ;
#49344=CARTESIAN_POINT ( 'NONE',  ( 200.3414094930810165, 283.6454952284590263, 16.87912319229835489 ) ) ;
#49345=CARTESIAN_POINT ( 'NONE',  ( 190.2621123344814293, 301.1033500117378026, -1.456161902152197651 ) ) ;
#49346=EDGE_LOOP ( 'NONE', ( #97799, #66281, #807, #50899, #88143, #9030, #6335, #78588, #72406, #13591, #20671, #31372, #80236, #8063, #22117, #52639, #31361, #5192, #94817, #352, #59258, #11609 ) ) ;
#49347=CYLINDRICAL_SURFACE ( 'NONE', #26810, 17.82106496071139645 ) ;
#49349=ADVANCED_FACE ( 'NONE', ( #9763 ), #99175, .F. ) ;
#49350=CARTESIAN_POINT ( 'NONE',  ( 28.87159617421086821, 174.1427522451417644, 1.119607411625061291E-15 ) ) ;
#49351=CARTESIAN_POINT ( 'NONE',  ( 96.30395630197683943, 238.6589784336661637, -6.496448406907676862E-16 ) ) ;
#49354=CARTESIAN_POINT ( 'NONE',  ( 163.2124973040920111, 247.9546575695509887, 10.85238219581215269 ) ) ;
#49355=CARTESIAN_POINT ( 'NONE',  ( 29.78290061743214423, 181.8768266524160140, 9.188101187500098632 ) ) ;
#49356=CARTESIAN_POINT ( 'NONE',  ( -22.42236680055709641, 157.8615022471902591, 0.000000000000000000 ) ) ;
#49357=ORIENTED_EDGE ( 'NONE', *, *, #22281, .T. ) ;
#49358=ORIENTED_EDGE ( 'NONE', *, *, #88321, .F. ) ;
#49359=CARTESIAN_POINT ( 'NONE',  ( 188.5398260611945886, 261.4740634840828761, -5.959129374122240641 ) ) ;
#49363=CARTESIAN_POINT ( 'NONE',  ( 161.7767236248226084, 250.4414905302161287, -13.15904643207033153 ) ) ;
#49364=CARTESIAN_POINT ( 'NONE',  ( 182.4502648671029874, 284.2291850766257539, 14.94454483467801609 ) ) ;
#49365=CARTESIAN_POINT ( 'NONE',  ( 166.8938901919198088, 251.4769634964625880, 10.27092145616306595 ) ) ;
#49366=CARTESIAN_POINT ( 'NONE',  ( 41.69040282370317385, 201.0024278399160949, -9.188101187500093303 ) ) ;
#49367=CARTESIAN_POINT ( 'NONE',  ( 71.81202244518919997, 222.2677522451419065, -5.000000000000047962 ) ) ;
#49368=VERTEX_POINT ( 'NONE', #82182 ) ;
#49370=EDGE_CURVE ( 'NONE', #93959, #23594, #36426, .T. ) ;
#49371=CARTESIAN_POINT ( 'NONE',  ( 157.9059535858343111, 282.4144519034085192, -1.690885285080969025 ) ) ;
#49372=CARTESIAN_POINT ( 'NONE',  ( -8.782727014549898570, 174.9244531367911293, -4.594050593750046652 ) ) ;
#49374=CARTESIAN_POINT ( 'NONE',  ( 150.8247211172754589, 269.4109153179094278, -14.37608026040300402 ) ) ;
#49375=CARTESIAN_POINT ( 'NONE',  ( -17.42236680055705023, 149.2012482093457777, 0.000000000000000000 ) ) ;
#49376=CARTESIAN_POINT ( 'NONE',  ( 193.1169444172380167, 296.1586357973259283, -13.13373377033755318 ) ) ;
#49377=CARTESIAN_POINT ( 'NONE',  ( 180.2008674086625888, 256.3788900776044102, -7.862092545524210330 ) ) ;
#49378=CARTESIAN_POINT ( 'NONE',  ( 171.6625166626804457, 279.7479999435336140, 15.02938966302312984 ) ) ;
#49380=CARTESIAN_POINT ( 'NONE',  ( 146.5689048584090699, 276.7822053059436485, -0.4306668706573002492 ) ) ;
#49381=CARTESIAN_POINT ( 'NONE',  ( 207.2824254892180704, 271.6233028670009162, 6.274396967990798046 ) ) ;
#49383=ADVANCED_FACE ( 'NONE', ( #43619 ), #74560, .T. ) ;
#49384=CARTESIAN_POINT ( 'NONE',  ( -7.266922234329455499, 176.6115022471903160, -5.000000000000047962 ) ) ;
#49385=CARTESIAN_POINT ( 'NONE',  ( 7.868168403658736487, 186.8967562850346837, -4.648177544792955347E-16 ) ) ;
#49386=CARTESIAN_POINT ( 'NONE',  ( 124.5044291563551297, 236.5643266524159856, -9.188101187500093303 ) ) ;
#49390=CARTESIAN_POINT ( 'NONE',  ( 157.6673516573649181, 257.5591315650518141, 16.79781451397666103 ) ) ;
#49391=CARTESIAN_POINT ( 'NONE',  ( 149.3212960838965557, 247.0177522451417644, 5.000000000000051514 ) ) ;
#49392=CARTESIAN_POINT ( 'NONE',  ( 150.2464011702103335, 270.4125948492565499, -14.58086855962074857 ) ) ;
#49394=CARTESIAN_POINT ( 'NONE',  ( 192.9033750020381603, 263.8409475788059808, -4.418838240603300882 ) ) ;
#49395=CARTESIAN_POINT ( 'NONE',  ( 196.4242782546697015, 290.4301655533025155, -16.42402868779123537 ) ) ;
#49397=CARTESIAN_POINT ( 'NONE',  ( 176.3882048470632071, 292.4445974135971369, -1.112347119103176407 ) ) ;
#49401=CARTESIAN_POINT ( 'NONE',  ( 182.6925099381910513, 273.1766224467805841, 17.62059484408636933 ) ) ;
#49402=CARTESIAN_POINT ( 'NONE',  ( 165.3945084580352329, 269.6251128436156250, -16.31137091215674317 ) ) ;
#49403=CARTESIAN_POINT ( 'NONE',  ( 196.5709421020591776, 271.0089200914278535, 12.02914684137526358 ) ) ;
#49407=CARTESIAN_POINT ( 'NONE',  ( 192.5712965840290849, 297.1037255674836501, 11.03742858512898906 ) ) ;
#49408=EDGE_CURVE ( 'NONE', #34337, #85402, #60643, .T. ) ;
#49409=CARTESIAN_POINT ( 'NONE',  ( 199.4414920144331234, 281.2339203804377235, 17.34600695621782052 ) ) ;
#49411=CARTESIAN_POINT ( 'NONE',  ( 191.8645708310420446, 287.9879281313274646, -15.85676223221169856 ) ) ;
#49414=CARTESIAN_POINT ( 'NONE',  ( 194.7900911235093133, 293.2606606935473792, -14.66228443412922999 ) ) ;
#49415=CARTESIAN_POINT ( 'NONE',  ( 10.58227001879649620, 188.4637435831425023, 2.679491924311251605 ) ) ;
#49418=CARTESIAN_POINT ( 'NONE',  ( 139.9899443387551230, 263.1772991869740395, 1.224646799147364892E-15 ) ) ;
#49419=DIRECTION ( 'NONE',  ( -0.8660254037844387076, -0.4999999999999998890, -0.000000000000000000 ) ) ;
#49420=CARTESIAN_POINT ( 'NONE',  ( 151.4025156491502742, 268.4101458323662541, 14.71049357081981235 ) ) ;
#49423=CARTESIAN_POINT ( 'NONE',  ( 203.4682009197399566, 278.2297336128146412, -15.36039508894693206 ) ) ;
#49425=CARTESIAN_POINT ( 'NONE',  ( 94.85736712102178103, 237.1199935810940929, 2.679491924311251605 ) ) ;
#49427=CARTESIAN_POINT ( 'NONE',  ( 193.4652038833492611, 294.2243501988812682, 14.02643700387929648 ) ) ;
#49430=CARTESIAN_POINT ( 'NONE',  ( 202.7676489560256528, 279.4431252073101746, -16.04062356091568020 ) ) ;
#49431=EDGE_LOOP ( 'NONE', ( #78461, #55367, #53292, #72922 ) ) ;
#49432=CARTESIAN_POINT ( 'NONE',  ( 184.0276249361047007, 281.0631757112061564, -16.18422146133542583 ) ) ;
#49434=CARTESIAN_POINT ( 'NONE',  ( 147.1571408241294705, 275.7633507264765740, -6.825926678015840743 ) ) ;
#49436=CARTESIAN_POINT ( 'NONE',  ( 146.8868584395697781, 276.2314935489248455, -3.891417269505058396 ) ) ;
#49437=CARTESIAN_POINT ( 'NONE',  ( 201.4463813434794019, 281.7316278426353620, -17.16864527463587820 ) ) ;
#49439=CARTESIAN_POINT ( 'NONE',  ( 183.5616576129386033, 284.3076914609734445, -16.02499936821387649 ) ) ;
#49440=CARTESIAN_POINT ( 'NONE',  ( 142.3662031094091844, 246.8768266524159856, -9.188101187500091527 ) ) ;
#49443=ADVANCED_FACE ( 'NONE', ( #19370 ), #44103, .F. ) ;
#49444=ORIENTED_EDGE ( 'NONE', *, *, #88809, .T. ) ;
#49447=ORIENTED_EDGE ( 'NONE', *, *, #42911, .T. ) ;
#49448=CARTESIAN_POINT ( 'NONE',  ( 162.8042930031641049, 248.6616881586264469, 11.14389129512055554 ) ) ;
#49450=DIRECTION ( 'NONE',  ( -0.8660254037844387076, -0.4999999999999998890, -0.000000000000000000 ) ) ;
#49451=CARTESIAN_POINT ( 'NONE',  ( 156.1835980877939960, 279.5352826047603685, 7.598597465648954774 ) ) ;
#49454=CARTESIAN_POINT ( 'NONE',  ( 174.7165626157769509, 282.0434896912144040, 14.26103646697991678 ) ) ;
#49456=CARTESIAN_POINT ( 'NONE',  ( 176.8882704868359781, 255.8434036686267348, -7.282961206419556355 ) ) ;
#49458=CARTESIAN_POINT ( 'NONE',  ( 183.8301289239822722, 272.2411597453489662, -17.34995410509954183 ) ) ;
#49460=EDGE_LOOP ( 'NONE', ( #40904, #35759, #55968, #1201 ) ) ;
#49462=B_SPLINE_CURVE_WITH_KNOTS ( 'NONE', 3,
 ( #97104, #87027, #17559, #41850, #26661, #57545, #49961, #73270, #79407, #65649, #96606, #27168, #40834, #22039, #20568, #29157, #58539, #60028, #83888, #59021, #89992, #51446, #68136, #90504 ),
 .UNSPECIFIED., .F., .F.,
 ( 4, 2, 2, 2, 2, 2, 2, 2, 2, 2, 2, 4 ),
 ( 0.0002849336745323140284, 0.001954281156355254252, 0.002162949591583106668, 0.002267283809196996881, 0.002293367363600446775, 0.002319450918003896668, 0.002345534472407346128, 0.002371618026810796021, 0.002580286462039149773, 0.002788954897267503525, 0.003206291767724232713, 0.003623628638180961467 ),
 .UNSPECIFIED. ) ;
#49463=CARTESIAN_POINT ( 'NONE',  ( 201.8725009077853656, 268.2699010817517546, -2.859759887887624252 ) ) ;
#49464=CARTESIAN_POINT ( 'NONE',  ( 191.5817909860246573, 298.8175995376009837, -10.84987806275361422 ) ) ;
#49465=CARTESIAN_POINT ( 'NONE',  ( 148.9719199701866899, 272.6200610409887872, 12.59512981512031438 ) ) ;
#49466=CARTESIAN_POINT ( 'NONE',  ( 162.6264071486809542, 248.9697954965390920, 10.36322805486644683 ) ) ;
#49470=VERTEX_POINT ( 'NONE', #99342 ) ;
#49472=CARTESIAN_POINT ( 'NONE',  ( 190.2874339040999132, 273.3649718585393771, -16.54444726514628528 ) ) ;
#49474=AXIS2_PLACEMENT_3D ( 'NONE', #24312, #92739, #39477 ) ;
#49475=CARTESIAN_POINT ( 'NONE',  ( 153.4578721839791342, 264.8501638863745029, 16.85421393845643223 ) ) ;
#49477=CARTESIAN_POINT ( 'NONE',  ( -22.42236680055709641, 157.8615022471902591, 0.000000000000000000 ) ) ;
#49478=CARTESIAN_POINT ( 'NONE',  ( 202.2576150004249200, 280.3265299319959354, 16.24828394350762295 ) ) ;
#49479=CARTESIAN_POINT ( 'NONE',  ( 4.126898030318161936, 167.0643266524160140, 9.188101187500095079 ) ) ;
#49480=CARTESIAN_POINT ( 'NONE',  ( 103.3950599391094443, 224.3768266524160140, -9.188101187500091527 ) ) ;
#49481=CARTESIAN_POINT ( 'NONE',  ( 202.9881971861223917, 279.0611244672630278, -15.16231470264511927 ) ) ;
#49484=CARTESIAN_POINT ( 'NONE',  ( 74.00414925029257063, 213.5333772461660544, 9.188101187500095079 ) ) ;
#49487=CARTESIAN_POINT ( 'NONE',  ( 160.5082202113964058, 282.2950551440661684, 5.085134855888336247 ) ) ;
#49488=CARTESIAN_POINT ( 'NONE',  ( 189.6418160314586601, 300.5678929089384042, -1.578015730609050093 ) ) ;
#49489=CARTESIAN_POINT ( 'NONE',  ( 162.0470192796247488, 249.9733247230335280, 13.57526672572842408 ) ) ;
#49490=CARTESIAN_POINT ( 'NONE',  ( 5.633247839328403117, 167.3927522451417929, -10.00000000000009237 ) ) ;
#49492=B_SPLINE_CURVE_WITH_KNOTS ( 'NONE', 3,
 ( #89144, #3973, #35864, #58163 ),
 .UNSPECIFIED., .F., .F.,
 ( 4, 4 ),
 ( 0.006719243664021112145, 0.01482884518371295826 ),
 .UNSPECIFIED. ) ;
#49494=CARTESIAN_POINT ( 'NONE',  ( 196.2350291401047571, 264.4780031501763347, 5.359379669934941859 ) ) ;
#49496=CARTESIAN_POINT ( 'NONE',  ( 175.0296968597178306, 264.6864531019056699, -16.70299667166197466 ) ) ;
#49497=ADVANCED_FACE ( 'NONE', ( #75047 ), #69420, .T. ) ;
#49498=EDGE_CURVE ( 'NONE', #59274, #72102, #86033, .T. ) ;
#49499=CARTESIAN_POINT ( 'NONE',  ( 88.80803131805656392, 212.8923013555409796, 4.594050593750050204 ) ) ;
#49500=CARTESIAN_POINT ( 'NONE',  ( 161.5757715694810770, 250.7895496999525449, -14.51803553215175135 ) ) ;
#49502=CARTESIAN_POINT ( 'NONE',  ( 163.2515686412894240, 258.2197170105911823, 16.67045586147303027 ) ) ;
#49504=CARTESIAN_POINT ( 'NONE',  ( 151.8693293926424133, 267.6016007109669204, 16.84127110976715969 ) ) ;
#49505=CARTESIAN_POINT ( 'NONE',  ( 173.4020954499399636, 268.3532267536930362, -16.29294589187022524 ) ) ;
#49509=CARTESIAN_POINT ( 'NONE',  ( 1.663964738649697406, 171.7677522451418781, 10.00000000000009592 ) ) ;
#49510=ORIENTED_EDGE ( 'NONE', *, *, #54624, .F. ) ;
#49512=CARTESIAN_POINT ( 'NONE',  ( 77.06204113558260360, 224.4869531367911293, 4.594050593750046652 ) ) ;
#49514=CARTESIAN_POINT ( 'NONE',  ( 169.8070512275697865, 289.2548177291374714, -1.145209284012313589 ) ) ;
#49515=CARTESIAN_POINT ( 'NONE',  ( 146.9978162861947908, 276.0393089210717790, -5.134868500856280882 ) ) ;
#49516=CARTESIAN_POINT ( 'NONE',  ( 201.5573355828420290, 281.5394494627441304, 17.77782387441517642 ) ) ;
#49522=CARTESIAN_POINT ( 'NONE',  ( 129.1320788617196911, 245.3615022471902591, -10.00000000000009592 ) ) ;
#49523=CARTESIAN_POINT ( 'NONE',  ( 205.3465787480556344, 274.9762877783610406, -13.79319041940166279 ) ) ;
#49528=CARTESIAN_POINT ( 'NONE',  ( 163.2919429874875448, 247.8170536094679903, 9.876785378511263147 ) ) ;
#49534=CARTESIAN_POINT ( 'NONE',  ( 192.8618517578005935, 292.5118789037293254, 15.26420307798650988 ) ) ;
#49535=CARTESIAN_POINT ( 'NONE',  ( 168.9111548808109831, 249.2523013957518572, 3.445451539549450271 ) ) ;
#49537=CARTESIAN_POINT ( 'NONE',  ( 201.4463813434794019, 281.7316278426353620, -17.16864527463587820 ) ) ;
#49538=VERTEX_POINT ( 'NONE', #2539 ) ;
#49539=CARTESIAN_POINT ( 'NONE',  ( 101.3989120123781191, 240.8967562850346837, -4.648177544792955347E-16 ) ) ;
#49542=B_SPLINE_CURVE_WITH_KNOTS ( 'NONE', 3,
 ( #58659, #29285, #28268, #42461 ),
 .UNSPECIFIED., .F., .F.,
 ( 4, 4 ),
 ( 0.0004980378164629916185, 0.005738741390616254080 ),
 .UNSPECIFIED. ) ;
#49547=CARTESIAN_POINT ( 'NONE',  ( 189.5749590748330604, 276.2698024016027034, 17.49222575591110029 ) ) ;
#49548=CARTESIAN_POINT ( 'NONE',  ( 204.2133777088835700, 276.9390495533970693, 13.75768580338462144 ) ) ;
#49549=CARTESIAN_POINT ( 'NONE',  ( 194.9385458806846430, 293.0035295114944347, -15.70518692812489192 ) ) ;
#49553=CARTESIAN_POINT ( 'NONE',  ( 187.4971950882544434, 291.4527388498394203, -14.03054952020046287 ) ) ;
#49554=CARTESIAN_POINT ( 'NONE',  ( 163.9664443306652970, 246.6487830133108901, 5.061536945078034755 ) ) ;
#49555=CARTESIAN_POINT ( 'NONE',  ( 169.6143685303033521, 267.3532035066224353, 16.95358291501599268 ) ) ;
#49557=CARTESIAN_POINT ( 'NONE',  ( 94.81556191316359161, 234.7369531367911009, -4.594050593750048428 ) ) ;
#49558=VERTEX_POINT ( 'NONE', #62808 ) ;
#49564=ORIENTED_EDGE ( 'NONE', *, *, #31210, .T. ) ;
#49566=CARTESIAN_POINT ( 'NONE',  ( 197.0146455733971607, 286.4246647896720219, -17.74745810526840728 ) ) ;
#49568=CARTESIAN_POINT ( 'NONE',  ( 159.2186641046529303, 254.8721795879351646, -15.96198087403305443 ) ) ;
#49569=CARTESIAN_POINT ( 'NONE',  ( 207.0603918771781764, 270.3690891701808141, -3.414019917217335998 ) ) ;
#49570=CARTESIAN_POINT ( 'NONE',  ( 93.65192705076950119, 231.0024278399160949, -9.188101187500093303 ) ) ;
#49573=CARTESIAN_POINT ( 'NONE',  ( 163.3939361803663246, 247.6403962173759226, -10.78041711314006790 ) ) ;
#49575=EDGE_CURVE ( 'NONE', #23023, #2236, #19620, .T. ) ;
#49577=CARTESIAN_POINT ( 'NONE',  ( 153.4689407916852701, 266.8309924954582470, 16.62268559038933091 ) ) ;
#49579=CARTESIAN_POINT ( 'NONE',  ( 132.2983106946500982, 253.3149278399160949, -9.188101187500095079 ) ) ;
#49582=CARTESIAN_POINT ( 'NONE',  ( -1.387478102835363769, 181.5530062829863596, 2.649461200531984646E-14 ) ) ;
#49584=CARTESIAN_POINT ( 'NONE',  ( 156.8572647664473152, 258.9622432186664014, 16.97926827742052325 ) ) ;
#49588=CARTESIAN_POINT ( 'NONE',  ( 175.3476828388916715, 283.8530321168340151, 13.26393746783803884 ) ) ;
#49589=( BOUNDED_CURVE ( )  B_SPLINE_CURVE ( 2, ( #73159, #28025, #74657, #27552, #88402, #11370, #28518, #26550, #12344 ),
 .UNSPECIFIED., .F., .T. ) 
 B_SPLINE_CURVE_WITH_KNOTS ( ( 3, 2, 2, 2, 3 ),
 ( 0.8346774193548387455, 0.8360215053763441206, 0.8387096774193548709, 0.8413978494623656212, 0.8427419354838709964 ),
 .UNSPECIFIED. ) 
 CURVE ( )  GEOMETRIC_REPRESENTATION_ITEM ( )  RATIONAL_B_SPLINE_CURVE ( ( 0.9330127018922194093, 0.9330127018922194093, 1.000000000000000000, 0.8660254037844387076, 1.000000000000000000, 0.8660254037844387076, 1.000000000000000000, 0.9330127018922194093, 0.9330127018922194093 ) ) 
 REPRESENTATION_ITEM ( '' )  );
#49592=CARTESIAN_POINT ( 'NONE',  ( 197.3270082884988881, 280.8508283618238011, -16.59807545582490818 ) ) ;
#49593=CARTESIAN_POINT ( 'NONE',  ( 148.9284654111854422, 274.1387509264121718, 8.943080486779532379 ) ) ;
#49594=CARTESIAN_POINT ( 'NONE',  ( 200.9110265982630779, 282.6588894614233141, 17.52479721249226685 ) ) ;
#49596=CARTESIAN_POINT ( 'NONE',  ( 167.7287655016564258, 249.9781926236658762, 6.962022607689601017 ) ) ;
#49598=CARTESIAN_POINT ( 'NONE',  ( 175.2034740169264069, 290.8617031373823920, -6.552222927434346644 ) ) ;
#49601=CIRCLE ( 'NONE', #62532, 16.82106496071157764 ) ;
#49603=CARTESIAN_POINT ( 'NONE',  ( 180.1950043829998265, 266.5822710862183840, -14.77280089193513390 ) ) ;
#49604=CARTESIAN_POINT ( 'NONE',  ( 196.4287751515431921, 269.1031666285815618, -12.09581130873691279 ) ) ;
#49609=DIRECTION ( 'NONE',  ( 0.4999999999999992784, -0.8660254037844390407, 0.000000000000000000 ) ) ;
#49610=CARTESIAN_POINT ( 'NONE',  ( 183.7008669673737700, 274.9450795675618338, 16.36284127036905289 ) ) ;
#49614=CARTESIAN_POINT ( 'NONE',  ( 19.44454881187291662, 182.0333772461660544, 9.188101187500095079 ) ) ;
#49616=ORIENTED_EDGE ( 'NONE', *, *, #62643, .T. ) ;
#49621=CARTESIAN_POINT ( 'NONE',  ( 34.43744006700849525, 196.8149278399161233, 9.188101187500093303 ) ) ;
#49623=CARTESIAN_POINT ( 'NONE',  ( 190.8545714895799392, 300.0771806536980648, -5.516553996882049837 ) ) ;
#49625=CARTESIAN_POINT ( 'NONE',  ( 180.2734563701938555, 292.7663661626478415, 6.129196057519468610 ) ) ;
#49626=CARTESIAN_POINT ( 'NONE',  ( 191.0481192767711036, 299.7419460525905492, -9.103377665618040737 ) ) ;
#49627=CARTESIAN_POINT ( 'NONE',  ( 181.8559320684326224, 273.7276056269956257, 17.73031764801637067 ) ) ;
#49628=CARTESIAN_POINT ( 'NONE',  ( 163.1700791268402497, 270.5728986487383168, 17.16554465343218894 ) ) ;
#49631=CARTESIAN_POINT ( 'NONE',  ( 81.06766895168337328, 207.6115022471902023, -5.000000000000041744 ) ) ;
#49634=CARTESIAN_POINT ( 'NONE',  ( 35.49282175392953320, 200.4869531367911293, 4.594050593750046652 ) ) ;
#49637=CARTESIAN_POINT ( 'NONE',  ( 198.4344074287054696, 286.9485196940960918, -17.83642855442570152 ) ) ;
#49640=CARTESIAN_POINT ( 'NONE',  ( 170.8054577101068219, 287.4915981561377976, 8.526299399445241178 ) ) ;
#49641=CARTESIAN_POINT ( 'NONE',  ( 164.4440639631384045, 245.8215215431751233, -2.910115319305802029 ) ) ;
#49642=CARTESIAN_POINT ( 'NONE',  ( 193.4301016519987400, 295.6162315559625426, 13.49693599934615662 ) ) ;
#49647=CARTESIAN_POINT ( 'NONE',  ( 171.3689516288318089, 255.6897779434656002, 12.22461471063935257 ) ) ;
#49648=VERTEX_POINT ( 'NONE', #25839 ) ;
#49652=CARTESIAN_POINT ( 'NONE',  ( 20.01287798488040437, 182.3615022471902591, -10.00000000000009592 ) ) ;
#49653=CARTESIAN_POINT ( 'NONE',  ( 166.1070111784138703, 253.4115428555481344, -13.60050710122670559 ) ) ;
#49656=CARTESIAN_POINT ( 'NONE',  ( 191.4941427383744781, 298.9694107557253346, 8.584406880462095657 ) ) ;
#49659=VERTEX_POINT ( 'NONE', #10630 ) ;
#49662=CARTESIAN_POINT ( 'NONE',  ( 207.2707369601997982, 271.6435479931266173, -5.381413637561199614 ) ) ;
#49665=CIRCLE ( 'NONE', #55324, 17.82106496071138224 ) ;
#49667=CARTESIAN_POINT ( 'NONE',  ( 152.9607371460978129, 265.7112270302071124, -16.17698032818104537 ) ) ;
#49668=CARTESIAN_POINT ( 'NONE',  ( 159.4889735931715222, 254.4039898200529706, 16.88104032092801887 ) ) ;
#49671=CARTESIAN_POINT ( 'NONE',  ( 204.6149525604204769, 276.2435015074934199, -13.22810747389629960 ) ) ;
#49672=CARTESIAN_POINT ( 'NONE',  ( 111.5140480995885639, 229.0643266524159856, -9.188101187500093303 ) ) ;
#49673=CARTESIAN_POINT ( 'NONE',  ( 183.5953950971229744, 289.9057545191589043, -13.74357891376704544 ) ) ;
#49675=ORIENTED_EDGE ( 'NONE', *, *, #88875, .T. ) ;
#49677=CARTESIAN_POINT ( 'NONE',  ( 207.6590484093196096, 270.9709728340903894, 3.402057849327809524 ) ) ;
#49678=VERTEX_POINT ( 'NONE', #28299 ) ;
#49683=CARTESIAN_POINT ( 'NONE',  ( 65.07308872588301085, 214.5024278399160949, -9.188101187500093303 ) ) ;
#49685=CARTESIAN_POINT ( 'NONE',  ( 151.0099717111976076, 269.0900518771037468, 15.84752309685681659 ) ) ;
#49686=CARTESIAN_POINT ( 'NONE',  ( 150.5824154016292198, 269.8306011283729617, 15.30661888403989046 ) ) ;
#49687=B_SPLINE_CURVE_WITH_KNOTS ( 'NONE', 3,
 ( #5298, #81833, #90940, #90444, #75207, #20508, #98512, #51896, #66593, #37180, #73705, #67580, #88974, #21015, #75700, #28583, #6287, #21491, #89930, #43776, #5784, #50389, #27109, #52381, #58958, #74222, #57993, #35187, #19529, #97043, #81341, #12410, #36177, #11915, #42771, #51383, #98003, #44277, #59462, #82837, #58477, #13406, #89450, #50885, #4811, #99500, #14872, #54869, #14391, #45761 ),
 .UNSPECIFIED., .F., .F.,
 ( 4, 2, 2, 2, 2, 2, 2, 2, 2, 2, 2, 2, 2, 2, 2, 2, 2, 2, 2, 2, 2, 2, 2, 2, 4 ),
 ( 0.0002878354312401214233, 0.0007598946772537885311, 0.001231953923267455585, 0.001467983546274291388, 0.001585998357777737696, 0.001704013169281184438, 0.001822027980784630746, 0.001940042792288077488, 0.002176072415294993522, 0.002648131661308826025, 0.003120190907322658094, 0.004064309399350322233, 0.005008427891377987239, 0.005480487137391740378, 0.005716516760398653377, 0.005834531571902066074, 0.005952546383405478772, 0.006011553789157129610, 0.006070561194908782182, 0.006188576006412259065, 0.006424605629419186809, 0.006896664875433114288, 0.007368724121447040899, 0.007604753744453974715, 0.007840783367460907663 ),
 .UNSPECIFIED. ) ;
#49688=ORIENTED_EDGE ( 'NONE', *, *, #70437, .T. ) ;
#49693=ORIENTED_EDGE ( 'NONE', *, *, #67444, .T. ) ;
#49694=CARTESIAN_POINT ( 'NONE',  ( 172.3726553231756498, 259.9039163444838891, -13.86549437502850779 ) ) ;
#49698=CARTESIAN_POINT ( 'NONE',  ( 207.1875246860671211, 270.9789124136162854, 2.454475744023529415 ) ) ;
#49699=CARTESIAN_POINT ( 'NONE',  ( 149.4539134692060145, 271.7852238117696402, 12.95627816374690688 ) ) ;
#49700=CARTESIAN_POINT ( 'NONE',  ( 31.25085430583858681, 200.3967562850347122, -4.648177544792955347E-16 ) ) ;
#49701=CARTESIAN_POINT ( 'NONE',  ( 152.4039861250167576, 270.1776706740954523, -14.65162667463488511 ) ) ;
#49703=CARTESIAN_POINT ( 'NONE',  ( 164.2776907674634970, 254.2239456688865573, 14.24022417734382451 ) ) ;
#49705=CARTESIAN_POINT ( 'NONE',  ( 208.2555382576270233, 269.9378221106229034, 3.215405476967123199 ) ) ;
#49706=CARTESIAN_POINT ( 'NONE',  ( 124.1257165900819359, 230.2202760586659736, -5.415160957724236172E-17 ) ) ;
#49709=CARTESIAN_POINT ( 'NONE',  ( 198.2505066714982149, 285.2670451491296149, 0.000000000000000000 ) ) ;
#49710=CARTESIAN_POINT ( 'NONE',  ( 174.2379957965557651, 251.2590728793752248, 3.639292605338433795 ) ) ;
#49711=ADVANCED_FACE ( 'NONE', ( #24205 ), #77917, .T. ) ;
#49712=CARTESIAN_POINT ( 'NONE',  ( 163.8990931530087494, 246.7654386749614162, 5.873176884778091633 ) ) ;
#49713=CARTESIAN_POINT ( 'NONE',  ( 0.09429369783835704621, 160.8615022471902023, 5.000000000000051514 ) ) ;
#49718=DIRECTION ( 'NONE',  ( 0.4999999999999992784, -0.8660254037844390407, 0.000000000000000000 ) ) ;
#49720=CARTESIAN_POINT ( 'NONE',  ( 206.2880451275741223, 273.3456201754175368, -11.28869033117385534 ) ) ;
#49721=CARTESIAN_POINT ( 'NONE',  ( 138.3604885211411215, 256.8149278399160949, 9.188101187500093303 ) ) ;
#49722=CARTESIAN_POINT ( 'NONE',  ( 188.0737869051473012, 299.5124861214166572, -3.734995909225475863 ) ) ;
#49725=CARTESIAN_POINT ( 'NONE',  ( 59.90443346675090908, 196.2048013555409796, 4.594050593750051981 ) ) ;
#49728=CARTESIAN_POINT ( 'NONE',  ( 191.7653887625562561, 297.2434025333955674, 10.91538051584371338 ) ) ;
#49733=CARTESIAN_POINT ( 'NONE',  ( 190.6094661480870798, 300.5017155583701083, 4.598210453186021951 ) ) ;
#49734=CARTESIAN_POINT ( 'NONE',  ( 155.3771721686844955, 279.7991985491945002, -1.232760055725913961 ) ) ;
#49735=CARTESIAN_POINT ( 'NONE',  ( 172.2711439251446848, 287.1981181489559276, -8.134297672120377243 ) ) ;
#49736=CARTESIAN_POINT ( 'NONE',  ( 155.4495868485232108, 261.4004128932040203, -18.48326470492642315 ) ) ;
#49737=CARTESIAN_POINT ( 'NONE',  ( 149.0239636976596955, 274.5272459498808644, 9.114559754079525788 ) ) ;
#49738=EDGE_CURVE ( 'NONE', #71254, #63287, #62996, .T. ) ;
#49739=CARTESIAN_POINT ( 'NONE',  ( 130.3409059842875024, 259.3927522451419918, 2.944929066748280225E-16 ) ) ;
#49743=CARTESIAN_POINT ( 'NONE',  ( 196.3341081413628899, 290.5863447708742342, 16.12390540996472410 ) ) ;
#49744=FACE_OUTER_BOUND ( 'NONE', #2470, .T. ) ;
#49745=CARTESIAN_POINT ( 'NONE',  ( -8.160010933756074891, 166.0958772461660544, -9.188101187500095079 ) ) ;
#49746=CARTESIAN_POINT ( 'NONE',  ( 33.21950506899538880, 199.1744531367911293, 4.594050593750047540 ) ) ;
#49747=CARTESIAN_POINT ( 'NONE',  ( 177.9283168337505856, 258.7219139204152611, -10.33080451080644835 ) ) ;
#49751=CARTESIAN_POINT ( 'NONE',  ( 205.2941531242069857, 275.0670916224857478, -13.92605142593109058 ) ) ;
#49753=CARTESIAN_POINT ( 'NONE',  ( 146.9376205018946848, 276.1435710778808925, 5.066564108429441937 ) ) ;
#49756=CARTESIAN_POINT ( 'NONE',  ( 171.4364905295525148, 258.3445811437964608, 14.25707489073475820 ) ) ;
#49757=CARTESIAN_POINT ( 'NONE',  ( 60.04851071045058575, 212.1427522451419065, -10.00000000000009415 ) ) ;
#49759=CARTESIAN_POINT ( 'NONE',  ( 6.176825452568912134, 162.8262482093457777, 3.021315404115420679E-15 ) ) ;
#49760=CARTESIAN_POINT ( 'NONE',  ( 172.7217183343613272, 250.6623360901680826, 4.659671216799099902 ) ) ;
#49761=CARTESIAN_POINT ( 'NONE',  ( 46.06580888206229929, 190.7365022471902023, -10.00000000000009059 ) ) ;
#49762=DIRECTION ( 'NONE',  ( -0.8660254037844387076, -0.4999999999999998890, 0.000000000000000000 ) ) ;
#49764=CARTESIAN_POINT ( 'NONE',  ( 2.232293911657190488, 172.0958772461660544, -9.188101187500095079 ) ) ;
#49766=CARTESIAN_POINT ( 'NONE',  ( 164.3503491577412206, 246.9192647184853797, 5.874781936951689154 ) ) ;
#49767=CARTESIAN_POINT ( 'NONE',  ( 192.0332533962074706, 298.0356437054567778, 11.70630383928353346 ) ) ;
#49770=CARTESIAN_POINT ( 'NONE',  ( 207.3062152119541679, 271.5820978585240368, 7.879821064966149535 ) ) ;
#49772=CARTESIAN_POINT ( 'NONE',  ( 196.3174919959537306, 290.6151247789487684, -17.61248417473235151 ) ) ;
#49773=CARTESIAN_POINT ( 'NONE',  ( 176.4591198490730903, 260.2994120462323622, -13.48214217372917467 ) ) ;
#49776=CARTESIAN_POINT ( 'NONE',  ( 168.8659486881605858, 288.0201417398660624, 0.5198760491440675979 ) ) ;
#49778=CARTESIAN_POINT ( 'NONE',  ( 158.9079007699492081, 259.3251291931981655, 16.70475046150345477 ) ) ;
#49779=CARTESIAN_POINT ( 'NONE',  ( 153.1962011273530209, 277.8089822112107186, -4.949296756707812328 ) ) ;
#49780=CARTESIAN_POINT ( 'NONE',  ( 156.6797689995629810, 276.8288829890643683, 11.48459988132798770 ) ) ;
#49781=CARTESIAN_POINT ( 'NONE',  ( 159.2186641046529303, 254.8721795879351646, -15.96198087403305443 ) ) ;
#49783=CARTESIAN_POINT ( 'NONE',  ( 152.6372694546979574, 266.7629011907697532, 15.66192084360741177 ) ) ;
#49784=CARTESIAN_POINT ( 'NONE',  ( 164.5416088356626290, 245.6525688679454618, -1.463507744092769292 ) ) ;
#49788=DIRECTION ( 'NONE',  ( 0.4999999999999992784, -0.8660254037844390407, 0.000000000000000000 ) ) ;
#49789=CARTESIAN_POINT ( 'NONE',  ( -22.42236680055709641, 157.8615022471902591, 0.000000000000000000 ) ) ;
#49791=ORIENTED_EDGE ( 'NONE', *, *, #39597, .T. ) ;
#49795=CARTESIAN_POINT ( 'NONE',  ( 183.6215648671697522, 257.5753772875778509, -6.308267261209747012 ) ) ;
#49797=CARTESIAN_POINT ( 'NONE',  ( 197.0313051377892748, 289.3787641501790517, -17.15509075150697882 ) ) ;
#49800=EDGE_CURVE ( 'NONE', #47930, #4325, #43797, .T. ) ;
#49802=CARTESIAN_POINT ( 'NONE',  ( 200.5621507313343557, 283.2631601884785368, 16.81037192529623425 ) ) ;
#49803=CARTESIAN_POINT ( 'NONE',  ( 169.4682171067899219, 276.3332340018203581, -15.66424579517577698 ) ) ;
#49804=CIRCLE ( 'NONE', #41694, 17.82106496071138935 ) ;
#49807=CARTESIAN_POINT ( 'NONE',  ( 170.6915967899095676, 255.4523109143232489, -11.49442897741288760 ) ) ;
#49810=ORIENTED_EDGE ( 'NONE', *, *, #55817, .F. ) ;
#49811=CARTESIAN_POINT ( 'NONE',  ( -22.42236680055709641, 157.8615022471902591, 0.000000000000000000 ) ) ;
#49813=CARTESIAN_POINT ( 'NONE',  ( 157.5163452712333481, 268.9055778063874413, 15.60794413863430030 ) ) ;
#49814=ORIENTED_EDGE ( 'NONE', *, *, #57378, .F. ) ;
#49816=CARTESIAN_POINT ( 'NONE',  ( 168.7855823332611749, 272.8000461963538896, 15.99225062755306404 ) ) ;
#49817=CARTESIAN_POINT ( 'NONE',  ( 147.2424361040780525, 275.6156149679597434, 7.148024958481665081 ) ) ;
#49818=CARTESIAN_POINT ( 'NONE',  ( 177.3637675892562697, 288.7201378008653023, -9.706580938851226747 ) ) ;
#49820=CARTESIAN_POINT ( 'NONE',  ( 193.6538297768585153, 294.3106073703939387, 13.99927879369582406 ) ) ;
#49822=CARTESIAN_POINT ( 'NONE',  ( 178.5150000607630147, 291.6227694413174163, 6.743235598791427421 ) ) ;
#49823=CARTESIAN_POINT ( 'NONE',  ( 158.7282104597116756, 255.7216702197306404, -17.63877974206365451 ) ) ;
#49828=CARTESIAN_POINT ( 'NONE',  ( 205.9642072045669465, 273.9065239114831911, 10.22128930895731536 ) ) ;
#49830=CARTESIAN_POINT ( 'NONE',  ( 159.9307118030769175, 253.6388767968520881, 16.60600887889890487 ) ) ;
#49832=CARTESIAN_POINT ( 'NONE',  ( 147.0341782662149512, 275.9763281242129551, -2.570835274536595438 ) ) ;
#49833=CARTESIAN_POINT ( 'NONE',  ( 171.5796386137203910, 259.5337856624209962, -13.92799914495203772 ) ) ;
#49837=EDGE_CURVE ( 'NONE', #58518, #78498, #69402, .T. ) ;
#49838=CARTESIAN_POINT ( 'NONE',  ( 160.6711157858514412, 252.3564594805604031, -15.48854669559399078 ) ) ;
#49839=CARTESIAN_POINT ( 'NONE',  ( 190.5061062016229698, 300.6807402371136959, -0.1226455231808365465 ) ) ;
#49843=DIRECTION ( 'NONE',  ( -0.8660254037844387076, -0.4999999999999998890, -0.000000000000000000 ) ) ;
#49844=CARTESIAN_POINT ( 'NONE',  ( 186.6673878995319455, 276.5074556901925007, 17.73048906045012529 ) ) ;
#49845=CARTESIAN_POINT ( 'NONE',  ( 34.93377400070185956, 197.6427522451419065, 10.00000000000009237 ) ) ;
#49846=CARTESIAN_POINT ( 'NONE',  ( 100.9591899430832029, 229.0958772461660260, -9.188101187500095079 ) ) ;
#49847=CARTESIAN_POINT ( 'NONE',  ( 180.9559662842916907, 294.1923438242872066, -2.650091675432668215 ) ) ;
#49849=CARTESIAN_POINT ( 'NONE',  ( 162.6859166034911652, 248.8667220972772611, 10.26171246773997758 ) ) ;
#49850=CARTESIAN_POINT ( 'NONE',  ( 19.11978928545374501, 181.8458772461660544, 9.188101187500095079 ) ) ;
#49851=CARTESIAN_POINT ( 'NONE',  ( 177.5789271328089569, 256.9092084430625960, 10.75158368189463154 ) ) ;
#49853=CARTESIAN_POINT ( 'NONE',  ( 185.1442001806119890, 259.9352252026162091, -5.714739739034400579 ) ) ;
#49857=CARTESIAN_POINT ( 'NONE',  ( 207.1158949475991164, 271.9117422260973740, -5.823035679195911918 ) ) ;
#49858=CARTESIAN_POINT ( 'NONE',  ( 185.6362014350900722, 286.2933592875990030, 15.44405011100975855 ) ) ;
#49859=CARTESIAN_POINT ( 'NONE',  ( 97.33941792859064890, 238.5530062829863027, -4.648177544792955347E-16 ) ) ;
#49861=CARTESIAN_POINT ( 'NONE',  ( 50.89226983467786170, 194.0643266524160140, 9.188101187500095079 ) ) ;
#49862=CARTESIAN_POINT ( 'NONE',  ( 83.43119661263041564, 225.6427522451419065, -10.00000000000009415 ) ) ;
#49866=EDGE_CURVE ( 'NONE', #79979, #81112, #48511, .T. ) ;
#49867=CARTESIAN_POINT ( 'NONE',  ( 158.6735398351655988, 282.4669076978136104, -1.658533933206339350 ) ) ;
#49869=CARTESIAN_POINT ( 'NONE',  ( -12.49048504844327745, 175.8464784336661353, 1.353441290958777327E-15 ) ) ;
#49871=EDGE_CURVE ( 'NONE', #87863, #45170, #34491, .T. ) ;
#49873=CARTESIAN_POINT ( 'NONE',  ( 151.1230807375396807, 268.8941412966845519, -14.26613110909109849 ) ) ;
#49875=CARTESIAN_POINT ( 'NONE',  ( 192.4743214706506365, 297.2716913909250707, -12.17804856100553046 ) ) ;
#49877=CARTESIAN_POINT ( 'NONE',  ( 204.9432097630379417, 275.6749433546094679, 13.74700047688257776 ) ) ;
#49878=CARTESIAN_POINT ( 'NONE',  ( 68.51030059680894624, 220.3615022471903160, 5.000000000000046185 ) ) ;
#49882=( BOUNDED_CURVE ( )  B_SPLINE_CURVE ( 2, ( #56290, #87288, #92121, #51185, #45940, #58776, #50686, #11719, #22674 ),
 .UNSPECIFIED., .F., .T. ) 
 B_SPLINE_CURVE_WITH_KNOTS ( ( 3, 2, 2, 2, 3 ),
 ( 0.4233870967741935609, 0.4247311827956989361, 0.4274193548387096864, 0.4301075268817204367, 0.4314516129032258118 ),
 .UNSPECIFIED. ) 
 CURVE ( )  GEOMETRIC_REPRESENTATION_ITEM ( )  RATIONAL_B_SPLINE_CURVE ( ( 0.9330127018922194093, 0.9330127018922194093, 1.000000000000000000, 0.8660254037844387076, 1.000000000000000000, 0.8660254037844387076, 1.000000000000000000, 0.9330127018922194093, 0.9330127018922194093 ) ) 
 REPRESENTATION_ITEM ( '' )  );
#49883=CARTESIAN_POINT ( 'NONE',  ( -5.174027508517048624, 174.4865022471902876, 10.00000000000009237 ) ) ;
#49885=CARTESIAN_POINT ( 'NONE',  ( 118.1714448432989144, 239.0333772461660544, 9.188101187500095079 ) ) ;
#49888=CARTESIAN_POINT ( 'NONE',  ( -15.51451749852110495, 173.3967562850347406, 6.972266317189433612E-15 ) ) ;
#49891=CARTESIAN_POINT ( 'NONE',  ( 185.6268485153956362, 288.2895463531142468, 15.19883395034924156 ) ) ;
#49894=CARTESIAN_POINT ( 'NONE',  ( 191.4685399627163633, 299.0137560639802814, 7.545791216288330716 ) ) ;
#49895=CARTESIAN_POINT ( 'NONE',  ( 149.0598351764325002, 272.4677874370131576, -11.59078276432863674 ) ) ;
#49896=CARTESIAN_POINT ( 'NONE',  ( 190.2531537072969172, 300.2272130020738246, 3.269838540422708384 ) ) ;
#49897=CARTESIAN_POINT ( 'NONE',  ( 176.3276157809688698, 292.5524778291284065, -1.120248480450068307 ) ) ;
#49900=CARTESIAN_POINT ( 'NONE',  ( 139.9313959742916325, 240.0494855054051584, -2.679491924311248496 ) ) ;
#49901=CARTESIAN_POINT ( 'NONE',  ( 165.6308188219810802, 269.8697111906062673, -16.28193825780852677 ) ) ;
#49904=CARTESIAN_POINT ( 'NONE',  ( 200.2698671084199304, 272.3682649667838405, 12.72613294923287164 ) ) ;
#49905=CARTESIAN_POINT ( 'NONE',  ( 156.0412994658168202, 261.1582083806645755, 17.21098171226111262 ) ) ;
#49907=CARTESIAN_POINT ( 'NONE',  ( 152.9489295551198893, 265.7316783776963121, 17.71675637597311237 ) ) ;
#49910=CARTESIAN_POINT ( 'NONE',  ( 194.4672199338309895, 282.9685410809637460, 17.39323676395655127 ) ) ;
#49912=CARTESIAN_POINT ( 'NONE',  ( 174.2161637736558646, 273.0081352261942698, -16.36149965205150636 ) ) ;
#49913=ORIENTED_EDGE ( 'NONE', *, *, #12347, .F. ) ;
#49914=CARTESIAN_POINT ( 'NONE',  ( 164.3041378677445437, 280.0744590447591804, 12.54842942910348391 ) ) ;
#49915=ADVANCED_FACE ( 'NONE', ( #81440 ), #59279, .T. ) ;
#49916=CARTESIAN_POINT ( 'NONE',  ( 194.2900850603946310, 294.1266965989547657, -15.88613936555681505 ) ) ;
#49917=CARTESIAN_POINT ( 'NONE',  ( 159.7390991980013268, 264.1538480117934569, -17.57393616107441758 ) ) ;
#49926=CARTESIAN_POINT ( 'NONE',  ( 185.3516594888635041, 259.5148316134143442, -6.839491391714221713 ) ) ;
#49927=ORIENTED_EDGE ( 'NONE', *, *, #72657, .T. ) ;
#49928=ORIENTED_EDGE ( 'NONE', *, *, #46192, .T. ) ;
#49929=CARTESIAN_POINT ( 'NONE',  ( 179.0457787397059235, 259.9863029104557199, 12.57728703070772980 ) ) ;
#49930=VERTEX_POINT ( 'NONE', #49494 ) ;
#49934=CARTESIAN_POINT ( 'NONE',  ( 203.5080190724872011, 278.1607665491929993, -15.47044080916498743 ) ) ;
#49936=B_SPLINE_CURVE_WITH_KNOTS ( 'NONE', 3,
 ( #6588, #14680, #21293, #76490 ),
 .UNSPECIFIED., .F., .F.,
 ( 4, 4 ),
 ( 0.02883180965995480252, 0.03048461901537222879 ),
 .UNSPECIFIED. ) ;
#49937=CARTESIAN_POINT ( 'NONE',  ( 151.3011447763744570, 269.1990464485573966, 14.21186556778774168 ) ) ;
#49938=CARTESIAN_POINT ( 'NONE',  ( 162.0143107678314607, 277.5073529415977873, -13.05376659552506347 ) ) ;
#49939=CARTESIAN_POINT ( 'NONE',  ( 147.3715240516018810, 275.3920280842035595, -3.728968767617475866 ) ) ;
#49941=CARTESIAN_POINT ( 'NONE',  ( 201.2535035105529744, 282.0657020489176716, -18.08976065250591958 ) ) ;
#49944=CIRCLE ( 'NONE', #71000, 17.82106496071138935 ) ;
#49946=CARTESIAN_POINT ( 'NONE',  ( 137.1700506867025808, 243.8768266524160140, -9.188101187500091527 ) ) ;
#49952=CARTESIAN_POINT ( 'NONE',  ( 200.0230348527707918, 270.2077458102232299, 9.270856234837108190 ) ) ;
#49955=CARTESIAN_POINT ( 'NONE',  ( 181.4712052382458012, 255.0843802102731956, 0.8439431145092127773 ) ) ;
#49956=CARTESIAN_POINT ( 'NONE',  ( 171.0331961513450381, 287.8115977397300753, -5.235742780808191554 ) ) ;
#49957=CARTESIAN_POINT ( 'NONE',  ( 157.4266892601732764, 279.9775888384338600, -6.903949925214651451 ) ) ;
#49960=B_SPLINE_CURVE_WITH_KNOTS ( 'NONE', 3,
 ( #29255, #28749, #83990, #44435 ),
 .UNSPECIFIED., .F., .F.,
 ( 4, 4 ),
 ( 0.000000000000000000, 0.0002315650517813498070 ),
 .UNSPECIFIED. ) ;
#49961=CARTESIAN_POINT ( 'NONE',  ( 192.7136452730116787, 292.4147829832277807, -14.35829535037222549 ) ) ;
#49962=EDGE_CURVE ( 'NONE', #69383, #14295, #18108, .T. ) ;
#49967=CARTESIAN_POINT ( 'NONE',  ( 147.7467138384290308, 274.7421803109381813, -9.190172068879620682 ) ) ;
#49969=ORIENTED_EDGE ( 'NONE', *, *, #81979, .F. ) ;
#49970=CARTESIAN_POINT ( 'NONE',  ( 163.3780808840420207, 277.4266273750775440, 12.96822648644490350 ) ) ;
#49971=CARTESIAN_POINT ( 'NONE',  ( 156.1857201963304362, 277.6936791020598889, 10.39727624116721749 ) ) ;
#49973=CARTESIAN_POINT ( 'NONE',  ( 190.4841013044967042, 300.7188538369516095, 4.682298117523464143 ) ) ;
#49974=CARTESIAN_POINT ( 'NONE',  ( 203.0535368433499457, 278.9479528611958585, 16.46202213522710167 ) ) ;
#49975=CARTESIAN_POINT ( 'NONE',  ( 161.2233037901852697, 281.7567412870793078, -7.606728900846287722 ) ) ;
#49978=CARTESIAN_POINT ( 'NONE',  ( 161.5295548613449625, 262.2726132182542642, 17.75576853186118598 ) ) ;
#49988=CARTESIAN_POINT ( 'NONE',  ( 9.323050453024791295, 170.0643266524160140, 9.188101187500095079 ) ) ;
#49989=CARTESIAN_POINT ( 'NONE',  ( 113.4086522182495145, 224.0327760586659451, 1.948934522072303157E-15 ) ) ;
#49990=CARTESIAN_POINT ( 'NONE',  ( 154.9792334219179679, 262.2150889255981951, -17.21325849938693153 ) ) ;
#49992=CARTESIAN_POINT ( 'NONE',  ( 184.6829044896801690, 294.7002800362207608, -7.708189250272898363 ) ) ;
#49996=CARTESIAN_POINT ( 'NONE',  ( 147.9311236323648870, 274.4227731784279172, -7.799459659034405412 ) ) ;
#49997=CARTESIAN_POINT ( 'NONE',  ( 181.8064089908095013, 291.5401130331068771, 9.400625256126808438 ) ) ;
#49999=CARTESIAN_POINT ( 'NONE',  ( 180.4232100707751840, 278.0586175385776642, -17.62785496320838519 ) ) ;
#50000=CARTESIAN_POINT ( 'NONE',  ( 168.8221748259757931, 288.8596753763678180, 0.1258535561669744951 ) ) ;
#50002=CARTESIAN_POINT ( 'NONE',  ( 166.1124712730374711, 253.7145057436913191, -13.29400677092769101 ) ) ;
#50003=CARTESIAN_POINT ( 'NONE',  ( 176.1427204184975039, 265.6242702382210723, -16.01709430928111288 ) ) ;
#50005=CARTESIAN_POINT ( 'NONE',  ( 87.75264963113552596, 209.2202760586659167, -5.415160957724236172E-17 ) ) ;
#50006=CARTESIAN_POINT ( 'NONE',  ( 207.1019571622349815, 271.9358831784929293, -5.989975140547304733 ) ) ;
#50010=CARTESIAN_POINT ( 'NONE',  ( 151.8386188729356547, 267.6547928914259842, 15.62558980430495126 ) ) ;
#50013=CARTESIAN_POINT ( 'NONE',  ( 176.4203288667277718, 270.0400164863470991, -16.69789413301970882 ) ) ;
#50019=CARTESIAN_POINT ( 'NONE',  ( 76.27746593522670082, 214.8458772461660544, 9.188101187500095079 ) ) ;
#50020=CARTESIAN_POINT ( 'NONE',  ( 172.6419814482584059, 289.4122052211230880, -1.058254457564594464 ) ) ;
#50022=CARTESIAN_POINT ( 'NONE',  ( 188.6147648084645425, 286.2025555478231809, -16.06153253298101902 ) ) ;
#50024=CARTESIAN_POINT ( 'NONE',  ( 193.4694490986788082, 288.4501677614762229, 16.06150681008983483 ) ) ;
#50025=EDGE_CURVE ( 'NONE', #759, #66266, #11173, .T. ) ;
#50028=CARTESIAN_POINT ( 'NONE',  ( 125.2349645446897455, 233.1115022471901739, -5.000000000000041744 ) ) ;
#50032=CARTESIAN_POINT ( 'NONE',  ( 169.3476482064008337, 248.6764527704247882, -1.911158280328731474 ) ) ;
#50034=CARTESIAN_POINT ( 'NONE',  ( 162.6476498368881494, 248.9330020812748785, 10.75824100428386743 ) ) ;
#50035=CARTESIAN_POINT ( 'NONE',  ( 154.8332767207531901, 280.7459370637686220, -0.9958211956073632631 ) ) ;
#50036=EDGE_CURVE ( 'NONE', #69871, #38097, #17637, .T. ) ;
#50038=ORIENTED_EDGE ( 'NONE', *, *, #19988, .F. ) ;
#50041=CARTESIAN_POINT ( 'NONE',  ( 189.0767208543637139, 290.4732453595815969, 14.36254912788081839 ) ) ;
#50042=CARTESIAN_POINT ( 'NONE',  ( 51.36475398071000598, 188.9155109091896065, 2.679491924311254714 ) ) ;
#50043=CARTESIAN_POINT ( 'NONE',  ( 143.0153750664825054, 259.5024278399160949, -9.188101187500093303 ) ) ;
#50044=CARTESIAN_POINT ( 'NONE',  ( 201.2535035105529744, 282.0657020489176716, -18.08976065250591958 ) ) ;
#50045=AXIS2_PLACEMENT_3D ( 'NONE', #56484, #80334, #72725 ) ;
#50046=CARTESIAN_POINT ( 'NONE',  ( 112.5819247142704427, 224.2592609112379876, 2.679491924311254714 ) ) ;
#50049=CARTESIAN_POINT ( 'NONE',  ( 164.1286765816565207, 275.3158857940874782, 15.02251480813967888 ) ) ;
#50050=CARTESIAN_POINT ( 'NONE',  ( -22.42236680055709641, 157.8615022471902591, 0.000000000000000000 ) ) ;
#50052=VERTEX_POINT ( 'NONE', #91518 ) ;
#50053=CARTESIAN_POINT ( 'NONE',  ( 184.6801771164089416, 296.8040060832889253, 1.022975585509389163 ) ) ;
#50054=CARTESIAN_POINT ( 'NONE',  ( 204.5831314780710954, 276.2986172388744421, 13.28075685133257089 ) ) ;
#50056=CARTESIAN_POINT ( 'NONE',  ( 150.0694502760089222, 271.4680435213315945, -12.17790201236558545 ) ) ;
#50058=CARTESIAN_POINT ( 'NONE',  ( 161.9775247817796924, 252.0936927241524472, 14.33142805341373283 ) ) ;
#50059=CARTESIAN_POINT ( 'NONE',  ( 161.2535912560966551, 263.0844709175967182, -17.80682751047658030 ) ) ;
#50060=CARTESIAN_POINT ( 'NONE',  ( 164.7389676833716976, 245.3107333163898716, 5.284562706098457241 ) ) ;
#50061=CARTESIAN_POINT ( 'NONE',  ( 196.0587100571994483, 289.0633482449420626, -17.27351923437598913 ) ) ;
#50063=CARTESIAN_POINT ( 'NONE',  ( 102.2582280487598609, 229.8458772461660544, 9.188101187500095079 ) ) ;
#50065=CARTESIAN_POINT ( 'NONE',  ( 150.0102862277170743, 271.3788846064419999, 12.09021458032355056 ) ) ;
#50066=CARTESIAN_POINT ( 'NONE',  ( 117.3505249275209934, 231.8927522451417360, -10.00000000000009237 ) ) ;
#50069=CARTESIAN_POINT ( 'NONE',  ( 182.3292780454827096, 296.5739854331435481, -1.651664298513513041 ) ) ;
#50070=DIRECTION ( 'NONE',  ( -0.8660254037844387076, -0.4999999999999998890, -0.000000000000000000 ) ) ;
#50073=CARTESIAN_POINT ( 'NONE',  ( 206.9942764641839688, 270.1223916185117560, -3.431663675821580828 ) ) ;
#50074=CARTESIAN_POINT ( 'NONE',  ( 96.25000326212280299, 232.5024278399160664, -9.188101187500093303 ) ) ;
#50076=EDGE_CURVE ( 'NONE', #53637, #52411, #47378, .T. ) ;
#50078=CARTESIAN_POINT ( 'NONE',  ( 208.2124092825819162, 270.0125236866795149, -2.339659020816897694 ) ) ;
#50081=EDGE_CURVE ( 'NONE', #99571, #97906, #6307, .T. ) ;
#50082=VECTOR ( 'NONE', #77676, 1000.000000000000000 ) ;
#50083=CARTESIAN_POINT ( 'NONE',  ( 194.6143112939460309, 266.3039560675284179, -7.756514573897542064 ) ) ;
#50085=CARTESIAN_POINT ( 'NONE',  ( 129.7002344832967538, 251.8149278399160949, -9.188101187500095079 ) ) ;
#50088=DIRECTION ( 'NONE',  ( -0.5000000000000006661, 0.8660254037844382635, -1.877843081442121204E-16 ) ) ;
#50091=CARTESIAN_POINT ( 'NONE',  ( 204.9214210856886496, 275.7126824508080176, 13.23219655298346709 ) ) ;
#50092=CARTESIAN_POINT ( 'NONE',  ( 160.6921517183488390, 275.5961185789591354, 13.91821361452047334 ) ) ;
#50098=DIRECTION ( 'NONE',  ( -0.8660254037844387076, -0.4999999999999998890, -0.000000000000000000 ) ) ;
#50100=CARTESIAN_POINT ( 'NONE',  ( 172.7264208856190919, 290.8582626858774347, 2.771863430787652849 ) ) ;
#50102=CARTESIAN_POINT ( 'NONE',  ( 159.9531724557437826, 253.5999738052623229, -15.71074128491364874 ) ) ;
#50104=CARTESIAN_POINT ( 'NONE',  ( -12.91644128716779072, 174.8967562850347690, 1.347971487989956912E-14 ) ) ;
#50106=CARTESIAN_POINT ( 'NONE',  ( 189.8375740044709801, 294.2633537128526768, 13.17988706671251720 ) ) ;
#50110=CARTESIAN_POINT ( 'NONE',  ( 162.9203612012105111, 256.0174525517487609, 16.09041223595896852 ) ) ;
#50114=CARTESIAN_POINT ( 'NONE',  ( 203.3041373168503299, 278.5139001086923827, -16.61929732091214973 ) ) ;
#50115=CARTESIAN_POINT ( 'NONE',  ( 157.6418352378513816, 271.0230738774055226, -14.72348240588997825 ) ) ;
#50117=CARTESIAN_POINT ( 'NONE',  ( 161.1061647010182583, 251.6029326557136585, -13.56144933775657613 ) ) ;
#50118=CARTESIAN_POINT ( 'NONE',  ( 19.09298631340924501, 172.6423013555409796, -4.594050593750043987 ) ) ;
#50119=CARTESIAN_POINT ( 'NONE',  ( 207.3594494688759085, 271.0859767844725638, 2.519715249304678828 ) ) ;
#50123=CARTESIAN_POINT ( 'NONE',  ( 164.2647213391612979, 246.1321520798662164, -5.830872732487307530 ) ) ;
#50125=CARTESIAN_POINT ( 'NONE',  ( 33.40920844789697952, 190.0958772461660544, -9.188101187500095079 ) ) ;
#50128=CARTESIAN_POINT ( 'NONE',  ( 147.1199024702499969, 275.8278494473859723, 5.224467159276165340 ) ) ;
#50130=CARTESIAN_POINT ( 'NONE',  ( 199.5733002173658690, 267.3584479166742653, -6.689480323808837170 ) ) ;
#50131=CARTESIAN_POINT ( 'NONE',  ( 178.2475648503018704, 293.8761651525964567, 2.747118326088546336 ) ) ;
#50132=CARTESIAN_POINT ( 'NONE',  ( 179.5554748665543059, 278.7501255867640566, -17.25862896719455009 ) ) ;
#50136=B_SPLINE_CURVE_WITH_KNOTS ( 'NONE', 3,
 ( #15554, #77387, #43802, #22004 ),
 .UNSPECIFIED., .F., .F.,
 ( 4, 4 ),
 ( 0.03394374891021562091, 0.04279985253772465581 ),
 .UNSPECIFIED. ) ;
#50137=CARTESIAN_POINT ( 'NONE',  ( 84.96478326871331888, 219.8615022471902591, -10.00000000000009592 ) ) ;
#50138=CARTESIAN_POINT ( 'NONE',  ( 19.16720650933548953, 170.3262482093457777, 3.021315404115420679E-15 ) ) ;
#50139=CARTESIAN_POINT ( 'NONE',  ( 176.6775373737683879, 280.6285440243045741, 16.49000606930484736 ) ) ;
#50140=CARTESIAN_POINT ( 'NONE',  ( 44.31597619863101301, 187.2048013555409796, 4.594050593750051981 ) ) ;
#50142=CARTESIAN_POINT ( 'NONE',  ( 162.6641061006424138, 263.2818470139165470, 17.66040242672044869 ) ) ;
#50143=CARTESIAN_POINT ( 'NONE',  ( 146.9324727656309335, 276.1524872186338371, 3.813717745456558728 ) ) ;
#50144=AXIS2_PLACEMENT_3D ( 'NONE', #52789, #76134, #13329 ) ;
#50147=CARTESIAN_POINT ( 'NONE',  ( 167.6847463121813462, 285.6965240061992972, 7.996140646124640483 ) ) ;
#50148=CARTESIAN_POINT ( 'NONE',  ( 164.8251969117060298, 245.1613799118173063, -1.508678420156898348 ) ) ;
#50150=B_SPLINE_CURVE_WITH_KNOTS ( 'NONE', 3,
 ( #26257, #9054, #40431, #10559, #40923, #39922, #41434, #17658, #32842, #71870, #2468, #33348, #72375, #18156, #90083, #98162, #42912, #97667, #28235, #66249, #20652, #59111, #51540, #35840, #98666, #97185, #4959, #27751, #57633, #96686, #67232, #82502, #12558, #27256, #88610, #58139, #13066, #43925, #67741, #74865, #12057, #19177, #89119, #50049, #66734, #43433, #81002, #73360 ),
 .UNSPECIFIED., .F., .F.,
 ( 4, 2, 2, 2, 2, 2, 2, 2, 2, 2, 2, 2, 2, 2, 2, 2, 2, 2, 2, 2, 2, 2, 2, 4 ),
 ( 0.001113145979540773644, 0.001586597418653406784, 0.002060048857766039708, 0.002296774577322319415, 0.002533500296878601291, 0.002651863156656742663, 0.002770226016434883601, 0.003006951735991266091, 0.003480403175104027601, 0.003953854614216789978, 0.004900757492442405806, 0.005847660370668021634, 0.006321111809780829982, 0.006794563248893638330, 0.006912926108671802253, 0.006972107538560923246, 0.007031288968450044238, 0.007149651828228287091, 0.007268014688006530812, 0.007504740407563156163, 0.007741466127119781514, 0.007978191846676406865, 0.008214917566233031349, 0.008688369005346287255 ),
 .UNSPECIFIED. ) ;
#50152=CARTESIAN_POINT ( 'NONE',  ( 185.8221718112685039, 262.9784142112231393, 11.29663378258160655 ) ) ;
#50154=CARTESIAN_POINT ( 'NONE',  ( 174.2371165158130566, 257.1234833113948071, 11.35068822046578774 ) ) ;
#50158=CARTESIAN_POINT ( 'NONE',  ( 174.2468074326821181, 254.8252884221085992, 8.251842399806214701 ) ) ;
#50159=CARTESIAN_POINT ( 'NONE',  ( -27.42236680055714260, 166.5217562850347406, 1.224646799147364892E-15 ) ) ;
#50160=ORIENTED_EDGE ( 'NONE', *, *, #67139, .F. ) ;
#50162=CARTESIAN_POINT ( 'NONE',  ( 191.0900422946452011, 299.6693332556258724, 8.872191398975367349 ) ) ;
#50163=CARTESIAN_POINT ( 'NONE',  ( 177.5411558806154062, 255.6075609413517213, -6.847706546168232045 ) ) ;
#50168=CARTESIAN_POINT ( 'NONE',  ( 161.2133744761260061, 251.4172398781588811, -14.30368667312104058 ) ) ;
#50170=CARTESIAN_POINT ( 'NONE',  ( 186.5128128464827455, 296.3652354721813822, -8.829210103799347564 ) ) ;
#50176=CARTESIAN_POINT ( 'NONE',  ( 205.1300674467857164, 275.3512963525735131, -12.60245643603069610 ) ) ;
#50177=CARTESIAN_POINT ( 'NONE',  ( 117.0346129529493311, 244.5024278399160949, -9.188101187500093303 ) ) ;
#50178=CARTESIAN_POINT ( 'NONE',  ( 182.4502886106904214, 259.6876753163259650, 10.69873880494191631 ) ) ;
#50180=CARTESIAN_POINT ( 'NONE',  ( 164.4989226152910646, 245.7265035704120351, -6.575810094723514965 ) ) ;
#50184=CARTESIAN_POINT ( 'NONE',  ( 194.5725374088679871, 291.6374747806817140, -16.23208319182986870 ) ) ;
#50185=CARTESIAN_POINT ( 'NONE',  ( 70.10703493326258240, 211.2833772461660544, -9.188101187500095079 ) ) ;
#50186=CARTESIAN_POINT ( 'NONE',  ( 15.08735849730845402, 189.5177522451419065, 5.000000000000046185 ) ) ;
#50187=( BOUNDED_CURVE ( )  B_SPLINE_CURVE ( 2, ( #876, #76872, #71297, #70268, #24181, #38867, #8484, #54550, #69774 ),
 .UNSPECIFIED., .F., .T. ) 
 B_SPLINE_CURVE_WITH_KNOTS ( ( 3, 2, 2, 2, 3 ),
 ( 0.2540322580645161255, 0.2553763440860215006, 0.2580645161290322509, 0.2607526881720430012, 0.2620967741935483764 ),
 .UNSPECIFIED. ) 
 CURVE ( )  GEOMETRIC_REPRESENTATION_ITEM ( )  RATIONAL_B_SPLINE_CURVE ( ( 0.9330127018922194093, 0.9330127018922194093, 1.000000000000000000, 0.8660254037844387076, 1.000000000000000000, 0.8660254037844387076, 1.000000000000000000, 0.9330127018922194093, 0.9330127018922194093 ) ) 
 REPRESENTATION_ITEM ( '' )  );
#50188=CARTESIAN_POINT ( 'NONE',  ( 151.0715479399129606, 268.9833987204304435, 14.24612252017116987 ) ) ;
#50189=CARTESIAN_POINT ( 'NONE',  ( 150.8360166798673561, 269.3913508296000145, 13.81437070545826806 ) ) ;
#50190=CARTESIAN_POINT ( 'NONE',  ( 175.0975211258509603, 278.2292065890057984, 15.47011627292242508 ) ) ;
#50194=CARTESIAN_POINT ( 'NONE',  ( 203.3684377202211522, 278.4025285431072803, -16.56116267537666076 ) ) ;
#50196=CARTESIAN_POINT ( 'NONE',  ( 148.0654368686451221, 274.1901358290616031, 9.010908242870014462 ) ) ;
#50198=CARTESIAN_POINT ( 'NONE',  ( 161.3773209892555371, 251.1332761876949746, -14.50043705923759241 ) ) ;
#50200=CARTESIAN_POINT ( 'NONE',  ( 146.9700173529739970, 276.0874580858064746, -5.099093031535578469 ) ) ;
#50201=CARTESIAN_POINT ( 'NONE',  ( 199.6130415427998344, 283.1155522273526230, -17.53316870511595127 ) ) ;
#50202=CARTESIAN_POINT ( 'NONE',  ( 205.7639495959071212, 274.2533802642843170, 10.79039487422292432 ) ) ;
#50203=CARTESIAN_POINT ( 'NONE',  ( 152.3377091156085896, 270.0594875778499500, -14.54836364073420008 ) ) ;
#50204=CARTESIAN_POINT ( 'NONE',  ( 157.7255603307123408, 268.5163524934444013, 16.86592485641857309 ) ) ;
#50205=CARTESIAN_POINT ( 'NONE',  ( 167.4844004446328256, 256.4883897734646894, 13.70360325908868049 ) ) ;
#50207=CARTESIAN_POINT ( 'NONE',  ( 122.6094779419291712, 253.8464784336661353, 1.353441290958777327E-15 ) ) ;
#50212=CARTESIAN_POINT ( 'NONE',  ( 164.1259971043086239, 246.3724295028720519, 5.761669507629934905 ) ) ;
#50217=CARTESIAN_POINT ( 'NONE',  ( 165.1786760834411609, 247.4249377785339448, -5.585047393798932447 ) ) ;
#50218=CARTESIAN_POINT ( 'NONE',  ( 164.5379227956242687, 245.6589532765702870, -2.440899697315300987 ) ) ;
#50221=CARTESIAN_POINT ( 'NONE',  ( 27.01324999880465327, 179.7365022471902307, 10.00000000000009948 ) ) ;
#50223=CARTESIAN_POINT ( 'NONE',  ( 157.1269483542914998, 258.4951375425532092, -17.15328932028234377 ) ) ;
#50224=CARTESIAN_POINT ( 'NONE',  ( 174.4776468927544499, 252.1408974215496528, 3.505067343168197347 ) ) ;
#50226=CARTESIAN_POINT ( 'NONE',  ( 190.1751179328237242, 301.2540287353828035, 3.252640783176552475 ) ) ;
#50227=CARTESIAN_POINT ( 'NONE',  ( 154.2298868780514454, 279.0943400367102072, -1.589968555053201449 ) ) ;
#50228=CARTESIAN_POINT ( 'NONE',  ( 170.1001268420399697, 285.5941755235542701, -7.968252287399715250 ) ) ;
#50229=CARTESIAN_POINT ( 'NONE',  ( 206.8073682671177664, 270.4461261121818438, -4.970999383176901709 ) ) ;
#50231=CARTESIAN_POINT ( 'NONE',  ( 193.1495885362050160, 289.2521248809247254, 16.30406654585521053 ) ) ;
#50232=CARTESIAN_POINT ( 'NONE',  ( 136.7639277290221571, 249.7677522451418497, 10.00000000000009592 ) ) ;
#50235=CARTESIAN_POINT ( 'NONE',  ( 196.0355168007595523, 291.1035201434990540, 17.55377893960077884 ) ) ;
#50236=CARTESIAN_POINT ( 'NONE',  ( 147.7870527676176948, 274.6723112360602386, 9.257357958194809555 ) ) ;
#50237=CARTESIAN_POINT ( 'NONE',  ( -6.860972828079417773, 166.8458772461660544, 9.188101187500095079 ) ) ;
#50239=CARTESIAN_POINT ( 'NONE',  ( 31.29809797828990270, 195.0024278399160664, -9.188101187500093303 ) ) ;
#50243=LINE ( 'NONE', #89311, #96605 ) ;
#50244=CARTESIAN_POINT ( 'NONE',  ( 192.6136217801248449, 292.3795896600195761, -14.34082932734286508 ) ) ;
#50245=CARTESIAN_POINT ( 'NONE',  ( 190.1635032421960148, 301.2741459696644029, -5.047660290019184259 ) ) ;
#50247=CARTESIAN_POINT ( 'NONE',  ( 167.6162704737794229, 256.6000348849465240, 13.71821036101052371 ) ) ;
#50248=CARTESIAN_POINT ( 'NONE',  ( 66.61587002248261058, 209.2677522451418497, 10.00000000000009592 ) ) ;
#50253=CARTESIAN_POINT ( 'NONE',  ( 33.07542782529563397, 203.2365022471903444, 2.944929066748280225E-16 ) ) ;
#50254=CARTESIAN_POINT ( 'NONE',  ( 181.5004962646415265, 292.1248343589982710, 8.982815215163469702 ) ) ;
#50255=CARTESIAN_POINT ( 'NONE',  ( 203.0535368433499457, 278.9479528611958585, 16.46202213522710167 ) ) ;
#50256=CARTESIAN_POINT ( 'NONE',  ( -6.076397627723526540, 176.4869531367911293, 4.594050593750046652 ) ) ;
#50259=CARTESIAN_POINT ( 'NONE',  ( 192.2431834237441706, 297.6720342317289578, 11.07782187406058938 ) ) ;
#50261=CARTESIAN_POINT ( 'NONE',  ( 155.8365007042834520, 261.3224821757460177, -17.11083130380785633 ) ) ;
#50262=CARTESIAN_POINT ( 'NONE',  ( 179.3274614371453595, 277.6279536742436562, 17.03900687375964296 ) ) ;
#50263=CYLINDRICAL_SURFACE ( 'NONE', #77241, 17.82106496071139645 ) ;
#50264=CARTESIAN_POINT ( 'NONE',  ( 65.14187045721612890, 219.9637435831425023, 2.679491924311251605 ) ) ;
#50265=CARTESIAN_POINT ( 'NONE',  ( 177.6585084262452767, 260.6037935310539524, -13.90472577101287932 ) ) ;
#50269=CARTESIAN_POINT ( 'NONE',  ( 68.53065452504849020, 198.8262482093457777, 3.021315404115420679E-15 ) ) ;
#50270=CARTESIAN_POINT ( 'NONE',  ( 193.7114073116034945, 295.1289958610702797, 14.86160832869823345 ) ) ;
#50272=CARTESIAN_POINT ( 'NONE',  ( 155.6531420801174761, 275.9231362174812148, 10.30624812126558076 ) ) ;
#50274=CARTESIAN_POINT ( 'NONE',  ( 159.5895502557670795, 254.2297859303815244, -16.92708575547316485 ) ) ;
#50276=CARTESIAN_POINT ( 'NONE',  ( 192.2943420783192323, 297.5834248427583475, 12.53393473147773562 ) ) ;
#50277=CARTESIAN_POINT ( 'NONE',  ( 164.3524132573224392, 245.9802652221976587, -2.749586949851067441 ) ) ;
#50278=B_SPLINE_CURVE_WITH_KNOTS ( 'NONE', 3,
 ( #28295, #50110, #43494, #36392 ),
 .UNSPECIFIED., .F., .F.,
 ( 4, 4 ),
 ( 0.003801382972845887033, 0.008042818574261435469 ),
 .UNSPECIFIED. ) ;
#50283=CARTESIAN_POINT ( 'NONE',  ( 159.7762908497461467, 278.5220354493135915, -9.751953824713970320 ) ) ;
#50284=CARTESIAN_POINT ( 'NONE',  ( 164.1224127655298730, 246.3786377597482158, 7.356982420601481998 ) ) ;
#50285=CARTESIAN_POINT ( 'NONE',  ( 153.3100492430090753, 265.1062007306585997, 16.32434963471121492 ) ) ;
#50288=CARTESIAN_POINT ( 'NONE',  ( 178.0262838233909974, 263.6630881215525051, 15.29339064780925206 ) ) ;
#50292=CARTESIAN_POINT ( 'NONE',  ( 34.86956345232661647, 202.4860189848785978, -2.679491924311252493 ) ) ;
#50293=VERTEX_POINT ( 'NONE', #64961 ) ;
#50294=CARTESIAN_POINT ( 'NONE',  ( 161.4726291907278721, 250.9681975403669867, 14.52346149734912117 ) ) ;
#50295=CARTESIAN_POINT ( 'NONE',  ( 167.3161501383444261, 274.8626071502216064, -15.20120324154985880 ) ) ;
#50296=LINE ( 'NONE', #80765, #59064 ) ;
#50298=ADVANCED_FACE ( 'NONE', ( #22584 ), #53471, .F. ) ;
#50299=ADVANCED_FACE ( 'NONE', ( #5150 ), #42629, .T. ) ;
#50300=CARTESIAN_POINT ( 'NONE',  ( 177.3307538467140319, 279.0261758493545017, -15.97343219706607442 ) ) ;
#50301=CARTESIAN_POINT ( 'NONE',  ( 163.2437751800324293, 247.9004826992694461, 9.806027032984305336 ) ) ;
#50303=CARTESIAN_POINT ( 'NONE',  ( 157.1587696251558555, 266.8444457941050700, -16.20406809633236023 ) ) ;
#50310=CARTESIAN_POINT ( 'NONE',  ( 141.3286032983506004, 245.7365022471902307, 10.00000000000009948 ) ) ;
#50311=CARTESIAN_POINT ( 'NONE',  ( 193.1255195334355506, 295.1544621841915159, 13.26913244492654265 ) ) ;
#50313=EDGE_CURVE ( 'NONE', #77820, #33752, #50243, .T. ) ;
#50314=CARTESIAN_POINT ( 'NONE',  ( 197.3765505787902441, 288.7807815052838123, -16.66600386213448814 ) ) ;
#50317=ADVANCED_FACE ( 'NONE', ( #35544 ), #5304, .F. ) ;
#50320=CARTESIAN_POINT ( 'NONE',  ( 164.3022921857394749, 246.0670774647090582, 1.862798784958315856 ) ) ;
#50323=VERTEX_POINT ( 'NONE', #76067 ) ;
#50324=CARTESIAN_POINT ( 'NONE',  ( 187.0393956332045775, 276.8356235671391232, 16.76004927575691639 ) ) ;
#50325=CARTESIAN_POINT ( 'NONE',  ( 171.4620979185174292, 259.3841603946243595, -13.88139083577690869 ) ) ;
#50326=EDGE_CURVE ( 'NONE', #48318, #59756, #10538, .T. ) ;
#50329=CARTESIAN_POINT ( 'NONE',  ( 160.6249589658661137, 252.4364054378906985, -15.80515328853796042 ) ) ;
#50334=DIRECTION ( 'NONE',  ( 0.4999999999999998890, -0.8660254037844385966, 0.000000000000000000 ) ) ;
#50335=B_SPLINE_CURVE_WITH_KNOTS ( 'NONE', 3,
 ( #16372, #8774, #78186, #55841, #33583, #71594, #71094, #80215, #86329, #62445, #39644, #47264, #31556, #79720, #10282, #33073, #16868, #18385, #40152, #2189, #93918, #86836, #48276, #64476, #62969, #24471, #55351, #1693, #63966, #78691, #17370, #41153, #79223, #9279, #10784, #9796, #93413, #32577, #70057, #63473, #94909, #94410, #24964, #25471, #674, #72090 ),
 .UNSPECIFIED., .F., .F.,
 ( 4, 2, 2, 2, 2, 2, 2, 2, 2, 2, 2, 2, 2, 2, 2, 2, 2, 2, 2, 2, 2, 2, 4 ),
 ( 0.0002401535358040922863, 0.001257124250616875431, 0.001765609608023326581, 0.002019852286726482767, 0.002146973626077981062, 0.002274094965429479791, 0.002401216304780978521, 0.002528337644132477250, 0.002782580322835466902, 0.003291065680241447074, 0.004308036395053377494, 0.005325007109865307481, 0.005833492467271272908, 0.006087735145974259958, 0.006341977824677245273, 0.006405538494353034754, 0.006469099164028824234, 0.006532659833704612846, 0.006596220503380401459, 0.006850463182083436214, 0.007358948539489502255, 0.007867433896895570031, 0.008375919254301636072 ),
 .UNSPECIFIED. ) ;
#50336=CARTESIAN_POINT ( 'NONE',  ( 207.6826438088389750, 270.9301044032979462, 7.252082088659585146 ) ) ;
#50337=CARTESIAN_POINT ( 'NONE',  ( 22.44857442947618154, 193.7677522451419350, -5.000000000000047962 ) ) ;
#50338=CARTESIAN_POINT ( 'NONE',  ( 93.70588009062352342, 237.1589784336661637, -6.496448406907676862E-16 ) ) ;
#50340=CARTESIAN_POINT ( 'NONE',  ( 162.7678667286918142, 249.1757505475115977, -10.38966524845342754 ) ) ;
#50342=CARTESIAN_POINT ( 'NONE',  ( 207.6821401748263156, 270.9309767229963768, 1.759036204183980878 ) ) ;
#50343=CARTESIAN_POINT ( 'NONE',  ( 26.12944271915780448, 176.7048013555409796, 4.594050593750051981 ) ) ;
#50348=CARTESIAN_POINT ( 'NONE',  ( 185.5908111669773177, 260.2313112761727325, -5.804257864100332398 ) ) ;
#50349=CARTESIAN_POINT ( 'NONE',  ( 21.94339294393528306, 190.1427522451419350, 10.00000000000009415 ) ) ;
#50350=CARTESIAN_POINT ( 'NONE',  ( 190.5653282632609091, 300.5781646174276602, -5.775635208185608604 ) ) ;
#50351=FACE_OUTER_BOUND ( 'NONE', #45453, .T. ) ;
#50353=CARTESIAN_POINT ( 'NONE',  ( 182.3152758659521169, 284.3638893697801677, 14.89189215024058299 ) ) ;
#50355=CARTESIAN_POINT ( 'NONE',  ( 52.43496435911014686, 191.8923013555410080, 4.594050593750050204 ) ) ;
#50356=CARTESIAN_POINT ( 'NONE',  ( 92.59663213601577070, 224.2677522451418497, 10.00000000000009592 ) ) ;
#50357=ORIENTED_EDGE ( 'NONE', *, *, #35890, .F. ) ;
#50359=CARTESIAN_POINT ( 'NONE',  ( 179.1448022382906515, 259.4449191438238813, -10.30622490606055308 ) ) ;
#50361=CARTESIAN_POINT ( 'NONE',  ( 1.609577830863368586, 180.9244531367911577, -4.594050593750046652 ) ) ;
#50362=B_SPLINE_CURVE_WITH_KNOTS ( 'NONE', 3,
 ( #7430, #69230, #100160, #2353, #87004, #9440, #1848, #95086, #48440, #25649, #86498, #87518, #48946, #88004, #72261, #71255, #96083, #9952, #34239, #71758, #18552, #32730, #32231, #63634, #94077, #49432, #70734, #41826, #56531, #65135, #11466, #57524, #88500, #1345, #24629, #55510, #47919, #94571, #5339, #50428, #12450, #89017, #42321, #96585, #19568, #35231, #36220, #89492, #98046, #67123 ),
 .UNSPECIFIED., .F., .F.,
 ( 4, 2, 2, 2, 2, 2, 2, 2, 2, 2, 2, 2, 2, 2, 2, 2, 2, 2, 2, 2, 2, 2, 2, 2, 4 ),
 ( 0.0003511452654897985752, 0.0008110166299435485121, 0.001040952312170387783, 0.001270887994397226946, 0.001385855835510643600, 0.001500823676624060687, 0.001615791517737477341, 0.001730759358850894429, 0.001960695041077721665, 0.002190630723304548468, 0.002650502087758290978, 0.003110373452212033922, 0.004030116181119518942, 0.004949858910027003962, 0.005409730274480709609, 0.005639665956707606669, 0.005754633797821010095, 0.005869601638934414389, 0.005927085559491183757, 0.005984569480047953992, 0.006099537321161371296, 0.006329473003388079271, 0.006789344367841503892, 0.007249215732294928514, 0.007709087096748353136 ),
 .UNSPECIFIED. ) ;
#50364=CARTESIAN_POINT ( 'NONE',  ( 151.3681950933278983, 268.4695907787949523, -15.50699599486383917 ) ) ;
#50366=CARTESIAN_POINT ( 'NONE',  ( 146.7943851877206214, 276.3916619194686746, -4.608908220452185844 ) ) ;
#50371=CARTESIAN_POINT ( 'NONE',  ( 164.8251969117060298, 245.1613799118173063, -1.508678420156898348 ) ) ;
#50372=EDGE_LOOP ( 'NONE', ( #65754, #91895, #32742, #350, #43952 ) ) ;
#50374=CARTESIAN_POINT ( 'NONE',  ( 208.3135187673106543, 269.8373969220020285, 2.829653198597726682 ) ) ;
#50375=CARTESIAN_POINT ( 'NONE',  ( 0.9603191016227148324, 181.3615022471903444, 5.000000000000046185 ) ) ;
#50377=CARTESIAN_POINT ( 'NONE',  ( 122.2307653756559773, 247.5024278399160949, -9.188101187500093303 ) ) ;
#50380=EDGE_CURVE ( 'NONE', #90058, #71349, #70148, .T. ) ;
#50381=LINE ( 'NONE', #26598, #11233 ) ;
#50382=CARTESIAN_POINT ( 'NONE',  ( 157.8763546842245376, 257.1971277035954699, 17.68444922773363004 ) ) ;
#50386=CARTESIAN_POINT ( 'NONE',  ( 191.2729698983822288, 299.3524933518466469, 8.871011392605806734 ) ) ;
#50388=CARTESIAN_POINT ( 'NONE',  ( 190.4179675745853899, 261.7305499122562651, -6.837651125279566422 ) ) ;
#50389=CARTESIAN_POINT ( 'NONE',  ( 170.8539755607556856, 266.8602971898987448, -16.49407833488313102 ) ) ;
#50391=ORIENTED_EDGE ( 'NONE', *, *, #23185, .F. ) ;
#50393=CARTESIAN_POINT ( 'NONE',  ( 168.4118925024307316, 271.5375153668513803, -16.56645075760022223 ) ) ;
#50395=EDGE_CURVE ( 'NONE', #41928, #39162, #99883, .T. ) ;
#50398=CARTESIAN_POINT ( 'NONE',  ( 185.8564171466189805, 296.7006670448145655, 4.687756417891510985 ) ) ;
#50400=CARTESIAN_POINT ( 'NONE',  ( 149.0244553356880886, 274.5290671187512999, 9.114935767028397251 ) ) ;
#50403=CARTESIAN_POINT ( 'NONE',  ( 173.8216752892163868, 272.7590265814922077, -16.35953687348087726 ) ) ;
#50405=DIRECTION ( 'NONE',  ( 0.4999999999999998890, -0.8660254037844385966, 0.000000000000000000 ) ) ;
#50406=CARTESIAN_POINT ( 'NONE',  ( 148.1632261683078013, 274.0207597936089883, -7.853210555358286271 ) ) ;
#50408=ORIENTED_EDGE ( 'NONE', *, *, #86807, .T. ) ;
#50409=LINE ( 'NONE', #67102, #55543 ) ;
#50412=ORIENTED_EDGE ( 'NONE', *, *, #75861, .T. ) ;
#50413=CARTESIAN_POINT ( 'NONE',  ( 76.95378796010953693, 224.4244531367911293, -4.594050593750046652 ) ) ;
#50415=DIRECTION ( 'NONE',  ( 0.4999999999999992784, -0.8660254037844390407, 0.000000000000000000 ) ) ;
#50416=CARTESIAN_POINT ( 'NONE',  ( 185.4773086304266485, 259.3004018688347969, -6.871889497688444592 ) ) ;
#50418=ADVANCED_FACE ( 'NONE', ( #18247 ), #52209, .F. ) ;
#50420=CARTESIAN_POINT ( 'NONE',  ( 207.2604828555043639, 270.4328560034130646, 1.704576742114322974 ) ) ;
#50421=ORIENTED_EDGE ( 'NONE', *, *, #5026, .T. ) ;
#50422=CARTESIAN_POINT ( 'NONE',  ( 177.5830009069409243, 288.2251281501418703, -12.31337555878815593 ) ) ;
#50424=DIRECTION ( 'NONE',  ( -0.8660254037844387076, -0.4999999999999998890, -0.000000000000000000 ) ) ;
#50425=CARTESIAN_POINT ( 'NONE',  ( 155.2193237801463113, 261.7992402267395846, -18.58295809893692407 ) ) ;
#50428=CARTESIAN_POINT ( 'NONE',  ( 182.7415947523957414, 280.1175424322439653, -16.15561972179322581 ) ) ;
#50431=CARTESIAN_POINT ( 'NONE',  ( 160.0082391144745770, 275.8370785871085218, -12.54704109973508430 ) ) ;
#50432=CARTESIAN_POINT ( 'NONE',  ( 152.6740002182599767, 266.2078699576288159, -17.16212636348624088 ) ) ;
#50434=CARTESIAN_POINT ( 'NONE',  ( 11.37297787527554327, 165.8262482093457777, 3.021315404115420679E-15 ) ) ;
#50435=EDGE_CURVE ( 'NONE', #7044, #45081, #58150, .T. ) ;
#50436=CARTESIAN_POINT ( 'NONE',  ( 139.3894143317827172, 239.0327760586659736, 1.948934522072303157E-15 ) ) ;
#50445=CARTESIAN_POINT ( 'NONE',  ( -3.532187684056935062, 168.7677522451418781, 10.00000000000009592 ) ) ;
#50447=CARTESIAN_POINT ( 'NONE',  ( 171.0538495004223876, 287.7798256178718361, -5.161094478304363520 ) ) ;
#50448=CARTESIAN_POINT ( 'NONE',  ( 156.3189285634391297, 279.5595592535279934, 7.576391211794518910 ) ) ;
#50449=CARTESIAN_POINT ( 'NONE',  ( 165.5268399678854507, 246.9190504269991777, -1.962147731062478861 ) ) ;
#50450=CARTESIAN_POINT ( 'NONE',  ( 171.0551658227854830, 280.8129418237058985, 14.02084244714893302 ) ) ;
#50451=CARTESIAN_POINT ( 'NONE',  ( 170.4855375986076638, 248.6613294790634541, -0.2716024841417116753 ) ) ;
#50452=CARTESIAN_POINT ( 'NONE',  ( 194.0301671551565335, 292.9381004227619201, 15.31542839880081708 ) ) ;
#50453=ORIENTED_EDGE ( 'NONE', *, *, #31342, .F. ) ;
#50454=CARTESIAN_POINT ( 'NONE',  ( 196.1714484216475114, 286.8573191425118125, -17.65736119903840873 ) ) ;
#50457=CARTESIAN_POINT ( 'NONE',  ( 161.3479856134717636, 276.1092341099754321, 12.81212134750285081 ) ) ;
#50458=CARTESIAN_POINT ( 'NONE',  ( 205.1121091515972523, 269.0638940746846970, -3.021909147741778323 ) ) ;
#50461=CARTESIAN_POINT ( 'NONE',  ( 164.6727963122121423, 274.3640629835949198, 16.11238128926960655 ) ) ;
#50464=CARTESIAN_POINT ( 'NONE',  ( 203.7017578282252828, 269.5031481065263961, 5.505061929047487368 ) ) ;
#50468=CARTESIAN_POINT ( 'NONE',  ( 170.3178023250738420, 289.0326318653803241, -4.561300590322002080 ) ) ;
#50470=( BOUNDED_CURVE ( )  B_SPLINE_CURVE ( 2, ( #93130, #23679, #63196, #94136, #85555, #24692, #47000, #17090, #47983 ),
 .UNSPECIFIED., .F., .T. ) 
 B_SPLINE_CURVE_WITH_KNOTS ( ( 3, 2, 2, 2, 3 ),
 ( 0.04435483870967742159, 0.04569892473118279674, 0.04838709677419354704, 0.05107526881720430428, 0.05241935483870967943 ),
 .UNSPECIFIED. ) 
 CURVE ( )  GEOMETRIC_REPRESENTATION_ITEM ( )  RATIONAL_B_SPLINE_CURVE ( ( 0.9330127018922194093, 0.9330127018922194093, 1.000000000000000000, 0.8660254037844387076, 1.000000000000000000, 0.8660254037844387076, 1.000000000000000000, 0.9330127018922194093, 0.9330127018922194093 ) ) 
 REPRESENTATION_ITEM ( '' )  );
#50472=CARTESIAN_POINT ( 'NONE',  ( 47.29267820409023670, 198.1115022471902591, 10.00000000000009592 ) ) ;
#50473=CARTESIAN_POINT ( 'NONE',  ( -3.153561889951042474, 178.1744531367911577, 4.594050593750047540 ) ) ;
#50474=CARTESIAN_POINT ( 'NONE',  ( 112.9213393807382886, 229.8768266524160140, 9.188101187500098632 ) ) ;
#50475=CARTESIAN_POINT ( 'NONE',  ( 203.4682009197399566, 278.2297336128146412, -15.36039508894693206 ) ) ;
#50477=CARTESIAN_POINT ( 'NONE',  ( 183.2060477292669702, 294.1525339459620909, -7.844440212064340834 ) ) ;
#50478=CARTESIAN_POINT ( 'NONE',  ( 190.4356836585210431, 300.3996184492839916, -0.5836641476860114919 ) ) ;
#50480=CARTESIAN_POINT ( 'NONE',  ( 197.5165420832383063, 285.5553545344866393, 17.81061140909387674 ) ) ;
#50481=CARTESIAN_POINT ( 'NONE',  ( 160.3874973637684036, 282.4990615666047233, 5.130977648321134232 ) ) ;
#50482=CARTESIAN_POINT ( 'NONE',  ( 194.4032909867620447, 293.9306181827685123, -16.05392006271526384 ) ) ;
#50484=CARTESIAN_POINT ( 'NONE',  ( 86.26382137439000530, 210.6115022471902023, -5.000000000000041744 ) ) ;
#50485=CARTESIAN_POINT ( 'NONE',  ( 165.9388254541857179, 253.6912615456542994, -13.21544657617518403 ) ) ;
#50487=CARTESIAN_POINT ( 'NONE',  ( 175.9503686591639280, 265.5728256660283932, -15.87756521623894379 ) ) ;
#50488=CARTESIAN_POINT ( 'NONE',  ( 73.73334276372743545, 219.5024278399160664, 9.188101187500095079 ) ) ;
#50491=EDGE_CURVE ( 'NONE', #87238, #65763, #9730, .T. ) ;
#50493=CARTESIAN_POINT ( 'NONE',  ( 157.7365441389748923, 257.4392866714015895, 18.13124212464487073 ) ) ;
#50494=CARTESIAN_POINT ( 'NONE',  ( 151.7175356514093778, 267.8645151830532996, 16.34156987408047357 ) ) ;
#50495=CARTESIAN_POINT ( 'NONE',  ( 199.1526122334580862, 285.7045524820243259, -17.32174362185583050 ) ) ;
#50496=CARTESIAN_POINT ( 'NONE',  ( 173.3473246007907846, 267.7778430732650463, -16.37773085552635166 ) ) ;
#50502=B_SPLINE_CURVE_WITH_KNOTS ( 'NONE', 3,
 ( #20253, #83577, #22230, #91172, #21735, #52619 ),
 .UNSPECIFIED., .F., .F.,
 ( 4, 2, 4 ),
 ( 0.01896109736145757188, 0.02348162480702983140, 0.02800215225260209440 ),
 .UNSPECIFIED. ) ;
#50503=CARTESIAN_POINT ( 'NONE',  ( 173.0805693784550101, 289.6645751659409029, -1.032230538571357936 ) ) ;
#50505=CARTESIAN_POINT ( 'NONE',  ( 191.7410529245223358, 288.0106247083093081, -15.82820023231783857 ) ) ;
#50510=CARTESIAN_POINT ( 'NONE',  ( 154.6022411851589311, 267.2721739202577851, 16.02776763618498990 ) ) ;
#50512=CARTESIAN_POINT ( 'NONE',  ( 144.6483673461909518, 240.9865022471901455, 1.119607411625061291E-15 ) ) ;
#50513=CARTESIAN_POINT ( 'NONE',  ( 204.7237927799493775, 276.0549847173622879, -12.81020997223575364 ) ) ;
#50516=CARTESIAN_POINT ( 'NONE',  ( 169.0920981158736538, 248.6540344453142097, -1.899181296268086294 ) ) ;
#50518=CARTESIAN_POINT ( 'NONE',  ( 163.3543347837650686, 247.7089878483399730, 10.92686688779373405 ) ) ;
#50521=CARTESIAN_POINT ( 'NONE',  ( 173.8805019302338621, 250.6242863632701585, 0.4030408839048176262 ) ) ;
#50522=ORIENTED_EDGE ( 'NONE', *, *, #90380, .T. ) ;
#50523=CARTESIAN_POINT ( 'NONE',  ( 192.8119174027878273, 292.5372173574173758, 15.34371058135056209 ) ) ;
#50524=CARTESIAN_POINT ( 'NONE',  ( 206.1123153341301304, 273.6499931060659492, 10.83704338634689002 ) ) ;
#50525=CARTESIAN_POINT ( 'NONE',  ( 147.8871150585349881, 250.0643266524159287, -9.188101187500093303 ) ) ;
#50526=B_SPLINE_CURVE_WITH_KNOTS ( 'NONE', 3,
 ( #40940, #81023, #19687, #71885, #2483, #50065, #33365, #18173, #18678, #95218, #56661, #3002, #80512, #49075 ),
 .UNSPECIFIED., .F., .F.,
 ( 4, 2, 2, 2, 2, 2, 4 ),
 ( 0.001362149104930265647, 0.001570548566876670557, 0.001778948028823075685, 0.001987347490769480595, 0.002195746952715885505, 0.002612545876608731322, 0.003029344800501577138 ),
 .UNSPECIFIED. ) ;
#50528=CARTESIAN_POINT ( 'NONE',  ( 192.9518127100452034, 296.0217619941561793, -12.12386602825073645 ) ) ;
#50530=CARTESIAN_POINT ( 'NONE',  ( 184.5123196318015459, 277.1383014161853566, -17.82024832176989904 ) ) ;
#50532=CARTESIAN_POINT ( 'NONE',  ( 52.94219725692860834, 189.8262482093458061, 3.021315404115420679E-15 ) ) ;
#50536=ADVANCED_FACE ( 'NONE', ( #37944 ), #92222, .T. ) ;
#50537=CARTESIAN_POINT ( 'NONE',  ( 204.7235752877335244, 276.0553614249301972, 14.82397698933823271 ) ) ;
#50540=CARTESIAN_POINT ( 'NONE',  ( 154.9683083969241011, 262.2340116239618055, 18.33261662430134109 ) ) ;
#50542=CARTESIAN_POINT ( 'NONE',  ( 187.1789365411204926, 291.3781964708418286, -14.15416893886036220 ) ) ;
#50543=CARTESIAN_POINT ( 'NONE',  ( 207.3573038884736377, 271.4936096751011974, -4.269021768143928419 ) ) ;
#50547=CARTESIAN_POINT ( 'NONE',  ( 98.36111373172988692, 227.5958772461660260, -9.188101187500095079 ) ) ;
#50550=CARTESIAN_POINT ( 'NONE',  ( 163.0703755039977239, 276.5390454317725926, -13.97308584741530346 ) ) ;
#50554=CARTESIAN_POINT ( 'NONE',  ( 187.3985626036974281, 299.4490219941366149, -2.047446009836666025 ) ) ;
#50557=B_SPLINE_SURFACE_WITH_KNOTS ( 'NONE', 3, 1, ( 
 ( #92471, #74775 ),
 ( #67142, #98063 ),
 ( #59522, #21074 ),
 ( #51950, #82890 ),
 ( #92959, #93474 ),
 ( #94470, #8338 ),
 ( #38721, #85381 ),
 ( #77233, #9338 ),
 ( #39698, #32633 ),
 ( #23512, #69627 ),
 ( #63530, #55407 ),
 ( #70116, #94979 ),
 ( #1755, #727 ),
 ( #8829, #53911 ),
 ( #236, #70628 ),
 ( #63031, #31613 ),
 ( #64035, #62507 ),
 ( #48341, #71664 ),
 ( #86898, #9860 ),
 ( #47324, #31118 ),
 ( #24026, #62008 ),
 ( #25024, #86393 ),
 ( #54925, #54405 ),
 ( #84870, #85903 ),
 ( #55905, #2254 ),
 ( #93975, #15926 ),
 ( #79287, #46832 ),
 ( #78250, #16427 ),
 ( #77753, #71156 ),
 ( #7840, #39207 ),
 ( #40209, #24528 ),
 ( #1238, #32121 ),
 ( #16925, #47813 ),
 ( #17433, #78750 ) ),
 .UNSPECIFIED., .T., .F., .F.,
 ( 4, 2, 2, 2, 2, 2, 2, 2, 2, 2, 2, 2, 2, 2, 2, 2, 4 ),
 ( 2, 2 ),
 ( 0.000000000000000000, 0.06250000000000000000, 0.1250000000000000000, 0.1875000000000000000, 0.2500000000000000000, 0.3125000000000000000, 0.3750000000000000000, 0.4375000000000000000, 0.5000000000000000000, 0.5625000000000000000, 0.6250000000000000000, 0.6875000000000000000, 0.7500000000000000000, 0.8125000000000000000, 0.8750000000000000000, 0.9375000000000000000, 1.000000000000000000 ),
 ( 0.000000000000000000, 1.000000000000000000 ),
 .UNSPECIFIED. ) ;
#50558=CARTESIAN_POINT ( 'NONE',  ( 177.0591519751789633, 293.1615183139489886, -2.811523650733721791 ) ) ;
#50559=CARTESIAN_POINT ( 'NONE',  ( 164.2415456882844467, 249.8884775249601375, 10.08728766743346661 ) ) ;
#50560=CARTESIAN_POINT ( 'NONE',  ( 206.8851632406098702, 272.3113812655195716, -9.957011741946159233 ) ) ;
#50562=CARTESIAN_POINT ( 'NONE',  ( 88.83448719433606300, 234.3464784336661353, 1.353441290958777327E-15 ) ) ;
#50564=B_SPLINE_CURVE_WITH_KNOTS ( 'NONE', 3,
 ( #90088, #68229, #51544, #52046, #13069, #82984 ),
 .UNSPECIFIED., .F., .F.,
 ( 4, 2, 4 ),
 ( 0.02200203206105470419, 0.02659844398923805545, 0.03119485591742140670 ),
 .UNSPECIFIED. ) ;
#50566=CARTESIAN_POINT ( 'NONE',  ( 207.5959034698703078, 271.0803430774575418, -1.830000129038042544 ) ) ;
#50567=ORIENTED_EDGE ( 'NONE', *, *, #13120, .T. ) ;
#50569=CARTESIAN_POINT ( 'NONE',  ( 192.6872782779862234, 265.0988251606153199, -7.785220727510485439 ) ) ;
#50570=CARTESIAN_POINT ( 'NONE',  ( 153.8831531307005207, 265.2158041805028006, 16.69057008619190441 ) ) ;
#50572=CARTESIAN_POINT ( 'NONE',  ( 139.3894143317827172, 239.0327760586659736, 1.948934522072303157E-15 ) ) ;
#50573=CARTESIAN_POINT ( 'NONE',  ( 199.9089016888823664, 283.9562045477092056, 16.92683867318715585 ) ) ;
#50574=CARTESIAN_POINT ( 'NONE',  ( -10.02737821244022776, 165.0177522451418781, -10.00000000000009592 ) ) ;
#50577=CARTESIAN_POINT ( 'NONE',  ( 204.5773065883323056, 276.3087062438502812, 13.12907315817041187 ) ) ;
#50579=CARTESIAN_POINT ( 'NONE',  ( 206.4640281786353171, 273.0408085897082060, -10.81921452789957883 ) ) ;
#50581=CARTESIAN_POINT ( 'NONE',  ( 36.39519187313601378, 198.4865022471903160, 10.00000000000009415 ) ) ;
#50583=CARTESIAN_POINT ( 'NONE',  ( 199.0871366603265642, 281.9144776629251510, -16.60803299114443732 ) ) ;
#50584=CARTESIAN_POINT ( 'NONE',  ( 131.0005090013125084, 234.8932355074535394, -2.679491924311248496 ) ) ;
#50586=CARTESIAN_POINT ( 'NONE',  ( 206.7740269583881059, 271.5600005004544641, 6.228629494778278541 ) ) ;
#50587=CARTESIAN_POINT ( 'NONE',  ( 190.2629546459234859, 273.4080951500121159, -16.67925241984795903 ) ) ;
#50589=CARTESIAN_POINT ( 'NONE',  ( 162.6257765080958677, 248.9708877980734485, -10.42859054881151160 ) ) ;
#50590=B_SPLINE_CURVE_WITH_KNOTS ( 'NONE', 3,
 ( #77772, #33152, #15947, #9877 ),
 .UNSPECIFIED., .F., .F.,
 ( 4, 4 ),
 ( 0.02382166921119689001, 0.03306032650752911001 ),
 .UNSPECIFIED. ) ;
#50591=EDGE_CURVE ( 'NONE', #46582, #15352, #10988, .T. ) ;
#50592=CARTESIAN_POINT ( 'NONE',  ( 163.1628776802707534, 248.0406012790621446, -11.41865110901116331 ) ) ;
#50594=B_SPLINE_CURVE_WITH_KNOTS ( 'NONE', 3,
 ( #11384, #3277, #42234, #73173 ),
 .UNSPECIFIED., .F., .F.,
 ( 4, 4 ),
 ( 0.000000000000000000, 0.003125900356142441959 ),
 .UNSPECIFIED. ) ;
#50595=CARTESIAN_POINT ( 'NONE',  ( 185.0497311390575703, 266.3498828813088153, 13.18479497404900869 ) ) ;
#50599=CARTESIAN_POINT ( 'NONE',  ( 174.9358745049650565, 292.2217799751211942, 2.235529367806339263 ) ) ;
#50600=CARTESIAN_POINT ( 'NONE',  ( 157.6009339926387725, 270.9537869527873681, -14.75016313519251376 ) ) ;
#50602=CARTESIAN_POINT ( 'NONE',  ( 20.74358691754956396, 182.7833772461660544, -9.188101187500095079 ) ) ;
#50604=ORIENTED_EDGE ( 'NONE', *, *, #18119, .T. ) ;
#50607=CARTESIAN_POINT ( 'NONE',  ( 37.65788526339063225, 201.7369531367911293, -4.594050593750048428 ) ) ;
#50610=CARTESIAN_POINT ( 'NONE',  ( 146.8516045228164160, 276.2925551239072774, 3.995954059407343273 ) ) ;
#50612=CARTESIAN_POINT ( 'NONE',  ( 201.6080342170015456, 269.2650188364875703, -6.427773377030693069 ) ) ;
#50613=CARTESIAN_POINT ( 'NONE',  ( 191.0478321355427624, 299.7424433957868928, -9.006798842970001218 ) ) ;
#50616=CARTESIAN_POINT ( 'NONE',  ( 86.02927282398376008, 227.1427522451419634, -10.00000000000009592 ) ) ;
#50617=AXIS2_PLACEMENT_3D ( 'NONE', #3679, #58829, #75068 ) ;
#50620=EDGE_CURVE ( 'NONE', #79192, #84750, #35176, .T. ) ;
#50623=CARTESIAN_POINT ( 'NONE',  ( 92.68684311912460316, 210.9865022471901455, 1.119607411625061291E-15 ) ) ;
#50627=CARTESIAN_POINT ( 'NONE',  ( 37.65788526339063225, 201.7369531367911293, -4.594050593750048428 ) ) ;
#50628=ORIENTED_EDGE ( 'NONE', *, *, #28954, .F. ) ;
#50630=CARTESIAN_POINT ( 'NONE',  ( 198.4860348845112981, 286.8590983175747056, -18.20461732983060088 ) ) ;
#50632=ORIENTED_EDGE ( 'NONE', *, *, #99796, .F. ) ;
#50634=CARTESIAN_POINT ( 'NONE',  ( 171.2817005452050694, 286.5486442799788733, 7.499153033049632100 ) ) ;
#50635=CARTESIAN_POINT ( 'NONE',  ( 164.9779129355220562, 244.8968679994381148, -1.771286574179712803 ) ) ;
#50638=CARTESIAN_POINT ( 'NONE',  ( 189.7727577176825946, 264.4083146814396628, 11.16063339008121247 ) ) ;
#50639=CARTESIAN_POINT ( 'NONE',  ( 149.6148422561466305, 277.4437614652936190, 3.137689077364430368 ) ) ;
#50640=CARTESIAN_POINT ( 'NONE',  ( 171.4377511654674606, 255.6847064655358110, 11.24916129175043977 ) ) ;
#50641=VERTEX_POINT ( 'NONE', #56145 ) ;
#50645=CARTESIAN_POINT ( 'NONE',  ( 156.6812872898450735, 261.2670451491295012, 0.000000000000000000 ) ) ;
#50647=CARTESIAN_POINT ( 'NONE',  ( 182.4728335610948875, 284.0645720853299281, 16.33027959180494548 ) ) ;
#50648=DIRECTION ( 'NONE',  ( 0.4999999999999998890, -0.8660254037844385966, 0.000000000000000000 ) ) ;
#50649=DIRECTION ( 'NONE',  ( -0.8660254037844387076, -0.4999999999999998890, -0.000000000000000000 ) ) ;
#50650=ORIENTED_EDGE ( 'NONE', *, *, #79346, .T. ) ;
#50653=CARTESIAN_POINT ( 'NONE',  ( 161.7767236248226084, 250.4414905302161287, -13.15904643207033153 ) ) ;
#50654=DIRECTION ( 'NONE',  ( -0.8660254037844387076, -0.4999999999999998890, -0.000000000000000000 ) ) ;
#50655=CARTESIAN_POINT ( 'NONE',  ( 196.3507576896697344, 290.5575069072837664, -17.68249398312240928 ) ) ;
#50658=CARTESIAN_POINT ( 'NONE',  ( 198.0006249058153003, 287.6998530631771587, 18.31850453277666801 ) ) ;
#50661=CARTESIAN_POINT ( 'NONE',  ( 198.0442595703406141, 286.6951278662819504, 16.97370723237650481 ) ) ;
#50662=CARTESIAN_POINT ( 'NONE',  ( 125.1810982770029881, 233.8923013555409796, 4.594050593750050204 ) ) ;
#50663=CARTESIAN_POINT ( 'NONE',  ( 164.2712161151136172, 246.1209027979328710, 7.276091357954241445 ) ) ;
#50664=CARTESIAN_POINT ( 'NONE',  ( 185.7745234481418777, 262.1685992436391075, 11.32557499152616032 ) ) ;
#50666=CARTESIAN_POINT ( 'NONE',  ( 207.6932907333322191, 270.9116633891313199, 2.120963121341169710 ) ) ;
#50670=CARTESIAN_POINT ( 'NONE',  ( 204.7736914288410048, 274.4078475787994194, -12.22241593628383960 ) ) ;
#50671=CARTESIAN_POINT ( 'NONE',  ( 78.84873917453550973, 207.1423013555409796, -4.594050593750043987 ) ) ;
#50673=CARTESIAN_POINT ( 'NONE',  ( 117.9459173961706995, 232.2365022471902307, 10.00000000000009948 ) ) ;
#50674=CARTESIAN_POINT ( 'NONE',  ( 193.7999837595647250, 294.9755769528473479, 15.24609078262870199 ) ) ;
#50675=CARTESIAN_POINT ( 'NONE',  ( 175.8504680664171360, 278.0623914581425993, 16.26995051269672743 ) ) ;
#50678=B_SPLINE_CURVE_WITH_KNOTS ( 'NONE', 3,
 ( #14009, #68192, #22601, #45873 ),
 .UNSPECIFIED., .F., .F.,
 ( 4, 4 ),
 ( 0.004396866609976072399, 0.01239144977271805503 ),
 .UNSPECIFIED. ) ;
#50680=CARTESIAN_POINT ( 'NONE',  ( 203.5477091018662748, 278.0920214017542662, -16.09930363698006062 ) ) ;
#50682=CARTESIAN_POINT ( 'NONE',  ( 148.6952969693375337, 273.0991861330020924, 9.368475775849525178 ) ) ;
#50684=CARTESIAN_POINT ( 'NONE',  ( 163.9376361691041382, 260.4867098386596354, -16.17183962581199808 ) ) ;
#50685=CARTESIAN_POINT ( 'NONE',  ( 206.5733357898135978, 270.6748578492084789, 2.446890652106714636 ) ) ;
#50686=CARTESIAN_POINT ( 'NONE',  ( 60.98670489788378291, 196.0177522451417929, 5.000000000000051514 ) ) ;
#50688=CARTESIAN_POINT ( 'NONE',  ( 176.9854258871597779, 269.8460570511770129, 17.36332301788626609 ) ) ;
#50690=CARTESIAN_POINT ( 'NONE',  ( 165.0087721269838710, 244.8434183119457543, 2.604344609212914108 ) ) ;
#50692=CARTESIAN_POINT ( 'NONE',  ( 163.8455942243524248, 246.8581015375447691, -7.178103170949780676 ) ) ;
#50693=CARTESIAN_POINT ( 'NONE',  ( 132.2986577904150920, 241.0643266524159856, -9.188101187500093303 ) ) ;
#50698=CARTESIAN_POINT ( 'NONE',  ( 155.3716771045260714, 261.5353565282119348, -18.54934131471355840 ) ) ;
#50706=FACE_OUTER_BOUND ( 'NONE', #19760, .T. ) ;
#50707=CARTESIAN_POINT ( 'NONE',  ( 38.60642373151230800, 181.5494855054051868, -2.679491924311248496 ) ) ;
#50708=CARTESIAN_POINT ( 'NONE',  ( 160.8697417715285951, 254.0124291816641176, 15.72951850990217437 ) ) ;
#50713=CARTESIAN_POINT ( 'NONE',  ( 204.9184781223158609, 275.7177798128946620, -12.59106622113254126 ) ) ;
#50714=CARTESIAN_POINT ( 'NONE',  ( 192.1278788183472841, 297.0771818909656190, 10.94873614883879576 ) ) ;
#50716=CARTESIAN_POINT ( 'NONE',  ( 190.4249800432324662, 300.8212548652687133, 3.085047376053959400 ) ) ;
#50717=CARTESIAN_POINT ( 'NONE',  ( 75.70913676221920241, 214.5177522451418497, -10.00000000000009592 ) ) ;
#50718=CARTESIAN_POINT ( 'NONE',  ( 172.5844283141995845, 287.5847935883521131, -8.232867506822959314 ) ) ;
#50719=CARTESIAN_POINT ( 'NONE',  ( 155.3250150347760723, 261.6161776038049425, -18.57420904020362684 ) ) ;
#50720=CARTESIAN_POINT ( 'NONE',  ( 193.3367189744437837, 288.9287801845792956, 16.05736209422542871 ) ) ;
#50721=CARTESIAN_POINT ( 'NONE',  ( 125.8664413980679342, 250.1427522451419350, 10.00000000000009237 ) ) ;
#50722=CARTESIAN_POINT ( 'NONE',  ( 183.2938132151843149, 279.0290616485760893, 17.21975379680048235 ) ) ;
#50723=ORIENTED_EDGE ( 'NONE', *, *, #80304, .F. ) ;
#50724=CARTESIAN_POINT ( 'NONE',  ( 196.0727848089514964, 291.0389700598140621, 17.56388901715066808 ) ) ;
#50725=CARTESIAN_POINT ( 'NONE',  ( 148.3190727836317535, 273.7508255376806119, 8.080277324579027365 ) ) ;
#50726=CARTESIAN_POINT ( 'NONE',  ( 3.179769518870181777, 163.4548013555410080, -4.594050593750042211 ) ) ;
#50728=CARTESIAN_POINT ( 'NONE',  ( 35.38456857845647363, 200.4244531367911293, -4.594050593750046652 ) ) ;
#50732=CARTESIAN_POINT ( 'NONE',  ( 157.6668627405778409, 257.5599783937680058, -16.78811156090270629 ) ) ;
#50734=CARTESIAN_POINT ( 'NONE',  ( 190.8907028847385448, 300.0145992415348815, -5.421341690443150618 ) ) ;
#50736=CARTESIAN_POINT ( 'NONE',  ( 171.4130652328503004, 258.2459473316166623, 14.36335968337128755 ) ) ;
#50737=CARTESIAN_POINT ( 'NONE',  ( 71.37900974329706116, 202.0177522451417929, 5.000000000000051514 ) ) ;
#50739=CARTESIAN_POINT ( 'NONE',  ( 160.4962995477943650, 275.9333967852908813, 14.18032076246626794 ) ) ;
#50740=CARTESIAN_POINT ( 'NONE',  ( 150.5824154016292198, 269.8306011283729617, 15.30661888403989046 ) ) ;
#50743=CARTESIAN_POINT ( 'NONE',  ( 44.69460199273692069, 196.6115022471902591, 10.00000000000009592 ) ) ;
#50744=CARTESIAN_POINT ( 'NONE',  ( 181.8078859840880170, 291.6367625042899476, 9.277818018440548542 ) ) ;
#50745=CARTESIAN_POINT ( 'NONE',  ( 172.9311764467664716, 268.4779053881692334, -17.72160738022306603 ) ) ;
#50747=CARTESIAN_POINT ( 'NONE',  ( -5.021015940802497468, 180.1589784336661637, -6.496448406907675876E-16 ) ) ;
#50748=CARTESIAN_POINT ( 'NONE',  ( 167.9225537833162889, 286.9219355629304005, 5.061554283893224593 ) ) ;
#50753=CARTESIAN_POINT ( 'NONE',  ( 207.2383675728608239, 271.6996134166075763, 7.873592648726489784 ) ) ;
#50763=CARTESIAN_POINT ( 'NONE',  ( 153.0760735463355786, 278.0209436513679861, -4.743639997390301843 ) ) ;
#50764=ORIENTED_EDGE ( 'NONE', *, *, #61642, .T. ) ;
#50766=CARTESIAN_POINT ( 'NONE',  ( 206.7893622945242385, 272.4773133715531230, -10.52881283832460291 ) ) ;
#50767=ORIENTED_EDGE ( 'NONE', *, *, #88375, .T. ) ;
#50768=( BOUNDED_CURVE ( )  B_SPLINE_CURVE ( 2, ( #38172, #47775, #69090, #78713, #100016, #61487, #92437, #69590, #35086 ),
 .UNSPECIFIED., .F., .T. ) 
 B_SPLINE_CURVE_WITH_KNOTS ( ( 3, 2, 2, 2, 3 ),
 ( 0.1491935483870967805, 0.1505376344086021556, 0.1532258064516129059, 0.1559139784946236562, 0.1572580645161290314 ),
 .UNSPECIFIED. ) 
 CURVE ( )  GEOMETRIC_REPRESENTATION_ITEM ( )  RATIONAL_B_SPLINE_CURVE ( ( 0.9330127018922194093, 0.9330127018922194093, 1.000000000000000000, 0.8660254037844387076, 1.000000000000000000, 0.8660254037844387076, 1.000000000000000000, 0.9330127018922194093, 0.9330127018922194093 ) ) 
 REPRESENTATION_ITEM ( '' )  );
#50769=CARTESIAN_POINT ( 'NONE',  ( 192.7507137768506880, 296.7929658737652971, 11.30364540927242345 ) ) ;
#50774=VERTEX_POINT ( 'NONE', #12576 ) ;
#50776=CARTESIAN_POINT ( 'NONE',  ( 159.3056354669941470, 256.7215407695565546, 17.03060606420897471 ) ) ;
#50777=CARTESIAN_POINT ( 'NONE',  ( 204.3371846825755824, 276.7246095846310823, 14.72513001683937262 ) ) ;
#50778=CARTESIAN_POINT ( 'NONE',  ( 153.3616370783189211, 265.0168479788495688, 17.48287904751960653 ) ) ;
#50781=CARTESIAN_POINT ( 'NONE',  ( 178.0913507944972309, 264.0370130977514123, 14.77546117709988671 ) ) ;
#50787=ORIENTED_EDGE ( 'NONE', *, *, #46761, .T. ) ;
#50788=CARTESIAN_POINT ( 'NONE',  ( 202.9994410512713614, 268.1261253757152758, 2.508732235296817326 ) ) ;
#50789=CARTESIAN_POINT ( 'NONE',  ( 166.2742916145368781, 273.7115028302620203, -15.76541653470950699 ) ) ;
#50792=B_SPLINE_SURFACE_WITH_KNOTS ( 'NONE', 3, 1, ( 
 ( #12838, #6706 ),
 ( #43698, #51293 ),
 ( #13803, #60877 ),
 ( #5216, #36096 ),
 ( #37584, #68494 ),
 ( #4728, #13326 ),
 ( #99418, #29021 ),
 ( #20427, #59892 ),
 ( #5703, #74641 ),
 ( #35611, #51818 ),
 ( #59380, #97924 ),
 ( #90860, #29995 ),
 ( #37098, #21412 ),
 ( #75128, #28499 ),
 ( #20937, #44189 ),
 ( #36594, #98430 ),
 ( #52297, #83235 ),
 ( #75614, #6203 ),
 ( #68002, #98926 ),
 ( #60381, #91337 ),
 ( #52786, #83743 ),
 ( #45192, #93332 ),
 ( #63398, #71020 ),
 ( #8700, #30499 ),
 ( #93845, #69985 ),
 ( #16294, #1620 ),
 ( #9202, #24399 ),
 ( #40074, #32506 ),
 ( #99913, #23885 ),
 ( #76604, #22400 ),
 ( #92831, #53295 ),
 ( #1106, #84248 ),
 ( #31483, #14796 ),
 ( #7190, #45678 ) ),
 .UNSPECIFIED., .T., .F., .F.,
 ( 4, 2, 2, 2, 2, 2, 2, 2, 2, 2, 2, 2, 2, 2, 2, 2, 4 ),
 ( 2, 2 ),
 ( 0.000000000000000000, 0.06250000000000000000, 0.1250000000000000000, 0.1875000000000000000, 0.2500000000000000000, 0.3125000000000000000, 0.3750000000000000000, 0.4375000000000000000, 0.5000000000000000000, 0.5625000000000000000, 0.6250000000000000000, 0.6875000000000000000, 0.7500000000000000000, 0.8125000000000000000, 0.8750000000000000000, 0.9375000000000000000, 1.000000000000000000 ),
 ( 0.000000000000000000, 1.000000000000000000 ),
 .UNSPECIFIED. ) ;
#50793=ORIENTED_EDGE ( 'NONE', *, *, #93109, .T. ) ;
#50794=CARTESIAN_POINT ( 'NONE',  ( 190.0274641710971082, 301.5097725526222803, 3.738976720635653450 ) ) ;
#50795=CARTESIAN_POINT ( 'NONE',  ( 171.3756802470358593, 263.0934282751447313, -15.50830625591261658 ) ) ;
#50796=ORIENTED_EDGE ( 'NONE', *, *, #84717, .T. ) ;
#50798=ORIENTED_EDGE ( 'NONE', *, *, #92042, .T. ) ;
#50800=VERTEX_POINT ( 'NONE', #59128 ) ;
#50802=CARTESIAN_POINT ( 'NONE',  ( 168.9116873843033488, 272.6398075186710344, 17.37279472990924134 ) ) ;
#50804=CARTESIAN_POINT ( 'NONE',  ( 188.2735287570237688, 299.1710073388255751, -5.251721556916531419 ) ) ;
#50806=CYLINDRICAL_SURFACE ( 'NONE', #50144, 17.82106496071139645 ) ;
#50807=CARTESIAN_POINT ( 'NONE',  ( 28.65277809448527080, 198.8967562850347122, -4.648177544792955347E-16 ) ) ;
#50808=CARTESIAN_POINT ( 'NONE',  ( 158.5236181937289928, 256.0760344192481739, -17.53025359445634024 ) ) ;
#50811=EDGE_CURVE ( 'NONE', #39107, #12301, #73772, .T. ) ;
#50813=CARTESIAN_POINT ( 'NONE',  ( 196.5114383562724072, 290.2791998289336561, -17.87308875047256862 ) ) ;
#50814=CARTESIAN_POINT ( 'NONE',  ( 165.0297293518065658, 244.8071193337670195, 2.517333243890161665 ) ) ;
#50815=CARTESIAN_POINT ( 'NONE',  ( 198.6012358295098750, 286.6595644277572887, 18.21911298807435386 ) ) ;
#50818=CARTESIAN_POINT ( 'NONE',  ( 190.7696186671953740, 300.2243232583145414, 6.802752300423729359 ) ) ;
#50821=CARTESIAN_POINT ( 'NONE',  ( 180.2261984326610218, 279.1782745765357276, -17.42438828499370729 ) ) ;
#50823=CARTESIAN_POINT ( 'NONE',  ( 198.9850252958828776, 285.9948215725895011, -17.02341478767141325 ) ) ;
#50824=CARTESIAN_POINT ( 'NONE',  ( 148.6479252781755633, 273.1812363089349560, -10.09608632811856488 ) ) ;
#50825=EDGE_LOOP ( 'NONE', ( #7347, #99170, #32030, #100001 ) ) ;
#50826=CARTESIAN_POINT ( 'NONE',  ( 163.0424334805279045, 248.2492167524936804, -9.671494865076915914 ) ) ;
#50827=CARTESIAN_POINT ( 'NONE',  ( 189.4381674897702794, 265.0040801212285828, 12.03645615491573828 ) ) ;
#50828=CARTESIAN_POINT ( 'NONE',  ( 59.05618993882887224, 198.2365022471902023, -10.00000000000009237 ) ) ;
#50829=CARTESIAN_POINT ( 'NONE',  ( 207.2824254892180704, 271.6233028670009162, 6.274396967990798046 ) ) ;
#50831=CARTESIAN_POINT ( 'NONE',  ( 29.73762157799522399, 194.6427522451419065, 10.00000000000009237 ) ) ;
#50832=CARTESIAN_POINT ( 'NONE',  ( 95.24857461505581568, 234.9869531367911293, 4.594050593750046652 ) ) ;
#50834=CARTESIAN_POINT ( 'NONE',  ( 163.2329522299293956, 249.6859758605342279, -11.67970021474453723 ) ) ;
#50836=CARTESIAN_POINT ( 'NONE',  ( 163.2109138634145609, 247.9574001692554077, 11.18215713980082171 ) ) ;
#50837=CARTESIAN_POINT ( 'NONE',  ( 32.86828966629671811, 177.5327760586659736, 1.948934522072303157E-15 ) ) ;
#50838=DIRECTION ( 'NONE',  ( -0.8660254037844387076, -0.4999999999999998890, -0.000000000000000000 ) ) ;
#50847=CARTESIAN_POINT ( 'NONE',  ( 207.4541616930702617, 271.3258470364304458, -6.834942797545373594 ) ) ;
#50848=CARTESIAN_POINT ( 'NONE',  ( 182.5213470551811952, 284.2517036362584122, 14.95339142714455782 ) ) ;
#50849=CARTESIAN_POINT ( 'NONE',  ( 107.7520767022434853, 223.0177522451418213, 5.000000000000051514 ) ) ;
#50850=CARTESIAN_POINT ( 'NONE',  ( 54.35637144981560454, 196.0643266524159856, -9.188101187500093303 ) ) ;
#50851=CARTESIAN_POINT ( 'NONE',  ( 99.01965388075039698, 214.6427522451417644, 1.119607411625061291E-15 ) ) ;
#50853=CARTESIAN_POINT ( 'NONE',  ( 198.7749709662292048, 267.8112567065418830, -8.151866048833305456 ) ) ;
#50854=AXIS2_PLACEMENT_3D ( 'NONE', #63514, #64016, #79267 ) ;
#50855=CARTESIAN_POINT ( 'NONE',  ( 3.578749241215597010, 161.3262482093458061, 3.021315404115420679E-15 ) ) ;
#50857=CARTESIAN_POINT ( 'NONE',  ( -3.153561889951042474, 178.1744531367911577, 4.594050593750047540 ) ) ;
#50858=CARTESIAN_POINT ( 'NONE',  ( 184.1240780222136095, 289.0015729834078684, -14.54488561116068901 ) ) ;
#50860=CARTESIAN_POINT ( 'NONE',  ( 147.3715240516018810, 275.3920280842035595, -3.728968767617475866 ) ) ;
#50862=EDGE_CURVE ( 'NONE', #39984, #24856, #85765, .T. ) ;
#50863=CARTESIAN_POINT ( 'NONE',  ( 56.57573509489573382, 191.2202760586659736, -5.415160957724236172E-17 ) ) ;
#50864=CARTESIAN_POINT ( 'NONE',  ( 163.7183543885751078, 247.0784873978576854, -6.786164904910574336 ) ) ;
#50867=CARTESIAN_POINT ( 'NONE',  ( 206.9026071836525205, 272.2811674698855313, 7.240992997279449561 ) ) ;
#50868=ORIENTED_EDGE ( 'NONE', *, *, #33847, .F. ) ;
#50869=CARTESIAN_POINT ( 'NONE',  ( 164.4915767550571957, 245.7392269735623529, -6.407198159945809657 ) ) ;
#50870=CARTESIAN_POINT ( 'NONE',  ( 4.424420716760506522, 173.3615022471902591, -10.00000000000009592 ) ) ;
#50872=CARTESIAN_POINT ( 'NONE',  ( 122.6094779419291712, 253.8464784336661353, 1.353441290958777327E-15 ) ) ;
#50875=CARTESIAN_POINT ( 'NONE',  ( 206.8103133316597564, 272.4410251107632348, -7.853031083480094487 ) ) ;
#50877=CARTESIAN_POINT ( 'NONE',  ( 183.1207986101861138, 294.8225010653632694, -8.165837621905515320 ) ) ;
#50878=CARTESIAN_POINT ( 'NONE',  ( 181.2440676231241241, 294.5520841294345473, -6.623935519155441654 ) ) ;
#50879=CARTESIAN_POINT ( 'NONE',  ( 189.3296586673964725, 289.9008618244355375, 14.45166222766822450 ) ) ;
#50882=CARTESIAN_POINT ( 'NONE',  ( 151.1926529451685326, 268.7736386982768408, 14.30343427984827365 ) ) ;
#50883=CARTESIAN_POINT ( 'NONE',  ( 208.0836152412896922, 270.2356015099098840, -1.823998521107428328 ) ) ;
#50885=CARTESIAN_POINT ( 'NONE',  ( 172.7539835797103933, 268.7884175745374478, -17.03505160535703311 ) ) ;
#50893=CARTESIAN_POINT ( 'NONE',  ( 183.2522050184455509, 295.3237902215792019, 4.692948607239561198 ) ) ;
#50895=CARTESIAN_POINT ( 'NONE',  ( 150.6398013895194197, 278.2883321928695182, -3.066054659821555001E-05 ) ) ;
#50897=CARTESIAN_POINT ( 'NONE',  ( 194.5266718979755751, 283.0022525440393224, 17.46869296283346884 ) ) ;
#50899=ORIENTED_EDGE ( 'NONE', *, *, #56346, .T. ) ;
#50900=DIRECTION ( 'NONE',  ( 0.4999999999999998890, -0.8660254037844385966, 0.000000000000000000 ) ) ;
#50901=CARTESIAN_POINT ( 'NONE',  ( 148.1004780136491377, 274.1294427855589788, -7.811560775291159331 ) ) ;
#50905=CARTESIAN_POINT ( 'NONE',  ( 185.9275958459120375, 291.3127718750328654, 12.18038867512309231 ) ) ;
#50909=CARTESIAN_POINT ( 'NONE',  ( 85.18102929606172324, 229.1744531367911293, 4.594050593750047540 ) ) ;
#50910=CARTESIAN_POINT ( 'NONE',  ( 203.1337100355901839, 278.8090888188308440, 15.01049473222304442 ) ) ;
#50912=CARTESIAN_POINT ( 'NONE',  ( 185.3936852094165602, 259.4458236461365459, -6.858812480693883273 ) ) ;
#50915=CARTESIAN_POINT ( 'NONE',  ( 207.3589495855971450, 271.0586446502292119, 2.456771036675355457 ) ) ;
#50917=CARTESIAN_POINT ( 'NONE',  ( 192.6411016462967609, 294.0235828830534501, 14.35569275358684393 ) ) ;
#50921=CARTESIAN_POINT ( 'NONE',  ( 154.8545429534089237, 262.4310591522755089, -17.81746354318405778 ) ) ;
#50923=CARTESIAN_POINT ( 'NONE',  ( 207.5267809074749721, 271.2000668674752433, -7.171564386559168724 ) ) ;
#50925=CARTESIAN_POINT ( 'NONE',  ( 147.1831281302520154, 275.7183393919203809, -6.957138126403704881 ) ) ;
#50930=CARTESIAN_POINT ( 'NONE',  ( 144.9642793207625004, 248.3768266524159856, -9.188101187500091527 ) ) ;
#50931=CARTESIAN_POINT ( 'NONE',  ( 167.4161476617964865, 266.6887600003616967, -16.78267018717890124 ) ) ;
#50932=ORIENTED_EDGE ( 'NONE', *, *, #56009, .F. ) ;
#50937=CARTESIAN_POINT ( 'NONE',  ( 165.8206990081297931, 283.8978799598649516, 9.576760697357309837 ) ) ;
#50938=CARTESIAN_POINT ( 'NONE',  ( 202.3159758243612316, 271.2934567965075416, 9.391350104624100581 ) ) ;
#50943=CARTESIAN_POINT ( 'NONE',  ( 153.5156304082400425, 276.9426167816297948, 7.161423272292579689 ) ) ;
#50945=CARTESIAN_POINT ( 'NONE',  ( 157.8973161155885805, 257.8193490992549073, 16.76962879910869120 ) ) ;
#50946=CYLINDRICAL_SURFACE ( 'NONE', #88843, 2.471954595299370006 ) ;
#50948=ORIENTED_EDGE ( 'NONE', *, *, #39884, .F. ) ;
#50953=CARTESIAN_POINT ( 'NONE',  ( 201.5238370281167022, 268.0995926086904433, -2.854707868619844824 ) ) ;
#50954=CARTESIAN_POINT ( 'NONE',  ( 192.1478677531999608, 280.9830581577164708, -17.81712158036913252 ) ) ;
#50955=CARTESIAN_POINT ( 'NONE',  ( 190.7516742497373059, 300.2554039010641418, 4.342609251298632067 ) ) ;
#50957=CARTESIAN_POINT ( 'NONE',  ( 161.4272922886058836, 281.4068005242934305, -7.043569301989234255 ) ) ;
#50959=AXIS2_PLACEMENT_3D ( 'NONE', #23706, #7019, #37904 ) ;
#50963=CARTESIAN_POINT ( 'NONE',  ( 122.6368883333364010, 241.6115022471902591, 10.00000000000009592 ) ) ;
#50964=B_SPLINE_CURVE_WITH_KNOTS ( 'NONE', 3,
 ( #23852, #40042, #17258, #48163 ),
 .UNSPECIFIED., .F., .F.,
 ( 4, 4 ),
 ( 0.008192639775029337407, 0.01433920746624550366 ),
 .UNSPECIFIED. ) ;
#50967=CARTESIAN_POINT ( 'NONE',  ( 171.6880688175457408, 289.7684859944451432, 2.704731161792437888 ) ) ;
#50968=DIRECTION ( 'NONE',  ( -0.8660254037844387076, -0.4999999999999998890, -0.000000000000000000 ) ) ;
#50971=CARTESIAN_POINT ( 'NONE',  ( 14.51920287573142510, 173.0643266524160424, 9.188101187500095079 ) ) ;
#50972=CARTESIAN_POINT ( 'NONE',  ( 101.9066655502961964, 220.4548013555409511, -4.594050593750042211 ) ) ;
#50973=CARTESIAN_POINT ( 'NONE',  ( 44.69460199273694911, 186.6115022471902023, -5.000000000000041744 ) ) ;
#50974=CARTESIAN_POINT ( 'NONE',  ( 186.5064012131073810, 296.3665785887476432, -7.270687472978205612 ) ) ;
#50977=CARTESIAN_POINT ( 'NONE',  ( 153.1747891862213748, 277.6390251779605478, -8.000862867047169757 ) ) ;
#50978=CARTESIAN_POINT ( 'NONE',  ( 194.8708600166808651, 293.1207648669033006, -14.79199694356877970 ) ) ;
#50979=EDGE_CURVE ( 'NONE', #22323, #76711, #55182, .T. ) ;
#50981=CARTESIAN_POINT ( 'NONE',  ( 182.9159104275373977, 268.0747678481671414, -14.89985435326638630 ) ) ;
#50983=CARTESIAN_POINT ( 'NONE',  ( 178.7452121208765448, 291.6717820129654228, -9.156458492754065759 ) ) ;
#50985=CARTESIAN_POINT ( 'NONE',  ( 172.5304191843750345, 263.6019457708129039, -15.41392963016842721 ) ) ;
#50986=CARTESIAN_POINT ( 'NONE',  ( 74.78872445064843077, 223.1744531367911293, 4.594050593750047540 ) ) ;
#50990=CARTESIAN_POINT ( 'NONE',  ( 157.0848929289108469, 258.5679796760466047, 17.57466231005294688 ) ) ;
#50992=CARTESIAN_POINT ( 'NONE',  ( 148.9671336697298045, 272.6283511565604840, 12.24371685916078611 ) ) ;
#50993=CARTESIAN_POINT ( 'NONE',  ( 199.0363797504450929, 285.9058730480928716, -17.12190301149298222 ) ) ;
#50994=CARTESIAN_POINT ( 'NONE',  ( 160.6734846709049691, 282.6943762970620924, -6.583290857611773461 ) ) ;
#50996=CARTESIAN_POINT ( 'NONE',  ( 192.6679047218190135, 296.9363953644068488, -13.34486378385621386 ) ) ;
#50997=CARTESIAN_POINT ( 'NONE',  ( 127.3796741259112792, 255.8967562850346553, -4.648177544792955347E-16 ) ) ;
#51001=CARTESIAN_POINT ( 'NONE',  ( 192.4743214706506365, 297.2716913909250707, -12.17804856100553046 ) ) ;
#51002=CARTESIAN_POINT ( 'NONE',  ( 60.28305926085680966, 205.6115022471902591, 10.00000000000009592 ) ) ;
#51008=CARTESIAN_POINT ( 'NONE',  ( 193.8475705658754578, 288.0377294361514373, 16.93899091255358869 ) ) ;
#51010=CARTESIAN_POINT ( 'NONE',  ( 130.8641296692885305, 256.3615022471903444, 5.000000000000046185 ) ) ;
#51011=CARTESIAN_POINT ( 'NONE',  ( 205.1300674467857164, 275.3512963525735131, -12.60245643603069610 ) ) ;
#51014=CARTESIAN_POINT ( 'NONE',  ( 190.5844311467533316, 299.4370547860769989, -6.522056084446611557 ) ) ;
#51015=CARTESIAN_POINT ( 'NONE',  ( 188.7150346277363155, 272.5491880637262057, 16.57045186533353487 ) ) ;
#51017=CARTESIAN_POINT ( 'NONE',  ( 163.2442700311756596, 247.8996255919473697, 11.14021925110252020 ) ) ;
#51020=ORIENTED_EDGE ( 'NONE', *, *, #83508, .F. ) ;
#51021=CARTESIAN_POINT ( 'NONE',  ( 191.1374494863389373, 291.0598754717474890, 14.59185211929525749 ) ) ;
#51022=CARTESIAN_POINT ( 'NONE',  ( 158.8391802440265508, 255.5294649151923636, 17.60341940305819364 ) ) ;
#51023=CARTESIAN_POINT ( 'NONE',  ( 151.1618603905361624, 248.8923013555409796, 4.594050593750050204 ) ) ;
#51024=CARTESIAN_POINT ( 'NONE',  ( 205.1877054856971938, 273.8747620413109871, 10.81913124959201689 ) ) ;
#51025=CARTESIAN_POINT ( 'NONE',  ( 201.1755594471486859, 282.2007051268825535, -18.15567516623250910 ) ) ;
#51028=FACE_OUTER_BOUND ( 'NONE', #7815, .T. ) ;
#51029=FACE_OUTER_BOUND ( 'NONE', #74837, .T. ) ;
#51034=CARTESIAN_POINT ( 'NONE',  ( 163.8040269124969939, 246.9300982336122559, 6.025552750865228013 ) ) ;
#51035=CARTESIAN_POINT ( 'NONE',  ( 162.7552554279882031, 272.8056902114326476, -16.37138898352977634 ) ) ;
#51037=CYLINDRICAL_SURFACE ( 'NONE', #26276, 10.00000000000010658 ) ;
#51038=CARTESIAN_POINT ( 'NONE',  ( 152.5423653171682474, 268.4358682943698682, -15.78187745328793490 ) ) ;
#51040=CARTESIAN_POINT ( 'NONE',  ( 167.1313658916855900, 286.5916946420441604, -4.904932445929851781 ) ) ;
#51041=CARTESIAN_POINT ( 'NONE',  ( 169.5532941354267962, 267.3202395055815259, 16.92450780793635090 ) ) ;
#51042=CARTESIAN_POINT ( 'NONE',  ( 180.9973211531476238, 256.8713260056199488, 4.953687155094200101 ) ) ;
#51043=CARTESIAN_POINT ( 'NONE',  ( 100.7969837277561282, 222.8768266524159856, -9.188101187500091527 ) ) ;
#51044=VERTEX_POINT ( 'NONE', #65278 ) ;
#51045=CARTESIAN_POINT ( 'NONE',  ( 190.8623743139412454, 300.0636657654615647, 8.577953960666059530 ) ) ;
#51046=CARTESIAN_POINT ( 'NONE',  ( 166.8260628573998474, 278.3289732347862468, -13.29658692297307176 ) ) ;
#51051=CARTESIAN_POINT ( 'NONE',  ( 176.9023546970497875, 292.4662729303109927, -2.727046248897896596 ) ) ;
#51052=CARTESIAN_POINT ( 'NONE',  ( 157.5520850189458884, 257.7587792392113215, 16.71892742266126319 ) ) ;
#51054=LINE ( 'NONE', #97211, #18824 ) ;
#51055=EDGE_LOOP ( 'NONE', ( #59994, #14792, #49814, #80658, #61751, #87391, #36961, #44258, #12701, #46519, #19920, #88098, #69944, #34124, #23713, #89691, #93946, #26144, #96073, #94059 ) ) ;
#51057=( BOUNDED_CURVE ( )  B_SPLINE_CURVE ( 2, ( #55698, #1036, #49137, #23818, #17218, #31915, #62819, #85692, #93775 ),
 .UNSPECIFIED., .F., .F. ) 
 B_SPLINE_CURVE_WITH_KNOTS ( ( 3, 2, 2, 2, 3 ),
 ( 0.4959677419354838745, 0.4973118279569892497, 0.5000000000000000000, 0.5026881720430107503, 0.5040322580645161255 ),
 .UNSPECIFIED. ) 
 CURVE ( )  GEOMETRIC_REPRESENTATION_ITEM ( )  RATIONAL_B_SPLINE_CURVE ( ( 0.9330127018922194093, 0.9330127018922194093, 1.000000000000000000, 0.8660254037844387076, 1.000000000000000000, 0.8660254037844387076, 1.000000000000000000, 0.9330127018922194093, 0.9330127018922194093 ) ) 
 REPRESENTATION_ITEM ( '' )  );
#51058=CARTESIAN_POINT ( 'NONE',  ( 187.1504858166771896, 267.1035762790165222, -14.63698944013293968 ) ) ;
#51063=CARTESIAN_POINT ( 'NONE',  ( 191.4217213000991364, 263.9549948794881971, -7.974474884843431255 ) ) ;
#51064=CARTESIAN_POINT ( 'NONE',  ( 13.95070015838929400, 188.8615022471903160, 5.000000000000046185 ) ) ;
#51066=CARTESIAN_POINT ( 'NONE',  ( 127.4808708382166316, 256.6589784336661637, -6.496448406907675876E-16 ) ) ;
#51069=ORIENTED_EDGE ( 'NONE', *, *, #31427, .F. ) ;
#51070=CARTESIAN_POINT ( 'NONE',  ( 204.9134960529544287, 275.7264090101555212, 14.56629498631681408 ) ) ;
#51073=CARTESIAN_POINT ( 'NONE',  ( 192.9064638172013417, 270.9369261147751331, 14.92505667092759758 ) ) ;
#51074=CARTESIAN_POINT ( 'NONE',  ( 178.6016452153454850, 285.1529245495667624, 13.66975983559747831 ) ) ;
#51075=EDGE_CURVE ( 'NONE', #21534, #88756, #41080, .T. ) ;
#51078=CARTESIAN_POINT ( 'NONE',  ( 196.0123035030964047, 280.0493583844649947, -16.77947975799478542 ) ) ;
#51079=CARTESIAN_POINT ( 'NONE',  ( 142.9371257517045137, 259.7655487066560340, -7.305945665944389766 ) ) ;
#51081=CARTESIAN_POINT ( 'NONE',  ( 206.8014039808918199, 271.9024147334357053, 6.414352906864584369 ) ) ;
#51082=CARTESIAN_POINT ( 'NONE',  ( 206.8317058779879574, 272.4039721336197317, -10.41591514895975834 ) ) ;
#51084=CARTESIAN_POINT ( 'NONE',  ( 163.3723087697842971, 247.6778559913402091, -10.08585062664141319 ) ) ;
#51086=DIRECTION ( 'NONE',  ( -0.8660254037844387076, -0.4999999999999998890, -0.000000000000000000 ) ) ;
#51087=VECTOR ( 'NONE', #72913, 1000.000000000000000 ) ;
#51088=CARTESIAN_POINT ( 'NONE',  ( 185.9501193373536125, 265.4400708382679568, 13.68843392893370314 ) ) ;
#51096=EDGE_CURVE ( 'NONE', #48833, #40485, #20906, .T. ) ;
#51097=CARTESIAN_POINT ( 'NONE',  ( 15.54743449484293372, 179.7833772461660544, -9.188101187500095079 ) ) ;
#51098=CARTESIAN_POINT ( 'NONE',  ( 207.3567728362337732, 271.1044343289145218, 2.587868728010163100 ) ) ;
#51099=ORIENTED_EDGE ( 'NONE', *, *, #27553, .F. ) ;
#51102=ADVANCED_FACE ( 'NONE', ( #93424 ), #18397, .T. ) ;
#51104=CARTESIAN_POINT ( 'NONE',  ( 164.4405316900629259, 245.8276396196081350, -6.144538123479245328 ) ) ;
#51106=CARTESIAN_POINT ( 'NONE',  ( 51.43353571204313823, 194.3768266524159856, -9.188101187500093303 ) ) ;
#51108=CARTESIAN_POINT ( 'NONE',  ( 171.5767533171608932, 286.7469205890667467, 7.455704898055432572 ) ) ;
#51109=CARTESIAN_POINT ( 'NONE',  ( 190.4240181651484818, 300.8229208869809668, -4.214281362166949485 ) ) ;
#51111=CARTESIAN_POINT ( 'NONE',  ( 178.3571982967953602, 292.6181790745828835, -7.174879954037646002 ) ) ;
#51112=CARTESIAN_POINT ( 'NONE',  ( 147.0721334091522294, 275.9105878882373304, 0.7242168585908188572 ) ) ;
#51113=EDGE_CURVE ( 'NONE', #16838, #77804, #86342, .T. ) ;
#51115=CARTESIAN_POINT ( 'NONE',  ( 176.1048462933576388, 274.8593126533075974, 17.09347264305319314 ) ) ;
#51118=EDGE_CURVE ( 'NONE', #87111, #28084, #96763, .T. ) ;
#51119=CARTESIAN_POINT ( 'NONE',  ( 88.69951781898578247, 222.0177522451418781, -10.00000000000009592 ) ) ;
#51122=CARTESIAN_POINT ( 'NONE',  ( 105.6772241758911832, 218.4865022471901455, 1.119607411625061291E-15 ) ) ;
#51124=CARTESIAN_POINT ( 'NONE',  ( 161.6384288741144815, 267.7291502596664259, -17.04636140397435895 ) ) ;
#51125=VERTEX_POINT ( 'NONE', #12294 ) ;
#51126=CARTESIAN_POINT ( 'NONE',  ( 64.42391676880970408, 201.8768266524159856, -9.188101187500091527 ) ) ;
#51127=VERTEX_POINT ( 'NONE', #43153 ) ;
#51129=CARTESIAN_POINT ( 'NONE',  ( 146.8201187048455267, 276.3470901603510015, 4.112223577763169047 ) ) ;
#51132=CARTESIAN_POINT ( 'NONE',  ( 171.3634068529735828, 286.5179807154004834, 7.728413769772275899 ) ) ;
#51133=CARTESIAN_POINT ( 'NONE',  ( 207.2824254892180704, 271.6233028670009162, 6.274396967990798046 ) ) ;
#51136=CARTESIAN_POINT ( 'NONE',  ( 185.9440050421480919, 263.4269226037905014, 11.01369690752849984 ) ) ;
#51137=CARTESIAN_POINT ( 'NONE',  ( 174.5432515410337544, 282.4104588529930311, -15.15290805577315680 ) ) ;
#51138=CARTESIAN_POINT ( 'NONE',  ( 204.3531539698473978, 276.6969499677158524, 13.47943239092699841 ) ) ;
#51141=LINE ( 'NONE', #81109, #33274 ) ;
#51144=ORIENTED_EDGE ( 'NONE', *, *, #85057, .F. ) ;
#51145=CARTESIAN_POINT ( 'NONE',  ( 181.7035363212127379, 283.7571070694220907, 14.95731429925001343 ) ) ;
#51147=CARTESIAN_POINT ( 'NONE',  ( 190.8860811105559208, 300.0226043892405414, 8.636347304323541252 ) ) ;
#51148=CARTESIAN_POINT ( 'NONE',  ( 206.0930919633010774, 273.6832889610345774, -9.866500005465628220 ) ) ;
#51151=CARTESIAN_POINT ( 'NONE',  ( 161.5757715694810770, 250.7895496999525449, -14.51803553215175135 ) ) ;
#51160=CARTESIAN_POINT ( 'NONE',  ( 129.3483248890680954, 254.6744531367911577, 4.594050593750047540 ) ) ;
#51161=CARTESIAN_POINT ( 'NONE',  ( 191.0900422946452011, 299.6693332556258724, 8.872191398975367349 ) ) ;
#51163=CARTESIAN_POINT ( 'NONE',  ( 183.6064328101875844, 289.8855053871136533, -13.59221500815075423 ) ) ;
#51165=ORIENTED_EDGE ( 'NONE', *, *, #66531, .F. ) ;
#51166=CARTESIAN_POINT ( 'NONE',  ( 163.9354095869165633, 246.7025367662834014, -7.289870401565430313 ) ) ;
#51169=CARTESIAN_POINT ( 'NONE',  ( 159.6898930778639283, 254.0559870643349143, 16.90891900388599822 ) ) ;
#51171=CARTESIAN_POINT ( 'NONE',  ( 79.95842099707557793, 204.7202760586659167, -5.415160957724236172E-17 ) ) ;
#51174=CARTESIAN_POINT ( 'NONE',  ( 150.4255120825602887, 270.1023656488765710, 15.17857413906334507 ) ) ;
#51175=CARTESIAN_POINT ( 'NONE',  ( 171.8445276903575518, 276.6680178762132982, 16.23204015318158966 ) ) ;
#51176=ORIENTED_EDGE ( 'NONE', *, *, #28876, .F. ) ;
#51178=CARTESIAN_POINT ( 'NONE',  ( 201.4463813434794019, 281.7316278426353620, -17.16864527463587820 ) ) ;
#51179=CARTESIAN_POINT ( 'NONE',  ( 203.0862352702880003, 278.8913175244117610, -15.09542727681365015 ) ) ;
#51180=EDGE_LOOP ( 'NONE', ( #28267, #32713 ) ) ;
#51181=CARTESIAN_POINT ( 'NONE',  ( 191.9824032073976241, 287.6194387751458521, -17.05427143794285882 ) ) ;
#51182=CARTESIAN_POINT ( 'NONE',  ( 163.8291868588114255, 260.4160011549212754, -16.17568023803453414 ) ) ;
#51185=CARTESIAN_POINT ( 'NONE',  ( 53.12030748017507165, 208.1427522451419350, 10.00000000000009415 ) ) ;
#51188=CARTESIAN_POINT ( 'NONE',  ( 126.7502486777147794, 253.1744531367911009, 4.594050593750047540 ) ) ;
#51191=CARTESIAN_POINT ( 'NONE',  ( 191.0862225170008628, 299.6759493045793192, -9.402218231374108726 ) ) ;
#51193=CARTESIAN_POINT ( 'NONE',  ( 205.4608097893652996, 273.5822659152986489, -10.72688443308411088 ) ) ;
#51196=CARTESIAN_POINT ( 'NONE',  ( 204.8189571845487080, 275.8901551335242175, 13.43702398685204358 ) ) ;
#51197=EDGE_CURVE ( 'NONE', #14773, #27771, #12236, .T. ) ;
#51199=CARTESIAN_POINT ( 'NONE',  ( 178.7600897929267774, 254.1784503161647706, 4.743017227330367014 ) ) ;
#51202=CARTESIAN_POINT ( 'NONE',  ( 126.8768043691498377, 237.3927522451418497, 10.00000000000009948 ) ) ;
#51204=CARTESIAN_POINT ( 'NONE',  ( 152.8894687064977234, 278.3516875449029158, -6.243347624783317507 ) ) ;
#51205=CARTESIAN_POINT ( 'NONE',  ( 198.5119022532241786, 266.2458289876958588, 0.9081415792431625222 ) ) ;
#51209=CARTESIAN_POINT ( 'NONE',  ( 204.7519188734507622, 276.0062688943993408, -12.76027478560537531 ) ) ;
#51210=CARTESIAN_POINT ( 'NONE',  ( 194.0638893473842757, 269.5056305575998863, 12.07270889207231157 ) ) ;
#51212=CARTESIAN_POINT ( 'NONE',  ( 190.2935937139882299, 301.0488226629397559, 4.649863831023156813 ) ) ;
#51215=CARTESIAN_POINT ( 'NONE',  ( 155.5066938333533528, 261.3015006940112244, -18.40036130547566273 ) ) ;
#51216=CARTESIAN_POINT ( 'NONE',  ( 161.5454122949074645, 250.8421335059953776, 14.24337924419696932 ) ) ;
#51218=CARTESIAN_POINT ( 'NONE',  ( 140.5888732624034674, 238.6427522451417644, 1.119607411625061291E-15 ) ) ;
#51219=CARTESIAN_POINT ( 'NONE',  ( 175.9353947587521816, 285.3059048581015986, -12.02703367433279169 ) ) ;
#51221=CARTESIAN_POINT ( 'NONE',  ( 196.4351339088274813, 290.4113630087520050, 17.20526457544535504 ) ) ;
#51222=CARTESIAN_POINT ( 'NONE',  ( 151.2964716097791325, 268.5938194963972592, -15.66250187539618111 ) ) ;
#51223=CARTESIAN_POINT ( 'NONE',  ( 3.802138503898990329, 166.8768266524160140, 9.188101187500096856 ) ) ;
#51225=CARTESIAN_POINT ( 'NONE',  ( 48.02338713675939630, 198.5333772461660828, 9.188101187500095079 ) ) ;
#51229=CARTESIAN_POINT ( 'NONE',  ( 157.4211152037729562, 257.9856256133486454, -16.71526195140576831 ) ) ;
#51230=CARTESIAN_POINT ( 'NONE',  ( 191.9832910268169996, 291.9740856320129296, -14.33083625909805825 ) ) ;
#51231=AXIS2_PLACEMENT_3D ( 'NONE', #3103, #79616, #42545 ) ;
#51233=CARTESIAN_POINT ( 'NONE',  ( 167.4739133672058529, 256.7134934739360688, 13.89013134216980738 ) ) ;
#51234=EDGE_CURVE ( 'NONE', #68688, #14532, #66582, .T. ) ;
#51235=CARTESIAN_POINT ( 'NONE',  ( 181.1603734054039876, 255.6401209734635529, 2.176029259874446176 ) ) ;
#51236=CARTESIAN_POINT ( 'NONE',  ( 150.4572752258758612, 270.0473502708459250, 15.21885120838634187 ) ) ;
#51238=B_SPLINE_CURVE_WITH_KNOTS ( 'NONE', 3,
 ( #787, #91533, #92533, #6893, #85964, #52994, #39269, #31673, #78310, #100117, #8891, #54465, #39760, #7387, #84929, #45869 ),
 .UNSPECIFIED., .F., .F.,
 ( 4, 2, 2, 2, 2, 2, 2, 4 ),
 ( 0.0001980335298249143758, 0.0002838333738372856088, 0.0003267332958434711982, 0.0003696332178496568419, 0.0004125331398558424855, 0.0004554330618620280749, 0.0005412329058743169628, 0.0008844322819235596843 ),
 .UNSPECIFIED. ) ;
#51239=CARTESIAN_POINT ( 'NONE',  ( 54.65389413625798909, 192.3615022471901739, 5.000000000000051514 ) ) ;
#51241=CARTESIAN_POINT ( 'NONE',  ( 189.8314329296643450, 301.8493086226544619, -0.8085564604676659384 ) ) ;
#51242=CARTESIAN_POINT ( 'NONE',  ( 11.67712314985746858, 186.7369531367911293, -4.594050593750048428 ) ) ;
#51246=CARTESIAN_POINT ( 'NONE',  ( 155.5207183646172950, 261.6826666266933898, -16.99780945766855922 ) ) ;
#51247=CARTESIAN_POINT ( 'NONE',  ( 179.7554519724740487, 276.9442998558859586, 16.29670716075235859 ) ) ;
#51248=CARTESIAN_POINT ( 'NONE',  ( 185.0684497205900527, 286.3477220876792444, 16.15350733335134237 ) ) ;
#51249=CARTESIAN_POINT ( 'NONE',  ( 148.6023484834014425, 275.2601776331305814, 7.517535991345212665 ) ) ;
#51250=CARTESIAN_POINT ( 'NONE',  ( 176.9896994409250510, 260.9405379847559630, -13.11837235889534625 ) ) ;
#51256=CARTESIAN_POINT ( 'NONE',  ( 183.8754313647489198, 256.5225093191261294, -2.022205659181245174 ) ) ;
#51257=CARTESIAN_POINT ( 'NONE',  ( 193.8913555215501390, 294.8173164187117550, 15.40725395879721837 ) ) ;
#51262=CARTESIAN_POINT ( 'NONE',  ( 159.9470087484377814, 253.6106496594791508, -16.54933891566789939 ) ) ;
#51264=CARTESIAN_POINT ( 'NONE',  ( 153.4619471835925708, 264.8431057800031567, 16.95044998314351758 ) ) ;
#51268=CARTESIAN_POINT ( 'NONE',  ( 203.1044072055706806, 278.8598428092302584, -16.67109798570195878 ) ) ;
#51270=CARTESIAN_POINT ( 'NONE',  ( 164.1439264839012822, 246.7246349093515221, -4.787792474024944234 ) ) ;
#51271=CARTESIAN_POINT ( 'NONE',  ( 164.3010377730689981, 246.0692501711882869, 7.247566249275159578 ) ) ;
#51272=CARTESIAN_POINT ( 'NONE',  ( 153.4289928607825573, 264.9001843414388873, 17.27358709529985958 ) ) ;
#51274=FACE_OUTER_BOUND ( 'NONE', #28126, .T. ) ;
#51276=CARTESIAN_POINT ( 'NONE',  ( 177.9668643227034579, 263.6129378440573987, 15.31797677519840306 ) ) ;
#51282=CARTESIAN_POINT ( 'NONE',  ( 164.3939401533646958, 245.9083385283718712, 2.844462461176849200 ) ) ;
#51284=ORIENTED_EDGE ( 'NONE', *, *, #97710, .T. ) ;
#51285=CARTESIAN_POINT ( 'NONE',  ( 177.8477507594193412, 279.4524148463787583, -16.32274502148586492 ) ) ;
#51286=CARTESIAN_POINT ( 'NONE',  ( 172.3780232790210789, 263.7810319789855384, -15.48897907228803206 ) ) ;
#51289=ORIENTED_EDGE ( 'NONE', *, *, #59614, .F. ) ;
#51290=CARTESIAN_POINT ( 'NONE',  ( 157.6127312046615145, 268.8539850385699879, 15.63345059891010891 ) ) ;
#51292=CARTESIAN_POINT ( 'NONE',  ( 156.4161679080374370, 267.1311002716061012, -16.29285210311729060 ) ) ;
#51293=CARTESIAN_POINT ( 'NONE',  ( 146.8516045228164160, 276.2925551239072774, 3.995954059407343273 ) ) ;
#51296=CARTESIAN_POINT ( 'NONE',  ( 192.1859061758433143, 297.7712413352111298, 11.15082371775444336 ) ) ;
#51298=CARTESIAN_POINT ( 'NONE',  ( 197.0632481487482437, 289.3234372322515924, -16.88857388075149046 ) ) ;
#51299=ORIENTED_EDGE ( 'NONE', *, *, #42975, .F. ) ;
#51302=CARTESIAN_POINT ( 'NONE',  ( 165.0087721269838710, 244.8434183119457543, 2.604344609212914108 ) ) ;
#51304=CARTESIAN_POINT ( 'NONE',  ( 164.4573439719129340, 245.7985198932525748, 1.541132361166968501 ) ) ;
#51306=ORIENTED_EDGE ( 'NONE', *, *, #62519, .F. ) ;
#51307=CARTESIAN_POINT ( 'NONE',  ( 170.4038350149297685, 287.7086646401646135, 4.116642393818346513 ) ) ;
#51310=VERTEX_POINT ( 'NONE', #98393 ) ;
#51313=CARTESIAN_POINT ( 'NONE',  ( 179.5569193005887030, 256.8711241645506220, 9.238826761386862430 ) ) ;
#51315=CARTESIAN_POINT ( 'NONE',  ( 198.6322367969459322, 286.6058691770745099, -18.00064234861828538 ) ) ;
#51316=EDGE_CURVE ( 'NONE', #48457, #75612, #61688, .T. ) ;
#51317=CARTESIAN_POINT ( 'NONE',  ( 190.5563804489516713, 300.5936626864281607, -0.2587918834769942222 ) ) ;
#51319=CARTESIAN_POINT ( 'NONE',  ( 208.1912724900461740, 270.0491336852600170, -0.9856800448607289100 ) ) ;
#51321=CARTESIAN_POINT ( 'NONE',  ( 205.5714613402004431, 274.0961078821768524, 10.65137002167587887 ) ) ;
#51322=CARTESIAN_POINT ( 'NONE',  ( 153.0790963368640689, 265.5062228982576471, -17.74594954892339160 ) ) ;
#51325=CARTESIAN_POINT ( 'NONE',  ( 207.6918009085542849, 270.9142438413412037, 7.009114282139513818 ) ) ;
#51326=ADVANCED_FACE ( 'NONE', ( #82977 ), #66246, .T. ) ;
#51327=CARTESIAN_POINT ( 'NONE',  ( 40.20209520705726192, 184.0177522451417929, 5.000000000000051514 ) ) ;
#51328=CARTESIAN_POINT ( 'NONE',  ( 117.0621101165238542, 229.2048013555409796, 4.594050593750051981 ) ) ;
#51329=CARTESIAN_POINT ( 'NONE',  ( 183.2680676362570296, 295.8844131031794404, -2.692372112000086748 ) ) ;
#51330=CARTESIAN_POINT ( 'NONE',  ( 165.0908032838305530, 280.5488345782329134, -11.11949073998667892 ) ) ;
#51331=FACE_OUTER_BOUND ( 'NONE', #70215, .T. ) ;
#51332=CARTESIAN_POINT ( 'NONE',  ( 162.8491774010308575, 248.5839461010540390, 10.21539626359008146 ) ) ;
#51333=CARTESIAN_POINT ( 'NONE',  ( 37.03551627836181126, 198.3149278399160664, 9.188101187500093303 ) ) ;
#51341=B_SPLINE_CURVE_WITH_KNOTS ( 'NONE', 3,
 ( #7382, #60076, #99112, #52000, #82465, #67192, #14000, #43889, #45864, #59070, #52486, #98115 ),
 .UNSPECIFIED., .F., .F.,
 ( 4, 2, 2, 2, 2, 4 ),
 ( 0.002214587119218288519, 0.002343824639362031628, 0.002473062159505774738, 0.002731537199793260522, 0.003248487280368166173, 0.004282387441517975304 ),
 .UNSPECIFIED. ) ;
#51344=DIRECTION ( 'NONE',  ( -0.8660254037844387076, -0.4999999999999998890, -0.000000000000000000 ) ) ;
#51347=CARTESIAN_POINT ( 'NONE',  ( 168.1712790018757460, 251.6228654270802849, 10.65815083953225084 ) ) ;
#51349=CARTESIAN_POINT ( 'NONE',  ( 93.96783902534114929, 218.3927522451417929, -10.00000000000009059 ) ) ;
#51350=ORIENTED_EDGE ( 'NONE', *, *, #14912, .F. ) ;
#51352=CARTESIAN_POINT ( 'NONE',  ( 154.9707648754391016, 280.5157924140515320, -2.443790094235759547 ) ) ;
#51353=CARTESIAN_POINT ( 'NONE',  ( 207.5886452961740076, 271.0929146030698007, -1.661373005306138184 ) ) ;
#51354=CARTESIAN_POINT ( 'NONE',  ( 16.57566611395445477, 186.5024278399161233, 9.188101187500095079 ) ) ;
#51355=CARTESIAN_POINT ( 'NONE',  ( 151.3124059063077311, 268.5662204852269497, -14.45542936000225609 ) ) ;
#51359=CARTESIAN_POINT ( 'NONE',  ( 61.77188751760236585, 194.2202760586659736, -5.415160957724236172E-17 ) ) ;
#51360=CARTESIAN_POINT ( 'NONE',  ( 164.2647213391612979, 246.1321520798662164, -5.830872732487307530 ) ) ;
#51361=CARTESIAN_POINT ( 'NONE',  ( 164.3961040135806968, 245.9045906125373904, 7.095190383188031191 ) ) ;
#51366=CARTESIAN_POINT ( 'NONE',  ( 164.4698008747318738, 245.7769439046653019, -6.272955660526681854 ) ) ;
#51367=CARTESIAN_POINT ( 'NONE',  ( 9.692741923115875124, 169.7365022471902023, -10.00000000000009059 ) ) ;
#51368=CARTESIAN_POINT ( 'NONE',  ( 201.5036534377215958, 270.3153034880852488, -10.25451236307256409 ) ) ;
#51369=CARTESIAN_POINT ( 'NONE',  ( 113.7598676209481994, 245.6744531367911293, 4.594050593750047540 ) ) ;
#51371=CARTESIAN_POINT ( 'NONE',  ( 164.9718327055057898, 244.9073992667478876, 1.131110055229076039 ) ) ;
#51375=CARTESIAN_POINT ( 'NONE',  ( 189.3632560013180353, 289.9061821024489518, 14.46060578062359880 ) ) ;
#51376=CARTESIAN_POINT ( 'NONE',  ( 150.5629864978592707, 269.8642529768378040, -13.73391103862138607 ) ) ;
#51377=VERTEX_POINT ( 'NONE', #81483 ) ;
#51378=CARTESIAN_POINT ( 'NONE',  ( 151.4327733764141612, 268.3577379114237829, 14.90862905801242100 ) ) ;
#51379=CARTESIAN_POINT ( 'NONE',  ( 208.1511065278944557, 270.1187031724418830, -0.2859582466342852625 ) ) ;
#51380=AXIS2_PLACEMENT_3D ( 'NONE', #93973, #24526, #71661 ) ;
#51382=CARTESIAN_POINT ( 'NONE',  ( 151.4581065015725869, 268.7005504512642915, -14.40868859785765999 ) ) ;
#51383=CARTESIAN_POINT ( 'NONE',  ( 173.0391163831423569, 268.2137988250248668, -16.30552455123574873 ) ) ;
#51384=CARTESIAN_POINT ( 'NONE',  ( 194.0277586765656963, 270.7140688648943865, -14.04450335696146723 ) ) ;
#51389=B_SPLINE_SURFACE_WITH_KNOTS ( 'NONE', 3, 1, ( 
 ( #18788, #49668 ),
 ( #26881, #35466 ),
 ( #28359, #65371 ),
 ( #66370, #44043 ),
 ( #81126, #65859 ),
 ( #50658, #82625 ),
 ( #57760, #43560 ),
 ( #97301, #58749 ),
 ( #96819, #13187 ),
 ( #19307, #88736 ),
 ( #20282, #11693 ),
 ( #74499, #5077 ),
 ( #73002, #80624 ),
 ( #35958, #66860 ),
 ( #3592, #42552 ),
 ( #97789, #90212 ),
 ( #20785, #34000 ),
 ( #27377, #64885 ),
 ( #26384, #84114 ),
 ( #53159, #91693 ),
 ( #7054, #29371 ),
 ( #38442, #61745 ),
 ( #99278, #90720 ),
 ( #83600, #13671 ),
 ( #22256, #22766 ),
 ( #14167, #52645 ),
 ( #29861, #75478 ),
 ( #46033, #5564 ),
 ( #60731, #92212 ),
 ( #45542, #6062 ),
 ( #36956, #69356 ),
 ( #67867, #53643 ),
 ( #59749, #14666 ),
 ( #46538, #84598 ) ),
 .UNSPECIFIED., .T., .F., .F.,
 ( 4, 2, 2, 2, 2, 2, 2, 2, 2, 2, 2, 2, 2, 2, 2, 2, 4 ),
 ( 2, 2 ),
 ( 0.000000000000000000, 0.06250000000000000000, 0.1250000000000000000, 0.1875000000000000000, 0.2500000000000000000, 0.3125000000000000000, 0.3750000000000000000, 0.4375000000000000000, 0.5000000000000000000, 0.5625000000000000000, 0.6250000000000000000, 0.6875000000000000000, 0.7500000000000000000, 0.8125000000000000000, 0.8750000000000000000, 0.9375000000000000000, 1.000000000000000000 ),
 ( 0.000000000000000000, 1.000000000000000000 ),
 .UNSPECIFIED. ) ;
#51391=CARTESIAN_POINT ( 'NONE',  ( 196.2821550604401466, 270.8744879265028658, 12.03960231697079664 ) ) ;
#51392=B_SPLINE_CURVE_WITH_KNOTS ( 'NONE', 3,
 ( #59790, #74535, #45580, #35994, #29895, #60768, #13226, #14205, #53196, #84151, #5605, #14697, #29407, #75515, #98324, #28397, #67399, #44581, #90254, #60276, #52683, #4614, #66409, #97335, #99809, #70903, #39968, #54168, #55174, #1511, #94232, #85134, #24783, #998, #47087, #69885, #61286, #77514, #15683, #84632, #23279, #86158, #8599, #31878, #16692, #46576, #70389, #86652, #8105, #30894 ),
 .UNSPECIFIED., .F., .F.,
 ( 4, 2, 2, 2, 2, 2, 2, 2, 2, 2, 2, 2, 2, 2, 2, 2, 2, 2, 2, 2, 2, 2, 2, 2, 4 ),
 ( 0.0001611619350887445517, 0.001178274281826848739, 0.001686830455195882997, 0.001813969498538121287, 0.001941108541880359577, 0.002068247585222597433, 0.002195386628564835723, 0.002449664715249311436, 0.002703942801933786715, 0.003212498975302860871, 0.004229611322040959312, 0.005246723668779058186, 0.005755279842148062520, 0.006009557928832644919, 0.006263836015517227317, 0.006327405537188392215, 0.006390975058859557113, 0.006454544580530722012, 0.006518114102201886910, 0.006772392188886545636, 0.007280948362255976712, 0.007535226448940692684, 0.007789504535625407788, 0.008043782622310124628, 0.008298060708994839732 ),
 .UNSPECIFIED. ) ;
#51393=CARTESIAN_POINT ( 'NONE',  ( 185.6230494993405671, 297.1728990862582691, 5.637358840499950396 ) ) ;
#51394=CARTESIAN_POINT ( 'NONE',  ( 208.1303168694798273, 270.1547119170880364, -0.9257663487928086132 ) ) ;
#51397=ORIENTED_EDGE ( 'NONE', *, *, #82460, .F. ) ;
#51401=ORIENTED_EDGE ( 'NONE', *, *, #58928, .T. ) ;
#51402=FACE_OUTER_BOUND ( 'NONE', #972, .T. ) ;
#51406=CARTESIAN_POINT ( 'NONE',  ( 147.2999496562918296, 275.5159985734018164, -0.1418322875769767455 ) ) ;
#51407=CARTESIAN_POINT ( 'NONE',  ( 204.7070208051621876, 272.9836748357583360, -9.755963162871239547 ) ) ;
#51408=AXIS2_PLACEMENT_3D ( 'NONE', #44034, #52144, #83093 ) ;
#51409=CARTESIAN_POINT ( 'NONE',  ( 204.5831314780710954, 276.2986172388744421, 13.28075685133257089 ) ) ;
#51412=CARTESIAN_POINT ( 'NONE',  ( 88.29356841273579448, 221.7833772461660544, -9.188101187500095079 ) ) ;
#51416=CARTESIAN_POINT ( 'NONE',  ( 178.8786591484599455, 269.4121626077708243, -17.24761370402104177 ) ) ;
#51418=ORIENTED_EDGE ( 'NONE', *, *, #82817, .F. ) ;
#51419=ORIENTED_EDGE ( 'NONE', *, *, #62203, .T. ) ;
#51422=CARTESIAN_POINT ( 'NONE',  ( 193.6538297768585153, 294.3106073703939387, 13.99927879369582406 ) ) ;
#51424=CARTESIAN_POINT ( 'NONE',  ( 159.1608936441631670, 258.2911997636435899, 17.40761412644028994 ) ) ;
#51425=CARTESIAN_POINT ( 'NONE',  ( 202.8549823380854491, 279.2918593523859272, -16.39745931995414807 ) ) ;
#51427=CARTESIAN_POINT ( 'NONE',  ( 206.9008466447795627, 272.2842168126622369, -7.000122840392532630 ) ) ;
#51428=AXIS2_PLACEMENT_3D ( 'NONE', #7489, #38382, #85031 ) ;
#51431=CARTESIAN_POINT ( 'NONE',  ( 194.6356465353167948, 293.5281665672507643, -16.13180903283129197 ) ) ;
#51433=CARTESIAN_POINT ( 'NONE',  ( 164.8232333123806654, 265.1872998416218934, -16.61854591372365419 ) ) ;
#51438=CARTESIAN_POINT ( 'NONE',  ( 167.1384944754526032, 284.3002062084726731, 9.379343144590123416 ) ) ;
#51439=CARTESIAN_POINT ( 'NONE',  ( 199.9340980646776700, 270.2282918247154839, 9.381492668529142875 ) ) ;
#51442=CARTESIAN_POINT ( 'NONE',  ( -9.181706736895311138, 177.0530062829863027, -4.648177544792955347E-16 ) ) ;
#51443=CARTESIAN_POINT ( 'NONE',  ( 170.9564544596932194, 287.9465792427529323, -5.428517921301809324 ) ) ;
#51444=CARTESIAN_POINT ( 'NONE',  ( 149.1928685617267831, 276.2413934580336559, -5.465481129197618415 ) ) ;
#51446=CARTESIAN_POINT ( 'NONE',  ( 192.8028085474765021, 292.0655250527965450, -15.27648668737578141 ) ) ;
#51450=CARTESIAN_POINT ( 'NONE',  ( 182.0923320409109465, 271.6029700406237453, -15.99347964086035567 ) ) ;
#51454=CARTESIAN_POINT ( 'NONE',  ( 160.5373035959516415, 275.8859140749689232, 12.69512463838454508 ) ) ;
#51456=CARTESIAN_POINT ( 'NONE',  ( 190.8252190424821890, 261.7436831218522002, 6.354606126879223105 ) ) ;
#51457=CARTESIAN_POINT ( 'NONE',  ( 204.1742785453265299, 277.0067712912111233, -14.60822391153214461 ) ) ;
#51460=CARTESIAN_POINT ( 'NONE',  ( 160.8117895914568010, 272.6511186442759822, 15.47829891388946244 ) ) ;
#51461=CARTESIAN_POINT ( 'NONE',  ( -13.87062626178347813, 171.9869531367911293, 4.594050593750046652 ) ) ;
#51463=CARTESIAN_POINT ( 'NONE',  ( 200.2706162234322562, 268.0192582847963081, 6.103686053348833518 ) ) ;
#51464=EDGE_LOOP ( 'NONE', ( #70076, #48433, #56740, #87174 ) ) ;
#51465=CIRCLE ( 'NONE', #61210, 17.82106496071138935 ) ;
#51468=CARTESIAN_POINT ( 'NONE',  ( 185.2570508126727873, 282.0811717828997303, -17.42469797758589678 ) ) ;
#51470=CARTESIAN_POINT ( 'NONE',  ( 171.7460074610065135, 289.4413739377905017, 2.655714547348211330 ) ) ;
#51471=CARTESIAN_POINT ( 'NONE',  ( 153.4477557824949940, 264.8676860077344486, 17.16010094972647693 ) ) ;
#51474=CARTESIAN_POINT ( 'NONE',  ( 42.52953848327577191, 205.3615022471903160, 5.000000000000046185 ) ) ;
#51475=CARTESIAN_POINT ( 'NONE',  ( -0.04102277327696322862, 170.7833772461660828, -9.188101187500095079 ) ) ;
#51476=CARTESIAN_POINT ( 'NONE',  ( 105.1271107466783121, 225.3768266524159856, 9.188101187500098632 ) ) ;
#51478=CARTESIAN_POINT ( 'NONE',  ( 180.0732687355215944, 254.9075906842349752, -2.440557160824225136 ) ) ;
#51484=CARTESIAN_POINT ( 'NONE',  ( 194.6356465353167948, 293.5281665672507643, -16.13180903283129197 ) ) ;
#51486=CARTESIAN_POINT ( 'NONE',  ( 195.3144667888438164, 266.4868967755442100, 7.916038506172456302 ) ) ;
#51487=CARTESIAN_POINT ( 'NONE',  ( 55.65629887206635829, 191.3932355074535678, -2.679491924311248496 ) ) ;
#51488=CARTESIAN_POINT ( 'NONE',  ( 163.3712170204604774, 252.4875253277900526, -12.92986515194776587 ) ) ;
#51489=FACE_OUTER_BOUND ( 'NONE', #2231, .T. ) ;
#51491=CARTESIAN_POINT ( 'NONE',  ( 172.5050055919510328, 263.7176657671190583, -15.44007813853843736 ) ) ;
#51492=CARTESIAN_POINT ( 'NONE',  ( 81.79837788435251866, 218.0333772461660544, 9.188101187500095079 ) ) ;
#51494=CARTESIAN_POINT ( 'NONE',  ( 190.8001679306945277, 300.1714103817999444, 7.815449226872675403 ) ) ;
#51496=CARTESIAN_POINT ( 'NONE',  ( 195.7291850945597957, 291.6341022226063160, 17.08310330964873813 ) ) ;
#51497=CARTESIAN_POINT ( 'NONE',  ( 200.3816788769131279, 283.5757466096723078, 17.26062989396512393 ) ) ;
#51498=CARTESIAN_POINT ( 'NONE',  ( 196.4758289992203117, 290.3408770445727782, 16.47704128718402572 ) ) ;
#51500=CARTESIAN_POINT ( 'NONE',  ( 204.5203606882526230, 276.0073328462628979, -12.85725516468893836 ) ) ;
#51501=VECTOR ( 'NONE', #36516, 1000.000000000000000 ) ;
#51502=EDGE_CURVE ( 'NONE', #20047, #7177, #42154, .T. ) ;
#51504=CARTESIAN_POINT ( 'NONE',  ( 147.1034852426517148, 275.8562849197056153, -3.648177088342072327 ) ) ;
#51509=CARTESIAN_POINT ( 'NONE',  ( 192.6170194583582429, 297.0245312260774995, -11.90166228306590490 ) ) ;
#51510=CARTESIAN_POINT ( 'NONE',  ( 187.9734438986738780, 286.0035705317766315, -16.48521393606941743 ) ) ;
#51513=CARTESIAN_POINT ( 'NONE',  ( 198.2040940955416488, 287.3474340887963763, 16.95806375232200480 ) ) ;
#51514=CARTESIAN_POINT ( 'NONE',  ( 157.0099022660245112, 268.5004079842800593, 15.67285573416865674 ) ) ;
#51516=CARTESIAN_POINT ( 'NONE',  ( 189.6957203118188318, 279.0266125994497202, 17.78851986857808853 ) ) ;
#51518=CARTESIAN_POINT ( 'NONE',  ( 136.9984762794283881, 243.2365022471902023, -10.00000000000009059 ) ) ;
#51526=EDGE_CURVE ( 'NONE', #56977, #16138, #76822, .T. ) ;
#51528=CARTESIAN_POINT ( 'NONE',  ( -22.42236680055709641, 157.8615022471902591, 0.000000000000000000 ) ) ;
#51531=CARTESIAN_POINT ( 'NONE',  ( 49.45774171355136417, 189.3615022471902023, 5.000000000000051514 ) ) ;
#51532=CARTESIAN_POINT ( 'NONE',  ( 205.6353699412782703, 274.4760867589209852, 10.94919351699760668 ) ) ;
#51533=CARTESIAN_POINT ( 'NONE',  ( 194.1209507349113039, 280.7511396460085962, -17.56060529715742291 ) ) ;
#51534=CARTESIAN_POINT ( 'NONE',  ( 204.1149192591630026, 272.7050794302332406, 11.20582280168199318 ) ) ;
#51535=CARTESIAN_POINT ( 'NONE',  ( 201.3715986869907510, 281.8611552031986776, -17.89433714524984964 ) ) ;
#51537=VECTOR ( 'NONE', #54489, 1000.000000000000000 ) ;
#51540=CARTESIAN_POINT ( 'NONE',  ( 165.9163065983553906, 275.1867875828022534, 14.76689463513480938 ) ) ;
#51541=CARTESIAN_POINT ( 'NONE',  ( 63.31414817410230000, 217.3615022471903160, 5.000000000000046185 ) ) ;
#51542=ORIENTED_EDGE ( 'NONE', *, *, #88908, .T. ) ;
#51543=ORIENTED_EDGE ( 'NONE', *, *, #26638, .F. ) ;
#51544=CARTESIAN_POINT ( 'NONE',  ( 178.0285553443036974, 273.4130338747266933, 17.82266553853486712 ) ) ;
#51546=CARTESIAN_POINT ( 'NONE',  ( 204.9780665305064531, 275.6145696623662502, 14.10615427165218883 ) ) ;
#51552=CARTESIAN_POINT ( 'NONE',  ( 167.0998337208708904, 286.2756947182164708, -4.828926102446922108 ) ) ;
#51555=CARTESIAN_POINT ( 'NONE',  ( 88.50972766791686297, 234.1589784336661637, -6.496448406907675876E-16 ) ) ;
#51558=CARTESIAN_POINT ( 'NONE',  ( 165.4582102121029550, 271.3011006785229711, 17.16042223052847859 ) ) ;
#51559=CARTESIAN_POINT ( 'NONE',  ( 165.4201252317303101, 277.4485869903318189, -13.43193553334254808 ) ) ;
#51567=CARTESIAN_POINT ( 'NONE',  ( 164.3163527186429178, 249.7635482851873974, 9.980485951392335409 ) ) ;
#51574=CARTESIAN_POINT ( 'NONE',  ( 162.7738416911812180, 248.7144313781379310, -11.09964294874192525 ) ) ;
#51575=VERTEX_POINT ( 'NONE', #25634 ) ;
#51577=CARTESIAN_POINT ( 'NONE',  ( 192.7686961758011250, 263.9209412561240811, -8.347089341778378468 ) ) ;
#51578=CARTESIAN_POINT ( 'NONE',  ( 13.06432082636536762, 189.8967562850346837, -4.648177544792955347E-16 ) ) ;
#51580=CARTESIAN_POINT ( 'NONE',  ( 138.6312950077063135, 250.8458772461660260, 9.188101187500095079 ) ) ;
#51583=ORIENTED_EDGE ( 'NONE', *, *, #80026, .F. ) ;
#51589=CARTESIAN_POINT ( 'NONE',  ( 173.0281810805265081, 251.5097863470425068, -0.2592435778029959503 ) ) ;
#51590=CARTESIAN_POINT ( 'NONE',  ( 33.84893051719189572, 201.8967562850347122, -4.648177544792955347E-16 ) ) ;
#51592=CARTESIAN_POINT ( 'NONE',  ( 198.9203168616069206, 282.2040875469349999, -16.77493235761543744 ) ) ;
#51595=CARTESIAN_POINT ( 'NONE',  ( 168.5910505471324257, 286.4687829538495976, 8.106709794022206594 ) ) ;
#51597=CARTESIAN_POINT ( 'NONE',  ( 64.07166007881600933, 216.9869531367911293, 4.594050593750046652 ) ) ;
#51600=CARTESIAN_POINT ( 'NONE',  ( 184.1240780222136095, 289.0015729834078684, -14.54488561116068901 ) ) ;
#51605=FACE_OUTER_BOUND ( 'NONE', #77848, .T. ) ;
#51608=CARTESIAN_POINT ( 'NONE',  ( 190.4234964968757424, 262.2385936383186049, -7.810700279455712547 ) ) ;
#51612=VECTOR ( 'NONE', #90818, 1000.000000000000000 ) ;
#51613=CARTESIAN_POINT ( 'NONE',  ( 16.49491010205593255, 171.1423013555409796, -4.594050593750043987 ) ) ;
#51615=VERTEX_POINT ( 'NONE', #12432 ) ;
#51616=CARTESIAN_POINT ( 'NONE',  ( 186.2134270706513632, 260.6652835500024707, -9.163389403908340114 ) ) ;
#51617=CARTESIAN_POINT ( 'NONE',  ( 199.5045416813903785, 277.5812092268299693, 15.20258081764992220 ) ) ;
#51618=FACE_OUTER_BOUND ( 'NONE', #15001, .T. ) ;
#51619=CARTESIAN_POINT ( 'NONE',  ( 164.0854748117396582, 246.4426161724408928, -5.757837433625331514 ) ) ;
#51621=CARTESIAN_POINT ( 'NONE',  ( 48.48320281069610616, 207.9869531367911009, 4.594050593750046652 ) ) ;
#51625=CARTESIAN_POINT ( 'NONE',  ( 156.6812872898450735, 261.2670451491295012, 0.000000000000000000 ) ) ;
#51626=CARTESIAN_POINT ( 'NONE',  ( 146.7879906441258129, 276.4027375938661635, 4.347255311287614887 ) ) ;
#51628=CARTESIAN_POINT ( 'NONE',  ( 202.9355525415089687, 270.0989142730967387, -6.790151509681939146 ) ) ;
#51629=CARTESIAN_POINT ( 'NONE',  ( 176.9907319409991544, 291.8589342268469977, 2.570357995431835185 ) ) ;
#51630=CARTESIAN_POINT ( 'NONE',  ( 179.7109432054668332, 276.7948752059230060, 16.30604964765089093 ) ) ;
#51634=CARTESIAN_POINT ( 'NONE',  ( 108.6181021060278198, 243.5177522451419065, 5.000000000000046185 ) ) ;
#51635=EDGE_CURVE ( 'NONE', #40420, #36946, #69965, .T. ) ;
#51636=B_SPLINE_CURVE_WITH_KNOTS ( 'NONE', 3,
 ( #80932, #11501, #42353, #73285 ),
 .UNSPECIFIED., .F., .F.,
 ( 4, 4 ),
 ( 0.009298372984062181629, 0.01507961473026592919 ),
 .UNSPECIFIED. ) ;
#51638=CARTESIAN_POINT ( 'NONE',  ( 92.68684311912451790, 230.9865022471903444, -10.00000000000009415 ) ) ;
#51639=CARTESIAN_POINT ( 'NONE',  ( 167.5421813246326792, 287.5986610761024167, 3.969292590682533373 ) ) ;
#51641=CARTESIAN_POINT ( 'NONE',  ( 165.2023859949471785, 269.8983204201427384, -16.28018730636620148 ) ) ;
#51642=ORIENTED_EDGE ( 'NONE', *, *, #68937, .T. ) ;
#51643=CARTESIAN_POINT ( 'NONE',  ( 57.73936995728981714, 194.9548013555410080, -4.594050593750042211 ) ) ;
#51645=CARTESIAN_POINT ( 'NONE',  ( 166.5418805794664934, 264.7512503615053561, 17.71810435351582669 ) ) ;
#51646=CARTESIAN_POINT ( 'NONE',  ( 190.9559560067148425, 299.9015775189195665, -4.895152914295826108 ) ) ;
#51654=CARTESIAN_POINT ( 'NONE',  ( 186.6908513136935426, 264.0735798317851959, 10.85260789151241667 ) ) ;
#51656=CARTESIAN_POINT ( 'NONE',  ( 204.9214210856886496, 275.7126824508080176, 13.23219655298346709 ) ) ;
#51660=CARTESIAN_POINT ( 'NONE',  ( 166.1279696197224496, 286.9939195634048588, -3.073011414649855499 ) ) ;
#51665=CARTESIAN_POINT ( 'NONE',  ( 151.0778907302193943, 268.9724126853576536, 15.84769371787143832 ) ) ;
#51668=ORIENTED_EDGE ( 'NONE', *, *, #65390, .F. ) ;
#51670=( BOUNDED_CURVE ( )  B_SPLINE_CURVE ( 2, ( #1287, #41634, #32171, #10760, #85946, #38256, #8384, #46355, #54967 ),
 .UNSPECIFIED., .F., .F. ) 
 B_SPLINE_CURVE_WITH_KNOTS ( ( 3, 2, 2, 2, 3 ),
 ( 0.2217741935483870941, 0.2231182795698924692, 0.2258064516129032195, 0.2284946236559139698, 0.2298387096774193450 ),
 .UNSPECIFIED. ) 
 CURVE ( )  GEOMETRIC_REPRESENTATION_ITEM ( )  RATIONAL_B_SPLINE_CURVE ( ( 0.9330127018922194093, 0.9330127018922194093, 1.000000000000000000, 0.8660254037844387076, 1.000000000000000000, 0.8660254037844387076, 1.000000000000000000, 0.9330127018922194093, 0.9330127018922194093 ) ) 
 REPRESENTATION_ITEM ( '' )  );
#51671=CARTESIAN_POINT ( 'NONE',  ( 159.8725050261465128, 283.2831117594137709, -3.366638177617166772 ) ) ;
#51673=CARTESIAN_POINT ( 'NONE',  ( 149.3141802193904368, 272.0272488999566463, -11.40332369054239336 ) ) ;
#51676=DIRECTION ( 'NONE',  ( -0.8660254037844387076, -0.4999999999999998890, -0.000000000000000000 ) ) ;
#51678=CARTESIAN_POINT ( 'NONE',  ( 163.0435180267337216, 264.1668671365804926, -16.76137116000093386 ) ) ;
#51679=CARTESIAN_POINT ( 'NONE',  ( 121.5540962550081190, 250.1744531367911009, 4.594050593750047540 ) ) ;
#51681=CARTESIAN_POINT ( 'NONE',  ( 150.6790040019602088, 269.6633047651677089, 15.38315204620803378 ) ) ;
#51682=ORIENTED_EDGE ( 'NONE', *, *, #10193, .F. ) ;
#51683=CARTESIAN_POINT ( 'NONE',  ( 173.5938284679934895, 265.1703973603451345, 16.93138633957164529 ) ) ;
#51684=CARTESIAN_POINT ( 'NONE',  ( -17.42236680055705023, 149.2012482093457777, 0.000000000000000000 ) ) ;
#51687=CARTESIAN_POINT ( 'NONE',  ( 148.9935118239307315, 275.4129331016238211, 7.652191349186828973 ) ) ;
#51691=CARTESIAN_POINT ( 'NONE',  ( 198.3150362131025588, 287.1552767044814800, 18.53472937702030521 ) ) ;
#51693=CARTESIAN_POINT ( 'NONE',  ( 74.27495573685769159, 207.5643266524160424, 9.188101187500095079 ) ) ;
#51694=CARTESIAN_POINT ( 'NONE',  ( 25.50001727096127979, 173.9824982072973967, 3.021315404115420679E-15 ) ) ;
#51696=CARTESIAN_POINT ( 'NONE',  ( 150.9462701294987141, 269.2003862531290110, 13.98983978186602073 ) ) ;
#51697=CARTESIAN_POINT ( 'NONE',  ( 175.7055647658949056, 278.3009567096344767, 15.59727287267344664 ) ) ;
#51702=CARTESIAN_POINT ( 'NONE',  ( 153.0444155045374544, 265.5662918618958201, -16.15173036748435109 ) ) ;
#51703=B_SPLINE_SURFACE_WITH_KNOTS ( 'NONE', 3, 1, ( 
 ( #93898, #15333 ),
 ( #55333, #32556 ),
 ( #63454, #46228 ),
 ( #94390, #17347 ),
 ( #79201, #7754 ),
 ( #35039, #94888 ),
 ( #2671, #87827 ),
 ( #2168, #42631 ),
 ( #72583, #87338 ),
 ( #18870, #25450 ),
 ( #42141, #56339 ),
 ( #26466, #3189 ),
 ( #50734, #19867 ),
 ( #25972, #63948 ),
 ( #26957, #81689 ),
 ( #17870, #34072 ),
 ( #33049, #80197 ),
 ( #64963, #48767 ),
 ( #79700, #57840 ),
 ( #72069, #10262 ),
 ( #33561, #41131 ),
 ( #64456, #95416 ),
 ( #10766, #56842 ),
 ( #18366, #49261 ),
 ( #88820, #41640 ),
 ( #95908, #49753 ),
 ( #57342, #12262 ),
 ( #88316, #80705 ),
 ( #11281, #3671 ),
 ( #73073, #34549 ),
 ( #65447, #81199 ),
 ( #96392, #19386 ),
 ( #50245, #11768 ),
 ( #73560, #4144 ) ),
 .UNSPECIFIED., .T., .F., .F.,
 ( 4, 2, 2, 2, 2, 2, 2, 2, 2, 2, 2, 2, 2, 2, 2, 2, 4 ),
 ( 2, 2 ),
 ( 0.000000000000000000, 0.06250000000000000000, 0.1250000000000000000, 0.1875000000000000000, 0.2500000000000000000, 0.3125000000000000000, 0.3750000000000000000, 0.4375000000000000000, 0.5000000000000000000, 0.5625000000000000000, 0.6250000000000000000, 0.6875000000000000000, 0.7500000000000000000, 0.8125000000000000000, 0.8750000000000000000, 0.9375000000000000000, 1.000000000000000000 ),
 ( 0.000000000000000000, 1.000000000000000000 ),
 .UNSPECIFIED. ) ;
#51704=LINE ( 'NONE', #82147, #60914 ) ;
#51707=CARTESIAN_POINT ( 'NONE',  ( 33.84893051719189572, 201.8967562850347122, -4.648177544792955347E-16 ) ) ;
#51708=CARTESIAN_POINT ( 'NONE',  ( 173.9947827226785364, 253.3674607417906088, -7.620349097399602201 ) ) ;
#51711=CARTESIAN_POINT ( 'NONE',  ( 200.3160299054414395, 283.2016034839092526, -16.83023095068803343 ) ) ;
#51714=CARTESIAN_POINT ( 'NONE',  ( 196.4501996009505831, 290.3852684645433442, -17.82325615854289680 ) ) ;
#51715=CARTESIAN_POINT ( 'NONE',  ( 198.7848905689980086, 281.0584550262959738, 16.97065934373781815 ) ) ;
#51717=ADVANCED_FACE ( 'NONE', ( #63000 ), #27920, .F. ) ;
#51718=CARTESIAN_POINT ( 'NONE',  ( 135.5998589986957086, 261.3464784336661637, 1.353441290958777327E-15 ) ) ;
#51719=ORIENTED_EDGE ( 'NONE', *, *, #47417, .F. ) ;
#51722=CARTESIAN_POINT ( 'NONE',  ( 155.9056400618096916, 261.9057474521822542, -16.97057099444750605 ) ) ;
#51724=FACE_OUTER_BOUND ( 'NONE', #3229, .T. ) ;
#51728=CARTESIAN_POINT ( 'NONE',  ( 184.8621414469888862, 277.3522383734357959, -16.75809678382782053 ) ) ;
#51729=CARTESIAN_POINT ( 'NONE',  ( 167.5934518032285325, 249.2213856889920578, -5.568558665174853317 ) ) ;
#51732=CARTESIAN_POINT ( 'NONE',  ( 198.6207901071857691, 266.0158434972533996, 0.2628236463959363056 ) ) ;
#51733=CARTESIAN_POINT ( 'NONE',  ( 190.9441801652054096, 299.9219738747156043, -4.765040093794296716 ) ) ;
#51734=B_SPLINE_CURVE_WITH_KNOTS ( 'NONE', 3,
 ( #43537, #20764, #6041, #82601 ),
 .UNSPECIFIED., .F., .F.,
 ( 4, 4 ),
 ( 0.04073415133443882008, 0.04887066958154930030 ),
 .UNSPECIFIED. ) ;
#51736=CARTESIAN_POINT ( 'NONE',  ( 157.1539462478114615, 258.4483758192793061, -17.96006278656275867 ) ) ;
#51737=CARTESIAN_POINT ( 'NONE',  ( 193.2382381725520872, 268.8873971962033806, 12.20118083718656443 ) ) ;
#51739=CARTESIAN_POINT ( 'NONE',  ( 149.6676065383367416, 271.4150965588098074, 11.80358707172367261 ) ) ;
#51742=CARTESIAN_POINT ( 'NONE',  ( 191.2190380946134951, 260.9445496458436651, 3.106810577783889915 ) ) ;
#51744=CARTESIAN_POINT ( 'NONE',  ( 136.2587462434811982, 256.1427522451419350, 10.00000000000009237 ) ) ;
#51745=CARTESIAN_POINT ( 'NONE',  ( 175.4001851152161464, 286.5081113820362475, -12.63027609277786567 ) ) ;
#51749=CARTESIAN_POINT ( 'NONE',  ( 199.2383506163646132, 285.5560492466715345, -17.78808061564097898 ) ) ;
#51750=CARTESIAN_POINT ( 'NONE',  ( 17.65854496445001587, 174.8768266524159856, -9.188101187500093303 ) ) ;
#51751=CARTESIAN_POINT ( 'NONE',  ( 176.7567624778341440, 257.9301109217140038, -10.40897364086542254 ) ) ;
#51754=CARTESIAN_POINT ( 'NONE',  ( 204.6149525604204769, 276.2435015074934199, -13.22810747389629960 ) ) ;
#51756=FACE_OUTER_BOUND ( 'NONE', #41249, .T. ) ;
#51757=CARTESIAN_POINT ( 'NONE',  ( 22.90194105960797089, 172.4824982072973967, 3.021315404115420679E-15 ) ) ;
#51758=CARTESIAN_POINT ( 'NONE',  ( 66.61587002248256795, 219.2677522451419065, -5.000000000000047962 ) ) ;
#51759=CARTESIAN_POINT ( 'NONE',  ( 181.4632975752175525, 255.1188003790442167, 1.936479460681336695 ) ) ;
#51760=CARTESIAN_POINT ( 'NONE',  ( 198.7430995078048284, 286.4138493292020371, 18.01120443222870193 ) ) ;
#51761=CARTESIAN_POINT ( 'NONE',  ( 179.4303423924146443, 294.0762619279377077, 1.040177563636374147 ) ) ;
#51762=CARTESIAN_POINT ( 'NONE',  ( 51.98364914125590985, 207.4865022471902876, 10.00000000000009237 ) ) ;
#51763=CARTESIAN_POINT ( 'NONE',  ( 184.7458354044235591, 293.7380398689933827, 9.593738941526117614 ) ) ;
#51764=CARTESIAN_POINT ( 'NONE',  ( 190.2476911738421848, 301.1283281946692796, -1.360079143321618611 ) ) ;
#51765=CARTESIAN_POINT ( 'NONE',  ( 21.44705901024191874, 189.3149278399161233, 9.188101187500093303 ) ) ;
#51766=CARTESIAN_POINT ( 'NONE',  ( 166.0706209929512340, 285.2106937319115332, 4.119889468574966074 ) ) ;
#51767=CARTESIAN_POINT ( 'NONE',  ( 13.08467475460494001, 168.3615022471902023, 5.000000000000051514 ) ) ;
#51770=EDGE_CURVE ( 'NONE', #75836, #65652, #24035, .T. ) ;
#51771=CARTESIAN_POINT ( 'NONE',  ( 207.6007741873543750, 271.0719067473055475, 7.587922723682903658 ) ) ;
#51772=CARTESIAN_POINT ( 'NONE',  ( 185.5568049818104726, 266.1438378612298834, 14.60334785453874140 ) ) ;
#51774=CARTESIAN_POINT ( 'NONE',  ( 160.1884772505443379, 280.3385904657917536, 9.408981587793775248 ) ) ;
#51779=AXIS2_PLACEMENT_3D ( 'NONE', #52975, #12506, #51988 ) ;
#51781=CARTESIAN_POINT ( 'NONE',  ( 194.1153812227096864, 294.4292925221022870, 15.54001482840963710 ) ) ;
#51783=CARTESIAN_POINT ( 'NONE',  ( 181.5727239729958455, 289.2385163777758521, 12.59120802838236663 ) ) ;
#51784=CARTESIAN_POINT ( 'NONE',  ( 112.6979501180548766, 224.3262482093458061, 3.021315404115420679E-15 ) ) ;
#51787=ORIENTED_EDGE ( 'NONE', *, *, #78226, .T. ) ;
#51788=CARTESIAN_POINT ( 'NONE',  ( 196.6401797514039629, 289.6109730388196226, -16.42068076416023459 ) ) ;
#51792=CARTESIAN_POINT ( 'NONE',  ( 154.8786460229866577, 262.3893114111486398, -18.06164891362396929 ) ) ;
#51793=EDGE_LOOP ( 'NONE', ( #86934, #93023, #68258, #54998 ) ) ;
#51795=CARTESIAN_POINT ( 'NONE',  ( 164.3636283963731159, 246.5961090085728245, -4.466486389993993278 ) ) ;
#51797=CARTESIAN_POINT ( 'NONE',  ( 192.6470966816805230, 296.9724359471326807, 11.11268290051284424 ) ) ;
#51801=CARTESIAN_POINT ( 'NONE',  ( 54.19488099963222538, 190.5494855054051868, -2.679491924311248496 ) ) ;
#51803=FACE_OUTER_BOUND ( 'NONE', #9569, .T. ) ;
#51805=CARTESIAN_POINT ( 'NONE',  ( 164.9103019330012216, 245.0139736909548560, 2.841678961959298810 ) ) ;
#51807=EDGE_LOOP ( 'NONE', ( #44027, #56613, #64952, #86270 ) ) ;
#51808=CARTESIAN_POINT ( 'NONE',  ( 175.0586189538327346, 277.5951793296135861, -15.65476470407738852 ) ) ;
#51810=CARTESIAN_POINT ( 'NONE',  ( 169.5394509045560767, 261.5465616151283257, -16.63734821970730948 ) ) ;
#51813=CARTESIAN_POINT ( 'NONE',  ( 192.4335622838504207, 297.3422883733380786, -12.83044365323471325 ) ) ;
#51815=ORIENTED_EDGE ( 'NONE', *, *, #50811, .T. ) ;
#51817=CARTESIAN_POINT ( 'NONE',  ( 156.6873744850167611, 266.6461852411879931, -16.20640834931786500 ) ) ;
#51818=CARTESIAN_POINT ( 'NONE',  ( 147.4317198359019301, 275.2877659273946733, 3.797273160043843188 ) ) ;
#51820=DIRECTION ( 'NONE',  ( -0.8660254037844387076, -0.4999999999999998890, -0.000000000000000000 ) ) ;
#51821=CARTESIAN_POINT ( 'NONE',  ( 192.1640094933931096, 297.8091675017319062, 12.36911124822534447 ) ) ;
#51822=CARTESIAN_POINT ( 'NONE',  ( 147.2990839561455800, 275.5174980100389348, 0.1083234189483078536 ) ) ;
#51823=CARTESIAN_POINT ( 'NONE',  ( 191.0604813119340690, 299.7205343796033503, -9.270812881586136811 ) ) ;
#51824=VERTEX_POINT ( 'NONE', #57765 ) ;
#51825=ADVANCED_FACE ( 'NONE', ( #42557 ), #58755, .T. ) ;
#51828=CARTESIAN_POINT ( 'NONE',  ( 196.7130436017243653, 289.9300093007386749, -16.33278734947153765 ) ) ;
#51831=CARTESIAN_POINT ( 'NONE',  ( 168.5642857825677368, 286.4821439168015331, 4.072950439418188573 ) ) ;
#51834=CARTESIAN_POINT ( 'NONE',  ( 149.2987140599570921, 272.0540370738933689, -11.50637251393979454 ) ) ;
#51836=EDGE_CURVE ( 'NONE', #17132, #12659, #84549, .T. ) ;
#51837=CARTESIAN_POINT ( 'NONE',  ( 202.7516255845870603, 278.9848387806140977, 15.23277972257327129 ) ) ;
#51839=CARTESIAN_POINT ( 'NONE',  ( 198.6984454753927594, 286.4911923821024970, -17.36054842559500599 ) ) ;
#51843=CARTESIAN_POINT ( 'NONE',  ( 170.4725219931047207, 255.4922488510977132, -11.62136048534125798 ) ) ;
#51844=CARTESIAN_POINT ( 'NONE',  ( 205.5791761573774181, 272.5734172477073116, 10.13670412909801044 ) ) ;
#51845=CARTESIAN_POINT ( 'NONE',  ( 206.9878665138179770, 272.1334939782196329, 6.566295309274049252 ) ) ;
#51846=CARTESIAN_POINT ( 'NONE',  ( 37.60401899570393880, 182.5177522451417929, 5.000000000000051514 ) ) ;
#51847=CARTESIAN_POINT ( 'NONE',  ( 114.4640339051705666, 227.7048013555410080, 4.594050593750051981 ) ) ;
#51848=CARTESIAN_POINT ( 'NONE',  ( 151.1451503555562113, 268.8559155969762742, -15.81507177720227553 ) ) ;
#51849=CARTESIAN_POINT ( 'NONE',  ( 164.2528612105914192, 280.3318051388083063, -11.32557250155417705 ) ) ;
#51850=CARTESIAN_POINT ( 'NONE',  ( 196.0034224882197975, 291.1591091234520263, 17.53794140922627776 ) ) ;
#51851=CARTESIAN_POINT ( 'NONE',  ( 172.4983949698107892, 251.2745399082947415, -3.985004546235816569 ) ) ;
#51852=CARTESIAN_POINT ( 'NONE',  ( 41.20343708195693466, 194.5958772461660544, -9.188101187500095079 ) ) ;
#51853=CARTESIAN_POINT ( 'NONE',  ( 147.7567117497646052, 276.1838835526310731, -2.437780156652150421 ) ) ;
#51854=ORIENTED_EDGE ( 'NONE', *, *, #2597, .T. ) ;
#51856=CARTESIAN_POINT ( 'NONE',  ( 181.8794332036203798, 266.9208721406195082, 15.44781841919039600 ) ) ;
#51857=B_SPLINE_CURVE_WITH_KNOTS ( 'NONE', 3,
 ( #20868, #12267, #82700, #4656, #35549, #66451, #97377, #36534, #58826, #89787, #95911, #14737, #7128, #38011, #68430, #37036, #68925, #23323, #76071, #75555, #99357, #91773, #6140, #83181, #59833, #21351, #13741, #77026, #21841, #7633, #6650, #45620, #52236, #84188, #91275, #46112, #29936, #22338, #53236, #52724, #15217, #99850, #76549, #60813, #30434, #29442, #44621, #49, #37524, #54210 ),
 .UNSPECIFIED., .F., .F.,
 ( 4, 2, 2, 2, 2, 2, 2, 2, 2, 2, 2, 2, 2, 2, 2, 2, 2, 2, 2, 2, 2, 2, 2, 2, 4 ),
 ( 0.001289879915731821603, 0.001760445656852789847, 0.002231011397973757873, 0.002466294268534241670, 0.002583935703814484001, 0.002701577139094726333, 0.002819218574374968665, 0.002936860009655210997, 0.003172142880215804515, 0.003642708621336909584, 0.004113274362458015088, 0.005054405844700225227, 0.005995537326942436233, 0.006466103068063580768, 0.006936668809184724435, 0.007054310244465032687, 0.007113130962105199823, 0.007171951679745365224, 0.007289593115025630975, 0.007407234550305896725, 0.007642517420866428227, 0.007877800291426959728, 0.008113083161987491229, 0.008348366032548022730, 0.008818931773669085733 ),
 .UNSPECIFIED. ) ;
#51858=CARTESIAN_POINT ( 'NONE',  ( 28.14990833772381151, 180.3927522451418497, 10.00000000000009948 ) ) ;
#51860=EDGE_CURVE ( 'NONE', #37198, #57617, #2358, .T. ) ;
#51861=CARTESIAN_POINT ( 'NONE',  ( 207.8431546909062320, 270.6520914003897360, -6.441273666418043220 ) ) ;
#51862=CARTESIAN_POINT ( 'NONE',  ( 179.3101858657603884, 287.6933342559568132, -12.46481062744024726 ) ) ;
#51863=CARTESIAN_POINT ( 'NONE',  ( 164.1895775543868581, 249.9821507493112733, 11.20547600539854116 ) ) ;
#51864=CARTESIAN_POINT ( 'NONE',  ( 92.59663213601581333, 214.2677522451417929, -5.000000000000041744 ) ) ;
#51866=B_SPLINE_CURVE_WITH_KNOTS ( 'NONE', 3,
 ( #75193, #59953, #42756, #35171, #98497, #6270, #38658, #37649, #54855, #30063, #168, #61941, #14376, #85308, #76668, #61454, #15854, #663, #8764, #93402, #60952, #16363, #84310, #7256, #53841, #38139, #41648, #48263, #80714, #16856, #79211, #9785, #24462, #72590, #18880, #42148, #40141, #71583, #78680, #64464, #2680, #71083 ),
 .UNSPECIFIED., .F., .F.,
 ( 4, 2, 2, 2, 2, 2, 2, 2, 2, 2, 2, 2, 2, 2, 2, 2, 2, 2, 2, 2, 4 ),
 ( 0.002125255516391542313, 0.002560878705408519730, 0.002778690299917009957, 0.002996501894425500617, 0.003105407691679724913, 0.003214313488933949643, 0.003432125083442451145, 0.003867748272459595963, 0.004738994650493884297, 0.005610241028528172198, 0.006481487406562460099, 0.006917110595579561982, 0.007352733784596663866, 0.007461639581850977934, 0.007516092480478200888, 0.007570545379105423842, 0.007679451176359996384, 0.007788356973614568926, 0.008223980162633185223, 0.008659603351651801520, 0.009095226540670417817 ),
 .UNSPECIFIED. ) ;
#51868=CARTESIAN_POINT ( 'NONE',  ( 198.7995061717253975, 267.7512988405533179, -8.185998893406019050 ) ) ;
#51869=CARTESIAN_POINT ( 'NONE',  ( 162.6476498368881494, 248.9330020812748785, 10.75824100428386743 ) ) ;
#51870=CARTESIAN_POINT ( 'NONE',  ( 153.8835784885725104, 264.7437728202501148, 16.55976697655874119 ) ) ;
#51871=CARTESIAN_POINT ( 'NONE',  ( 23.85612603422365297, 175.3923013555409796, 4.594050593750050204 ) ) ;
#51873=CARTESIAN_POINT ( 'NONE',  ( 192.3798651076289445, 272.0250015905760961, 14.19073807892398698 ) ) ;
#51876=CARTESIAN_POINT ( 'NONE',  ( 53.57110205792969282, 210.9244531367911577, -4.594050593750046652 ) ) ;
#51877=CARTESIAN_POINT ( 'NONE',  ( 164.3890147726454813, 245.9168695380243435, -6.010262808998044548 ) ) ;
#51878=CARTESIAN_POINT ( 'NONE',  ( 204.0436569602353245, 275.5599050935638843, 13.20187375397782858 ) ) ;
#51879=CARTESIAN_POINT ( 'NONE',  ( 167.5861325596884797, 256.5095974891418109, 15.03189046419509367 ) ) ;
#51880=CARTESIAN_POINT ( 'NONE',  ( 150.1819311511804642, 277.9734069837974744, -1.930257866626041707 ) ) ;
#51882=CARTESIAN_POINT ( 'NONE',  ( 21.81709757609801770, 176.7365022471902023, 10.00000000000009592 ) ) ;
#51884=CARTESIAN_POINT ( 'NONE',  ( 138.1979352100490530, 262.8464784336661637, 1.353441290958777327E-15 ) ) ;
#51886=CARTESIAN_POINT ( 'NONE',  ( 207.5676051492868339, 271.1293572064768682, -7.361967423939656641 ) ) ;
#51890=CARTESIAN_POINT ( 'NONE',  ( 185.8092585116022804, 288.0989997903241147, 14.76281570939348775 ) ) ;
#51893=CARTESIAN_POINT ( 'NONE',  ( 198.0816276881963915, 264.5915495180347534, -1.723934393811154182E-14 ) ) ;
#51894=CARTESIAN_POINT ( 'NONE',  ( 163.6574618462221906, 247.1839563750149011, 8.953931665434316400 ) ) ;
#51896=CARTESIAN_POINT ( 'NONE',  ( 169.6026530775712331, 266.0157843702824039, -17.26773840881970656 ) ) ;
#51898=EDGE_LOOP ( 'NONE', ( #17735, #87510, #87616, #80662 ) ) ;
#51902=CARTESIAN_POINT ( 'NONE',  ( 200.5914588262792222, 282.7033700937254821, -16.73555027083989444 ) ) ;
#51903=CARTESIAN_POINT ( 'NONE',  ( 196.2456956133878521, 270.8883091705321249, 12.07148411369787055 ) ) ;
#51904=CARTESIAN_POINT ( 'NONE',  ( 185.8273479531363250, 296.6862851380694792, 4.675326410034602809 ) ) ;
#51908=CARTESIAN_POINT ( 'NONE',  ( 149.7609858458625638, 276.9949590675715285, -0.0001241879625487765464 ) ) ;
#51912=DIRECTION ( 'NONE',  ( -0.8660254037844387076, -0.4999999999999998890, -0.000000000000000000 ) ) ;
#51913=ORIENTED_EDGE ( 'NONE', *, *, #67685, .T. ) ;
#51914=CARTESIAN_POINT ( 'NONE',  ( 168.3139509857544454, 277.6662850288790310, 15.73022063764310730 ) ) ;
#51916=CARTESIAN_POINT ( 'NONE',  ( 157.2489658521533613, 262.6752155823469934, -16.93568676516632365 ) ) ;
#51917=ORIENTED_EDGE ( 'NONE', *, *, #26405, .F. ) ;
#51918=CARTESIAN_POINT ( 'NONE',  ( 191.1747001918821525, 299.5227014763493116, -9.654804683100723040 ) ) ;
#51919=DIRECTION ( 'NONE',  ( -0.8660254037844387076, -0.4999999999999998890, -0.000000000000000000 ) ) ;
#51920=CARTESIAN_POINT ( 'NONE',  ( 204.3371846825755824, 276.7246095846310823, 14.72513001683937262 ) ) ;
#51922=ORIENTED_EDGE ( 'NONE', *, *, #21916, .T. ) ;
#51923=CARTESIAN_POINT ( 'NONE',  ( 87.77910550741502504, 230.6744531367911293, 4.594050593750047540 ) ) ;
#51924=CARTESIAN_POINT ( 'NONE',  ( 202.9132053460394900, 279.1910141444395776, 16.06438581368443863 ) ) ;
#51925=CARTESIAN_POINT ( 'NONE',  ( 182.7359208079271014, 258.3743599538522062, -5.878668705868922650 ) ) ;
#51927=ORIENTED_EDGE ( 'NONE', *, *, #57166, .T. ) ;
#51932=EDGE_LOOP ( 'NONE', ( #39842, #94933, #76957, #55951, #7422 ) ) ;
#51934=ORIENTED_EDGE ( 'NONE', *, *, #34687, .F. ) ;
#51935=CARTESIAN_POINT ( 'NONE',  ( 207.4508013134534110, 271.3316673846591129, -6.981098720164411908 ) ) ;
#51939=CARTESIAN_POINT ( 'NONE',  ( 194.4826705584825390, 293.7931287314651740, -16.11258321617245315 ) ) ;
#51941=CARTESIAN_POINT ( 'NONE',  ( 164.7413213274116117, 265.1114538392643567, -16.62100242902791791 ) ) ;
#51946=CARTESIAN_POINT ( 'NONE',  ( 167.0371890489551845, 283.5610238238203351, 9.003790523892211795 ) ) ;
#51947=CARTESIAN_POINT ( 'NONE',  ( 199.9947097613220706, 270.1151134968761767, 10.21374482337263245 ) ) ;
#51950=CARTESIAN_POINT ( 'NONE',  ( 206.8659638600981623, 272.3446355680395641, -10.26115277030573125 ) ) ;
#51951=CARTESIAN_POINT ( 'NONE',  ( 149.0807665407234026, 276.4376266709116408, -5.539133476438467873 ) ) ;
#51952=CARTESIAN_POINT ( 'NONE',  ( 165.3590881290603534, 246.8046831517908686, -1.872135347154431084 ) ) ;
#51953=LINE ( 'NONE', #37722, #1073 ) ;
#51955=CARTESIAN_POINT ( 'NONE',  ( 194.7141629039813040, 292.6873139064718998, 15.09280609635813342 ) ) ;
#51958=CARTESIAN_POINT ( 'NONE',  ( 194.3703447720679094, 293.9876827005354585, -15.62866922547675941 ) ) ;
#51961=CARTESIAN_POINT ( 'NONE',  ( 160.7849810028513673, 275.7942143859138469, 12.80952477407467249 ) ) ;
#51963=CARTESIAN_POINT ( 'NONE',  ( 204.2530634011613131, 276.8703119180381691, -15.12695148340227647 ) ) ;
#51967=CARTESIAN_POINT ( 'NONE',  ( -2.449395605728673875, 160.2048013555409796, 4.594050593750051981 ) ) ;
#51969=CARTESIAN_POINT ( 'NONE',  ( 189.0874221891241689, 297.0145170083281982, 8.224122883010650753 ) ) ;
#51971=ORIENTED_EDGE ( 'NONE', *, *, #69578, .F. ) ;
#51975=CARTESIAN_POINT ( 'NONE',  ( 171.6778415374343467, 289.4884753385041449, 2.667625303753221377 ) ) ;
#51980=CARTESIAN_POINT ( 'NONE',  ( 24.91150772114469092, 179.0643266524160424, 9.188101187500095079 ) ) ;
#51981=CARTESIAN_POINT ( 'NONE',  ( 111.3514947884964670, 235.0958772461660544, -9.188101187500095079 ) ) ;
#51984=B_SPLINE_CURVE_WITH_KNOTS ( 'NONE', 3,
 ( #97252, #50119, #51098, #73432, #38259, #99597, #43504, #43989, #96760, #58211, #27328, #68672 ),
 .UNSPECIFIED., .F., .F.,
 ( 4, 2, 2, 2, 2, 4 ),
 ( 0.001395616302646774960, 0.001599850232781533516, 0.001804084162916292072, 0.002212552023185749769, 0.002621019883455207033, 0.003029487743724664298 ),
 .UNSPECIFIED. ) ;
#51986=CARTESIAN_POINT ( 'NONE',  ( 177.5915495411956329, 283.6330961496328769, -15.30728232117395571 ) ) ;
#51987=CARTESIAN_POINT ( 'NONE',  ( 189.9405379874402513, 299.8870043450095295, -5.547851184193374863 ) ) ;
#51988=DIRECTION ( 'NONE',  ( 0.4999999999999992784, -0.8660254037844390407, 0.000000000000000000 ) ) ;
#51989=CARTESIAN_POINT ( 'NONE',  ( 161.8668411317136986, 250.2854024296290447, -13.43522912998426655 ) ) ;
#51990=CARTESIAN_POINT ( 'NONE',  ( 194.9636675848471441, 292.9600174435121289, -15.57898232594655319 ) ) ;
#51992=CARTESIAN_POINT ( 'NONE',  ( 196.0051728737935832, 265.8263463907475170, 8.406970388261065352 ) ) ;
#51994=CARTESIAN_POINT ( 'NONE',  ( 162.8384627734353387, 250.8402808221231624, -13.07578932517241732 ) ) ;
#51995=CARTESIAN_POINT ( 'NONE',  ( 48.42933654300939139, 198.7677522451418781, 10.00000000000009592 ) ) ;
#51996=CARTESIAN_POINT ( 'NONE',  ( 172.5032623719975220, 263.6776432955721816, -15.43083978726737726 ) ) ;
#51997=CARTESIAN_POINT ( 'NONE',  ( 91.05385083941617097, 229.5024278399160949, -9.188101187500093303 ) ) ;
#52000=CARTESIAN_POINT ( 'NONE',  ( 159.1193133772090675, 259.3124530707970052, -17.41573675653881637 ) ) ;
#52001=CARTESIAN_POINT ( 'NONE',  ( 195.8449251089225811, 291.4336346372613775, 16.14492769602857081 ) ) ;
#52004=CARTESIAN_POINT ( 'NONE',  ( 199.0773057068961123, 285.8349872121713702, -17.17316764978006560 ) ) ;
#52007=CARTESIAN_POINT ( 'NONE',  ( 147.0314375879888757, 275.9810751181479986, -5.168577011192616588 ) ) ;
#52009=ORIENTED_EDGE ( 'NONE', *, *, #99095, .T. ) ;
#52012=CARTESIAN_POINT ( 'NONE',  ( 180.2721358938293861, 265.6478004954673793, 15.92854085767422134 ) ) ;
#52013=CARTESIAN_POINT ( 'NONE',  ( 147.4271219180435253, 275.2957297547342819, -3.800519706258907782 ) ) ;
#52014=CARTESIAN_POINT ( 'NONE',  ( 188.2550976195534815, 286.0444469117322228, -16.18375812693026461 ) ) ;
#52015=ORIENTED_EDGE ( 'NONE', *, *, #7772, .F. ) ;
#52016=EDGE_CURVE ( 'NONE', #90285, #58638, #51141, .T. ) ;
#52019=CARTESIAN_POINT ( 'NONE',  ( 155.6995334974659215, 267.8060086419009735, 15.80633252148572510 ) ) ;
#52021=CARTESIAN_POINT ( 'NONE',  ( 170.4685145883027815, 252.7986105568807886, -8.763900896819295738 ) ) ;
#52022=CARTESIAN_POINT ( 'NONE',  ( 143.4214980241629576, 243.6115022471902023, -5.000000000000041744 ) ) ;
#52026=ORIENTED_EDGE ( 'NONE', *, *, #57421, .F. ) ;
#52027=DIRECTION ( 'NONE',  ( 0.4999999999999992784, -0.8660254037844390407, 0.000000000000000000 ) ) ;
#52031=ORIENTED_EDGE ( 'NONE', *, *, #13280, .T. ) ;
#52032=CARTESIAN_POINT ( 'NONE',  ( 167.5505310038667517, 261.6318463984700315, 17.07012949051403439 ) ) ;
#52033=CARTESIAN_POINT ( 'NONE',  ( 158.5390849126119974, 256.0492452763162987, 17.54477686596875330 ) ) ;
#52035=CARTESIAN_POINT ( 'NONE',  ( 204.0780454880880370, 272.9041813273606749, 11.05065144861194959 ) ) ;
#52036=CARTESIAN_POINT ( 'NONE',  ( 152.9251141908703175, 265.7729277985770864, -16.20110192949203309 ) ) ;
#52041=CARTESIAN_POINT ( 'NONE',  ( 173.6535785093707318, 257.7390071365238668, 13.58861338155497833 ) ) ;
#52042=CARTESIAN_POINT ( 'NONE',  ( 190.2204363742943656, 300.4646209966566062, -1.328626404316530739E-11 ) ) ;
#52043=ORIENTED_EDGE ( 'NONE', *, *, #55653, .T. ) ;
#52045=ORIENTED_EDGE ( 'NONE', *, *, #57233, .F. ) ;
#52046=CARTESIAN_POINT ( 'NONE',  ( 180.9205682475781600, 274.4254913274602359, 17.80862408263999441 ) ) ;
#52047=CARTESIAN_POINT ( 'NONE',  ( 174.4931704626366979, 257.1244136714613546, -12.18714520188626871 ) ) ;
#52048=CARTESIAN_POINT ( 'NONE',  ( 162.2191009146380622, 272.3218988927615101, -16.01639894604743830 ) ) ;
#52049=DIRECTION ( 'NONE',  ( -0.8660254037844387076, -0.4999999999999998890, -0.000000000000000000 ) ) ;
#52051=CARTESIAN_POINT ( 'NONE',  ( 201.8011112540905856, 277.2526834103201168, 15.54517447768417249 ) ) ;
#52053=CARTESIAN_POINT ( 'NONE',  ( 170.6405224136658489, 288.4786343240789392, -4.060171941529054251 ) ) ;
#52056=CARTESIAN_POINT ( 'NONE',  ( 116.3854409958760385, 231.8768266524160140, -9.188101187500091527 ) ) ;
#52058=CARTESIAN_POINT ( 'NONE',  ( 148.3413330264368710, 274.8204906787375990, -6.989116326937312884 ) ) ;
#52059=CARTESIAN_POINT ( 'NONE',  ( 191.9162138939681483, 293.2888617811998415, -14.67284693752439217 ) ) ;
#52061=CYLINDRICAL_SURFACE ( 'NONE', #93506, 17.82106496071139645 ) ;
#52063=CARTESIAN_POINT ( 'NONE',  ( 195.7291534503633272, 291.6341570319625021, 16.44925029361851543 ) ) ;
#52066=ORIENTED_EDGE ( 'NONE', *, *, #53150, .T. ) ;
#52067=ORIENTED_EDGE ( 'NONE', *, *, #7066, .T. ) ;
#52071=CARTESIAN_POINT ( 'NONE',  ( -11.89580835203306997, 175.4860189848785410, -2.679491924311245832 ) ) ;
#52074=CARTESIAN_POINT ( 'NONE',  ( 186.5376491172117994, 290.3301725222095229, -13.38673431320972185 ) ) ;
#52076=CARTESIAN_POINT ( 'NONE',  ( 201.3715986869907510, 281.8611552031986776, -17.89433714524984964 ) ) ;
#52077=ORIENTED_EDGE ( 'NONE', *, *, #31466, .T. ) ;
#52078=CARTESIAN_POINT ( 'NONE',  ( 190.4976253092930278, 300.6954295735222900, -5.764807383508308902 ) ) ;
#52080=CARTESIAN_POINT ( 'NONE',  ( 190.0207397430023661, 264.2850639489738001, -9.260904495796658864 ) ) ;
#52081=CARTESIAN_POINT ( 'NONE',  ( 173.6074067815649471, 251.0877831565759379, -1.045464715229854846 ) ) ;
#52085=CARTESIAN_POINT ( 'NONE',  ( 130.8844835975280887, 234.8262482093457493, 3.021315404115420679E-15 ) ) ;
#52088=CARTESIAN_POINT ( 'NONE',  ( 60.68900866710680475, 205.8458772461660544, 9.188101187500095079 ) ) ;
#52089=CARTESIAN_POINT ( 'NONE',  ( 206.7408728089182546, 272.5612996242556960, -10.63134519248043475 ) ) ;
#52091=CARTESIAN_POINT ( 'NONE',  ( 178.6049202613385773, 292.1719165999419943, -5.671730975596174673 ) ) ;
#52093=CARTESIAN_POINT ( 'NONE',  ( 207.8996209429610360, 270.5542889829179103, -5.987818313449536411 ) ) ;
#52094=CARTESIAN_POINT ( 'NONE',  ( 160.7489855951974675, 254.2215850144021658, 15.85577744295692248 ) ) ;
#52100=CARTESIAN_POINT ( 'NONE',  ( 196.0034224882197975, 291.1591091234520263, 17.53794140922627776 ) ) ;
#52102=CARTESIAN_POINT ( 'NONE',  ( 30.59497298136257726, 176.2202760586660020, -5.415160957724236172E-17 ) ) ;
#52103=CARTESIAN_POINT ( 'NONE',  ( 196.4351339088274813, 290.4113630087520050, 17.20526457544535504 ) ) ;
#52105=FACE_OUTER_BOUND ( 'NONE', #22233, .T. ) ;
#52107=CARTESIAN_POINT ( 'NONE',  ( 46.94050828626381389, 210.1589784336661637, -6.496448406907676862E-16 ) ) ;
#52109=CARTESIAN_POINT ( 'NONE',  ( 199.0773057068961123, 285.8349872121713702, -17.17316764978006560 ) ) ;
#52110=CARTESIAN_POINT ( 'NONE',  ( 196.5114383562724072, 290.2791998289336561, -17.87308875047256862 ) ) ;
#52112=CARTESIAN_POINT ( 'NONE',  ( 202.9443444632182434, 270.0342760574297358, -6.450216370591072668 ) ) ;
#52113=CARTESIAN_POINT ( 'NONE',  ( 175.6179495818389000, 291.0503388302134340, 2.344001588397030655 ) ) ;
#52114=CARTESIAN_POINT ( 'NONE',  ( 180.0951113711093114, 276.2838145191387298, 17.28842147576117938 ) ) ;
#52117=CARTESIAN_POINT ( 'NONE',  ( 163.3226323906401376, 255.9179029620415804, -14.86657747175461886 ) ) ;
#52119=CARTESIAN_POINT ( 'NONE',  ( 98.02733310912854847, 240.7365022471903444, 2.944929066748280225E-16 ) ) ;
#52120=CARTESIAN_POINT ( 'NONE',  ( 172.7264208856190919, 290.8582626858774347, 2.771863430787652849 ) ) ;
#52121=CARTESIAN_POINT ( 'NONE',  ( 194.6050500505458842, 285.5465367126718093, -17.70104686455487553 ) ) ;
#52123=CARTESIAN_POINT ( 'NONE',  ( 54.19381813872350762, 202.0958772461660544, -9.188101187500095079 ) ) ;
#52126=FACE_OUTER_BOUND ( 'NONE', #94172, .T. ) ;
#52127=CARTESIAN_POINT ( 'NONE',  ( 146.8058449195592061, 276.3718130816831149, 4.181814292810413392 ) ) ;
#52130=ORIENTED_EDGE ( 'NONE', *, *, #83285, .F. ) ;
#52131=DIRECTION ( 'NONE',  ( 0.5000000000000048850, -0.8660254037844358210, 0.000000000000000000 ) ) ;
#52134=CARTESIAN_POINT ( 'NONE',  ( 176.7483101607716094, 274.5073097362626982, -16.69060033052792136 ) ) ;
#52136=CARTESIAN_POINT ( 'NONE',  ( 157.1886094632603772, 258.3883373689681093, 18.40926891635499985 ) ) ;
#52137=AXIS2_PLACEMENT_3D ( 'NONE', #58632, #89606, #81994 ) ;
#52144=DIRECTION ( 'NONE',  ( -0.8660254037844387076, -0.4999999999999998890, -0.000000000000000000 ) ) ;
#52145=CARTESIAN_POINT ( 'NONE',  ( 168.4094709548043909, 262.4968943922261815, 16.00215286889127952 ) ) ;
#52146=CARTESIAN_POINT ( 'NONE',  ( 206.0946696452135427, 273.6805563358039421, -10.19627505985792837 ) ) ;
#52149=CARTESIAN_POINT ( 'NONE',  ( 57.52260328274599033, 204.0177522451418497, -10.00000000000009592 ) ) ;
#52150=CARTESIAN_POINT ( 'NONE',  ( 162.7738416911812180, 248.7144313781379310, -11.09964294874192525 ) ) ;
#52152=CARTESIAN_POINT ( 'NONE',  ( 188.6709712689815888, 295.3709411350409937, -11.33238897680398161 ) ) ;
#52153=CARTESIAN_POINT ( 'NONE',  ( 154.8332767207531901, 280.7459370637686220, -0.9958211956073632631 ) ) ;
#52154=CARTESIAN_POINT ( 'NONE',  ( 164.5265381092526695, 265.3812344335186140, -16.69521587732905843 ) ) ;
#52155=CARTESIAN_POINT ( 'NONE',  ( 127.1025053677084742, 238.0643266524160424, -9.188101187500093303 ) ) ;
#52159=CARTESIAN_POINT ( 'NONE',  ( 170.8702574392256111, 263.9852486083733538, 15.82437772357654993 ) ) ;
#52160=CARTESIAN_POINT ( 'NONE',  ( 187.1230481695341439, 299.1666633132790594, 2.832346326993921082 ) ) ;
#52161=ORIENTED_EDGE ( 'NONE', *, *, #8873, .T. ) ;
#52162=CARTESIAN_POINT ( 'NONE',  ( 200.9622342365141208, 281.7300170448321524, 16.66537280693965783 ) ) ;
#52163=ORIENTED_EDGE ( 'NONE', *, *, #4083, .F. ) ;
#52164=ORIENTED_EDGE ( 'NONE', *, *, #23725, .F. ) ;
#52167=CARTESIAN_POINT ( 'NONE',  ( 197.9354048063467246, 286.8717951656539640, 16.93488075601821308 ) ) ;
#52168=CARTESIAN_POINT ( 'NONE',  ( 191.8453338867844877, 298.3611298435110371, -9.039024722281077118 ) ) ;
#52170=CARTESIAN_POINT ( 'NONE',  ( 154.8556227199321427, 262.4291889417971788, 17.77326384500479861 ) ) ;
#52172=ORIENTED_CLOSED_SHELL ( 'NONE', *, #78266, .F. );
#52175=CARTESIAN_POINT ( 'NONE',  ( 200.6680263064462792, 283.0797783131037022, -17.21821073473145347 ) ) ;
#52176=CARTESIAN_POINT ( 'NONE',  ( 155.1398527401465230, 261.9368881057492899, -17.02245700497956449 ) ) ;
#52177=ORIENTED_EDGE ( 'NONE', *, *, #4992, .F. ) ;
#52178=CARTESIAN_POINT ( 'NONE',  ( 206.9985020284622408, 270.1150727264914053, 3.388313042214953441 ) ) ;
#52180=CARTESIAN_POINT ( 'NONE',  ( 174.4614454034193614, 253.2380414006159413, -7.790172112357452328 ) ) ;
#52181=CARTESIAN_POINT ( 'NONE',  ( 164.2801755739368446, 246.1053845600426087, 2.518777461081745717 ) ) ;
#52183=CARTESIAN_POINT ( 'NONE',  ( 195.1641141409822353, 279.2228943756692274, 16.33334675340180908 ) ) ;
#52184=CARTESIAN_POINT ( 'NONE',  ( 208.2939409893161553, 269.8713066281881083, 2.523744790997269227 ) ) ;
#52185=CARTESIAN_POINT ( 'NONE',  ( 139.2268610206906203, 245.0643266524160140, 9.188101187500095079 ) ) ;
#52189=EDGE_CURVE ( 'NONE', #62377, #759, #56703, .T. ) ;
#52193=CARTESIAN_POINT ( 'NONE',  ( 178.5408147360961379, 254.5644880976646220, 4.355285803803885081 ) ) ;
#52196=CARTESIAN_POINT ( 'NONE',  ( 182.4010281170673693, 275.0942260036622429, -17.56270495112026708 ) ) ;
#52198=CARTESIAN_POINT ( 'NONE',  ( 185.9727729040138797, 263.9344659017438630, -12.79113566482517328 ) ) ;
#52199=CARTESIAN_POINT ( 'NONE',  ( 202.0157110946482248, 267.6599266906877119, 0.8488657683144487098 ) ) ;
#52201=CARTESIAN_POINT ( 'NONE',  ( 190.1813752874636805, 301.2431906792259042, -4.710625539811892359 ) ) ;
#52203=B_SPLINE_CURVE_WITH_KNOTS ( 'NONE', 3,
 ( #36871, #99188, #46446, #98702 ),
 .UNSPECIFIED., .F., .F.,
 ( 4, 4 ),
 ( 0.004322650378965082335, 0.009836291497043285481 ),
 .UNSPECIFIED. ) ;
#52206=CARTESIAN_POINT ( 'NONE',  ( 193.0262075147481937, 268.6915971079139922, 12.26736561304707251 ) ) ;
#52208=EDGE_CURVE ( 'NONE', #65003, #79412, #48270, .T. ) ;
#52209=B_SPLINE_SURFACE_WITH_KNOTS ( 'NONE', 3, 1, ( 
 ( #95293, #56728 ),
 ( #25328, #32925 ),
 ( #31918, #9137 ),
 ( #49140, #93778 ),
 ( #23821, #62822 ),
 ( #24336, #16731 ),
 ( #80074, #55213 ),
 ( #63829, #86195 ),
 ( #56214, #31421 ),
 ( #40009, #39014 ),
 ( #535, #70949 ),
 ( #1552, #32435 ),
 ( #85695, #94271 ),
 ( #62310, #16234 ),
 ( #63330, #55701 ),
 ( #17221, #48128 ),
 ( #87211, #89200 ),
 ( #4029, #95788 ),
 ( #88694, #81567 ),
 ( #26342, #51112 ),
 ( #65813, #96270 ),
 ( #80581, #73938 ),
 ( #57218, #58221 ),
 ( #96774, #88193 ),
 ( #35918, #72961 ),
 ( #3553, #72463 ),
 ( #11160, #27829 ),
 ( #82077, #34915 ),
 ( #27340, #19748 ),
 ( #50613, #42027 ),
 ( #49626, #43517 ),
 ( #34431, #58705 ),
 ( #12138, #43000 ),
 ( #66330, #65331 ) ),
 .UNSPECIFIED., .T., .F., .F.,
 ( 4, 2, 2, 2, 2, 2, 2, 2, 2, 2, 2, 2, 2, 2, 2, 2, 4 ),
 ( 2, 2 ),
 ( 0.000000000000000000, 0.06250000000000000000, 0.1250000000000000000, 0.1875000000000000000, 0.2500000000000000000, 0.3125000000000000000, 0.3750000000000000000, 0.4375000000000000000, 0.5000000000000000000, 0.5625000000000000000, 0.6250000000000000000, 0.6875000000000000000, 0.7500000000000000000, 0.8125000000000000000, 0.8750000000000000000, 0.9375000000000000000, 1.000000000000000000 ),
 ( 0.000000000000000000, 1.000000000000000000 ),
 .UNSPECIFIED. ) ;
#52211=EDGE_CURVE ( 'NONE', #98884, #30031, #37725, .T. ) ;
#52213=CARTESIAN_POINT ( 'NONE',  ( 167.6010540021560189, 247.4270797612363708, 3.638657435017179864 ) ) ;
#52215=CARTESIAN_POINT ( 'NONE',  ( 160.0105735053945182, 253.5005522708592594, 16.10371386499367929 ) ) ;
#52217=CARTESIAN_POINT ( 'NONE',  ( 150.2594902713296676, 250.8927522451418213, 10.00000000000009592 ) ) ;
#52218=CARTESIAN_POINT ( 'NONE',  ( 172.9107215740591244, 283.7979364891335194, -12.27551315198952331 ) ) ;
#52219=VERTEX_POINT ( 'NONE', #37027 ) ;
#52224=CARTESIAN_POINT ( 'NONE',  ( 198.6363782946250183, 286.5986958926748116, -18.50260615857378355 ) ) ;
#52225=CARTESIAN_POINT ( 'NONE',  ( 4.668163907683432257, 167.3768266524159856, -9.188101187500093303 ) ) ;
#52226=CARTESIAN_POINT ( 'NONE',  ( 181.9027420907709143, 275.9322372300953816, -16.46933526673500126 ) ) ;
#52232=B_SPLINE_SURFACE_WITH_KNOTS ( 'NONE', 3, 1, ( 
 ( #93245, #60784 ),
 ( #14223, #54689 ),
 ( #68902, #84166 ),
 ( #92265, #78024 ),
 ( #31897, #91250 ),
 ( #37499, #85673 ),
 ( #69413, #14712 ),
 ( #76527, #21814 ),
 ( #53693, #76044 ),
 ( #6624, #68406 ),
 ( #46091, #99334 ),
 ( #37990, #30413 ),
 ( #61303, #77003 ),
 ( #38498, #24 ),
 ( #32900, #17721 ),
 ( #3044, #95268 ),
 ( #94742, #32412 ),
 ( #10116, #42005 ),
 ( #40495, #24315 ),
 ( #2529, #33411 ),
 ( #63810, #71425 ),
 ( #48103, #48623 ),
 ( #16708, #49115 ),
 ( #55190, #71926 ),
 ( #86174, #25305 ),
 ( #47601, #78529 ),
 ( #87690, #25831 ),
 ( #9114, #72438 ),
 ( #72939, #70926 ),
 ( #26319, #64312 ),
 ( #3530, #11134 ),
 ( #62801, #56707 ),
 ( #56192, #39986 ),
 ( #93757, #18221 ) ),
 .UNSPECIFIED., .T., .F., .F.,
 ( 4, 2, 2, 2, 2, 2, 2, 2, 2, 2, 2, 2, 2, 2, 2, 2, 4 ),
 ( 2, 2 ),
 ( 0.000000000000000000, 0.06250000000000000000, 0.1250000000000000000, 0.1875000000000000000, 0.2500000000000000000, 0.3125000000000000000, 0.3750000000000000000, 0.4375000000000000000, 0.5000000000000000000, 0.5625000000000000000, 0.6250000000000000000, 0.6875000000000000000, 0.7500000000000000000, 0.8125000000000000000, 0.8750000000000000000, 0.9375000000000000000, 1.000000000000000000 ),
 ( 0.000000000000000000, 1.000000000000000000 ),
 .UNSPECIFIED. ) ;
#52234=CARTESIAN_POINT ( 'NONE',  ( 196.2760436623706823, 269.3890986055657208, -10.67377300597419776 ) ) ;
#52235=CARTESIAN_POINT ( 'NONE',  ( 74.91528014208348907, 207.3927522451417929, 10.00000000000009592 ) ) ;
#52236=CARTESIAN_POINT ( 'NONE',  ( 175.5289232728569004, 253.5710909141142224, -3.838295042954765979 ) ) ;
#52237=CARTESIAN_POINT ( 'NONE',  ( 150.7108765041139691, 269.6080999720726936, 13.72660302980452407 ) ) ;
#52238=EDGE_CURVE ( 'NONE', #62095, #53306, #7169, .T. ) ;
#52239=CARTESIAN_POINT ( 'NONE',  ( 179.1211563714144859, 294.1662014525638256, 1.054073793073138532 ) ) ;
#52240=CARTESIAN_POINT ( 'NONE',  ( 66.70608100559145726, 195.9865022471901455, 1.119607411625061291E-15 ) ) ;
#52242=CARTESIAN_POINT ( 'NONE',  ( 190.3144310910409445, 301.0127312671879167, -1.334877248546042949 ) ) ;
#52243=CARTESIAN_POINT ( 'NONE',  ( 15.38488118375084390, 185.8149278399160949, -9.188101187500095079 ) ) ;
#52244=CARTESIAN_POINT ( 'NONE',  ( 164.2608904025049128, 285.0127816252062303, 4.307465260048421563 ) ) ;
#52248=CARTESIAN_POINT ( 'NONE',  ( 165.0387478276132072, 244.7914988754632191, -2.473354058663827626 ) ) ;
#52250=CARTESIAN_POINT ( 'NONE',  ( 189.1815913259335105, 268.0942611344048032, 13.94827899188442721 ) ) ;
#52251=CARTESIAN_POINT ( 'NONE',  ( 127.3796741259112792, 255.8967562850346553, -4.648177544792955347E-16 ) ) ;
#52252=CARTESIAN_POINT ( 'NONE',  ( 160.7682838322721466, 280.9513019390540194, 9.562328407288063659 ) ) ;
#52254=CARTESIAN_POINT ( 'NONE',  ( 116.4123307400877820, 248.0177522451419065, 5.000000000000046185 ) ) ;
#52257=EDGE_CURVE ( 'NONE', #63007, #71681, #38565, .T. ) ;
#52258=CARTESIAN_POINT ( 'NONE',  ( 155.0197698005585494, 262.1448778582381465, 18.42918111182112284 ) ) ;
#52259=ORIENTED_EDGE ( 'NONE', *, *, #76177, .T. ) ;
#52260=CARTESIAN_POINT ( 'NONE',  ( 184.6389624118809252, 290.5370850536020271, 12.15673895467454280 ) ) ;
#52262=ADVANCED_FACE ( 'NONE', ( #25322 ), #28766, .F. ) ;
#52267=CARTESIAN_POINT ( 'NONE',  ( 70.22199747613832699, 222.8967562850346837, -4.648177544792955347E-16 ) ) ;
#52269=CARTESIAN_POINT ( 'NONE',  ( 202.7973612924478743, 279.3916619310153919, -15.54732529288344089 ) ) ;
#52270=ORIENTED_EDGE ( 'NONE', *, *, #65455, .F. ) ;
#52272=DIRECTION ( 'NONE',  ( 0.4999999999999992784, -0.8660254037844390407, 0.000000000000000000 ) ) ;
#52273=CARTESIAN_POINT ( 'NONE',  ( -27.42236680055714260, 166.5217562850347406, 1.224646799147364892E-15 ) ) ;
#52275=CARTESIAN_POINT ( 'NONE',  ( 150.6487462746963502, 269.7157126861102370, 15.18501655901553704 ) ) ;
#52281=ORIENTED_EDGE ( 'NONE', *, *, #22388, .T. ) ;
#52282=CARTESIAN_POINT ( 'NONE',  ( 164.7297297678022403, 245.3267338555121455, 3.020078936458732599 ) ) ;
#52284=ORIENTED_EDGE ( 'NONE', *, *, #63108, .T. ) ;
#52285=CARTESIAN_POINT ( 'NONE',  ( 190.7805732161387766, 300.2053494229706985, 4.237982805666590025 ) ) ;
#52286=CARTESIAN_POINT ( 'NONE',  ( 172.2019080879319120, 264.1397931956042271, -16.46918750876103132 ) ) ;
#52288=ORIENTED_EDGE ( 'NONE', *, *, #5435, .T. ) ;
#52289=CARTESIAN_POINT ( 'NONE',  ( 158.6117737028674242, 274.9709143987748803, -12.58280590594613813 ) ) ;
#52295=CARTESIAN_POINT ( 'NONE',  ( 168.9434124915611903, 272.5888371849330838, 17.32495137616924907 ) ) ;
#52297=CARTESIAN_POINT ( 'NONE',  ( 190.9559560067148425, 299.9015775189195665, -4.895152914295826108 ) ) ;
#52298=CARTESIAN_POINT ( 'NONE',  ( 188.4285301707691076, 298.9031352353757711, -5.166013069444586492 ) ) ;
#52299=DIRECTION ( 'NONE',  ( 0.4999999999999992784, -0.8660254037844390407, 0.000000000000000000 ) ) ;
#52300=CARTESIAN_POINT ( 'NONE',  ( 192.4202172926039793, 297.3654025762033370, 10.98569444949570872 ) ) ;
#52301=CARTESIAN_POINT ( 'NONE',  ( 191.4524900926791702, 299.0415552543392437, 8.268219431103382533 ) ) ;
#52302=CARTESIAN_POINT ( 'NONE',  ( 191.3041230083617563, 299.2985345825480863, -9.819045872446528378 ) ) ;
#52307=CARTESIAN_POINT ( 'NONE',  ( 196.8104339078508076, 289.7613243423628546, -16.40335862274955403 ) ) ;
#52310=CARTESIAN_POINT ( 'NONE',  ( 170.6717880471474871, 287.9187896612353370, 4.129465665201498936 ) ) ;
#52311=CARTESIAN_POINT ( 'NONE',  ( 168.8244094625508751, 257.0541383169796745, -14.93690306707719628 ) ) ;
#52312=VERTEX_POINT ( 'NONE', #75683 ) ;
#52313=CARTESIAN_POINT ( 'NONE',  ( 149.2693755472542136, 272.1048528685130350, -13.07444463944290547 ) ) ;
#52315=CARTESIAN_POINT ( 'NONE',  ( 202.6833006059332263, 277.5892208352050829, 15.45935665133711900 ) ) ;
#52317=DIRECTION ( 'NONE',  ( -0.8660254037844387076, -0.4999999999999998890, -0.000000000000000000 ) ) ;
#52320=CARTESIAN_POINT ( 'NONE',  ( 170.7306893209106988, 255.3552208224515425, -12.88177093387596450 ) ) ;
#52322=CARTESIAN_POINT ( 'NONE',  ( 207.3502731283117555, 271.5057873089173768, 6.280625384230454245 ) ) ;
#52323=CARTESIAN_POINT ( 'NONE',  ( 47.99632384111720995, 188.5177522451417929, 5.000000000000051514 ) ) ;
#52324=CARTESIAN_POINT ( 'NONE',  ( 123.8009570636627785, 230.0327760586659451, 1.948934522072302763E-15 ) ) ;
#52326=CARTESIAN_POINT ( 'NONE',  ( 180.4629368410562620, 294.6297622202381490, -3.542282447166476445 ) ) ;
#52327=CARTESIAN_POINT ( 'NONE',  ( 156.9763224152064822, 271.9908631200777904, -15.29896765642516776 ) ) ;
#52328=CARTESIAN_POINT ( 'NONE',  ( 103.2234855318352373, 223.7365022471902023, -10.00000000000009237 ) ) ;
#52329=CARTESIAN_POINT ( 'NONE',  ( 173.7730331013573277, 252.4040569639470846, -3.903565288969256475 ) ) ;
#52330=CARTESIAN_POINT ( 'NONE',  ( 43.63930707798317599, 189.8768266524159856, -9.188101187500091527 ) ) ;
#52331=CARTESIAN_POINT ( 'NONE',  ( 147.8030175879119099, 276.3716628640393651, -2.406150248769625133 ) ) ;
#52332=ORIENTED_EDGE ( 'NONE', *, *, #23907, .F. ) ;
#52333=CARTESIAN_POINT ( 'NONE',  ( 190.4867865949766781, 299.1946217176854930, 7.408943446041265979 ) ) ;
#52334=CARTESIAN_POINT ( 'NONE',  ( 180.6467591333264409, 267.4216841736908350, 15.01138547461691530 ) ) ;
#52335=EDGE_CURVE ( 'NONE', #41077, #24776, #51866, .T. ) ;
#52337=EDGE_CURVE ( 'NONE', #22391, #77084, #60266, .T. ) ;
#52338=CARTESIAN_POINT ( 'NONE',  ( 146.8195026170398023, 276.3481572557323034, 4.765869558735466249 ) ) ;
#52343=CARTESIAN_POINT ( 'NONE',  ( 105.1540004908901693, 221.5177522451418213, 5.000000000000051514 ) ) ;
#52345=CARTESIAN_POINT ( 'NONE',  ( 195.0119942166254248, 266.5109991209683358, -7.745506184336903743 ) ) ;
#52346=CARTESIAN_POINT ( 'NONE',  ( 155.2511492336869310, 280.0303029816861908, -2.338817866916156785 ) ) ;
#52347=CARTESIAN_POINT ( 'NONE',  ( 154.4564338973504789, 263.9603729957919995, 16.89342759845790809 ) ) ;
#52348=CLOSED_SHELL ( 'NONE', ( #49198, #36063, #6735, #68783, #97478, #57939, #66269, #45442, #12960, #85855, #1502, #79496, #29363, #15853, #45545, #56561, #42618, #75835, #47058, #67238, #77027, #76630, #84078, #43046, #70613, #73703, #7158, #40789, #40600, #61476, #22780, #2170, #28058, #2775, #12353, #33627, #2120, #91695, #8305, #72787, #4503, #37830, #67290, #71769, #43957, #19976, #12854, #63995, #6677, #18157, #95755, #59364, #49114, #42059, #41860, #4010, #82902, #27673, #1618, #41363, #82381, #83122, #26749, #44246, #59797, #2077, #97972, #63598, #50299, #52445, #94838, #98806, #28290, #85135, #81036, #88125, #16013, #70856, #33995, #66877, #80808, #31761, #71501, #3165, #91986, #49146, #75413, #53395, #23038, #57847, #75783, #61693, #13045, #51102, #85396, #87556, #91793, #39508, #1440, #87756, #58509, #60014, #12225, #4088, #84882, #66005, #84196, #48039, #92122, #67775, #57252, #4008, #40347, #49383, #24364, #6725, #68189, #61678, #18182, #13768, #86272, #4134, #56348, #10182, #1326, #51825, #96265, #16102, #59803, #7284, #76350, #32705, #56620, #61270, #29042, #98087, #32237, #64178, #72589, #94978, #52828, #24908, #69080, #25500, #65385, #66434, #4339, #67812, #32441, #83869, #5818, #64697, #83166, #14482, #62272, #77212, #76383, #88475, #47600, #70216, #99108, #43830, #35150, #61144, #10301, #54760, #36079, #48694, #77244, #21279, #92374, #22834, #82141, #70597, #64566, #96559, #52896, #57, #69606, #28831, #60406, #53025, #17147, #30070, #31082, #42495, #77289, #2634, #32106, #84384, #65268, #49497, #70193, #66067, #82611, #79799, #86373, #31825, #86611, #27776, #68027, #55491, #75530, #55975, #36891, #88673, #25442, #94499, #66685, #59432, #98148, #5041, #33259, #225, #52777, #39739, #27785, #83678, #85546, #88185, #7866, #38642, #38167, #90638, #58189, #79228, #31645, #9581, #1032, #57976, #20716, #97005, #21047, #92237, #18333, #9784, #5843, #70850, #37873, #8558, #93129, #14426, #42966, #38465, #26256, #46730, #96509, #90298, #79978, #95780, #13835, #58311, #42959, #32878, #61640, #16314, #25638, #12087, #79031, #44101, #2769, #55256, #72055, #71429, #86047, #51326, #25958, #62065, #82562, #18982, #56231, #30726, #81484, #48555, #49711, #62018, #23757, #100137, #45870, #15974, #95094, #74422, #47776, #10070, #54900, #22190, #58801, #84763, #9721, #928, #94516, #90462, #491, #39142, #30289, #28320, #41086, #83996, #55442, #71827, #64059, #85363, #63806, #5266, #89195, #39308, #50298, #48952, #17197, #26280, #64368, #87835, #12610, #50536, #2721, #45014, #7046, #82247, #81347, #2400, #46294, #49915, #344, #35103, #32741, #96283, #5356, #73336, #31294, #59143, #22406, #39060, #54769, #99210, #23284, #65505, #16224, #98468, #8243, #79109, #42485, #33042, #47572, #25426, #90156, #4657, #8351, #31134, #77286, #33179, #43576, #44623, #35639, #90693, #48751, #27089, #20012, #94650, #50418, #90712, #58624, #31139, #18651, #93459, #7995, #90741, #78000, #78759, #96218, #25158, #9564, #43314, #71615, #66282, #74180, #5692, #57453, #98694, #14156, #67112, #51717, #100207, #77754, #7632, #86215, #82501, #48425, #63437, #71055, #52818, #91831, #6210, #27945, #22642, #6468, #11785, #46589, #48038, #49349, #29838, #92753, #44996, #3417, #20220, #50317, #95204, #83180, #80818, #44807, #6520, #3468, #61448, #68078, #59305, #79368, #30587, #48942, #35194, #89981, #85655, #2044, #7533, #57669, #18065, #27094, #25717, #11720, #53814, #37467, #15848, #55517, #42418, #52262, #47337, #36783, #70187, #40594, #83293, #88306, #94024, #69218, #63098, #39365, #20801, #89491, #21263, #39769, #77503, #57404, #42621, #35777, #4397, #85724, #37532, #56483, #6531, #67526, #33920, #82392, #76408, #35576, #39241, #53161, #15881, #3231, #73394, #87766, #45496, #49443, #43, #60446, #86056, #19609, #84427, #89602, #43990, #72724, #65425, #72904, #4452, #12425, #79188, #79659, #71191, #8665, #81437, #76937, #1588, #82868, #74410, #10751, #65009, #6466, #4257, #41026, #86406, #23785, #44403, #21599, #13388, #23150, #61130, #85953, #24929, #82395, #95157, #78560, #37635, #29510, #69152, #63463, #31929, #8221, #14040, #31376, #13265, #99292 ) ) ;
#52349=CARTESIAN_POINT ( 'NONE',  ( 11.29875767934929520, 168.1423013555409796, -4.594050593750043987 ) ) ;
#52354=CARTESIAN_POINT ( 'NONE',  ( 196.2529602075856303, 276.1688732195831335, -15.37645340877904232 ) ) ;
#52355=CARTESIAN_POINT ( 'NONE',  ( 43.17879721251643588, 204.9244531367911293, -4.594050593750046652 ) ) ;
#52356=CARTESIAN_POINT ( 'NONE',  ( 207.8060684685902686, 270.7163266217015689, 2.015725026008670540 ) ) ;
#52363=CARTESIAN_POINT ( 'NONE',  ( 4.352251933111777049, 179.9865022471903160, -10.00000000000009415 ) ) ;
#52364=CARTESIAN_POINT ( 'NONE',  ( 164.4989226152910646, 245.7265035704120351, -6.575810094723514965 ) ) ;
#52365=CIRCLE ( 'NONE', #45916, 17.82106496071138224 ) ;
#52366=CARTESIAN_POINT ( 'NONE',  ( 133.7599021114188247, 248.0333772461660544, 9.188101187500095079 ) ) ;
#52368=CARTESIAN_POINT ( 'NONE',  ( 207.4128166479680999, 271.3974587551883246, -8.231682050742898937 ) ) ;
#52370=EDGE_CURVE ( 'NONE', #69971, #22854, #77346, .T. ) ;
#52374=CARTESIAN_POINT ( 'NONE',  ( 186.1237447414861208, 288.2118312591220501, 14.66121385500803243 ) ) ;
#52377=ORIENTED_EDGE ( 'NONE', *, *, #91127, .F. ) ;
#52378=CARTESIAN_POINT ( 'NONE',  ( 150.7226148805041817, 269.5877685077668957, 15.52819754351937576 ) ) ;
#52379=CARTESIAN_POINT ( 'NONE',  ( 208.4117778882290395, 269.6672071322645934, -0.9948548485616270920 ) ) ;
#52381=CARTESIAN_POINT ( 'NONE',  ( 171.6540594275769820, 267.3410371765079958, -16.37976297547299254 ) ) ;
#52382=CARTESIAN_POINT ( 'NONE',  ( 197.2267182245235801, 273.1434563419713868, -13.38223132498687740 ) ) ;
#52383=EDGE_LOOP ( 'NONE', ( #23876, #61375, #95746, #48696, #56526 ) ) ;
#52388=CARTESIAN_POINT ( 'NONE',  ( 196.3539419194680704, 270.6706703227201842, 13.29218896581975962 ) ) ;
#52392=CARTESIAN_POINT ( 'NONE',  ( 190.8353261179822766, 280.9707072899906848, 16.64952221345274808 ) ) ;
#52401=CARTESIAN_POINT ( 'NONE',  ( 179.0685761320505947, 258.5468394390073286, -11.57600102548048149 ) ) ;
#52402=CARTESIAN_POINT ( 'NONE',  ( 204.6780326111993986, 276.1342436545999703, 14.85609018352459287 ) ) ;
#52404=ORIENTED_EDGE ( 'NONE', *, *, #90618, .T. ) ;
#52405=CARTESIAN_POINT ( 'NONE',  ( 94.43719644265542001, 216.1423013555410080, -4.594050593750043987 ) ) ;
#52406=CARTESIAN_POINT ( 'NONE',  ( 155.0836044121125212, 262.0343130677450745, 18.31269374395214200 ) ) ;
#52411=VERTEX_POINT ( 'NONE', #66714 ) ;
#52417=CARTESIAN_POINT ( 'NONE',  ( 164.3990608653545848, 245.8994691950343565, 2.256889790035259136 ) ) ;
#52423=CARTESIAN_POINT ( 'NONE',  ( 165.0952605416836718, 264.4120569475813340, -17.48790325852768746 ) ) ;
#52425=CARTESIAN_POINT ( 'NONE',  ( 198.8683739244561082, 276.4215138120039796, -15.93986209720707414 ) ) ;
#52427=ORIENTED_EDGE ( 'NONE', *, *, #60429, .T. ) ;
#52428=CARTESIAN_POINT ( 'NONE',  ( 164.2034818126556388, 281.6578577422810099, 8.819376076490621941 ) ) ;
#52431=CARTESIAN_POINT ( 'NONE',  ( 202.4323889586180201, 280.0238125565655878, 15.69595176008160919 ) ) ;
#52432=CARTESIAN_POINT ( 'NONE',  ( 188.1054269039565554, 260.7416112581689731, 2.841567442216401229 ) ) ;
#52433=CARTESIAN_POINT ( 'NONE',  ( 160.7588997986945856, 282.5491429314030825, -6.341079064894056927 ) ) ;
#52437=CARTESIAN_POINT ( 'NONE',  ( 171.3610447788964848, 255.5874900960222078, 11.20421736224005471 ) ) ;
#52438=CARTESIAN_POINT ( 'NONE',  ( 157.7190474710035062, 281.4620898344580837, 1.428472196222973389 ) ) ;
#52440=CARTESIAN_POINT ( 'NONE',  ( 194.4754212959730353, 293.8056848224490523, -15.50536285337042486 ) ) ;
#52442=CARTESIAN_POINT ( 'NONE',  ( 193.8271347420676420, 294.1030254116506626, -14.13191673250339164 ) ) ;
#52443=CARTESIAN_POINT ( 'NONE',  ( -4.903394573382326094, 174.6427522451419350, -10.00000000000009415 ) ) ;
#52445=ADVANCED_FACE ( 'NONE', ( #54739 ), #70455, .T. ) ;
#52446=CARTESIAN_POINT ( 'NONE',  ( 194.2120287517171846, 268.3159770147244103, -10.84597068469714110 ) ) ;
#52447=CARTESIAN_POINT ( 'NONE',  ( 174.6775312387305519, 281.2009762962929358, -14.18005191487551997 ) ) ;
#52448=CARTESIAN_POINT ( 'NONE',  ( 163.3833816344594538, 247.6586772271373889, -8.552920238416389154 ) ) ;
#52449=CARTESIAN_POINT ( 'NONE',  ( 173.2717237769409451, 287.6101323724053032, -10.33903262687377023 ) ) ;
#52450=CARTESIAN_POINT ( 'NONE',  ( 161.0428786693140637, 272.6820104255564274, 15.30257686379266602 ) ) ;
#52451=CARTESIAN_POINT ( 'NONE',  ( -6.102853504003019403, 155.0327760586659451, 1.948934522072303157E-15 ) ) ;
#52452=CARTESIAN_POINT ( 'NONE',  ( -6.467605121757557640, 178.6199935810940929, 2.679491924311251605 ) ) ;
#52453=CARTESIAN_POINT ( 'NONE',  ( 185.8119420094102168, 295.3841422132845196, 8.236304765045641574 ) ) ;
#52457=CARTESIAN_POINT ( 'NONE',  ( 170.8054577101068219, 287.4915981561377976, 8.526299399445241178 ) ) ;
#52459=CARTESIAN_POINT ( 'NONE',  ( 175.1279731406782787, 290.6895847248729865, 2.563404365050127698 ) ) ;
#52460=CYLINDRICAL_SURFACE ( 'NONE', #85812, 10.00000000000010658 ) ;
#52464=CARTESIAN_POINT ( 'NONE',  ( 150.2998784792504807, 276.6058365846234324, 3.694584881749327643 ) ) ;
#52465=CARTESIAN_POINT ( 'NONE',  ( 28.37560933628243731, 181.0643266524159856, -9.188101187500093303 ) ) ;
#52466=CARTESIAN_POINT ( 'NONE',  ( 120.4447615282330588, 240.3458772461660544, 9.188101187500095079 ) ) ;
#52467=LINE ( 'NONE', #83412, #35373 ) ;
#52470=CARTESIAN_POINT ( 'NONE',  ( 178.4791421146993571, 283.9042546283926072, -14.94796090157607971 ) ) ;
#52471=CARTESIAN_POINT ( 'NONE',  ( 69.21394623383595501, 200.7677522451417929, -5.000000000000041744 ) ) ;
#52473=CARTESIAN_POINT ( 'NONE',  ( 183.9255502157922422, 275.0530541881162776, 16.36233669867407414 ) ) ;
#52477=CARTESIAN_POINT ( 'NONE',  ( 186.8181860056460550, 298.9265138730379476, -0.6012193119006525865 ) ) ;
#52478=CARTESIAN_POINT ( 'NONE',  ( 46.83931157395847578, 209.3967562850346837, 1.101618078115930403E-13 ) ) ;
#52479=CARTESIAN_POINT ( 'NONE',  ( 64.52297529667023923, 201.3927522451418213, 10.00000000000009948 ) ) ;
#52482=CARTESIAN_POINT ( 'NONE',  ( 181.8281974864600272, 268.1150286880662748, 15.00885672120805481 ) ) ;
#52483=CARTESIAN_POINT ( 'NONE',  ( 94.00418374076319594, 215.8923013555410080, 4.594050593750050204 ) ) ;
#52484=CARTESIAN_POINT ( 'NONE',  ( 161.8882824960653579, 250.2482648971885340, -13.83574485983625557 ) ) ;
#52486=CARTESIAN_POINT ( 'NONE',  ( 157.8230096946041954, 258.6542051802886135, -16.94987972545947841 ) ) ;
#52487=CARTESIAN_POINT ( 'NONE',  ( 157.8740713127050981, 257.2010826190796706, 17.31862062017425075 ) ) ;
#52488=CARTESIAN_POINT ( 'NONE',  ( 152.5108720042611026, 266.4904163124226670, 16.32854172121686531 ) ) ;
#52489=CARTESIAN_POINT ( 'NONE',  ( 201.1851683271005413, 270.3619535279936485, -10.11376747734130532 ) ) ;
#52490=CARTESIAN_POINT ( 'NONE',  ( -22.42236680055709641, 157.8615022471902591, 0.000000000000000000 ) ) ;
#52491=CARTESIAN_POINT ( 'NONE',  ( 173.4606779374792325, 267.5814416807811540, -17.58000433512257032 ) ) ;
#52493=CARTESIAN_POINT ( 'NONE',  ( 147.4323331177958494, 275.2867036919951147, -5.064030047414062707 ) ) ;
#52497=CARTESIAN_POINT ( 'NONE',  ( 156.3709700504638818, 275.5026625584495719, -12.72272160619075088 ) ) ;
#52498=CARTESIAN_POINT ( 'NONE',  ( 147.4563929227680603, 275.2450308873625886, -3.847749617713808412 ) ) ;
#52499=CARTESIAN_POINT ( 'NONE',  ( 149.3801359649374092, 271.9130101976182914, -11.41245530317637424 ) ) ;
#52505=CARTESIAN_POINT ( 'NONE',  ( 173.0163677133065789, 253.2660320162962080, -9.300034630933833313 ) ) ;
#52507=CARTESIAN_POINT ( 'NONE',  ( 148.6176504468695896, 246.6115022471902023, -5.000000000000041744 ) ) ;
#52508=ORIENTED_EDGE ( 'NONE', *, *, #80079, .F. ) ;
#52509=CARTESIAN_POINT ( 'NONE',  ( 86.94711308317737064, 232.5530062829863027, -4.648177544792955347E-16 ) ) ;
#52511=CARTESIAN_POINT ( 'NONE',  ( 163.1332433029523372, 248.0919295262283981, 11.24052392390482957 ) ) ;
#52512=FACE_OUTER_BOUND ( 'NONE', #51807, .T. ) ;
#52513=EDGE_LOOP ( 'NONE', ( #59234, #29663, #55717, #62610, #54804, #95520, #17909, #87999, #86681, #86629, #50628, #12367, #66406, #82385, #56285, #20035, #91966, #27767, #84245, #62778 ) ) ;
#52514=CARTESIAN_POINT ( 'NONE',  ( 184.8823494725930345, 293.3934917266262232, -10.47977162542887797 ) ) ;
#52519=CARTESIAN_POINT ( 'NONE',  ( 190.6920532893590234, 278.3349890342503272, -16.61725499987922916 ) ) ;
#52520=CARTESIAN_POINT ( 'NONE',  ( 153.4580622222703710, 264.8498347303985838, -17.93314668316356375 ) ) ;
#52521=CARTESIAN_POINT ( 'NONE',  ( 152.8651171364917900, 265.8768457450651113, -16.25664868183201861 ) ) ;
#52522=EDGE_CURVE ( 'NONE', #44273, #74117, #26792, .T. ) ;
#52524=CARTESIAN_POINT ( 'NONE',  ( 149.2341712975190546, 276.7904698848887506, 4.784570376893943155 ) ) ;
#52531=( BOUNDED_CURVE ( )  B_SPLINE_CURVE ( 2, ( #96836, #97810, #28378, #89737, #66389 ),
 .UNSPECIFIED., .F., .T. ) 
 B_SPLINE_CURVE_WITH_KNOTS ( ( 3, 2, 3 ),
 ( 0.000000000000000000, 0.002688172043010752903, 0.004032258064516129788 ),
 .UNSPECIFIED. ) 
 CURVE ( )  GEOMETRIC_REPRESENTATION_ITEM ( )  RATIONAL_B_SPLINE_CURVE ( ( 1.000000000000000000, 0.8660254037844387076, 1.000000000000000000, 0.9330127018922194093, 0.9330127018922194093 ) ) 
 REPRESENTATION_ITEM ( '' )  );
#52532=CARTESIAN_POINT ( 'NONE',  ( 164.3961040135806968, 245.9045906125373904, 7.095190383188031191 ) ) ;
#52533=CARTESIAN_POINT ( 'NONE',  ( 162.3275777969640785, 272.2924995007368238, -15.82782416072089582 ) ) ;
#52534=CARTESIAN_POINT ( 'NONE',  ( 164.8329707752360491, 245.1479151852119855, -0.9471001479485156027 ) ) ;
#52536=CARTESIAN_POINT ( 'NONE',  ( 148.0427192501136062, 274.2294838985851015, 9.385226820296049155 ) ) ;
#52537=CARTESIAN_POINT ( 'NONE',  ( 167.8377799047650853, 286.2760919531912123, -4.720521751261225418 ) ) ;
#52539=B_SPLINE_CURVE_WITH_KNOTS ( 'NONE', 3,
 ( #6323, #68610, #6818, #45795 ),
 .UNSPECIFIED., .F., .F.,
 ( 4, 4 ),
 ( 0.009431354028234023926, 0.01481778605290438866 ),
 .UNSPECIFIED. ) ;
#52540=CARTESIAN_POINT ( 'NONE',  ( 185.8250471888061099, 286.2195783377563316, -15.25737745182902927 ) ) ;
#52541=CARTESIAN_POINT ( 'NONE',  ( 114.4904897814500515, 249.1589784336661069, -6.496448406907675876E-16 ) ) ;
#52542=CARTESIAN_POINT ( 'NONE',  ( 183.6651092691634801, 260.0572973937465804, -9.581159380197425079 ) ) ;
#52544=CARTESIAN_POINT ( 'NONE',  ( 189.2781344870356861, 274.0445645723327743, 15.70124837302617316 ) ) ;
#52546=AXIS2_PLACEMENT_3D ( 'NONE', #77708, #54877, #30092 ) ;
#52548=CARTESIAN_POINT ( 'NONE',  ( 164.8050118924691958, 246.2012700071148572, -2.717544611603450733 ) ) ;
#52549=CARTESIAN_POINT ( 'NONE',  ( 157.1837449796689725, 258.3967629017010381, 16.97243084443542216 ) ) ;
#52553=FACE_OUTER_BOUND ( 'NONE', #98399, .T. ) ;
#52554=ORIENTED_EDGE ( 'NONE', *, *, #47452, .F. ) ;
#52556=ORIENTED_EDGE ( 'NONE', *, *, #61642, .F. ) ;
#52557=CARTESIAN_POINT ( 'NONE',  ( 205.9240884482826175, 273.9760116357041966, 10.27504561427317142 ) ) ;
#52558=CARTESIAN_POINT ( 'NONE',  ( 195.6450799796529054, 265.3427675445001910, 4.393462682352039295 ) ) ;
#52561=FACE_OUTER_BOUND ( 'NONE', #27792, .T. ) ;
#52562=CYLINDRICAL_SURFACE ( 'NONE', #41472, 17.82106496071139645 ) ;
#52563=CARTESIAN_POINT ( 'NONE',  ( 199.1744935446041893, 274.6029352898955267, -14.95876376616611125 ) ) ;
#52565=CARTESIAN_POINT ( 'NONE',  ( 157.2674082780516471, 258.2518538181732879, 18.34755329151241554 ) ) ;
#52568=CARTESIAN_POINT ( 'NONE',  ( 170.0871025661366787, 249.0337905125704765, -0.2639721576281350846 ) ) ;
#52569=CARTESIAN_POINT ( 'NONE',  ( 191.9809540880537497, 271.5427279282940276, -14.38588033665278410 ) ) ;
#52576=CARTESIAN_POINT ( 'NONE',  ( 191.1760382422123428, 283.2354439422711039, -16.61270921724900518 ) ) ;
#52578=EDGE_CURVE ( 'NONE', #93829, #59249, #16683, .T. ) ;
#52579=CARTESIAN_POINT ( 'NONE',  ( 85.88519558028406209, 211.2048013555409796, 4.594050593750051981 ) ) ;
#52580=CARTESIAN_POINT ( 'NONE',  ( 206.6298919378964740, 272.7535241315335384, -9.267551915974392429 ) ) ;
#52583=EDGE_CURVE ( 'NONE', #46006, #73115, #8255, .T. ) ;
#52585=CARTESIAN_POINT ( 'NONE',  ( 161.5083988044524119, 250.9062427520286178, -14.53522982831775856 ) ) ;
#52587=CARTESIAN_POINT ( 'NONE',  ( 108.7544814380518403, 222.0494855054051868, -2.679491924311248496 ) ) ;
#52590=CARTESIAN_POINT ( 'NONE',  ( 182.5686778644665083, 296.6873302901632314, 1.787712280751329708 ) ) ;
#52593=CARTESIAN_POINT ( 'NONE',  ( 22.39418752168989712, 192.9244531367911293, -4.594050593750046652 ) ) ;
#52598=CARTESIAN_POINT ( 'NONE',  ( 56.25097556847656932, 191.0327760586659451, 1.948934522072302763E-15 ) ) ;
#52601=DIRECTION ( 'NONE',  ( -0.4999999999999987788, 0.8660254037844392627, 0.000000000000000000 ) ) ;
#52602=CARTESIAN_POINT ( 'NONE',  ( -6.813555604197667037, 155.3262482093457777, -6.972266317189433020E-16 ) ) ;
#52604=CARTESIAN_POINT ( 'NONE',  ( 204.8878784573704195, 275.7707799872745795, -14.13380496213581594 ) ) ;
#52605=CARTESIAN_POINT ( 'NONE',  ( 197.7454084947095225, 287.3707299168542590, 17.08123495905502764 ) ) ;
#52607=CARTESIAN_POINT ( 'NONE',  ( 180.0410653043650484, 276.3720869110510421, 17.51637908678287303 ) ) ;
#52609=CARTESIAN_POINT ( 'NONE',  ( 153.1402462294643385, 276.7372565758790302, 7.179079264927311854 ) ) ;
#52610=CARTESIAN_POINT ( 'NONE',  ( 163.3011861648808178, 256.0630655445800130, -14.91776478601246048 ) ) ;
#52611=FACE_OUTER_BOUND ( 'NONE', #88854, .T. ) ;
#52613=CARTESIAN_POINT ( 'NONE',  ( 94.05805000844988228, 235.1115022471902876, -5.000000000000047962 ) ) ;
#52614=CARTESIAN_POINT ( 'NONE',  ( 161.1611771195837548, 251.5076483517112536, 14.17749514252127163 ) ) ;
#52615=CARTESIAN_POINT ( 'NONE',  ( 194.7136160084532719, 285.5689873031276989, -17.40128518539645697 ) ) ;
#52617=CARTESIAN_POINT ( 'NONE',  ( 66.15596757637857195, 202.8768266524160140, 9.188101187500098632 ) ) ;
#52618=VERTEX_POINT ( 'NONE', #19218 ) ;
#52619=CARTESIAN_POINT ( 'NONE',  ( 185.5568049818104726, 266.1438378612298834, 14.60334785453874140 ) ) ;
#52620=CARTESIAN_POINT ( 'NONE',  ( 190.3625087333586521, 300.9294583479858147, -4.271886578030237303 ) ) ;
#52621=CARTESIAN_POINT ( 'NONE',  ( -22.42236680055709641, 157.8615022471902591, 0.000000000000000000 ) ) ;
#52627=CARTESIAN_POINT ( 'NONE',  ( 206.9068930164517894, 271.8479423001995769, -5.981710879645867784 ) ) ;
#52629=CARTESIAN_POINT ( 'NONE',  ( 204.8467418195402843, 275.8420307340491036, 13.15258587511997135 ) ) ;
#52633=CARTESIAN_POINT ( 'NONE',  ( 175.4496532655798262, 254.2869214701858880, 7.959120167633201071 ) ) ;
#52634=CARTESIAN_POINT ( 'NONE',  ( 176.5950604002042326, 276.4255102086987108, 17.53915386444770519 ) ) ;
#52637=CARTESIAN_POINT ( 'NONE',  ( 159.6962080797732710, 254.0450491601782232, -15.33973334987084947 ) ) ;
#52639=ORIENTED_EDGE ( 'NONE', *, *, #20338, .F. ) ;
#52644=CARTESIAN_POINT ( 'NONE',  ( 204.7610021263893429, 275.9905362388115577, 13.36619428527026976 ) ) ;
#52645=CARTESIAN_POINT ( 'NONE',  ( 159.9671766634011192, 253.5757178060795809, 16.49140845334465411 ) ) ;
#52647=CARTESIAN_POINT ( 'NONE',  ( 164.4290154601662550, 264.9784679568533079, -16.63390713968286860 ) ) ;
#52650=CARTESIAN_POINT ( 'NONE',  ( 127.8056303646358032, 256.8464784336661637, 1.353441290958777525E-15 ) ) ;
#52651=CARTESIAN_POINT ( 'NONE',  ( 160.2740869459746023, 254.0686150970925610, -15.36085255641610914 ) ) ;
#52652=B_SPLINE_CURVE_WITH_KNOTS ( 'NONE', 3,
 ( #14344, #45718, #99456, #59927 ),
 .UNSPECIFIED., .F., .F.,
 ( 4, 4 ),
 ( 0.004744422519644171318, 0.01275308626033747235 ),
 .UNSPECIFIED. ) ;
#52653=CARTESIAN_POINT ( 'NONE',  ( 68.75404378773190217, 204.3768266524160140, 9.188101187500098632 ) ) ;
#52656=CARTESIAN_POINT ( 'NONE',  ( 174.1529052279448706, 265.6236375338058906, 16.55384635694815287 ) ) ;
#52658=EDGE_LOOP ( 'NONE', ( #95727, #32709, #88096 ) ) ;
#52659=CARTESIAN_POINT ( 'NONE',  ( 166.7004263218490223, 257.9657675534214718, 15.99763568028711092 ) ) ;
#52664=CARTESIAN_POINT ( 'NONE',  ( 194.7767398707621282, 285.0350113515720523, 17.12152913950285082 ) ) ;
#52665=CARTESIAN_POINT ( 'NONE',  ( 147.2592533090473239, 275.5864867145116932, -0.3770461397900867762 ) ) ;
#52667=CARTESIAN_POINT ( 'NONE',  ( 194.4904290197884507, 293.7796906822950973, 14.50206953321744940 ) ) ;
#52668=CARTESIAN_POINT ( 'NONE',  ( 77.17055463465335663, 215.3615022471902591, -10.00000000000009592 ) ) ;
#52674=CARTESIAN_POINT ( 'NONE',  ( 174.5345741576458920, 253.2528832121751634, -7.801788862502708533 ) ) ;
#52675=CARTESIAN_POINT ( 'NONE',  ( 191.0843498247698733, 299.6791929026704793, 6.354791142140047810 ) ) ;
#52676=CARTESIAN_POINT ( 'NONE',  ( 206.5479446040613141, 272.8954610772809133, 10.74757481123993230 ) ) ;
#52677=VECTOR ( 'NONE', #89413, 1000.000000000000000 ) ;
#52678=CARTESIAN_POINT ( 'NONE',  ( 37.33338606056913989, 202.3615022471903160, 5.000000000000046185 ) ) ;
#52679=CARTESIAN_POINT ( 'NONE',  ( 198.4160757083882345, 267.1808215963346242, -8.346050686629251203 ) ) ;
#52680=CARTESIAN_POINT ( 'NONE',  ( 138.1714793337695824, 241.3923013555409796, 4.594050593750050204 ) ) ;
#52681=VERTEX_POINT ( 'NONE', #49582 ) ;
#52683=CARTESIAN_POINT ( 'NONE',  ( 183.1817924123992327, 258.9247982590615607, 6.387075791788588752 ) ) ;
#52687=CARTESIAN_POINT ( 'NONE',  ( 147.7840609055601817, 276.6774932931532476, -0.9735537997635442808 ) ) ;
#52689=ORIENTED_EDGE ( 'NONE', *, *, #14832, .T. ) ;
#52690=CARTESIAN_POINT ( 'NONE',  ( 199.4720805209845196, 266.1420231043892954, 4.760232788326643316 ) ) ;
#52691=CARTESIAN_POINT ( 'NONE',  ( 188.2520712372829621, 265.6420100395978920, -13.17850047611677766 ) ) ;
#52694=CARTESIAN_POINT ( 'NONE',  ( 198.8095285574927118, 266.4036850393262625, 0.8273979317567071723 ) ) ;
#52695=CARTESIAN_POINT ( 'NONE',  ( 197.8117387002072860, 265.8538865084539111, 0.8196971304707719730 ) ) ;
#52696=ADVANCED_FACE ( 'NONE', ( #65773 ), #82539, .F. ) ;
#52697=CARTESIAN_POINT ( 'NONE',  ( 190.2648877593310317, 301.0985428348857340, -4.426259207433023590 ) ) ;
#52698=CARTESIAN_POINT ( 'NONE',  ( 185.3455588379956112, 281.9002770091811385, 16.19074574515159526 ) ) ;
#52701=CARTESIAN_POINT ( 'NONE',  ( 157.7847820078105201, 257.3557362317297361, -18.02899742403477035 ) ) ;
#52705=CARTESIAN_POINT ( 'NONE',  ( 205.3750807262146907, 274.5182765027618075, 11.14488729068320616 ) ) ;
#52708=CARTESIAN_POINT ( 'NONE',  ( 159.6419305724666344, 254.1390605605417079, 16.92015248457581933 ) ) ;
#52710=CARTESIAN_POINT ( 'NONE',  ( 143.2591182574054187, 253.5177522451418497, -10.00000000000009592 ) ) ;
#52711=CARTESIAN_POINT ( 'NONE',  ( 175.9106323274208705, 285.6143439489698039, -11.86405137256001296 ) ) ;
#52716=CARTESIAN_POINT ( 'NONE',  ( 198.7357616895271804, 286.4265588032756114, -17.04018524297827497 ) ) ;
#52717=CARTESIAN_POINT ( 'NONE',  ( 2.773212693257451900, 184.6589784336661637, -6.496448406907676862E-16 ) ) ;
#52718=CARTESIAN_POINT ( 'NONE',  ( 181.7028333219653291, 276.2859026444305073, -16.76116147531152833 ) ) ;
#52721=CARTESIAN_POINT ( 'NONE',  ( 171.3171204526115616, 271.4791138034659070, -17.75561031716327420 ) ) ;
#52723=CARTESIAN_POINT ( 'NONE',  ( 149.9796301194747343, 276.8100220917153251, 4.535783967717629928 ) ) ;
#52724=CARTESIAN_POINT ( 'NONE',  ( 175.5717179822201217, 253.3804273325372378, -3.507250143043896262 ) ) ;
#52725=CARTESIAN_POINT ( 'NONE',  ( 198.7564336180209068, 286.3907539728338634, 17.89468790901915796 ) ) ;
#52726=CARTESIAN_POINT ( 'NONE',  ( 56.31377616017817900, 189.9865022471901455, 1.119607411625061291E-15 ) ) ;
#52728=CARTESIAN_POINT ( 'NONE',  ( 190.1158090214649405, 301.3567547831981983, -1.340987185199551845 ) ) ;
#52729=CARTESIAN_POINT ( 'NONE',  ( 16.87327557256410060, 189.7369531367911293, -4.594050593750048428 ) ) ;
#52734=CARTESIAN_POINT ( 'NONE',  ( -22.42236680055709641, 157.8615022471902591, 0.000000000000000000 ) ) ;
#52735=CARTESIAN_POINT ( 'NONE',  ( 188.6005607789109320, 267.5261675405737378, 14.22050808917637887 ) ) ;
#52736=CARTESIAN_POINT ( 'NONE',  ( 153.8480465357228013, 265.0660884932569843, -16.61306390558784685 ) ) ;
#52737=CARTESIAN_POINT ( 'NONE',  ( 164.2037877926934470, 281.4932537616303421, 9.235950372291741317 ) ) ;
#52740=CARTESIAN_POINT ( 'NONE',  ( 148.4049257185216106, 273.6021238924720365, 8.639190357831699529 ) ) ;
#52742=AXIS2_PLACEMENT_3D ( 'NONE', #20463, #67537, #90399 ) ;
#52744=CARTESIAN_POINT ( 'NONE',  ( 203.6925490392534925, 269.5270927311577793, 7.084861529579629114 ) ) ;
#52749=EDGE_CURVE ( 'NONE', #77084, #7044, #85640, .T. ) ;
#52754=CARTESIAN_POINT ( 'NONE',  ( 154.8545429534089237, 262.4310591522755089, -17.81746354318405778 ) ) ;
#52755=ORIENTED_EDGE ( 'NONE', *, *, #81928, .T. ) ;
#52757=FACE_OUTER_BOUND ( 'NONE', #34584, .T. ) ;
#52758=CARTESIAN_POINT ( 'NONE',  ( 204.9004517216375518, 275.7490024547470853, 14.55104398969427670 ) ) ;
#52760=CARTESIAN_POINT ( 'NONE',  ( 151.2648146047323507, 268.6486510375538614, 15.71323890031163550 ) ) ;
#52766=DIRECTION ( 'NONE',  ( 0.4999999999999998890, -0.8660254037844385966, 0.000000000000000000 ) ) ;
#52767=CARTESIAN_POINT ( 'NONE',  ( 196.8435556370661459, 289.7039558245273838, -16.43899056939217118 ) ) ;
#52769=CARTESIAN_POINT ( 'NONE',  ( 206.5318754762992910, 272.9232936229979032, 10.63244694018452741 ) ) ;
#52771=CARTESIAN_POINT ( 'NONE',  ( 194.5725374088679871, 291.6374747806817140, -16.23208319182986870 ) ) ;
#52773=CARTESIAN_POINT ( 'NONE',  ( 190.8187029736043883, 300.1393067457597681, 3.941064102378585954 ) ) ;
#52774=CARTESIAN_POINT ( 'NONE',  ( 200.0577211067540873, 278.4141957227807325, 16.45782674848881300 ) ) ;
#52777=ADVANCED_FACE ( 'NONE', ( #91119 ), #22684, .T. ) ;
#52778=CARTESIAN_POINT ( 'NONE',  ( 188.7267243920021542, 295.1910411013678299, 11.79826141631466463 ) ) ;
#52786=CARTESIAN_POINT ( 'NONE',  ( 190.8683709797118411, 300.0532792356709706, -4.461919767133968762 ) ) ;
#52787=CARTESIAN_POINT ( 'NONE',  ( 190.5969391768923913, 300.5234129089444650, -0.7564693504096553500 ) ) ;
#52789=CARTESIAN_POINT ( 'NONE',  ( -22.42236680055709641, 157.8615022471902591, 0.000000000000000000 ) ) ;
#52791=CARTESIAN_POINT ( 'NONE',  ( 146.6138605399200117, 276.7043397814778132, -0.5394499176159462950 ) ) ;
#52792=B_SPLINE_CURVE_WITH_KNOTS ( 'NONE', 3,
 ( #34740, #3379, #42823, #43833, #42334, #65148, #65642, #5350, #66642, #19076, #97096, #27664, #58532, #82887, #89506, #50938, #81887, #36231, #35746, #97572, #89030, #74282, #72788, #12972, #12463, #96096, #43334, #49952, #96597, #59014, #89983, #26654, #20561, #51439, #74772, #88514, #27161, #67137, #98059, #28636, #59519, #90498, #21071, #51947, #13461, #37232, #68130, #77229 ),
 .UNSPECIFIED., .F., .F.,
 ( 4, 2, 2, 2, 2, 2, 2, 2, 2, 2, 2, 2, 2, 2, 2, 2, 2, 2, 2, 2, 2, 2, 2, 4 ),
 ( 0.0008860715642980536997, 0.0009820465975983500191, 0.001078021630898646230, 0.001173996664198942441, 0.001269971697499238869, 0.001461921764099907185, 0.001653871830700575935, 0.002421672097103298640, 0.003957272629908744482, 0.004725072896311395196, 0.005108973029512683256, 0.005300923096113327286, 0.005396898129413611571, 0.005444885646063752846, 0.005492873162713894121, 0.005540860679364035396, 0.005588848196014176671, 0.005684823229314512130, 0.005876773295915232488, 0.006068723362515953713, 0.006260673429116674071, 0.006452623495717395297, 0.006644573562318115655, 0.007028473695519553768 ),
 .UNSPECIFIED. ) ;
#52794=DIRECTION ( 'NONE',  ( -0.8660254037844387076, -0.4999999999999998890, -0.000000000000000000 ) ) ;
#52797=CARTESIAN_POINT ( 'NONE',  ( 171.3163111156538321, 289.1506865685547041, 4.320660422964803793 ) ) ;
#52798=B_SPLINE_CURVE_WITH_KNOTS ( 'NONE', 3,
 ( #16697, #47589, #70910, #48090, #79032, #9621, #40484, #2004, #25293, #58673, #96741, #20206, #67282, #19718, #57684, #51078, #35388, #98208, #89645, #65783, #49592, #97714, #27304, #66788, #20704, #58188, #88661, #82039, #12614, #28792, #4493, #50583, #13112, #43478, #74423, #5007, #51592, #88162, #35885, #82547, #90132, #41993 ),
 .UNSPECIFIED., .F., .F.,
 ( 4, 2, 2, 2, 2, 2, 2, 2, 2, 2, 2, 2, 2, 2, 2, 2, 2, 2, 2, 2, 4 ),
 ( 0.003272589128710177292, 0.003466937949059250689, 0.003564112359233767655, 0.003661286769408285055, 0.003758461179582802021, 0.003855635589757318987, 0.004049984410106313021, 0.004438682050804295884, 0.004827379691502279614, 0.005604774972898246208, 0.006382170254294213668, 0.007936960817085992465, 0.008131309637435015988, 0.008155603239978690550, 0.008179896842522363376, 0.008204190445066034468, 0.008228484047609709029, 0.008325658457784452376, 0.008714356098483127394, 0.009103053739181800677, 0.009491751379880475695 ),
 .UNSPECIFIED. ) ;
#52801=CARTESIAN_POINT ( 'NONE',  ( 149.5520331575485500, 271.6152755263370295, -13.01004061128467626 ) ) ;
#52802=EDGE_CURVE ( 'NONE', #65018, #30521, #32483, .T. ) ;
#52807=CARTESIAN_POINT ( 'NONE',  ( 191.8650071060532412, 297.4868766427842388, -10.36821096227007288 ) ) ;
#52809=CARTESIAN_POINT ( 'NONE',  ( 169.2499022714398791, 285.3069777449377398, -7.727577981700628484 ) ) ;
#52811=CARTESIAN_POINT ( 'NONE',  ( 163.1096928939807924, 248.1327200311062882, -9.690381021358412283 ) ) ;
#52812=EDGE_CURVE ( 'NONE', #38189, #97286, #79533, .T. ) ;
#52813=CARTESIAN_POINT ( 'NONE',  ( 206.8106726053982811, 272.4404028303941914, -10.47827087991598560 ) ) ;
#52815=CARTESIAN_POINT ( 'NONE',  ( 42.00631479827482195, 188.3927522451418213, -10.00000000000009059 ) ) ;
#52816=CARTESIAN_POINT ( 'NONE',  ( 121.5815934185826421, 234.8768266524159856, -9.188101187500093303 ) ) ;
#52817=CARTESIAN_POINT ( 'NONE',  ( 180.7189620564184054, 294.1892054117222415, -3.206099072908067615 ) ) ;
#52818=ADVANCED_FACE ( 'NONE', ( #61162 ), #74043, .F. ) ;
#52820=CARTESIAN_POINT ( 'NONE',  ( 195.7291534503633272, 291.6341570319625021, 16.44925029361851543 ) ) ;
#52821=CARTESIAN_POINT ( 'NONE',  ( 175.4457714882561561, 253.5523854228639493, -3.987518762506754744 ) ) ;
#52822=CARTESIAN_POINT ( 'NONE',  ( 28.75397480679061246, 199.6589784336661637, -6.496448406907675876E-16 ) ) ;
#52828=ADVANCED_FACE ( 'NONE', ( #32766 ), #24175, .T. ) ;
#52829=CARTESIAN_POINT ( 'NONE',  ( 178.0210747266523867, 265.4709656426701940, 15.86782561207190945 ) ) ;
#52830=EDGE_CURVE ( 'NONE', #52219, #26620, #25165, .T. ) ;
#52831=B_SPLINE_SURFACE_WITH_KNOTS ( 'NONE', 3, 1, ( 
 ( #62555, #8385 ),
 ( #39252, #78293 ),
 ( #23063, #32172 ),
 ( #14493, #63076 ),
 ( #45856, #31658 ),
 ( #70163, #772 ),
 ( #24075, #69171 ),
 ( #45373, #54969 ),
 ( #92515, #17996 ),
 ( #79331, #64589 ),
 ( #88444, #72203 ),
 ( #94519, #3790 ),
 ( #48387, #24571 ),
 ( #71708, #1793 ),
 ( #32676, #2300 ),
 ( #95026, #9382 ),
 ( #48890, #87464 ),
 ( #41260, #26089 ),
 ( #9899, #80839 ),
 ( #10392, #63575 ),
 ( #19003, #25071 ),
 ( #25588, #40757 ),
 ( #55456, #33182 ),
 ( #95542, #55949 ),
 ( #64081, #56475 ),
 ( #41769, #79824 ),
 ( #16968, #86945 ),
 ( #2808, #33696 ),
 ( #56964, #87950 ),
 ( #17478, #18494 ),
 ( #40260, #86441 ),
 ( #26590, #49380 ),
 ( #80323, #94020 ),
 ( #10893, #57463 ) ),
 .UNSPECIFIED., .T., .F., .F.,
 ( 4, 2, 2, 2, 2, 2, 2, 2, 2, 2, 2, 2, 2, 2, 2, 2, 4 ),
 ( 2, 2 ),
 ( 0.000000000000000000, 0.06250000000000000000, 0.1250000000000000000, 0.1875000000000000000, 0.2500000000000000000, 0.3125000000000000000, 0.3750000000000000000, 0.4375000000000000000, 0.5000000000000000000, 0.5625000000000000000, 0.6250000000000000000, 0.6875000000000000000, 0.7500000000000000000, 0.8125000000000000000, 0.8750000000000000000, 0.9375000000000000000, 1.000000000000000000 ),
 ( 0.000000000000000000, 1.000000000000000000 ),
 .UNSPECIFIED. ) ;
#52832=( BOUNDED_CURVE ( )  B_SPLINE_CURVE ( 2, ( #88318, #81691, #18873, #27471, #65449, #4654, #72585, #73562, #65946 ),
 .UNSPECIFIED., .F., .T. ) 
 B_SPLINE_CURVE_WITH_KNOTS ( ( 3, 2, 2, 2, 3 ),
 ( 0.5201612903225806273, 0.5215053763440860024, 0.5241935483870967527, 0.5268817204301075030, 0.5282258064516128782 ),
 .UNSPECIFIED. ) 
 CURVE ( )  GEOMETRIC_REPRESENTATION_ITEM ( )  RATIONAL_B_SPLINE_CURVE ( ( 0.9330127018922194093, 0.9330127018922194093, 1.000000000000000000, 0.8660254037844387076, 1.000000000000000000, 0.8660254037844387076, 1.000000000000000000, 0.9330127018922194093, 0.9330127018922194093 ) ) 
 REPRESENTATION_ITEM ( '' )  );
#52833=DIRECTION ( 'NONE',  ( 0.4999999999999997780, -0.8660254037844388186, 0.000000000000000000 ) ) ;
#52839=CARTESIAN_POINT ( 'NONE',  ( 181.9343943630181855, 262.2755151286456794, 13.05455344133680207 ) ) ;
#52840=( BOUNDED_CURVE ( )  B_SPLINE_CURVE ( 2, ( #40411, #79475, #87098, #31317, #17638, #48536, #33328, #8041, #54104 ),
 .UNSPECIFIED., .F., .T. ) 
 B_SPLINE_CURVE_WITH_KNOTS ( ( 3, 2, 2, 2, 3 ),
 ( 0.1733870967741935609, 0.1747311827956989361, 0.1774193548387096864, 0.1801075268817204367, 0.1814516129032258118 ),
 .UNSPECIFIED. ) 
 CURVE ( )  GEOMETRIC_REPRESENTATION_ITEM ( )  RATIONAL_B_SPLINE_CURVE ( ( 0.9330127018922194093, 0.9330127018922194093, 1.000000000000000000, 0.8660254037844387076, 1.000000000000000000, 0.8660254037844387076, 1.000000000000000000, 0.9330127018922194093, 0.9330127018922194093 ) ) 
 REPRESENTATION_ITEM ( '' )  );
#52841=CARTESIAN_POINT ( 'NONE',  ( 103.4219496833212162, 240.5177522451419350, 5.000000000000046185 ) ) ;
#52844=CARTESIAN_POINT ( 'NONE',  ( 201.5074933251657399, 279.6257787853921286, 16.58790246189369100 ) ) ;
#52845=CARTESIAN_POINT ( 'NONE',  ( 158.8095040752041882, 282.2712473417889782, -1.635881903422608419 ) ) ;
#52847=CARTESIAN_POINT ( 'NONE',  ( 3.585285057187872493, 179.0024278399160949, 9.188101187500095079 ) ) ;
#52849=CARTESIAN_POINT ( 'NONE',  ( 196.1470069647167804, 273.5382448026506381, 15.10109762947431022 ) ) ;
#52852=CARTESIAN_POINT ( 'NONE',  ( 175.5129311542572736, 286.7531494202563067, 10.50704365649472116 ) ) ;
#52853=CARTESIAN_POINT ( 'NONE',  ( 68.45643432912224569, 201.1423013555409796, -4.594050593750043987 ) ) ;
#52854=CARTESIAN_POINT ( 'NONE',  ( 207.5408646414791178, 271.1756731246201753, 3.050859480894625886 ) ) ;
#52858=VERTEX_POINT ( 'NONE', #72300 ) ;
#52860=CARTESIAN_POINT ( 'NONE',  ( 20.01287798488040437, 182.3615022471902591, -10.00000000000009592 ) ) ;
#52861=CARTESIAN_POINT ( 'NONE',  ( 164.0854748117396582, 246.4426161724408928, -5.757837433625331514 ) ) ;
#52862=CARTESIAN_POINT ( 'NONE',  ( 130.4037065759891334, 258.3464784336661637, 1.353441290958777327E-15 ) ) ;
#52868=CARTESIAN_POINT ( 'NONE',  ( 184.7889694759585666, 277.2988950505619528, -17.76348561330697962 ) ) ;
#52869=CARTESIAN_POINT ( 'NONE',  ( 168.4449364156751585, 258.1664367055781213, -15.63070130756588938 ) ) ;
#52871=CARTESIAN_POINT ( 'NONE',  ( 165.3552783545318050, 246.2432519206945472, 4.078954813822171843 ) ) ;
#52872=CARTESIAN_POINT ( 'NONE',  ( 185.9608592076092464, 288.5956984647530703, 15.36535719480430018 ) ) ;
#52873=CARTESIAN_POINT ( 'NONE',  ( 172.4369982594507746, 275.8394585651928423, 17.18367144343603670 ) ) ;
#52874=CARTESIAN_POINT ( 'NONE',  ( 156.5693519948572430, 280.4191655658614764, -5.442758104603233171 ) ) ;
#52875=CARTESIAN_POINT ( 'NONE',  ( 196.6986986009438283, 272.8388821338493244, -13.37107033830584513 ) ) ;
#52877=CARTESIAN_POINT ( 'NONE',  ( 206.8429133553250949, 272.3845602134468322, 7.956126979824590606 ) ) ;
#52880=CARTESIAN_POINT ( 'NONE',  ( 170.9098063187821310, 283.9312053951169901, -11.13929243000735170 ) ) ;
#52882=B_SPLINE_CURVE_WITH_KNOTS ( 'NONE', 3,
 ( #8905, #77827, #30213, #14524, #22115, #8411 ),
 .UNSPECIFIED., .F., .F.,
 ( 4, 2, 4 ),
 ( 0.02030182656484812165, 0.02486100877575732337, 0.02942019098666652857 ),
 .UNSPECIFIED. ) ;
#52883=FACE_OUTER_BOUND ( 'NONE', #71005, .T. ) ;
#52884=CARTESIAN_POINT ( 'NONE',  ( 7.868168403658736487, 186.8967562850346837, -4.648177544792955347E-16 ) ) ;
#52885=CARTESIAN_POINT ( 'NONE',  ( 97.79278455872243114, 217.2677522451417644, -5.000000000000041744 ) ) ;
#52886=CARTESIAN_POINT ( 'NONE',  ( 208.3226489551340990, 269.8215829728092103, -1.240262689467544366 ) ) ;
#52888=CARTESIAN_POINT ( 'NONE',  ( 193.8652130780152731, 280.5836658925297229, -17.72338988841175933 ) ) ;
#52891=ORIENTED_EDGE ( 'NONE', *, *, #81421, .F. ) ;
#52892=CARTESIAN_POINT ( 'NONE',  ( 190.0707697440390689, 301.4347651000360884, 4.271360729158901748 ) ) ;
#52894=CARTESIAN_POINT ( 'NONE',  ( 189.3904159748659310, 297.2581566609080141, 8.144294695757311686 ) ) ;
#52896=ADVANCED_FACE ( 'NONE', ( #39347 ), #87554, .T. ) ;
#52897=CARTESIAN_POINT ( 'NONE',  ( 191.8232488616404225, 298.3993822291468518, -9.342381338555176384 ) ) ;
#52899=CARTESIAN_POINT ( 'NONE',  ( 164.2413944571582078, 246.1725554246774834, 7.304616466633322425 ) ) ;
#52900=AXIS2_PLACEMENT_3D ( 'NONE', #88387, #2240, #18941 ) ;
#52903=CARTESIAN_POINT ( 'NONE',  ( 90.37718171876834106, 232.1744531367911293, 4.594050593750047540 ) ) ;
#52904=CARTESIAN_POINT ( 'NONE',  ( 198.7305186980039480, 282.8878823269354825, 17.40725258201084813 ) ) ;
#52906=CARTESIAN_POINT ( 'NONE',  ( 180.9789598105594450, 270.9731600656857040, -15.98183179343307891 ) ) ;
#52909=EDGE_CURVE ( 'NONE', #36946, #68704, #44482, .T. ) ;
#52910=EDGE_CURVE ( 'NONE', #91334, #55290, #31205, .T. ) ;
#52911=ORIENTED_EDGE ( 'NONE', *, *, #87627, .T. ) ;
#52914=CARTESIAN_POINT ( 'NONE',  ( 148.3010860587701814, 276.5068540982774721, -3.904121881399305050 ) ) ;
#52917=CARTESIAN_POINT ( 'NONE',  ( 208.1415148974628266, 270.1353163636768500, 3.453641150550738725 ) ) ;
#52919=CYLINDRICAL_SURFACE ( 'NONE', #56246, 17.82106496071139645 ) ;
#52924=ORIENTED_EDGE ( 'NONE', *, *, #73643, .F. ) ;
#52927=CARTESIAN_POINT ( 'NONE',  ( 164.6189477058751720, 281.8792342857743165, 8.841444651024419343 ) ) ;
#52929=CARTESIAN_POINT ( 'NONE',  ( 19.41748551623073027, 172.0177522451417929, 5.000000000000051514 ) ) ;
#52930=ORIENTED_EDGE ( 'NONE', *, *, #39194, .F. ) ;
#52931=B_SPLINE_CURVE_WITH_KNOTS ( 'NONE', 3,
 ( #99886, #30469, #14276, #61362, #85213, #68465, #75590, #92319, #53270, #15758, #53751, #45168, #67474, #69467 ),
 .UNSPECIFIED., .F., .F.,
 ( 4, 2, 2, 2, 2, 2, 4 ),
 ( 0.0008179948676130699859, 0.001094431477128116623, 0.001370868086643163477, 0.001647304696158210114, 0.001923741305673259136, 0.002476614524703403802, 0.003029487743733548684 ),
 .UNSPECIFIED. ) ;
#52932=CARTESIAN_POINT ( 'NONE',  ( 186.4974067573569414, 258.2722711272355127, 3.096644213909161003 ) ) ;
#52933=CARTESIAN_POINT ( 'NONE',  ( 160.6901349803147809, 282.6678928203291434, -6.515548818033365386 ) ) ;
#52936=CARTESIAN_POINT ( 'NONE',  ( 170.9161164754127924, 255.3377101464579937, 11.24084812399238231 ) ) ;
#52937=CARTESIAN_POINT ( 'NONE',  ( 193.7393920959428613, 263.3242207741936340, -0.7651321868841867158 ) ) ;
#52939=CARTESIAN_POINT ( 'NONE',  ( 183.5431746618634747, 272.4062028040541463, -16.12888619052139205 ) ) ;
#52944=CARTESIAN_POINT ( 'NONE',  ( -2.160980794731627519, 182.8927522451419634, 2.944929066748280225E-16 ) ) ;
#52945=EDGE_CURVE ( 'NONE', #20189, #36064, #97625, .T. ) ;
#52946=CARTESIAN_POINT ( 'NONE',  ( 193.8848781386269309, 267.1185884883711879, -11.59377028749509364 ) ) ;
#52948=CARTESIAN_POINT ( 'NONE',  ( 171.4375308913269009, 279.6678964921788975, -14.69119404553828367 ) ) ;
#52949=CARTESIAN_POINT ( 'NONE',  ( 163.6998542325049755, 247.1105306081193760, -8.966021225103816050 ) ) ;
#52952=CARTESIAN_POINT ( 'NONE',  ( -12.32793173735119652, 169.8149278399160664, 9.188101187500093303 ) ) ;
#52953=CARTESIAN_POINT ( 'NONE',  ( 113.6157903772485298, 229.7365022471902023, -10.00000000000009237 ) ) ;
#52954=CARTESIAN_POINT ( 'NONE',  ( 58.82164138842261991, 214.7677522451419350, -5.000000000000047962 ) ) ;
#52955=ORIENTED_EDGE ( 'NONE', *, *, #92160, .T. ) ;
#52956=EDGE_CURVE ( 'NONE', #45286, #99390, #78422, .T. ) ;
#52957=ORIENTED_EDGE ( 'NONE', *, *, #3177, .T. ) ;
#52959=CYLINDRICAL_SURFACE ( 'NONE', #69041, 17.82106496071139645 ) ;
#52960=CARTESIAN_POINT ( 'NONE',  ( 171.7868853588355194, 289.4288941846863850, 2.650751707507049915 ) ) ;
#52962=CARTESIAN_POINT ( 'NONE',  ( 162.5139888333388001, 249.1645097304130445, -10.50570364880316987 ) ) ;
#52965=CARTESIAN_POINT ( 'NONE',  ( 16.08835327644320401, 192.3464784336661637, 1.353441290958777525E-15 ) ) ;
#52966=CARTESIAN_POINT ( 'NONE',  ( 126.7777458412893026, 237.8768266524160140, -9.188101187500091527 ) ) ;
#52967=CARTESIAN_POINT ( 'NONE',  ( 180.8060382252356817, 293.0948058857328533, -6.206326745275219103 ) ) ;
#52971=DIRECTION ( 'NONE',  ( 0.4999999999999998890, -0.8660254037844385966, 0.000000000000000000 ) ) ;
#52975=CARTESIAN_POINT ( 'NONE',  ( -22.42236680055709641, 157.8615022471902591, 0.000000000000000000 ) ) ;
#52977=CARTESIAN_POINT ( 'NONE',  ( 188.2922251827820332, 283.6369852287460276, 16.32093764900332644 ) ) ;
#52978=CARTESIAN_POINT ( 'NONE',  ( 165.0526092925929333, 249.7680750122055997, -10.69339827416780331 ) ) ;
#52979=CARTESIAN_POINT ( 'NONE',  ( 186.8617808892419987, 298.9052062963050389, -0.5998036538631226211 ) ) ;
#52981=CARTESIAN_POINT ( 'NONE',  ( 184.0948723531174096, 268.2408243536854116, -15.81992226484194752 ) ) ;
#52986=CARTESIAN_POINT ( 'NONE',  ( 89.59260651841245249, 222.5333772461660544, 9.188101187500095079 ) ) ;
#52990=CARTESIAN_POINT ( 'NONE',  ( 157.2744851780909414, 258.2395962677452985, 18.17792129701959070 ) ) ;
#52992=CARTESIAN_POINT ( 'NONE',  ( 202.9173117703535354, 271.9582023543367768, -9.750645975005012289 ) ) ;
#52994=CARTESIAN_POINT ( 'NONE',  ( 149.9292047088740674, 271.6423542473470434, -11.68677213707093010 ) ) ;
#52995=CARTESIAN_POINT ( 'NONE',  ( 130.3409059842875877, 239.3927522451417929, -10.00000000000009237 ) ) ;
#52996=CARTESIAN_POINT ( 'NONE',  ( 171.9845623806598667, 285.9329635774786880, -11.40154151993822040 ) ) ;
#52999=CIRCLE ( 'NONE', #99952, 5.000000000000116351 ) ;
#53001=CARTESIAN_POINT ( 'NONE',  ( 192.6789561813392595, 296.9172536750198219, -11.84591848451790952 ) ) ;
#53002=CARTESIAN_POINT ( 'NONE',  ( 149.4456112649506281, 271.7996036513546869, -12.95648166494593667 ) ) ;
#53005=CARTESIAN_POINT ( 'NONE',  ( 198.5966822647444587, 286.6674514332866579, 17.25284514431582750 ) ) ;
#53006=CARTESIAN_POINT ( 'NONE',  ( 180.5583831666531580, 263.2404611678256288, -12.85138873749756705 ) ) ;
#53007=CARTESIAN_POINT ( 'NONE',  ( 173.2310685956476561, 253.5757068955384455, -9.200971831753770758 ) ) ;
#53008=CARTESIAN_POINT ( 'NONE',  ( 192.0332533962074706, 298.0356437054567778, 11.70630383928353346 ) ) ;
#53013=CARTESIAN_POINT ( 'NONE',  ( 167.6676185881502477, 249.8298146214289943, 6.804182726411844406 ) ) ;
#53014=CARTESIAN_POINT ( 'NONE',  ( 185.2439515868709350, 292.7630553371902806, -10.53029436427169507 ) ) ;
#53017=CARTESIAN_POINT ( 'NONE',  ( 177.7634369230092091, 252.8608366103077856, -4.270187854574569275E-12 ) ) ;
#53018=CARTESIAN_POINT ( 'NONE',  ( -15.01183432020139286, 145.0260834800747602, 0.000000000000000000 ) ) ;
#53019=CARTESIAN_POINT ( 'NONE',  ( 190.5241654256948607, 278.7784361898847578, -16.51215372604780285 ) ) ;
#53020=CARTESIAN_POINT ( 'NONE',  ( 192.7090279274952991, 296.8651678828053946, -12.06870058016504288 ) ) ;
#53021=CARTESIAN_POINT ( 'NONE',  ( 188.0035612729766115, 279.2325960380115362, 17.82077010991123700 ) ) ;
#53023=CARTESIAN_POINT ( 'NONE',  ( 164.2981700896163773, 253.9203781951923133, 14.63367134977796802 ) ) ;
#53025=ADVANCED_FACE ( 'NONE', ( #26676 ), #18591, .T. ) ;
#53027=EDGE_CURVE ( 'NONE', #38097, #71334, #48093, .T. ) ;
#53029=EDGE_LOOP ( 'NONE', ( #18212, #50948, #83, #53543 ) ) ;
#53031=CARTESIAN_POINT ( 'NONE',  ( 169.3875294710099979, 269.0930465024870841, 17.17133023712824169 ) ) ;
#53032=CARTESIAN_POINT ( 'NONE',  ( 164.4990934228277411, 245.7262077230798809, 6.470820838822735510 ) ) ;
#53033=CARTESIAN_POINT ( 'NONE',  ( 165.5093369583051128, 275.0219039653110258, -16.16693748275729803 ) ) ;
#53035=CARTESIAN_POINT ( 'NONE',  ( 186.0715527847238207, 298.7753624933060337, 1.084710433360843940 ) ) ;
#53036=CARTESIAN_POINT ( 'NONE',  ( 202.6833006059332263, 277.5892208352050829, 15.45935665133711900 ) ) ;
#53037=CARTESIAN_POINT ( 'NONE',  ( 190.3049670482083684, 301.0291234702190764, 0.2225066852051815758 ) ) ;
#53039=CARTESIAN_POINT ( 'NONE',  ( 168.4778631746381734, 286.4770891300594258, -4.677790519826849902 ) ) ;
#53041=CARTESIAN_POINT ( 'NONE',  ( 186.6454664138524606, 287.0855943654420344, -15.99430129440811754 ) ) ;
#53042=CARTESIAN_POINT ( 'NONE',  ( 118.9835172072293403, 233.3768266524159856, -9.188101187500091527 ) ) ;
#53044=CARTESIAN_POINT ( 'NONE',  ( 148.4608825321785446, 275.1491132871843206, -7.142904470870874434 ) ) ;
#53045=B_SPLINE_CURVE_WITH_KNOTS ( 'NONE', 3,
 ( #89814, #66960, #12798, #43661, #59343, #13292, #14265, #36556, #37546, #74604, #90321, #51783, #76568, #44644, #7149, #45157, #44152, #99873, #75087, #76095, #98390, #75578, #59857, #21373, #6669, #52260, #29959, #83201, #68452, #6164, #13765, #37061, #67967, #98885, #99380, #60836, #91797, #22360, #53258, #70978, #47643, #92789, #562, #48157, #77576, #8164, #16255, #85722 ),
 .UNSPECIFIED., .F., .F.,
 ( 4, 2, 2, 2, 2, 2, 2, 2, 2, 2, 2, 2, 2, 2, 2, 2, 2, 2, 2, 2, 2, 2, 2, 4 ),
 ( 0.002037292597442118790, 0.002480311735260100434, 0.002701821304169148719, 0.002923330873078197004, 0.003034085657532719846, 0.003144840441987242254, 0.003255595226441765529, 0.003366350010896287936, 0.003587859579805333619, 0.003809369148714379302, 0.004695407424350640097, 0.005581445699986900023, 0.006467483975623159950, 0.006910503113441253918, 0.007353522251259347019, 0.007464277035713889376, 0.007519654427941122390, 0.007575031820168354538, 0.007685786604622705208, 0.007796541389077054143, 0.008239560526894465498, 0.008682579664711875117, 0.008904089233620637173, 0.009125598802529399228 ),
 .UNSPECIFIED. ) ;
#53047=CARTESIAN_POINT ( 'NONE',  ( 188.1090581172104805, 273.6250799618885026, 15.75090146302019889 ) ) ;
#53051=ORIENTED_EDGE ( 'NONE', *, *, #84417, .F. ) ;
#53055=CARTESIAN_POINT ( 'NONE',  ( 203.9648368022151601, 269.0477214045654364, 5.644613064108824574 ) ) ;
#53057=ORIENTED_EDGE ( 'NONE', *, *, #53148, .T. ) ;
#53058=CARTESIAN_POINT ( 'NONE',  ( 195.3331298895125201, 292.3200899603503444, 15.25153430865447390 ) ) ;
#53061=EDGE_CURVE ( 'NONE', #80515, #87229, #20302, .T. ) ;
#53063=VERTEX_POINT ( 'NONE', #14939 ) ;
#53066=CARTESIAN_POINT ( 'NONE',  ( 195.3876898667038517, 265.2072342455722946, 4.415210603996274408 ) ) ;
#53069=CARTESIAN_POINT ( 'NONE',  ( 151.3011447763744570, 269.1990464485573966, 14.21186556778774168 ) ) ;
#53070=CARTESIAN_POINT ( 'NONE',  ( 157.0463493773329162, 280.1323627575716273, 5.834371214722025911 ) ) ;
#53071=CARTESIAN_POINT ( 'NONE',  ( 152.9607371460978129, 265.7112270302071124, -16.17698032818104537 ) ) ;
#53072=ORIENTED_EDGE ( 'NONE', *, *, #7315, .F. ) ;
#53073=CARTESIAN_POINT ( 'NONE',  ( 190.1693911629507738, 301.2639477917662703, -5.112716700269980485 ) ) ;
#53074=B_SPLINE_SURFACE_WITH_KNOTS ( 'NONE', 3, 1, ( 
 ( #83855, #60488 ),
 ( #98033, #5327 ),
 ( #14421, #58988 ),
 ( #20037, #76237 ),
 ( #58505, #21523 ),
 ( #51924, #52406 ),
 ( #99030, #82864 ),
 ( #91447, #68603 ),
 ( #81860, #20535 ),
 ( #75731, #89478 ),
 ( #29616, #82376 ),
 ( #22008, #13917 ),
 ( #50910, #12437 ),
 ( #12946, #13437 ),
 ( #75232, #43806 ),
 ( #43304, #74252 ),
 ( #5814, #74747 ),
 ( #4838, #36204 ),
 ( #35718, #67609 ),
 ( #44795, #66617 ),
 ( #62479, #78219 ),
 ( #100026, #206 ),
 ( #7302, #46804 ),
 ( #15896, #92448 ),
 ( #8311, #91960 ),
 ( #86365, #70600 ),
 ( #69601, #77206 ),
 ( #78720, #61497 ),
 ( #14898, #8804 ),
 ( #93444, #55380 ),
 ( #39672, #69099 ),
 ( #53885, #85349 ),
 ( #30110, #7811 ),
 ( #1211, #70092 ) ),
 .UNSPECIFIED., .T., .F., .F.,
 ( 4, 2, 2, 2, 2, 2, 2, 2, 2, 2, 2, 2, 2, 2, 2, 2, 4 ),
 ( 2, 2 ),
 ( 0.000000000000000000, 0.06250000000000000000, 0.1250000000000000000, 0.1875000000000000000, 0.2500000000000000000, 0.3125000000000000000, 0.3750000000000000000, 0.4375000000000000000, 0.5000000000000000000, 0.5625000000000000000, 0.6250000000000000000, 0.6875000000000000000, 0.7500000000000000000, 0.8125000000000000000, 0.8750000000000000000, 0.9375000000000000000, 1.000000000000000000 ),
 ( 0.000000000000000000, 1.000000000000000000 ),
 .UNSPECIFIED. ) ;
#53076=CARTESIAN_POINT ( 'NONE',  ( 189.6282526764183842, 264.1678331799054149, -9.198679507049698501 ) ) ;
#53079=CARTESIAN_POINT ( 'NONE',  ( 189.4677816960851544, 269.1499146606108752, -14.21597690008461257 ) ) ;
#53083=CARTESIAN_POINT ( 'NONE',  ( 191.1909263933080751, 283.2087925905971701, -16.62349056250532797 ) ) ;
#53084=AXIS2_PLACEMENT_3D ( 'NONE', #25567, #17980, #81306 ) ;
#53086=CARTESIAN_POINT ( 'NONE',  ( 73.40858323730823543, 219.3149278399160664, 9.188101187500093303 ) ) ;
#53088=CARTESIAN_POINT ( 'NONE',  ( 146.9700173529739970, 276.0874580858064746, -5.099093031535578469 ) ) ;
#53089=CARTESIAN_POINT ( 'NONE',  ( 163.3409975114459485, 247.7320886816312111, -10.96358124877083640 ) ) ;
#53091=CARTESIAN_POINT ( 'NONE',  ( 207.4541616930702617, 271.3258470364304458, -6.834942797545373594 ) ) ;
#53092=DIRECTION ( 'NONE',  ( -0.4999999999999987788, 0.8660254037844392627, 0.000000000000000000 ) ) ;
#53097=B_SPLINE_CURVE_WITH_KNOTS ( 'NONE', 3,
 ( #16653, #39431, #94197, #93697 ),
 .UNSPECIFIED., .F., .F.,
 ( 4, 4 ),
 ( 0.006120916150806869280, 0.01419598930506990771 ),
 .UNSPECIFIED. ) ;
#53098=DIRECTION ( 'NONE',  ( -0.8660254037844387076, -0.4999999999999998890, -0.000000000000000000 ) ) ;
#53102=CARTESIAN_POINT ( 'NONE',  ( 31.65035466828360100, 179.8923013555409796, 4.594050593750050204 ) ) ;
#53103=EDGE_CURVE ( 'NONE', #18680, #78112, #75924, .T. ) ;
#53104=CARTESIAN_POINT ( 'NONE',  ( 55.46605327235566563, 193.6423013555410080, -4.594050593750043987 ) ) ;
#53105=CARTESIAN_POINT ( 'NONE',  ( 196.0395593785976018, 291.0965181932902510, 15.97855489120023087 ) ) ;
#53106=CARTESIAN_POINT ( 'NONE',  ( 199.6508179728032815, 277.6496187303415013, 15.20395581979866861 ) ) ;
#53109=CARTESIAN_POINT ( 'NONE',  ( 145.1264855360895751, 254.5958772461660544, -9.188101187500095079 ) ) ;
#53110=CARTESIAN_POINT ( 'NONE',  ( 48.83545950068980801, 192.8768266524159856, -9.188101187500093303 ) ) ;
#53112=CARTESIAN_POINT ( 'NONE',  ( 171.0170784859788000, 287.1471327868096637, 7.033863407631240960 ) ) ;
#53113=CARTESIAN_POINT ( 'NONE',  ( 149.5390997184345281, 271.6376768999995761, -11.52989534384373016 ) ) ;
#53115=CARTESIAN_POINT ( 'NONE',  ( 205.2121761402296443, 275.2090799237855094, -14.05269615702442465 ) ) ;
#53117=CARTESIAN_POINT ( 'NONE',  ( 175.4120841302475071, 291.3965204062699286, 1.943475587933318982 ) ) ;
#53119=FACE_OUTER_BOUND ( 'NONE', #85354, .T. ) ;
#53120=CARTESIAN_POINT ( 'NONE',  ( 182.3870610246802926, 280.6993384506884581, -16.15232590179551053 ) ) ;
#53121=CARTESIAN_POINT ( 'NONE',  ( 149.1618037898029172, 275.5005916956379792, 7.607269316218690847 ) ) ;
#53124=CARTESIAN_POINT ( 'NONE',  ( 99.25420243115655694, 228.1115022471902307, 10.00000000000009592 ) ) ;
#53125=( BOUNDED_CURVE ( )  B_SPLINE_CURVE ( 2, ( #43969, #42962, #13596, #74907, #90643, #67280, #26797, #73904, #88659 ),
 .UNSPECIFIED., .F., .T. ) 
 B_SPLINE_CURVE_WITH_KNOTS ( ( 3, 2, 2, 2, 3 ),
 ( 0.8185483870967742437, 0.8198924731182796188, 0.8225806451612903691, 0.8252688172043011194, 0.8266129032258064946 ),
 .UNSPECIFIED. ) 
 CURVE ( )  GEOMETRIC_REPRESENTATION_ITEM ( )  RATIONAL_B_SPLINE_CURVE ( ( 0.9330127018922194093, 0.9330127018922194093, 1.000000000000000000, 0.8660254037844387076, 1.000000000000000000, 0.8660254037844387076, 1.000000000000000000, 0.9330127018922194093, 0.9330127018922194093 ) ) 
 REPRESENTATION_ITEM ( '' )  );
#53126=CARTESIAN_POINT ( 'NONE',  ( 200.3765029811139584, 283.5847115241710981, 16.85207472104531590 ) ) ;
#53127=CARTESIAN_POINT ( 'NONE',  ( 168.5165758536381873, 288.6662250410414003, -0.7359078604044604344 ) ) ;
#53129=CARTESIAN_POINT ( 'NONE',  ( 61.98804677278346986, 206.5958772461660828, -9.188101187500095079 ) ) ;
#53130=ORIENTED_EDGE ( 'NONE', *, *, #44772, .F. ) ;
#53131=FACE_OUTER_BOUND ( 'NONE', #40174, .T. ) ;
#53132=CARTESIAN_POINT ( 'NONE',  ( 190.2648877593310317, 301.0985428348857340, -4.426259207433023590 ) ) ;
#53133=CARTESIAN_POINT ( 'NONE',  ( 183.8043731368310603, 268.5938253857621589, 16.29461355553033997 ) ) ;
#53134=ORIENTED_EDGE ( 'NONE', *, *, #98609, .T. ) ;
#53137=CARTESIAN_POINT ( 'NONE',  ( 194.8432095198904221, 293.1686569321988145, -14.74101036184996616 ) ) ;
#53138=CARTESIAN_POINT ( 'NONE',  ( 177.2942696745171247, 274.8600937621219487, -17.06932773013303262 ) ) ;
#53140=CARTESIAN_POINT ( 'NONE',  ( 156.7173554537088194, 259.2045732567815435, 17.96992492779905959 ) ) ;
#53145=CARTESIAN_POINT ( 'NONE',  ( 172.3136996429396675, 274.9537642369339778, 17.36053840881438859 ) ) ;
#53148=EDGE_CURVE ( 'NONE', #73330, #48184, #34787, .T. ) ;
#53149=CARTESIAN_POINT ( 'NONE',  ( 206.1062572280473546, 273.6604860535989587, -9.773577984388410300 ) ) ;
#53150=EDGE_CURVE ( 'NONE', #57780, #19194, #50590, .T. ) ;
#53154=CARTESIAN_POINT ( 'NONE',  ( 163.1747956065615028, 283.6804097174056665, -3.098853972138146506 ) ) ;
#53156=CARTESIAN_POINT ( 'NONE',  ( 163.2256942281324541, 247.9317998266098471, -9.780520296312531059 ) ) ;
#53159=CARTESIAN_POINT ( 'NONE',  ( 198.4264492142971221, 286.9623037257889564, 17.00126466006521397 ) ) ;
#53160=CARTESIAN_POINT ( 'NONE',  ( 161.6806056053058853, 263.3655989262382491, -17.06081503136075028 ) ) ;
#53161=ADVANCED_FACE ( 'NONE', ( #86916 ), #35193, .F. ) ;
#53162=CARTESIAN_POINT ( 'NONE',  ( 128.5637496887121927, 245.0333772461660544, 9.188101187500095079 ) ) ;
#53163=CARTESIAN_POINT ( 'NONE',  ( 177.1315819580615027, 269.3555979632168942, 16.09210694347321180 ) ) ;
#53164=CARTESIAN_POINT ( 'NONE',  ( 195.3624787578944222, 290.3824063481519602, -16.76522224015156226 ) ) ;
#53165=B_SPLINE_CURVE_WITH_KNOTS ( 'NONE', 3,
 ( #36413, #6022, #45995, #44003 ),
 .UNSPECIFIED., .F., .F.,
 ( 4, 4 ),
 ( 0.04550866176299273036, 0.04887066958154935581 ),
 .UNSPECIFIED. ) ;
#53166=CARTESIAN_POINT ( 'NONE',  ( 62.52896555438372417, 219.1589784336661637, -6.496448406907675876E-16 ) ) ;
#53167=ORIENTED_EDGE ( 'NONE', *, *, #30478, .T. ) ;
#53168=CARTESIAN_POINT ( 'NONE',  ( 173.2130610185342334, 264.9127892606105661, 17.04138321073628148 ) ) ;
#53174=ORIENTED_EDGE ( 'NONE', *, *, #34910, .F. ) ;
#53177=CARTESIAN_POINT ( 'NONE',  ( 197.8265573649375142, 286.7779075425210635, 16.93047688356437419 ) ) ;
#53178=CARTESIAN_POINT ( 'NONE',  ( 191.2111338740054975, 299.4595964878050154, -9.718193530796334301 ) ) ;
#53180=CARTESIAN_POINT ( 'NONE',  ( 155.4186054393023255, 261.4540742680644598, 17.05753227160644769 ) ) ;
#53185=ORIENTED_EDGE ( 'NONE', *, *, #35547, .F. ) ;
#53189=AXIS2_PLACEMENT_3D ( 'NONE', #3962, #35855, #82517 ) ;
#53190=CARTESIAN_POINT ( 'NONE',  ( 206.3106310032756596, 273.3065002911688453, 10.17860425536756175 ) ) ;
#53191=CARTESIAN_POINT ( 'NONE',  ( 199.0159380930694226, 281.1150505206304615, 17.25796289221863233 ) ) ;
#53192=CARTESIAN_POINT ( 'NONE',  ( 162.7773628798197194, 261.4912393770340486, 17.07172388677674491 ) ) ;
#53193=CARTESIAN_POINT ( 'NONE',  ( 137.8192226437758450, 256.5024278399160949, -9.188101187500093303 ) ) ;
#53196=CARTESIAN_POINT ( 'NONE',  ( 182.1659242776092924, 257.5230415930786876, 6.683065253742526579 ) ) ;
#53198=CARTESIAN_POINT ( 'NONE',  ( 201.2949053258274148, 281.9939920013367782, -18.04004790210578335 ) ) ;
#53200=CARTESIAN_POINT ( 'NONE',  ( 178.8595466249924755, 265.0989930076032124, -16.03772641351113748 ) ) ;
#53201=ORIENTED_EDGE ( 'NONE', *, *, #86734, .T. ) ;
#53202=CARTESIAN_POINT ( 'NONE',  ( 196.0966283236085417, 264.7156248001706444, 5.418721370419348204 ) ) ;
#53204=CARTESIAN_POINT ( 'NONE',  ( 181.8578577305817419, 291.4847624314589325, 9.597431263652177691 ) ) ;
#53205=B_SPLINE_CURVE_WITH_KNOTS ( 'NONE', 3,
 ( #18734, #64834, #27820, #81075 ),
 .UNSPECIFIED., .F., .F.,
 ( 4, 4 ),
 ( 7.943821393640659065E-17, 0.006184891004078511487 ),
 .UNSPECIFIED. ) ;
#53208=CARTESIAN_POINT ( 'NONE',  ( 198.6294664808700077, 266.3094093603824604, 0.8324587486580483642 ) ) ;
#53209=CARTESIAN_POINT ( 'NONE',  ( 195.5055827311261964, 264.2059424127278930, 0.8350436053642301681 ) ) ;
#53211=CARTESIAN_POINT ( 'NONE',  ( 146.7845206192450007, 276.4087478532630939, 4.443586170796542945 ) ) ;
#53212=CARTESIAN_POINT ( 'NONE',  ( 186.7843925653488668, 282.2516066892422941, 17.48446008842761401 ) ) ;
#53213=EDGE_CURVE ( 'NONE', #39058, #54972, #25105, .T. ) ;
#53216=CARTESIAN_POINT ( 'NONE',  ( 177.2746010927298812, 264.5551300243030255, -15.37364360889636750 ) ) ;
#53217=CARTESIAN_POINT ( 'NONE',  ( 196.4589140796189213, 270.4767738285896712, 11.79566246125468254 ) ) ;
#53220=DIRECTION ( 'NONE',  ( 0.4999999999999998890, -0.8660254037844385966, 0.000000000000000000 ) ) ;
#53222=CARTESIAN_POINT ( 'NONE',  ( 198.5612432604688991, 286.7288335892616260, 18.30793681285053509 ) ) ;
#53223=CARTESIAN_POINT ( 'NONE',  ( 147.1562325744354496, 245.7677522451417929, -5.000000000000041744 ) ) ;
#53225=VERTEX_POINT ( 'NONE', #26064 ) ;
#53228=CARTESIAN_POINT ( 'NONE',  ( 151.2567985338353935, 268.6625352796243646, -15.71756535662528798 ) ) ;
#53229=CARTESIAN_POINT ( 'NONE',  ( 8.456677953475336906, 181.8149278399161233, 9.188101187500093303 ) ) ;
#53230=CARTESIAN_POINT ( 'NONE',  ( 181.5169748047240716, 275.4304238179468598, -16.43353661735662286 ) ) ;
#53233=CARTESIAN_POINT ( 'NONE',  ( 170.3568046055088701, 270.8355684487424924, -16.86163208226229315 ) ) ;
#53235=CARTESIAN_POINT ( 'NONE',  ( 130.9362984529373080, 239.7365022471902307, 10.00000000000009948 ) ) ;
#53236=CARTESIAN_POINT ( 'NONE',  ( 175.5389217430812607, 253.4453625803252521, -3.600109118078927306 ) ) ;
#53237=CARTESIAN_POINT ( 'NONE',  ( 187.4956075105807827, 259.3323774093973952, -0.7818960507064889320 ) ) ;
#53238=CARTESIAN_POINT ( 'NONE',  ( 61.50992858288481813, 192.9865022471901739, 1.119607411625061291E-15 ) ) ;
#53239=DIRECTION ( 'NONE',  ( 0.4999999999999992784, -0.8660254037844390407, 0.000000000000000000 ) ) ;
#53240=CARTESIAN_POINT ( 'NONE',  ( 148.3707431749605234, 273.6613297946520902, 8.912574527564540716 ) ) ;
#53242=CARTESIAN_POINT ( 'NONE',  ( 25.45277359850996390, 179.3768266524160140, -9.188101187500091527 ) ) ;
#53246=CARTESIAN_POINT ( 'NONE',  ( 202.0995849165119012, 279.2814632178312308, -15.97000401044184414 ) ) ;
#53247=CARTESIAN_POINT ( 'NONE',  ( 207.2824254892180704, 271.6233028670009162, 6.274396967990798046 ) ) ;
#53248=CARTESIAN_POINT ( 'NONE',  ( 185.4224844400474126, 266.5931547338063865, 13.20453509119197832 ) ) ;
#53249=CARTESIAN_POINT ( 'NONE',  ( 162.5249628567144384, 281.0953062916516956, -10.43707322529907877 ) ) ;
#53250=CARTESIAN_POINT ( 'NONE',  ( 160.3162220307800112, 280.5258973909593010, 9.471671026417038064 ) ) ;
#53253=CARTESIAN_POINT ( 'NONE',  ( 190.4281805785508084, 300.8157113754859893, -1.233909217199055774 ) ) ;
#53255=CARTESIAN_POINT ( 'NONE',  ( 193.9966098916996771, 294.6350105018939871, 13.97117019253516013 ) ) ;
#53258=CARTESIAN_POINT ( 'NONE',  ( 185.5142048876550689, 290.8592545809869421, 12.38599642959644243 ) ) ;
#53259=CARTESIAN_POINT ( 'NONE',  ( 162.7879170537843834, 283.1953112578214018, -7.983003719734843351 ) ) ;
#53265=CARTESIAN_POINT ( 'NONE',  ( 203.5477091018662748, 278.0920214017542662, -16.09930363698006062 ) ) ;
#53270=CARTESIAN_POINT ( 'NONE',  ( 202.1973601604639157, 279.9586468202055016, 15.74103291435646668 ) ) ;
#53271=CARTESIAN_POINT ( 'NONE',  ( 150.8581383233440931, 273.8175834856673418, 11.30189666945060623 ) ) ;
#53272=EDGE_LOOP ( 'NONE', ( #55059, #62471, #96433, #3602 ) ) ;
#53273=CARTESIAN_POINT ( 'NONE',  ( 201.4463813434794019, 281.7316278426353620, -17.16864527463587820 ) ) ;
#53278=CARTESIAN_POINT ( 'NONE',  ( 190.3049670482083684, 301.0291234702190764, 0.2225066852051815758 ) ) ;
#53282=CARTESIAN_POINT ( 'NONE',  ( 206.5508451493652444, 272.8904371854448527, 11.05407534521577695 ) ) ;
#53285=CARTESIAN_POINT ( 'NONE',  ( 149.7119746935222793, 271.3382486597900538, 12.05352563709836922 ) ) ;
#53287=VERTEX_POINT ( 'NONE', #10366 ) ;
#53292=ORIENTED_EDGE ( 'NONE', *, *, #45383, .F. ) ;
#53295=CARTESIAN_POINT ( 'NONE',  ( 146.7879906441258129, 276.4027375938661635, 4.347255311287614887 ) ) ;
#53297=CARTESIAN_POINT ( 'NONE',  ( 149.4491471355718772, 271.7934793437897270, 11.43912701239353780 ) ) ;
#53299=CARTESIAN_POINT ( 'NONE',  ( 146.7933720846101551, 276.3934166655288891, -0.7715638482002741272 ) ) ;
#53300=CARTESIAN_POINT ( 'NONE',  ( 147.0721334091522294, 275.9105878882373304, 0.7242168585908188572 ) ) ;
#53301=CARTESIAN_POINT ( 'NONE',  ( 190.0226014859668453, 301.5181949703289774, 3.835066345245774500 ) ) ;
#53304=CARTESIAN_POINT ( 'NONE',  ( 167.5734009011913201, 287.5402412053340981, 3.813278936258391205 ) ) ;
#53306=VERTEX_POINT ( 'NONE', #81788 ) ;
#53307=CARTESIAN_POINT ( 'NONE',  ( 149.4340984048157850, 271.8195445100486154, -13.08951326935260617 ) ) ;
#53309=CARTESIAN_POINT ( 'NONE',  ( 202.8576051359847838, 278.8876414770759311, 15.11413215307486091 ) ) ;
#53311=CARTESIAN_POINT ( 'NONE',  ( 179.8080204723898987, 283.1032712615998435, -15.92647367223843524 ) ) ;
#53312=CARTESIAN_POINT ( 'NONE',  ( 147.9905646369332999, 274.3198183384625395, -9.173503928458199397 ) ) ;
#53313=CARTESIAN_POINT ( 'NONE',  ( 168.8622422750650287, 285.9893830644730883, -7.604670509767990083 ) ) ;
#53315=CARTESIAN_POINT ( 'NONE',  ( 208.2912792141756029, 269.8759169579697641, -2.198672330625011995 ) ) ;
#53318=CARTESIAN_POINT ( 'NONE',  ( 40.63510790894940072, 204.2677522451419350, -5.000000000000047962 ) ) ;
#53319=CARTESIAN_POINT ( 'NONE',  ( 113.9495709998497688, 236.5958772461660544, -9.188101187500095079 ) ) ;
#53320=CARTESIAN_POINT ( 'NONE',  ( 180.7653681401676238, 294.1091613165833110, -3.018679760699134906 ) ) ;
#53324=CARTESIAN_POINT ( 'NONE',  ( 173.1062955787805322, 251.8696176234196855, -3.934703316205188983 ) ) ;
#53325=CARTESIAN_POINT ( 'NONE',  ( 31.35205101814392847, 201.1589784336661353, -6.496448406907675876E-16 ) ) ;
#53326=EDGE_CURVE ( 'NONE', #86358, #82234, #84364, .T. ) ;
#53327=CARTESIAN_POINT ( 'NONE',  ( 162.5148320529283126, 285.2034568178174254, 0.5437328601018158736 ) ) ;
#53329=VERTEX_POINT ( 'NONE', #58435 ) ;
#53330=CARTESIAN_POINT ( 'NONE',  ( 1.158783253108745637, 178.1427522451419350, 10.00000000000009415 ) ) ;
#53331=CARTESIAN_POINT ( 'NONE',  ( 178.1940240703611380, 265.8106693507822342, 15.39809615566641554 ) ) ;
#53333=B_SPLINE_CURVE_WITH_KNOTS ( 'NONE', 3,
 ( #26760, #27761, #43443, #66744 ),
 .UNSPECIFIED., .F., .F.,
 ( 4, 4 ),
 ( 1.588764278728131813E-16, 0.007655728206563773564 ),
 .UNSPECIFIED. ) ;
#53334=CARTESIAN_POINT ( 'NONE',  ( 190.8683709797118411, 300.0532792356709706, -4.461919767133968762 ) ) ;
#53338=AXIS2_PLACEMENT_3D ( 'NONE', #30427, #93773, #84666 ) ;
#53340=CARTESIAN_POINT ( 'NONE',  ( 102.4837554958880901, 236.6427522451419350, 10.00000000000009237 ) ) ;
#53341=B_SPLINE_SURFACE_WITH_KNOTS ( 'NONE', 3, 1, ( 
 ( #33069, #88836 ),
 ( #19400, #18381 ),
 ( #64977, #86833 ),
 ( #34563, #87357 ),
 ( #41656, #87842 ),
 ( #72087, #42156 ),
 ( #49767, #25987 ),
 ( #80213, #79716 ),
 ( #17886, #57356 ),
 ( #10781, #94906 ),
 ( #50259, #64474 ),
 ( #73574, #25468 ),
 ( #40653, #73091 ),
 ( #96405, #95920 ),
 ( #3203, #27481 ),
 ( #88332, #26974 ),
 ( #48785, #57856 ),
 ( #10279, #81212 ),
 ( #2688, #72599 ),
 ( #63963, #80723 ),
 ( #11297, #48273 ),
 ( #79219, #11786 ),
 ( #4157, #35052 ),
 ( #65960, #21849 ),
 ( #14254, #44630 ),
 ( #59843, #12275 ),
 ( #20373, #12782 ),
 ( #37533, #60327 ),
 ( #43647, #98873 ),
 ( #44138, #59327 ),
 ( #90307, #29451 ),
 ( #35558, #91283 ),
 ( #36541, #74077 ),
 ( #68438, #99366 ) ),
 .UNSPECIFIED., .T., .F., .F.,
 ( 4, 2, 2, 2, 2, 2, 2, 2, 2, 2, 2, 2, 2, 2, 2, 2, 4 ),
 ( 2, 2 ),
 ( 0.000000000000000000, 0.06250000000000000000, 0.1250000000000000000, 0.1875000000000000000, 0.2500000000000000000, 0.3125000000000000000, 0.3750000000000000000, 0.4375000000000000000, 0.5000000000000000000, 0.5625000000000000000, 0.6250000000000000000, 0.6875000000000000000, 0.7500000000000000000, 0.8125000000000000000, 0.8750000000000000000, 0.9375000000000000000, 1.000000000000000000 ),
 ( 0.000000000000000000, 1.000000000000000000 ),
 .UNSPECIFIED. ) ;
#53343=ORIENTED_EDGE ( 'NONE', *, *, #77658, .F. ) ;
#53345=CARTESIAN_POINT ( 'NONE',  ( 202.8211298556536804, 279.3504935719197988, 17.07914446815911447 ) ) ;
#53346=CARTESIAN_POINT ( 'NONE',  ( 153.9000638729780519, 264.8647237507889258, 16.61098735674968907 ) ) ;
#53348=CARTESIAN_POINT ( 'NONE',  ( 17.98330449086917682, 175.0643266524160140, -9.188101187500093303 ) ) ;
#53350=CARTESIAN_POINT ( 'NONE',  ( 193.5726236920921792, 272.6483137682516258, 14.24630395148186146 ) ) ;
#53353=CARTESIAN_POINT ( 'NONE',  ( 195.2398765441725743, 275.4993714954396182, -15.53986780429037928 ) ) ;
#53354=CARTESIAN_POINT ( 'NONE',  ( 57.65757265809627086, 216.3464784336661353, 1.353441290958777327E-15 ) ) ;
#53355=CARTESIAN_POINT ( 'NONE',  ( 164.4915767550571957, 245.7392269735623529, -6.407198159945809657 ) ) ;
#53359=CARTESIAN_POINT ( 'NONE',  ( 207.6209998424140792, 271.0368748851258260, 6.610167240481342965 ) ) ;
#53361=CARTESIAN_POINT ( 'NONE',  ( 3.558395312976033065, 182.8615022471903444, 5.000000000000046185 ) ) ;
#53362=CARTESIAN_POINT ( 'NONE',  ( 163.7423057141168385, 247.0370024851108610, -6.909410042141566066 ) ) ;
#53363=CARTESIAN_POINT ( 'NONE',  ( 132.4608640057421667, 247.2833772461660544, -9.188101187500095079 ) ) ;
#53365=CARTESIAN_POINT ( 'NONE',  ( 164.8280002253160319, 260.9906286863443370, -16.15074254659257846 ) ) ;
#53367=CARTESIAN_POINT ( 'NONE',  ( 177.3945811460199309, 252.6478776281709315, -0.09019740402004521040 ) ) ;
#53368=CARTESIAN_POINT ( 'NONE',  ( 206.9349434189263661, 269.8064106017384916, 1.784245431258210113 ) ) ;
#53372=CARTESIAN_POINT ( 'NONE',  ( 152.7730629122270898, 271.2363297891400293, 14.33490734661111610 ) ) ;
#53373=CARTESIAN_POINT ( 'NONE',  ( 151.7688189367730445, 268.5115722919948098, -14.80711862932078482 ) ) ;
#53374=CARTESIAN_POINT ( 'NONE',  ( 196.5882727079285530, 289.1336862968285004, 16.81565452615681977 ) ) ;
#53375=CARTESIAN_POINT ( 'NONE',  ( 197.3142096324615693, 273.2062379081899053, -13.39448277848560309 ) ) ;
#53376=ORIENTED_EDGE ( 'NONE', *, *, #64237, .T. ) ;
#53378=DIRECTION ( 'NONE',  ( 0.5000000000000003331, -0.8660254037844384856, 0.000000000000000000 ) ) ;
#53380=EDGE_CURVE ( 'NONE', #7185, #71334, #35141, .T. ) ;
#53382=CARTESIAN_POINT ( 'NONE',  ( 196.2549875969139066, 270.8803193507863512, 12.05863901870844046 ) ) ;
#53389=CARTESIAN_POINT ( 'NONE',  ( 190.4163244163388242, 300.8362468508201459, 4.691083071570470331 ) ) ;
#53395=ADVANCED_FACE ( 'NONE', ( #35645 ), #18469, .T. ) ;
#53397=CARTESIAN_POINT ( 'NONE',  ( 149.4171629335945681, 271.8488776066536730, -11.42564036194071520 ) ) ;
#53401=CARTESIAN_POINT ( 'NONE',  ( 98.84807947347611901, 234.0024278399160949, -9.188101187500093303 ) ) ;
#53402=CARTESIAN_POINT ( 'NONE',  ( 200.1662314894802819, 283.9489124310637180, 17.19420058542677054 ) ) ;
#53403=CARTESIAN_POINT ( 'NONE',  ( 181.1247500054012392, 271.0610771650950142, -15.98018870080622200 ) ) ;
#53405=ORIENTED_EDGE ( 'NONE', *, *, #85928, .T. ) ;
#53406=ORIENTED_EDGE ( 'NONE', *, *, #58942, .F. ) ;
#53411=AXIS2_PLACEMENT_3D ( 'NONE', #81293, #87437, #17970 ) ;
#53413=CARTESIAN_POINT ( 'NONE',  ( 207.8302079587528794, 270.6745157982714431, 3.572475529330238153 ) ) ;
#53418=CARTESIAN_POINT ( 'NONE',  ( 204.8008807586744524, 272.7600038595665524, -10.89009281376315741 ) ) ;
#53420=CARTESIAN_POINT ( 'NONE',  ( 198.3788960466430069, 277.4004215258680688, -15.34290956586492349 ) ) ;
#53421=CARTESIAN_POINT ( 'NONE',  ( 189.7493380202622291, 294.8126471784881915, -12.68491631734921299 ) ) ;
#53422=DIRECTION ( 'NONE',  ( 0.4999999999999992784, -0.8660254037844390407, 0.000000000000000000 ) ) ;
#53424=CARTESIAN_POINT ( 'NONE',  ( 162.6937333994314656, 248.8531830095558632, 10.02305144031113926 ) ) ;
#53425=CARTESIAN_POINT ( 'NONE',  ( 188.2838305778037409, 260.6970239875658990, 2.538272036997531789 ) ) ;
#53427=( BOUNDED_CURVE ( )  B_SPLINE_CURVE ( 2, ( #53511, #36822, #22124, #5439, #75853, #98150, #51531, #67732, #83970 ),
 .UNSPECIFIED., .F., .T. ) 
 B_SPLINE_CURVE_WITH_KNOTS ( ( 3, 2, 2, 2, 3 ),
 ( 0.3588709677419354982, 0.3602150537634408733, 0.3629032258064516236, 0.3655913978494623739, 0.3669354838709677491 ),
 .UNSPECIFIED. ) 
 CURVE ( )  GEOMETRIC_REPRESENTATION_ITEM ( )  RATIONAL_B_SPLINE_CURVE ( ( 0.9330127018922194093, 0.9330127018922194093, 1.000000000000000000, 0.8660254037844387076, 1.000000000000000000, 0.8660254037844387076, 1.000000000000000000, 0.9330127018922194093, 0.9330127018922194093 ) ) 
 REPRESENTATION_ITEM ( '' )  );
#53429=CARTESIAN_POINT ( 'NONE',  ( 176.3101768776420215, 291.3056225515143183, 7.435599247236559961 ) ) ;
#53430=CARTESIAN_POINT ( 'NONE',  ( 161.3138715957851161, 283.5633977043666505, 2.146130691252540856 ) ) ;
#53431=ORIENTED_EDGE ( 'NONE', *, *, #96431, .T. ) ;
#53432=CARTESIAN_POINT ( 'NONE',  ( 93.60468337831815688, 236.3967562850347122, -4.648177544792955347E-16 ) ) ;
#53434=CARTESIAN_POINT ( 'NONE',  ( 8.231324050681719129, 168.8927522451418213, -10.00000000000009059 ) ) ;
#53435=CARTESIAN_POINT ( 'NONE',  ( 196.1497905407457836, 269.5260199243853663, -10.84959131364318630 ) ) ;
#53436=CARTESIAN_POINT ( 'NONE',  ( 172.8824701414635285, 280.2431502589070078, -14.30495993044576331 ) ) ;
#53440=CARTESIAN_POINT ( 'NONE',  ( -10.59588092978231266, 170.8149278399160949, -9.188101187500095079 ) ) ;
#53442=EDGE_CURVE ( 'NONE', #88529, #45286, #6988, .T. ) ;
#53443=CARTESIAN_POINT ( 'NONE',  ( 189.0628780359570840, 297.0621672202208856, 8.938274956999553211 ) ) ;
#53446=CARTESIAN_POINT ( 'NONE',  ( 202.5128468779458331, 267.1751508879428343, 0.8823122286173835649 ) ) ;
#53447=EDGE_CURVE ( 'NONE', #56117, #37792, #77142, .T. ) ;
#53448=B_SPLINE_CURVE_WITH_KNOTS ( 'NONE', 3,
 ( #28596, #36687, #98526, #29603 ),
 .UNSPECIFIED., .F., .F.,
 ( 4, 4 ),
 ( 0.01664341470350885061, 0.02552166612420159880 ),
 .UNSPECIFIED. ) ;
#53449=CARTESIAN_POINT ( 'NONE',  ( -22.42236680055709641, 157.8615022471902591, 0.000000000000000000 ) ) ;
#53451=CARTESIAN_POINT ( 'NONE',  ( 163.0339123139343656, 248.2639758459733343, -11.68896797671248322 ) ) ;
#53454=CARTESIAN_POINT ( 'NONE',  ( 29.05227845693028854, 178.3923013555409796, 4.594050593750050204 ) ) ;
#53455=CARTESIAN_POINT ( 'NONE',  ( 113.0020953926368037, 245.2369531367911009, -4.594050593750048428 ) ) ;
#53460=CYLINDRICAL_SURFACE ( 'NONE', #17783, 17.82106496071139645 ) ;
#53462=CARTESIAN_POINT ( 'NONE',  ( 157.1135969804030310, 258.5182628004787944, 17.19660297500358226 ) ) ;
#53464=CARTESIAN_POINT ( 'NONE',  ( 207.3646600298985447, 271.4808684644054324, -5.284084612275558257 ) ) ;
#53465=CARTESIAN_POINT ( 'NONE',  ( 189.9640924866416185, 284.8439010332405701, 17.27955391728670165 ) ) ;
#53467=CARTESIAN_POINT ( 'NONE',  ( 165.0466594235693094, 249.7004948130006881, -10.73553599785811485 ) ) ;
#53471=PLANE ( 'NONE',  #15605 ) ;
#53473=EDGE_LOOP ( 'NONE', ( #48214, #72768 ) ) ;
#53475=CIRCLE ( 'NONE', #43786, 2.471954595299370006 ) ;
#53476=CARTESIAN_POINT ( 'NONE',  ( 207.5408646414791178, 271.1756731246201753, 3.050859480894625886 ) ) ;
#53478=CARTESIAN_POINT ( 'NONE',  ( 105.4518702730974979, 225.5643266524160140, 9.188101187500095079 ) ) ;
#53482=CARTESIAN_POINT ( 'NONE',  ( 157.3025066944120454, 258.1910615777721887, 18.21299529665260053 ) ) ;
#53483=CARTESIAN_POINT ( 'NONE',  ( 111.2883471010299274, 228.3927522451418213, 10.00000000000009948 ) ) ;
#53485=CARTESIAN_POINT ( 'NONE',  ( 182.8075329105516289, 285.5996758505444291, -15.91971760981349071 ) ) ;
#53486=CARTESIAN_POINT ( 'NONE',  ( 196.5114383562724072, 290.2791998289336561, -17.87308875047256862 ) ) ;
#53493=CARTESIAN_POINT ( 'NONE',  ( 200.3191154286411972, 269.5421802034505276, 8.895171844116440241 ) ) ;
#53494=CARTESIAN_POINT ( 'NONE',  ( 196.7491951525289835, 289.8673929779723721, -16.35352603081977207 ) ) ;
#53498=CARTESIAN_POINT ( 'NONE',  ( 198.3449891235413531, 287.1033967417670283, 16.95540786497457120 ) ) ;
#53499=CARTESIAN_POINT ( 'NONE',  ( 180.2627280979794193, 263.0731415412748788, -12.84391273256747112 ) ) ;
#53501=CARTESIAN_POINT ( 'NONE',  ( 150.7827139563306957, 247.8615022471901739, 5.000000000000051514 ) ) ;
#53503=B_SPLINE_CURVE_WITH_KNOTS ( 'NONE', 3,
 ( #21070, #89982, #59013, #68128 ),
 .UNSPECIFIED., .F., .F.,
 ( 4, 4 ),
 ( 2.189838513871484750E-15, 0.002576580807713663504 ),
 .UNSPECIFIED. ) ;
#53509=CARTESIAN_POINT ( 'NONE',  ( 181.4256177755142403, 290.8855465862295659, -11.11246407318897234 ) ) ;
#53511=CARTESIAN_POINT ( 'NONE',  ( 39.04508293989853485, 204.8967562850347122, -4.648177544792955347E-16 ) ) ;
#53513=CARTESIAN_POINT ( 'NONE',  ( 158.8709510117273567, 255.4744363313390920, 17.58515796180118329 ) ) ;
#53516=CARTESIAN_POINT ( 'NONE',  ( 153.2283961777204695, 265.2476279883323400, -17.66880461074566000 ) ) ;
#53520=EDGE_CURVE ( 'NONE', #4197, #96323, #37311, .T. ) ;
#53522=EDGE_LOOP ( 'NONE', ( #72881, #65000, #58005, #33552, #93596 ) ) ;
#53523=CYLINDRICAL_SURFACE ( 'NONE', #57816, 17.82106496071139645 ) ;
#53525=VERTEX_POINT ( 'NONE', #30535 ) ;
#53527=CARTESIAN_POINT ( 'NONE',  ( 170.4004368708347670, 269.6954681395467333, 17.78991379675761664 ) ) ;
#53528=CARTESIAN_POINT ( 'NONE',  ( 164.4761815919938215, 245.7658921781788592, 6.833796894895563412 ) ) ;
#53531=CARTESIAN_POINT ( 'NONE',  ( 197.8594538715673536, 272.3702523096476398, -13.40354871589081398 ) ) ;
#53533=CARTESIAN_POINT ( 'NONE',  ( 146.9978162861947908, 276.0393089210717790, -5.134868500856280882 ) ) ;
#53534=CARTESIAN_POINT ( 'NONE',  ( 183.6422324172568210, 264.5785696717482551, 14.31652553825990104 ) ) ;
#53535=CARTESIAN_POINT ( 'NONE',  ( 165.8099488291475154, 266.0266196162687038, 17.45967265355124809 ) ) ;
#53536=CARTESIAN_POINT ( 'NONE',  ( 183.4288137002880319, 284.5585098770374088, -15.07552829229580915 ) ) ;
#53537=CARTESIAN_POINT ( 'NONE',  ( 108.7534185771431510, 233.5958772461660260, -9.188101187500095079 ) ) ;
#53540=CARTESIAN_POINT ( 'NONE',  ( 161.1894491815656352, 283.7774907297039135, 2.177303784804435871 ) ) ;
#53541=CARTESIAN_POINT ( 'NONE',  ( 189.5402112412503186, 274.1870215229640166, 15.72462957861923272 ) ) ;
#53543=ORIENTED_EDGE ( 'NONE', *, *, #48180, .F. ) ;
#53547=CARTESIAN_POINT ( 'NONE',  ( 205.8516076510241533, 269.9921726889444926, 5.257599149465654875 ) ) ;
#53550=EDGE_LOOP ( 'NONE', ( #58009, #88271, #100131, #39942 ) ) ;
#53551=CARTESIAN_POINT ( 'NONE',  ( 194.9041981377178274, 293.0630215474379838, 15.24265665161630956 ) ) ;
#53553=EDGE_LOOP ( 'NONE', ( #19547, #58979, #62515 ) ) ;
#53556=ORIENTED_EDGE ( 'NONE', *, *, #91115, .T. ) ;
#53557=CARTESIAN_POINT ( 'NONE',  ( 190.9474291326297930, 266.7645650087163745, -12.82661358031884546 ) ) ;
#53558=CARTESIAN_POINT ( 'NONE',  ( 151.9991393430420601, 267.3767632815465731, -16.97304508723421179 ) ) ;
#53561=CARTESIAN_POINT ( 'NONE',  ( 184.4758362669423093, 288.9580515395709881, -13.18921054981714924 ) ) ;
#53563=CARTESIAN_POINT ( 'NONE',  ( 201.1388841337167435, 282.2642286331299601, -18.17233400608081340 ) ) ;
#53564=VERTEX_POINT ( 'NONE', #13360 ) ;
#53565=CARTESIAN_POINT ( 'NONE',  ( 204.7166734748386716, 272.9112136331068541, -9.669763598799834270 ) ) ;
#53569=CARTESIAN_POINT ( 'NONE',  ( 192.6969673322854248, 271.7607060277501887, -14.66458718008113138 ) ) ;
#53573=CARTESIAN_POINT ( 'NONE',  ( 191.1479367720956475, 283.2912585338079907, -16.59553443474640133 ) ) ;
#53575=CARTESIAN_POINT ( 'NONE',  ( 72.54255783352381570, 218.8149278399160664, -9.188101187500095079 ) ) ;
#53576=CARTESIAN_POINT ( 'NONE',  ( 147.4047294057049271, 275.3345147238139248, 0.000000000000000000 ) ) ;
#53577=CARTESIAN_POINT ( 'NONE',  ( 147.4563929227680603, 275.2450308873625886, -3.847749617713808412 ) ) ;
#53581=CARTESIAN_POINT ( 'NONE',  ( 161.7412967960748915, 250.5028515975580774, -14.36228887024421041 ) ) ;
#53583=FACE_OUTER_BOUND ( 'NONE', #81224, .T. ) ;
#53588=CARTESIAN_POINT ( 'NONE',  ( 205.5852664446427411, 274.5628685607306920, -12.83526618994635449 ) ) ;
#53589=CARTESIAN_POINT ( 'NONE',  ( 196.2609093297512857, 290.7131288316392670, 16.03897268885959448 ) ) ;
#53592=CARTESIAN_POINT ( 'NONE',  ( 21.28450569914983248, 195.3464784336661637, 1.353441290958777327E-15 ) ) ;
#53593=CARTESIAN_POINT ( 'NONE',  ( 48.37494963522306080, 207.9244531367911293, -4.594050593750046652 ) ) ;
#53594=CARTESIAN_POINT ( 'NONE',  ( 157.4656258344471098, 257.9085309395441641, 18.30485740784190796 ) ) ;
#53595=CARTESIAN_POINT ( 'NONE',  ( 199.3359313799735162, 277.8054090533971134, 16.38672730308284997 ) ) ;
#53597=CARTESIAN_POINT ( 'NONE',  ( 147.1836429658426084, 243.5327760586659451, 1.948934522072303157E-15 ) ) ;
#53600=CARTESIAN_POINT ( 'NONE',  ( 198.5511052797322975, 286.7463930869835167, -17.24711022262289006 ) ) ;
#53601=CARTESIAN_POINT ( 'NONE',  ( 149.3801359649374092, 271.9130101976182914, -11.41245530317637424 ) ) ;
#53603=CARTESIAN_POINT ( 'NONE',  ( 53.67935523340274528, 210.9869531367911009, 4.594050593750046652 ) ) ;
#53604=CARTESIAN_POINT ( 'NONE',  ( 158.6590954928334440, 256.3327925383782144, -16.23563070158754584 ) ) ;
#53605=CARTESIAN_POINT ( 'NONE',  ( 194.3162776146270119, 290.4640039533715026, 16.60662885859720816 ) ) ;
#53606=CARTESIAN_POINT ( 'NONE',  ( 159.6419305724666344, 254.1390605605417079, 16.92015248457581933 ) ) ;
#53608=CARTESIAN_POINT ( 'NONE',  ( 153.3155690579966688, 265.0966401306517923, 17.21748418396146363 ) ) ;
#53609=AXIS2_PLACEMENT_3D ( 'NONE', #32197, #70189, #15487 ) ;
#53612=CARTESIAN_POINT ( 'NONE',  ( 120.0388121219831277, 230.1115022471901739, -5.000000000000041744 ) ) ;
#53613=CARTESIAN_POINT ( 'NONE',  ( 200.6129772034685175, 283.1751261563724142, 18.36811917402039640 ) ) ;
#53615=CARTESIAN_POINT ( 'NONE',  ( 162.8484966408963714, 268.3243502197477142, -16.55345495915420528 ) ) ;
#53616=VERTEX_POINT ( 'NONE', #53327 ) ;
#53618=ORIENTED_EDGE ( 'NONE', *, *, #59917, .F. ) ;
#53619=CARTESIAN_POINT ( 'NONE',  ( 159.7132918459648181, 254.0154592091499239, -16.90058287995827158 ) ) ;
#53620=CARTESIAN_POINT ( 'NONE',  ( 190.3130917849182424, 278.9726400120082417, -16.58120985382013046 ) ) ;
#53621=CARTESIAN_POINT ( 'NONE',  ( 205.1140127274842655, 272.9918749453946702, -10.94721916815361062 ) ) ;
#53623=CARTESIAN_POINT ( 'NONE',  ( 62.37595398666918811, 213.4865022471903444, 10.00000000000009415 ) ) ;
#53626=CARTESIAN_POINT ( 'NONE',  ( 148.0637215040603394, 274.1931069276759558, -7.795633835291665648 ) ) ;
#53633=EDGE_CURVE ( 'NONE', #55290, #74173, #27454, .T. ) ;
#53637=VERTEX_POINT ( 'NONE', #92375 ) ;
#53638=CARTESIAN_POINT ( 'NONE',  ( 174.7360925947785972, 286.2149905754307042, 10.56760205176437672 ) ) ;
#53639=CARTESIAN_POINT ( 'NONE',  ( 163.2243841140381733, 283.7100838097323958, -3.089421799144727920 ) ) ;
#53641=CARTESIAN_POINT ( 'NONE',  ( 163.4139553296302267, 247.6057220337265505, -10.31482883765270842 ) ) ;
#53642=CARTESIAN_POINT ( 'NONE',  ( 204.3951397407346064, 276.6242284793436852, 14.79595971842109137 ) ) ;
#53643=CARTESIAN_POINT ( 'NONE',  ( 159.5573297132660002, 254.2855935470410031, 16.91607698584599007 ) ) ;
#53644=CARTESIAN_POINT ( 'NONE',  ( 161.3533544474441612, 263.1708485045204498, -17.19112518918186083 ) ) ;
#53645=CARTESIAN_POINT ( 'NONE',  ( 164.6623933277139997, 245.4433639909459544, 5.552253915569078657 ) ) ;
#53646=CARTESIAN_POINT ( 'NONE',  ( 177.6810254821819797, 268.6267531607944079, 17.00611995725074621 ) ) ;
#53647=CARTESIAN_POINT ( 'NONE',  ( 181.7393891144199642, 260.2674940340181138, 9.489685412558293010 ) ) ;
#53648=CARTESIAN_POINT ( 'NONE',  ( 66.66973629016931113, 218.4869531367911293, 4.594050593750046652 ) ) ;
#53649=ORIENTED_EDGE ( 'NONE', *, *, #40629, .F. ) ;
#53650=CARTESIAN_POINT ( 'NONE',  ( 172.5238994923043947, 264.9055888575895779, 15.91205857390302292 ) ) ;
#53651=CARTESIAN_POINT ( 'NONE',  ( 163.7226971571442675, 281.6571063072398715, -10.85737102627868467 ) ) ;
#53653=CARTESIAN_POINT ( 'NONE',  ( 172.0910100529608258, 260.0785035667472584, 15.53398388876759206 ) ) ;
#53657=CARTESIAN_POINT ( 'NONE',  ( 195.7585776938734625, 285.5848788086319701, 16.95618921707195170 ) ) ;
#53659=B_SPLINE_SURFACE_WITH_KNOTS ( 'NONE', 3, 1, ( 
 ( #79057, #56202 ),
 ( #71935, #94258 ),
 ( #78538, #47611 ),
 ( #95278, #8624 ),
 ( #85683, #17731 ),
 ( #2026, #25841 ),
 ( #37632, #39490 ),
 ( #32911, #9125 ),
 ( #63818, #25315 ),
 ( #94753, #56715 ),
 ( #87199, #48634 ),
 ( #68543, #60932 ),
 ( #93255, #47113 ),
 ( #97249, #80565 ),
 ( #82063, #72948 ),
 ( #80062, #26822 ),
 ( #33942, #50117 ),
 ( #12121, #11635 ),
 ( #89187, #74442 ),
 ( #43500, #58690 ),
 ( #10631, #41507 ),
 ( #19736, #96758 ),
 ( #27326, #1417 ),
 ( #71822, #8508 ),
 ( #2421, #71321 ),
 ( #1913, #86562 ),
 ( #47495, #16101 ),
 ( #405, #85036 ),
 ( #93639, #63201 ),
 ( #16598, #93134 ),
 ( #62685, #15584 ),
 ( #48512, #40381 ),
 ( #33299, #78420 ),
 ( #47990, #25194 ) ),
 .UNSPECIFIED., .T., .F., .F.,
 ( 4, 2, 2, 2, 2, 2, 2, 2, 2, 2, 2, 2, 2, 2, 2, 2, 4 ),
 ( 2, 2 ),
 ( 0.000000000000000000, 0.06250000000000000000, 0.1250000000000000000, 0.1875000000000000000, 0.2500000000000000000, 0.3125000000000000000, 0.3750000000000000000, 0.4375000000000000000, 0.5000000000000000000, 0.5625000000000000000, 0.6250000000000000000, 0.6875000000000000000, 0.7500000000000000000, 0.8125000000000000000, 0.8750000000000000000, 0.9375000000000000000, 1.000000000000000000 ),
 ( 0.000000000000000000, 1.000000000000000000 ),
 .UNSPECIFIED. ) ;
#53661=CARTESIAN_POINT ( 'NONE',  ( 155.2419697281468416, 261.7600162942170527, 18.58580762350309357 ) ) ;
#53663=B_SPLINE_CURVE_WITH_KNOTS ( 'NONE', 3,
 ( #46491, #40388, #94647, #8514, #39383, #94149, #55093, #24702, #911, #56086, #55584, #47996, #24212, #47502, #78940, #17614, #48520, #10021, #40883, #69801, #71832, #25725, #411, #31300, #62188, #79951, #27715, #57592, #42388, #95668, #96648, #97149, #11028, #26712, #56605, #26216, #80964, #57092, #2943, #66693, #3910, #18625, #4401, #97629, #49502, #73321 ),
 .UNSPECIFIED., .F., .F.,
 ( 4, 2, 2, 2, 2, 2, 2, 2, 2, 2, 2, 2, 2, 2, 2, 2, 2, 2, 2, 2, 2, 2, 4 ),
 ( 0.002655933148385926021, 0.003065569018622698195, 0.003270386953741059345, 0.003372795921300235367, 0.003475204888859411822, 0.003680022823977764299, 0.003884840759096116775, 0.004294476629332821295, 0.005113748369806233804, 0.005933020110279646313, 0.006752291850753057954, 0.007571563591226471331, 0.007673972558785656893, 0.007725177042565249674, 0.007776381526344843323, 0.007827586010124435237, 0.007878790493904028885, 0.007981199461463143324, 0.008186017396581375671, 0.008390835331699609753, 0.008595653266817843835, 0.008800471201936079652, 0.009210107072172546080 ),
 .UNSPECIFIED. ) ;
#53664=CARTESIAN_POINT ( 'NONE',  ( 86.20995510670323370, 211.3923013555409796, 4.594050593750050204 ) ) ;
#53666=FACE_OUTER_BOUND ( 'NONE', #56984, .T. ) ;
#53667=ORIENTED_EDGE ( 'NONE', *, *, #81114, .T. ) ;
#53669=CARTESIAN_POINT ( 'NONE',  ( 163.7627442285549080, 260.9594149212073262, -17.29108549316627119 ) ) ;
#53670=B_SPLINE_CURVE_WITH_KNOTS ( 'NONE', 3,
 ( #84610, #29381, #37454, #82636, #14676, #60248, #6583, #90226, #13681, #75488, #90729, #6074, #21769, #36967, #37947, #68858 ),
 .UNSPECIFIED., .F., .F.,
 ( 4, 2, 2, 2, 2, 2, 2, 4 ),
 ( 0.000000000000000000, 0.0003786681000628067551, 0.0007573362001256135102, 0.001136004300188420265, 0.001514672400251227020, 0.001893340500314033992, 0.002272008600376840531, 0.003029344800502390290 ),
 .UNSPECIFIED. ) ;
#53672=CARTESIAN_POINT ( 'NONE',  ( 206.4229368915142686, 273.1119807867502800, 10.31819530520674810 ) ) ;
#53673=CARTESIAN_POINT ( 'NONE',  ( 162.0589963607739321, 283.8874982432868705, 0.5155476865025827582 ) ) ;
#53674=CARTESIAN_POINT ( 'NONE',  ( 194.9499559406243918, 279.5747724307917679, 17.51673600049429780 ) ) ;
#53678=CARTESIAN_POINT ( 'NONE',  ( 156.6772991465628309, 274.1558122050410020, 13.60064047269150400 ) ) ;
#53679=CARTESIAN_POINT ( 'NONE',  ( 164.2312669802896892, 282.6376396295875111, -10.04520723185695097 ) ) ;
#53680=CARTESIAN_POINT ( 'NONE',  ( 201.4463813434794019, 281.7316278426353620, -17.16864527463587820 ) ) ;
#53681=CARTESIAN_POINT ( 'NONE',  ( 151.3511865740561007, 278.6745403919405248, -1.693856907688049862 ) ) ;
#53683=CARTESIAN_POINT ( 'NONE',  ( 195.9563588169494892, 264.9583988535660524, 5.383380191835067663 ) ) ;
#53684=CARTESIAN_POINT ( 'NONE',  ( 165.8975677354378035, 271.5909624305264174, 17.28637137770206067 ) ) ;
#53686=CARTESIAN_POINT ( 'NONE',  ( 184.6470863607480339, 263.8121736845355940, -12.21359121072102560 ) ) ;
#53688=CARTESIAN_POINT ( 'NONE',  ( 195.2218307224750902, 263.8590524788139646, 0.8427596141219795278 ) ) ;
#53690=EDGE_CURVE ( 'NONE', #55671, #88888, #72079, .T. ) ;
#53691=CARTESIAN_POINT ( 'NONE',  ( 190.8545714895799392, 300.0771806536980648, -5.516553996882049837 ) ) ;
#53693=CARTESIAN_POINT ( 'NONE',  ( 207.2383675728608239, 271.6996134166075763, 7.873592648726489784 ) ) ;
#53694=CARTESIAN_POINT ( 'NONE',  ( 155.6518451030846961, 261.0500913200531841, 17.91778754207898317 ) ) ;
#53699=CARTESIAN_POINT ( 'NONE',  ( 166.3564281690869677, 285.9358929195967107, -3.185848211132425334 ) ) ;
#53701=CARTESIAN_POINT ( 'NONE',  ( 159.5204760365350012, 254.3494259875849082, 16.90107507090185379 ) ) ;
#53702=EDGE_CURVE ( 'NONE', #25608, #18420, #40705, .T. ) ;
#53703=( BOUNDED_CURVE ( )  B_SPLINE_CURVE ( 2, ( #84904, #7879, #70661, #61557, #47357, #76766, #86429, #94008, #23049 ),
 .UNSPECIFIED., .F., .T. ) 
 B_SPLINE_CURVE_WITH_KNOTS ( ( 3, 2, 2, 2, 3 ),
 ( 0.2701612903225806273, 0.2715053763440860024, 0.2741935483870967527, 0.2768817204301075030, 0.2782258064516128782 ),
 .UNSPECIFIED. ) 
 CURVE ( )  GEOMETRIC_REPRESENTATION_ITEM ( )  RATIONAL_B_SPLINE_CURVE ( ( 0.9330127018922194093, 0.9330127018922194093, 1.000000000000000000, 0.8660254037844387076, 1.000000000000000000, 0.8660254037844387076, 1.000000000000000000, 0.9330127018922194093, 0.9330127018922194093 ) ) 
 REPRESENTATION_ITEM ( '' )  );
#53704=CARTESIAN_POINT ( 'NONE',  ( 147.6614140599763232, 249.3927522451418213, 10.00000000000009592 ) ) ;
#53709=CARTESIAN_POINT ( 'NONE',  ( 138.5626868278036454, 239.2592609112380160, 2.679491924311254714 ) ) ;
#53710=CARTESIAN_POINT ( 'NONE',  ( 198.7829547491859330, 286.3448180261817129, -18.59838968157616179 ) ) ;
#53711=CARTESIAN_POINT ( 'NONE',  ( 10.18872876104421366, 182.8149278399160664, -9.188101187500095079 ) ) ;
#53715=CARTESIAN_POINT ( 'NONE',  ( 171.3229631070106223, 271.3642985138579320, -16.56375429974980662 ) ) ;
#53718=CARTESIAN_POINT ( 'NONE',  ( 187.6248024056100689, 259.1780923452019465, -0.7908679967713718728 ) ) ;
#53719=CARTESIAN_POINT ( 'NONE',  ( 183.0741553274718001, 295.7116116299331452, 1.042336010579862915 ) ) ;
#53720=CARTESIAN_POINT ( 'NONE',  ( 66.70608100559137199, 215.9865022471902591, -10.00000000000009415 ) ) ;
#53722=EDGE_CURVE ( 'NONE', #64894, #96192, #8071, .T. ) ;
#53723=CARTESIAN_POINT ( 'NONE',  ( 190.6036479972031259, 300.5117928913073797, -0.6824572005520307405 ) ) ;
#53724=CARTESIAN_POINT ( 'NONE',  ( 27.18482440607884243, 180.3768266524160140, 9.188101187500098632 ) ) ;
#53728=CARTESIAN_POINT ( 'NONE',  ( 199.1944722252943905, 285.6320488493591938, -18.17555833707144686 ) ) ;
#53729=CARTESIAN_POINT ( 'NONE',  ( 207.0200405408487541, 272.0777669287182334, 6.494273599193515878 ) ) ;
#53730=CARTESIAN_POINT ( 'NONE',  ( 186.1634877655031346, 266.9843438079278144, 13.21246304542636629 ) ) ;
#53731=CARTESIAN_POINT ( 'NONE',  ( 162.4616894431812284, 280.2021887225156433, -9.893998380673561854 ) ) ;
#53732=CARTESIAN_POINT ( 'NONE',  ( 162.1586611819999177, 280.6028376852936503, 8.927607144935116423 ) ) ;
#53737=CARTESIAN_POINT ( 'NONE',  ( 194.2321518193436987, 294.2270399159019121, 13.98132384850917020 ) ) ;
#53742=CARTESIAN_POINT ( 'NONE',  ( 153.4232513496498598, 270.1086993216917449, 15.21047082690287588 ) ) ;
#53743=EDGE_LOOP ( 'NONE', ( #9682, #31975, #17136, #95235 ) ) ;
#53747=CARTESIAN_POINT ( 'NONE',  ( 181.0230579576209209, 257.1489723966709562, -7.736786952959286978 ) ) ;
#53750=B_SPLINE_CURVE_WITH_KNOTS ( 'NONE', 3,
 ( #12264, #82699, #57344, #35041, #74066, #97864, #50736, #5154, #49756, #35548, #80707, #58339, #96395, #66449, #3191, #4146, #96900, #11770, #13266, #11283, #82201, #59317, #97376, #58824, #27942, #19388, #89315, #50247, #20362, #34074, #12771, #64965, #3673, #36034, #51233, #66934, #42633, #43636, #28435, #74576, #90297, #26468 ),
 .UNSPECIFIED., .F., .F.,
 ( 4, 2, 2, 2, 2, 2, 2, 2, 2, 2, 2, 2, 2, 2, 2, 2, 2, 2, 2, 2, 4 ),
 ( 0.002186794962226318740, 0.002620931419558167677, 0.002837999648224146573, 0.003055067876890125468, 0.003163601991223173246, 0.003272136105556221024, 0.003489204334222307038, 0.003923340791554368913, 0.004791613706218474447, 0.005659886620882579981, 0.006528159535546685516, 0.006962295992878701420, 0.007396432450210717324, 0.007504966564543741683, 0.007559233621710246057, 0.007613500678876752165, 0.007722034793209806014, 0.007830568907542859863, 0.008264705364875214039, 0.008698841822207566479, 0.009132978279539920655 ),
 .UNSPECIFIED. ) ;
#53751=CARTESIAN_POINT ( 'NONE',  ( 201.8854650512935507, 280.0099856999216854, 16.08627997847975166 ) ) ;
#53753=ORIENTED_EDGE ( 'NONE', *, *, #7738, .T. ) ;
#53754=CARTESIAN_POINT ( 'NONE',  ( 201.1755594471486859, 282.2007051268825535, -18.15567516623250910 ) ) ;
#53757=CARTESIAN_POINT ( 'NONE',  ( 54.07885559584777013, 190.4824982072973967, 3.021315404115420679E-15 ) ) ;
#53758=ORIENTED_EDGE ( 'NONE', *, *, #35961, .T. ) ;
#53759=CARTESIAN_POINT ( 'NONE',  ( 189.8533352240220893, 301.8113727360248504, -0.2033756396389863053 ) ) ;
#53764=ORIENTED_EDGE ( 'NONE', *, *, #15160, .F. ) ;
#53765=CARTESIAN_POINT ( 'NONE',  ( 190.1751179328237242, 301.2540287353828035, 3.252640783176552475 ) ) ;
#53767=EDGE_LOOP ( 'NONE', ( #15237, #80256, #98296, #61720, #41932 ) ) ;
#53769=CARTESIAN_POINT ( 'NONE',  ( 190.7779368023172708, 300.2099158256590385, 8.142228434510803581 ) ) ;
#53770=CARTESIAN_POINT ( 'NONE',  ( 177.5337925685473408, 280.1858537220425092, 16.79564202278857721 ) ) ;
#53776=CARTESIAN_POINT ( 'NONE',  ( 148.3997536239841679, 273.6110822229926498, 8.713694244701960301 ) ) ;
#53777=CARTESIAN_POINT ( 'NONE',  ( 149.5633513747893346, 271.5956717990251832, 12.83777201928511325 ) ) ;
#53780=CARTESIAN_POINT ( 'NONE',  ( 147.0276296945837373, 275.9876705829954062, 0.7617065417431535534 ) ) ;
#53781=CARTESIAN_POINT ( 'NONE',  ( 163.5652124800741944, 257.6669317359933302, 15.50305180493005075 ) ) ;
#53789=VERTEX_POINT ( 'NONE', #50104 ) ;
#53790=CARTESIAN_POINT ( 'NONE',  ( 206.4044394810958067, 269.6475539527112346, -2.777257397153266361 ) ) ;
#53795=CARTESIAN_POINT ( 'NONE',  ( 179.7730072551474905, 282.8179472056182817, -15.42817071794396000 ) ) ;
#53796=CARTESIAN_POINT ( 'NONE',  ( 190.7982574810033611, 262.8194055429554510, 8.405793748174573921 ) ) ;
#53797=CARTESIAN_POINT ( 'NONE',  ( 169.2038551074579402, 285.0728575209601559, -7.946202499671376707 ) ) ;
#53799=CARTESIAN_POINT ( 'NONE',  ( 162.6541320028305506, 248.9217746405196294, -10.16950121496441817 ) ) ;
#53801=CARTESIAN_POINT ( 'NONE',  ( 47.05812965368398437, 204.6427522451419350, -10.00000000000009415 ) ) ;
#53802=CARTESIAN_POINT ( 'NONE',  ( 126.9399520566163773, 244.0958772461660544, -9.188101187500095079 ) ) ;
#53803=CARTESIAN_POINT ( 'NONE',  ( 151.3124059063077311, 268.5662204852269497, -14.45542936000225609 ) ) ;
#53806=CARTESIAN_POINT ( 'NONE',  ( 187.4521490836430360, 281.3311025107105934, -17.05609064705406297 ) ) ;
#53808=CARTESIAN_POINT ( 'NONE',  ( 48.05019010880389629, 207.7369531367911293, -4.594050593750048428 ) ) ;
#53809=CARTESIAN_POINT ( 'NONE',  ( 178.7939207709925427, 291.7564144783525535, -6.099094555038819365 ) ) ;
#53811=VERTEX_POINT ( 'NONE', #42971 ) ;
#53813=CARTESIAN_POINT ( 'NONE',  ( 178.9271355275119504, 266.3440916513727643, 15.18250009252006016 ) ) ;
#53814=ADVANCED_FACE ( 'NONE', ( #36385 ), #2833, .F. ) ;
#53816=CARTESIAN_POINT ( 'NONE',  ( 147.5634954182374372, 275.0595239235922236, 4.682022975662822439 ) ) ;
#53818=B_SPLINE_CURVE_WITH_KNOTS ( 'NONE', 3,
 ( #71603, #46385, #62084, #68696, #99627, #48797, #15486, #2201, #95448, #79728, #77310, #10291, #94919, #25481, #41163, #97398, #11801, #50272, #3698, #96421, #43151, #97890, #20895, #80739, #73106, #36059, #43662, #74091, #81225, #88851, #27965, #66961, #42169, #3215, #34099, #28464, #34577, #82724, #81717, #66473, #42657, #4684, #49780, #59344 ),
 .UNSPECIFIED., .F., .F.,
 ( 4, 2, 2, 2, 2, 2, 2, 2, 2, 2, 2, 2, 2, 2, 2, 2, 2, 2, 2, 2, 2, 4 ),
 ( 0.0008670981119040801436, 0.001065074094278789692, 0.001164062085466145875, 0.001263050076653502059, 0.001461026059028214426, 0.001659002041402926793, 0.002054954006152456911, 0.002450905970901987030, 0.004034713829900430163, 0.004826617759399616167, 0.005222569724149247333, 0.005420545706524099346, 0.005519533697711450325, 0.005569027693305126682, 0.005618521688898802172, 0.005668015684492478529, 0.005717509680086154886, 0.005816497671273505865, 0.006014473653648208691, 0.006410425618397620415, 0.006806377583147032138, 0.007202329547896444729 ),
 .UNSPECIFIED. ) ;
#53821=CARTESIAN_POINT ( 'NONE',  ( 181.5591343598143794, 261.9482418225283027, 13.16139462748061284 ) ) ;
#53822=CARTESIAN_POINT ( 'NONE',  ( 113.3812418268423414, 226.2677522451417929, -5.000000000000041744 ) ) ;
#53827=CARTESIAN_POINT ( 'NONE',  ( 202.9689790241539242, 279.0944113002206564, 15.85114608332523289 ) ) ;
#53828=CARTESIAN_POINT ( 'NONE',  ( 208.3194307158603067, 269.8271571267425770, -2.120200867047394855 ) ) ;
#53829=CARTESIAN_POINT ( 'NONE',  ( 24.28913873611587348, 175.6423013555409796, -4.594050593750043987 ) ) ;
#53831=CARTESIAN_POINT ( 'NONE',  ( 196.0499355695823169, 273.7105960426958973, 14.77316126107874084 ) ) ;
#53832=CARTESIAN_POINT ( 'NONE',  ( 31.13482890205414222, 200.3297689869269220, -2.679491924311252493 ) ) ;
#53834=CARTESIAN_POINT ( 'NONE',  ( 198.2724843312039695, 277.3699619827796710, -15.35028023985861800 ) ) ;
#53835=CARTESIAN_POINT ( 'NONE',  ( 64.91088251055593616, 208.2833772461660544, -9.188101187500095079 ) ) ;
#53836=CARTESIAN_POINT ( 'NONE',  ( 200.3134965941964651, 283.6938417875134064, 18.29802468362849766 ) ) ;
#53839=CARTESIAN_POINT ( 'NONE',  ( 161.5029716424245407, 251.3413373469583973, -13.00020995489466458 ) ) ;
#53841=CARTESIAN_POINT ( 'NONE',  ( 162.1551341473669652, 267.3145892873122875, 16.48403697670416079 ) ) ;
#53842=CARTESIAN_POINT ( 'NONE',  ( 9.620573139467140322, 176.3615022471902307, -10.00000000000009592 ) ) ;
#53843=CARTESIAN_POINT ( 'NONE',  ( 164.3602934812760452, 245.9666162739349318, -7.171958108566009571 ) ) ;
#53844=CARTESIAN_POINT ( 'NONE',  ( 135.2211464324225858, 255.0024278399160949, -9.188101187500093303 ) ) ;
#53846=CARTESIAN_POINT ( 'NONE',  ( 164.5218961637583277, 259.6528873143451506, -16.87288754656431422 ) ) ;
#53847=CARTESIAN_POINT ( 'NONE',  ( 186.9066306565648858, 261.1604336654457938, 6.359003367118981842 ) ) ;
#53848=CARTESIAN_POINT ( 'NONE',  ( 206.4768661561222984, 273.0185725604343361, 11.39716120335626925 ) ) ;
#53852=ORIENTED_EDGE ( 'NONE', *, *, #84624, .F. ) ;
#53854=CARTESIAN_POINT ( 'NONE',  ( 178.0663898851194062, 286.0990649869549998, 12.90514440047635780 ) ) ;
#53855=CARTESIAN_POINT ( 'NONE',  ( 156.4379917615520696, 279.8315861724353226, -5.297762579854731868 ) ) ;
#53858=CARTESIAN_POINT ( 'NONE',  ( 206.6530282164287939, 272.7134509216173228, 9.408948237097369827 ) ) ;
#53860=CARTESIAN_POINT ( 'NONE',  ( 157.3661765229227285, 258.0807821998820373, -18.27254492731150748 ) ) ;
#53864=CARTESIAN_POINT ( 'NONE',  ( 191.5040086904573684, 295.9693678529874887, 12.56124033758404934 ) ) ;
#53866=CARTESIAN_POINT ( 'NONE',  ( 207.7625791259561652, 270.7916523727319031, -1.015623356719550063 ) ) ;
#53867=CARTESIAN_POINT ( 'NONE',  ( 201.0356089830534643, 282.4431064412383989, -18.18835788025466371 ) ) ;
#53869=CARTESIAN_POINT ( 'NONE',  ( 190.9414684426061797, 280.9540955606099715, 16.64794557087773796 ) ) ;
#53870=CARTESIAN_POINT ( 'NONE',  ( 192.6361035247282985, 294.0892689374524593, 14.43747539422717630 ) ) ;
#53872=CARTESIAN_POINT ( 'NONE',  ( 148.9232972370683399, 272.7042780851529642, 12.27045554427055940 ) ) ;
#53874=CARTESIAN_POINT ( 'NONE',  ( 190.7684124627589313, 298.2021613433544758, 8.215386510820527732 ) ) ;
#53875=ORIENTED_EDGE ( 'NONE', *, *, #29235, .F. ) ;
#53876=CARTESIAN_POINT ( 'NONE',  ( 183.8274263638271577, 281.3324037098167310, 17.41033114534894111 ) ) ;
#53877=CARTESIAN_POINT ( 'NONE',  ( 185.0921216717482025, 263.1328331163757639, -12.61684766275084790 ) ) ;
#53878=CIRCLE ( 'NONE', #8570, 17.82106496071138224 ) ;
#53879=CARTESIAN_POINT ( 'NONE',  ( 197.0313051377892748, 289.3787641501790517, -17.15509075150697882 ) ) ;
#53884=CARTESIAN_POINT ( 'NONE',  ( 104.9102572999672276, 237.5024278399160949, 9.188101187500095079 ) ) ;
#53885=CARTESIAN_POINT ( 'NONE',  ( 203.1954647288614240, 278.7021265524792852, 16.53270523508054879 ) ) ;
#53886=CARTESIAN_POINT ( 'NONE',  ( 150.8757650385446993, 269.3225046528533539, 14.31332712971473953 ) ) ;
#53888=B_SPLINE_SURFACE_WITH_KNOTS ( 'NONE', 3, 1, ( 
 ( #10840, #19462 ),
 ( #50813, #81762 ),
 ( #12336, #33643 ),
 ( #56915, #43201 ),
 ( #4737, #35621 ),
 ( #41716, #45201 ),
 ( #75623, #5226 ),
 ( #29516, #21906 ),
 ( #99426, #6714 ),
 ( #76140, #29030 ),
 ( #90870, #82275 ),
 ( #20945, #91850 ),
 ( #44693, #12848 ),
 ( #68504, #44200 ),
 ( #76613, #30003 ),
 ( #14804, #97934 ),
 ( #52307, #28509 ),
 ( #83245, #13811 ),
 ( #51828, #37105 ),
 ( #22899, #38083 ),
 ( #92349, #36104 ),
 ( #37593, #7199 ),
 ( #99923, #67009 ),
 ( #59390, #90366 ),
 ( #29401, #20315 ),
 ( #36989, #91725 ),
 ( #74529, #5108 ),
 ( #45574, #45089 ),
 ( #90753, #22290 ),
 ( #97328, #28392 ),
 ( #60270, #76502 ),
 ( #83131, #91226 ),
 ( #51714, #35987 ),
 ( #67899, #13219 ) ),
 .UNSPECIFIED., .T., .F., .F.,
 ( 4, 2, 2, 2, 2, 2, 2, 2, 2, 2, 2, 2, 2, 2, 2, 2, 4 ),
 ( 2, 2 ),
 ( 0.000000000000000000, 0.06250000000000000000, 0.1250000000000000000, 0.1875000000000000000, 0.2500000000000000000, 0.3125000000000000000, 0.3750000000000000000, 0.4375000000000000000, 0.5000000000000000000, 0.5625000000000000000, 0.6250000000000000000, 0.6875000000000000000, 0.7500000000000000000, 0.8125000000000000000, 0.8750000000000000000, 0.9375000000000000000, 1.000000000000000000 ),
 ( 0.000000000000000000, 1.000000000000000000 ),
 .UNSPECIFIED. ) ;
#53889=VERTEX_POINT ( 'NONE', #38879 ) ;
#53897=CARTESIAN_POINT ( 'NONE',  ( 163.7595992360150490, 247.0070492265414828, -6.976205010573520049 ) ) ;
#53900=CARTESIAN_POINT ( 'NONE',  ( 169.0161032148113236, 281.7934031441919842, 11.67333235455804363 ) ) ;
#53904=ORIENTED_EDGE ( 'NONE', *, *, #59673, .F. ) ;
#53910=CARTESIAN_POINT ( 'NONE',  ( 202.8499463704053198, 279.3005819042728604, 17.04674939340617001 ) ) ;
#53911=CARTESIAN_POINT ( 'NONE',  ( 159.3586121662929713, 254.6297824347537642, -15.50090345830412630 ) ) ;
#53912=CARTESIAN_POINT ( 'NONE',  ( -22.42236680055709641, 157.8615022471902591, 0.000000000000000000 ) ) ;
#53913=CARTESIAN_POINT ( 'NONE',  ( 183.8210692855788864, 257.9504670327482927, 6.873620218444065344 ) ) ;
#53914=CARTESIAN_POINT ( 'NONE',  ( 200.4592688079413847, 283.4413569069752725, 18.39277739746426832 ) ) ;
#53915=CARTESIAN_POINT ( 'NONE',  ( 157.9042112748594775, 281.1459165152564310, 1.688126963922599755 ) ) ;
#53916=VERTEX_POINT ( 'NONE', #29308 ) ;
#53917=CARTESIAN_POINT ( 'NONE',  ( 155.5408495238017395, 261.2423413027869969, -17.06121474717059527 ) ) ;
#53920=CARTESIAN_POINT ( 'NONE',  ( -2.233149578380279721, 169.5177522451418781, -10.00000000000009592 ) ) ;
#53921=CARTESIAN_POINT ( 'NONE',  ( 192.8989532340791300, 266.9009477387879201, -11.33294346249175000 ) ) ;
#53922=CARTESIAN_POINT ( 'NONE',  ( 166.7681478528634216, 248.8687067081767452, 8.283836764471310232 ) ) ;
#53925=CARTESIAN_POINT ( 'NONE',  ( 11.59636713795893925, 171.3768266524160140, 9.188101187500098632 ) ) ;
#53927=AXIS2_PLACEMENT_3D ( 'NONE', #64219, #19146, #72350 ) ;
#53928=CARTESIAN_POINT ( 'NONE',  ( 27.21171415029068186, 176.5177522451417929, 5.000000000000051514 ) ) ;
#53929=ORIENTED_EDGE ( 'NONE', *, *, #80108, .T. ) ;
#53930=B_SPLINE_CURVE_WITH_KNOTS ( 'NONE', 3,
 ( #44266, #5287, #97033, #28076 ),
 .UNSPECIFIED., .F., .F.,
 ( 4, 4 ),
 ( 0.01837538304589518209, 0.02737905013630983694 ),
 .UNSPECIFIED. ) ;
#53932=CARTESIAN_POINT ( 'NONE',  ( 165.4781454232152953, 246.0304399151612245, -2.837517270351797016 ) ) ;
#53933=CARTESIAN_POINT ( 'NONE',  ( 199.1041333440138317, 265.1832257255362038, 0.2027868546939186056 ) ) ;
#53934=EDGE_CURVE ( 'NONE', #37554, #312, #82484, .T. ) ;
#53935=DIRECTION ( 'NONE',  ( -0.8660254037844387076, -0.4999999999999998890, -0.000000000000000000 ) ) ;
#53936=FACE_OUTER_BOUND ( 'NONE', #78021, .T. ) ;
#53937=CARTESIAN_POINT ( 'NONE',  ( 162.4213055719747274, 249.3250418481068778, -10.93467306481309187 ) ) ;
#53939=CARTESIAN_POINT ( 'NONE',  ( 149.6775418821061123, 277.3372939425368031, 3.097505863387055580 ) ) ;
#53940=B_SPLINE_CURVE_WITH_KNOTS ( 'NONE', 3,
 ( #5824, #66130, #96582, #74260 ),
 .UNSPECIFIED., .F., .F.,
 ( 4, 4 ),
 ( 0.009217897952540354822, 0.01511262126107456444 ),
 .UNSPECIFIED. ) ;
#53941=CARTESIAN_POINT ( 'NONE',  ( 12.00188267627663308, 186.9244531367911293, -4.594050593750046652 ) ) ;
#53942=VECTOR ( 'NONE', #38785, 1000.000000000000000 ) ;
#53943=CARTESIAN_POINT ( 'NONE',  ( 117.4951228184160783, 229.4548013555409796, -4.594050593750042211 ) ) ;
#53944=CARTESIAN_POINT ( 'NONE',  ( 178.9323954259722314, 291.8122831636629826, -6.158156483446289187 ) ) ;
#53945=CARTESIAN_POINT ( 'NONE',  ( 195.8821561183051188, 275.1718881706996171, 15.74945206926084040 ) ) ;
#53949=CARTESIAN_POINT ( 'NONE',  ( 175.8908519962235459, 273.1107590772576827, -17.81327592954072259 ) ) ;
#53950=CARTESIAN_POINT ( 'NONE',  ( -5.778093977583854013, 155.2202760586659451, -5.415160957724236172E-17 ) ) ;
#53951=CARTESIAN_POINT ( 'NONE',  ( 195.7617614321055157, 291.5776783508526364, 16.33009124109666033 ) ) ;
#53952=CARTESIAN_POINT ( 'NONE',  ( 155.6518451030846961, 261.0500913200531841, 17.91778754207898317 ) ) ;
#53953=CARTESIAN_POINT ( 'NONE',  ( 161.1061647010182583, 251.6029326557136585, -13.56144933775657613 ) ) ;
#53954=CARTESIAN_POINT ( 'NONE',  ( 190.1170242653768128, 284.8971620602226267, 17.14187718570638097 ) ) ;
#53956=CARTESIAN_POINT ( 'NONE',  ( 171.5938502359046822, 279.8409701536578496, 13.97011670356616975 ) ) ;
#53957=CARTESIAN_POINT ( 'NONE',  ( 192.5511529533421822, 265.2447470188456009, 7.887563979430734840 ) ) ;
#53959=CARTESIAN_POINT ( 'NONE',  ( 190.3691966041315311, 300.9178746160123410, 0.1783449565851275009 ) ) ;
#53960=CARTESIAN_POINT ( 'NONE',  ( 150.5917955345242376, 274.2788540000528315, 10.61926890178174965 ) ) ;
#53963=CARTESIAN_POINT ( 'NONE',  ( 184.3681170320605247, 268.9686055817056172, 16.19769924168502229 ) ) ;
#53964=CARTESIAN_POINT ( 'NONE',  ( 100.7430306879021202, 216.7202760586659736, -5.415160957724236172E-17 ) ) ;
#53966=CARTESIAN_POINT ( 'NONE',  ( 191.5544531425776427, 298.8649500714207647, 8.366689293739112188 ) ) ;
#53969=CARTESIAN_POINT ( 'NONE',  ( 193.3110229662232484, 278.0645543825088453, 16.34055514812991916 ) ) ;
#53970=CARTESIAN_POINT ( 'NONE',  ( 196.3454718165693862, 290.5666623080560385, 17.52957579560619905 ) ) ;
#53971=CARTESIAN_POINT ( 'NONE',  ( 198.6363782946250183, 286.5986958926748116, -18.50260615857378355 ) ) ;
#53972=CARTESIAN_POINT ( 'NONE',  ( -16.97593537095525917, 172.5530062829863027, 9.296355089585912665E-16 ) ) ;
#53973=CARTESIAN_POINT ( 'NONE',  ( 86.26382137438996267, 220.6115022471902591, 10.00000000000009592 ) ) ;
#53974=CARTESIAN_POINT ( 'NONE',  ( 131.5677753063155251, 236.7677522451417929, -5.000000000000041744 ) ) ;
#53978=CARTESIAN_POINT ( 'NONE',  ( 163.2942584940569191, 258.1478583562382028, 16.77787020301746779 ) ) ;
#53979=CARTESIAN_POINT ( 'NONE',  ( 196.7852062865125902, 267.4955962336644006, 9.737905958038332699 ) ) ;
#53980=CARTESIAN_POINT ( 'NONE',  ( 197.0313051377892748, 289.3787641501790517, -17.15509075150697882 ) ) ;
#53985=CARTESIAN_POINT ( 'NONE',  ( 169.8457105410257668, 251.1523016893514750, -8.510778188974899905 ) ) ;
#53987=DIRECTION ( 'NONE',  ( 0.8660254037844393737, 0.4999999999999986677, 0.000000000000000000 ) ) ;
#53989=CARTESIAN_POINT ( 'NONE',  ( 188.9081020563885716, 279.7620193737561181, 16.69253326113207336 ) ) ;
#53992=CARTESIAN_POINT ( 'NONE',  ( -22.42236680055709641, 157.8615022471902591, 0.000000000000000000 ) ) ;
#53993=DIRECTION ( 'NONE',  ( -0.8660254037844387076, -0.4999999999999998890, -0.000000000000000000 ) ) ;
#53996=CARTESIAN_POINT ( 'NONE',  ( 158.8995732337010054, 255.8553380628405591, 16.02046230101960589 ) ) ;
#53997=CARTESIAN_POINT ( 'NONE',  ( 190.8429499865819707, 278.0757709512191695, -17.64141544901220371 ) ) ;
#53998=CARTESIAN_POINT ( 'NONE',  ( 153.6416917630915862, 264.5317790359255810, -18.09859318578890708 ) ) ;
#53999=CARTESIAN_POINT ( 'NONE',  ( 182.6098810326567445, 277.4798346879709925, 17.79761443238625418 ) ) ;
#54003=EDGE_CURVE ( 'NONE', #80416, #33600, #83536, .T. ) ;
#54005=( BOUNDED_CURVE ( )  B_SPLINE_CURVE ( 2, ( #13846, #73668, #58921, #50349, #90899, #51858, #82307, #21449, #12878 ),
 .UNSPECIFIED., .F., .T. ) 
 B_SPLINE_CURVE_WITH_KNOTS ( ( 3, 2, 2, 2, 3 ),
 ( 0.2298387096774193450, 0.2311827956989247201, 0.2338709677419354704, 0.2365591397849462485, 0.2379032258064516236 ),
 .UNSPECIFIED. ) 
 CURVE ( )  GEOMETRIC_REPRESENTATION_ITEM ( )  RATIONAL_B_SPLINE_CURVE ( ( 0.9330127018922194093, 0.9330127018922194093, 1.000000000000000000, 0.8660254037844387076, 1.000000000000000000, 0.8660254037844387076, 1.000000000000000000, 0.9330127018922194093, 0.9330127018922194093 ) ) 
 REPRESENTATION_ITEM ( '' )  );
#54007=CARTESIAN_POINT ( 'NONE',  ( 207.1609884636329184, 269.8336379652346295, -0.06011041530970540059 ) ) ;
#54010=CARTESIAN_POINT ( 'NONE',  ( 169.9943822607803838, 269.4584602086645191, 17.68792189269073489 ) ) ;
#54011=ORIENTED_EDGE ( 'NONE', *, *, #79736, .F. ) ;
#54012=DIRECTION ( 'NONE',  ( -0.8660254037844387076, -0.4999999999999998890, -0.000000000000000000 ) ) ;
#54014=CARTESIAN_POINT ( 'NONE',  ( 197.4972225514353852, 278.9538932286835689, 17.08281588120735606 ) ) ;
#54015=CARTESIAN_POINT ( 'NONE',  ( 197.5405048943464124, 273.3027842733730495, -13.38352526854320601 ) ) ;
#54017=CARTESIAN_POINT ( 'NONE',  ( 192.6946760137320780, 261.4813915186712165, 3.932628284434791966E-12 ) ) ;
#54018=CARTESIAN_POINT ( 'NONE',  ( 170.1908625819879148, 250.5941916552922351, -5.502416923392919657 ) ) ;
#54020=CARTESIAN_POINT ( 'NONE',  ( -22.42236680055709641, 157.8615022471902591, 0.000000000000000000 ) ) ;
#54022=CARTESIAN_POINT ( 'NONE',  ( 178.5299698652597726, 254.5949104052269263, 5.887118732947904221 ) ) ;
#54023=CARTESIAN_POINT ( 'NONE',  ( 113.7873647845227225, 230.3768266524160140, -9.188101187500091527 ) ) ;
#54026=CARTESIAN_POINT ( 'NONE',  ( 179.7478462366760539, 290.5198049800060858, -9.475730908087831139 ) ) ;
#54028=ORIENTED_EDGE ( 'NONE', *, *, #53520, .F. ) ;
#54032=CARTESIAN_POINT ( 'NONE',  ( 192.5715242950574009, 297.1033311604131200, 11.04771845794762619 ) ) ;
#54034=CARTESIAN_POINT ( 'NONE',  ( 200.8665851640556070, 282.7358642834317948, -16.69422397739980823 ) ) ;
#54035=CARTESIAN_POINT ( 'NONE',  ( 88.29250555182709093, 233.3297689869268936, -2.679491924311252493 ) ) ;
#54037=ORIENTED_EDGE ( 'NONE', *, *, #36453, .F. ) ;
#54038=CARTESIAN_POINT ( 'NONE',  ( 148.1128072303691283, 274.1080879557827643, 10.32046898584627925 ) ) ;
#54040=CARTESIAN_POINT ( 'NONE',  ( 194.3442947553755005, 294.0328026529847421, -15.97648891113594871 ) ) ;
#54042=CARTESIAN_POINT ( 'NONE',  ( 191.8700694318469289, 267.7572204393412107, -12.41388222293339894 ) ) ;
#54043=CARTESIAN_POINT ( 'NONE',  ( 159.8863521765906341, 279.1613695579630416, 10.84044400854919843 ) ) ;
#54044=CARTESIAN_POINT ( 'NONE',  ( 195.5930400684863741, 265.3186233137946033, 4.406227592133483029 ) ) ;
#54047=CARTESIAN_POINT ( 'NONE',  ( 184.3838639634485617, 288.5488729356416115, -13.88906064327808387 ) ) ;
#54049=CARTESIAN_POINT ( 'NONE',  ( 152.9251141908703175, 265.7729277985770864, -16.20110192949203309 ) ) ;
#54051=CARTESIAN_POINT ( 'NONE',  ( 190.9498149295421570, 299.9122141765958531, -5.138500224925297566 ) ) ;
#54054=CARTESIAN_POINT ( 'NONE',  ( 186.8270895101041447, 262.8347829455524334, -9.018193060954537543 ) ) ;
#54055=CARTESIAN_POINT ( 'NONE',  ( 182.2991478702006134, 275.2734891516705034, -17.80812521087705846 ) ) ;
#54058=CARTESIAN_POINT ( 'NONE',  ( 189.0215474952646559, 269.9904085317868976, -14.04715979591349040 ) ) ;
#54059=CARTESIAN_POINT ( 'NONE',  ( 188.1045636728014472, 299.4598449876921791, -3.709602300402848218 ) ) ;
#54063=CARTESIAN_POINT ( 'NONE',  ( 155.4216552449402684, 261.4487918497463284, 18.51722274565528892 ) ) ;
#54066=CARTESIAN_POINT ( 'NONE',  ( 71.86588871287597158, 221.4869531367911293, 4.594050593750046652 ) ) ;
#54069=CARTESIAN_POINT ( 'NONE',  ( 154.9528145190857344, 262.2608478075840708, -17.26679351315302213 ) ) ;
#54071=CARTESIAN_POINT ( 'NONE',  ( 161.8807657183444064, 250.2612843381103573, -13.52770735624900311 ) ) ;
#54072=DIRECTION ( 'NONE',  ( -0.8660254037844387076, -0.4999999999999998890, -0.000000000000000000 ) ) ;
#54076=EDGE_CURVE ( 'NONE', #25397, #75682, #35870, .T. ) ;
#54079=CARTESIAN_POINT ( 'NONE',  ( 167.1283625793575425, 250.6242252090678448, -8.897399544333461918 ) ) ;
#54080=CARTESIAN_POINT ( 'NONE',  ( 204.8617891913918925, 275.8159679214818425, -13.46007153234462450 ) ) ;
#54081=CARTESIAN_POINT ( 'NONE',  ( 196.3720681610792553, 290.5205960880691691, 16.18360420724715354 ) ) ;
#54082=CARTESIAN_POINT ( 'NONE',  ( 147.6095992045671323, 244.4824982072973967, 3.021315404115420679E-15 ) ) ;
#54083=VECTOR ( 'NONE', #37379, 1000.000000000000114 ) ;
#54084=CARTESIAN_POINT ( 'NONE',  ( 51.75829523846228852, 194.5643266524159856, -9.188101187500093303 ) ) ;
#54087=CARTESIAN_POINT ( 'NONE',  ( 147.8819534105757043, 274.5079385007862811, -9.338341377131436971 ) ) ;
#54088=CARTESIAN_POINT ( 'NONE',  ( -10.37017993122368154, 171.4865022471902876, 10.00000000000009237 ) ) ;
#54089=FACE_OUTER_BOUND ( 'NONE', #37742, .T. ) ;
#54090=CARTESIAN_POINT ( 'NONE',  ( 196.8298363030699250, 269.8487463528495596, -10.82627680366021750 ) ) ;
#54092=CARTESIAN_POINT ( 'NONE',  ( 151.0426280674448378, 269.0334894088936153, -15.84467774422408581 ) ) ;
#54093=CARTESIAN_POINT ( 'NONE',  ( 197.0184425104562820, 289.4010428742387262, -16.90752553128928426 ) ) ;
#54095=CARTESIAN_POINT ( 'NONE',  ( 62.93552237999645627, 197.9548013555410080, -4.594050593750042211 ) ) ;
#54097=CARTESIAN_POINT ( 'NONE',  ( 202.9490938173916561, 279.1288534886517709, -16.56031645010252973 ) ) ;
#54098=CARTESIAN_POINT ( 'NONE',  ( 197.9598023461055902, 287.7705598106892921, 18.23120408239484291 ) ) ;
#54100=CARTESIAN_POINT ( 'NONE',  ( 149.5435553735961491, 275.3446937576266578, 7.453328770706503015 ) ) ;
#54103=CARTESIAN_POINT ( 'NONE',  ( 106.5432495796755603, 238.9865022471903160, 10.00000000000009237 ) ) ;
#54104=CARTESIAN_POINT ( 'NONE',  ( 11.60290295393121696, 189.0530062829863027, -4.648177544792955347E-16 ) ) ;
#54105=CARTESIAN_POINT ( 'NONE',  ( 165.0532575723395041, 244.7663672603923715, -2.144843157699870773 ) ) ;
#54106=ORIENTED_EDGE ( 'NONE', *, *, #63979, .T. ) ;
#54110=CARTESIAN_POINT ( 'NONE',  ( 159.4491226731523454, 254.4730136382542582, -15.39140229921534520 ) ) ;
#54111=CARTESIAN_POINT ( 'NONE',  ( 189.7589793277493868, 278.3644573459904450, -16.50316607585832784 ) ) ;
#54116=CARTESIAN_POINT ( 'NONE',  ( 194.2900850603946310, 294.1266965989547657, -15.88613936555681505 ) ) ;
#54122=VERTEX_POINT ( 'NONE', #95137 ) ;
#54124=B_SPLINE_CURVE_WITH_KNOTS ( 'NONE', 3,
 ( #41289, #33726, #50895, #28099, #89463, #58970, #90455, #58003, #21024, #19539, #65600, #12928, #89942, #96550, #35704, #51908, #27120, #88985, #43787, #28592, #67091, #81354 ),
 .UNSPECIFIED., .F., .F.,
 ( 4, 2, 2, 2, 2, 2, 2, 2, 2, 2, 4 ),
 ( 0.003530854327582292826, 0.003674460630036895971, 0.003818066932491499116, 0.003961673234946102261, 0.004105279537400705406, 0.004392492142309911696, 0.004679704747219117986, 0.005254129957037643323, 0.005828555166856168659, 0.006977405586493288722, 0.008126256006130408785 ),
 .UNSPECIFIED. ) ;
#54125=CARTESIAN_POINT ( 'NONE',  ( 189.6666044902458168, 284.7049877867155487, 17.41007887138588117 ) ) ;
#54126=ORIENTED_EDGE ( 'NONE', *, *, #17228, .F. ) ;
#54127=CARTESIAN_POINT ( 'NONE',  ( 174.7537062242112995, 286.2005298146486894, 10.60273640048973398 ) ) ;
#54130=CARTESIAN_POINT ( 'NONE',  ( 208.3829315663354862, 269.7171704273955015, -1.768817828503133072 ) ) ;
#54131=CARTESIAN_POINT ( 'NONE',  ( 163.8040269124969939, 246.9300982336122559, 6.025552750865228013 ) ) ;
#54132=CARTESIAN_POINT ( 'NONE',  ( 187.7470681246648780, 294.2386427693206201, -10.89872421713186590 ) ) ;
#54133=CARTESIAN_POINT ( 'NONE',  ( 164.3306481956919924, 265.7257225416949495, -17.70433004990753645 ) ) ;
#54134=CARTESIAN_POINT ( 'NONE',  ( 140.4172988551291894, 258.0024278399160949, -9.188101187500093303 ) ) ;
#54135=EDGE_CURVE ( 'NONE', #68457, #10970, #25703, .T. ) ;
#54136=CARTESIAN_POINT ( 'NONE',  ( 159.8591301300080261, 254.2983864834555447, -15.29415641145932803 ) ) ;
#54137=CARTESIAN_POINT ( 'NONE',  ( 178.8348794910443758, 257.7124399359195195, 10.03872504014272771 ) ) ;
#54138=CARTESIAN_POINT ( 'NONE',  ( 76.54827242179186442, 208.8768266524160140, 9.188101187500098632 ) ) ;
#54140=CARTESIAN_POINT ( 'NONE',  ( 191.1489696025915919, 299.5672681643093256, 8.892130899335590755 ) ) ;
#54143=CARTESIAN_POINT ( 'NONE',  ( 185.2824853868734181, 297.7695098558858149, 4.231266468330407093 ) ) ;
#54148=B_SPLINE_CURVE_WITH_KNOTS ( 'NONE', 3,
 ( #39630, #23948, #54848, #79206, #24457, #1167, #16358, #8758, #32041, #33567, #40137, #64461, #32561, #2174, #55339, #40642, #71077, #2676, #55826, #9780, #71577, #94396, #86315, #94893, #33056, #86820, #87343, #63459, #17875, #87831, #48772, #80203, #79705, #10267, #49266, #41137, #10771, #85829, #57346, #88320, #20363, #42145, #51235, #18875, #12773, #51759 ),
 .UNSPECIFIED., .F., .F.,
 ( 4, 2, 2, 2, 2, 2, 2, 2, 2, 2, 2, 2, 2, 2, 2, 2, 2, 2, 2, 2, 2, 2, 4 ),
 ( 0.0004825194710001968449, 0.001489721961729743209, 0.001993323207094548077, 0.002119223518435738723, 0.002245123829776929369, 0.002371024141118120016, 0.002496924452459310662, 0.002748725075141691954, 0.003000525697824073246, 0.003504126943188788125, 0.004511329433918270793, 0.005518531924647753460, 0.006022133170012418900, 0.006273933792694715190, 0.006525734415377010614, 0.006588684571047504455, 0.006651634726717998297, 0.006714584882388492139, 0.006777535038058985981, 0.007029335660740964817, 0.007532936906104987541, 0.008036538151469010266, 0.008540139396833033858 ),
 .UNSPECIFIED. ) ;
#54150=DIRECTION ( 'NONE',  ( 0.4999999999999998890, -0.8660254037844385966, 0.000000000000000000 ) ) ;
#54153=EDGE_CURVE ( 'NONE', #39418, #83741, #45544, .T. ) ;
#54154=CARTESIAN_POINT ( 'NONE',  ( 81.79837788435251866, 218.0333772461660544, 9.188101187500095079 ) ) ;
#54155=ORIENTED_EDGE ( 'NONE', *, *, #51770, .T. ) ;
#54156=VECTOR ( 'NONE', #7201, 1000.000000000000000 ) ;
#54158=CARTESIAN_POINT ( 'NONE',  ( 161.3512397267719791, 251.1784502594418598, -12.94313244495258530 ) ) ;
#54162=CARTESIAN_POINT ( 'NONE',  ( 184.3861787086252662, 275.3536848780280479, 16.37667645762307700 ) ) ;
#54163=CARTESIAN_POINT ( 'NONE',  ( 207.1609884636329184, 269.8336379652346295, -0.06011041530970540059 ) ) ;
#54164=CARTESIAN_POINT ( 'NONE',  ( 207.3562937958418217, 270.9032348272035051, -2.066387192265693340 ) ) ;
#54165=CARTESIAN_POINT ( 'NONE',  ( 153.2593913506692616, 267.1939427739956727, -16.45456985337825984 ) ) ;
#54166=VERTEX_POINT ( 'NONE', #18604 ) ;
#54167=CARTESIAN_POINT ( 'NONE',  ( 158.4333560722609775, 259.8736997123415904, 17.69911652888126952 ) ) ;
#54168=CARTESIAN_POINT ( 'NONE',  ( 184.9983038504436479, 260.1326763968729097, 6.322520505052498407 ) ) ;
#54170=CARTESIAN_POINT ( 'NONE',  ( 200.6583719735737645, 283.0965001081523269, -17.35266956530146132 ) ) ;
#54175=EDGE_CURVE ( 'NONE', #76828, #60981, #44293, .T. ) ;
#54177=CARTESIAN_POINT ( 'NONE',  ( 29.55951135474875358, 176.3262482093457777, 3.021315404115420679E-15 ) ) ;
#54178=CARTESIAN_POINT ( 'NONE',  ( 171.5399254682851051, 251.6352709114593722, 7.166479175369310894 ) ) ;
#54179=CARTESIAN_POINT ( 'NONE',  ( 198.5359561926482570, 266.1776289375414990, 1.198487561129841339 ) ) ;
#54180=CARTESIAN_POINT ( 'NONE',  ( 153.2819998794291791, 270.3646030198663084, 13.95166877408641248 ) ) ;
#54181=EDGE_CURVE ( 'NONE', #86304, #74262, #99941, .T. ) ;
#54182=ORIENTED_EDGE ( 'NONE', *, *, #28525, .T. ) ;
#54183=EDGE_CURVE ( 'NONE', #40233, #2331, #98606, .T. ) ;
#54185=AXIS2_PLACEMENT_3D ( 'NONE', #27834, #58711, #90684 ) ;
#54188=CARTESIAN_POINT ( 'NONE',  ( 167.9211111253673323, 249.4040118433879627, 8.061254949035708606 ) ) ;
#54190=CARTESIAN_POINT ( 'NONE',  ( 176.1762632841285381, 285.4164495326317024, -12.05309685415307186 ) ) ;
#54193=CARTESIAN_POINT ( 'NONE',  ( 163.0172387208063753, 284.2669704625143368, -4.045436010492660550 ) ) ;
#54194=CARTESIAN_POINT ( 'NONE',  ( 125.2349645446896886, 253.1115022471903160, -5.000000000000047962 ) ) ;
#54196=CARTESIAN_POINT ( 'NONE',  ( -5.399381411310668177, 161.5643266524160140, -9.188101187500093303 ) ) ;
#54197=CARTESIAN_POINT ( 'NONE',  ( 146.7678550509543811, 269.9772791071537199, -2.458545531893916687E-15 ) ) ;
#54199=CARTESIAN_POINT ( 'NONE',  ( 160.1603183234873313, 253.8555898246377467, -15.06084538093693936 ) ) ;
#54201=CARTESIAN_POINT ( 'NONE',  ( 202.6051175132338926, 273.9538057854381350, -13.19822448684500849 ) ) ;
#54203=CARTESIAN_POINT ( 'NONE',  ( 31.75860784375665702, 179.9548013555409796, -4.594050593750042211 ) ) ;
#54205=CARTESIAN_POINT ( 'NONE',  ( 181.9103902747559687, 275.6752150453591526, -16.43134084343946455 ) ) ;
#54208=CARTESIAN_POINT ( 'NONE',  ( 205.0994677818405023, 275.4042965269534307, -14.14519517703424789 ) ) ;
#54209=CARTESIAN_POINT ( 'NONE',  ( 5.723458822437122784, 184.1115022471903160, -5.000000000000047962 ) ) ;
#54210=CARTESIAN_POINT ( 'NONE',  ( 176.1640045926653499, 252.3529155287689321, -3.563159428949892682 ) ) ;
#54211=CARTESIAN_POINT ( 'NONE',  ( 166.4153639104449383, 286.7629316800744164, -4.632910421625811459 ) ) ;
#54213=CARTESIAN_POINT ( 'NONE',  ( 72.76825883208245216, 219.4865022471902876, 10.00000000000009237 ) ) ;
#54215=DIRECTION ( 'NONE',  ( 0.4999999999999992784, -0.8660254037844390407, 0.000000000000000000 ) ) ;
#54216=CARTESIAN_POINT ( 'NONE',  ( 29.16053163240333745, 178.4548013555409796, -4.594050593750042211 ) ) ;
#54219=CARTESIAN_POINT ( 'NONE',  ( 206.4192790749514188, 271.4707676162397547, -6.632096683787595204 ) ) ;
#54220=CARTESIAN_POINT ( 'NONE',  ( 151.1451503555562113, 268.8559155969762742, -15.81507177720227553 ) ) ;
#54222=CARTESIAN_POINT ( 'NONE',  ( 206.9258336080761183, 272.2409381227055292, 6.776000910836894597 ) ) ;
#54224=CARTESIAN_POINT ( 'NONE',  ( 159.8766461922783719, 278.4588112948835601, -9.911155033800223890 ) ) ;
#54225=CARTESIAN_POINT ( 'NONE',  ( 165.8866640751390094, 265.8956478032751534, 17.81115609982314751 ) ) ;
#54230=CARTESIAN_POINT ( 'NONE',  ( 188.4483461232879336, 269.7271065142691668, -14.07674267906546639 ) ) ;
#54231=ORIENTED_EDGE ( 'NONE', *, *, #1627, .T. ) ;
#54235=CARTESIAN_POINT ( 'NONE',  ( 18.47929132879751890, 188.1427522451419350, -10.00000000000009592 ) ) ;
#54238=CARTESIAN_POINT ( 'NONE',  ( 180.3524760431470497, 257.5751156092176188, -7.390589067125090672 ) ) ;
#54239=ORIENTED_EDGE ( 'NONE', *, *, #30478, .F. ) ;
#54240=CYLINDRICAL_SURFACE ( 'NONE', #21188, 10.00000000000010658 ) ;
#54242=ORIENTED_EDGE ( 'NONE', *, *, #62695, .T. ) ;
#54243=CARTESIAN_POINT ( 'NONE',  ( 191.0900422946452011, 299.6693332556258724, 8.872191398975367349 ) ) ;
#54248=CARTESIAN_POINT ( 'NONE',  ( 147.7157269441172218, 274.7958511862549926, 8.036290321896261801 ) ) ;
#54250=CARTESIAN_POINT ( 'NONE',  ( 196.4242782546697015, 290.4301655533025155, -16.42402868779123537 ) ) ;
#54254=CARTESIAN_POINT ( 'NONE',  ( 196.0034224882197975, 291.1591091234520263, 17.53794140922627776 ) ) ;
#54255=CARTESIAN_POINT ( 'NONE',  ( 162.1392933197202808, 266.6552078212308174, 16.85513656058302345 ) ) ;
#54258=CARTESIAN_POINT ( 'NONE',  ( 149.2511585606875428, 272.1364056148075292, 11.40684181024752242 ) ) ;
#54266=CARTESIAN_POINT ( 'NONE',  ( 157.4655681218829670, 259.9086309006383431, -17.75190047967350893 ) ) ;
#54268=EDGE_CURVE ( 'NONE', #32604, #48299, #32283, .T. ) ;
#54271=CARTESIAN_POINT ( 'NONE',  ( -27.42236680055714260, 166.5217562850347406, 1.224646799147364892E-15 ) ) ;
#54272=CARTESIAN_POINT ( 'NONE',  ( 68.64455419991973883, 221.9860189848785410, -2.679491924311252493 ) ) ;
#54273=CARTESIAN_POINT ( 'NONE',  ( 190.2476911738421848, 301.1283281946692796, -1.360079143321618611 ) ) ;
#54274=VERTEX_POINT ( 'NONE', #68661 ) ;
#54275=CARTESIAN_POINT ( 'NONE',  ( 148.9230895364621574, 272.7046378331555161, 12.20434325797056019 ) ) ;
#54276=CARTESIAN_POINT ( 'NONE',  ( 174.0620471294585059, 277.0282672862553000, -15.64145360528607043 ) ) ;
#54277=CARTESIAN_POINT ( 'NONE',  ( 161.8882824960653579, 250.2482648971885340, -13.83574485983625557 ) ) ;
#54278=CARTESIAN_POINT ( 'NONE',  ( 147.2567621633200474, 275.5908015054806128, -3.647191014543873955 ) ) ;
#54279=CARTESIAN_POINT ( 'NONE',  ( 148.9266665119372703, 272.6984423298952152, 12.06339424062075061 ) ) ;
#54281=CYLINDRICAL_SURFACE ( 'NONE', #43414, 10.00000000000010658 ) ;
#54283=CARTESIAN_POINT ( 'NONE',  ( 154.1288763713144192, 264.1723049937594965, -16.63665840739514579 ) ) ;
#54285=CARTESIAN_POINT ( 'NONE',  ( 111.1353355333153843, 222.7202760586659167, -5.415160957724236172E-17 ) ) ;
#54287=CARTESIAN_POINT ( 'NONE',  ( 191.6823192895500370, 298.6434794082964572, -8.424208857102787107 ) ) ;
#54290=CARTESIAN_POINT ( 'NONE',  ( 202.7676489560256528, 279.4431252073101746, -16.04062356091568020 ) ) ;
#54291=CIRCLE ( 'NONE', #34859, 17.82106496071138224 ) ;
#54295=ORIENTED_EDGE ( 'NONE', *, *, #79693, .F. ) ;
#54296=CARTESIAN_POINT ( 'NONE',  ( 208.0421103033489771, 270.3074901711881353, -2.473242163239977476 ) ) ;
#54300=CARTESIAN_POINT ( 'NONE',  ( 48.42933654300939139, 198.7677522451418781, 10.00000000000009592 ) ) ;
#54301=CARTESIAN_POINT ( 'NONE',  ( 133.7059490715647883, 241.8768266524159856, 9.188101187500096856 ) ) ;
#54302=CARTESIAN_POINT ( 'NONE',  ( 198.4344074287054696, 286.9485196940960918, -17.83642855442570152 ) ) ;
#54303=CARTESIAN_POINT ( 'NONE',  ( 114.3892930691446850, 248.3967562850347122, -4.648177544792955347E-16 ) ) ;
#54304=CARTESIAN_POINT ( 'NONE',  ( 187.9181207603909911, 281.6813620558751836, -17.66056584057218259 ) ) ;
#54306=CARTESIAN_POINT ( 'NONE',  ( 44.34243207491050498, 208.6589784336661637, -6.496448406907675876E-16 ) ) ;
#54311=EDGE_CURVE ( 'NONE', #17408, #36668, #15400, .T. ) ;
#54312=CARTESIAN_POINT ( 'NONE',  ( 164.2897805489690768, 249.8104079013010335, 11.36607573508163505 ) ) ;
#54313=CARTESIAN_POINT ( 'NONE',  ( 190.1813752874636805, 301.2431906792259042, -4.710625539811892359 ) ) ;
#54315=CYLINDRICAL_SURFACE ( 'NONE', #55952, 10.00000000000010658 ) ;
#54316=CARTESIAN_POINT ( 'NONE',  ( 180.6243441928988887, 262.2958008669023116, 12.30780204317005655 ) ) ;
#54317=CARTESIAN_POINT ( 'NONE',  ( 104.3601438707543565, 244.3927522451419350, 2.944929066748280225E-16 ) ) ;
#54319=ORIENTED_EDGE ( 'NONE', *, *, #37222, .T. ) ;
#54320=CARTESIAN_POINT ( 'NONE',  ( 148.0389988358468827, 274.2359278451201590, 7.783622668412842671 ) ) ;
#54324=CARTESIAN_POINT ( 'NONE',  ( 36.84650709099022947, 182.8923013555409796, 4.594050593750050204 ) ) ;
#54329=CARTESIAN_POINT ( 'NONE',  ( 176.1992339320817962, 287.1978759562800860, 10.54343790665076419 ) ) ;
#54330=CARTESIAN_POINT ( 'NONE',  ( 68.04987750350953490, 222.3464784336661637, 1.353441290958777327E-15 ) ) ;
#54331=CARTESIAN_POINT ( 'NONE',  ( 200.4116241316243645, 283.5238799070667142, 18.37703770054986663 ) ) ;
#54335=ORIENTED_EDGE ( 'NONE', *, *, #39709, .F. ) ;
#54336=VECTOR ( 'NONE', #4453, 1000.000000000000000 ) ;
#54337=CARTESIAN_POINT ( 'NONE',  ( 36.46736065678477701, 181.8615022471902023, 5.000000000000051514 ) ) ;
#54338=CARTESIAN_POINT ( 'NONE',  ( 208.2555382576270233, 269.9378221106229034, 3.215405476967123199 ) ) ;
#54339=CARTESIAN_POINT ( 'NONE',  ( 140.7960114214023974, 264.3464784336661637, 1.353441290958777327E-15 ) ) ;
#54341=CARTESIAN_POINT ( 'NONE',  ( 167.2515702596184042, 262.0622343731731689, -17.21809106051008342 ) ) ;
#54343=CARTESIAN_POINT ( 'NONE',  ( 187.5228883593873093, 261.4347505834685990, 6.388304628836355192 ) ) ;
#54344=CARTESIAN_POINT ( 'NONE',  ( 164.7462163020046262, 245.2981783406326599, 1.451255823150352064 ) ) ;
#54348=CARTESIAN_POINT ( 'NONE',  ( 191.0900422946452011, 299.6693332556258724, 8.872191398975367349 ) ) ;
#54349=CARTESIAN_POINT ( 'NONE',  ( 177.8882589859629491, 286.4065610622367331, 13.19283280512425094 ) ) ;
#54352=ORIENTED_EDGE ( 'NONE', *, *, #55697, .F. ) ;
#54353=CARTESIAN_POINT ( 'NONE',  ( 160.0613190107378614, 253.4126584773486854, 14.75620464716950764 ) ) ;
#54355=B_SPLINE_CURVE_WITH_KNOTS ( 'NONE', 3,
 ( #72276, #2881, #33778, #64663 ),
 .UNSPECIFIED., .F., .F.,
 ( 4, 4 ),
 ( 0.009427079270958907756, 0.01489411771146553591 ),
 .UNSPECIFIED. ) ;
#54357=CARTESIAN_POINT ( 'NONE',  ( 192.0712386031329686, 297.9698513971258649, 12.12276320360788873 ) ) ;
#54358=CARTESIAN_POINT ( 'NONE',  ( 163.3740049908953438, 249.6749180501957710, -11.76522313559978627 ) ) ;
#54360=CARTESIAN_POINT ( 'NONE',  ( 208.3586375946586315, 269.7592488206576604, -1.970210487958146128 ) ) ;
#54361=CARTESIAN_POINT ( 'NONE',  ( 153.1627746953036535, 265.3612877299463548, -17.72069958822647351 ) ) ;
#54362=ORIENTED_EDGE ( 'NONE', *, *, #69340, .T. ) ;
#54364=CARTESIAN_POINT ( 'NONE',  ( 190.4780531826553442, 281.5641646806880658, 17.56433427958257454 ) ) ;
#54365=CARTESIAN_POINT ( 'NONE',  ( 183.1207986101861138, 294.8225010653632694, -8.165837621905515320 ) ) ;
#54366=ORIENTED_EDGE ( 'NONE', *, *, #91254, .F. ) ;
#54372=CARTESIAN_POINT ( 'NONE',  ( 204.8762144138505903, 275.7909827032724479, 14.60855957933206817 ) ) ;
#54375=CARTESIAN_POINT ( 'NONE',  ( 161.3644539559160478, 251.1555625431813894, 12.97746593258196413 ) ) ;
#54376=CARTESIAN_POINT ( 'NONE',  ( 191.5281967176683509, 298.9104275333885994, 7.715154960566919407 ) ) ;
#54380=EDGE_CURVE ( 'NONE', #49338, #25811, #31807, .T. ) ;
#54382=CARTESIAN_POINT ( 'NONE',  ( 160.1863252117574064, 268.8609356850063250, -17.02858764381097956 ) ) ;
#54383=ORIENTED_EDGE ( 'NONE', *, *, #19669, .T. ) ;
#54387=CARTESIAN_POINT ( 'NONE',  ( 207.8725590214046406, 270.6011616060040410, 1.988011721677743093 ) ) ;
#54392=CARTESIAN_POINT ( 'NONE',  ( 194.1972774922283236, 294.2874440223457100, -15.09915398317898649 ) ) ;
#54396=CARTESIAN_POINT ( 'NONE',  ( 167.0957737472305666, 246.8272050136007749, 1.963998143010642128 ) ) ;
#54399=CARTESIAN_POINT ( 'NONE',  ( 163.4495156451401670, 282.8190555064526279, 8.951327301367555833 ) ) ;
#54401=CARTESIAN_POINT ( 'NONE',  ( 115.4099260042794270, 248.9860189848785126, -2.679491924311252493 ) ) ;
#54404=CARTESIAN_POINT ( 'NONE',  ( 61.92489908531692322, 199.8927522451418213, 10.00000000000009948 ) ) ;
#54405=CARTESIAN_POINT ( 'NONE',  ( 159.2651917302844993, 254.7915913763855258, -16.53922207549818424 ) ) ;
#54406=CARTESIAN_POINT ( 'NONE',  ( 165.6682284193261978, 246.6824036188616560, -2.565596566166696846 ) ) ;
#54408=CARTESIAN_POINT ( 'NONE',  ( 155.3626990048841492, 275.8588059374729369, -11.87708972044752187 ) ) ;
#54409=CARTESIAN_POINT ( 'NONE',  ( 171.0910052398126027, 255.4451962542384535, 11.23270455455271133 ) ) ;
#54410=CARTESIAN_POINT ( 'NONE',  ( 158.0731130136125842, 281.0592270188419093, 2.063127701874739373 ) ) ;
#54411=ORIENTED_EDGE ( 'NONE', *, *, #15583, .F. ) ;
#54412=CARTESIAN_POINT ( 'NONE',  ( 194.1719470998206418, 294.3313175489715263, -14.09883309033929599 ) ) ;
#54413=CARTESIAN_POINT ( 'NONE',  ( 137.2691092145630876, 243.3927522451418497, 10.00000000000009948 ) ) ;
#54415=CARTESIAN_POINT ( 'NONE',  ( 4.262040950002970341, 183.2677522451419065, -5.000000000000047962 ) ) ;
#54416=CARTESIAN_POINT ( 'NONE',  ( 93.00275509369618021, 218.3768266524159856, -9.188101187500093303 ) ) ;
#54417=CARTESIAN_POINT ( 'NONE',  ( 196.1211713645807890, 269.6255699324162833, -11.03082859017656858 ) ) ;
#54419=CARTESIAN_POINT ( 'NONE',  ( 170.2967212533610564, 280.7145836319469367, -13.97955410212758487 ) ) ;
#54420=CARTESIAN_POINT ( 'NONE',  ( 8.774901663922227257, 164.3262482093457777, 3.021315404115420679E-15 ) ) ;
#54421=CARTESIAN_POINT ( 'NONE',  ( 1.284818304444202530, 180.7369531367911293, -4.594050593750048428 ) ) ;
#54422=DIRECTION ( 'NONE',  ( -0.8660254037844387076, -0.4999999999999998890, -0.000000000000000000 ) ) ;
#54423=CARTESIAN_POINT ( 'NONE',  ( 161.8873598795597388, 250.2498629158519350, 13.90822209621415873 ) ) ;
#54424=ORIENTED_EDGE ( 'NONE', *, *, #24576, .T. ) ;
#54426=VERTEX_POINT ( 'NONE', #54266 ) ;
#54428=CARTESIAN_POINT ( 'NONE',  ( 197.6036480476475958, 265.0526450946206865, -2.974152093784073525 ) ) ;
#54432=CARTESIAN_POINT ( 'NONE',  ( 185.6922465440033250, 286.5916479858942694, 15.93746842189364799 ) ) ;
#54434=CARTESIAN_POINT ( 'NONE',  ( 31.29809797828990270, 195.0024278399160949, -9.188101187500093303 ) ) ;
#54435=CARTESIAN_POINT ( 'NONE',  ( 126.9399520566163773, 244.0958772461660544, -9.188101187500095079 ) ) ;
#54436=CARTESIAN_POINT ( 'NONE',  ( 199.4166635728208234, 277.5177111250312123, 15.19222490148100846 ) ) ;
#54438=CARTESIAN_POINT ( 'NONE',  ( 152.5568709919297987, 273.2141159824016086, -11.74195484041754156 ) ) ;
#54439=CARTESIAN_POINT ( 'NONE',  ( 175.0472144265203838, 281.5570299394952372, -15.61366602656669400 ) ) ;
#54443=CARTESIAN_POINT ( 'NONE',  ( 194.5051734451974426, 293.7541525883582381, 14.61790433731063921 ) ) ;
#54444=CARTESIAN_POINT ( 'NONE',  ( 207.4541616930702617, 271.3258470364304458, -6.834942797545373594 ) ) ;
#54445=CARTESIAN_POINT ( 'NONE',  ( 189.6793199455043464, 284.5195100320480606, 16.64680879193300811 ) ) ;
#54446=CARTESIAN_POINT ( 'NONE',  ( 194.1789525331299728, 294.3191837825503967, -15.34533909744314961 ) ) ;
#54447=CARTESIAN_POINT ( 'NONE',  ( 189.3315619462889572, 262.8718067175192914, 7.989062115483674731 ) ) ;
#54448=CARTESIAN_POINT ( 'NONE',  ( 171.0879638105105585, 279.6763734742275460, 13.89733606482576889 ) ) ;
#54449=DIRECTION ( 'NONE',  ( 0.4999999999999992784, -0.8660254037844390407, 0.000000000000000000 ) ) ;
#54451=CARTESIAN_POINT ( 'NONE',  ( 190.1158090214649405, 301.3567547831981983, -1.340987185199551845 ) ) ;
#54453=CARTESIAN_POINT ( 'NONE',  ( 152.3302930170243314, 267.2945999775473638, -15.38153796020247732 ) ) ;
#54456=CARTESIAN_POINT ( 'NONE',  ( 116.3314879560220163, 225.7202760586659736, -5.415160957724236172E-17 ) ) ;
#54458=B_SPLINE_CURVE_WITH_KNOTS ( 'NONE', 3,
 ( #50827, #66536, #90886, #59407 ),
 .UNSPECIFIED., .F., .F.,
 ( 4, 4 ),
 ( 0.01080040790777650125, 0.01647322660403158570 ),
 .UNSPECIFIED. ) ;
#54459=CARTESIAN_POINT ( 'NONE',  ( 190.8443993347725325, 300.0947993426467519, 8.522468760355437212 ) ) ;
#54462=CARTESIAN_POINT ( 'NONE',  ( 195.6701525283530714, 278.3163088474954634, 17.11539662884900537 ) ) ;
#54463=CARTESIAN_POINT ( 'NONE',  ( 191.0207652119315753, 299.7893246826858444, -8.025593426971470379 ) ) ;
#54464=CARTESIAN_POINT ( 'NONE',  ( 191.1041736655189140, 261.3211040730838590, -4.687602006059129245 ) ) ;
#54465=CARTESIAN_POINT ( 'NONE',  ( 149.9090183420942424, 271.7417389411527893, -11.59929054339867349 ) ) ;
#54467=CARTESIAN_POINT ( 'NONE',  ( 179.5344296421649233, 268.6052087499922436, -17.09315547090865905 ) ) ;
#54468=CARTESIAN_POINT ( 'NONE',  ( 164.0651280066704771, 248.4778578725967861, 9.975266483072225299 ) ) ;
#54475=CARTESIAN_POINT ( 'NONE',  ( 149.6564118588553924, 271.4344863124460971, -11.76165597393390172 ) ) ;
#54477=B_SPLINE_SURFACE_WITH_KNOTS ( 'NONE', 3, 1, ( 
 ( #14580, #69262 ),
 ( #45458, #53558 ),
 ( #84510, #15054 ),
 ( #24169, #10991 ),
 ( #9478, #8966 ),
 ( #88037, #63164 ),
 ( #33267, #2901 ),
 ( #40349, #72806 ),
 ( #31744, #71789 ),
 ( #48977, #62648 ),
 ( #94109, #1878 ),
 ( #17568, #95118 ),
 ( #47950, #39836 ),
 ( #41864, #93602 ),
 ( #70766, #87035 ),
 ( #33795, #79913 ),
 ( #48475, #78892 ),
 ( #64679, #24661 ),
 ( #40842, #25160 ),
 ( #25683, #95629 ),
 ( #18585, #80419 ),
 ( #56563, #56043 ),
 ( #55545, #2387 ),
 ( #79417, #9983 ),
 ( #64170, #87549 ),
 ( #18082, #55053 ),
 ( #26177, #86036 ),
 ( #10476, #32262 ),
 ( #41353, #57055 ),
 ( #49464, #72295 ),
 ( #16564, #47460 ),
 ( #78385, #1382 ),
 ( #86529, #17059 ),
 ( #71286, #32760 ) ),
 .UNSPECIFIED., .T., .F., .F.,
 ( 4, 2, 2, 2, 2, 2, 2, 2, 2, 2, 2, 2, 2, 2, 2, 2, 4 ),
 ( 2, 2 ),
 ( 0.000000000000000000, 0.06250000000000000000, 0.1250000000000000000, 0.1875000000000000000, 0.2500000000000000000, 0.3125000000000000000, 0.3750000000000000000, 0.4375000000000000000, 0.5000000000000000000, 0.5625000000000000000, 0.6250000000000000000, 0.6875000000000000000, 0.7500000000000000000, 0.8125000000000000000, 0.8750000000000000000, 0.9375000000000000000, 1.000000000000000000 ),
 ( 0.000000000000000000, 1.000000000000000000 ),
 .UNSPECIFIED. ) ;
#54479=CARTESIAN_POINT ( 'NONE',  ( 182.9889844305354245, 264.4095531704369364, -13.10990340061844073 ) ) ;
#54480=CARTESIAN_POINT ( 'NONE',  ( 165.3207990934748750, 285.3707166551773753, 6.626286169182803221 ) ) ;
#54481=CARTESIAN_POINT ( 'NONE',  ( -13.19378359325312466, 163.1896272461660544, -10.00000000000009592 ) ) ;
#54484=CARTESIAN_POINT ( 'NONE',  ( 189.6749581198630210, 280.2046705077256092, 16.64219758661014126 ) ) ;
#54487=ORIENTED_EDGE ( 'NONE', *, *, #53061, .F. ) ;
#54488=CARTESIAN_POINT ( 'NONE',  ( 176.5752601597114335, 288.5842064133888130, 11.38490813771325350 ) ) ;
#54489=DIRECTION ( 'NONE',  ( -0.8660254037844387076, -0.4999999999999998890, -0.000000000000000000 ) ) ;
#54492=DIRECTION ( 'NONE',  ( 0.4999999999999998335, -0.8660254037844389297, 0.000000000000000000 ) ) ;
#54501=CARTESIAN_POINT ( 'NONE',  ( 165.9903072508455466, 286.3044248736204622, 5.270287258096775673 ) ) ;
#54504=VERTEX_POINT ( 'NONE', #44677 ) ;
#54505=CARTESIAN_POINT ( 'NONE',  ( 169.4836806320240612, 269.1565945087554041, 17.44706958315075340 ) ) ;
#54506=VERTEX_POINT ( 'NONE', #91834 ) ;
#54507=CARTESIAN_POINT ( 'NONE',  ( 165.4895756769140007, 275.0579021241501323, -15.80007132412031368 ) ) ;
#54509=CARTESIAN_POINT ( 'NONE',  ( 147.2720785848982530, 275.5642726851167481, -7.209059498816540845 ) ) ;
#54510=CARTESIAN_POINT ( 'NONE',  ( 190.0445576990143195, 301.4801656937889902, 4.140328216824785912 ) ) ;
#54511=CARTESIAN_POINT ( 'NONE',  ( 147.2658550951450422, 275.5750520855697800, -5.215660180131691526 ) ) ;
#54512=CARTESIAN_POINT ( 'NONE',  ( 167.8763609878610339, 248.7503499377862681, -4.961192906137089409 ) ) ;
#54515=CARTESIAN_POINT ( 'NONE',  ( 178.0456222035626297, 255.4355507755199994, 5.346306856010867747 ) ) ;
#54516=CARTESIAN_POINT ( 'NONE',  ( 121.2293367285889616, 249.9869531367911293, 4.594050593750046652 ) ) ;
#54518=CARTESIAN_POINT ( 'NONE',  ( 160.3128597929971306, 283.6975250075342387, 2.223783518518671176 ) ) ;
#54519=CARTESIAN_POINT ( 'NONE',  ( 180.5790958426250086, 291.5328203877501210, -9.792797898500380072 ) ) ;
#54523=CARTESIAN_POINT ( 'NONE',  ( 177.7757808709156109, 253.3576871789891527, 1.393605394853308699 ) ) ;
#54524=CARTESIAN_POINT ( 'NONE',  ( 173.9708202189197550, 290.6014801153625626, -4.921738911677555173 ) ) ;
#54525=CARTESIAN_POINT ( 'NONE',  ( 157.5710319558766344, 257.7259621817996162, 18.28704422422941533 ) ) ;
#54527=CARTESIAN_POINT ( 'NONE',  ( 152.8651171364917900, 265.8768457450651113, -16.25664868183201861 ) ) ;
#54529=ORIENTED_EDGE ( 'NONE', *, *, #81541, .F. ) ;
#54530=CARTESIAN_POINT ( 'NONE',  ( 194.7295074538898803, 293.3655946874374081, 16.09945624218667959 ) ) ;
#54531=CARTESIAN_POINT ( 'NONE',  ( 174.1271922040128572, 253.6654629759184161, -7.526141489418877839 ) ) ;
#54532=EDGE_LOOP ( 'NONE', ( #18992, #46429, #89760, #72784 ) ) ;
#54533=CARTESIAN_POINT ( 'NONE',  ( 194.5298665426430489, 293.7113828889860656, -16.13302716640051315 ) ) ;
#54537=CARTESIAN_POINT ( 'NONE',  ( 156.8430461297778891, 276.5937385669784021, 10.19580746110867508 ) ) ;
#54538=CARTESIAN_POINT ( 'NONE',  ( 195.7544032369005436, 265.2869026655097855, 4.183226695583321941 ) ) ;
#54539=CARTESIAN_POINT ( 'NONE',  ( 190.0607312434325138, 301.4521522931182176, 3.538147641957853473 ) ) ;
#54541=CARTESIAN_POINT ( 'NONE',  ( 160.3733185927383715, 282.5102941377067509, 6.606729549618552078 ) ) ;
#54542=CARTESIAN_POINT ( 'NONE',  ( 162.9302848195957267, 282.3798764647056032, -6.613031290533573525 ) ) ;
#54545=ORIENTED_EDGE ( 'NONE', *, *, #57496, .F. ) ;
#54548=CARTESIAN_POINT ( 'NONE',  ( 163.9055806673350162, 247.5346603069789921, -7.472254527550087566 ) ) ;
#54549=CARTESIAN_POINT ( 'NONE',  ( 118.1240276194171770, 250.5530062829863311, -4.648177544792955347E-16 ) ) ;
#54550=CARTESIAN_POINT ( 'NONE',  ( 24.47725860691335598, 196.4860189848785126, -2.679491924311252493 ) ) ;
#54551=CARTESIAN_POINT ( 'NONE',  ( 188.2332414194945898, 299.2348910183464454, -3.671804926528876134 ) ) ;
#54552=CARTESIAN_POINT ( 'NONE',  ( 192.3606619183491091, 297.4685555102766443, 10.99569063633359889 ) ) ;
#54553=CARTESIAN_POINT ( 'NONE',  ( 50.57404612423096069, 211.5530062829863027, -4.648177544792955347E-16 ) ) ;
#54555=CARTESIAN_POINT ( 'NONE',  ( 154.9683083969241011, 262.2340116239618055, 18.33261662430134109 ) ) ;
#54556=CARTESIAN_POINT ( 'NONE',  ( 191.3843761966370209, 282.8631020262318430, -17.76976768207862278 ) ) ;
#54558=CARTESIAN_POINT ( 'NONE',  ( 90.72909131299699936, 229.3149278399160949, -9.188101187500095079 ) ) ;
#54560=CARTESIAN_POINT ( 'NONE',  ( 193.1649355862271591, 296.0755126543221536, -12.21556774862162698 ) ) ;
#54562=CARTESIAN_POINT ( 'NONE',  ( 202.7676489560256528, 279.4431252073101746, -16.04062356091568020 ) ) ;
#54565=FACE_OUTER_BOUND ( 'NONE', #58559, .T. ) ;
#54570=CARTESIAN_POINT ( 'NONE',  ( 207.6414258450697616, 271.0014960107308752, 6.436373232459713378 ) ) ;
#54571=CARTESIAN_POINT ( 'NONE',  ( 166.3640306902089492, 249.9463895289820243, -9.022950769094974177 ) ) ;
#54572=CARTESIAN_POINT ( 'NONE',  ( 164.7588300145904441, 245.2763307495621632, -4.895387527856912335 ) ) ;
#54573=CARTESIAN_POINT ( 'NONE',  ( 157.0848929289108469, 258.5679796760466047, 17.57466231005294688 ) ) ;
#54575=EDGE_CURVE ( 'NONE', #45578, #59881, #77614, .T. ) ;
#54576=( BOUNDED_CURVE ( )  B_SPLINE_CURVE ( 2, ( #5983, #83522, #73900, #42958, #43966, #5002, #67277, #97225, #14085 ),
 .UNSPECIFIED., .F., .T. ) 
 B_SPLINE_CURVE_WITH_KNOTS ( ( 3, 2, 2, 2, 3 ),
 ( 0.4395161290322580627, 0.4408602150537634379, 0.4435483870967741882, 0.4462365591397849385, 0.4475806451612903136 ),
 .UNSPECIFIED. ) 
 CURVE ( )  GEOMETRIC_REPRESENTATION_ITEM ( )  RATIONAL_B_SPLINE_CURVE ( ( 0.9330127018922194093, 0.9330127018922194093, 1.000000000000000000, 0.8660254037844387076, 1.000000000000000000, 0.8660254037844387076, 1.000000000000000000, 0.9330127018922194093, 0.9330127018922194093 ) ) 
 REPRESENTATION_ITEM ( '' )  );
#54577=CARTESIAN_POINT ( 'NONE',  ( 35.81758128034870481, 200.6744531367911293, 4.594050593750047540 ) ) ;
#54579=EDGE_CURVE ( 'NONE', #90499, #54274, #25391, .T. ) ;
#54580=CARTESIAN_POINT ( 'NONE',  ( 65.42534541587671981, 199.3923013555409796, 4.594050593750050204 ) ) ;
#54584=CARTESIAN_POINT ( 'NONE',  ( -13.76211276271270556, 162.8615022471902591, -10.00000000000009592 ) ) ;
#54585=CYLINDRICAL_SURFACE ( 'NONE', #91098, 17.82106496071139645 ) ;
#54586=B_SPLINE_CURVE_WITH_KNOTS ( 'NONE', 3,
 ( #95987, #73642, #51313, #58419 ),
 .UNSPECIFIED., .F., .F.,
 ( 4, 4 ),
 ( 0.009149324415700987867, 0.01512556512898982457 ),
 .UNSPECIFIED. ) ;
#54588=CARTESIAN_POINT ( 'NONE',  ( 199.9966929353907972, 271.1012207858159400, -11.25541782042054706 ) ) ;
#54590=CARTESIAN_POINT ( 'NONE',  ( 130.1965684169901181, 252.6427522451419065, -10.00000000000009592 ) ) ;
#54591=CARTESIAN_POINT ( 'NONE',  ( 196.6288634187112052, 290.0758136547079289, -16.31544900032282186 ) ) ;
#54593=CARTESIAN_POINT ( 'NONE',  ( 62.52896555438372417, 219.1589784336661637, -6.496448406907676862E-16 ) ) ;
#54595=CARTESIAN_POINT ( 'NONE',  ( 154.9903553346911735, 262.1958252075976361, -18.39016733948542637 ) ) ;
#54596=CARTESIAN_POINT ( 'NONE',  ( 197.9552487813401456, 287.7784468162186613, 17.26493623863614602 ) ) ;
#54597=CARTESIAN_POINT ( 'NONE',  ( 47.97596991287763757, 210.0530062829863027, 1.101618078115930403E-13 ) ) ;
#54598=CARTESIAN_POINT ( 'NONE',  ( 153.3379181194665080, 265.0579304206846132, 17.59725599559538978 ) ) ;
#54599=( BOUNDED_CURVE ( )  B_SPLINE_CURVE ( 2, ( #84366, #43824, #21061, #91977, #75250, #37223, #28626, #74764, #13453 ),
 .UNSPECIFIED., .F., .T. ) 
 B_SPLINE_CURVE_WITH_KNOTS ( ( 3, 2, 2, 2, 3 ),
 ( 0.1733870967741935609, 0.1747311827956989361, 0.1774193548387096864, 0.1801075268817204367, 0.1814516129032258118 ),
 .UNSPECIFIED. ) 
 CURVE ( )  GEOMETRIC_REPRESENTATION_ITEM ( )  RATIONAL_B_SPLINE_CURVE ( ( 0.9330127018922194093, 0.9330127018922194093, 1.000000000000000000, 0.8660254037844387076, 1.000000000000000000, 0.8660254037844387076, 1.000000000000000000, 0.9330127018922194093, 0.9330127018922194093 ) ) 
 REPRESENTATION_ITEM ( '' )  );
#54601=CARTESIAN_POINT ( 'NONE',  ( 120.5439936075240155, 233.7365022471902307, 10.00000000000009592 ) ) ;
#54602=CARTESIAN_POINT ( 'NONE',  ( 185.9487007927320974, 279.8905167439364732, -17.76757602008028769 ) ) ;
#54603=CARTESIAN_POINT ( 'NONE',  ( 165.0387478276132072, 244.7914988754632191, -2.473354058663827626 ) ) ;
#54608=VERTEX_POINT ( 'NONE', #9196 ) ;
#54609=CARTESIAN_POINT ( 'NONE',  ( 159.9470087484377814, 253.6106496594791508, -16.54933891566789939 ) ) ;
#54610=CARTESIAN_POINT ( 'NONE',  ( 190.1660438660940429, 279.2337011502113455, -16.80628667824917954 ) ) ;
#54611=CARTESIAN_POINT ( 'NONE',  ( -22.42236680055709641, 157.8615022471902591, 0.000000000000000000 ) ) ;
#54613=CARTESIAN_POINT ( 'NONE',  ( 173.5665296885054261, 251.8413114671298558, -0.2508721732096706458 ) ) ;
#54614=ORIENTED_EDGE ( 'NONE', *, *, #78363, .T. ) ;
#54616=CARTESIAN_POINT ( 'NONE',  ( 148.2352135776142177, 273.8960739431854563, -9.245976304249309052 ) ) ;
#54617=CARTESIAN_POINT ( 'NONE',  ( 177.5865089022509551, 268.7852845103913069, 17.37969943402860906 ) ) ;
#54624=EDGE_CURVE ( 'NONE', #81475, #34164, #72139, .T. ) ;
#54626=VERTEX_POINT ( 'NONE', #56279 ) ;
#54627=CARTESIAN_POINT ( 'NONE',  ( 150.5780525126727980, 271.8381578737140103, 12.98431582152410968 ) ) ;
#54629=ORIENTED_EDGE ( 'NONE', *, *, #71819, .F. ) ;
#54630=CARTESIAN_POINT ( 'NONE',  ( 171.7130254469920487, 284.7891961508439067, 10.67702735494407662 ) ) ;
#54634=CARTESIAN_POINT ( 'NONE',  ( 163.1369207721744772, 248.0855599626920593, -11.24692769914530110 ) ) ;
#54635=CARTESIAN_POINT ( 'NONE',  ( 164.3330377059402849, 246.0138246616164110, 7.208046019122525294 ) ) ;
#54636=CARTESIAN_POINT ( 'NONE',  ( 185.3933647707513330, 292.5380661828041866, -10.79500138365868978 ) ) ;
#54637=CARTESIAN_POINT ( 'NONE',  ( 205.4029933437358295, 274.8785748323546159, -13.50815392427034922 ) ) ;
#54638=CARTESIAN_POINT ( 'NONE',  ( 139.2268610206906203, 245.0643266524160140, 9.188101187500095079 ) ) ;
#54640=LINE ( 'NONE', #47060, #42040 ) ;
#54642=CARTESIAN_POINT ( 'NONE',  ( 178.9917773741442204, 257.7053463395453150, 10.09848434317354737 ) ) ;
#54643=CARTESIAN_POINT ( 'NONE',  ( 69.26781250152264136, 219.9869531367911293, 4.594050593750046652 ) ) ;
#54644=VERTEX_POINT ( 'NONE', #72523 ) ;
#54645=CARTESIAN_POINT ( 'NONE',  ( 151.0099717111976076, 269.0900518771037468, 15.84752309685681659 ) ) ;
#54646=CARTESIAN_POINT ( 'NONE',  ( 180.2546767116767228, 254.3082820442907348, 0.6097036191673013139 ) ) ;
#54648=FACE_OUTER_BOUND ( 'NONE', #67765, .T. ) ;
#54650=EDGE_LOOP ( 'NONE', ( #87659, #65883, #41713, #93937, #4825 ) ) ;
#54652=EDGE_CURVE ( 'NONE', #5719, #39984, #52531, .T. ) ;
#54656=CARTESIAN_POINT ( 'NONE',  ( 56.22356517706937495, 193.2677522451418213, -5.000000000000041744 ) ) ;
#54658=CARTESIAN_POINT ( 'NONE',  ( 78.06346978264959091, 222.0024278399160949, -9.188101187500093303 ) ) ;
#54660=AXIS2_PLACEMENT_3D ( 'NONE', #83434, #98627, #68183 ) ;
#54661=ORIENTED_EDGE ( 'NONE', *, *, #46768, .T. ) ;
#54662=CARTESIAN_POINT ( 'NONE',  ( 200.3112178831040922, 283.6977886309012433, -17.53557373623702986 ) ) ;
#54663=ORIENTED_EDGE ( 'NONE', *, *, #92662, .F. ) ;
#54666=CARTESIAN_POINT ( 'NONE',  ( 202.6051175132338926, 273.9538057854381350, -13.19822448684500849 ) ) ;
#54667=FACE_OUTER_BOUND ( 'NONE', #93169, .T. ) ;
#54669=ORIENTED_EDGE ( 'NONE', *, *, #35728, .T. ) ;
#54672=CARTESIAN_POINT ( 'NONE',  ( 147.7355616822484023, 275.2941310105550770, -3.966930963970487056 ) ) ;
#54673=CARTESIAN_POINT ( 'NONE',  ( 200.6985908945154335, 283.0268388936558495, -17.74173253065502820 ) ) ;
#54676=DIRECTION ( 'NONE',  ( 0.4999999999999998890, -0.8660254037844385966, 0.000000000000000000 ) ) ;
#54677=CARTESIAN_POINT ( 'NONE',  ( 76.55480823776410659, 226.5530062829863027, -4.648177544792955347E-16 ) ) ;
#54678=CARTESIAN_POINT ( 'NONE',  ( 21.31191609055701974, 193.1115022471903160, -5.000000000000047962 ) ) ;
#54680=CARTESIAN_POINT ( 'NONE',  ( 187.9004646343075819, 266.2528347880879096, -12.82234703419135968 ) ) ;
#54684=CARTESIAN_POINT ( 'NONE',  ( 168.9909194888004436, 268.4774312744898452, 17.82429104036862100 ) ) ;
#54685=CARTESIAN_POINT ( 'NONE',  ( 162.6937333994314656, 248.8531830095558632, 10.02305144031113926 ) ) ;
#54687=EDGE_CURVE ( 'NONE', #23380, #72513, #28695, .T. ) ;
#54689=CARTESIAN_POINT ( 'NONE',  ( 164.9586510554008782, 244.9302305544571823, -1.717556444319656039 ) ) ;
#54690=CARTESIAN_POINT ( 'NONE',  ( 194.4165969972361552, 293.9075714965812267, 14.23342188338008718 ) ) ;
#54692=CARTESIAN_POINT ( 'NONE',  ( 176.1647493927595178, 285.2037997243469363, -12.30204738051347668 ) ) ;
#54695=CARTESIAN_POINT ( 'NONE',  ( 171.7482759404909700, 274.6702854657700072, 16.24998979151664713 ) ) ;
#54696=CARTESIAN_POINT ( 'NONE',  ( 166.3380819770355856, 286.5636595477255923, -3.292484512480813308 ) ) ;
#54697=CARTESIAN_POINT ( 'NONE',  ( 177.7742028453001240, 274.7292553766789638, -17.79112673411210821 ) ) ;
#54698=CARTESIAN_POINT ( 'NONE',  ( 191.8959889624703408, 262.3180493352597864, 2.955584705640112997 ) ) ;
#54699=CARTESIAN_POINT ( 'NONE',  ( 190.7404869014439726, 298.2747809567102308, -9.591077548819823662 ) ) ;
#54701=CARTESIAN_POINT ( 'NONE',  ( 3.097972219676621730, 184.8464784336661637, 1.353441290958777327E-15 ) ) ;
#54704=EDGE_CURVE ( 'NONE', #89705, #2785, #62887, .T. ) ;
#54706=CARTESIAN_POINT ( 'NONE',  ( 175.1487349639535864, 254.8191230408430954, 9.407919966538676348 ) ) ;
#54707=CARTESIAN_POINT ( 'NONE',  ( 187.4676533354318906, 272.4601757945604845, -16.88503403312462936 ) ) ;
#54708=CARTESIAN_POINT ( 'NONE',  ( -22.42236680055709641, 157.8615022471902591, 0.000000000000000000 ) ) ;
#54709=CARTESIAN_POINT ( 'NONE',  ( 18.36166996137734841, 193.6589784336661637, -6.496448406907676862E-16 ) ) ;
#54713=CARTESIAN_POINT ( 'NONE',  ( 173.6440257905655642, 272.7457858960242447, -16.35518571657235398 ) ) ;
#54715=B_SPLINE_SURFACE_WITH_KNOTS ( 'NONE', 3, 1, ( 
 ( #17385, #72109 ),
 ( #47279, #16882 ),
 ( #94929, #33599 ),
 ( #18406, #41171 ),
 ( #94426, #32074 ),
 ( #9293, #78202 ),
 ( #70581, #2208 ),
 ( #40168, #49296 ),
 ( #1709, #55858 ),
 ( #79242, #48805 ),
 ( #33090, #25489 ),
 ( #55366, #24487 ),
 ( #56878, #1196 ),
 ( #62987, #63488 ),
 ( #40675, #87861 ),
 ( #63986, #86853 ),
 ( #56380, #87378 ),
 ( #17907, #79738 ),
 ( #10298, #2712 ),
 ( #54690, #15699 ),
 ( #31898, #7610 ),
 ( #38996, #69902 ),
 ( #61798, #53694 ),
 ( #47602, #45597 ),
 ( #1017, #46597 ),
 ( #92744, #85153 ),
 ( #77004, #23299 ),
 ( #69414, #62802 ),
 ( #39483, #61304 ),
 ( #47104, #23801 ),
 ( #68903, #92266 ),
 ( #30414, #6625 ),
 ( #38499, #55191 ),
 ( #76528, #14713 ) ),
 .UNSPECIFIED., .T., .F., .F.,
 ( 4, 2, 2, 2, 2, 2, 2, 2, 2, 2, 2, 2, 2, 2, 2, 2, 4 ),
 ( 2, 2 ),
 ( 0.000000000000000000, 0.06250000000000000000, 0.1250000000000000000, 0.1875000000000000000, 0.2500000000000000000, 0.3125000000000000000, 0.3750000000000000000, 0.4375000000000000000, 0.5000000000000000000, 0.5625000000000000000, 0.6250000000000000000, 0.6875000000000000000, 0.7500000000000000000, 0.8125000000000000000, 0.8750000000000000000, 0.9375000000000000000, 1.000000000000000000 ),
 ( 0.000000000000000000, 1.000000000000000000 ),
 .UNSPECIFIED. ) ;
#54718=CARTESIAN_POINT ( 'NONE',  ( 187.6689946892134913, 259.7079214702496870, -0.7711235126620424873 ) ) ;
#54720=CARTESIAN_POINT ( 'NONE',  ( 77.24272341830209143, 208.7365022471902023, -10.00000000000009059 ) ) ;
#54723=CARTESIAN_POINT ( 'NONE',  ( 203.5193203535926330, 270.1419797252951298, 6.025390116349934821 ) ) ;
#54724=CARTESIAN_POINT ( 'NONE',  ( 29.78290061743214423, 181.8768266524160140, 9.188101187500098632 ) ) ;
#54726=CARTESIAN_POINT ( 'NONE',  ( 124.8976233183423972, 254.4637435831425023, 2.679491924311251605 ) ) ;
#54727=CARTESIAN_POINT ( 'NONE',  ( 203.0311039195969443, 269.9456838946036328, -6.239233117507705373 ) ) ;
#54728=CARTESIAN_POINT ( 'NONE',  ( 150.9363692955544991, 269.2175350005573478, -14.27857383982596140 ) ) ;
#54731=CARTESIAN_POINT ( 'NONE',  ( 159.8617658264064119, 278.4604067758004931, -10.61854734195418537 ) ) ;
#54732=CARTESIAN_POINT ( 'NONE',  ( 207.3988330342936877, 270.8564699888902396, -1.301389719878858875 ) ) ;
#54734=CARTESIAN_POINT ( 'NONE',  ( 163.1332433029523372, 248.0919295262283981, 11.24052392390482957 ) ) ;
#54736=CARTESIAN_POINT ( 'NONE',  ( 188.7811494455037860, 270.3288468973258887, -14.97842902622537231 ) ) ;
#54739=FACE_OUTER_BOUND ( 'NONE', #40680, .T. ) ;
#54751=CYLINDRICAL_SURFACE ( 'NONE', #63317, 17.82106496071139645 ) ;
#54754=CARTESIAN_POINT ( 'NONE',  ( 153.4495116231415750, 264.8646448025247082, -16.73555355292144498 ) ) ;
#54759=CARTESIAN_POINT ( 'NONE',  ( 147.6088797830324779, 274.9809158978982850, 8.531536684623960198 ) ) ;
#54760=ADVANCED_FACE ( 'NONE', ( #56158 ), #16675, .T. ) ;
#54762=EDGE_CURVE ( 'NONE', #8176, #90906, #66128, .T. ) ;
#54764=CARTESIAN_POINT ( 'NONE',  ( 180.4468251236610854, 287.2605667330827828, -13.89116134381312584 ) ) ;
#54766=ORIENTED_EDGE ( 'NONE', *, *, #97037, .T. ) ;
#54767=CARTESIAN_POINT ( 'NONE',  ( 157.2744851780909414, 258.2395962677452985, 18.17792129701959070 ) ) ;
#54769=ADVANCED_FACE ( 'NONE', ( #70371 ), #80518, .F. ) ;
#54770=CARTESIAN_POINT ( 'NONE',  ( 174.3697573357644899, 277.1653490889620457, -17.12727634137145571 ) ) ;
#54774=CARTESIAN_POINT ( 'NONE',  ( 159.2303255284352304, 254.8519814094557603, 16.39103317446447150 ) ) ;
#54775=CARTESIAN_POINT ( 'NONE',  ( 191.4282440714642917, 263.9101566603287665, -9.496572910043623139 ) ) ;
#54776=EDGE_CURVE ( 'NONE', #34725, #83448, #51054, .T. ) ;
#54777=CARTESIAN_POINT ( 'NONE',  ( 64.91088251055593616, 208.2833772461660544, -9.188101187500095079 ) ) ;
#54782=CARTESIAN_POINT ( 'NONE',  ( 102.5559242795368391, 220.0177522451417929, 5.000000000000051514 ) ) ;
#54788=CARTESIAN_POINT ( 'NONE',  ( 147.7157269441172218, 274.7958511862549926, 8.036290321896261801 ) ) ;
#54789=ORIENTED_EDGE ( 'NONE', *, *, #19895, .T. ) ;
#54790=CARTESIAN_POINT ( 'NONE',  ( 149.6700657135140489, 271.4108371424580355, 12.58635654151485284 ) ) ;
#54791=CARTESIAN_POINT ( 'NONE',  ( 172.7859815943955084, 252.0003099901749692, 7.695973030949746274 ) ) ;
#54792=CARTESIAN_POINT ( 'NONE',  ( 84.11911179316838627, 207.8262482093457777, 3.021315404115420679E-15 ) ) ;
#54793=CARTESIAN_POINT ( 'NONE',  ( 193.0065576635309412, 296.3498312632291913, -11.90044991639595295 ) ) ;
#54794=B_SPLINE_CURVE_WITH_KNOTS ( 'NONE', 3,
 ( #64906, #62891, #57286, #18312 ),
 .UNSPECIFIED., .F., .F.,
 ( 4, 4 ),
 ( 0.008648408712914583060, 0.01500284571837401729 ),
 .UNSPECIFIED. ) ;
#54799=CARTESIAN_POINT ( 'NONE',  ( 184.6885808911535207, 260.6528513612950064, 10.31057805081157852 ) ) ;
#54800=CARTESIAN_POINT ( 'NONE',  ( 200.3804403721752578, 281.5778917628034606, 17.30444700233937994 ) ) ;
#54803=CARTESIAN_POINT ( 'NONE',  ( 118.9295641673753181, 227.2202760586659736, -5.415160957724236172E-17 ) ) ;
#54804=ORIENTED_EDGE ( 'NONE', *, *, #75707, .F. ) ;
#54805=CARTESIAN_POINT ( 'NONE',  ( 147.2405539530007559, 275.6188749492528132, 0.4306668706573002492 ) ) ;
#54808=CARTESIAN_POINT ( 'NONE',  ( 202.8874463667715133, 279.2356300052831557, -15.29930322226033468 ) ) ;
#54809=CARTESIAN_POINT ( 'NONE',  ( 192.5726205457860942, 296.4466972196345296, 11.71797434446428987 ) ) ;
#54811=CARTESIAN_POINT ( 'NONE',  ( 165.3840372259151366, 283.6698659644395093, -8.347863386361117577 ) ) ;
#54813=CARTESIAN_POINT ( 'NONE',  ( 162.6257765080958677, 248.9708877980734485, -10.42859054881151160 ) ) ;
#54815=CARTESIAN_POINT ( 'NONE',  ( 205.8477028968504783, 272.4695280978870073, 9.472321179085877674 ) ) ;
#54816=CARTESIAN_POINT ( 'NONE',  ( 151.0801312611820890, 268.9685319718947198, -15.83903210480701240 ) ) ;
#54817=CARTESIAN_POINT ( 'NONE',  ( 185.8848700110949039, 296.7474278773313472, 4.608973075700647293 ) ) ;
#54818=CARTESIAN_POINT ( 'NONE',  ( 177.9552638626009298, 260.7378092407702184, -13.94576028113082877 ) ) ;
#54820=CARTESIAN_POINT ( 'NONE',  ( 48.45674693441662129, 186.5327760586659451, 1.948934522072303157E-15 ) ) ;
#54821=CARTESIAN_POINT ( 'NONE',  ( 164.9335952247126045, 244.9736285262353306, -1.661461410667423255 ) ) ;
#54822=ORIENTED_EDGE ( 'NONE', *, *, #45199, .F. ) ;
#54826=CARTESIAN_POINT ( 'NONE',  ( 174.1447466443229359, 262.0166869877857607, 14.36471543667183681 ) ) ;
#54828=CARTESIAN_POINT ( 'NONE',  ( 203.1705638993064156, 278.7452560544191442, -15.08126533799095093 ) ) ;
#54829=CARTESIAN_POINT ( 'NONE',  ( 154.3368938251639406, 269.3942069059096411, -15.13873655495052262 ) ) ;
#54830=CARTESIAN_POINT ( 'NONE',  ( 102.9889369814290347, 230.2677522451418497, 10.00000000000009592 ) ) ;
#54835=CARTESIAN_POINT ( 'NONE',  ( 163.0171530587457767, 248.2930037274571191, 9.677214176418313940 ) ) ;
#54838=CARTESIAN_POINT ( 'NONE',  ( 19.17374232530777078, 188.0024278399161233, 9.188101187500095079 ) ) ;
#54845=CARTESIAN_POINT ( 'NONE',  ( 70.26924114858965709, 217.5024278399160664, -9.188101187500093303 ) ) ;
#54846=CARTESIAN_POINT ( 'NONE',  ( 208.1757572214753793, 270.0760069187178374, 2.172546422564154867 ) ) ;
#54848=CARTESIAN_POINT ( 'NONE',  ( 184.1672717435397431, 256.7531923835571774, 1.415796120779537093 ) ) ;
#54849=EDGE_CURVE ( 'NONE', #34337, #29477, #98814, .T. ) ;
#54852=EDGE_LOOP ( 'NONE', ( #49154, #64268, #70241, #38550 ) ) ;
#54855=CARTESIAN_POINT ( 'NONE',  ( 165.4802685333492320, 269.3555218720375137, 17.18790657701241642 ) ) ;
#54856=CARTESIAN_POINT ( 'NONE',  ( 34.30229714732364954, 190.6115022471902591, 10.00000000000009592 ) ) ;
#54859=CARTESIAN_POINT ( 'NONE',  ( -15.79203335248894469, 167.8149278399160949, -9.188101187500095079 ) ) ;
#54861=CARTESIAN_POINT ( 'NONE',  ( 200.3283417415170220, 283.2787895630095250, 16.79050732642456012 ) ) ;
#54862=CARTESIAN_POINT ( 'NONE',  ( 189.2791439001235290, 261.6176991415632642, 6.688689801143334002 ) ) ;
#54863=CARTESIAN_POINT ( 'NONE',  ( 164.6869624841032191, 245.4008089637804346, 1.435659848726088317 ) ) ;
#54869=CARTESIAN_POINT ( 'NONE',  ( 172.8705364283385961, 268.5860898973321014, -17.62214513231522872 ) ) ;
#54872=CARTESIAN_POINT ( 'NONE',  ( 165.8564336512527291, 246.0288987632202407, -1.146165424362591612 ) ) ;
#54874=DIRECTION ( 'NONE',  ( 0.4999999999999992784, -0.8660254037844390407, 0.000000000000000000 ) ) ;
#54877=DIRECTION ( 'NONE',  ( -0.8660254037844387076, -0.4999999999999998890, -0.000000000000000000 ) ) ;
#54878=CARTESIAN_POINT ( 'NONE',  ( 207.5886452961740076, 271.0929146030698007, -1.661373005306138184 ) ) ;
#54879=CARTESIAN_POINT ( 'NONE',  ( 152.7729059155601021, 266.0365602647466972, -17.50667083025758686 ) ) ;
#54881=EDGE_LOOP ( 'NONE', ( #31594, #21309, #7238, #97552, #6881 ) ) ;
#54883=CARTESIAN_POINT ( 'NONE',  ( 130.4311169673963207, 256.1115022471902876, -5.000000000000047962 ) ) ;
#54885=ORIENTED_EDGE ( 'NONE', *, *, #74606, .T. ) ;
#54887=CARTESIAN_POINT ( 'NONE',  ( 203.4435754520237651, 276.2723861740593634, 14.48166091637323483 ) ) ;
#54892=CARTESIAN_POINT ( 'NONE',  ( 186.3211539507438772, 284.5818887155355696, -17.00132214566409417 ) ) ;
#54895=CARTESIAN_POINT ( 'NONE',  ( 161.3227470381586102, 251.2278010437646856, 14.45097375514160731 ) ) ;
#54897=CARTESIAN_POINT ( 'NONE',  ( 190.8001679306945277, 300.1714103817999444, 7.815449226872675403 ) ) ;
#54900=ADVANCED_FACE ( 'NONE', ( #92596 ), #21671, .T. ) ;
#54903=CARTESIAN_POINT ( 'NONE',  ( 160.3325118702422571, 268.9022058081687874, -16.89581317083065315 ) ) ;
#54907=CARTESIAN_POINT ( 'NONE',  ( 164.3602934812760452, 245.9666162739349318, -7.171958108566009571 ) ) ;
#54908=( BOUNDED_CURVE ( )  B_SPLINE_CURVE ( 2, ( #42881, #72846, #66217, #58590, #73817, #11535, #97637, #42395, #50997 ),
 .UNSPECIFIED., .F., .T. ) 
 B_SPLINE_CURVE_WITH_KNOTS ( ( 3, 2, 2, 2, 3 ),
 ( 0.8991935483870967527, 0.9005376344086021279, 0.9032258064516128782, 0.9059139784946236285, 0.9072580645161290036 ),
 .UNSPECIFIED. ) 
 CURVE ( )  GEOMETRIC_REPRESENTATION_ITEM ( )  RATIONAL_B_SPLINE_CURVE ( ( 0.9330127018922194093, 0.9330127018922194093, 1.000000000000000000, 0.8660254037844387076, 1.000000000000000000, 0.8660254037844387076, 1.000000000000000000, 0.9330127018922194093, 0.9330127018922194093 ) ) 
 REPRESENTATION_ITEM ( '' )  );
#54910=CARTESIAN_POINT ( 'NONE',  ( 165.2222719793527972, 271.1331909122671959, 17.05175473187279778 ) ) ;
#54911=CARTESIAN_POINT ( 'NONE',  ( 170.9894191764510083, 283.3192944120900734, 12.01118185074416012 ) ) ;
#54912=CARTESIAN_POINT ( 'NONE',  ( 194.2389208611690492, 294.2153155915419802, -15.75132567904764791 ) ) ;
#54915=CARTESIAN_POINT ( 'NONE',  ( 159.0092078971553633, 255.2349683812814476, -17.41003440661054213 ) ) ;
#54918=CARTESIAN_POINT ( 'NONE',  ( 198.3474120736350983, 277.3537790377902752, -15.33034485771529098 ) ) ;
#54919=CARTESIAN_POINT ( 'NONE',  ( 187.6777693585253814, 293.2028220897474853, -13.03854654741220997 ) ) ;
#54921=CARTESIAN_POINT ( 'NONE',  ( 206.9949618004799561, 271.7276603789779870, 5.520981849004880537 ) ) ;
#54922=ORIENTED_EDGE ( 'NONE', *, *, #21173, .F. ) ;
#54923=CARTESIAN_POINT ( 'NONE',  ( 146.6887764566487533, 276.5745816074078789, -3.628288772073474888 ) ) ;
#54924=CARTESIAN_POINT ( 'NONE',  ( 179.6160012257981862, 295.0481727651569486, 1.085779272287555663 ) ) ;
#54925=CARTESIAN_POINT ( 'NONE',  ( 206.0946696452135427, 273.6805563358039421, -10.19627505985792837 ) ) ;
#54928=CARTESIAN_POINT ( 'NONE',  ( 200.1662314894802819, 283.9489124310637180, 17.19420058542677054 ) ) ;
#54929=CARTESIAN_POINT ( 'NONE',  ( 190.9055077653416674, 262.0587109976776219, -0.7351936343916617433 ) ) ;
#54932=CARTESIAN_POINT ( 'NONE',  ( 194.3072059070401849, 294.0970424226961768, -15.66788609332525617 ) ) ;
#54935=EDGE_CURVE ( 'NONE', #35157, #61620, #69252, .T. ) ;
#54936=CARTESIAN_POINT ( 'NONE',  ( 19.85049821812286908, 192.2677522451419350, -5.000000000000047962 ) ) ;
#54937=CARTESIAN_POINT ( 'NONE',  ( 92.13672968991174628, 217.8768266524160140, 9.188101187500096856 ) ) ;
#54938=CARTESIAN_POINT ( 'NONE',  ( 196.1696074310564200, 269.5488462819374718, -11.79737468409024892 ) ) ;
#54941=CARTESIAN_POINT ( 'NONE',  ( 13.92363686274711299, 178.8458772461660544, 9.188101187500095079 ) ) ;
#54944=CARTESIAN_POINT ( 'NONE',  ( 161.3644539559160478, 251.1555625431813894, 12.97746593258196413 ) ) ;
#54948=CARTESIAN_POINT ( 'NONE',  ( 201.1151172693584783, 267.4386146601190717, -3.692085840245449724 ) ) ;
#54951=CARTESIAN_POINT ( 'NONE',  ( 161.1492466472929266, 251.5283125358769212, -13.33353587056634915 ) ) ;
#54954=CARTESIAN_POINT ( 'NONE',  ( 32.78649236710315762, 198.9244531367911293, -4.594050593750046652 ) ) ;
#54958=CARTESIAN_POINT ( 'NONE',  ( -13.55913805958770624, 162.9786897466781852, -9.594050593750095501 ) ) ;
#54960=DIRECTION ( 'NONE',  ( -0.8660254037844387076, -0.4999999999999998890, -0.000000000000000000 ) ) ;
#54962=CARTESIAN_POINT ( 'NONE',  ( 189.0920916512246208, 280.9571135833196536, -17.80812859110469404 ) ) ;
#54964=CARTESIAN_POINT ( 'NONE',  ( 148.0637215040603394, 274.1931069276759558, -7.795633835291665648 ) ) ;
#54965=CARTESIAN_POINT ( 'NONE',  ( 191.6817669736708467, 264.6815271297149366, 7.777474833780424923 ) ) ;
#54966=CARTESIAN_POINT ( 'NONE',  ( 164.7171516385412815, 249.8514189067689131, -10.51224052795927300 ) ) ;
#54967=CARTESIAN_POINT ( 'NONE',  ( 18.26047324907200675, 192.8967562850347122, -4.648177544792955347E-16 ) ) ;
#54969=CARTESIAN_POINT ( 'NONE',  ( 147.0660117096331874, 275.9211909828330249, -0.7354350123930680772 ) ) ;
#54970=CARTESIAN_POINT ( 'NONE',  ( 147.6300909839706321, 274.9441770201837585, 8.328755691084779755 ) ) ;
#54971=CARTESIAN_POINT ( 'NONE',  ( 181.2305971022323661, 265.9781236237157032, -15.82518789413146010 ) ) ;
#54972=VERTEX_POINT ( 'NONE', #75894 ) ;
#54973=B_SPLINE_CURVE_WITH_KNOTS ( 'NONE', 3,
 ( #16398, #54892, #31088, #56766 ),
 .UNSPECIFIED., .F., .F.,
 ( 4, 4 ),
 ( 0.008151151042490834345, 0.01635116468880294660 ),
 .UNSPECIFIED. ) ;
#54975=EDGE_CURVE ( 'NONE', #84992, #86705, #94002, .T. ) ;
#54976=CARTESIAN_POINT ( 'NONE',  ( 161.4289481915915587, 251.7506084730134432, -13.50114579149946259 ) ) ;
#54977=CARTESIAN_POINT ( 'NONE',  ( 119.9849458542963561, 230.8923013555409796, 4.594050593750050204 ) ) ;
#54979=CARTESIAN_POINT ( 'NONE',  ( -11.16403655135938955, 164.3615022471902591, -10.00000000000009592 ) ) ;
#54982=CARTESIAN_POINT ( 'NONE',  ( 191.6453933565204295, 276.9075887682292887, 17.07476665461427245 ) ) ;
#54983=CARTESIAN_POINT ( 'NONE',  ( 191.2547573475860361, 299.3840384151609442, -6.665042208860675110 ) ) ;
#54986=CARTESIAN_POINT ( 'NONE',  ( 177.2783070499642406, 266.6479886748795707, -16.91666554439952108 ) ) ;
#54987=CARTESIAN_POINT ( 'NONE',  ( 146.8574506849497538, 276.2824292740633041, -4.888313306692038118 ) ) ;
#54989=ORIENTED_EDGE ( 'NONE', *, *, #7592, .T. ) ;
#54990=CARTESIAN_POINT ( 'NONE',  ( 192.6608248749084851, 267.1914924341284063, 11.10020417146784588 ) ) ;
#54991=CARTESIAN_POINT ( 'NONE',  ( 178.7256942771215051, 280.7533503143234270, 16.50221326603510263 ) ) ;
#54993=CARTESIAN_POINT ( 'NONE',  ( 179.9209375999747351, 276.5811748711908535, 17.74520275588677265 ) ) ;
#54994=CARTESIAN_POINT ( 'NONE',  ( 180.4746716150172574, 261.7121554277162545, -13.47270644325290156 ) ) ;
#54995=CARTESIAN_POINT ( 'NONE',  ( 162.7020145476934090, 284.0983276010327359, 6.051621772638641872 ) ) ;
#54997=CARTESIAN_POINT ( 'NONE',  ( 192.1640094933931096, 297.8091675017319062, 12.36911124822534447 ) ) ;
#54998=ORIENTED_EDGE ( 'NONE', *, *, #18403, .F. ) ;
#54999=EDGE_CURVE ( 'NONE', #97286, #71770, #96305, .T. ) ;
#55001=B_SPLINE_SURFACE_WITH_KNOTS ( 'NONE', 3, 1, ( 
 ( #43166, #67478 ),
 ( #90837, #52275 ),
 ( #98404, #74620 ),
 ( #66976, #97903 ),
 ( #59871, #67980 ),
 ( #59359, #33739 ),
 ( #90335, #48930 ),
 ( #64632, #13309 ),
 ( #5682, #44658 ),
 ( #83215, #57008 ),
 ( #87988, #98900 ),
 ( #95585, #18537 ),
 ( #20912, #13780 ),
 ( #82738, #87503 ),
 ( #29482, #44168 ),
 ( #79868, #49420 ),
 ( #72244, #80366 ),
 ( #4701, #75104 ),
 ( #45656, #46666 ),
 ( #68965, #61365 ),
 ( #1081, #16269 ),
 ( #15253, #76109 ),
 ( #60355, #84713 ),
 ( #6683, #52760 ),
 ( #37559, #69961 ),
 ( #576, #99888 ),
 ( #68468, #92805 ),
 ( #39049, #92321 ),
 ( #54243, #30472 ),
 ( #84, #77067 ),
 ( #69470, #22374 ),
 ( #22869, #46150 ),
 ( #31460, #8675 ),
 ( #7165, #99396 ) ),
 .UNSPECIFIED., .T., .F., .F.,
 ( 4, 2, 2, 2, 2, 2, 2, 2, 2, 2, 2, 2, 2, 2, 2, 2, 4 ),
 ( 2, 2 ),
 ( 0.000000000000000000, 0.06250000000000000000, 0.1250000000000000000, 0.1875000000000000000, 0.2500000000000000000, 0.3125000000000000000, 0.3750000000000000000, 0.4375000000000000000, 0.5000000000000000000, 0.5625000000000000000, 0.6250000000000000000, 0.6875000000000000000, 0.7500000000000000000, 0.8125000000000000000, 0.8750000000000000000, 0.9375000000000000000, 1.000000000000000000 ),
 ( 0.000000000000000000, 1.000000000000000000 ),
 .UNSPECIFIED. ) ;
#55003=VERTEX_POINT ( 'NONE', #60637 ) ;
#55004=CARTESIAN_POINT ( 'NONE',  ( 166.0902728679650693, 248.8705385957478882, 7.015670575385891894 ) ) ;
#55009=LINE ( 'NONE', #10937, #26580 ) ;
#55010=CARTESIAN_POINT ( 'NONE',  ( 163.7010375032499212, 247.1084811230698506, 6.649922295230481950 ) ) ;
#55014=ORIENTED_EDGE ( 'NONE', *, *, #30294, .F. ) ;
#55023=CARTESIAN_POINT ( 'NONE',  ( 190.3455805766996605, 300.1776048065829059, -3.435469494870868612 ) ) ;
#55024=CARTESIAN_POINT ( 'NONE',  ( 164.2960764465929060, 246.0778434407177713, -1.520364048796653877 ) ) ;
#55025=CARTESIAN_POINT ( 'NONE',  ( 147.5030091739506588, 275.1642891718561259, -5.824350960008994882 ) ) ;
#55028=CARTESIAN_POINT ( 'NONE',  ( 167.6432305260580051, 249.2069326997503538, -5.439418313667148119 ) ) ;
#55030=CARTESIAN_POINT ( 'NONE',  ( 157.7427020192611451, 281.4113889458213862, 2.901906572848928167 ) ) ;
#55031=CARTESIAN_POINT ( 'NONE',  ( 125.3701074643745841, 249.3149278399160949, 9.188101187500093303 ) ) ;
#55039=CARTESIAN_POINT ( 'NONE',  ( 178.8222888093016820, 253.5684133990675946, 1.420763099363733906 ) ) ;
#55041=CARTESIAN_POINT ( 'NONE',  ( 147.0770520072680654, 275.9020686263983180, 2.568669615083420954 ) ) ;
#55044=CARTESIAN_POINT ( 'NONE',  ( 171.3910097907696013, 265.7400108419894309, -17.48696717007155144 ) ) ;
#55045=CARTESIAN_POINT ( 'NONE',  ( 174.7976338077968421, 282.4145131704060532, 14.70753238353839265 ) ) ;
#55048=CARTESIAN_POINT ( 'NONE',  ( 200.5783178365889796, 282.7758977645278264, -16.72421819799698639 ) ) ;
#55049=CARTESIAN_POINT ( 'NONE',  ( 152.8311844419622503, 273.8830713642822730, 12.16002972492639422 ) ) ;
#55050=ORIENTED_EDGE ( 'NONE', *, *, #48498, .F. ) ;
#55052=CARTESIAN_POINT ( 'NONE',  ( 160.2823167370213184, 279.0841748587739630, 10.63415498209442589 ) ) ;
#55053=CARTESIAN_POINT ( 'NONE',  ( 151.7203664365511031, 267.8596121193626232, -16.04302167993712658 ) ) ;
#55055=CARTESIAN_POINT ( 'NONE',  ( 199.3359313799735162, 277.8054090533971134, 16.38672730308284997 ) ) ;
#55056=CARTESIAN_POINT ( 'NONE',  ( 162.2513340404218241, 281.9508718976948103, -6.600334769067247365 ) ) ;
#55057=CARTESIAN_POINT ( 'NONE',  ( 154.7665789146825830, 277.6802373535633137, -9.031277582128581116 ) ) ;
#55059=ORIENTED_EDGE ( 'NONE', *, *, #3900, .F. ) ;
#55060=CARTESIAN_POINT ( 'NONE',  ( 190.3625087333586521, 300.9294583479858147, -4.271886578030237303 ) ) ;
#55061=CARTESIAN_POINT ( 'NONE',  ( 163.5341610023646126, 247.8889313856435876, -8.119019177482972083 ) ) ;
#55062=CARTESIAN_POINT ( 'NONE',  ( 190.2895893073217337, 274.5542638304875140, -15.68163590285366205 ) ) ;
#55064=CARTESIAN_POINT ( 'NONE',  ( 168.9579038699606315, 279.3139280689009070, 15.08363371378442608 ) ) ;
#55065=CARTESIAN_POINT ( 'NONE',  ( 200.1778674013334012, 279.3308388275589778, -16.74461585440090161 ) ) ;
#55069=FACE_OUTER_BOUND ( 'NONE', #67966, .T. ) ;
#55070=CARTESIAN_POINT ( 'NONE',  ( -16.57695564860984661, 170.4244531367911293, -4.594050593750046652 ) ) ;
#55071=CARTESIAN_POINT ( 'NONE',  ( 93.16496130902324069, 224.5958772461660260, -9.188101187500095079 ) ) ;
#55072=CARTESIAN_POINT ( 'NONE',  ( 203.3684377202211522, 278.4025285431072803, -16.56116267537666076 ) ) ;
#55073=CARTESIAN_POINT ( 'NONE',  ( 147.0456760057551833, 275.9564134551570760, -3.678503029046952033 ) ) ;
#55074=CARTESIAN_POINT ( 'NONE',  ( 182.9399940311841135, 294.6164125958089812, -8.120217072990003615 ) ) ;
#55075=CARTESIAN_POINT ( 'NONE',  ( 155.0453531195792038, 262.1005662498678817, -18.46987289964740953 ) ) ;
#55081=CARTESIAN_POINT ( 'NONE',  ( 207.8404471368518216, 270.6567810215766485, 6.233406202017039099 ) ) ;
#55082=CARTESIAN_POINT ( 'NONE',  ( 166.1201540932435705, 249.6576623637213004, -9.102047968603363515 ) ) ;
#55083=CARTESIAN_POINT ( 'NONE',  ( 161.3351705126590332, 251.7324723637383670, 13.41138257763892305 ) ) ;
#55085=CARTESIAN_POINT ( 'NONE',  ( 157.8360072705708603, 257.2670114739976839, 17.12122855844125269 ) ) ;
#55088=CARTESIAN_POINT ( 'NONE',  ( 40.98727782677583065, 182.2202760586659451, -5.415160957724236172E-17 ) ) ;
#55090=CARTESIAN_POINT ( 'NONE',  ( 64.74867629522887569, 202.0643266524159856, -9.188101187500093303 ) ) ;
#55093=CARTESIAN_POINT ( 'NONE',  ( 167.2881153130185794, 259.8033680499513594, 16.14645104202834602 ) ) ;
#55094=CARTESIAN_POINT ( 'NONE',  ( 138.3604885211411499, 256.8149278399160949, 9.188101187500093303 ) ) ;
#55097=CARTESIAN_POINT ( 'NONE',  ( 200.2305960855333353, 271.0184197120956355, -11.41732784617588692 ) ) ;
#55099=CARTESIAN_POINT ( 'NONE',  ( 150.9003228897357189, 269.2799692068659283, -14.30003212299500781 ) ) ;
#55100=CARTESIAN_POINT ( 'NONE',  ( 196.4808189786114951, 290.3322341467384717, -17.84817245450773271 ) ) ;
#55102=CARTESIAN_POINT ( 'NONE',  ( 52.13666070897046012, 213.1589784336661637, -6.496448406907676862E-16 ) ) ;
#55104=CARTESIAN_POINT ( 'NONE',  ( 155.1601726304954809, 261.9016930232608615, -18.56587418422714464 ) ) ;
#55105=CARTESIAN_POINT ( 'NONE',  ( 159.9880386575927957, 253.5395837721924863, 15.85893018594752846 ) ) ;
#55107=CARTESIAN_POINT ( 'NONE',  ( 201.7940041625137724, 281.1295274581978560, 16.26334312466084953 ) ) ;
#55108=CARTESIAN_POINT ( 'NONE',  ( 107.0484310652165192, 232.6115022471902307, 10.00000000000009592 ) ) ;
#55110=CARTESIAN_POINT ( 'NONE',  ( 207.6826438088389750, 270.9301044032979462, 7.252082088659585146 ) ) ;
#55111=ORIENTED_EDGE ( 'NONE', *, *, #5774, .F. ) ;
#55113=CARTESIAN_POINT ( 'NONE',  ( 186.9334442694681684, 272.7010231022609332, 15.66575838895225736 ) ) ;
#55115=CARTESIAN_POINT ( 'NONE',  ( 159.5221561062548972, 254.3465160214695118, -16.91023001054109542 ) ) ;
#55116=CARTESIAN_POINT ( 'NONE',  ( 187.1232320155474156, 276.7967530242608518, -16.86548313267018528 ) ) ;
#55119=CARTESIAN_POINT ( 'NONE',  ( 177.2864851724368123, 253.0591412921742176, -0.2646061339184051509 ) ) ;
#55122=CARTESIAN_POINT ( 'NONE',  ( 194.9819925439454664, 292.9282776833073285, -15.33279721168237586 ) ) ;
#55123=CARTESIAN_POINT ( 'NONE',  ( 148.6500818154487433, 275.1775010768142238, 7.719411301773694944 ) ) ;
#55126=CARTESIAN_POINT ( 'NONE',  ( 155.4246291545472616, 271.4210554887007447, -15.13027500041984830 ) ) ;
#55129=CARTESIAN_POINT ( 'NONE',  ( 130.8641296692885305, 256.3615022471903444, 5.000000000000046185 ) ) ;
#55130=CARTESIAN_POINT ( 'NONE',  ( 163.6530677658052753, 285.1143415345633230, 4.800695543634067697 ) ) ;
#55132=AXIS2_PLACEMENT_3D ( 'NONE', #89825, #57382, #49788 ) ;
#55137=CARTESIAN_POINT ( 'NONE',  ( 166.9078262434662747, 265.1710354609668912, -17.73982523066521821 ) ) ;
#55138=CARTESIAN_POINT ( 'NONE',  ( 193.7901930790854976, 294.9925349088783264, 14.24765323155741115 ) ) ;
#55140=CARTESIAN_POINT ( 'NONE',  ( 205.2941531242069857, 275.0670916224857478, -13.92605142593109058 ) ) ;
#55141=FACE_OUTER_BOUND ( 'NONE', #49346, .T. ) ;
#55143=CARTESIAN_POINT ( 'NONE',  ( 182.1143333712344656, 260.2409841647984763, 9.281406274060142181 ) ) ;
#55144=CARTESIAN_POINT ( 'NONE',  ( 94.11243691623624841, 215.9548013555409796, -4.594050593750042211 ) ) ;
#55146=CARTESIAN_POINT ( 'NONE',  ( 191.5694459269389824, 298.8389818071599962, 7.944420692511652504 ) ) ;
#55147=CARTESIAN_POINT ( 'NONE',  ( 181.4954090331713417, 255.0423029034424189, 0.9094182891644410072 ) ) ;
#55150=CARTESIAN_POINT ( 'NONE',  ( 196.0371429460125796, 291.1007035773004645, -15.98343019695849776 ) ) ;
#55151=VERTEX_POINT ( 'NONE', #39333 ) ;
#55157=CARTESIAN_POINT ( 'NONE',  ( 162.8493988834005677, 248.5835624823365322, 11.81438570587263470 ) ) ;
#55158=CARTESIAN_POINT ( 'NONE',  ( 87.26533679362427165, 215.0643266524160140, 9.188101187500095079 ) ) ;
#55161=EDGE_CURVE ( 'NONE', #47416, #13304, #10506, .T. ) ;
#55163=CARTESIAN_POINT ( 'NONE',  ( 208.3829315663354862, 269.7171704273955015, -1.768817828503133072 ) ) ;
#55164=EDGE_LOOP ( 'NONE', ( #58998, #52427, #39945, #9295 ) ) ;
#55165=EDGE_CURVE ( 'NONE', #38435, #39058, #95249, .T. ) ;
#55167=CARTESIAN_POINT ( 'NONE',  ( 183.8037341582430884, 275.4624792557407318, 17.77592483611231700 ) ) ;
#55169=CARTESIAN_POINT ( 'NONE',  ( 189.6768609436964539, 274.4077930505946483, -17.07046811116321550 ) ) ;
#55173=CARTESIAN_POINT ( 'NONE',  ( 157.6466783816650832, 259.5949387289228412, 17.71616314254395519 ) ) ;
#55174=CARTESIAN_POINT ( 'NONE',  ( 185.0706190396982151, 260.1753711840241863, 6.321521495746559971 ) ) ;
#55175=CARTESIAN_POINT ( 'NONE',  ( 159.3451320108506764, 254.6531307488737355, -16.72997986213134425 ) ) ;
#55176=CARTESIAN_POINT ( 'NONE',  ( 148.1295332417885504, 275.8061709343286907, -5.314593380240301812 ) ) ;
#55177=CARTESIAN_POINT ( 'NONE',  ( 174.7897835487166276, 284.0530019150879184, 13.84973856136962844 ) ) ;
#55178=CARTESIAN_POINT ( 'NONE',  ( 198.7291624623985058, 284.6509008601083224, -17.69774185455217008 ) ) ;
#55180=ORIENTED_EDGE ( 'NONE', *, *, #28094, .F. ) ;
#55182=( BOUNDED_CURVE ( )  B_SPLINE_CURVE ( 2, ( #985, #87158, #48591, #32382, #18193, #86148, #9603, #39957, #86641 ),
 .UNSPECIFIED., .F., .T. ) 
 B_SPLINE_CURVE_WITH_KNOTS ( ( 3, 2, 2, 2, 3 ),
 ( 0.8104838709677418818, 0.8118279569892472569, 0.8145161290322581182, 0.8172043010752688685, 0.8185483870967742437 ),
 .UNSPECIFIED. ) 
 CURVE ( )  GEOMETRIC_REPRESENTATION_ITEM ( )  RATIONAL_B_SPLINE_CURVE ( ( 0.9330127018922194093, 0.9330127018922194093, 1.000000000000000000, 0.8660254037844387076, 1.000000000000000000, 0.8660254037844387076, 1.000000000000000000, 0.9330127018922194093, 0.9330127018922194093 ) ) 
 REPRESENTATION_ITEM ( '' )  );
#55183=CARTESIAN_POINT ( 'NONE',  ( 161.8948331661419218, 250.2369188037922356, 13.64419044796309777 ) ) ;
#55185=CARTESIAN_POINT ( 'NONE',  ( 185.8323446419325364, 264.8229110950202880, -11.92140045508744883 ) ) ;
#55187=CARTESIAN_POINT ( 'NONE',  ( 156.8397658254749842, 272.7276435997338808, 14.63702169103162731 ) ) ;
#55188=VERTEX_POINT ( 'NONE', #97939 ) ;
#55190=CARTESIAN_POINT ( 'NONE',  ( 207.2824254892180704, 271.6233028670009162, 6.274396967990798046 ) ) ;
#55191=CARTESIAN_POINT ( 'NONE',  ( 154.9910882912764123, 262.1945556895526579, 18.38052604520346023 ) ) ;
#55193=CARTESIAN_POINT ( 'NONE',  ( 175.7824178399792174, 285.8628427244275372, -13.39878279634721103 ) ) ;
#55196=CARTESIAN_POINT ( 'NONE',  ( 164.9031621293093508, 284.7306714147449611, -3.125257715394198055 ) ) ;
#55199=CARTESIAN_POINT ( 'NONE',  ( 189.3293204741634383, 297.6371524027489954, -9.350876801542840511 ) ) ;
#55200=CARTESIAN_POINT ( 'NONE',  ( -5.751638101304356709, 176.6744531367911293, 4.594050593750047540 ) ) ;
#55205=CARTESIAN_POINT ( 'NONE',  ( 174.8650114509604521, 255.3214838289419788, 8.489119280892019503 ) ) ;
#55206=CARTESIAN_POINT ( 'NONE',  ( 183.0423515620436490, 268.5971907196498023, -16.46882057410648414 ) ) ;
#55207=CARTESIAN_POINT ( 'NONE',  ( 194.5253693406981483, 291.7191722712467481, 16.18900132190417551 ) ) ;
#55209=CARTESIAN_POINT ( 'NONE',  ( 20.58103360645747770, 188.8149278399160949, -9.188101187500095079 ) ) ;
#55213=CARTESIAN_POINT ( 'NONE',  ( 146.9456733906991417, 276.1296230653242105, -0.7988785540157754550 ) ) ;
#55216=CARTESIAN_POINT ( 'NONE',  ( 190.9034043754504921, 261.7470625323397826, -1.404837864312324935 ) ) ;
#55218=CARTESIAN_POINT ( 'NONE',  ( 59.05618993882879408, 218.2365022471903444, 2.944929066748280225E-16 ) ) ;
#55221=CARTESIAN_POINT ( 'NONE',  ( 32.46173284068399312, 198.7369531367911293, -4.594050593750048428 ) ) ;
#55222=CYLINDRICAL_SURFACE ( 'NONE', #63394, 10.00000000000010658 ) ;
#55223=CARTESIAN_POINT ( 'NONE',  ( 203.5726949774746117, 269.0034548673361883, -6.096665150295551783 ) ) ;
#55227=CARTESIAN_POINT ( 'NONE',  ( 202.6275056595488593, 279.1946885124775690, -15.35640559527740123 ) ) ;
#55228=CARTESIAN_POINT ( 'NONE',  ( 205.9961433675841818, 269.8120887608272369, -1.317021689134348250 ) ) ;
#55230=CARTESIAN_POINT ( 'NONE',  ( 202.9972156839127990, 279.0455039708822937, 16.77197898838388213 ) ) ;
#55231=CARTESIAN_POINT ( 'NONE',  ( 196.9098758191317700, 289.5890858996224324, -16.54412079817003800 ) ) ;
#55232=CARTESIAN_POINT ( 'NONE',  ( 175.3120577001922413, 257.3065038543072660, 11.69806524060765973 ) ) ;
#55235=B_SPLINE_CURVE_WITH_KNOTS ( 'NONE', 3,
 ( #31233, #91578, #91092, #22150, #53041, #83998, #30753, #343, #68739, #37833, #70234, #99662, #60130, #84977, #83490, #46424, #21658, #62119, #52540, #37338, #30248, #68240, #14056, #44936, #99164, #14560, #15523, #76370, #77349, #7956, #16041, #61131, #45435, #22652, #38830, #93067, #53536, #15030, #45922, #69736, #23621, #46943, #39317, #94580, #49439, #64143, #2875, #26152 ),
 .UNSPECIFIED., .F., .F.,
 ( 4, 2, 2, 2, 2, 2, 2, 2, 2, 2, 2, 2, 2, 2, 2, 2, 2, 2, 2, 2, 2, 2, 2, 4 ),
 ( 0.0005391196255988237344, 0.0009791966357432153358, 0.001199235140815413034, 0.001309254393351469165, 0.001419273645887525297, 0.001529292898423581862, 0.001639312150959637993, 0.001859350656031800563, 0.002299427666176084937, 0.003179581686464589500, 0.004059735706753093629, 0.004939889727041598191, 0.005379966737185807105, 0.005600005242257832631, 0.005710024494793798991, 0.005765034121061732297, 0.005820043747329665604, 0.005875053373597598910, 0.005930062999865532217, 0.006040082252401401432, 0.006260120757473031441, 0.006700197767616386871, 0.007140274777759743167, 0.007580351787903099464 ),
 .UNSPECIFIED. ) ;
#55236=B_SPLINE_CURVE_WITH_KNOTS ( 'NONE', 3,
 ( #34123, #9314, #100159, #30745 ),
 .UNSPECIFIED., .F., .F.,
 ( 4, 4 ),
 ( 0.0003686392678639645488, 0.008300137104892135742 ),
 .UNSPECIFIED. ) ;
#55240=ORIENTED_EDGE ( 'NONE', *, *, #15635, .T. ) ;
#55241=CARTESIAN_POINT ( 'NONE',  ( 17.25242200676955306, 190.7677522451419065, -5.000000000000047962 ) ) ;
#55242=CARTESIAN_POINT ( 'NONE',  ( 169.4692019312130924, 260.3030467232334786, 16.29845513612216479 ) ) ;
#55243=CARTESIAN_POINT ( 'NONE',  ( 151.2455280670316711, 268.6820563007532314, 14.35914944935941229 ) ) ;
#55249=EDGE_LOOP ( 'NONE', ( #16644, #32097, #40996 ) ) ;
#55250=CARTESIAN_POINT ( 'NONE',  ( 200.9061540366740246, 282.6673289856585143, -18.13083321883407351 ) ) ;
#55254=CARTESIAN_POINT ( 'NONE',  ( 189.9457600613112902, 301.6512882219586800, 0.04117870562599101891 ) ) ;
#55255=CARTESIAN_POINT ( 'NONE',  ( 183.7220472628443986, 289.6844837637199817, -13.20203550471168441 ) ) ;
#55256=ADVANCED_FACE ( 'NONE', ( #75627 ), #75139, .T. ) ;
#55258=CARTESIAN_POINT ( 'NONE',  ( 176.8860313499903612, 264.3628659159850827, -16.20694568242408806 ) ) ;
#55259=CARTESIAN_POINT ( 'NONE',  ( 161.8978992285310312, 267.0481668204226366, 16.51610106046594595 ) ) ;
#55262=CARTESIAN_POINT ( 'NONE',  ( 159.5764336135613632, 254.2525046211064819, 15.32981087583629076 ) ) ;
#55265=CARTESIAN_POINT ( 'NONE',  ( 59.71473008784930414, 205.2833772461660828, -9.188101187500095079 ) ) ;
#55266=ORIENTED_EDGE ( 'NONE', *, *, #56721, .F. ) ;
#55269=CARTESIAN_POINT ( 'NONE',  ( 150.3737790450080354, 270.1919698983467697, 15.09624067603409969 ) ) ;
#55270=CARTESIAN_POINT ( 'NONE',  ( 173.4413173480490400, 271.4189269517506204, 16.42543431503443330 ) ) ;
#55275=CARTESIAN_POINT ( 'NONE',  ( 198.2505066714982149, 285.2670451491296149, 0.000000000000000000 ) ) ;
#55277=CARTESIAN_POINT ( 'NONE',  ( 171.7283412409539665, 259.5113726030776888, -13.85753488430609615 ) ) ;
#55280=CARTESIAN_POINT ( 'NONE',  ( 161.7767236248226084, 250.4414905302161287, -13.15904643207033153 ) ) ;
#55281=CARTESIAN_POINT ( 'NONE',  ( 192.6247335881259630, 297.0111699613833594, -13.30158778996737290 ) ) ;
#55282=B_SPLINE_CURVE_WITH_KNOTS ( 'NONE', 3,
 ( #96798, #4544, #60216, #28852 ),
 .UNSPECIFIED., .F., .F.,
 ( 4, 4 ),
 ( 0.001595800230172596777, 0.002938264775114524108 ),
 .UNSPECIFIED. ) ;
#55283=CYLINDRICAL_SURFACE ( 'NONE', #99569, 17.82106496071139645 ) ;
#55284=CARTESIAN_POINT ( 'NONE',  ( 179.4583960273904211, 270.4090523040318885, 17.47970616590194837 ) ) ;
#55285=CARTESIAN_POINT ( 'NONE',  ( 205.7867067512454184, 274.2139637150027056, 10.62737868262404106 ) ) ;
#55288=CARTESIAN_POINT ( 'NONE',  ( 207.6172352878830907, 271.0433952848413810, 3.316653249540578496 ) ) ;
#55289=CARTESIAN_POINT ( 'NONE',  ( 108.9159718882352479, 227.5643266524159856, -9.188101187500093303 ) ) ;
#55290=VERTEX_POINT ( 'NONE', #5717 ) ;
#55291=CARTESIAN_POINT ( 'NONE',  ( 190.2298193533280255, 301.1592830958237528, -4.701752374740866713 ) ) ;
#55294=CARTESIAN_POINT ( 'NONE',  ( 154.9067123643522734, 262.3406990819208886, -18.18534662427576265 ) ) ;
#55296=CARTESIAN_POINT ( 'NONE',  ( 164.1224127655298730, 246.3786377597482158, 7.356982420601481998 ) ) ;
#55300=CARTESIAN_POINT ( 'NONE',  ( 207.6050568035884680, 271.0644890383991310, -1.456818755242089702 ) ) ;
#55301=CARTESIAN_POINT ( 'NONE',  ( 168.4888447738411230, 284.0319032102881351, -11.26574698934179253 ) ) ;
#55302=CARTESIAN_POINT ( 'NONE',  ( 182.4502886106904214, 259.6876753163259650, 10.69873880494191631 ) ) ;
#55304=CARTESIAN_POINT ( 'NONE',  ( 133.4351425849996531, 247.8458772461660544, 9.188101187500095079 ) ) ;
#55305=CARTESIAN_POINT ( 'NONE',  ( 150.6626254231123880, 269.6916732958875969, -15.32062296289003811 ) ) ;
#55306=CARTESIAN_POINT ( 'NONE',  ( 185.7479194277017882, 296.9610668245633178, 4.257868302861396614 ) ) ;
#55307=CARTESIAN_POINT ( 'NONE',  ( 157.6286460899086137, 257.6261715744221306, 18.25526781158026779 ) ) ;
#55309=CARTESIAN_POINT ( 'NONE',  ( 45.10055139898691579, 196.8458772461660544, 9.188101187500095079 ) ) ;
#55312=ORIENTED_EDGE ( 'NONE', *, *, #98662, .T. ) ;
#55316=B_SPLINE_SURFACE_WITH_KNOTS ( 'NONE', 3, 1, ( 
 ( #65893, #58777 ),
 ( #13702, #82153 ),
 ( #59269, #3623 ),
 ( #96848, #74527 ),
 ( #90247, #28909 ),
 ( #34991, #20819 ),
 ( #12725, #75015 ),
 ( #82658, #13217 ),
 ( #73030, #44076 ),
 ( #90751, #21305 ),
 ( #36487, #52181 ),
 ( #83130, #34501 ),
 ( #96344, #26911 ),
 ( #57790, #88769 ),
 ( #50202, #11721 ),
 ( #73516, #61279 ),
 ( #77507, #69878 ),
 ( #85645, #30388 ),
 ( #69387, #15675 ),
 ( #23273, #93218 ),
 ( #85125, #46569 ),
 ( #91224, #8098 ),
 ( #22793, #14199 ),
 ( #91724, #21792 ),
 ( #53190, #44574 ),
 ( #53672, #38474 ),
 ( #492, #31379 ),
 ( #6600, #84626 ),
 ( #52676, #75508 ),
 ( #45088, #68384 ),
 ( #22289, #62264 ),
 ( #23777, #6094 ),
 ( #36988, #76022 ),
 ( #98820, #29400 ) ),
 .UNSPECIFIED., .T., .F., .F.,
 ( 4, 2, 2, 2, 2, 2, 2, 2, 2, 2, 2, 2, 2, 2, 2, 2, 4 ),
 ( 2, 2 ),
 ( 0.000000000000000000, 0.06250000000000000000, 0.1250000000000000000, 0.1875000000000000000, 0.2500000000000000000, 0.3125000000000000000, 0.3750000000000000000, 0.4375000000000000000, 0.5000000000000000000, 0.5625000000000000000, 0.6250000000000000000, 0.6875000000000000000, 0.7500000000000000000, 0.8125000000000000000, 0.8750000000000000000, 0.9375000000000000000, 1.000000000000000000 ),
 ( 0.000000000000000000, 1.000000000000000000 ),
 .UNSPECIFIED. ) ;
#55320=CARTESIAN_POINT ( 'NONE',  ( 203.3041373168503299, 278.5139001086923827, -16.61929732091214973 ) ) ;
#55321=CARTESIAN_POINT ( 'NONE',  ( 8.888801338793459905, 187.4860189848785410, -2.679491924311252493 ) ) ;
#55322=EDGE_CURVE ( 'NONE', #83827, #41296, #28619, .T. ) ;
#55323=CARTESIAN_POINT ( 'NONE',  ( 121.6806519464431773, 234.3927522451418213, 10.00000000000009592 ) ) ;
#55324=AXIS2_PLACEMENT_3D ( 'NONE', #72716, #3305, #34185 ) ;
#55328=CARTESIAN_POINT ( 'NONE',  ( 162.9148248802443106, 248.4702413316674381, 9.709394404200100581 ) ) ;
#55329=CARTESIAN_POINT ( 'NONE',  ( -22.42236680055709641, 157.8615022471902591, 0.000000000000000000 ) ) ;
#55330=CARTESIAN_POINT ( 'NONE',  ( 33.73396797431614402, 190.2833772461660544, -9.188101187500095079 ) ) ;
#55333=CARTESIAN_POINT ( 'NONE',  ( 190.1752790837055045, 301.2537496138681945, -5.177773110520776711 ) ) ;
#55337=CARTESIAN_POINT ( 'NONE',  ( 53.12030748017507165, 208.1427522451419350, 10.00000000000009237 ) ) ;
#55338=CARTESIAN_POINT ( 'NONE',  ( 128.2864073861747727, 233.3262482093457493, 3.021315404115420679E-15 ) ) ;
#55339=CARTESIAN_POINT ( 'NONE',  ( 184.4818116536155514, 257.8287756997602287, 1.353309037794695024 ) ) ;
#55340=CARTESIAN_POINT ( 'NONE',  ( 157.2104826425669728, 258.3504519110855995, -16.92635148710569482 ) ) ;
#55341=CARTESIAN_POINT ( 'NONE',  ( 162.2080922643726240, 251.7946761793016321, -12.96017575965868396 ) ) ;
#55342=ORIENTED_EDGE ( 'NONE', *, *, #38969, .F. ) ;
#55343=CARTESIAN_POINT ( 'NONE',  ( 21.31191609055706593, 183.1115022471902591, 10.00000000000009592 ) ) ;
#55346=CARTESIAN_POINT ( 'NONE',  ( 143.8814004702669536, 260.0024278399161517, 9.188101187500095079 ) ) ;
#55348=CARTESIAN_POINT ( 'NONE',  ( 170.0801020929759204, 263.5121983774269552, 15.83860714571988915 ) ) ;
#55349=CARTESIAN_POINT ( 'NONE',  ( 185.3894397174689175, 260.3747351616150354, 6.351723045801915823 ) ) ;
#55350=CARTESIAN_POINT ( 'NONE',  ( 74.86346528667428402, 202.4824982072973967, 3.021315404115420679E-15 ) ) ;
#55351=CARTESIAN_POINT ( 'NONE',  ( 183.5770085761344887, 258.0265213594843772, -2.300074763849718540 ) ) ;
#55353=EDGE_LOOP ( 'NONE', ( #96678, #92415, #70096 ) ) ;
#55354=B_SPLINE_CURVE_WITH_KNOTS ( 'NONE', 3,
 ( #32625, #63523, #48843, #10340 ),
 .UNSPECIFIED., .F., .F.,
 ( 4, 4 ),
 ( 0.008727764669621856930, 0.01504605018596882372 ),
 .UNSPECIFIED. ) ;
#55355=B_SPLINE_CURVE_WITH_KNOTS ( 'NONE', 3,
 ( #61836, #17245, #10164, #63849 ),
 .UNSPECIFIED., .F., .F.,
 ( 4, 4 ),
 ( 0.04383130453832326245, 0.04887120950165268346 ),
 .UNSPECIFIED. ) ;
#55356=CARTESIAN_POINT ( 'NONE',  ( 179.8738126827349788, 255.7374587583702237, -7.018155654023178869 ) ) ;
#55358=CARTESIAN_POINT ( 'NONE',  ( 153.2539470794098122, 277.7226751097910551, -5.798683309584624190 ) ) ;
#55360=CARTESIAN_POINT ( 'NONE',  ( 206.1062572280473546, 273.6604860535989587, -9.773577984388410300 ) ) ;
#55364=CARTESIAN_POINT ( 'NONE',  ( 93.60468337831815688, 236.3967562850347122, -4.648177544792955347E-16 ) ) ;
#55366=CARTESIAN_POINT ( 'NONE',  ( 193.9401685343300699, 294.7327698005063326, 14.01047396938887069 ) ) ;
#55367=ORIENTED_EDGE ( 'NONE', *, *, #427, .F. ) ;
#55371=ORIENTED_EDGE ( 'NONE', *, *, #44100, .T. ) ;
#55372=CARTESIAN_POINT ( 'NONE',  ( 160.0581542544236697, 283.4287238101934463, 3.385839116031148510 ) ) ;
#55374=ORIENTED_EDGE ( 'NONE', *, *, #72185, .T. ) ;
#55375=CYLINDRICAL_SURFACE ( 'NONE', #57208, 10.00000000000010658 ) ;
#55378=AXIS2_PLACEMENT_3D ( 'NONE', #1309, #85449, #60200 ) ;
#55380=CARTESIAN_POINT ( 'NONE',  ( 155.5508027672438516, 261.2251017794452537, 18.53492801382433797 ) ) ;
#55381=B_SPLINE_CURVE_WITH_KNOTS ( 'NONE', 3,
 ( #61616, #76356, #92571, #39794, #70218, #1338, #30234, #24621, #825, #62609, #93053, #32223, #63126, #9943, #58027, #3836, #41309, #72253, #64128, #95078, #11458, #79380, #56001, #88493, #72765, #73243, #96075, #47910, #2858, #95591, #42314, #48432, #34721, #56523, #87511, #32723, #94563, #33749, #19055, #64641, #26137, #40805, #9433, #25642, #78851, #49929, #57016, #18044 ),
 .UNSPECIFIED., .F., .F.,
 ( 4, 2, 2, 2, 2, 2, 2, 2, 2, 2, 2, 2, 2, 2, 2, 2, 2, 2, 2, 2, 2, 2, 2, 4 ),
 ( 0.0002339713884637640586, 0.0007176085954676936045, 0.001201245802471623096, 0.001443064405973626656, 0.001563973707724620630, 0.001684883009475614604, 0.001805792311226608578, 0.001926701612977602552, 0.002168520216479427436, 0.002652157423483079805, 0.003135794630486731741, 0.004103069044493933698, 0.005070343458501136956, 0.005553980665504702589, 0.005795799269006407343, 0.005916708570757258853, 0.006037617872508110363, 0.006098072523383518337, 0.006158527174258925443, 0.006279436476009738789, 0.006521255079511365481, 0.007004892286514617997, 0.007488529493517870513, 0.007972166700521123028 ),
 .UNSPECIFIED. ) ;
#55382=CARTESIAN_POINT ( 'NONE',  ( 151.4384131719918685, 268.3479694989391078, 14.98299707687648841 ) ) ;
#55384=ORIENTED_EDGE ( 'NONE', *, *, #25704, .T. ) ;
#55386=B_SPLINE_CURVE_WITH_KNOTS ( 'NONE', 3,
 ( #50542, #33885, #4451, #88124, #49553, #80506, #34358, #41956, #3483, #96200, #26761, #90632, #76394, #61160, #99687, #28779, #52074, #45948, #36873, #46450, #44462, #22682, #61660, #77381, #53561, #59660, #14583, #67779, #36366, #6970, #92129, #37854, #68763, #67271, #30270, #45461, #84513, #30779, #92609, #15057, #54047, #37362, #76865, #23156, #98198, #7463 ),
 .UNSPECIFIED., .F., .F.,
 ( 4, 2, 2, 2, 2, 2, 2, 2, 2, 2, 2, 2, 2, 2, 2, 2, 2, 2, 2, 2, 2, 2, 4 ),
 ( 0.0007152033892065767741, 0.0009241115395241573677, 0.001133019689841737853, 0.001237473765000528421, 0.001341927840159318555, 0.001550835990476795608, 0.001968652291111705043, 0.002386468591746614912, 0.003222101193016370033, 0.004057733794286125587, 0.004893366395555881140, 0.005311182696190713814, 0.005520090846508093722, 0.005624544921666784110, 0.005676771959246130171, 0.005728998996825474498, 0.005833453071984298459, 0.005937907147143122420, 0.006146815297460746924, 0.006355723447778373163, 0.006564631598095997667, 0.006982447898731253613, 0.007400264199366509560 ),
 .UNSPECIFIED. ) ;
#55394=CARTESIAN_POINT ( 'NONE',  ( 148.4083960970861256, 273.5961130204771052, -8.574185186226726429 ) ) ;
#55395=EDGE_CURVE ( 'NONE', #469, #4764, #87912, .T. ) ;
#55401=CARTESIAN_POINT ( 'NONE',  ( 201.8642752310742026, 279.1281314597073901, -15.91742344199423975 ) ) ;
#55402=CARTESIAN_POINT ( 'NONE',  ( 191.4715169758341631, 298.5146068092147402, -8.393071345078833900 ) ) ;
#55403=CARTESIAN_POINT ( 'NONE',  ( 197.9598023461055902, 287.7705598106892921, 18.23120408239484291 ) ) ;
#55406=CARTESIAN_POINT ( 'NONE',  ( 168.2950000418480840, 257.1262184943008151, -14.43479976811267207 ) ) ;
#55407=CARTESIAN_POINT ( 'NONE',  ( 159.6288139302610887, 254.1617792512662675, -15.32287760493869477 ) ) ;
#55411=CARTESIAN_POINT ( 'NONE',  ( 161.5056331467593225, 250.9110330116698435, 14.52719814064025528 ) ) ;
#55414=CARTESIAN_POINT ( 'NONE',  ( 194.1856896721330941, 294.3075147154997353, -15.68532121655275091 ) ) ;
#55415=CARTESIAN_POINT ( 'NONE',  ( 136.3309150271299757, 239.5177522451417929, 5.000000000000051514 ) ) ;
#55417=CARTESIAN_POINT ( 'NONE',  ( 12.05626958406296367, 177.7677522451418497, 10.00000000000009592 ) ) ;
#55418=CARTESIAN_POINT ( 'NONE',  ( 82.93486267893706554, 224.8149278399160664, -9.188101187500095079 ) ) ;
#55419=CARTESIAN_POINT ( 'NONE',  ( 196.2856740628847660, 269.3488336749823020, -11.99430192484340729 ) ) ;
#55421=CARTESIAN_POINT ( 'NONE',  ( 170.2399687990647976, 280.5198609568276424, -13.78404537617314141 ) ) ;
#55422=CARTESIAN_POINT ( 'NONE',  ( 4.315907217689738395, 182.4869531367911293, 4.594050593750046652 ) ) ;
#55424=CARTESIAN_POINT ( 'NONE',  ( 200.1385401540174769, 283.9968752310148830, 17.30012534137638625 ) ) ;
#55427=EDGE_LOOP ( 'NONE', ( #75177, #40953, #12986, #75031 ) ) ;
#55428=CARTESIAN_POINT ( 'NONE',  ( 169.1311965936330353, 247.8770103324328034, 7.134965090537657859E-13 ) ) ;
#55429=CARTESIAN_POINT ( 'NONE',  ( 188.8744765375133454, 261.5075027424167615, -6.011881065006100755 ) ) ;
#55432=CARTESIAN_POINT ( 'NONE',  ( 207.8844858873204657, 270.5805036682629066, -6.251308616122969397 ) ) ;
#55433=CARTESIAN_POINT ( 'NONE',  ( 142.4863040978925142, 267.5053245118543828, -2.761272660171010366E-15 ) ) ;
#55436=CARTESIAN_POINT ( 'NONE',  ( 38.38920161542251464, 180.7202760586659451, -5.415160957724236172E-17 ) ) ;
#55437=CARTESIAN_POINT ( 'NONE',  ( 77.00817486789587463, 215.2677522451418497, 10.00000000000009592 ) ) ;
#55438=CARTESIAN_POINT ( 'NONE',  ( 199.4869826154170482, 277.5167049526704091, 15.17882519192913726 ) ) ;
#55442=ADVANCED_FACE ( 'NONE', ( #40593 ), #80659, .T. ) ;
#55443=CARTESIAN_POINT ( 'NONE',  ( 175.2553799847831897, 281.2052230826317327, -14.44794444881370943 ) ) ;
#55446=CARTESIAN_POINT ( 'NONE',  ( 157.0957870390718369, 258.5491105237443321, 17.69218919045495397 ) ) ;
#55447=CARTESIAN_POINT ( 'NONE',  ( 155.4917600441137324, 261.3273667757233056, 17.14261720787171939 ) ) ;
#55448=CARTESIAN_POINT ( 'NONE',  ( 207.6357208050208101, 271.0113774299547913, -6.790259683043212036 ) ) ;
#55450=CARTESIAN_POINT ( 'NONE',  ( 194.6310785344323904, 293.5360785768717165, -14.54510914272505495 ) ) ;
#55454=CARTESIAN_POINT ( 'NONE',  ( 163.8147431267737204, 246.9115372060205118, 7.125417796469586840 ) ) ;
#55455=CARTESIAN_POINT ( 'NONE',  ( 175.9532122701685921, 256.5273912432038514, -11.06277192129556042 ) ) ;
#55456=CARTESIAN_POINT ( 'NONE',  ( 191.5324528500417216, 298.9030556958743432, -8.286652526617016790 ) ) ;
#55457=CARTESIAN_POINT ( 'NONE',  ( 148.1672759425158290, 274.0137453789218398, 7.847779094015780110 ) ) ;
#55460=CARTESIAN_POINT ( 'NONE',  ( 135.0578773561867649, 260.3297689869269220, -2.679491924311252493 ) ) ;
#55461=CARTESIAN_POINT ( 'NONE',  ( 110.1064097226738312, 240.5024278399161233, 9.188101187500095079 ) ) ;
#55463=CARTESIAN_POINT ( 'NONE',  ( 191.5694459269389824, 298.8389818071599962, 7.944420692511652504 ) ) ;
#55467=CARTESIAN_POINT ( 'NONE',  ( 102.5355703512972809, 241.5530062829863027, -4.648177544792955347E-16 ) ) ;
#55469=CARTESIAN_POINT ( 'NONE',  ( 190.9252692466827455, 299.9547285464148558, -6.441337159356977260 ) ) ;
#55470=CARTESIAN_POINT ( 'NONE',  ( 189.7671801472840514, 261.0678685170981339, -4.565022058661969417 ) ) ;
#55471=CARTESIAN_POINT ( 'NONE',  ( 196.6800254274587019, 289.9871984561398222, -17.90749311895638129 ) ) ;
#55472=CARTESIAN_POINT ( 'NONE',  ( 89.36707907128423756, 215.7365022471902023, 10.00000000000009948 ) ) ;
#55473=CARTESIAN_POINT ( 'NONE',  ( 173.7827001204449004, 290.0886546788046303, -1.066826985794086191 ) ) ;
#55476=CARTESIAN_POINT ( 'NONE',  ( 132.7946446283434625, 254.1427522451419065, -10.00000000000009592 ) ) ;
#55478=CARTESIAN_POINT ( 'NONE',  ( 199.8507473897895750, 270.1007356502280459, 9.248113246699395162 ) ) ;
#55481=CARTESIAN_POINT ( 'NONE',  ( 187.5689534105982261, 259.0063497273899884, 3.853393514624363636 ) ) ;
#55483=CARTESIAN_POINT ( 'NONE',  ( 152.8522706834672533, 265.8990964544007056, 17.63080661522264947 ) ) ;
#55484=( BOUNDED_SURFACE ( )  B_SPLINE_SURFACE ( 1, 2, ( 
 ( #16958, #62546, #93508, #23052, #86432, #47847, #78786, #269, #64073, #53950, #40750, #9373, #40252, #9893, #71192, #1786, #25064, #32668, #63567, #86938, #17469, #48380, #71699, #2293, #84906, #15448, #2801, #49869, #10384, #12383, #95018, #18995, #33687, #41253, #87457, #48883, #72193, #4262, #49372, #35161, #3298, #73188, #79817, #11400, #18487, #73679, #26583, #80832, #42254, #80315, #42745, #74193, #97018, #27588, #66070, #58453, #3782, #34664, #96020, #65566, #57456, #19505, #56466, #11887, #50857, #26082, #89426, #64582, #19980, #95534, #43249, #96512, #81808, #25580, #4783, #87943, #27082, #17989, #56956, #10885, #41761, #72708, #57964, #34177, #65071, #88949, #50361, #81316, #35664, #52847, #97977, #68547, #13377, #13858, #52349, #44244, #84298, #75182, #44736, #75670, #6255, #37153, #68052, #67552, #36150, #98975, #22453, #5756, #74692, #98484, #99472, #36646, #89902, #37636, #29076, #76655, #82809, #14846, #60433, #20990, #59941, #66565, #5270, #90912, #67054, #12891, #7243, #97492, #45732, #29559, #21461, #53348, #83294, #14360, #30048, #76183, #91389, #21953, #83797, #43748, #45247, #6758, #60938, #20481, #28553, #91898, #82322, #28059, #58932, #51354, #59435, #90416, #51871, #92393, #53829, #47732, #92881, #78666, #46747, #16349, #22940, #54838, #61929, #16842, #70037, #93387, #62426, #23435, #86307, #17343, #40129, #71068, #9257, #1670, #23939, #85820, #39123, #47243, #650, #32553, #86811, #55818, #85295, #84789, #15330, #78163, #69042, #63451, #46225, #8750, #94387, #24940, #77147, #38643, #48251, #8258, #39621, #79197, #70543, #7751, #1159, #38125, #32033, #62944, #99972, #69549, #31537, #30557, #61441, #154, #31042, #93895, #54324, #15839, #24449, #77674, #55330, #50239, #63944, #26460, #33045, #81193, #40633, #18361, #19861, #72577, #80699, #41127, #25445, #3665, #88310, #41633, #49746, #64957, #64451, #11274, #42625, #42136, #96891, #95902, #4138, #57833, #50728, #96386, #34543, #80191, #94883, #73067, #57336, #3182, #18864, #72065, #56335, #73554, #49254, #65937, #10258, #65441, #35033, #87333, #11762, #33556, #71568, #2164, #26950, #10759, #88814, #19379, #27460, #95410, #58331, #48763, #25967, #89307, #17865, #9771, #79696, #2665, #56837, #87822, #45493, #84059, #51225, #74058, #29808, #27935, #85038, #54084, #15587, #14615, #4647, #61194, #81683, #7494, #30811, #82193, #89779, #37886, #53104, #22713, #36027, #38392, #53593, #15090, #91640, #12764, #76427, #74568, #84550, #7000, #68795, #43114, #92163, #68299, #61690, #46488, #69303, #22207, #45979, #99723, #30309, #5146, #76896, #20355, #99222, #100225, #35539, #92643, #58817, #93136, #23191, #77421, #8022, #38894, #43629, #66442, #60681, #69798, #407, #31297, #62183, #23685, #97369, #12256, #54580, #79453, #2426, #55090, #62688, #9524, #24699, #94643, #9004, #10018, #25199, #87077, #63204, #24209, #55581, #47498, #56082, #86565, #17095, #16106, #32803, #39876, #33303, #25722, #40880, #63707, #79948, #10514, #93644, #86076, #41391, #47993, #17609, #64205, #1916, #16600, #71325, #64716, #48517, #71829, #95154, #78423, #78936, #72334, #56601, #70813, #87587, #40385, #1419, #32302, #18112, #8511, #94146, #49015, #39379, #2939, #77919, #33827, #85561, #95665, #47005, #70296, #907, #31786, #41897, #20116, #4398, #58097, #66206, #50488, #80961, #97147, #59067, #27713, #13023, #81443, #20611, #74328, #36289, #12514, #50986, #96645, #11025, #58581, #42871, #89080, #35295, #88570, #72836, #90037, #34788, #82461, #26708, #12014, #51492, #3429, #28191, #50005, #88073, #18621, #81936, #89553, #19630, #65691, #34304, #43386, #42386, #27215, #49499, #65204, #73804, #96145, #43886, #26213, #4917, #57589, #19132, #80454, #11525, #73316, #35797, #3907, #66691, #97627, #74825, #5405, #67188, #57090, #76786, #29692, #52986, #22088, #52483, #45861, #77291, #100109, #30693, #7379, #38268, #83934, #14498, #99109, #45380, #60568, #69179, #46362, #15467, #44876, #13514, #51997, #76311, #28696, #61573, #44382, #22588, #59574, #14974, #53964, #29205, #92524, #36786, #23070, #67695, #7899, #68677, #84921, #90549, #38774, #91035, #91524, #21121, #98623, #83431, #5895, #82940, #6885, #6400, #13997, #30186, #60073, #75315, #98112, #84429, #21603, #75816, #37285, #37775, #99608, #68180, #61072, #92043, #53478, #78801, #16973, #9389, #40265, #70680, #39259, #71205, #25594, #78301, #77808, #1294, #2305, #47376, #93011, #40762, #32179, #79829, #85955, #18003, #63581, #24081, #39751, #69680, #8391, #94027, #70171, #15984, #10397, #284, #87468, #1797, #8883, #56480, #63082, #17483, #71713, #79334, #54456, #32681, #86448, #24578, #94523, #31665, #46883, #33186, #55461, #48895, #778, #47864, #95030, #62561, #64086, #93524, #31172, #62062, #25075, #55955, #86950, #48391, #9904, #54977, #23565, #16482, #85435, #11414, #64595, #80844, #18500, #51369, #73201, #49885, #3796, #42268, #10899, #33702, #88452, #87955, #43263, #12397, #74208, #34677, #95547, #19517, #41266, #66085, #89438, #41775, #49386, #96527, #65579, #81330, #96034, #97031, #11901, #73691, #27097, #72721, #57980, #34191, #42759, #88963, #50377, #2813, #4275, #26595, #19994, #4798, #27600, #35174, #66580, #97504, #80331, #3312, #28074, #58466, #50872, #81822, #35679, #65083, #58946, #82337, #89917, #20497, #72209, #57469, #26096, #56970, #19011, #75196, #84313, #98990, #44264, #98500, #99488, #67067, #21478, #53363, #97991, #29573, #36164, #14860, #43764, #52366, #22955, #75687, #83812, #5771, #28570, #6773, #91404, #44754, #52862, #37168, #67567, #14379, #45747, #45263, #99988, #68066, #7259, #60955, #53844, #30066, #37652, #83311, #91914, #6273, #60451, #21969, #29090, #22469, #92407, #76672, #38142, #69059, #30572, #76197, #68563, #13873, #61457, #12905, #74708, #5285, #59450, #59956, #90431, #21003, #51884, #82825, #13393, #36660, #90928, #46240, #1686, #40649, #15857, #55833, #23449, #63467, #54339, #2182, #55346, #32571, #15344, #94403, #77690, #78179, #7768, #85311 ),
 ( #46764, #54859, #8273, #86323, #85837, #16367, #77166, #62962, #39138, #24957, #86828, #40146, #93912, #9789, #71587, #92896, #70051, #33065, #47258, #16860, #17361, #32050, #666, #1176, #94901, #24466, #47747, #48268, #31551, #8768, #63959, #79215, #62440, #25464, #70559, #93407, #23956, #71087, #38661, #39637, #84804, #69564, #78684, #171, #31055, #61944, #9273, #66457, #18884, #26971, #87839, #72083, #50256, #34560, #88329, #96402, #80719, #10778, #57853, #89323, #88833, #43133, #11293, #50747, #58347, #19877, #4153, #35050, #42152, #73087, #57353, #3681, #49764, #96908, #4665, #74075, #3200, #2684, #10275, #65460, #87353, #81700, #33575, #81209, #17882, #73571, #12273, #18378, #27479, #95430, #65957, #25983, #35556, #19397, #97382, #48780, #56353, #49273, #11781, #79712, #56853, #41653, #64470, #41145, #42641, #64974, #72595, #80210, #34084, #95917, #26477, #14252, #59325, #29943, #75070, #75561, #13747, #5649, #45625, #36539, #6149, #37043, #67952, #98870, #29449, #28962, #97872, #60325, #84197, #67445, #36041, #59840, #60818, #98374, #51242, #99364, #90803, #38020, #44136, #76554, #21847, #82707, #21358, #27949, #66942, #52243, #28445, #74583, #68931, #58831, #7133, #91281, #83187, #14744, #44627, #76079, #91780, #37530, #52729, #83691, #45139, #5162, #6655, #68435, #22345, #82209, #90305, #53242, #43645, #89796, #20371, #12780, #20875, #51765, #13274, #53724, #15223, #9147, #54216, #40021, #8148, #78055, #84683, #16241, #23329, #78561, #31429, #54724, #23830, #85183, #47630, #79085, #39021, #7640, #547, #32447, #77559, #22840, #70961, #62320, #9667, #15730, #48141, #93787, #46634, #69929, #99856, #38532, #85705, #69438, #46118, #40528, #30441, #17234, #1049, #93273, #86700, #47132, #1562, #63343, #94281, #8644, #39514, #70439, #77034, #31927, #62831, #24347, #55, #30939, #55221, #61824, #61330, #92290, #86202, #92775, #16741, #24836, #55710, #87222, #81094, #25862, #11660, #80087, #49634, #25338, #88204, #95306, #50140, #3077, #26352, #95799, #56738, #19274, #50627, #73456, #4039, #42522, #34928, #57228, #18755, #72473, #80591, #33967, #65824, #19759, #89211, #18256, #17756, #56229, #11168, #2054, #96789, #48657, #96279, #32936, #88704, #27349, #2562, #58230, #10154, #81581, #41020, #12150, #42036, #71463, #63840, #94778, #64342, #64852, #79590, #71958, #87720, #33445, #49152, #72971, #10654, #41530, #3562, #34442, #65341, #26849, #57724, #74468, #45022, #90180, #90689, #28843, #20755, #60704, #51643, #21246, #52123, #83074, #13644, #44517, #44011, #12660, #75448, #99248, #5538, #6032, #5048, #89692, #75966, #82592, #29832, #43529, #59723, #68322, #20251, #6541, #66830, #4536, #35436, #67840, #13157, #36927, #98760, #74954, #97758, #29343, #82088, #28328, #36422, #66339, #67330, #51126, #53129, #98254, #60208, #91169, #21733, #35928, #97272, #52617, #59205, #37416, #14136, #91665, #83575, #27839, #22228, #43012, #84086, #73950, #58716, #52653, #99774, #14671, #84604, #99284, #100281, #15142, #76956, #53166, #14174, #45549, #37449, #46039, #76482, #7059, #6066, #22771, #29866, #23250, #15647, #30867, #53648, #69855, #468, #83606, #45059, #31357, #37941, #7556, #92700, #92219, #76000, #61250, #54643, #38448, #69362, #54138, #6577, #68853, #62240, #85100, #68359, #46545, #30367, #60737, #91699, #61750, #98794, #84120, #77480, #29375, #8077, #67873, #38950, #75483, #93194, #85620, #23747, #44549, #22262, #60243, #36960, #91202, #21763, #56142, #40448, #70874, #87141, #49073, #17672, #3000, #71383, #10574, #64263, #26272, #2481, #10073, #86623, #968, #48572, #32858, #95216, #57148, #33363, #40938, #17157, #31845, #79511, #63765, #78998, #25259, #78481, #62748, #80005, #24758, #72390, #16660, #1971, #41449, #93704, #18171, #39935, #77975, #8572, #71882, #48055, #25783, #94697, #9584, #1480, #56659, #55144, #32363, #87644, #39437, #33890, #24267, #16164, #64775, #95723, #47062, #70356, #86130, #47554, #63262, #9068, #94203, #59125, #51555, #19685, #11085, #66265, #88130, #12573, #35856, #88624, #96204, #42929, #58154, #27766, #42440, #43450, #89615, #20176, #96702, #57648, #89134, #81021, #51043, #50547, #12071, #49557, #97199, #73376, #66749, #90098, #74391, #82001, #13079, #43940, #26767, #19193, #5463, #73868, #4974, #97685, #35355, #50063, #4457, #98178, #28251, #82518, #36346, #11583, #67249, #28757, #18676, #3963, #80510, #41960, #34845, #65749, #72897, #3487, #27271, #34362, #65260, #76371, #82994, #30754, #90609, #68241, #69737, #22152, #30249, #91093, #75374, #53537, #37834, #91579, #99663, #84000, #14057, #61132, #23128, #92107, #46425, #14561, #54023, #75882, #99165, #13572, #67757, #45436, #5957, #77350, #59637, #6942, #98682, #36849, #52056, #44442, #29262, #69239, #44938, #100169, #29753, #68740, #60132, #22654, #83491, #38331, #53042, #84488, #15031, #6460, #7438, #38831, #61633, #84978, #15524, #7957, #45923, #76841, #60625, #345, #21176, #21659, #52541, #37339, #78364, #46944, #85494, #78867, #62120, #64144, #77862, #56018, #93068, #48449, #87528, #62624, #2364, #70235, #9961, #839, #48955, #1856, #79394, #23622, #40819, #24146, #24639, #54516, #31720, #16539, #39319, #16043, #9452, #39811, #86013, #63643, #93579, #8448, #71766, #17542, #55031, #33242, #8944, #40324, #17036, #70743, #79889, #1355, #71263, #32738, #94581, #25135, #87013, #32240, #47435, #95095, #18059, #63140, #94085, #55519, #25659, #86507, #47927, #56538, #10453, #41327, #72270, #31234, #50436, #65144, #49946, #2876, #10964, #3852, #41836, #18561, #4857, #33768, #74273, #81390, #19071, #43327, #34735, #35238, #89499, #97088, #27156, #65636, #80904, #80394, #11957, #64655, #11476, #72782, #49440, #58043, #26153, #20057, #3373, #73748, #57030, #66141, #95605, #26651, #81880, #96092, #50930, #57532, #88013, #12456, #34247, #88508, #42329, #4342, #73257, #89024, #27657, #58525, #42818, #19575, #96592, #1684, #47745, #25461, #62960, #16365, #10273, #79710, #24464, #95428, #40143, #40647 ) ),
 .UNSPECIFIED., .F., .F., .T. ) 
 B_SPLINE_SURFACE_WITH_KNOTS ( ( 2, 2 ),
 ( 3, 2, 2, 2, 2, 2, 2, 2, 2, 2, 2, 2, 2, 2, 2, 2, 2, 2, 2, 2, 2, 2, 2, 2, 2, 2, 2, 2, 2, 2, 2, 2, 2, 2, 2, 2, 2, 2, 2, 2, 2, 2, 2, 2, 2, 2, 2, 2, 2, 2, 2, 2, 2, 2, 2, 2, 2, 2, 2, 2, 2, 2, 2, 2, 2, 2, 2, 2, 2, 2, 2, 2, 2, 2, 2, 2, 2, 2, 2, 2, 2, 2, 2, 2, 2, 2, 2, 2, 2, 2, 2, 2, 2, 2, 2, 2, 2, 2, 2, 2, 2, 2, 2, 2, 2, 2, 2, 2, 2, 2, 2, 2, 2, 2, 2, 2, 2, 2, 2, 2, 2, 2, 2, 2, 2, 2, 2, 2, 2, 2, 2, 2, 2, 2, 2, 2, 2, 2, 2, 2, 2, 2, 2, 2, 2, 2, 2, 2, 2, 2, 2, 2, 2, 2, 2, 2, 2, 2, 2, 2, 2, 2, 2, 2, 2, 2, 2, 2, 2, 2, 2, 2, 2, 2, 2, 2, 2, 2, 2, 2, 2, 2, 2, 2, 2, 2, 2, 2, 2, 2, 2, 2, 2, 2, 2, 2, 2, 2, 2, 2, 2, 2, 2, 2, 2, 2, 2, 2, 2, 2, 2, 2, 2, 2, 2, 2, 2, 2, 2, 2, 2, 2, 2, 2, 2, 2, 2, 2, 2, 2, 2, 2, 2, 2, 2, 2, 2, 2, 2, 2, 2, 2, 2, 2, 2, 2, 2, 2, 2, 2, 2, 2, 2, 2, 2, 2, 2, 2, 2, 2, 2, 2, 2, 2, 2, 2, 2, 2, 2, 2, 2, 2, 2, 2, 2, 2, 2, 2, 2, 2, 2, 2, 2, 2, 2, 2, 2, 2, 2, 2, 2, 2, 2, 2, 2, 2, 2, 2, 2, 2, 2, 2, 2, 2, 2, 2, 2, 2, 2, 2, 2, 2, 2, 2, 2, 2, 2, 2, 2, 2, 2, 2, 2, 2, 2, 2, 2, 2, 2, 2, 2, 2, 2, 2, 2, 2, 2, 2, 2, 2, 2, 2, 2, 2, 2, 2, 2, 2, 2, 2, 2, 2, 2, 2, 2, 2, 2, 2, 2, 2, 2, 2, 2, 2, 2, 2, 2, 2, 2, 2, 2, 2, 3 ),
 ( 0.000000000000000000, 1.000000000000000000 ),
 ( 0.000000000000000000, 0.002688172043010752903, 0.005376344086021505805, 0.008064516129032257841, 0.01075268817204301161, 0.01344086021505376365, 0.01612903225806451568, 0.01881720430107526945, 0.02150537634408602322, 0.02419354838709677352, 0.02688172043010752729, 0.02956989247311828106, 0.03225806451612903136, 0.03494623655913978166, 0.03763440860215053890, 0.04032258064516128920, 0.04301075268817204644, 0.04569892473118279674, 0.04838709677419354704, 0.05107526881720430428, 0.05376344086021505458, 0.05645161290322580488, 0.05913978494623656212, 0.06182795698924731242, 0.06451612903225806273, 0.06720430107526881303, 0.06989247311827956333, 0.07258064516129032751, 0.07526881720430107781, 0.07795698924731182811, 0.08064516129032257841, 0.08333333333333332871, 0.08602150537634409289, 0.08870967741935484319, 0.09139784946236559349, 0.09408602150537634379, 0.09677419354838709409, 0.09946236559139784439, 0.1021505376344086086, 0.1048387096774193589, 0.1075268817204301092, 0.1102150537634408595, 0.1129032258064516098, 0.1155913978494623601, 0.1182795698924731242, 0.1209677419354838745, 0.1236559139784946248, 0.1263440860215053752, 0.1290322580645161255, 0.1317204301075268758, 0.1344086021505376261, 0.1370967741935483764, 0.1397849462365591267, 0.1424731182795699047, 0.1451612903225806550, 0.1478494623655914053, 0.1505376344086021556, 0.1532258064516129059, 0.1559139784946236562, 0.1586021505376344065, 0.1612903225806451568, 0.1639784946236559071, 0.1666666666666666574, 0.1693548387096774077, 0.1720430107526881858, 0.1747311827956989361, 0.1774193548387096864, 0.1801075268817204367, 0.1827956989247311870, 0.1854838709677419373, 0.1881720430107526876, 0.1908602150537634379, 0.1935483870967741882, 0.1962365591397849385, 0.1989247311827956888, 0.2016129032258064391, 0.2043010752688172171, 0.2069892473118279674, 0.2096774193548387177, 0.2123655913978494680, 0.2150537634408602183, 0.2177419354838709686, 0.2204301075268817189, 0.2231182795698924692, 0.2258064516129032195, 0.2284946236559139698, 0.2311827956989247201, 0.2338709677419354704, 0.2365591397849462485, 0.2392473118279569988, 0.2419354838709677491, 0.2446236559139784994, 0.2473118279569892497, 0.2500000000000000000, 0.2526881720430107503, 0.2553763440860215006, 0.2580645161290322509, 0.2607526881720430012, 0.2634408602150537515, 0.2661290322580645018, 0.2688172043010752521, 0.2715053763440860024, 0.2741935483870967527, 0.2768817204301075030, 0.2795698924731182533, 0.2822580645161290591, 0.2849462365591398094, 0.2876344086021505597, 0.2903225806451613100, 0.2930107526881720603, 0.2956989247311828106, 0.2983870967741935609, 0.3010752688172043112, 0.3037634408602150615, 0.3064516129032258118, 0.3091397849462365621, 0.3118279569892473124, 0.3145161290322580627, 0.3172043010752688130, 0.3198924731182795633, 0.3225806451612903136, 0.3252688172043010639, 0.3279569892473118142, 0.3306451612903225645, 0.3333333333333333148, 0.3360215053763440651, 0.3387096774193548154, 0.3413978494623655657, 0.3440860215053763715, 0.3467741935483871218, 0.3494623655913978721, 0.3521505376344086224, 0.3548387096774193727, 0.3575268817204301230, 0.3602150537634408733, 0.3629032258064516236, 0.3655913978494623739, 0.3682795698924731242, 0.3709677419354838745, 0.3736559139784946248, 0.3763440860215053752, 0.3790322580645161255, 0.3817204301075268758, 0.3844086021505376261, 0.3870967741935483764, 0.3897849462365591267, 0.3924731182795698770, 0.3951612903225806273, 0.3978494623655913776, 0.4005376344086021279, 0.4032258064516128782, 0.4059139784946236285, 0.4086021505376344343, 0.4112903225806451846, 0.4139784946236559349, 0.4166666666666666852, 0.4193548387096774355, 0.4220430107526881858, 0.4247311827956989361, 0.4274193548387096864, 0.4301075268817204367, 0.4327956989247311870, 0.4354838709677419373, 0.4381720430107526876, 0.4408602150537634379, 0.4435483870967741882, 0.4462365591397849385, 0.4489247311827956888, 0.4516129032258064391, 0.4543010752688171894, 0.4569892473118279397, 0.4596774193548386900, 0.4623655913978494403, 0.4650537634408601906, 0.4677419354838709409, 0.4704301075268817467, 0.4731182795698924970, 0.4758064516129032473, 0.4784946236559139976, 0.4811827956989247479, 0.4838709677419354982, 0.4865591397849462485, 0.4892473118279569988, 0.4919354838709677491, 0.4946236559139784994, 0.4973118279569892497, 0.5000000000000000000, 0.5026881720430107503, 0.5053763440860215006, 0.5080645161290322509, 0.5107526881720430012, 0.5134408602150537515, 0.5161290322580645018, 0.5188172043010752521, 0.5215053763440860024, 0.5241935483870967527, 0.5268817204301075030, 0.5295698924731182533, 0.5322580645161290036, 0.5349462365591397539, 0.5376344086021505042, 0.5403225806451612545, 0.5430107526881720048, 0.5456989247311827551, 0.5483870967741935054, 0.5510752688172042557, 0.5537634408602150060, 0.5564516129032257563, 0.5591397849462365066, 0.5618279569892472569, 0.5645161290322581182, 0.5672043010752688685, 0.5698924731182796188, 0.5725806451612903691, 0.5752688172043011194, 0.5779569892473118697, 0.5806451612903226200, 0.5833333333333333703, 0.5860215053763441206, 0.5887096774193548709, 0.5913978494623656212, 0.5940860215053763715, 0.5967741935483871218, 0.5994623655913978721, 0.6021505376344086224, 0.6048387096774193727, 0.6075268817204301230, 0.6102150537634408733, 0.6129032258064516236, 0.6155913978494623739, 0.6182795698924731242, 0.6209677419354838745, 0.6236559139784946248, 0.6263440860215053752, 0.6290322580645161255, 0.6317204301075268758, 0.6344086021505376261, 0.6370967741935483764, 0.6397849462365591267, 0.6424731182795698770, 0.6451612903225806273, 0.6478494623655913776, 0.6505376344086021279, 0.6532258064516128782, 0.6559139784946236285, 0.6586021505376343788, 0.6612903225806451291, 0.6639784946236558794, 0.6666666666666666297, 0.6693548387096773800, 0.6720430107526881303, 0.6747311827956988806, 0.6774193548387096309, 0.6801075268817203812, 0.6827956989247311315, 0.6854838709677418818, 0.6881720430107527431, 0.6908602150537634934, 0.6935483870967742437, 0.6962365591397849940, 0.6989247311827957443, 0.7016129032258064946, 0.7043010752688172449, 0.7069892473118279952, 0.7096774193548387455, 0.7123655913978494958, 0.7150537634408602461, 0.7177419354838709964, 0.7204301075268817467, 0.7231182795698924970, 0.7258064516129032473, 0.7284946236559139976, 0.7311827956989247479, 0.7338709677419354982, 0.7365591397849462485, 0.7392473118279569988, 0.7419354838709677491, 0.7446236559139784994, 0.7473118279569892497, 0.7500000000000000000, 0.7526881720430107503, 0.7553763440860215006, 0.7580645161290322509, 0.7607526881720430012, 0.7634408602150537515, 0.7661290322580645018, 0.7688172043010752521, 0.7715053763440860024, 0.7741935483870967527, 0.7768817204301075030, 0.7795698924731182533, 0.7822580645161290036, 0.7849462365591397539, 0.7876344086021505042, 0.7903225806451612545, 0.7930107526881720048, 0.7956989247311827551, 0.7983870967741935054, 0.8010752688172042557, 0.8037634408602150060, 0.8064516129032257563, 0.8091397849462365066, 0.8118279569892472569, 0.8145161290322581182, 0.8172043010752688685, 0.8198924731182796188, 0.8225806451612903691, 0.8252688172043011194, 0.8279569892473118697, 0.8306451612903226200, 0.8333333333333333703, 0.8360215053763441206, 0.8387096774193548709, 0.8413978494623656212, 0.8440860215053763715, 0.8467741935483871218, 0.8494623655913978721, 0.8521505376344086224, 0.8548387096774193727, 0.8575268817204301230, 0.8602150537634408733, 0.8629032258064516236, 0.8655913978494623739, 0.8682795698924731242, 0.8709677419354838745, 0.8736559139784946248, 0.8763440860215053752, 0.8790322580645161255, 0.8817204301075268758, 0.8844086021505376261, 0.8870967741935483764, 0.8897849462365591267, 0.8924731182795698770, 0.8951612903225806273, 0.8978494623655913776, 0.9005376344086021279, 0.9032258064516128782, 0.9059139784946236285, 0.9086021505376343788, 0.9112903225806451291, 0.9139784946236558794, 0.9166666666666666297, 0.9193548387096773800, 0.9220430107526881303, 0.9247311827956988806, 0.9274193548387096309, 0.9301075268817203812, 0.9327956989247311315, 0.9354838709677418818, 0.9381720430107527431, 0.9408602150537634934, 0.9435483870967742437, 0.9462365591397849940, 0.9489247311827957443, 0.9516129032258064946, 0.9543010752688172449, 0.9569892473118279952, 0.9596774193548387455, 0.9623655913978494958, 0.9650537634408602461, 0.9677419354838709964, 0.9704301075268817467, 0.9731182795698924970, 0.9758064516129032473, 0.9784946236559139976, 0.9811827956989247479, 0.9838709677419354982, 0.9865591397849462485, 0.9892473118279569988, 0.9919354838709677491, 0.9946236559139784994, 0.9973118279569892497, 1.000000000000000000 ),
 .UNSPECIFIED. ) 
 GEOMETRIC_REPRESENTATION_ITEM ( )  RATIONAL_B_SPLINE_SURFACE ( (
 ( 1.000000000000000000, 0.8660254037844387076, 1.000000000000000000, 0.8660254037844387076, 1.000000000000000000, 0.8660254037844387076, 1.000000000000000000, 0.8660254037844387076, 1.000000000000000000, 0.8660254037844387076, 1.000000000000000000, 0.8660254037844387076, 1.000000000000000000, 0.8660254037844387076, 1.000000000000000000, 0.8660254037844387076, 1.000000000000000000, 0.8660254037844387076, 1.000000000000000000, 0.8660254037844387076, 1.000000000000000000, 0.8660254037844387076, 1.000000000000000000, 0.8660254037844387076, 1.000000000000000000, 0.8660254037844387076, 1.000000000000000000, 0.8660254037844387076, 1.000000000000000000, 0.8660254037844387076, 1.000000000000000000, 0.8660254037844387076, 1.000000000000000000, 0.8660254037844387076, 1.000000000000000000, 0.8660254037844387076, 1.000000000000000000, 0.8660254037844387076, 1.000000000000000000, 0.8660254037844387076, 1.000000000000000000, 0.8660254037844387076, 1.000000000000000000, 0.8660254037844387076, 1.000000000000000000, 0.8660254037844387076, 1.000000000000000000, 0.8660254037844387076, 1.000000000000000000, 0.8660254037844387076, 1.000000000000000000, 0.8660254037844387076, 1.000000000000000000, 0.8660254037844387076, 1.000000000000000000, 0.8660254037844387076, 1.000000000000000000, 0.8660254037844387076, 1.000000000000000000, 0.8660254037844387076, 1.000000000000000000, 0.8660254037844387076, 1.000000000000000000, 0.8660254037844387076, 1.000000000000000000, 0.8660254037844387076, 1.000000000000000000, 0.8660254037844387076, 1.000000000000000000, 0.8660254037844387076, 1.000000000000000000, 0.8660254037844387076, 1.000000000000000000, 0.8660254037844387076, 1.000000000000000000, 0.8660254037844387076, 1.000000000000000000, 0.8660254037844387076, 1.000000000000000000, 0.8660254037844387076, 1.000000000000000000, 0.8660254037844387076, 1.000000000000000000, 0.8660254037844387076, 1.000000000000000000, 0.8660254037844387076, 1.000000000000000000, 0.8660254037844387076, 1.000000000000000000, 0.8660254037844387076, 1.000000000000000000, 0.8660254037844387076, 1.000000000000000000, 0.8660254037844387076, 1.000000000000000000, 0.8660254037844387076, 1.000000000000000000, 0.8660254037844387076, 1.000000000000000000, 0.8660254037844387076, 1.000000000000000000, 0.8660254037844387076, 1.000000000000000000, 0.8660254037844387076, 1.000000000000000000, 0.8660254037844387076, 1.000000000000000000, 0.8660254037844387076, 1.000000000000000000, 0.8660254037844387076, 1.000000000000000000, 0.8660254037844387076, 1.000000000000000000, 0.8660254037844387076, 1.000000000000000000, 0.8660254037844387076, 1.000000000000000000, 0.8660254037844387076, 1.000000000000000000, 0.8660254037844387076, 1.000000000000000000, 0.8660254037844387076, 1.000000000000000000, 0.8660254037844387076, 1.000000000000000000, 0.8660254037844387076, 1.000000000000000000, 0.8660254037844387076, 1.000000000000000000, 0.8660254037844387076, 1.000000000000000000, 0.8660254037844387076, 1.000000000000000000, 0.8660254037844387076, 1.000000000000000000, 0.8660254037844387076, 1.000000000000000000, 0.8660254037844387076, 1.000000000000000000, 0.8660254037844387076, 1.000000000000000000, 0.8660254037844387076, 1.000000000000000000, 0.8660254037844387076, 1.000000000000000000, 0.8660254037844387076, 1.000000000000000000, 0.8660254037844387076, 1.000000000000000000, 0.8660254037844387076, 1.000000000000000000, 0.8660254037844387076, 1.000000000000000000, 0.8660254037844387076, 1.000000000000000000, 0.8660254037844387076, 1.000000000000000000, 0.8660254037844387076, 1.000000000000000000, 0.8660254037844387076, 1.000000000000000000, 0.8660254037844387076, 1.000000000000000000, 0.8660254037844387076, 1.000000000000000000, 0.8660254037844387076, 1.000000000000000000, 0.8660254037844387076, 1.000000000000000000, 0.8660254037844387076, 1.000000000000000000, 0.8660254037844387076, 1.000000000000000000, 0.8660254037844387076, 1.000000000000000000, 0.8660254037844387076, 1.000000000000000000, 0.8660254037844387076, 1.000000000000000000, 0.8660254037844387076, 1.000000000000000000, 0.8660254037844387076, 1.000000000000000000, 0.8660254037844387076, 1.000000000000000000, 0.8660254037844387076, 1.000000000000000000, 0.8660254037844387076, 1.000000000000000000, 0.8660254037844387076, 1.000000000000000000, 0.8660254037844387076, 1.000000000000000000, 0.8660254037844387076, 1.000000000000000000, 0.8660254037844387076, 1.000000000000000000, 0.8660254037844387076, 1.000000000000000000, 0.8660254037844387076, 1.000000000000000000, 0.8660254037844387076, 1.000000000000000000, 0.8660254037844387076, 1.000000000000000000, 0.8660254037844387076, 1.000000000000000000, 0.8660254037844387076, 1.000000000000000000, 0.8660254037844387076, 1.000000000000000000, 0.8660254037844387076, 1.000000000000000000, 0.8660254037844387076, 1.000000000000000000, 0.8660254037844387076, 1.000000000000000000, 0.8660254037844387076, 1.000000000000000000, 0.8660254037844387076, 1.000000000000000000, 0.8660254037844387076, 1.000000000000000000, 0.8660254037844387076, 1.000000000000000000, 0.8660254037844387076, 1.000000000000000000, 0.8660254037844387076, 1.000000000000000000, 0.8660254037844387076, 1.000000000000000000, 0.8660254037844387076, 1.000000000000000000, 0.8660254037844387076, 1.000000000000000000, 0.8660254037844387076, 1.000000000000000000, 0.8660254037844387076, 1.000000000000000000, 0.8660254037844387076, 1.000000000000000000, 0.8660254037844387076, 1.000000000000000000, 0.8660254037844387076, 1.000000000000000000, 0.8660254037844387076, 1.000000000000000000, 0.8660254037844387076, 1.000000000000000000, 0.8660254037844387076, 1.000000000000000000, 0.8660254037844387076, 1.000000000000000000, 0.8660254037844387076, 1.000000000000000000, 0.8660254037844387076, 1.000000000000000000, 0.8660254037844387076, 1.000000000000000000, 0.8660254037844387076, 1.000000000000000000, 0.8660254037844387076, 1.000000000000000000, 0.8660254037844387076, 1.000000000000000000, 0.8660254037844387076, 1.000000000000000000, 0.8660254037844387076, 1.000000000000000000, 0.8660254037844387076, 1.000000000000000000, 0.8660254037844387076, 1.000000000000000000, 0.8660254037844387076, 1.000000000000000000, 0.8660254037844387076, 1.000000000000000000, 0.8660254037844387076, 1.000000000000000000, 0.8660254037844387076, 1.000000000000000000, 0.8660254037844387076, 1.000000000000000000, 0.8660254037844387076, 1.000000000000000000, 0.8660254037844387076, 1.000000000000000000, 0.8660254037844387076, 1.000000000000000000, 0.8660254037844387076, 1.000000000000000000, 0.8660254037844387076, 1.000000000000000000, 0.8660254037844387076, 1.000000000000000000, 0.8660254037844387076, 1.000000000000000000, 0.8660254037844387076, 1.000000000000000000, 0.8660254037844387076, 1.000000000000000000, 0.8660254037844387076, 1.000000000000000000, 0.8660254037844387076, 1.000000000000000000, 0.8660254037844387076, 1.000000000000000000, 0.8660254037844387076, 1.000000000000000000, 0.8660254037844387076, 1.000000000000000000, 0.8660254037844387076, 1.000000000000000000, 0.8660254037844387076, 1.000000000000000000, 0.8660254037844387076, 1.000000000000000000, 0.8660254037844387076, 1.000000000000000000, 0.8660254037844387076, 1.000000000000000000, 0.8660254037844387076, 1.000000000000000000, 0.8660254037844387076, 1.000000000000000000, 0.8660254037844387076, 1.000000000000000000, 0.8660254037844387076, 1.000000000000000000, 0.8660254037844387076, 1.000000000000000000, 0.8660254037844387076, 1.000000000000000000, 0.8660254037844387076, 1.000000000000000000, 0.8660254037844387076, 1.000000000000000000, 0.8660254037844387076, 1.000000000000000000, 0.8660254037844387076, 1.000000000000000000, 0.8660254037844387076, 1.000000000000000000, 0.8660254037844387076, 1.000000000000000000, 0.8660254037844387076, 1.000000000000000000, 0.8660254037844387076, 1.000000000000000000, 0.8660254037844387076, 1.000000000000000000, 0.8660254037844387076, 1.000000000000000000, 0.8660254037844387076, 1.000000000000000000, 0.8660254037844387076, 1.000000000000000000, 0.8660254037844387076, 1.000000000000000000, 0.8660254037844387076, 1.000000000000000000, 0.8660254037844387076, 1.000000000000000000, 0.8660254037844387076, 1.000000000000000000, 0.8660254037844387076, 1.000000000000000000, 0.8660254037844387076, 1.000000000000000000, 0.8660254037844387076, 1.000000000000000000, 0.8660254037844387076, 1.000000000000000000, 0.8660254037844387076, 1.000000000000000000, 0.8660254037844387076, 1.000000000000000000, 0.8660254037844387076, 1.000000000000000000, 0.8660254037844387076, 1.000000000000000000, 0.8660254037844387076, 1.000000000000000000, 0.8660254037844387076, 1.000000000000000000, 0.8660254037844387076, 1.000000000000000000, 0.8660254037844387076, 1.000000000000000000, 0.8660254037844387076, 1.000000000000000000, 0.8660254037844387076, 1.000000000000000000, 0.8660254037844387076, 1.000000000000000000, 0.8660254037844387076, 1.000000000000000000, 0.8660254037844387076, 1.000000000000000000, 0.8660254037844387076, 1.000000000000000000, 0.8660254037844387076, 1.000000000000000000, 0.8660254037844387076, 1.000000000000000000, 0.8660254037844387076, 1.000000000000000000, 0.8660254037844387076, 1.000000000000000000, 0.8660254037844387076, 1.000000000000000000, 0.8660254037844387076, 1.000000000000000000, 0.8660254037844387076, 1.000000000000000000, 0.8660254037844387076, 1.000000000000000000, 0.8660254037844387076, 1.000000000000000000, 0.8660254037844387076, 1.000000000000000000, 0.8660254037844387076, 1.000000000000000000, 0.8660254037844387076, 1.000000000000000000, 0.8660254037844387076, 1.000000000000000000, 0.8660254037844387076, 1.000000000000000000, 0.8660254037844387076, 1.000000000000000000, 0.8660254037844387076, 1.000000000000000000, 0.8660254037844387076, 1.000000000000000000, 0.8660254037844387076, 1.000000000000000000, 0.8660254037844387076, 1.000000000000000000, 0.8660254037844387076, 1.000000000000000000, 0.8660254037844387076, 1.000000000000000000, 0.8660254037844387076, 1.000000000000000000, 0.8660254037844387076, 1.000000000000000000, 0.8660254037844387076, 1.000000000000000000, 0.8660254037844387076, 1.000000000000000000, 0.8660254037844387076, 1.000000000000000000, 0.8660254037844387076, 1.000000000000000000, 0.8660254037844387076, 1.000000000000000000, 0.8660254037844387076, 1.000000000000000000, 0.8660254037844387076, 1.000000000000000000, 0.8660254037844387076, 1.000000000000000000, 0.8660254037844387076, 1.000000000000000000, 0.8660254037844387076, 1.000000000000000000, 0.8660254037844387076, 1.000000000000000000, 0.8660254037844387076, 1.000000000000000000, 0.8660254037844387076, 1.000000000000000000, 0.8660254037844387076, 1.000000000000000000, 0.8660254037844387076, 1.000000000000000000, 0.8660254037844387076, 1.000000000000000000, 0.8660254037844387076, 1.000000000000000000, 0.8660254037844387076, 1.000000000000000000, 0.8660254037844387076, 1.000000000000000000, 0.8660254037844387076, 1.000000000000000000, 0.8660254037844387076, 1.000000000000000000, 0.8660254037844387076, 1.000000000000000000, 0.8660254037844387076, 1.000000000000000000, 0.8660254037844387076, 1.000000000000000000, 0.8660254037844387076, 1.000000000000000000, 0.8660254037844387076, 1.000000000000000000, 0.8660254037844387076, 1.000000000000000000, 0.8660254037844387076, 1.000000000000000000, 0.8660254037844387076, 1.000000000000000000, 0.8660254037844387076, 1.000000000000000000, 0.8660254037844387076, 1.000000000000000000, 0.8660254037844387076, 1.000000000000000000, 0.8660254037844387076, 1.000000000000000000, 0.8660254037844387076, 1.000000000000000000, 0.8660254037844387076, 1.000000000000000000, 0.8660254037844387076, 1.000000000000000000, 0.8660254037844387076, 1.000000000000000000, 0.8660254037844387076, 1.000000000000000000, 0.8660254037844387076, 1.000000000000000000, 0.8660254037844387076, 1.000000000000000000, 0.8660254037844387076, 1.000000000000000000, 0.8660254037844387076, 1.000000000000000000, 0.8660254037844387076, 1.000000000000000000, 0.8660254037844387076, 1.000000000000000000, 0.8660254037844387076, 1.000000000000000000, 0.8660254037844387076, 1.000000000000000000, 0.8660254037844387076, 1.000000000000000000, 0.8660254037844387076, 1.000000000000000000, 0.8660254037844387076, 1.000000000000000000, 0.8660254037844387076, 1.000000000000000000, 0.8660254037844387076, 1.000000000000000000, 0.8660254037844387076, 1.000000000000000000, 0.8660254037844387076, 1.000000000000000000, 0.8660254037844387076, 1.000000000000000000, 0.8660254037844387076, 1.000000000000000000, 0.8660254037844387076, 1.000000000000000000, 0.8660254037844387076, 1.000000000000000000, 0.8660254037844387076, 1.000000000000000000, 0.8660254037844387076, 1.000000000000000000, 0.8660254037844387076, 1.000000000000000000, 0.8660254037844387076, 1.000000000000000000, 0.8660254037844387076, 1.000000000000000000, 0.8660254037844387076, 1.000000000000000000, 0.8660254037844387076, 1.000000000000000000, 0.8660254037844387076, 1.000000000000000000, 0.8660254037844387076, 1.000000000000000000, 0.8660254037844387076, 1.000000000000000000, 0.8660254037844387076, 1.000000000000000000, 0.8660254037844387076, 1.000000000000000000, 0.8660254037844387076, 1.000000000000000000, 0.8660254037844387076, 1.000000000000000000, 0.8660254037844387076, 1.000000000000000000, 0.8660254037844387076, 1.000000000000000000, 0.8660254037844387076, 1.000000000000000000, 0.8660254037844387076, 1.000000000000000000, 0.8660254037844387076, 1.000000000000000000, 0.8660254037844387076, 1.000000000000000000, 0.8660254037844387076, 1.000000000000000000, 0.8660254037844387076, 1.000000000000000000, 0.8660254037844387076, 1.000000000000000000, 0.8660254037844387076, 1.000000000000000000, 0.8660254037844387076, 1.000000000000000000, 0.8660254037844387076, 1.000000000000000000, 0.8660254037844387076, 1.000000000000000000, 0.8660254037844387076, 1.000000000000000000, 0.8660254037844387076, 1.000000000000000000, 0.8660254037844387076, 1.000000000000000000, 0.8660254037844387076, 1.000000000000000000, 0.8660254037844387076, 1.000000000000000000, 0.8660254037844387076, 1.000000000000000000, 0.8660254037844387076, 1.000000000000000000, 0.8660254037844387076, 1.000000000000000000, 0.8660254037844387076, 1.000000000000000000, 0.8660254037844387076, 1.000000000000000000, 0.8660254037844387076, 1.000000000000000000, 0.8660254037844387076, 1.000000000000000000, 0.8660254037844387076, 1.000000000000000000, 0.8660254037844387076, 1.000000000000000000, 0.8660254037844387076, 1.000000000000000000, 0.8660254037844387076, 1.000000000000000000, 0.8660254037844387076, 1.000000000000000000, 0.8660254037844387076, 1.000000000000000000, 0.8660254037844387076, 1.000000000000000000, 0.8660254037844387076, 1.000000000000000000, 0.8660254037844387076, 1.000000000000000000, 0.8660254037844387076, 1.000000000000000000, 0.8660254037844387076, 1.000000000000000000, 0.8660254037844387076, 1.000000000000000000, 0.8660254037844387076, 1.000000000000000000, 0.8660254037844387076, 1.000000000000000000, 0.8660254037844387076, 1.000000000000000000, 0.8660254037844387076, 1.000000000000000000, 0.8660254037844387076, 1.000000000000000000, 0.8660254037844387076, 1.000000000000000000, 0.8660254037844387076, 1.000000000000000000, 0.8660254037844387076, 1.000000000000000000, 0.8660254037844387076, 1.000000000000000000, 0.8660254037844387076, 1.000000000000000000, 0.8660254037844387076, 1.000000000000000000, 0.8660254037844387076, 1.000000000000000000, 0.8660254037844387076, 1.000000000000000000, 0.8660254037844387076, 1.000000000000000000, 0.8660254037844387076, 1.000000000000000000, 0.8660254037844387076, 1.000000000000000000, 0.8660254037844387076, 1.000000000000000000, 0.8660254037844387076, 1.000000000000000000, 0.8660254037844387076, 1.000000000000000000, 0.8660254037844387076, 1.000000000000000000, 0.8660254037844387076, 1.000000000000000000, 0.8660254037844387076, 1.000000000000000000, 0.8660254037844387076, 1.000000000000000000, 0.8660254037844387076, 1.000000000000000000, 0.8660254037844387076, 1.000000000000000000, 0.8660254037844387076, 1.000000000000000000, 0.8660254037844387076, 1.000000000000000000, 0.8660254037844387076, 1.000000000000000000, 0.8660254037844387076, 1.000000000000000000, 0.8660254037844387076, 1.000000000000000000, 0.8660254037844387076, 1.000000000000000000, 0.8660254037844387076, 1.000000000000000000, 0.8660254037844387076, 1.000000000000000000, 0.8660254037844387076, 1.000000000000000000, 0.8660254037844387076, 1.000000000000000000, 0.8660254037844387076, 1.000000000000000000, 0.8660254037844387076, 1.000000000000000000, 0.8660254037844387076, 1.000000000000000000, 0.8660254037844387076, 1.000000000000000000, 0.8660254037844387076, 1.000000000000000000, 0.8660254037844387076, 1.000000000000000000),
 ( 1.000000000000000000, 0.8660254037844387076, 1.000000000000000000, 0.8660254037844387076, 1.000000000000000000, 0.8660254037844387076, 1.000000000000000000, 0.8660254037844387076, 1.000000000000000000, 0.8660254037844387076, 1.000000000000000000, 0.8660254037844387076, 1.000000000000000000, 0.8660254037844387076, 1.000000000000000000, 0.8660254037844387076, 1.000000000000000000, 0.8660254037844387076, 1.000000000000000000, 0.8660254037844387076, 1.000000000000000000, 0.8660254037844387076, 1.000000000000000000, 0.8660254037844387076, 1.000000000000000000, 0.8660254037844387076, 1.000000000000000000, 0.8660254037844387076, 1.000000000000000000, 0.8660254037844387076, 1.000000000000000000, 0.8660254037844387076, 1.000000000000000000, 0.8660254037844387076, 1.000000000000000000, 0.8660254037844387076, 1.000000000000000000, 0.8660254037844387076, 1.000000000000000000, 0.8660254037844387076, 1.000000000000000000, 0.8660254037844387076, 1.000000000000000000, 0.8660254037844387076, 1.000000000000000000, 0.8660254037844387076, 1.000000000000000000, 0.8660254037844387076, 1.000000000000000000, 0.8660254037844387076, 1.000000000000000000, 0.8660254037844387076, 1.000000000000000000, 0.8660254037844387076, 1.000000000000000000, 0.8660254037844387076, 1.000000000000000000, 0.8660254037844387076, 1.000000000000000000, 0.8660254037844387076, 1.000000000000000000, 0.8660254037844387076, 1.000000000000000000, 0.8660254037844387076, 1.000000000000000000, 0.8660254037844387076, 1.000000000000000000, 0.8660254037844387076, 1.000000000000000000, 0.8660254037844387076, 1.000000000000000000, 0.8660254037844387076, 1.000000000000000000, 0.8660254037844387076, 1.000000000000000000, 0.8660254037844387076, 1.000000000000000000, 0.8660254037844387076, 1.000000000000000000, 0.8660254037844387076, 1.000000000000000000, 0.8660254037844387076, 1.000000000000000000, 0.8660254037844387076, 1.000000000000000000, 0.8660254037844387076, 1.000000000000000000, 0.8660254037844387076, 1.000000000000000000, 0.8660254037844387076, 1.000000000000000000, 0.8660254037844387076, 1.000000000000000000, 0.8660254037844387076, 1.000000000000000000, 0.8660254037844387076, 1.000000000000000000, 0.8660254037844387076, 1.000000000000000000, 0.8660254037844387076, 1.000000000000000000, 0.8660254037844387076, 1.000000000000000000, 0.8660254037844387076, 1.000000000000000000, 0.8660254037844387076, 1.000000000000000000, 0.8660254037844387076, 1.000000000000000000, 0.8660254037844387076, 1.000000000000000000, 0.8660254037844387076, 1.000000000000000000, 0.8660254037844387076, 1.000000000000000000, 0.8660254037844387076, 1.000000000000000000, 0.8660254037844387076, 1.000000000000000000, 0.8660254037844387076, 1.000000000000000000, 0.8660254037844387076, 1.000000000000000000, 0.8660254037844387076, 1.000000000000000000, 0.8660254037844387076, 1.000000000000000000, 0.8660254037844387076, 1.000000000000000000, 0.8660254037844387076, 1.000000000000000000, 0.8660254037844387076, 1.000000000000000000, 0.8660254037844387076, 1.000000000000000000, 0.8660254037844387076, 1.000000000000000000, 0.8660254037844387076, 1.000000000000000000, 0.8660254037844387076, 1.000000000000000000, 0.8660254037844387076, 1.000000000000000000, 0.8660254037844387076, 1.000000000000000000, 0.8660254037844387076, 1.000000000000000000, 0.8660254037844387076, 1.000000000000000000, 0.8660254037844387076, 1.000000000000000000, 0.8660254037844387076, 1.000000000000000000, 0.8660254037844387076, 1.000000000000000000, 0.8660254037844387076, 1.000000000000000000, 0.8660254037844387076, 1.000000000000000000, 0.8660254037844387076, 1.000000000000000000, 0.8660254037844387076, 1.000000000000000000, 0.8660254037844387076, 1.000000000000000000, 0.8660254037844387076, 1.000000000000000000, 0.8660254037844387076, 1.000000000000000000, 0.8660254037844387076, 1.000000000000000000, 0.8660254037844387076, 1.000000000000000000, 0.8660254037844387076, 1.000000000000000000, 0.8660254037844387076, 1.000000000000000000, 0.8660254037844387076, 1.000000000000000000, 0.8660254037844387076, 1.000000000000000000, 0.8660254037844387076, 1.000000000000000000, 0.8660254037844387076, 1.000000000000000000, 0.8660254037844387076, 1.000000000000000000, 0.8660254037844387076, 1.000000000000000000, 0.8660254037844387076, 1.000000000000000000, 0.8660254037844387076, 1.000000000000000000, 0.8660254037844387076, 1.000000000000000000, 0.8660254037844387076, 1.000000000000000000, 0.8660254037844387076, 1.000000000000000000, 0.8660254037844387076, 1.000000000000000000, 0.8660254037844387076, 1.000000000000000000, 0.8660254037844387076, 1.000000000000000000, 0.8660254037844387076, 1.000000000000000000, 0.8660254037844387076, 1.000000000000000000, 0.8660254037844387076, 1.000000000000000000, 0.8660254037844387076, 1.000000000000000000, 0.8660254037844387076, 1.000000000000000000, 0.8660254037844387076, 1.000000000000000000, 0.8660254037844387076, 1.000000000000000000, 0.8660254037844387076, 1.000000000000000000, 0.8660254037844387076, 1.000000000000000000, 0.8660254037844387076, 1.000000000000000000, 0.8660254037844387076, 1.000000000000000000, 0.8660254037844387076, 1.000000000000000000, 0.8660254037844387076, 1.000000000000000000, 0.8660254037844387076, 1.000000000000000000, 0.8660254037844387076, 1.000000000000000000, 0.8660254037844387076, 1.000000000000000000, 0.8660254037844387076, 1.000000000000000000, 0.8660254037844387076, 1.000000000000000000, 0.8660254037844387076, 1.000000000000000000, 0.8660254037844387076, 1.000000000000000000, 0.8660254037844387076, 1.000000000000000000, 0.8660254037844387076, 1.000000000000000000, 0.8660254037844387076, 1.000000000000000000, 0.8660254037844387076, 1.000000000000000000, 0.8660254037844387076, 1.000000000000000000, 0.8660254037844387076, 1.000000000000000000, 0.8660254037844387076, 1.000000000000000000, 0.8660254037844387076, 1.000000000000000000, 0.8660254037844387076, 1.000000000000000000, 0.8660254037844387076, 1.000000000000000000, 0.8660254037844387076, 1.000000000000000000, 0.8660254037844387076, 1.000000000000000000, 0.8660254037844387076, 1.000000000000000000, 0.8660254037844387076, 1.000000000000000000, 0.8660254037844387076, 1.000000000000000000, 0.8660254037844387076, 1.000000000000000000, 0.8660254037844387076, 1.000000000000000000, 0.8660254037844387076, 1.000000000000000000, 0.8660254037844387076, 1.000000000000000000, 0.8660254037844387076, 1.000000000000000000, 0.8660254037844387076, 1.000000000000000000, 0.8660254037844387076, 1.000000000000000000, 0.8660254037844387076, 1.000000000000000000, 0.8660254037844387076, 1.000000000000000000, 0.8660254037844387076, 1.000000000000000000, 0.8660254037844387076, 1.000000000000000000, 0.8660254037844387076, 1.000000000000000000, 0.8660254037844387076, 1.000000000000000000, 0.8660254037844387076, 1.000000000000000000, 0.8660254037844387076, 1.000000000000000000, 0.8660254037844387076, 1.000000000000000000, 0.8660254037844387076, 1.000000000000000000, 0.8660254037844387076, 1.000000000000000000, 0.8660254037844387076, 1.000000000000000000, 0.8660254037844387076, 1.000000000000000000, 0.8660254037844387076, 1.000000000000000000, 0.8660254037844387076, 1.000000000000000000, 0.8660254037844387076, 1.000000000000000000, 0.8660254037844387076, 1.000000000000000000, 0.8660254037844387076, 1.000000000000000000, 0.8660254037844387076, 1.000000000000000000, 0.8660254037844387076, 1.000000000000000000, 0.8660254037844387076, 1.000000000000000000, 0.8660254037844387076, 1.000000000000000000, 0.8660254037844387076, 1.000000000000000000, 0.8660254037844387076, 1.000000000000000000, 0.8660254037844387076, 1.000000000000000000, 0.8660254037844387076, 1.000000000000000000, 0.8660254037844387076, 1.000000000000000000, 0.8660254037844387076, 1.000000000000000000, 0.8660254037844387076, 1.000000000000000000, 0.8660254037844387076, 1.000000000000000000, 0.8660254037844387076, 1.000000000000000000, 0.8660254037844387076, 1.000000000000000000, 0.8660254037844387076, 1.000000000000000000, 0.8660254037844387076, 1.000000000000000000, 0.8660254037844387076, 1.000000000000000000, 0.8660254037844387076, 1.000000000000000000, 0.8660254037844387076, 1.000000000000000000, 0.8660254037844387076, 1.000000000000000000, 0.8660254037844387076, 1.000000000000000000, 0.8660254037844387076, 1.000000000000000000, 0.8660254037844387076, 1.000000000000000000, 0.8660254037844387076, 1.000000000000000000, 0.8660254037844387076, 1.000000000000000000, 0.8660254037844387076, 1.000000000000000000, 0.8660254037844387076, 1.000000000000000000, 0.8660254037844387076, 1.000000000000000000, 0.8660254037844387076, 1.000000000000000000, 0.8660254037844387076, 1.000000000000000000, 0.8660254037844387076, 1.000000000000000000, 0.8660254037844387076, 1.000000000000000000, 0.8660254037844387076, 1.000000000000000000, 0.8660254037844387076, 1.000000000000000000, 0.8660254037844387076, 1.000000000000000000, 0.8660254037844387076, 1.000000000000000000, 0.8660254037844387076, 1.000000000000000000, 0.8660254037844387076, 1.000000000000000000, 0.8660254037844387076, 1.000000000000000000, 0.8660254037844387076, 1.000000000000000000, 0.8660254037844387076, 1.000000000000000000, 0.8660254037844387076, 1.000000000000000000, 0.8660254037844387076, 1.000000000000000000, 0.8660254037844387076, 1.000000000000000000, 0.8660254037844387076, 1.000000000000000000, 0.8660254037844387076, 1.000000000000000000, 0.8660254037844387076, 1.000000000000000000, 0.8660254037844387076, 1.000000000000000000, 0.8660254037844387076, 1.000000000000000000, 0.8660254037844387076, 1.000000000000000000, 0.8660254037844387076, 1.000000000000000000, 0.8660254037844387076, 1.000000000000000000, 0.8660254037844387076, 1.000000000000000000, 0.8660254037844387076, 1.000000000000000000, 0.8660254037844387076, 1.000000000000000000, 0.8660254037844387076, 1.000000000000000000, 0.8660254037844387076, 1.000000000000000000, 0.8660254037844387076, 1.000000000000000000, 0.8660254037844387076, 1.000000000000000000, 0.8660254037844387076, 1.000000000000000000, 0.8660254037844387076, 1.000000000000000000, 0.8660254037844387076, 1.000000000000000000, 0.8660254037844387076, 1.000000000000000000, 0.8660254037844387076, 1.000000000000000000, 0.8660254037844387076, 1.000000000000000000, 0.8660254037844387076, 1.000000000000000000, 0.8660254037844387076, 1.000000000000000000, 0.8660254037844387076, 1.000000000000000000, 0.8660254037844387076, 1.000000000000000000, 0.8660254037844387076, 1.000000000000000000, 0.8660254037844387076, 1.000000000000000000, 0.8660254037844387076, 1.000000000000000000, 0.8660254037844387076, 1.000000000000000000, 0.8660254037844387076, 1.000000000000000000, 0.8660254037844387076, 1.000000000000000000, 0.8660254037844387076, 1.000000000000000000, 0.8660254037844387076, 1.000000000000000000, 0.8660254037844387076, 1.000000000000000000, 0.8660254037844387076, 1.000000000000000000, 0.8660254037844387076, 1.000000000000000000, 0.8660254037844387076, 1.000000000000000000, 0.8660254037844387076, 1.000000000000000000, 0.8660254037844387076, 1.000000000000000000, 0.8660254037844387076, 1.000000000000000000, 0.8660254037844387076, 1.000000000000000000, 0.8660254037844387076, 1.000000000000000000, 0.8660254037844387076, 1.000000000000000000, 0.8660254037844387076, 1.000000000000000000, 0.8660254037844387076, 1.000000000000000000, 0.8660254037844387076, 1.000000000000000000, 0.8660254037844387076, 1.000000000000000000, 0.8660254037844387076, 1.000000000000000000, 0.8660254037844387076, 1.000000000000000000, 0.8660254037844387076, 1.000000000000000000, 0.8660254037844387076, 1.000000000000000000, 0.8660254037844387076, 1.000000000000000000, 0.8660254037844387076, 1.000000000000000000, 0.8660254037844387076, 1.000000000000000000, 0.8660254037844387076, 1.000000000000000000, 0.8660254037844387076, 1.000000000000000000, 0.8660254037844387076, 1.000000000000000000, 0.8660254037844387076, 1.000000000000000000, 0.8660254037844387076, 1.000000000000000000, 0.8660254037844387076, 1.000000000000000000, 0.8660254037844387076, 1.000000000000000000, 0.8660254037844387076, 1.000000000000000000, 0.8660254037844387076, 1.000000000000000000, 0.8660254037844387076, 1.000000000000000000, 0.8660254037844387076, 1.000000000000000000, 0.8660254037844387076, 1.000000000000000000, 0.8660254037844387076, 1.000000000000000000, 0.8660254037844387076, 1.000000000000000000, 0.8660254037844387076, 1.000000000000000000, 0.8660254037844387076, 1.000000000000000000, 0.8660254037844387076, 1.000000000000000000, 0.8660254037844387076, 1.000000000000000000, 0.8660254037844387076, 1.000000000000000000, 0.8660254037844387076, 1.000000000000000000, 0.8660254037844387076, 1.000000000000000000, 0.8660254037844387076, 1.000000000000000000, 0.8660254037844387076, 1.000000000000000000, 0.8660254037844387076, 1.000000000000000000, 0.8660254037844387076, 1.000000000000000000, 0.8660254037844387076, 1.000000000000000000, 0.8660254037844387076, 1.000000000000000000, 0.8660254037844387076, 1.000000000000000000, 0.8660254037844387076, 1.000000000000000000, 0.8660254037844387076, 1.000000000000000000, 0.8660254037844387076, 1.000000000000000000, 0.8660254037844387076, 1.000000000000000000, 0.8660254037844387076, 1.000000000000000000, 0.8660254037844387076, 1.000000000000000000, 0.8660254037844387076, 1.000000000000000000, 0.8660254037844387076, 1.000000000000000000, 0.8660254037844387076, 1.000000000000000000, 0.8660254037844387076, 1.000000000000000000, 0.8660254037844387076, 1.000000000000000000, 0.8660254037844387076, 1.000000000000000000, 0.8660254037844387076, 1.000000000000000000, 0.8660254037844387076, 1.000000000000000000, 0.8660254037844387076, 1.000000000000000000, 0.8660254037844387076, 1.000000000000000000, 0.8660254037844387076, 1.000000000000000000, 0.8660254037844387076, 1.000000000000000000, 0.8660254037844387076, 1.000000000000000000, 0.8660254037844387076, 1.000000000000000000, 0.8660254037844387076, 1.000000000000000000, 0.8660254037844387076, 1.000000000000000000, 0.8660254037844387076, 1.000000000000000000, 0.8660254037844387076, 1.000000000000000000, 0.8660254037844387076, 1.000000000000000000, 0.8660254037844387076, 1.000000000000000000, 0.8660254037844387076, 1.000000000000000000, 0.8660254037844387076, 1.000000000000000000, 0.8660254037844387076, 1.000000000000000000, 0.8660254037844387076, 1.000000000000000000, 0.8660254037844387076, 1.000000000000000000, 0.8660254037844387076, 1.000000000000000000, 0.8660254037844387076, 1.000000000000000000, 0.8660254037844387076, 1.000000000000000000, 0.8660254037844387076, 1.000000000000000000, 0.8660254037844387076, 1.000000000000000000, 0.8660254037844387076, 1.000000000000000000, 0.8660254037844387076, 1.000000000000000000, 0.8660254037844387076, 1.000000000000000000, 0.8660254037844387076, 1.000000000000000000, 0.8660254037844387076, 1.000000000000000000, 0.8660254037844387076, 1.000000000000000000, 0.8660254037844387076, 1.000000000000000000, 0.8660254037844387076, 1.000000000000000000, 0.8660254037844387076, 1.000000000000000000, 0.8660254037844387076, 1.000000000000000000, 0.8660254037844387076, 1.000000000000000000, 0.8660254037844387076, 1.000000000000000000, 0.8660254037844387076, 1.000000000000000000, 0.8660254037844387076, 1.000000000000000000, 0.8660254037844387076, 1.000000000000000000, 0.8660254037844387076, 1.000000000000000000, 0.8660254037844387076, 1.000000000000000000, 0.8660254037844387076, 1.000000000000000000, 0.8660254037844387076, 1.000000000000000000, 0.8660254037844387076, 1.000000000000000000, 0.8660254037844387076, 1.000000000000000000, 0.8660254037844387076, 1.000000000000000000, 0.8660254037844387076, 1.000000000000000000, 0.8660254037844387076, 1.000000000000000000, 0.8660254037844387076, 1.000000000000000000, 0.8660254037844387076, 1.000000000000000000, 0.8660254037844387076, 1.000000000000000000, 0.8660254037844387076, 1.000000000000000000, 0.8660254037844387076, 1.000000000000000000, 0.8660254037844387076, 1.000000000000000000, 0.8660254037844387076, 1.000000000000000000, 0.8660254037844387076, 1.000000000000000000, 0.8660254037844387076, 1.000000000000000000, 0.8660254037844387076, 1.000000000000000000, 0.8660254037844387076, 1.000000000000000000, 0.8660254037844387076, 1.000000000000000000, 0.8660254037844387076, 1.000000000000000000, 0.8660254037844387076, 1.000000000000000000, 0.8660254037844387076, 1.000000000000000000, 0.8660254037844387076, 1.000000000000000000, 0.8660254037844387076, 1.000000000000000000, 0.8660254037844387076, 1.000000000000000000, 0.8660254037844387076, 1.000000000000000000, 0.8660254037844387076, 1.000000000000000000, 0.8660254037844387076, 1.000000000000000000, 0.8660254037844387076, 1.000000000000000000, 0.8660254037844387076, 1.000000000000000000, 0.8660254037844387076, 1.000000000000000000) ) ) 
 REPRESENTATION_ITEM ( '' )  SURFACE ( )  );
#55485=VERTEX_POINT ( 'NONE', #87294 ) ;
#55486=CARTESIAN_POINT ( 'NONE',  ( 190.8222259996342700, 280.8384348826126597, 16.64285960788097896 ) ) ;
#55489=ORIENTED_EDGE ( 'NONE', *, *, #54135, .F. ) ;
#55490=CARTESIAN_POINT ( 'NONE',  ( 164.2656921623427593, 279.4100564649723992, 11.98912045511763047 ) ) ;
#55491=ADVANCED_FACE ( 'NONE', ( #17825 ), #72026, .T. ) ;
#55492=CARTESIAN_POINT ( 'NONE',  ( 194.3708539535661259, 293.9868007723104029, -16.01585187499628304 ) ) ;
#55497=CARTESIAN_POINT ( 'NONE',  ( 61.08237637342866577, 217.6199935810940644, 2.679491924311251605 ) ) ;
#55503=CARTESIAN_POINT ( 'NONE',  ( 194.9471474500919896, 290.9886311562445371, 16.55118206508679890 ) ) ;
#55510=CARTESIAN_POINT ( 'NONE',  ( 182.7187161720513870, 280.2422681844545309, -16.11425770197665130 ) ) ;
#55511=CARTESIAN_POINT ( 'NONE',  ( 206.7074763235984562, 272.6191440336236838, -10.69202547607624609 ) ) ;
#55512=CARTESIAN_POINT ( 'NONE',  ( 147.7698481346699566, 274.7021105344513217, -7.287563475572640392 ) ) ;
#55513=CARTESIAN_POINT ( 'NONE',  ( 198.7408816115379864, 285.9624092822338071, -17.04496721243561197 ) ) ;
#55517=ADVANCED_FACE ( 'NONE', ( #64413 ), #91102, .F. ) ;
#55519=CARTESIAN_POINT ( 'NONE',  ( 132.1361044793229951, 247.0958772461660544, -9.188101187500095079 ) ) ;
#55520=CARTESIAN_POINT ( 'NONE',  ( 186.4053619253457157, 262.6073444215381301, -9.037681140890068576 ) ) ;
#55522=ORIENTED_EDGE ( 'NONE', *, *, #63690, .T. ) ;
#55523=AXIS2_PLACEMENT_3D ( 'NONE', #15482, #23581, #8897 ) ;
#55524=CARTESIAN_POINT ( 'NONE',  ( 156.6168467568483891, 276.9391697405689001, 11.51099842983860633 ) ) ;
#55527=CARTESIAN_POINT ( 'NONE',  ( 178.6718079657368605, 253.5168414102466556, 1.418467519481931172 ) ) ;
#55528=CARTESIAN_POINT ( 'NONE',  ( 174.0958964869310819, 290.5965046355827326, -4.902034896575071521 ) ) ;
#55529=CARTESIAN_POINT ( 'NONE',  ( 190.3035812936891205, 300.3508029452809751, 2.075471296006329514 ) ) ;
#55532=CARTESIAN_POINT ( 'NONE',  ( 152.7295469705997277, 266.1116601603806657, -17.40211458100010589 ) ) ;
#55536=CARTESIAN_POINT ( 'NONE',  ( 177.5477342733873058, 255.5783683057051974, -8.395856749569729160 ) ) ;
#55537=ORIENTED_EDGE ( 'NONE', *, *, #47040, .T. ) ;
#55538=CARTESIAN_POINT ( 'NONE',  ( 147.7785919239399846, 274.6869658471848652, -7.924750738206837397 ) ) ;
#55540=AXIS2_PLACEMENT_3D ( 'NONE', #68687, #20621, #92055 ) ;
#55541=ORIENTED_EDGE ( 'NONE', *, *, #94392, .F. ) ;
#55542=CARTESIAN_POINT ( 'NONE',  ( 188.2574254122442028, 265.6453801167639313, -11.59643318832059222 ) ) ;
#55543=VECTOR ( 'NONE', #43297, 1000.000000000000000 ) ;
#55544=CARTESIAN_POINT ( 'NONE',  ( 191.0385514471091142, 283.4162394903332256, -16.57259208637104564 ) ) ;
#55545=CARTESIAN_POINT ( 'NONE',  ( 191.5041680634890326, 298.9520463832649284, -9.652406396186668402 ) ) ;
#55546=CARTESIAN_POINT ( 'NONE',  ( 185.2824853868734181, 297.7695098558858149, 4.231266468330407093 ) ) ;
#55547=CARTESIAN_POINT ( 'NONE',  ( 163.1332433029523372, 248.0919295262283981, 11.24052392390482957 ) ) ;
#55548=CARTESIAN_POINT ( 'NONE',  ( 153.3453455745885776, 270.2083751330562791, 14.04681399919192764 ) ) ;
#55549=CARTESIAN_POINT ( 'NONE',  ( 154.5748677679694651, 277.6768200149726908, -9.086954252033812907 ) ) ;
#55550=CARTESIAN_POINT ( 'NONE',  ( 200.3729394803074797, 267.3312977064779830, 6.351288650702686667 ) ) ;
#55552=CARTESIAN_POINT ( 'NONE',  ( 204.6993599598945650, 272.9423004453971089, -9.711292078056779076 ) ) ;
#55553=B_SPLINE_SURFACE_WITH_KNOTS ( 'NONE', 3, 1, ( 
 ( #42875, #59578 ),
 ( #90554, #20615 ),
 ( #73808, #28702 ),
 ( #43890, #74829 ),
 ( #66694, #58584 ),
 ( #20119, #73322 ),
 ( #51496, #50990 ),
 ( #11530, #60077 ),
 ( #4402, #82466 ),
 ( #98116, #65695 ),
 ( #27219, #12019 ),
 ( #52001, #21124 ),
 ( #35299, #97150 ),
 ( #67700, #91040 ),
 ( #66211, #5898 ),
 ( #13027, #81940 ),
 ( #75320, #5409 ),
 ( #21607, #27716 ),
 ( #34792, #98628 ),
 ( #28195, #82944 ),
 ( #19633, #29208 ),
 ( #13517, #52487 ),
 ( #96649, #12518 ),
 ( #44385, #42389 ),
 ( #3911, #43390 ),
 ( #74333, #58102 ),
 ( #89084, #50493 ),
 ( #81447, #4921 ),
 ( #35800, #59071 ),
 ( #90042, #36292 ),
 ( #67193, #38272 ),
 ( #62565, #22092 ),
 ( #70175, #53482 ),
 ( #6889, #52990 ) ),
 .UNSPECIFIED., .T., .F., .F.,
 ( 4, 2, 2, 2, 2, 2, 2, 2, 2, 2, 2, 2, 2, 2, 2, 2, 4 ),
 ( 2, 2 ),
 ( 0.000000000000000000, 0.06250000000000000000, 0.1250000000000000000, 0.1875000000000000000, 0.2500000000000000000, 0.3125000000000000000, 0.3750000000000000000, 0.4375000000000000000, 0.5000000000000000000, 0.5625000000000000000, 0.6250000000000000000, 0.6875000000000000000, 0.7500000000000000000, 0.8125000000000000000, 0.8750000000000000000, 0.9375000000000000000, 1.000000000000000000 ),
 ( 0.000000000000000000, 1.000000000000000000 ),
 .UNSPECIFIED. ) ;
#55554=CARTESIAN_POINT ( 'NONE',  ( 186.9700126462538776, 262.9196008017059398, -9.025915536625742419 ) ) ;
#55555=CARTESIAN_POINT ( 'NONE',  ( 154.2351116723865232, 278.9542530893276648, 6.640610626432363439 ) ) ;
#55556=CARTESIAN_POINT ( 'NONE',  ( 170.3290958195750022, 289.6815776661216546, -1.151831906498994140 ) ) ;
#55557=CARTESIAN_POINT ( 'NONE',  ( 152.6757560589063303, 266.2048287524194166, 16.73757896668104195 ) ) ;
#55559=CARTESIAN_POINT ( 'NONE',  ( 194.4889937320412230, 293.7821766735966662, 14.99892588346621380 ) ) ;
#55560=CYLINDRICAL_SURFACE ( 'NONE', #22305, 17.82106496071139645 ) ;
#55561=EDGE_CURVE ( 'NONE', #23462, #42521, #14375, .T. ) ;
#55563=CARTESIAN_POINT ( 'NONE',  ( 87.96880888631662287, 221.5958772461660544, -9.188101187500095079 ) ) ;
#55569=CARTESIAN_POINT ( 'NONE',  ( 125.9182562534771677, 255.0530062829863311, -4.648177544792955347E-16 ) ) ;
#55571=CARTESIAN_POINT ( 'NONE',  ( 190.2138197578740630, 300.4348890635282601, -1.218754932262906321 ) ) ;
#55573=CARTESIAN_POINT ( 'NONE',  ( 207.5768482435486817, 271.1133476975963390, 4.854912217663986951 ) ) ;
#55575=CARTESIAN_POINT ( 'NONE',  ( 166.5514548696166628, 250.1203565289131916, -8.987830393236849957 ) ) ;
#55576=CYLINDRICAL_SURFACE ( 'NONE', #1292, 17.82106496071139645 ) ;
#55577=CARTESIAN_POINT ( 'NONE',  ( 196.3519702320103590, 290.5554067223432639, 17.39042812051341969 ) ) ;
#55578=CARTESIAN_POINT ( 'NONE',  ( 190.0398248856338057, 298.8169614316505545, -8.166243001185458539 ) ) ;
#55580=CARTESIAN_POINT ( 'NONE',  ( 40.58072100116311276, 203.4244531367911293, -4.594050593750046652 ) ) ;
#55581=CARTESIAN_POINT ( 'NONE',  ( 68.45643432912224569, 201.1423013555409796, -4.594050593750043987 ) ) ;
#55584=CARTESIAN_POINT ( 'NONE',  ( 167.1156311472931861, 259.7982583194432777, 15.94551010330511787 ) ) ;
#55585=CARTESIAN_POINT ( 'NONE',  ( 198.6196860892239897, 286.2322653470183127, -17.00643444671568716 ) ) ;
#55586=CARTESIAN_POINT ( 'NONE',  ( 202.6833006059332263, 277.5892208352050829, 15.45935665133711900 ) ) ;
#55587=EDGE_CURVE ( 'NONE', #32613, #82087, #60005, .T. ) ;
#55588=CARTESIAN_POINT ( 'NONE',  ( 199.8052201840724820, 271.0811423415471495, -11.18866198556676927 ) ) ;
#55590=CARTESIAN_POINT ( 'NONE',  ( 198.7829547491859330, 286.3448180261817129, -18.59838968157616179 ) ) ;
#55593=CARTESIAN_POINT ( 'NONE',  ( 66.66973629016931113, 218.4869531367911293, 4.594050593750046652 ) ) ;
#55596=CARTESIAN_POINT ( 'NONE',  ( 198.5558597050348908, 286.7381581807989051, 17.16554469393394200 ) ) ;
#55598=CARTESIAN_POINT ( 'NONE',  ( 201.6857638146347256, 281.3170052401528665, 17.84391605515014945 ) ) ;
#55600=CARTESIAN_POINT ( 'NONE',  ( 109.2134945746776538, 223.8615022471902023, 5.000000000000051514 ) ) ;
#55601=CARTESIAN_POINT ( 'NONE',  ( 161.8016137473484548, 250.3983795733946636, 14.25000412375400316 ) ) ;
#55602=CARTESIAN_POINT ( 'NONE',  ( 164.5416088356626290, 245.6525688679454618, -1.463507744092769292 ) ) ;
#55603=ORIENTED_EDGE ( 'NONE', *, *, #94471, .T. ) ;
#55606=CARTESIAN_POINT ( 'NONE',  ( 186.0400780920065529, 271.7087950812899066, 16.90619359840448510 ) ) ;
#55608=CARTESIAN_POINT ( 'NONE',  ( 159.2102594322688844, 254.8867369075254885, -16.13039487917589199 ) ) ;
#55609=CARTESIAN_POINT ( 'NONE',  ( 181.8774662184618194, 285.1120569720015965, 15.89814067624403116 ) ) ;
#55613=CARTESIAN_POINT ( 'NONE',  ( 177.0706589053032474, 253.3103952305708617, -0.2596013527085206940 ) ) ;
#55617=CARTESIAN_POINT ( 'NONE',  ( 42.72800263476181470, 202.1427522451419350, 10.00000000000009415 ) ) ;
#55624=ORIENTED_EDGE ( 'NONE', *, *, #52802, .T. ) ;
#55627=ORIENTED_EDGE ( 'NONE', *, *, #77498, .F. ) ;
#55628=CARTESIAN_POINT ( 'NONE',  ( 186.0541232522963639, 298.0217281582578721, 1.045760341051833908 ) ) ;
#55629=CARTESIAN_POINT ( 'NONE',  ( 163.1340607412760448, 284.0498969924611856, -2.585094881414993218 ) ) ;
#55630=CARTESIAN_POINT ( 'NONE',  ( 148.4042165687623083, 273.6033521758856750, -8.709765892313745539 ) ) ;
#55631=CARTESIAN_POINT ( 'NONE',  ( 163.3020905273760093, 247.7994775548095845, -11.05431316445765155 ) ) ;
#55632=CARTESIAN_POINT ( 'NONE',  ( 193.7118145980225279, 295.1282904202991517, 14.61271143546694162 ) ) ;
#55633=CARTESIAN_POINT ( 'NONE',  ( 185.9342682518984020, 292.9530047715350634, -10.72693318328547818 ) ) ;
#55634=CARTESIAN_POINT ( 'NONE',  ( 157.8820657059571033, 257.1872359237914338, -17.60412210594719440 ) ) ;
#55635=CARTESIAN_POINT ( 'NONE',  ( 146.3987206697217403, 246.1423013555409796, -4.594050593750043987 ) ) ;
#55636=DIRECTION ( 'NONE',  ( -0.8660254037844387076, -0.4999999999999998890, -0.000000000000000000 ) ) ;
#55637=CARTESIAN_POINT ( 'NONE',  ( 173.8665542827094725, 250.6399523573830095, -0.9454928766311748722 ) ) ;
#55638=VERTEX_POINT ( 'NONE', #68877 ) ;
#55639=CARTESIAN_POINT ( 'NONE',  ( 151.3589047706063582, 268.4856820897672378, 14.56544807350869419 ) ) ;
#55641=EDGE_LOOP ( 'NONE', ( #60595, #55737, #72910, #98297 ) ) ;
#55642=CARTESIAN_POINT ( 'NONE',  ( 157.1606728774482065, 258.4367249549846974, -18.41782236529479633 ) ) ;
#55644=VERTEX_POINT ( 'NONE', #7587 ) ;
#55646=CARTESIAN_POINT ( 'NONE',  ( 153.0305350670531936, 277.3750776671890890, 8.290292975357761662 ) ) ;
#55648=FACE_OUTER_BOUND ( 'NONE', #60963, .T. ) ;
#55649=EDGE_CURVE ( 'NONE', #45951, #86106, #18959, .T. ) ;
#55650=DIRECTION ( 'NONE',  ( -0.8660254037844387076, -0.4999999999999998890, -0.000000000000000000 ) ) ;
#55651=CARTESIAN_POINT ( 'NONE',  ( 73.24602992621615272, 225.3464784336661353, 1.353441290958777327E-15 ) ) ;
#55652=VERTEX_POINT ( 'NONE', #93222 ) ;
#55653=EDGE_CURVE ( 'NONE', #46249, #79661, #3361, .T. ) ;
#55655=CARTESIAN_POINT ( 'NONE',  ( 208.3764315856425640, 269.7284287242038658, -1.833640725398759441 ) ) ;
#55660=CARTESIAN_POINT ( 'NONE',  ( 164.0466959984708808, 284.5713585264927588, 0.5044889840302336781 ) ) ;
#55666=CARTESIAN_POINT ( 'NONE',  ( 206.6912923161529818, 272.6471755567893638, -9.325620632947922317 ) ) ;
#55668=CARTESIAN_POINT ( 'NONE',  ( 175.1469972352321633, 284.3759121112690309, 13.98116163681930146 ) ) ;
#55671=VERTEX_POINT ( 'NONE', #68387 ) ;
#55673=CARTESIAN_POINT ( 'NONE',  ( 200.8432122835317841, 282.7763473000181307, 17.15137370990203891 ) ) ;
#55675=CARTESIAN_POINT ( 'NONE',  ( 184.8630750434761296, 264.0504083588372168, -12.11215620985133512 ) ) ;
#55677=CARTESIAN_POINT ( 'NONE',  ( 203.9648368022151601, 269.0477214045654364, 5.644613064108824574 ) ) ;
#55682=CARTESIAN_POINT ( 'NONE',  ( 180.5897091146829609, 267.0577128828192031, -14.91057311322558476 ) ) ;
#55684=CARTESIAN_POINT ( 'NONE',  ( 175.9417783262450712, 285.5840353934577251, -13.36389416340276171 ) ) ;
#55686=CARTESIAN_POINT ( 'NONE',  ( 180.4105609632205756, 272.9652835783806495, 17.11323411940207606 ) ) ;
#55687=CARTESIAN_POINT ( 'NONE',  ( 181.7815785431583038, 276.1505370498239813, -17.81783396216490445 ) ) ;
#55688=CARTESIAN_POINT ( 'NONE',  ( 191.6505299071077104, 262.2872231605458069, 2.938842163976925104 ) ) ;
#55689=CARTESIAN_POINT ( 'NONE',  ( 188.5010067632256607, 276.1349817662086252, -17.56847558694355982 ) ) ;
#55690=CARTESIAN_POINT ( 'NONE',  ( -3.586574591843265658, 177.9244531367911577, -4.594050593750046652 ) ) ;
#55693=CARTESIAN_POINT ( 'NONE',  ( 175.3514250190609687, 255.5038543308169494, 8.239661746456338420 ) ) ;
#55696=CARTESIAN_POINT ( 'NONE',  ( 22.06942799527072907, 192.7369531367911293, -4.594050593750048428 ) ) ;
#55697=EDGE_CURVE ( 'NONE', #61969, #58437, #6001, .T. ) ;
#55698=CARTESIAN_POINT ( 'NONE',  ( 71.12873073640183463, 200.3262482093457777, 3.021315404115420679E-15 ) ) ;
#55700=CARTESIAN_POINT ( 'NONE',  ( 178.4923177964227250, 291.6910058127210164, 5.905753715927121839 ) ) ;
#55701=CARTESIAN_POINT ( 'NONE',  ( 147.2784190576484491, 275.5532906641692534, 0.2793038414862047958 ) ) ;
#55703=CARTESIAN_POINT ( 'NONE',  ( 187.6909010698966540, 296.4604880036308714, -7.720386555275442042 ) ) ;
#55705=CARTESIAN_POINT ( 'NONE',  ( 193.0502745353014689, 295.6857625178031412, -12.56346185710428998 ) ) ;
#55706=CARTESIAN_POINT ( 'NONE',  ( 61.50992858288472576, 212.9865022471903444, -10.00000000000009415 ) ) ;
#55708=CARTESIAN_POINT ( 'NONE',  ( 185.6631735345632706, 277.8091931743529699, -17.25901495274653286 ) ) ;
#55709=CARTESIAN_POINT ( 'NONE',  ( 203.6925490392534925, 269.5270927311577793, 7.084861529579629114 ) ) ;
#55710=CARTESIAN_POINT ( 'NONE',  ( 42.15091268916992817, 185.9548013555409796, -4.594050593750042211 ) ) ;
#55711=CARTESIAN_POINT ( 'NONE',  ( 197.8977219949227049, 287.8780861330898801, 17.48564646125164046 ) ) ;
#55713=CARTESIAN_POINT ( 'NONE',  ( 73.27344031762343946, 203.1115022471901739, -5.000000000000041744 ) ) ;
#55717=ORIENTED_EDGE ( 'NONE', *, *, #89156, .F. ) ;
#55719=CARTESIAN_POINT ( 'NONE',  ( 168.1103729947156751, 282.0138679452536508, -10.93130146384492996 ) ) ;
#55721=CARTESIAN_POINT ( 'NONE',  ( 160.8398227522241370, 262.6459064758317936, 17.80292298429472098 ) ) ;
#55723=CARTESIAN_POINT ( 'NONE',  ( 163.4004183463084416, 247.6291687766210146, 10.19167732382099345 ) ) ;
#55724=CARTESIAN_POINT ( 'NONE',  ( 196.9431415128477170, 289.5314680279574304, -16.61413060656005669 ) ) ;
#55725=CARTESIAN_POINT ( 'NONE',  ( 187.6748237365926286, 269.2623419302518073, -14.09746843418098905 ) ) ;
#55728=CARTESIAN_POINT ( 'NONE',  ( 189.2844570553383790, 299.8432624979336651, 4.996325856711115954 ) ) ;
#55735=CARTESIAN_POINT ( 'NONE',  ( 177.7080561073729257, 256.3275381662501786, -7.267023968690817348 ) ) ;
#55736=CARTESIAN_POINT ( 'NONE',  ( 190.0550686570564949, 301.4619601804237732, 4.203010638620038542 ) ) ;
#55737=ORIENTED_EDGE ( 'NONE', *, *, #62855, .T. ) ;
#55739=CARTESIAN_POINT ( 'NONE',  ( 189.2635003502843745, 273.9792018228808956, -15.65845025130167478 ) ) ;
#55741=ORIENTED_EDGE ( 'NONE', *, *, #34705, .F. ) ;
#55743=CARTESIAN_POINT ( 'NONE',  ( 187.9019955452718023, 260.0457317612239194, -6.306085470763082235 ) ) ;
#55746=CARTESIAN_POINT ( 'NONE',  ( 204.6475128369918082, 276.1871054541632020, -13.72068618491070779 ) ) ;
#55748=CARTESIAN_POINT ( 'NONE',  ( 106.9945647975297760, 223.3923013555410080, 4.594050593750050204 ) ) ;
#55749=CARTESIAN_POINT ( 'NONE',  ( 148.9831146496684084, 272.6006712873522133, -12.63706091291043343 ) ) ;
#55750=CARTESIAN_POINT ( 'NONE',  ( 180.6772252457255377, 287.0457239474706057, -13.49698767722689752 ) ) ;
#55751=EDGE_LOOP ( 'NONE', ( #49317, #53667, #35966, #13921, #67730, #58546, #19045, #29380, #2365, #88406, #86728, #25060, #79986, #12938, #66234, #32638, #69560, #91218, #38464, #68709 ) ) ;
#55752=CARTESIAN_POINT ( 'NONE',  ( 164.3890147726454813, 245.9168695380243435, -6.010262808998044548 ) ) ;
#55756=CARTESIAN_POINT ( 'NONE',  ( 157.1649673255039943, 259.2653790051248279, 17.12562605537966220 ) ) ;
#55758=CARTESIAN_POINT ( 'NONE',  ( 56.16917826928300883, 212.4244531367911577, -4.594050593750046652 ) ) ;
#55762=DIRECTION ( 'NONE',  ( -0.8660254037844387076, -0.4999999999999998890, -0.000000000000000000 ) ) ;
#55764=( BOUNDED_CURVE ( )  B_SPLINE_CURVE ( 2, ( #65672, #4896, #51474, #74806, #50472, #81425, #72818, #4379, #35279 ),
 .UNSPECIFIED., .F., .T. ) 
 B_SPLINE_CURVE_WITH_KNOTS ( ( 3, 2, 2, 2, 3 ),
 ( 0.3750000000000000000, 0.3763440860215053752, 0.3790322580645161255, 0.3817204301075268758, 0.3830645161290322509 ),
 .UNSPECIFIED. ) 
 CURVE ( )  GEOMETRIC_REPRESENTATION_ITEM ( )  RATIONAL_B_SPLINE_CURVE ( ( 0.9330127018922194093, 0.9330127018922194093, 1.000000000000000000, 0.8660254037844387076, 1.000000000000000000, 0.8660254037844387076, 1.000000000000000000, 0.9330127018922194093, 0.9330127018922194093 ) ) 
 REPRESENTATION_ITEM ( '' )  );
#55769=CARTESIAN_POINT ( 'NONE',  ( 171.7744858013287228, 259.2587365160856621, -13.76106460065646253 ) ) ;
#55771=CARTESIAN_POINT ( 'NONE',  ( 207.8575108622103755, 270.6272257822888037, -6.381720258959569847 ) ) ;
#55773=CARTESIAN_POINT ( 'NONE',  ( 192.6679047218190135, 296.9363953644068488, -13.34486378385621386 ) ) ;
#55774=CARTESIAN_POINT ( 'NONE',  ( 190.8072577185990610, 300.1591305089344814, 3.698484652594827171 ) ) ;
#55779=CARTESIAN_POINT ( 'NONE',  ( 154.3285155289529769, 264.0917920393945337, -16.81000869023829125 ) ) ;
#55781=CARTESIAN_POINT ( 'NONE',  ( 105.5326262849960131, 240.9244531367911293, -4.594050593750046652 ) ) ;
#55783=CARTESIAN_POINT ( 'NONE',  ( 191.8232488616404225, 298.3993822291468518, -9.342381338555176384 ) ) ;
#55785=CARTESIAN_POINT ( 'NONE',  ( 203.3205561747472814, 278.4854618126124706, -15.14439614831292147 ) ) ;
#55786=CARTESIAN_POINT ( 'NONE',  ( 163.8147431267737204, 246.9115372060205118, 7.125417796469586840 ) ) ;
#55788=CARTESIAN_POINT ( 'NONE',  ( 178.1484433634098536, 255.2371399336910827, 4.532319796120597211 ) ) ;
#55789=ORIENTED_EDGE ( 'NONE', *, *, #4440, .T. ) ;
#55791=CARTESIAN_POINT ( 'NONE',  ( 154.6130741698598854, 273.3603101155351851, -13.17814745200596427 ) ) ;
#55792=CARTESIAN_POINT ( 'NONE',  ( 182.0067218172421235, 260.4949756789683306, 9.583730042554169160 ) ) ;
#55793=CARTESIAN_POINT ( 'NONE',  ( 206.1569797555946195, 273.5726320587986038, -9.753408447412784454 ) ) ;
#55794=CARTESIAN_POINT ( 'NONE',  ( 133.1643360984345463, 253.8149278399160949, 9.188101187500093303 ) ) ;
#55795=B_SPLINE_CURVE_WITH_KNOTS ( 'NONE', 3,
 ( #67542, #21452, #13849, #94379 ),
 .UNSPECIFIED., .F., .F.,
 ( 4, 4 ),
 ( 0.04033338801658184480, 0.04875068421467537716 ),
 .UNSPECIFIED. ) ;
#55796=CARTESIAN_POINT ( 'NONE',  ( 198.4427928769277969, 286.9339956717308837, -17.97122743692687763 ) ) ;
#55798=CARTESIAN_POINT ( 'NONE',  ( 189.6721586819687957, 282.5493231147508482, -16.58139960728656703 ) ) ;
#55800=CARTESIAN_POINT ( 'NONE',  ( 48.48320281069610616, 207.9869531367911009, 4.594050593750046652 ) ) ;
#55804=CARTESIAN_POINT ( 'NONE',  ( 174.4129540281212201, 262.1633850759363895, 14.35098408255141322 ) ) ;
#55806=CARTESIAN_POINT ( 'NONE',  ( 178.8786119934938483, 291.7246583498065320, -6.365583027218077561 ) ) ;
#55808=CARTESIAN_POINT ( 'NONE',  ( 203.3684377202211522, 278.4025285431072803, -16.56116267537666076 ) ) ;
#55809=CARTESIAN_POINT ( 'NONE',  ( 153.6066505450084492, 269.2403879892464715, -15.56648601798310239 ) ) ;
#55810=CARTESIAN_POINT ( 'NONE',  ( 121.1754704609022468, 240.7677522451418497, 10.00000000000009592 ) ) ;
#55811=B_SPLINE_SURFACE_WITH_KNOTS ( 'NONE', 3, 1, ( 
 ( #13383, #66571 ),
 ( #68059, #89909 ),
 ( #91396, #97983 ),
 ( #81814, #51877 ),
 ( #29083, #27593 ),
 ( #83805, #51360 ),
 ( #44253, #58938 ),
 ( #13865, #12390 ),
 ( #28561, #28065 ),
 ( #14369, #29566 ),
 ( #59441, #68554 ),
 ( #82815, #97497 ),
 ( #45255, #19984 ),
 ( #21961, #60440 ),
 ( #52854, #20996 ),
 ( #44745, #75188 ),
 ( #43753, #50864 ),
 ( #74698, #58457 ),
 ( #5763, #5277 ),
 ( #36652, #67559 ),
 ( #43255, #98491 ),
 ( #59948, #90919 ),
 ( #75678, #21468 ),
 ( #52356, #37160 ),
 ( #76190, #6765 ),
 ( #89431, #74200 ),
 ( #4789, #79577 ),
 ( #54846, #7758 ),
 ( #69556, #33432 ),
 ( #22461, #85827 ),
 ( #22947, #92400 ),
 ( #39131, #53355 ),
 ( #92888, #657 ),
 ( #60947, #56725 ) ),
 .UNSPECIFIED., .T., .F., .F.,
 ( 4, 2, 2, 2, 2, 2, 2, 2, 2, 2, 2, 2, 2, 2, 2, 2, 4 ),
 ( 2, 2 ),
 ( 0.000000000000000000, 0.06250000000000000000, 0.1250000000000000000, 0.1875000000000000000, 0.2500000000000000000, 0.3125000000000000000, 0.3750000000000000000, 0.4375000000000000000, 0.5000000000000000000, 0.5625000000000000000, 0.6250000000000000000, 0.6875000000000000000, 0.7500000000000000000, 0.8125000000000000000, 0.8750000000000000000, 0.9375000000000000000, 1.000000000000000000 ),
 ( 0.000000000000000000, 1.000000000000000000 ),
 .UNSPECIFIED. ) ;
#55815=CARTESIAN_POINT ( 'NONE',  ( 163.3543347837650686, 247.7089878483399730, 10.92686688779373405 ) ) ;
#55817=EDGE_CURVE ( 'NONE', #78871, #20189, #47989, .T. ) ;
#55818=CARTESIAN_POINT ( 'NONE',  ( 23.50386934422995822, 190.5024278399160949, -9.188101187500093303 ) ) ;
#55820=CARTESIAN_POINT ( 'NONE',  ( 192.3060925962972476, 271.9899639347428888, 15.52435667988647516 ) ) ;
#55821=CARTESIAN_POINT ( 'NONE',  ( 149.2678550509543811, 265.6471520882315076, -1.519623991172852856E-15 ) ) ;
#55823=CARTESIAN_POINT ( 'NONE',  ( 192.7686961758011250, 263.9209412561240811, -8.347089341778378468 ) ) ;
#55824=CARTESIAN_POINT ( 'NONE',  ( 65.24466313315730304, 195.1427522451417644, 1.119607411625061291E-15 ) ) ;
#55825=CARTESIAN_POINT ( 'NONE',  ( 171.7216141583608930, 286.8318612379766819, 7.460387380223108877 ) ) ;
#55826=CARTESIAN_POINT ( 'NONE',  ( 183.8250474427275094, 257.7038322492317093, 1.335502332953788729 ) ) ;
#55827=CARTESIAN_POINT ( 'NONE',  ( -2.524136441754524451, 180.8967562850347406, 2.649461200531984646E-14 ) ) ;
#55830=CARTESIAN_POINT ( 'NONE',  ( 26.50806851326365532, 196.1115022471903160, -5.000000000000047962 ) ) ;
#55833=CARTESIAN_POINT ( 'NONE',  ( 145.4512450625087467, 254.7833772461660544, -9.188101187500095079 ) ) ;
#55835=CARTESIAN_POINT ( 'NONE',  ( 163.9100659486979907, 252.4955106033718835, 13.24059601348467297 ) ) ;
#55836=CARTESIAN_POINT ( 'NONE',  ( 200.4194242942598407, 282.7622742240619687, 16.88461573361379564 ) ) ;
#55838=CARTESIAN_POINT ( 'NONE',  ( 185.4274225405056882, 260.0935088849925592, 7.264075338455358910 ) ) ;
#55840=CARTESIAN_POINT ( 'NONE',  ( 205.8030308266901898, 274.1856895869457844, 10.55961490432110317 ) ) ;
#55841=CARTESIAN_POINT ( 'NONE',  ( 186.8289980366191685, 258.5750005707243417, -2.467696023248564074 ) ) ;
#55844=CARTESIAN_POINT ( 'NONE',  ( 55.65417314315315878, 214.4860189848785694, -2.679491924311252493 ) ) ;
#55845=CARTESIAN_POINT ( 'NONE',  ( 180.5920144538960699, 286.8105750589551235, 13.18251988290063004 ) ) ;
#55846=CARTESIAN_POINT ( 'NONE',  ( 168.7075216304318417, 287.6756853637114659, 0.5128971772568799992 ) ) ;
#55848=CARTESIAN_POINT ( 'NONE',  ( 207.1531864936216607, 271.8471513736934071, 8.161497146364244060 ) ) ;
#55851=CARTESIAN_POINT ( 'NONE',  ( 206.1408608592916494, 273.6005508061571732, -10.42739367433323494 ) ) ;
#55853=CARTESIAN_POINT ( 'NONE',  ( 192.3606619183491091, 297.4685555102766443, 10.99569063633359889 ) ) ;
#55854=CARTESIAN_POINT ( 'NONE',  ( 164.8251969117060298, 245.1613799118173063, -1.508678420156898348 ) ) ;
#55856=CARTESIAN_POINT ( 'NONE',  ( 191.3843761966370209, 282.8631020262318430, -17.76976768207862278 ) ) ;
#55858=CARTESIAN_POINT ( 'NONE',  ( 154.9344967692067598, 262.2925750810547356, 17.30210568643136781 ) ) ;
#55861=CARTESIAN_POINT ( 'NONE',  ( 155.9060408714371988, 277.3267832574535419, -10.46950353421899038 ) ) ;
#55863=EDGE_LOOP ( 'NONE', ( #61841, #82956, #87509, #27354 ) ) ;
#55864=LINE ( 'NONE', #31578, #75871 ) ;
#55870=CARTESIAN_POINT ( 'NONE',  ( 173.9119411810186193, 267.2826965128863890, 17.13893503472135649 ) ) ;
#55872=CARTESIAN_POINT ( 'NONE',  ( 175.0125019719911847, 292.0719086349095051, 3.303583340955516423 ) ) ;
#55874=CARTESIAN_POINT ( 'NONE',  ( 190.8264243556038195, 300.1259329198319961, 8.466983560044813117 ) ) ;
#55875=CARTESIAN_POINT ( 'NONE',  ( 151.3777100552970580, 274.9574019808734420, -8.625823521072360833 ) ) ;
#55876=VERTEX_POINT ( 'NONE', #87889 ) ;
#55885=CARTESIAN_POINT ( 'NONE',  ( 160.7087992090237663, 271.0393196853082145, 16.56332265730499387 ) ) ;
#55888=CARTESIAN_POINT ( 'NONE',  ( 197.2484515917759609, 283.9560669716739199, 17.81188092217798769 ) ) ;
#55890=CARTESIAN_POINT ( 'NONE',  ( 147.6884207308302450, 274.8431469350302336, -8.096293592099874203 ) ) ;
#55895=CARTESIAN_POINT ( 'NONE',  ( 96.49374645304573050, 226.5177522451418781, -10.00000000000009592 ) ) ;
#55897=CARTESIAN_POINT ( 'NONE',  ( 164.4494343874829099, 245.8122196953522121, 2.922779519406129456 ) ) ;
#55898=CARTESIAN_POINT ( 'NONE',  ( 191.5513189742059978, 298.4536868043492746, -8.478051802322086772 ) ) ;
#55899=CARTESIAN_POINT ( 'NONE',  ( 159.4285914931787431, 254.5085746851079023, 15.41072477910873673 ) ) ;
#55900=ORIENTED_EDGE ( 'NONE', *, *, #91995, .T. ) ;
#55901=EDGE_CURVE ( 'NONE', #1717, #21251, #70782, .T. ) ;
#55903=CARTESIAN_POINT ( 'NONE',  ( 168.8244094625508751, 257.0541383169796745, -14.93690306707719628 ) ) ;
#55905=CARTESIAN_POINT ( 'NONE',  ( 206.1798448551755598, 273.5330285446045195, -10.53862763475382813 ) ) ;
#55906=CYLINDRICAL_SURFACE ( 'NONE', #26292, 17.82106496071139645 ) ;
#55907=CARTESIAN_POINT ( 'NONE',  ( 200.8769374536528858, 282.7179335918746688, 17.26928237494566787 ) ) ;
#55910=CARTESIAN_POINT ( 'NONE',  ( 155.0691674984522308, 262.0593185357093944, -17.32141920768173904 ) ) ;
#55913=CARTESIAN_POINT ( 'NONE',  ( 207.5686001603237116, 271.1276337968068333, 7.659944433763431704 ) ) ;
#55914=CARTESIAN_POINT ( 'NONE',  ( 14.14916430987532792, 185.6427522451419065, 10.00000000000009237 ) ) ;
#55915=B_SPLINE_CURVE_WITH_KNOTS ( 'NONE', 3,
 ( #36605, #30509, #14317, #99429, #60392, #5229, #52797, #59394, #7202, #74652, #67511, #75626, #60890, #6213, #5716, #13338, #82278, #98442, #76143, #52310, #51307, #61400, #44695, #83248, #90370, #45689, #12850, #51831, #29033, #38086, #76616, #45204, #29519, #91348, #21909, #82771, #6717, #37596, #68507, #30006, #91853, #59904, #36108, #68998, #22412, #99925, #67013, #90873, #53304, #84259 ),
 .UNSPECIFIED., .F., .F.,
 ( 4, 2, 2, 2, 2, 2, 2, 2, 2, 2, 2, 2, 2, 2, 2, 2, 2, 2, 2, 2, 2, 2, 2, 2, 4 ),
 ( 0.0001608434559496862688, 0.001169039375235548118, 0.001673137334878438886, 0.001925186314699919290, 0.002051210804610674454, 0.002177235294521429401, 0.002303259784432184782, 0.002429284274342939729, 0.002681333254164449623, 0.003185431213807470279, 0.004193627133093571872, 0.005201823052379673032, 0.005705921012022679810, 0.005957969991844181898, 0.006210018971665684853, 0.006273031216621136053, 0.006336043461576586384, 0.006399055706532036716, 0.006462067951487487916, 0.006714116931309142659, 0.006966165911130798270, 0.007218214890952453014, 0.007470263870774108625, 0.007722312850595764236, 0.008226410810239198623 ),
 .UNSPECIFIED. ) ;
#55916=CARTESIAN_POINT ( 'NONE',  ( 97.82019495012963262, 215.0327760586659736, 1.948934522072302763E-15 ) ) ;
#55918=CARTESIAN_POINT ( 'NONE',  ( 174.5401493766550516, 282.4217946544197275, -14.57910214582674691 ) ) ;
#55919=CARTESIAN_POINT ( 'NONE',  ( 167.0407061306596290, 278.0018592765986227, -13.72108455681485317 ) ) ;
#55920=CARTESIAN_POINT ( 'NONE',  ( 12.08367997547019002, 165.5327760586659451, 1.948934522072303157E-15 ) ) ;
#55923=CARTESIAN_POINT ( 'NONE',  ( 188.8544700204132880, 297.4231428397746413, 9.261439979758030461 ) ) ;
#55925=EDGE_LOOP ( 'NONE', ( #38509, #90227, #96795, #66364 ) ) ;
#55926=CARTESIAN_POINT ( 'NONE',  ( 200.8035035346175619, 267.7285506604447392, -2.858260968050738704 ) ) ;
#55930=CARTESIAN_POINT ( 'NONE',  ( 35.52916646935157274, 197.9865022471903160, -10.00000000000009592 ) ) ;
#55931=CARTESIAN_POINT ( 'NONE',  ( 59.27500801855438795, 193.4824982072973683, 3.021315404115420679E-15 ) ) ;
#55933=CARTESIAN_POINT ( 'NONE',  ( 23.88258191050314494, 196.8464784336661637, 1.353441290958777525E-15 ) ) ;
#55934=CARTESIAN_POINT ( 'NONE',  ( 77.00817486789581778, 225.2677522451419350, -5.000000000000047962 ) ) ;
#55938=CARTESIAN_POINT ( 'NONE',  ( 178.9714194486930694, 253.6239517424200187, 1.422777586239305059 ) ) ;
#55942=CARTESIAN_POINT ( 'NONE',  ( 57.34764182315618797, 215.4637435831425307, 2.679491924311251605 ) ) ;
#55944=CARTESIAN_POINT ( 'NONE',  ( 186.6671973743490582, 282.6820187201159342, 16.18259547852653313 ) ) ;
#55945=CARTESIAN_POINT ( 'NONE',  ( 194.4032909867620447, 293.9306181827685123, -16.05392006271526384 ) ) ;
#55948=CARTESIAN_POINT ( 'NONE',  ( 171.7403546589055452, 279.6099264174512200, 14.56001095287713021 ) ) ;
#55949=CARTESIAN_POINT ( 'NONE',  ( 146.7434471017767521, 276.4798892723637209, 0.7354350123930684102 ) ) ;
#55950=CARTESIAN_POINT ( 'NONE',  ( 148.4016473149517594, 273.6078022540229426, 8.470066617688926769 ) ) ;
#55951=ORIENTED_EDGE ( 'NONE', *, *, #36707, .F. ) ;
#55952=AXIS2_PLACEMENT_3D ( 'NONE', #90902, #37139, #6244 ) ;
#55953=CARTESIAN_POINT ( 'NONE',  ( 207.8725590214046406, 270.6011616060040410, 1.988011721677743093 ) ) ;
#55954=CARTESIAN_POINT ( 'NONE',  ( 181.1274570500190464, 268.2429819168116296, 15.60512382003630982 ) ) ;
#55955=CARTESIAN_POINT ( 'NONE',  ( 111.1617914095948692, 244.1744531367911293, 4.594050593750047540 ) ) ;
#55962=CARTESIAN_POINT ( 'NONE',  ( 150.9165176611652157, 269.2519190399329432, -13.92901968401340262 ) ) ;
#55963=CYLINDRICAL_SURFACE ( 'NONE', #94101, 17.82106496071139645 ) ;
#55964=CARTESIAN_POINT ( 'NONE',  ( 149.7200635338602410, 271.3242383773507527, -12.12223662813266500 ) ) ;
#55965=CARTESIAN_POINT ( 'NONE',  ( 81.50068165357551209, 227.8615022471903160, 5.000000000000046185 ) ) ;
#55966=CARTESIAN_POINT ( 'NONE',  ( 172.7682828100511188, 290.3836512414355298, -1.901510031099399978 ) ) ;
#55967=CARTESIAN_POINT ( 'NONE',  ( -17.42236680055705023, 149.2012482093457777, 0.000000000000000000 ) ) ;
#55968=ORIENTED_EDGE ( 'NONE', *, *, #61510, .T. ) ;
#55970=CARTESIAN_POINT ( 'NONE',  ( 175.5198215696162265, 278.6707974891042454, 15.42220655511384564 ) ) ;
#55971=CARTESIAN_POINT ( 'NONE',  ( 165.5298684834693574, 269.3554679133272884, -17.63324793928101997 ) ) ;
#55972=EDGE_CURVE ( 'NONE', #13906, #57617, #79265, .T. ) ;
#55975=ADVANCED_FACE ( 'NONE', ( #61876 ), #16293, .T. ) ;
#55976=CYLINDRICAL_SURFACE ( 'NONE', #53609, 14.82106496071141066 ) ;
#55977=CARTESIAN_POINT ( 'NONE',  ( 155.8723835780803881, 261.2467561593892356, 17.10610717069041797 ) ) ;
#55979=CARTESIAN_POINT ( 'NONE',  ( 192.1883190596398094, 297.7670620978826150, 12.41391288785556668 ) ) ;
#55980=ORIENTED_EDGE ( 'NONE', *, *, #82033, .T. ) ;
#55981=CARTESIAN_POINT ( 'NONE',  ( 191.2104420009116836, 280.2857515794617598, 17.80337293751487593 ) ) ;
#55983=CARTESIAN_POINT ( 'NONE',  ( 188.7308569474326134, 285.6752924799993707, 17.07521345989996320 ) ) ;
#55984=VERTEX_POINT ( 'NONE', #46692 ) ;
#55985=CARTESIAN_POINT ( 'NONE',  ( 166.1807419043942673, 280.1926019274495161, 11.70936788950543495 ) ) ;
#55987=CARTESIAN_POINT ( 'NONE',  ( 164.6558840558436714, 246.1165554557707082, -1.230166818256332117 ) ) ;
#55988=ORIENTED_EDGE ( 'NONE', *, *, #41699, .F. ) ;
#55990=CARTESIAN_POINT ( 'NONE',  ( 188.7753597038515920, 293.7201965824127115, 12.88945448372762570 ) ) ;
#55991=B_SPLINE_CURVE_WITH_KNOTS ( 'NONE', 3,
 ( #46898, #22605, #69195, #53978 ),
 .UNSPECIFIED., .F., .F.,
 ( 4, 4 ),
 ( 0.000000000000000000, 0.004243563290278051271 ),
 .UNSPECIFIED. ) ;
#55997=CARTESIAN_POINT ( 'NONE',  ( 203.5629025532486196, 278.0657055720176913, -15.85226727704602823 ) ) ;
#56001=CARTESIAN_POINT ( 'NONE',  ( 176.4420281119471952, 259.8590673950340033, 12.32580266317428652 ) ) ;
#56003=ORIENTED_EDGE ( 'NONE', *, *, #38388, .T. ) ;
#56005=ORIENTED_EDGE ( 'NONE', *, *, #83531, .F. ) ;
#56006=CARTESIAN_POINT ( 'NONE',  ( 173.3310713462738306, 270.5831704705003631, 16.79086624453662679 ) ) ;
#56007=CARTESIAN_POINT ( 'NONE',  ( 203.3041373168503299, 278.5139001086923827, -16.61929732091214973 ) ) ;
#56008=ORIENTED_EDGE ( 'NONE', *, *, #4528, .F. ) ;
#56009=EDGE_CURVE ( 'NONE', #53637, #13224, #98620, .T. ) ;
#56010=CARTESIAN_POINT ( 'NONE',  ( 164.3231499090067302, 246.0309508282801971, -1.360008376207661573 ) ) ;
#56011=CARTESIAN_POINT ( 'NONE',  ( 190.0953138929461375, 301.3922533871005385, 3.399835324073681608 ) ) ;
#56013=CARTESIAN_POINT ( 'NONE',  ( 192.8607783413999073, 296.6023284558532396, -11.80574095728561446 ) ) ;
#56014=CARTESIAN_POINT ( 'NONE',  ( 153.0444155045374544, 265.5662918618958201, -16.15173036748435109 ) ) ;
#56016=CARTESIAN_POINT ( 'NONE',  ( 157.7016178275996481, 280.8566103467931043, 2.084903823814490131 ) ) ;
#56018=CARTESIAN_POINT ( 'NONE',  ( 121.7437996339097310, 241.0958772461660544, -9.188101187500095079 ) ) ;
#56021=VERTEX_POINT ( 'NONE', #34492 ) ;
#56026=CARTESIAN_POINT ( 'NONE',  ( 201.6144114969290229, 275.0453523290713065, 13.34253202614237033 ) ) ;
#56028=CARTESIAN_POINT ( 'NONE',  ( 174.2958066453992103, 290.3206272445223135, -4.802435633763557199 ) ) ;
#56029=CARTESIAN_POINT ( 'NONE',  ( 146.6773087776009277, 276.5944442101636582, 3.546544321270581612 ) ) ;
#56032=CARTESIAN_POINT ( 'NONE',  ( 173.9326749925096465, 287.2443000551036221, -9.522606441215669903 ) ) ;
#56036=VERTEX_POINT ( 'NONE', #65884 ) ;
#56037=CARTESIAN_POINT ( 'NONE',  ( 147.6512387128590262, 274.9075480792844246, -8.209968531507987777 ) ) ;
#56038=CARTESIAN_POINT ( 'NONE',  ( 152.8861948602045402, 273.8046404715449853, 12.06949787893822013 ) ) ;
#56040=CARTESIAN_POINT ( 'NONE',  ( 162.9254136962317148, 277.9293967287522946, 13.77390558128574760 ) ) ;
#56041=B_SPLINE_CURVE_WITH_KNOTS ( 'NONE', 3,
 ( #70297, #77422, #40386, #408 ),
 .UNSPECIFIED., .F., .F.,
 ( 4, 4 ),
 ( 0.01598569196496549966, 0.02481275599104538002 ),
 .UNSPECIFIED. ) ;
#56042=CARTESIAN_POINT ( 'NONE',  ( 159.8161384505802971, 279.1487373509320946, 10.85936962484722201 ) ) ;
#56043=CARTESIAN_POINT ( 'NONE',  ( 151.9574818334562565, 267.4489162046660340, -15.47372068035671155 ) ) ;
#56045=CARTESIAN_POINT ( 'NONE',  ( 163.3706531435203146, 247.6807236201477735, 10.06957846017757241 ) ) ;
#56046=CARTESIAN_POINT ( 'NONE',  ( 164.7244464148843690, 284.0693728551247546, -6.859052662106053688 ) ) ;
#56047=CARTESIAN_POINT ( 'NONE',  ( 154.4362440790400797, 276.8969399611219160, -8.726023671585549479 ) ) ;
#56048=CARTESIAN_POINT ( 'NONE',  ( 200.4385098325799675, 267.3393730264926376, 6.361263591900818248 ) ) ;
#56050=CARTESIAN_POINT ( 'NONE',  ( 167.1454213690836639, 281.4972382487084133, -10.93374221028199322 ) ) ;
#56051=CARTESIAN_POINT ( 'NONE',  ( 163.5491121955337803, 247.7522377084982281, -7.761536679276979989 ) ) ;
#56052=DIRECTION ( 'NONE',  ( -0.4999999999999987788, 0.8660254037844392627, 0.000000000000000000 ) ) ;
#56053=CARTESIAN_POINT ( 'NONE',  ( 85.25577013208754806, 208.4824982072973967, 3.021315404115420679E-15 ) ) ;
#56054=CARTESIAN_POINT ( 'NONE',  ( 188.6013203369844575, 298.5946043969738639, -4.227064913786014344 ) ) ;
#56055=CARTESIAN_POINT ( 'NONE',  ( 188.5612436805310779, 268.6432733723845558, 15.05044350854306323 ) ) ;
#56057=CARTESIAN_POINT ( 'NONE',  ( -12.91644128716779072, 174.8967562850347406, 1.347971487989956912E-14 ) ) ;
#56059=CARTESIAN_POINT ( 'NONE',  ( -9.892408837089959661, 177.3464784336661637, 1.353441290958777525E-15 ) ) ;
#56060=CARTESIAN_POINT ( 'NONE',  ( 83.80088808272151368, 225.3149278399160949, 9.188101187500093303 ) ) ;
#56063=CARTESIAN_POINT ( 'NONE',  ( 182.8053931574769422, 294.3809610745131522, -8.049654163022442077 ) ) ;
#56065=CIRCLE ( 'NONE', #35114, 17.82106496071138935 ) ;
#56066=DIRECTION ( 'NONE',  ( -0.8660254037844387076, -0.4999999999999998890, -0.000000000000000000 ) ) ;
#56071=CARTESIAN_POINT ( 'NONE',  ( 208.1303168694798273, 270.1547119170880364, -0.9257663487928086132 ) ) ;
#56072=CARTESIAN_POINT ( 'NONE',  ( 161.4650976420346637, 250.9812425653634023, 12.76171476511797565 ) ) ;
#56073=CARTESIAN_POINT ( 'NONE',  ( 168.8088173946568702, 251.8078635755704511, -8.785532002324718093 ) ) ;
#56074=( BOUNDED_CURVE ( )  B_SPLINE_CURVE ( 2, ( #76965, #99293, #29874, #59764, #67882, #90733, #98803, #7566, #60746 ),
 .UNSPECIFIED., .F., .T. ) 
 B_SPLINE_CURVE_WITH_KNOTS ( ( 3, 2, 2, 2, 3 ),
 ( 0.6008064516129032473, 0.6021505376344086224, 0.6048387096774193727, 0.6075268817204301230, 0.6088709677419354982 ),
 .UNSPECIFIED. ) 
 CURVE ( )  GEOMETRIC_REPRESENTATION_ITEM ( )  RATIONAL_B_SPLINE_CURVE ( ( 0.9330127018922194093, 0.9330127018922194093, 1.000000000000000000, 0.8660254037844387076, 1.000000000000000000, 0.8660254037844387076, 1.000000000000000000, 0.9330127018922194093, 0.9330127018922194093 ) ) 
 REPRESENTATION_ITEM ( '' )  );
#56080=CARTESIAN_POINT ( 'NONE',  ( 45.42531092540608029, 197.0333772461660828, 9.188101187500095079 ) ) ;
#56082=CARTESIAN_POINT ( 'NONE',  ( 64.91088251055593616, 208.2833772461660544, -9.188101187500095079 ) ) ;
#56086=CARTESIAN_POINT ( 'NONE',  ( 167.1743255730581552, 259.8161784781199231, 15.97983238844050824 ) ) ;
#56087=CARTESIAN_POINT ( 'NONE',  ( 198.6959030336114438, 286.1027943447343205, -17.01025293640724811 ) ) ;
#56093=CARTESIAN_POINT ( 'NONE',  ( 196.4242782546697015, 290.4301655533025155, -16.42402868779123537 ) ) ;
#56096=CARTESIAN_POINT ( 'NONE',  ( 74.46396492422927338, 222.9869531367911293, 4.594050593750046652 ) ) ;
#56100=CARTESIAN_POINT ( 'NONE',  ( 172.7227978551848651, 290.4444241243636498, -0.3282510524908365257 ) ) ;
#56101=CARTESIAN_POINT ( 'NONE',  ( 156.6812872898450735, 261.2670451491295012, 0.000000000000000000 ) ) ;
#56102=CARTESIAN_POINT ( 'NONE',  ( 201.9631990782953892, 280.8364732676815834, 16.42174701891640964 ) ) ;
#56103=EDGE_CURVE ( 'NONE', #75148, #60835, #2783, .T. ) ;
#56107=CARTESIAN_POINT ( 'NONE',  ( 193.4977959244270096, 288.4670934838076164, 16.06266015785881507 ) ) ;
#56108=CARTESIAN_POINT ( 'NONE',  ( 134.2560625007776878, 234.9865022471901455, 1.119607411625061291E-15 ) ) ;
#56110=CARTESIAN_POINT ( 'NONE',  ( 164.2672861321391053, 246.1277097281173667, -2.417001679502223777 ) ) ;
#56112=CARTESIAN_POINT ( 'NONE',  ( 188.4697100348334402, 272.9738383098946315, 15.64619135176044118 ) ) ;
#56113=ORIENTED_EDGE ( 'NONE', *, *, #82460, .T. ) ;
#56114=CARTESIAN_POINT ( 'NONE',  ( 202.6551236945213361, 279.6380246773706517, 15.55476940527561425 ) ) ;
#56117=VERTEX_POINT ( 'NONE', #57781 ) ;
#56119=ORIENTED_EDGE ( 'NONE', *, *, #67984, .F. ) ;
#56121=CARTESIAN_POINT ( 'NONE',  ( 170.8439429942262962, 250.1382644172885250, 2.884658875547349677 ) ) ;
#56128=CARTESIAN_POINT ( 'NONE',  ( 51.26196130476894552, 193.7365022471901739, -10.00000000000009237 ) ) ;
#56129=ORIENTED_EDGE ( 'NONE', *, *, #68249, .T. ) ;
#56134=CARTESIAN_POINT ( 'NONE',  ( 180.7942833579522812, 266.7097690628117448, -16.23795806611159520 ) ) ;
#56136=CARTESIAN_POINT ( 'NONE',  ( 194.2669918475045279, 294.1666952169902629, 14.00965265288584050 ) ) ;
#56137=CARTESIAN_POINT ( 'NONE',  ( 185.5198499209504064, 292.6877627818749374, -10.71450089700853070 ) ) ;
#56138=CARTESIAN_POINT ( 'NONE',  ( 157.0877926458200307, 258.5629572190321710, -17.40668770468195703 ) ) ;
#56139=CARTESIAN_POINT ( 'NONE',  ( 164.1007040320689612, 246.4162383890708270, 4.419515984332184289 ) ) ;
#56142=CARTESIAN_POINT ( 'NONE',  ( 82.61045024828291616, 212.3768266524159856, -9.188101187500091527 ) ) ;
#56144=CARTESIAN_POINT ( 'NONE',  ( 191.0816511748900268, 299.6838671013740623, 7.311127128005925790 ) ) ;
#56145=CARTESIAN_POINT ( 'NONE',  ( 164.7364331287320738, 247.3151232938002693, -7.618980141130590411 ) ) ;
#56148=CARTESIAN_POINT ( 'NONE',  ( 156.7071728003359965, 259.2222101297794552, -17.92398391197042073 ) ) ;
#56154=CARTESIAN_POINT ( 'NONE',  ( 191.4082244002820516, 299.1182256826033949, -8.271837126846561361 ) ) ;
#56155=B_SPLINE_SURFACE_WITH_KNOTS ( 'NONE', 3, 1, ( 
 ( #99929, #21426 ),
 ( #6721, #59907 ),
 ( #30010, #45208 ),
 ( #84751, #46190 ),
 ( #91857, #52313 ),
 ( #37600, #44699 ),
 ( #22416, #53307 ),
 ( #15291, #52801 ),
 ( #76147, #44205 ),
 ( #84262, #77107 ),
 ( #38089, #68015 ),
 ( #14809, #45692 ),
 ( #76620, #7711 ),
 ( #7205, #75630 ),
 ( #30512, #6216 ),
 ( #83251, #37112 ),
 ( #98445, #61403 ),
 ( #22904, #92356 ),
 ( #29522, #13817 ),
 ( #38603, #97941 ),
 ( #75141, #28515 ),
 ( #59398, #90374 ),
 ( #20952, #51834 ),
 ( #82775, #5720 ),
 ( #36608, #60395 ),
 ( #14321, #67515 ),
 ( #91351, #48729 ),
 ( #69507, #87297 ),
 ( #616, #79160 ),
 ( #93860, #24415 ),
 ( #9217, #46708 ),
 ( #70507, #40092 ),
 ( #55291, #39088 ),
 ( #39586, #122 ) ),
 .UNSPECIFIED., .T., .F., .F.,
 ( 4, 2, 2, 2, 2, 2, 2, 2, 2, 2, 2, 2, 2, 2, 2, 2, 4 ),
 ( 2, 2 ),
 ( 0.000000000000000000, 0.06250000000000000000, 0.1250000000000000000, 0.1875000000000000000, 0.2500000000000000000, 0.3125000000000000000, 0.3750000000000000000, 0.4375000000000000000, 0.5000000000000000000, 0.5625000000000000000, 0.6250000000000000000, 0.6875000000000000000, 0.7500000000000000000, 0.8125000000000000000, 0.8750000000000000000, 0.9375000000000000000, 1.000000000000000000 ),
 ( 0.000000000000000000, 1.000000000000000000 ),
 .UNSPECIFIED. ) ;
#56158=FACE_OUTER_BOUND ( 'NONE', #99525, .T. ) ;
#56159=CARTESIAN_POINT ( 'NONE',  ( 99.20033616346982797, 218.8923013555410080, 4.594050593750050204 ) ) ;
#56162=ORIENTED_EDGE ( 'NONE', *, *, #17619, .F. ) ;
#56163=CARTESIAN_POINT ( 'NONE',  ( 207.7625791259561652, 270.7916523727319031, -1.015623356719550063 ) ) ;
#56164=EDGE_LOOP ( 'NONE', ( #47146, #43049, #24721, #70197 ) ) ;
#56165=DIRECTION ( 'NONE',  ( 0.4999999999999998890, -0.8660254037844385966, 0.000000000000000000 ) ) ;
#56166=CARTESIAN_POINT ( 'NONE',  ( 164.9101359252495627, 286.5608941336866451, 1.040025780022917790 ) ) ;
#56167=DIRECTION ( 'NONE',  ( -0.4999999999999998890, 0.8660254037844385966, 0.000000000000000000 ) ) ;
#56171=CARTESIAN_POINT ( 'NONE',  ( 204.4345574087956550, 276.5559550755466489, 14.49589339982634861 ) ) ;
#56173=CARTESIAN_POINT ( 'NONE',  ( 206.0930919633010774, 273.6832889610345774, -9.866500005465628220 ) ) ;
#56176=B_SPLINE_CURVE_WITH_KNOTS ( 'NONE', 3,
 ( #18006, #10903, #3316, #72212, #71716, #27603, #42762, #64089, #41778, #81825, #34196, #73205, #2816, #48898 ),
 .UNSPECIFIED., .F., .F.,
 ( 4, 2, 2, 2, 2, 2, 4 ),
 ( 0.000000000000000000, 0.0004778436358628718899, 0.0007167654537943066693, 0.0009556872717257413946, 0.001194609089657176337, 0.001433530907588610953, 0.001911374543451394101 ),
 .UNSPECIFIED. ) ;
#56180=ORIENTED_EDGE ( 'NONE', *, *, #15402, .T. ) ;
#56181=CARTESIAN_POINT ( 'NONE',  ( 203.5600082621025138, 276.7824627000144915, -14.31784352948871586 ) ) ;
#56182=CARTESIAN_POINT ( 'NONE',  ( 200.5438717407500917, 283.2948203288816558, 18.39667691545567152 ) ) ;
#56184=FACE_OUTER_BOUND ( 'NONE', #53767, .T. ) ;
#56185=CARTESIAN_POINT ( 'NONE',  ( 170.8523262845096156, 251.5461551665960656, 7.045273212770799987 ) ) ;
#56187=CARTESIAN_POINT ( 'NONE',  ( 175.3650005030352190, 290.1543442456702451, -6.274446597477803422 ) ) ;
#56188=EDGE_CURVE ( 'NONE', #54274, #22323, #45426, .T. ) ;
#56191=CARTESIAN_POINT ( 'NONE',  ( 185.9406580756425171, 265.4572926502605128, 14.02042132963198817 ) ) ;
#56192=CARTESIAN_POINT ( 'NONE',  ( 207.6826438088389750, 270.9301044032979462, 7.252082088659585146 ) ) ;
#56193=CARTESIAN_POINT ( 'NONE',  ( 180.4105437470794868, 266.7128773822078074, -14.76931904508903770 ) ) ;
#56195=CARTESIAN_POINT ( 'NONE',  ( 199.5752298111263769, 281.0719457017619902, -17.16897691529692693 ) ) ;
#56198=CARTESIAN_POINT ( 'NONE',  ( 172.2871986639351292, 275.0669045666151646, 16.54537181790850653 ) ) ;
#56201=CARTESIAN_POINT ( 'NONE',  ( 189.0439077586675580, 261.2591905183114704, 2.867651556594005058 ) ) ;
#56202=CARTESIAN_POINT ( 'NONE',  ( 161.8882824960653579, 250.2482648971885340, -13.83574485983625557 ) ) ;
#56203=CARTESIAN_POINT ( 'NONE',  ( -3.938137090306929711, 168.5333772461660828, 9.188101187500095079 ) ) ;
#56205=DIRECTION ( 'NONE',  ( -0.8660254037844387076, -0.4999999999999998890, -0.000000000000000000 ) ) ;
#56207=CARTESIAN_POINT ( 'NONE',  ( 174.9515149362974000, 255.1616608167260267, 9.153033967938712934 ) ) ;
#56210=CARTESIAN_POINT ( 'NONE',  ( 19.90436448580963713, 191.4869531367911293, 4.594050593750046652 ) ) ;
#56213=CARTESIAN_POINT ( 'NONE',  ( 181.5751262769139771, 294.5022803070306736, 6.467137775781628406 ) ) ;
#56214=CARTESIAN_POINT ( 'NONE',  ( 191.5521510896938935, 298.8689373439769952, -9.847378829740700112 ) ) ;
#56215=CARTESIAN_POINT ( 'NONE',  ( 149.0195931398871494, 272.5374886889096047, 11.89322657225677560 ) ) ;
#56216=CARTESIAN_POINT ( 'NONE',  ( 141.9600801517288460, 242.7677522451417929, -5.000000000000041744 ) ) ;
#56218=CARTESIAN_POINT ( 'NONE',  ( 189.6629915901594075, 298.0196469402222874, -7.906960439105454874 ) ) ;
#56222=EDGE_CURVE ( 'NONE', #61618, #5477, #62316, .T. ) ;
#56224=CARTESIAN_POINT ( 'NONE',  ( 77.17055463465335663, 215.3615022471902591, -10.00000000000009592 ) ) ;
#56226=CARTESIAN_POINT ( 'NONE',  ( 159.3291946290163992, 279.0199804063916531, 10.96233109238993109 ) ) ;
#56227=CARTESIAN_POINT ( 'NONE',  ( 203.4122341679774877, 270.0895123793504240, 6.031633626111155166 ) ) ;
#56229=CARTESIAN_POINT ( 'NONE',  ( 42.23166870106845039, 201.3149278399160664, 9.188101187500093303 ) ) ;
#56231=ADVANCED_FACE ( 'NONE', ( #93586 ), #10461, .T. ) ;
#56232=EDGE_LOOP ( 'NONE', ( #41745, #23294, #76007, #98444 ) ) ;
#56234=CARTESIAN_POINT ( 'NONE',  ( 150.6438662863770332, 269.7241650738195631, -14.92510732909997628 ) ) ;
#56237=CARTESIAN_POINT ( 'NONE',  ( 83.66574516303664666, 219.1115022471902591, 10.00000000000009592 ) ) ;
#56239=CARTESIAN_POINT ( 'NONE',  ( 159.7955030658553994, 278.5790326856259185, -10.80603072003405352 ) ) ;
#56240=CARTESIAN_POINT ( 'NONE',  ( 163.7540506545266794, 282.2736363210526633, 10.04846317257458921 ) ) ;
#56242=CARTESIAN_POINT ( 'NONE',  ( 202.2712651538608668, 280.3028871727136675, 16.13191389836473988 ) ) ;
#56243=CARTESIAN_POINT ( 'NONE',  ( 149.6230451358742926, 271.4922791719315001, -12.72565967355361671 ) ) ;
#56244=CARTESIAN_POINT ( 'NONE',  ( 185.8660564411877374, 268.0232567166196418, -14.37360442507078417 ) ) ;
#56246=AXIS2_PLACEMENT_3D ( 'NONE', #45315, #89970, #20550 ) ;
#56249=CARTESIAN_POINT ( 'NONE',  ( 207.1610391518539984, 269.8335501706608284, 0.000000000000000000 ) ) ;
#56252=DIRECTION ( 'NONE',  ( -0.8660254037844387076, -0.4999999999999998890, -0.000000000000000000 ) ) ;
#56253=CARTESIAN_POINT ( 'NONE',  ( 177.3133037439327779, 256.0627534786006549, -7.214126111352222814 ) ) ;
#56254=CARTESIAN_POINT ( 'NONE',  ( 190.7805732161387766, 300.2053494229706985, 4.237982805666590025 ) ) ;
#56259=CARTESIAN_POINT ( 'NONE',  ( 189.6946965492525692, 274.3461288625165366, -15.70738189806986718 ) ) ;
#56260=CARTESIAN_POINT ( 'NONE',  ( 177.5665759502285539, 275.7863988818428993, 17.69313789786682989 ) ) ;
#56261=VERTEX_POINT ( 'NONE', #71774 ) ;
#56263=DIRECTION ( 'NONE',  ( 0.4999999999999998335, -0.8660254037844389297, 0.000000000000000000 ) ) ;
#56266=CARTESIAN_POINT ( 'NONE',  ( 157.3029956111992362, 258.1902147490555421, -18.22269824972649843 ) ) ;
#56267=CARTESIAN_POINT ( 'NONE',  ( 101.8248682511026573, 241.8464784336661637, 1.353441290958777525E-15 ) ) ;
#56268=CARTESIAN_POINT ( 'NONE',  ( 87.85384634344086408, 209.9824982072973683, 3.021315404115420679E-15 ) ) ;
#56270=CARTESIAN_POINT ( 'NONE',  ( 161.5510569556734026, 266.9624290277901082, 16.50852780982408063 ) ) ;
#56273=DIRECTION ( 'NONE',  ( -0.8660254037844387076, -0.4999999999999998890, -0.000000000000000000 ) ) ;
#56275=CARTESIAN_POINT ( 'NONE',  ( 63.26028190641562787, 198.1423013555410080, -4.594050593750043987 ) ) ;
#56277=CARTESIAN_POINT ( 'NONE',  ( 191.2056514706806070, 299.4690922889112699, 7.290007621276087590 ) ) ;
#56279=CARTESIAN_POINT ( 'NONE',  ( -2.524136441754524451, 180.8967562850347406, 2.649461200531984646E-14 ) ) ;
#56280=ORIENTED_EDGE ( 'NONE', *, *, #15389, .F. ) ;
#56282=CARTESIAN_POINT ( 'NONE',  ( 178.0023654785463236, 288.9504702553427933, 11.05621428587497590 ) ) ;
#56285=ORIENTED_EDGE ( 'NONE', *, *, #43673, .F. ) ;
#56286=CARTESIAN_POINT ( 'NONE',  ( 171.8293707807498265, 259.1554194294824924, -13.74145718453054954 ) ) ;
#56287=CARTESIAN_POINT ( 'NONE',  ( 174.2793283849268562, 277.1922490460319182, -15.62918738185294742 ) ) ;
#56288=CARTESIAN_POINT ( 'NONE',  ( 161.1150691641480535, 251.5875096731584506, -13.48836942566120101 ) ) ;
#56290=CARTESIAN_POINT ( 'NONE',  ( 50.57404612423096069, 211.5530062829863027, -4.648177544792955347E-16 ) ) ;
#56293=CARTESIAN_POINT ( 'NONE',  ( 180.8203030686837280, 271.2954033567903025, 17.04059064758568454 ) ) ;
#56294=FACE_OUTER_BOUND ( 'NONE', #24130, .T. ) ;
#56296=CARTESIAN_POINT ( 'NONE',  ( 153.8622324351665043, 264.6225750775929555, -16.50275939780754086 ) ) ;
#56297=CARTESIAN_POINT ( 'NONE',  ( 176.5738172124948164, 284.4749987453067774, 14.65120015815750421 ) ) ;
#56298=VECTOR ( 'NONE', #49450, 1000.000000000000000 ) ;
#56299=CARTESIAN_POINT ( 'NONE',  ( 110.1064097226738312, 240.5024278399161233, 9.188101187500095079 ) ) ;
#56300=ORIENTED_EDGE ( 'NONE', *, *, #77679, .T. ) ;
#56301=CARTESIAN_POINT ( 'NONE',  ( 147.1259762202154207, 275.8173294038533641, -0.6716460511724978710 ) ) ;
#56303=CARTESIAN_POINT ( 'NONE',  ( 202.9547455376043672, 279.1190644220934018, -15.19669173352461478 ) ) ;
#56304=CARTESIAN_POINT ( 'NONE',  ( 204.2457645315488719, 276.8829539310449945, 14.53406579917280261 ) ) ;
#56306=CARTESIAN_POINT ( 'NONE',  ( 175.0760097641222330, 252.5203264472857256, 5.202907413956480376 ) ) ;
#56307=EDGE_LOOP ( 'NONE', ( #48818, #82493, #35756, #74745 ) ) ;
#56309=CARTESIAN_POINT ( 'NONE',  ( 154.7226985476829384, 273.3457454102759812, -13.10063029118530586 ) ) ;
#56312=CARTESIAN_POINT ( 'NONE',  ( 164.5696622524448287, 245.6039789247527096, -0.9250471598561700315 ) ) ;
#56313=CARTESIAN_POINT ( 'NONE',  ( 144.0982539169780523, 247.8768266524160140, 9.188101187500096856 ) ) ;
#56314=CARTESIAN_POINT ( 'NONE',  ( 198.6363782946250183, 286.5986958926748116, -18.50260615857378355 ) ) ;
#56315=AXIS2_PLACEMENT_3D ( 'NONE', #13231, #75028, #47803 ) ;
#56316=B_SPLINE_CURVE_WITH_KNOTS ( 'NONE', 3,
 ( #43768, #53367, #21973, #59960 ),
 .UNSPECIFIED., .F., .F.,
 ( 4, 4 ),
 ( 0.01375087555092867168, 0.01505699899481918562 ),
 .UNSPECIFIED. ) ;
#56317=CARTESIAN_POINT ( 'NONE',  ( 190.0398248856338057, 298.8169614316505545, -8.166243001185458539 ) ) ;
#56319=CARTESIAN_POINT ( 'NONE',  ( 63.28708487846012076, 207.3458772461660544, 9.188101187500095079 ) ) ;
#56320=CARTESIAN_POINT ( 'NONE',  ( 164.9779129355220562, 244.8968679994381148, -1.771286574179712803 ) ) ;
#56321=CARTESIAN_POINT ( 'NONE',  ( 157.3198323354746435, 258.1610526871778006, -16.77630483474704093 ) ) ;
#56324=CARTESIAN_POINT ( 'NONE',  ( 174.6693944358695774, 261.9625217202849399, 14.25614487736958047 ) ) ;
#56325=CARTESIAN_POINT ( 'NONE',  ( 170.8865616681041786, 262.8912071418242817, 16.88624067591380040 ) ) ;
#56326=CARTESIAN_POINT ( 'NONE',  ( 178.3571982967953602, 292.6181790745828835, -7.174879954037646002 ) ) ;
#56328=CARTESIAN_POINT ( 'NONE',  ( 178.3225333605271317, 261.2550961346064469, 13.20358700637163096 ) ) ;
#56330=CARTESIAN_POINT ( 'NONE',  ( 119.9486011388742384, 253.3927522451419350, 2.944929066748280225E-16 ) ) ;
#56333=CARTESIAN_POINT ( 'NONE',  ( 148.1634546024981205, 274.0203641339852538, 9.324875965062235039 ) ) ;
#56335=CARTESIAN_POINT ( 'NONE',  ( 41.52819660837609916, 194.7833772461660544, -9.188101187500095079 ) ) ;
#56338=CARTESIAN_POINT ( 'NONE',  ( 82.65769392073423205, 206.9824982072973683, 3.021315404115420679E-15 ) ) ;
#56339=CARTESIAN_POINT ( 'NONE',  ( 147.4811722709131914, 275.2021117973970377, 3.890385073228495916 ) ) ;
#56342=CARTESIAN_POINT ( 'NONE',  ( 67.12105150802354103, 202.8927522451418213, 10.00000000000009592 ) ) ;
#56343=CARTESIAN_POINT ( 'NONE',  ( 163.0887663364496518, 256.3074304275255599, -16.05814244895578469 ) ) ;
#56344=CARTESIAN_POINT ( 'NONE',  ( -2.070769811622824363, 179.6115022471903160, -5.000000000000047962 ) ) ;
#56346=EDGE_CURVE ( 'NONE', #27863, #690, #11597, .T. ) ;
#56347=ORIENTED_EDGE ( 'NONE', *, *, #737, .F. ) ;
#56348=ADVANCED_FACE ( 'NONE', ( #58535 ), #27667, .T. ) ;
#56349=CARTESIAN_POINT ( 'NONE',  ( 33.00325904164698443, 189.8615022471902591, -10.00000000000009592 ) ) ;
#56350=CARTESIAN_POINT ( 'NONE',  ( 184.6123843791924912, 294.3808565314488419, 10.01802650564912867 ) ) ;
#56351=CARTESIAN_POINT ( 'NONE',  ( 202.4900219881211854, 279.9239892212719383, 15.63116161057562259 ) ) ;
#56353=CARTESIAN_POINT ( 'NONE',  ( 7.428446334363822956, 175.0958772461660544, -9.188101187500095079 ) ) ;
#56356=CARTESIAN_POINT ( 'NONE',  ( 170.4241003537304096, 263.6404983464951215, 15.81189019553032971 ) ) ;
#56357=EDGE_CURVE ( 'NONE', #90465, #28481, #37142, .T. ) ;
#56358=CARTESIAN_POINT ( 'NONE',  ( 32.40786657299730678, 179.5177522451417929, 5.000000000000051514 ) ) ;
#56365=CARTESIAN_POINT ( 'NONE',  ( 76.32488315910845245, 203.3262482093458061, 3.021315404115420679E-15 ) ) ;
#56370=CARTESIAN_POINT ( 'NONE',  ( 153.3589871089347128, 277.7324385553121147, -5.220324751481857817 ) ) ;
#56372=DIRECTION ( 'NONE',  ( 0.4999999999999988343, -0.8660254037844393737, 0.000000000000000000 ) ) ;
#56374=CARTESIAN_POINT ( 'NONE',  ( 206.7893622945242385, 272.4773133715531230, -10.52881283832460291 ) ) ;
#56376=CARTESIAN_POINT ( 'NONE',  ( 152.9262073036446168, 265.7710344717137900, 16.19159804214501008 ) ) ;
#56377=CARTESIAN_POINT ( 'NONE',  ( 165.0437781805843258, 244.7827860485373606, -2.050141714668513693 ) ) ;
#56378=CARTESIAN_POINT ( 'NONE',  ( 99.25420243115655694, 228.1115022471902307, 10.00000000000009592 ) ) ;
#56380=CARTESIAN_POINT ( 'NONE',  ( 194.2669918475045279, 294.1666952169902629, 14.00965265288584050 ) ) ;
#56385=CARTESIAN_POINT ( 'NONE',  ( 159.1645459798114359, 278.1651338649389800, -9.804895797930408108 ) ) ;
#56389=CARTESIAN_POINT ( 'NONE',  ( 205.8099205723994203, 269.1131406545866298, -1.356034389334280776 ) ) ;
#56395=CARTESIAN_POINT ( 'NONE',  ( 177.5865089022509551, 268.7852845103913069, 17.37969943402860906 ) ) ;
#56398=CARTESIAN_POINT ( 'NONE',  ( 166.1221895601162544, 273.9771594711654643, -16.55413630177630324 ) ) ;
#56399=CARTESIAN_POINT ( 'NONE',  ( 190.8443993347725325, 300.0947993426467519, 8.522468760355437212 ) ) ;
#56400=CARTESIAN_POINT ( 'NONE',  ( 176.6379055597627428, 265.0600181157752218, 16.52625651101184445 ) ) ;
#56402=ORIENTED_EDGE ( 'NONE', *, *, #13818, .T. ) ;
#56403=CARTESIAN_POINT ( 'NONE',  ( 171.0309627268963482, 255.8151653478954017, -11.60038586255653570 ) ) ;
#56405=ORIENTED_EDGE ( 'NONE', *, *, #51118, .F. ) ;
#56407=CYLINDRICAL_SURFACE ( 'NONE', #74194, 17.82106496071139645 ) ;
#56408=ORIENTED_EDGE ( 'NONE', *, *, #67141, .T. ) ;
#56410=VERTEX_POINT ( 'NONE', #20067 ) ;
#56412=CARTESIAN_POINT ( 'NONE',  ( 194.0457541550190967, 294.5498901409245036, 13.79567330127564517 ) ) ;
#56413=CARTESIAN_POINT ( 'NONE',  ( 179.8658285908990138, 290.6180032362764223, -9.493696763719416509 ) ) ;
#56415=CARTESIAN_POINT ( 'NONE',  ( 193.7068637079588598, 294.3397739674867921, 13.92549557170472774 ) ) ;
#56417=CARTESIAN_POINT ( 'NONE',  ( 158.8791574486372440, 255.4602223656619628, -17.57574691297732272 ) ) ;
#56422=CARTESIAN_POINT ( 'NONE',  ( 164.8537203408104972, 245.1119758834023230, 2.926011033004258355 ) ) ;
#56423=CARTESIAN_POINT ( 'NONE',  ( 191.4930805452865741, 298.1933573230298862, -9.154694743737874063 ) ) ;
#56425=EDGE_LOOP ( 'NONE', ( #54383, #10954, #13132, #21040 ) ) ;
#56427=FACE_OUTER_BOUND ( 'NONE', #38836, .T. ) ;
#56428=CARTESIAN_POINT ( 'NONE',  ( 169.9170831025614632, 258.3961534647858684, -13.99170300441150161 ) ) ;
#56429=CARTESIAN_POINT ( 'NONE',  ( 186.0715527847238207, 298.7753624933060337, 1.084710433360843940 ) ) ;
#56430=CARTESIAN_POINT ( 'NONE',  ( -22.42236680055709641, 157.8615022471902591, 0.000000000000000000 ) ) ;
#56432=CARTESIAN_POINT ( 'NONE',  ( 200.8432122835317841, 282.7763473000181307, 17.15137370990203891 ) ) ;
#56433=CARTESIAN_POINT ( 'NONE',  ( 191.4738032422262677, 260.7793432447242594, -0.2951778641931921410 ) ) ;
#56434=ORIENTED_EDGE ( 'NONE', *, *, #48838, .F. ) ;
#56437=CARTESIAN_POINT ( 'NONE',  ( 131.0625938207745662, 253.1427522451419350, 10.00000000000009415 ) ) ;
#56438=CARTESIAN_POINT ( 'NONE',  ( 189.4313974406659327, 277.5226620091338532, 17.67960062696096912 ) ) ;
#56440=CARTESIAN_POINT ( 'NONE',  ( 22.95375591501717594, 177.3927522451418497, 10.00000000000009592 ) ) ;
#56441=CARTESIAN_POINT ( 'NONE',  ( 88.99704050542813150, 228.3149278399160949, 9.188101187500093303 ) ) ;
#56444=CARTESIAN_POINT ( 'NONE',  ( 207.6470076888861342, 270.9918279736407385, 2.882721586646819212 ) ) ;
#56446=CARTESIAN_POINT ( 'NONE',  ( 20.93329029645117245, 173.7048013555409796, 4.594050593750051981 ) ) ;
#56447=CARTESIAN_POINT ( 'NONE',  ( 200.1662314894802819, 283.9489124310637180, 17.19420058542677054 ) ) ;
#56448=ORIENTED_EDGE ( 'NONE', *, *, #91408, .F. ) ;
#56452=CARTESIAN_POINT ( 'NONE',  ( 198.3425264013990272, 266.1585612424889291, -2.872493559038742372 ) ) ;
#56455=CARTESIAN_POINT ( 'NONE',  ( 194.8742882536625984, 264.7950142703134020, -4.379131112317717012 ) ) ;
#56460=CARTESIAN_POINT ( 'NONE',  ( 32.43492986863949312, 189.5333772461660544, 9.188101187500095079 ) ) ;
#56461=CARTESIAN_POINT ( 'NONE',  ( 88.62734903533713293, 208.6427522451417644, 1.119607411625061291E-15 ) ) ;
#56464=CARTESIAN_POINT ( 'NONE',  ( 179.0311786453646334, 258.6304024054584261, -10.01495405547345641 ) ) ;
#56466=CARTESIAN_POINT ( 'NONE',  ( -3.586574591843265658, 177.9244531367911577, -4.594050593750046652 ) ) ;
#56467=B_SPLINE_CURVE_WITH_KNOTS ( 'NONE', 3,
 ( #67978, #53271, #14277, #45169 ),
 .UNSPECIFIED., .F., .F.,
 ( 4, 4 ),
 ( 2.465251413651021934E-15, 0.003756095204294760022 ),
 .UNSPECIFIED. ) ;
#56469=CARTESIAN_POINT ( 'NONE',  ( 161.5083988044524119, 250.9062427520286178, -14.53522982831775856 ) ) ;
#56470=CARTESIAN_POINT ( 'NONE',  ( 187.8161210723351644, 283.3479265774896589, 16.26191486346292692 ) ) ;
#56471=CARTESIAN_POINT ( 'NONE',  ( 194.8067605455144076, 293.2317884077015151, -16.00245909155922774 ) ) ;
#56472=EDGE_CURVE ( 'NONE', #99390, #79855, #70647, .T. ) ;
#56474=CARTESIAN_POINT ( 'NONE',  ( 164.4864504671816690, 245.7481059646165704, 6.337356894698421783 ) ) ;
#56475=CARTESIAN_POINT ( 'NONE',  ( 146.6834825911944620, 276.5837508513432681, 0.6716460511724984261 ) ) ;
#56476=CARTESIAN_POINT ( 'NONE',  ( 207.0548180518391916, 272.0175305127218053, 7.721676452263806389 ) ) ;
#56478=CARTESIAN_POINT ( 'NONE',  ( 164.1146561143383167, 246.3920726737087534, -7.362905700427413436 ) ) ;
#56479=CARTESIAN_POINT ( 'NONE',  ( 161.4628698183636857, 251.3853568467309572, -13.03279659859947870 ) ) ;
#56480=CARTESIAN_POINT ( 'NONE',  ( 105.9656389868882513, 241.1744531367911577, 4.594050593750047540 ) ) ;
#56483=ADVANCED_FACE ( 'NONE', ( #88020 ), #57819, .F. ) ;
#56484=CARTESIAN_POINT ( 'NONE',  ( 156.6812872898450735, 261.2670451491295012, 0.000000000000000000 ) ) ;
#56485=CARTESIAN_POINT ( 'NONE',  ( 195.6986305151803549, 291.6870243064952888, 16.84182339398051909 ) ) ;
#56486=CARTESIAN_POINT ( 'NONE',  ( 185.5233448779797243, 288.1480361044887673, 15.07821780549886803 ) ) ;
#56487=CARTESIAN_POINT ( 'NONE',  ( 150.7975480795134615, 269.4579803999092178, -13.77803079712401590 ) ) ;
#56489=EDGE_CURVE ( 'NONE', #23455, #34725, #49601, .T. ) ;
#56490=CARTESIAN_POINT ( 'NONE',  ( 189.8073911343818452, 261.0592632349233781, -4.572445870894544129 ) ) ;
#56491=CARTESIAN_POINT ( 'NONE',  ( 149.3141802193904368, 272.0272488999566463, -11.40332369054239336 ) ) ;
#56493=CARTESIAN_POINT ( 'NONE',  ( 173.1255070585075941, 289.7719922078085233, -1.455481432696650979 ) ) ;
#56495=ORIENTED_EDGE ( 'NONE', *, *, #73975, .F. ) ;
#56496=CARTESIAN_POINT ( 'NONE',  ( 189.0598825607623326, 265.6785374324029476, 10.85450195960190634 ) ) ;
#56497=CARTESIAN_POINT ( 'NONE',  ( 175.0906617674605741, 279.3930328189767920, 16.49259839202913724 ) ) ;
#56498=CARTESIAN_POINT ( 'NONE',  ( 165.4679322623151734, 269.7639896636108006, -16.28713546330200046 ) ) ;
#56499=CARTESIAN_POINT ( 'NONE',  ( 200.2206280980474276, 272.4473840335176078, 12.62891601330385427 ) ) ;
#56502=CARTESIAN_POINT ( 'NONE',  ( 153.3616370783189211, 265.0168479788495688, 17.48287904751960653 ) ) ;
#56506=CARTESIAN_POINT ( 'NONE',  ( 192.0496571061401028, 288.1032038373080582, -15.86509381273373442 ) ) ;
#56509=CARTESIAN_POINT ( 'NONE',  ( 148.1974503712686158, 273.9614817352322120, -7.884397846570731616 ) ) ;
#56514=CYLINDRICAL_SURFACE ( 'NONE', #36248, 17.82106496071139645 ) ;
#56519=CARTESIAN_POINT ( 'NONE',  ( 183.8043731368310603, 268.5938253857621589, 16.29461355553033997 ) ) ;
#56520=CARTESIAN_POINT ( 'NONE',  ( 203.5258219653775313, 278.1299310341851765, -16.21052911601769608 ) ) ;
#56523=CARTESIAN_POINT ( 'NONE',  ( 178.3597279735877805, 261.0516804887051308, 12.18819909079894082 ) ) ;
#56526=ORIENTED_EDGE ( 'NONE', *, *, #49871, .T. ) ;
#56529=CARTESIAN_POINT ( 'NONE',  ( 203.5258219653775313, 278.1299310341851765, -16.21052911601769608 ) ) ;
#56531=CARTESIAN_POINT ( 'NONE',  ( 183.2409096537462290, 280.5924353467958667, -16.12459997820720758 ) ) ;
#56532=CARTESIAN_POINT ( 'NONE',  ( 147.2639185929470216, 275.5784062057657025, -6.046059379523592625 ) ) ;
#56533=CARTESIAN_POINT ( 'NONE',  ( 158.6745544753717354, 275.0482988461347986, -12.54501861896559056 ) ) ;
#56535=CARTESIAN_POINT ( 'NONE',  ( 200.9812045408918380, 282.5373376992193926, -16.61165062382494284 ) ) ;
#56537=CARTESIAN_POINT ( 'NONE',  ( 157.3303612352329424, 280.6659801480934107, 2.084183637465919059 ) ) ;
#56538=CARTESIAN_POINT ( 'NONE',  ( 129.0235653626489238, 254.4869531367911577, 4.594050593750046652 ) ) ;
#56543=EDGE_CURVE ( 'NONE', #68198, #49338, #21073, .T. ) ;
#56544=CARTESIAN_POINT ( 'NONE',  ( 153.9946444333862416, 274.9169454665982357, 12.01620693575389964 ) ) ;
#56545=VERTEX_POINT ( 'NONE', #22033 ) ;
#56546=CARTESIAN_POINT ( 'NONE',  ( 200.9975768615754248, 274.6372745081091580, 13.39944341616547163 ) ) ;
#56547=CARTESIAN_POINT ( 'NONE',  ( 178.1271951506071503, 254.3491337373919805, 1.338458689122108636 ) ) ;
#56548=EDGE_CURVE ( 'NONE', #47191, #26620, #92800, .T. ) ;
#56549=CARTESIAN_POINT ( 'NONE',  ( 173.2306762196021452, 290.4478550908166312, -4.991672751549263154 ) ) ;
#56551=CARTESIAN_POINT ( 'NONE',  ( 156.6787608129567673, 279.1700930814473622, 7.332212251875458442 ) ) ;
#56552=CARTESIAN_POINT ( 'NONE',  ( 200.6737073311291795, 283.0699384897140476, -17.61533935526990291 ) ) ;
#56553=CARTESIAN_POINT ( 'NONE',  ( 177.0600935255706077, 288.7082641331545574, -9.311180906940547786 ) ) ;
#56557=CARTESIAN_POINT ( 'NONE',  ( 184.4132702264047623, 272.8584048094892296, -16.31558729584348200 ) ) ;
#56561=ADVANCED_FACE ( 'NONE', ( #8337 ), #1753, .T. ) ;
#56562=CARTESIAN_POINT ( 'NONE',  ( 156.4559187165143612, 277.2225799599395373, 9.956371387236824688 ) ) ;
#56563=CARTESIAN_POINT ( 'NONE',  ( 191.5479541429108963, 298.8762066690417782, -9.571052778213795520 ) ) ;
#56564=CARTESIAN_POINT ( 'NONE',  ( 190.7705347155322499, 300.2227366160529414, 3.504769718465625239 ) ) ;
#56565=CARTESIAN_POINT ( 'NONE',  ( 163.1484656051875106, 248.0655637253488806, 9.714247672444804138 ) ) ;
#56566=CARTESIAN_POINT ( 'NONE',  ( 164.1916602900412840, 284.1804194194341449, -7.017349331522431122 ) ) ;
#56567=CARTESIAN_POINT ( 'NONE',  ( 160.4083209155708118, 282.4522129528954224, 6.632880642079271638 ) ) ;
#56575=CARTESIAN_POINT ( 'NONE',  ( 21.76528272068881265, 171.8262482093457777, 3.021315404115420679E-15 ) ) ;
#56579=CARTESIAN_POINT ( 'NONE',  ( -10.27112140336314994, 171.0024278399161233, -9.188101187500093303 ) ) ;
#56580=CARTESIAN_POINT ( 'NONE',  ( 90.40467888234286420, 216.8768266524159856, -9.188101187500091527 ) ) ;
#56581=CARTESIAN_POINT ( 'NONE',  ( 192.4172326059820648, 297.3705722050773943, -12.52563289807247848 ) ) ;
#56587=CARTESIAN_POINT ( 'NONE',  ( 164.1212835565148396, 284.3603666608088929, 5.877658627662431634 ) ) ;
#56590=CARTESIAN_POINT ( 'NONE',  ( 161.5437845330232278, 250.8449528722815387, 12.69943054604137700 ) ) ;
#56597=EDGE_CURVE ( 'NONE', #45081, #22391, #88982, .T. ) ;
#56598=CARTESIAN_POINT ( 'NONE',  ( 36.33204418566946714, 191.7833772461660544, -9.188101187500095079 ) ) ;
#56599=B_SPLINE_CURVE_WITH_KNOTS ( 'NONE', 3,
 ( #87462, #86943, #88955, #49377 ),
 .UNSPECIFIED., .F., .F.,
 ( 4, 4 ),
 ( 0.008971156174964484836, 0.01512143528327676567 ),
 .UNSPECIFIED. ) ;
#56600=CARTESIAN_POINT ( 'NONE',  ( 175.6775075963462882, 265.1320719190924819, -16.53680973885410310 ) ) ;
#56601=CARTESIAN_POINT ( 'NONE',  ( 66.99449581658849695, 218.6744531367911293, 4.594050593750047540 ) ) ;
#56602=CARTESIAN_POINT ( 'NONE',  ( 161.1232569692349443, 251.5733279787459367, -14.02750397520710557 ) ) ;
#56603=CARTESIAN_POINT ( 'NONE',  ( 143.8748646542946688, 242.3262482093457777, 3.021315404115420679E-15 ) ) ;
#56605=CARTESIAN_POINT ( 'NONE',  ( 163.3771092991411820, 258.0155440589538784, 15.65363653094946983 ) ) ;
#56607=CARTESIAN_POINT ( 'NONE',  ( 175.6771667394953340, 269.4680136230451808, -17.60694476279005372 ) ) ;
#56609=EDGE_CURVE ( 'NONE', #8540, #26223, #58739, .T. ) ;
#56613=ORIENTED_EDGE ( 'NONE', *, *, #52945, .T. ) ;
#56615=CARTESIAN_POINT ( 'NONE',  ( 83.28711936893076029, 209.7048013555409796, 4.594050593750051981 ) ) ;
#56617=CARTESIAN_POINT ( 'NONE',  ( 173.0983074211377470, 289.6757823250843558, -1.024440707233354564 ) ) ;
#56619=CARTESIAN_POINT ( 'NONE',  ( 202.0466495549300419, 280.6919328022345894, 16.59926557204200037 ) ) ;
#56620=ADVANCED_FACE ( 'NONE', ( #93974 ), #22198, .T. ) ;
#56623=CARTESIAN_POINT ( 'NONE',  ( 190.8236500841018426, 286.9672700043819873, 16.17145961683961275 ) ) ;
#56624=CARTESIAN_POINT ( 'NONE',  ( 119.5336306364421404, 246.4865022471903160, 10.00000000000009237 ) ) ;
#56625=CARTESIAN_POINT ( 'NONE',  ( 204.9184781223158609, 275.7177798128946620, -12.59106622113254126 ) ) ;
#56627=ORIENTED_EDGE ( 'NONE', *, *, #4791, .F. ) ;
#56630=CARTESIAN_POINT ( 'NONE',  ( 202.8499463704053198, 279.3005819042728604, 17.04674939340617001 ) ) ;
#56631=CARTESIAN_POINT ( 'NONE',  ( 207.4148751195968430, 270.8028853205232167, -0.5370135912211878582 ) ) ;
#56636=CARTESIAN_POINT ( 'NONE',  ( 189.2316387673287181, 290.2037436208335635, 14.34142323116202533 ) ) ;
#56637=CARTESIAN_POINT ( 'NONE',  ( 170.6604352838296847, 250.4273314685328558, 3.327069490116406847 ) ) ;
#56638=CARTESIAN_POINT ( 'NONE',  ( 206.9737897634393846, 271.6399641097157200, -5.521983748659117452 ) ) ;
#56645=FACE_OUTER_BOUND ( 'NONE', #16889, .T. ) ;
#56647=VERTEX_POINT ( 'NONE', #39697 ) ;
#56650=CARTESIAN_POINT ( 'NONE',  ( 148.1632261683078013, 274.0207597936089883, -7.853210555358286271 ) ) ;
#56652=CARTESIAN_POINT ( 'NONE',  ( 193.7114073116034945, 295.1289958610702797, 14.86160832869823345 ) ) ;
#56653=CARTESIAN_POINT ( 'NONE',  ( 185.1804351182116193, 292.8895488603085937, -11.95798946474453928 ) ) ;
#56654=CARTESIAN_POINT ( 'NONE',  ( 171.9695299662907360, 276.3046275190319534, -16.98996149290084645 ) ) ;
#56655=CARTESIAN_POINT ( 'NONE',  ( 207.6348398075022317, 271.0129033624181147, -3.614878161448662031 ) ) ;
#56657=CARTESIAN_POINT ( 'NONE',  ( 204.4836193250905012, 269.4642819889133989, 2.448151338453079973 ) ) ;
#56658=CARTESIAN_POINT ( 'NONE',  ( 181.1477013271936016, 287.8971774238942203, -14.15342935774602218 ) ) ;
#56659=CARTESIAN_POINT ( 'NONE',  ( 95.22211873877630239, 213.5327760586659451, 1.948934522072303157E-15 ) ) ;
#56661=CARTESIAN_POINT ( 'NONE',  ( 150.3288696065234262, 271.5028661687476301, 12.61327273338345734 ) ) ;
#56662=CARTESIAN_POINT ( 'NONE',  ( 164.8075539017095252, 280.4672370525465226, 12.63796469268613265 ) ) ;
#56665=CARTESIAN_POINT ( 'NONE',  ( 168.3202193441510701, 267.1935196533576686, -17.15840090500419635 ) ) ;
#56666=ORIENTED_EDGE ( 'NONE', *, *, #47497, .F. ) ;
#56670=CARTESIAN_POINT ( 'NONE',  ( 159.8732321751776624, 253.7384344327741132, -15.51998349828054202 ) ) ;
#56671=CARTESIAN_POINT ( 'NONE',  ( 207.6256228060221076, 271.0288676772754002, 1.885008341157026646 ) ) ;
#56672=CARTESIAN_POINT ( 'NONE',  ( 92.97525793012167128, 233.6744531367911293, 4.594050593750047540 ) ) ;
#56676=B_SPLINE_SURFACE_WITH_KNOTS ( 'NONE', 3, 1, ( 
 ( #69050, #17742 ),
 ( #46755, #162 ),
 ( #31544, #99980 ),
 ( #7250, #14853 ),
 ( #54331, #31049 ),
 ( #53836, #48642 ),
 ( #62432, #61936 ),
 ( #23442, #84796 ),
 ( #85303, #15846 ),
 ( #77683, #15337 ),
 ( #71945, #10138 ),
 ( #8266, #80070 ),
 ( #38132, #70044 ),
 ( #61449, #93395 ),
 ( #23946, #46232 ),
 ( #30055, #25848 ),
 ( #77156, #41003 ),
 ( #18243, #10641 ),
 ( #84305, #45740 ),
 ( #76662, #81079 ),
 ( #72957, #13139 ),
 ( #80576, #27336 ),
 ( #90164, #72459 ),
 ( #11156, #65809 ),
 ( #64837, #59188 ),
 ( #5031, #35420 ),
 ( #96770, #42023 ),
 ( #58217, #73933 ),
 ( #89196, #34427 ),
 ( #12133, #12642 ),
 ( #66814, #26831 ),
 ( #19744, #73441 ),
 ( #4025, #43512 ),
 ( #20737, #19260 ) ),
 .UNSPECIFIED., .T., .F., .F.,
 ( 4, 2, 2, 2, 2, 2, 2, 2, 2, 2, 2, 2, 2, 2, 2, 2, 4 ),
 ( 2, 2 ),
 ( 0.000000000000000000, 0.06250000000000000000, 0.1250000000000000000, 0.1875000000000000000, 0.2500000000000000000, 0.3125000000000000000, 0.3750000000000000000, 0.4375000000000000000, 0.5000000000000000000, 0.5625000000000000000, 0.6250000000000000000, 0.6875000000000000000, 0.7500000000000000000, 0.8125000000000000000, 0.8750000000000000000, 0.9375000000000000000, 1.000000000000000000 ),
 ( 0.000000000000000000, 1.000000000000000000 ),
 .UNSPECIFIED. ) ;
#56677=CARTESIAN_POINT ( 'NONE',  ( 162.6541320028305506, 248.9217746405196294, -10.16950121496441817 ) ) ;
#56678=ORIENTED_EDGE ( 'NONE', *, *, #9835, .T. ) ;
#56679=EDGE_CURVE ( 'NONE', #41296, #23987, #65924, .T. ) ;
#56681=CARTESIAN_POINT ( 'NONE',  ( 165.2848724275795291, 285.9158859995100102, 1.309848662535952224 ) ) ;
#56686=CARTESIAN_POINT ( 'NONE',  ( 156.7173554537088194, 259.2045732567815435, 17.96992492779905959 ) ) ;
#56687=CARTESIAN_POINT ( 'NONE',  ( 160.6540796618634488, 275.6309760589927578, 12.88432021873685329 ) ) ;
#56688=CARTESIAN_POINT ( 'NONE',  ( 159.9647205790309101, 253.5799718689968927, -16.48298384325780219 ) ) ;
#56690=CARTESIAN_POINT ( 'NONE',  ( 165.0391502558331069, 249.6778246878102436, -10.74756611015070717 ) ) ;
#56692=( BOUNDED_CURVE ( )  B_SPLINE_CURVE ( 2, ( #34804, #58595, #89568, #20130, #51002, #90055, #81954, #6420, #38286 ),
 .UNSPECIFIED., .F., .T. ) 
 B_SPLINE_CURVE_WITH_KNOTS ( ( 3, 2, 2, 2, 3 ),
 ( 0.4556451612903225645, 0.4569892473118279397, 0.4596774193548386900, 0.4623655913978494403, 0.4637096774193548154 ),
 .UNSPECIFIED. ) 
 CURVE ( )  GEOMETRIC_REPRESENTATION_ITEM ( )  RATIONAL_B_SPLINE_CURVE ( ( 0.9330127018922194093, 0.9330127018922194093, 1.000000000000000000, 0.8660254037844387076, 1.000000000000000000, 0.8660254037844387076, 1.000000000000000000, 0.9330127018922194093, 0.9330127018922194093 ) ) 
 REPRESENTATION_ITEM ( '' )  );
#56695=CARTESIAN_POINT ( 'NONE',  ( -22.42236680055709641, 157.8615022471902591, 0.000000000000000000 ) ) ;
#56697=CARTESIAN_POINT ( 'NONE',  ( 149.0802483013170558, 274.4411750002399231, 9.053613739816581685 ) ) ;
#56698=CARTESIAN_POINT ( 'NONE',  ( 200.1662314894802819, 283.9489124310637180, 17.19420058542677054 ) ) ;
#56700=CARTESIAN_POINT ( 'NONE',  ( 167.6894627267040221, 249.8065173834789618, 7.802750152793692884 ) ) ;
#56703=B_SPLINE_CURVE_WITH_KNOTS ( 'NONE', 3,
 ( #83856, #14422, #78220, #85876 ),
 .UNSPECIFIED., .F., .F.,
 ( 4, 4 ),
 ( 0.007911187398149459662, 0.01299107505613515852 ),
 .UNSPECIFIED. ) ;
#56704=LINE ( 'NONE', #72938, #5794 ) ;
#56707=CARTESIAN_POINT ( 'NONE',  ( 165.0156970625405108, 244.8314239717225007, -1.890480716182876719 ) ) ;
#56708=CARTESIAN_POINT ( 'NONE',  ( 182.1950578011920356, 264.4196723021682942, 13.52627809525725766 ) ) ;
#56709=CARTESIAN_POINT ( 'NONE',  ( 181.4632975752175525, 255.1188003790442167, 1.936479460681336695 ) ) ;
#56712=CARTESIAN_POINT ( 'NONE',  ( 180.7241246963670278, 273.1865840351073871, 16.76835723274534473 ) ) ;
#56713=CARTESIAN_POINT ( 'NONE',  ( 161.1099616491931386, 273.3624908465563408, -15.23233197322572074 ) ) ;
#56715=CARTESIAN_POINT ( 'NONE',  ( 161.4816992964961742, 250.9524876563463067, -12.92750327687364198 ) ) ;
#56717=CARTESIAN_POINT ( 'NONE',  ( 7.212287079182728711, 162.7202760586659736, -5.415160957724236172E-17 ) ) ;
#56721=EDGE_CURVE ( 'NONE', #49930, #91334, #26114, .T. ) ;
#56724=CARTESIAN_POINT ( 'NONE',  ( 41.71789998727770410, 185.7048013555409796, 4.594050593750051981 ) ) ;
#56725=CARTESIAN_POINT ( 'NONE',  ( 164.4698008747318738, 245.7769439046653019, -6.272955660526681854 ) ) ;
#56727=CARTESIAN_POINT ( 'NONE',  ( 200.1294354126899009, 267.3366221627135246, -6.812218948514619399 ) ) ;
#56728=CARTESIAN_POINT ( 'NONE',  ( 146.6138605399200117, 276.7043397814778132, -0.5394499176159462950 ) ) ;
#56729=CARTESIAN_POINT ( 'NONE',  ( 149.5042310455230563, 271.6980712130745701, 11.54652286044134613 ) ) ;
#56730=CARTESIAN_POINT ( 'NONE',  ( 182.5277673056334891, 280.1954785146588733, -16.09861734911579489 ) ) ;
#56732=CARTESIAN_POINT ( 'NONE',  ( 186.5436611748800999, 296.3120891398685899, -8.818239198042506999 ) ) ;
#56735=CARTESIAN_POINT ( 'NONE',  ( 80.56248746614240019, 223.9865022471902876, 10.00000000000009237 ) ) ;
#56738=CARTESIAN_POINT ( 'NONE',  ( 41.20343708195693466, 194.5958772461660544, -9.188101187500095079 ) ) ;
#56739=CARTESIAN_POINT ( 'NONE',  ( -1.617403181491035902, 158.3262482093458061, 3.021315404115420679E-15 ) ) ;
#56740=ORIENTED_EDGE ( 'NONE', *, *, #11054, .T. ) ;
#56742=CARTESIAN_POINT ( 'NONE',  ( 147.5848197185516142, 275.0225891520124151, 4.420251097676741736 ) ) ;
#56744=ORIENTED_EDGE ( 'NONE', *, *, #11433, .F. ) ;
#56745=CARTESIAN_POINT ( 'NONE',  ( 167.3695604279846805, 285.2551170359605521, 7.881098619243475767 ) ) ;
#56748=CARTESIAN_POINT ( 'NONE',  ( 191.1996875990947444, 299.0642907557634658, -7.109168602002305271 ) ) ;
#56750=CARTESIAN_POINT ( 'NONE',  ( 163.1484656051875106, 248.0655637253488806, 9.714247672444804138 ) ) ;
#56751=CARTESIAN_POINT ( 'NONE',  ( 196.5475899070771675, 290.2165835061676944, -17.89382743182097002 ) ) ;
#56752=CARTESIAN_POINT ( 'NONE',  ( 171.8181756328044116, 255.8907789784637998, 11.22456348869178910 ) ) ;
#56758=CARTESIAN_POINT ( 'NONE',  ( 178.6323200210636344, 282.3665200627499416, 15.66371996646872056 ) ) ;
#56759=CARTESIAN_POINT ( 'NONE',  ( 151.1926529451685326, 268.7736386982768408, 14.30343427984827365 ) ) ;
#56762=EDGE_LOOP ( 'NONE', ( #33339, #6605, #27104, #86969 ) ) ;
#56766=CARTESIAN_POINT ( 'NONE',  ( 182.2373335159190901, 280.9600371166583841, -17.30031729693378040 ) ) ;
#56767=ORIENTED_EDGE ( 'NONE', *, *, #9145, .F. ) ;
#56768=CARTESIAN_POINT ( 'NONE',  ( 200.7484899876179441, 282.9404111291507888, -16.88964748465601673 ) ) ;
#56772=EDGE_CURVE ( 'NONE', #77760, #43169, #78845, .T. ) ;
#56773=CARTESIAN_POINT ( 'NONE',  ( 157.1269483542914998, 258.4951375425532092, -17.15328932028234377 ) ) ;
#56774=CARTESIAN_POINT ( 'NONE',  ( 113.2460989071574460, 230.0643266524159856, 9.188101187500095079 ) ) ;
#56775=CARTESIAN_POINT ( 'NONE',  ( 184.1050185429027124, 288.7504959939380456, -13.16857183658926367 ) ) ;
#56776=ORIENTED_EDGE ( 'NONE', *, *, #38040, .F. ) ;
#56777=CARTESIAN_POINT ( 'NONE',  ( 208.0692320075777957, 270.2605140014760536, 2.043861372130216569 ) ) ;
#56778=ORIENTED_EDGE ( 'NONE', *, *, #51860, .T. ) ;
#56780=CARTESIAN_POINT ( 'NONE',  ( 159.2511875226268216, 254.8158473755685520, 15.75855490706745599 ) ) ;
#56782=CARTESIAN_POINT ( 'NONE',  ( 62.82726920452340380, 197.8923013555409796, 4.594050593750050204 ) ) ;
#56784=CARTESIAN_POINT ( 'NONE',  ( 190.8623743139412454, 300.0636657654615647, 8.577953960666059530 ) ) ;
#56785=CARTESIAN_POINT ( 'NONE',  ( 198.5799742811345823, 286.6963905097911152, 17.08859794237710261 ) ) ;
#56786=CARTESIAN_POINT ( 'NONE',  ( 176.0425021715459195, 272.9246667940608972, 16.74622359246633962 ) ) ;
#56789=CARTESIAN_POINT ( 'NONE',  ( 176.7233542493291907, 288.6475378244585954, 11.36909801418409494 ) ) ;
#56791=ORIENTED_EDGE ( 'NONE', *, *, #59835, .T. ) ;
#56792=CARTESIAN_POINT ( 'NONE',  ( 110.2158993104859945, 222.8932355074535678, -2.679491924311248496 ) ) ;
#56794=CARTESIAN_POINT ( 'NONE',  ( 161.8839333999304415, 250.2557977526613229, -13.90128376743482441 ) ) ;
#56797=CARTESIAN_POINT ( 'NONE',  ( 190.7862358025146534, 300.1955415356651429, 3.573119809004446257 ) ) ;
#56798=CARTESIAN_POINT ( 'NONE',  ( 177.1800844086890265, 269.5441809915307658, 16.12773907670574047 ) ) ;
#56799=CARTESIAN_POINT ( 'NONE',  ( 205.8452707775803390, 274.1125278458945900, 11.42742867493066328 ) ) ;
#56801=CARTESIAN_POINT ( 'NONE',  ( 164.5456390861338889, 254.4766699602316748, 14.11842207354146517 ) ) ;
#56802=CARTESIAN_POINT ( 'NONE',  ( 164.4698008747318738, 245.7769439046653019, -6.272955660526681854 ) ) ;
#56803=CARTESIAN_POINT ( 'NONE',  ( 124.5044291563551297, 236.5643266524159856, -9.188101187500093303 ) ) ;
#56807=CARTESIAN_POINT ( 'NONE',  ( 173.4505375608857491, 284.9503170016366198, -13.05978560202663452 ) ) ;
#56809=CARTESIAN_POINT ( 'NONE',  ( 204.1793240545508752, 276.9980322128846524, 14.17550310845996187 ) ) ;
#56811=CARTESIAN_POINT ( 'NONE',  ( 126.8249895137406043, 232.4824982072973683, 3.021315404115420679E-15 ) ) ;
#56814=EDGE_LOOP ( 'NONE', ( #15051, #34603, #52924, #96557, #5417, #1605, #90578, #1093, #13096, #49197, #36117, #68596, #42347, #81267, #10810, #97057, #84270, #9412, #1976, #88146 ) ) ;
#56816=CARTESIAN_POINT ( 'NONE',  ( 158.4257592686963392, 274.9310561177994714, -12.53665520930496236 ) ) ;
#56818=CARTESIAN_POINT ( 'NONE',  ( 206.2849804695184446, 273.3509283188774930, -9.687080623179198824 ) ) ;
#56819=CARTESIAN_POINT ( 'NONE',  ( 140.9585647324944659, 258.3149278399160380, 9.188101187500093303 ) ) ;
#56820=CARTESIAN_POINT ( 'NONE',  ( 195.7075834170777568, 263.4542553332885291, 0.8725129583350295093 ) ) ;
#56821=CARTESIAN_POINT ( 'NONE',  ( 186.4625004638162977, 297.1001920529987501, 4.671785278466259683 ) ) ;
#56823=CARTESIAN_POINT ( 'NONE',  ( 63.01627839189497138, 213.3149278399160949, 9.188101187500093303 ) ) ;
#56824=CARTESIAN_POINT ( 'NONE',  ( 157.8696211474012330, 257.2087905314882619, -17.27527248276125604 ) ) ;
#56825=CARTESIAN_POINT ( 'NONE',  ( 174.3370073287761670, 251.3632962845142629, 3.630733893980507609 ) ) ;
#56826=CARTESIAN_POINT ( 'NONE',  ( 171.9118076701954578, 260.5665906372238396, 14.62201537552227393 ) ) ;
#56827=CARTESIAN_POINT ( 'NONE',  ( 155.3846098364971056, 279.6728254248552048, -1.556306295007354956 ) ) ;
#56828=CARTESIAN_POINT ( 'NONE',  ( 172.6426272267430022, 287.7740647968764733, -8.307796791299765005 ) ) ;
#56829=CARTESIAN_POINT ( 'NONE',  ( 155.0304386007204016, 262.1263989543018056, -17.12961552904782181 ) ) ;
#56830=CARTESIAN_POINT ( 'NONE',  ( 156.9852748171393273, 271.9751496516061025, -15.17404613224120880 ) ) ;
#56832=CARTESIAN_POINT ( 'NONE',  ( 130.3409059842875877, 239.3927522451417929, -10.00000000000009059 ) ) ;
#56835=CARTESIAN_POINT ( 'NONE',  ( 160.3242080723612730, 258.1019776236436201, -17.22713985970005979 ) ) ;
#56836=CARTESIAN_POINT ( 'NONE',  ( 4.289451341410245533, 161.0327760586659451, 1.948934522072302763E-15 ) ) ;
#56837=CARTESIAN_POINT ( 'NONE',  ( 43.17879721251643588, 204.9244531367911293, -4.594050593750046652 ) ) ;
#56842=CARTESIAN_POINT ( 'NONE',  ( 147.2443490232117256, 275.6123016948292275, 5.226063659459642352 ) ) ;
#56845=CARTESIAN_POINT ( 'NONE',  ( 65.31683191680592415, 208.5177522451418497, -10.00000000000009592 ) ) ;
#56846=CARTESIAN_POINT ( 'NONE',  ( 120.0388121219830282, 250.1115022471903160, -5.000000000000047962 ) ) ;
#56847=CARTESIAN_POINT ( 'NONE',  ( 163.1238134150576968, 256.2434428063396581, -15.10086001857528970 ) ) ;
#56848=CARTESIAN_POINT ( 'NONE',  ( 157.3198323354746435, 258.1610526871778006, -16.77630483474704093 ) ) ;
#56849=CARTESIAN_POINT ( 'NONE',  ( 154.2194984598485519, 265.5309884801890234, 17.12742652472672944 ) ) ;
#56850=CARTESIAN_POINT ( 'NONE',  ( 45.19978347827785825, 190.2365022471902023, 10.00000000000009592 ) ) ;
#56852=CARTESIAN_POINT ( 'NONE',  ( 164.4698008747318738, 245.7769439046653019, -6.272955660526681854 ) ) ;
#56853=CARTESIAN_POINT ( 'NONE',  ( 4.315907217689738395, 182.4869531367911293, 4.594050593750046652 ) ) ;
#56859=CARTESIAN_POINT ( 'NONE',  ( -22.42236680055709641, 157.8615022471902591, 0.000000000000000000 ) ) ;
#56860=CARTESIAN_POINT ( 'NONE',  ( 196.2379679265050925, 290.7528645076583871, -16.93678934971137906 ) ) ;
#56861=B_SPLINE_CURVE_WITH_KNOTS ( 'NONE', 3,
 ( #100217, #92632, #23181, #18101, #11518, #49003, #18608, #57080, #65681, #56587, #79937, #10006, #11017, #10496, #2412, #88059, #87575, #12005, #81435, #42863, #41888, #80444, #80952, #33815, #33290, #41380, #65192, #25708, #27706, #40869, #34294, #72320, #2925, #64192, #95142, #64702, #4389, #73797, #73307, #35287, #96637, #71815, #95653, #26200, #49487, #72827, #50481, #3420, #96138, #26696 ),
 .UNSPECIFIED., .F., .F.,
 ( 4, 2, 2, 2, 2, 2, 2, 2, 2, 2, 2, 2, 2, 2, 2, 2, 2, 2, 2, 2, 2, 2, 2, 2, 4 ),
 ( 0.001054687649897483601, 0.001531829325746945436, 0.002008971001596407489, 0.002247541839521137973, 0.002486112677445868890, 0.002605398096408233916, 0.002724683515370599808, 0.002843968934332965267, 0.002963254353295330726, 0.003440396029144835929, 0.003917537704994342000, 0.004871821056693417459, 0.005826104408392492919, 0.006303246084241995520, 0.006780387760091497254, 0.006899673179053816309, 0.006959315888535009230, 0.007018958598016202151, 0.007138244016978573248, 0.007257529435940943477, 0.007496100273865653578, 0.007734671111790362812, 0.007973241949715072913, 0.008211812787639783881, 0.008688954463489200614 ),
 .UNSPECIFIED. ) ;
#56862=CARTESIAN_POINT ( 'NONE',  ( 150.0694502760089222, 271.4680435213315945, -12.17790201236558545 ) ) ;
#56866=CARTESIAN_POINT ( 'NONE',  ( 168.8436447018356716, 287.8931087461074299, 0.5168480269480507650 ) ) ;
#56868=CARTESIAN_POINT ( 'NONE',  ( 160.6031540345039446, 252.4741726868657281, 15.87852846076284763 ) ) ;
#56869=CARTESIAN_POINT ( 'NONE',  ( 153.2185337766395890, 277.6703050030072291, -5.188401963753405788 ) ) ;
#56871=CARTESIAN_POINT ( 'NONE',  ( 159.6288139302610887, 254.1617792512662675, -15.32287760493869477 ) ) ;
#56872=VERTEX_POINT ( 'NONE', #47697 ) ;
#56873=CARTESIAN_POINT ( 'NONE',  ( 152.4293375737637177, 267.0122523221186839, 15.45871950931433325 ) ) ;
#56874=CARTESIAN_POINT ( 'NONE',  ( 164.5867587387928950, 245.5743669417666126, -3.022048486790635202 ) ) ;
#56875=CARTESIAN_POINT ( 'NONE',  ( 104.9037214839949002, 219.8262482093457777, 3.021315404115420679E-15 ) ) ;
#56878=CARTESIAN_POINT ( 'NONE',  ( 193.9966098916996771, 294.6350105018939871, 13.97117019253516013 ) ) ;
#56886=ORIENTED_EDGE ( 'NONE', *, *, #29398, .T. ) ;
#56891=CARTESIAN_POINT ( 'NONE',  ( 173.7270898585821612, 267.2108298537337987, 16.98825523054146558 ) ) ;
#56892=CARTESIAN_POINT ( 'NONE',  ( 169.3652806017343835, 276.2350476629839591, -15.58549988110435258 ) ) ;
#56895=ORIENTED_EDGE ( 'NONE', *, *, #75807, .F. ) ;
#56897=CARTESIAN_POINT ( 'NONE',  ( 163.2835940097493790, 247.8315144631017404, 11.08416305054517359 ) ) ;
#56900=CARTESIAN_POINT ( 'NONE',  ( 157.8523751997425109, 267.2426576861807916, -16.20207976436619646 ) ) ;
#56901=ORIENTED_EDGE ( 'NONE', *, *, #57496, .T. ) ;
#56905=CARTESIAN_POINT ( 'NONE',  ( 193.5379746301957198, 295.4293900769612833, 13.37282311005296620 ) ) ;
#56906=CARTESIAN_POINT ( 'NONE',  ( 177.3353965951741316, 288.8196383795363431, -9.382684147788728168 ) ) ;
#56908=CARTESIAN_POINT ( 'NONE',  ( 192.0963028965829551, 297.9264387674147656, 11.34530024772836754 ) ) ;
#56909=CARTESIAN_POINT ( 'NONE',  ( 175.3742949935872844, 291.1603597146743141, 6.550094823951227774 ) ) ;
#56910=CARTESIAN_POINT ( 'NONE',  ( 192.9476382485522947, 262.0161990052710621, 3.467033003238014999 ) ) ;
#56911=ORIENTED_EDGE ( 'NONE', *, *, #29335, .T. ) ;
#56914=CARTESIAN_POINT ( 'NONE',  ( 206.2456893945931142, 273.4189824569319285, 10.13882547285618152 ) ) ;
#56915=CARTESIAN_POINT ( 'NONE',  ( 196.6317700900902139, 290.0707791521982131, -17.91116578096951883 ) ) ;
#56916=CARTESIAN_POINT ( 'NONE',  ( 206.0041637419966776, 273.8373171585603814, 11.66586596407113596 ) ) ;
#56917=CARTESIAN_POINT ( 'NONE',  ( 159.5204760365350012, 254.3494259875849082, 16.90107507090185379 ) ) ;
#56918=ORIENTED_EDGE ( 'NONE', *, *, #14892, .F. ) ;
#56919=CARTESIAN_POINT ( 'NONE',  ( 187.6303425324672958, 277.1110116237759939, 17.31978431366381699 ) ) ;
#56920=CARTESIAN_POINT ( 'NONE',  ( 171.2828659525146975, 259.2707523077851874, -13.88512410246953088 ) ) ;
#56924=B_SPLINE_CURVE_WITH_KNOTS ( 'NONE', 3,
 ( #19680, #57142, #35851, #51038 ),
 .UNSPECIFIED., .F., .F.,
 ( 4, 4 ),
 ( 0.04746404433603530065, 0.04887066958154934887 ),
 .UNSPECIFIED. ) ;
#56925=CARTESIAN_POINT ( 'NONE',  ( 199.3485334918771628, 285.3652069081594504, -18.27963836619689175 ) ) ;
#56927=CARTESIAN_POINT ( 'NONE',  ( 190.7990164375790130, 261.9893415206284430, -0.6577425147695087349 ) ) ;
#56929=CARTESIAN_POINT ( 'NONE',  ( 158.7247586461176354, 260.9712587547172689, -17.77758391712495012 ) ) ;
#56931=EDGE_CURVE ( 'NONE', #74125, #35225, #26802, .T. ) ;
#56932=CARTESIAN_POINT ( 'NONE',  ( -10.43439047959891397, 176.3297689869269220, -2.679491924311252493 ) ) ;
#56934=CARTESIAN_POINT ( 'NONE',  ( 18.47929132879760417, 168.1427522451417644, 1.119607411625061291E-15 ) ) ;
#56935=CARTESIAN_POINT ( 'NONE',  ( 101.4736528484039724, 220.2048013555409796, 4.594050593750051981 ) ) ;
#56937=B_SPLINE_CURVE_WITH_KNOTS ( 'NONE', 3,
 ( #34746, #12978, #74777, #67144, #21076, #27167, #51952, #66156, #82892, #96101, #26660, #96604, #58055, #19585, #50449, #11969, #97103, #75763, #60518, #23513, #38723, #54406, #30134, #90991, #83887, #92472 ),
 .UNSPECIFIED., .F., .F.,
 ( 4, 2, 2, 2, 2, 2, 2, 2, 2, 2, 2, 2, 4 ),
 ( 0.0002293139140671511035, 0.0008647663282778704844, 0.001182492535383264680, 0.001341355638935961669, 0.001420787190712275360, 0.001460502966600432315, 0.001500218742488589052, 0.001579650294264903177, 0.001659081846041217520, 0.001817944949593846421, 0.002135671156699089478, 0.002453397363804332536, 0.002771123570909575593 ),
 .UNSPECIFIED. ) ;
#56939=CARTESIAN_POINT ( 'NONE',  ( 162.7896496350696225, 248.6870512161599436, 11.81710663537990946 ) ) ;
#56940=CARTESIAN_POINT ( 'NONE',  ( 25.61497981383703149, 185.5958772461660544, -9.188101187500095079 ) ) ;
#56945=CARTESIAN_POINT ( 'NONE',  ( 187.4166251561426293, 263.4339899954952102, 11.64397722261905166 ) ) ;
#56948=CARTESIAN_POINT ( 'NONE',  ( 207.2707369601997982, 271.6435479931266173, -5.381413637561199614 ) ) ;
#56951=CARTESIAN_POINT ( 'NONE',  ( 42.55642822748762910, 201.5024278399160949, 9.188101187500095079 ) ) ;
#56952=CARTESIAN_POINT ( 'NONE',  ( 80.03926378114135787, 227.0177522451419350, 5.000000000000046185 ) ) ;
#56955=DIRECTION ( 'NONE',  ( -0.8660254037844387076, -0.4999999999999998890, -0.000000000000000000 ) ) ;
#56956=CARTESIAN_POINT ( 'NONE',  ( 3.856091543753019213, 173.0333772461660828, 9.188101187500095079 ) ) ;
#56958=CARTESIAN_POINT ( 'NONE',  ( 151.0388915836658725, 269.0399611886400635, -14.24896787280406585 ) ) ;
#56959=CARTESIAN_POINT ( 'NONE',  ( 186.3242389376556787, 283.0587387869642839, 16.24190855881933260 ) ) ;
#56960=CARTESIAN_POINT ( 'NONE',  ( 192.6247335881259630, 297.0111699613833594, -13.30158778996737290 ) ) ;
#56961=APPLICATION_CONTEXT ( 'automotive_design' ) ;
#56962=CARTESIAN_POINT ( 'NONE',  ( 166.5418805794664934, 264.7512503615053561, 17.71810435351582669 ) ) ;
#56963=CARTESIAN_POINT ( 'NONE',  ( 164.2297246530060875, 246.1927681183832988, 5.803160395959773510 ) ) ;
#56964=CARTESIAN_POINT ( 'NONE',  ( 191.0702043019150835, 299.7036936669546776, -8.800021049343948576 ) ) ;
#56965=CARTESIAN_POINT ( 'NONE',  ( 189.8147415777049218, 301.8782188922952514, -0.5019643756309712934 ) ) ;
#56968=CARTESIAN_POINT ( 'NONE',  ( 1.754175721758543638, 158.4865022471901739, 1.119607411625061291E-15 ) ) ;
#56970=CARTESIAN_POINT ( 'NONE',  ( 126.3172359758225554, 252.9244531367911293, -4.594050593750046652 ) ) ;
#56974=CARTESIAN_POINT ( 'NONE',  ( 157.2464636617698375, 258.2881309577184652, 18.14284729738657731 ) ) ;
#56975=CARTESIAN_POINT ( 'NONE',  ( 185.8594361394618204, 288.5116224014759041, 15.32760917146029200 ) ) ;
#56976=CARTESIAN_POINT ( 'NONE',  ( 150.2557873729419669, 270.3963374692353341, -14.33267926939609005 ) ) ;
#56977=VERTEX_POINT ( 'NONE', #3632 ) ;
#56978=CARTESIAN_POINT ( 'NONE',  ( 189.6617571741743689, 261.1287600027826556, -4.536318394431146928 ) ) ;
#56979=CARTESIAN_POINT ( 'NONE',  ( 149.6191398986701415, 271.4990432411842676, -11.66821883946526839 ) ) ;
#56984=EDGE_LOOP ( 'NONE', ( #51913, #54362, #74849, #21571, #26996, #87856, #21177, #26109, #100288, #61769, #14274, #92853, #27887, #87648, #67709, #50932, #13347, #1875, #13683, #8963, #18796, #17836 ) ) ;
#56985=CARTESIAN_POINT ( 'NONE',  ( 189.0176971330334368, 265.7359912712865366, 10.99843924538786233 ) ) ;
#56987=CARTESIAN_POINT ( 'NONE',  ( 195.2495212664957194, 275.1290853193528392, -16.26662379558266380 ) ) ;
#56988=CARTESIAN_POINT ( 'NONE',  ( 165.6504798027754646, 269.1482514364597591, -16.93297765974685021 ) ) ;
#56990=B_SPLINE_SURFACE_WITH_KNOTS ( 'NONE', 3, 1, ( 
 ( #85105, #55642 ),
 ( #39943, #100287 ),
 ( #48061, #69861 ),
 ( #87146, #76962 ),
 ( #473, #93199 ),
 ( #31852, #15654 ),
 ( #30872, #71389 ),
 ( #85625, #86628 ),
 ( #94703, #31362 ),
 ( #55150, #94209 ),
 ( #61756, #77982 ),
 ( #62246, #23753 ),
 ( #16170, #92705 ),
 ( #47067, #973 ),
 ( #70879, #17162 ),
 ( #86136, #9075 ),
 ( #23256, #70363 ),
 ( #8577, #93710 ),
 ( #38454, #39442 ),
 ( #62753, #69367 ),
 ( #1978, #63268 ),
 ( #16665, #47560 ),
 ( #78487, #24763 ),
 ( #79003, #9590 ),
 ( #32864, #63770 ),
 ( #25265, #56148 ),
 ( #17677, #90980 ),
 ( #25788, #12965 ),
 ( #98560, #12457 ),
 ( #36722, #98051 ),
 ( #89500, #74766 ),
 ( #44321, #49078 ),
 ( #43328, #43826 ),
 ( #87649, #97089 ) ),
 .UNSPECIFIED., .T., .F., .F.,
 ( 4, 2, 2, 2, 2, 2, 2, 2, 2, 2, 2, 2, 2, 2, 2, 2, 4 ),
 ( 2, 2 ),
 ( 0.000000000000000000, 0.06250000000000000000, 0.1250000000000000000, 0.1875000000000000000, 0.2500000000000000000, 0.3125000000000000000, 0.3750000000000000000, 0.4375000000000000000, 0.5000000000000000000, 0.5625000000000000000, 0.6250000000000000000, 0.6875000000000000000, 0.7500000000000000000, 0.8125000000000000000, 0.8750000000000000000, 0.9375000000000000000, 1.000000000000000000 ),
 ( 0.000000000000000000, 1.000000000000000000 ),
 .UNSPECIFIED. ) ;
#56991=CARTESIAN_POINT ( 'NONE',  ( 197.9494925845387456, 271.7022998954425361, 12.11704210009641969 ) ) ;
#56992=CARTESIAN_POINT ( 'NONE',  ( 155.8168635700358493, 261.2859049548226267, 17.07611989262474239 ) ) ;
#56994=CARTESIAN_POINT ( 'NONE',  ( 192.6797324865049745, 296.9159090750308110, 12.42053959885222625 ) ) ;
#56996=CARTESIAN_POINT ( 'NONE',  ( 190.5716289146250517, 280.7215959158480132, 16.63595715464797564 ) ) ;
#56999=ORIENTED_EDGE ( 'NONE', *, *, #64382, .T. ) ;
#57000=CARTESIAN_POINT ( 'NONE',  ( 164.6784601142441318, 280.3721143660208099, 12.61989482521711636 ) ) ;
#57002=CARTESIAN_POINT ( 'NONE',  ( 147.8308140999695866, 274.5965143850199865, -7.866624397492971710 ) ) ;
#57004=B_SPLINE_CURVE_WITH_KNOTS ( 'NONE', 3,
 ( #54666, #78002, #16687, #38974 ),
 .UNSPECIFIED., .F., .F.,
 ( 4, 4 ),
 ( 0.001918581007240343240, 0.009849387959984160987 ),
 .UNSPECIFIED. ) ;
#57007=CARTESIAN_POINT ( 'NONE',  ( 159.7080606971873920, 255.4347751002972871, 16.25053020610463861 ) ) ;
#57008=CARTESIAN_POINT ( 'NONE',  ( 151.0036289208911171, 269.1010379121764799, 14.24595189915657478 ) ) ;
#57012=CARTESIAN_POINT ( 'NONE',  ( 189.5797355942488025, 300.2297304461512795, 3.265020536630226733 ) ) ;
#57013=CARTESIAN_POINT ( 'NONE',  ( 155.5066938333533528, 261.3015006940112244, -18.40036130547566273 ) ) ;
#57015=ORIENTED_EDGE ( 'NONE', *, *, #87504, .T. ) ;
#57016=CARTESIAN_POINT ( 'NONE',  ( 179.0589298886251868, 259.9615930511803867, 12.73898565628910085 ) ) ;
#57019=ORIENTED_EDGE ( 'NONE', *, *, #95739, .T. ) ;
#57022=EDGE_LOOP ( 'NONE', ( #5767, #71127, #11825, #22153 ) ) ;
#57024=CARTESIAN_POINT ( 'NONE',  ( 151.3198218389669023, 269.0401608486226337, 14.23401639979100430 ) ) ;
#57025=CARTESIAN_POINT ( 'NONE',  ( 158.6150988756866127, 274.9578748594535682, -12.59651497174430013 ) ) ;
#57026=CARTESIAN_POINT ( 'NONE',  ( 193.1444937042664094, 296.1109190324805240, -12.15243020627156767 ) ) ;
#57027=CARTESIAN_POINT ( 'NONE',  ( 153.4495116231415750, 264.8646448025247082, -16.73555355292144498 ) ) ;
#57029=CARTESIAN_POINT ( 'NONE',  ( 202.0032530003042552, 275.2598398602717680, -14.36878956143956643 ) ) ;
#57030=CARTESIAN_POINT ( 'NONE',  ( 138.3604885211411499, 256.8149278399160949, 9.188101187500093303 ) ) ;
#57035=VERTEX_POINT ( 'NONE', #88276 ) ;
#57038=CARTESIAN_POINT ( 'NONE',  ( 162.8996025780091941, 248.4966071325470125, 11.23567065566008516 ) ) ;
#57041=CARTESIAN_POINT ( 'NONE',  ( 153.2891369107873345, 276.9440725079709296, 6.996015511654989361 ) ) ;
#57042=CARTESIAN_POINT ( 'NONE',  ( 200.6985908945154335, 283.0268388936558495, -17.74173253065502820 ) ) ;
#57044=B_SPLINE_CURVE_WITH_KNOTS ( 'NONE', 3,
 ( #27594, #80838, #59949, #58458, #81815, #97984, #73195, #57972, #43754, #5278, #28562, #88956, #19511, #20997, #81322, #90920, #11894, #35670, #13384, #51878, #42751, #73685 ),
 .UNSPECIFIED., .F., .F.,
 ( 4, 2, 2, 2, 2, 2, 2, 2, 2, 2, 4 ),
 ( 0.0002052773884520107852, 0.0006292189728194242651, 0.0007352043689112620429, 0.0007881970669571040618, 0.0008146934159800252881, 0.0008411897650029466229, 0.0008941824630486570197, 0.0009471751610943675249, 0.001053160557185625797, 0.001477102141550394989, 0.001901043725915164398 ),
 .UNSPECIFIED. ) ;
#57045=CARTESIAN_POINT ( 'NONE',  ( 171.5253789402676716, 280.0391282839272549, 13.83596625797474644 ) ) ;
#57048=EDGE_LOOP ( 'NONE', ( #44769, #22478, #28536, #56405, #56280 ) ) ;
#57052=CARTESIAN_POINT ( 'NONE',  ( 162.8901731922526039, 277.0746486824075419, 12.89396308544769276 ) ) ;
#57053=EDGE_CURVE ( 'NONE', #42536, #73611, #61014, .T. ) ;
#57054=CARTESIAN_POINT ( 'NONE',  ( 200.9393373695271805, 267.7870988455974270, -2.797138418476491584 ) ) ;
#57055=CARTESIAN_POINT ( 'NONE',  ( 151.7482317558875593, 267.8113479705027657, -16.53675092648768086 ) ) ;
#57056=CARTESIAN_POINT ( 'NONE',  ( 190.1190668544949460, 301.3511120508678118, 4.410340539513557090 ) ) ;
#57057=CARTESIAN_POINT ( 'NONE',  ( 202.6551236945213361, 279.6380246773706517, 15.55476940527561425 ) ) ;
#57058=CARTESIAN_POINT ( 'NONE',  ( 161.4341193711443054, 281.4014545508878768, -6.923656337983120856 ) ) ;
#57060=CIRCLE ( 'NONE', #34368, 10.00000000000011369 ) ;
#57069=FACE_OUTER_BOUND ( 'NONE', #9313, .T. ) ;
#57070=CARTESIAN_POINT ( 'NONE',  ( 162.8042930031641049, 248.6616881586264469, 11.14389129512055554 ) ) ;
#57071=CARTESIAN_POINT ( 'NONE',  ( -3.180017766230537557, 156.7202760586659451, -5.415160957724236172E-17 ) ) ;
#57072=CARTESIAN_POINT ( 'NONE',  ( 109.7008941843561445, 224.9548013555409796, -4.594050593750042211 ) ) ;
#57073=CARTESIAN_POINT ( 'NONE',  ( 155.0304386007204016, 262.1263989543018056, -17.12961552904782181 ) ) ;
#57075=CARTESIAN_POINT ( 'NONE',  ( 185.9470091674525349, 276.4697974381609242, -17.76503501984419131 ) ) ;
#57077=AXIS2_PLACEMENT_3D ( 'NONE', #66821, #67831, #82583 ) ;
#57078=CARTESIAN_POINT ( 'NONE',  ( 194.3413770922408617, 282.8930799310762723, 17.82077676852630077 ) ) ;
#57080=CARTESIAN_POINT ( 'NONE',  ( 163.9292450293648074, 284.3952669320320865, 5.923242389932828367 ) ) ;
#57081=DIRECTION ( 'NONE',  ( -0.8660254037844387076, -0.4999999999999998890, -0.000000000000000000 ) ) ;
#57082=CARTESIAN_POINT ( 'NONE',  ( 208.2874212803407090, 269.8825990953837390, -1.143705256421198690 ) ) ;
#57083=CARTESIAN_POINT ( 'NONE',  ( 162.0042060562265931, 250.0474794011949768, 13.08583584746748940 ) ) ;
#57088=CARTESIAN_POINT ( 'NONE',  ( 52.43496435911014686, 191.8923013555410080, 4.594050593750050204 ) ) ;
#57089=CARTESIAN_POINT ( 'NONE',  ( -22.42236680055709641, 157.8615022471902591, 0.000000000000000000 ) ) ;
#57090=CARTESIAN_POINT ( 'NONE',  ( 83.63833477162944519, 231.3464784336661637, 1.353441290958777327E-15 ) ) ;
#57091=CARTESIAN_POINT ( 'NONE',  ( 161.5083988044524119, 250.9062427520286178, -14.53522982831775856 ) ) ;
#57092=CARTESIAN_POINT ( 'NONE',  ( 163.2699323312932904, 258.1949546823035462, 15.87757944056416015 ) ) ;
#57095=CARTESIAN_POINT ( 'NONE',  ( 173.5451919912859182, 268.4384502063331297, -16.29429379470302308 ) ) ;
#57099=ORIENTED_EDGE ( 'NONE', *, *, #65428, .T. ) ;
#57101=CARTESIAN_POINT ( 'NONE',  ( 84.82981389336303835, 207.5327760586659451, 1.948934522072302763E-15 ) ) ;
#57102=CARTESIAN_POINT ( 'NONE',  ( 88.52455635939595879, 233.4637435831425023, 2.679491924311251605 ) ) ;
#57103=CYLINDRICAL_SURFACE ( 'NONE', #53927, 17.82106496071139645 ) ;
#57104=CARTESIAN_POINT ( 'NONE',  ( 147.1603453755519695, 275.7578002805973370, -5.230822882238410187 ) ) ;
#57105=CARTESIAN_POINT ( 'NONE',  ( 199.7408883951190717, 281.7026737086815160, 17.40441678530665470 ) ) ;
#57107=B_SPLINE_CURVE_WITH_KNOTS ( 'NONE', 3,
 ( #2762, #18454, #34628, #4745, #18957, #33653, #66034, #57927, #96981, #26549, #26050, #80282, #35629, #72670, #10848, #27550, #43209, #80793 ),
 .UNSPECIFIED., .F., .F.,
 ( 4, 2, 2, 2, 2, 2, 2, 2, 4 ),
 ( 0.000000000000000000, 0.0003250734011923252882, 0.0006501468023846505764, 0.0009752202035769758645, 0.001300293604769301153, 0.001625367005961621562, 0.001950440407153941971, 0.002275513808346262164, 0.002600587209538582790 ),
 .UNSPECIFIED. ) ;
#57109=CARTESIAN_POINT ( 'NONE',  ( 193.6538297768585153, 294.3106073703939387, 13.99927879369582406 ) ) ;
#57110=CARTESIAN_POINT ( 'NONE',  ( 191.2104420009116836, 280.2857515794617598, 17.80337293751487593 ) ) ;
#57111=CARTESIAN_POINT ( 'NONE',  ( 121.4100190113084636, 234.2365022471901739, -10.00000000000009059 ) ) ;
#57112=CARTESIAN_POINT ( 'NONE',  ( 205.0716081116550527, 275.4525508911965517, -12.57761053684872188 ) ) ;
#57114=CARTESIAN_POINT ( 'NONE',  ( 165.6167443952357416, 246.9696370225337603, -1.864274362100295734 ) ) ;
#57116=CARTESIAN_POINT ( 'NONE',  ( 163.0171530587457767, 248.2930037274571191, 9.677214176418313940 ) ) ;
#57117=CARTESIAN_POINT ( 'NONE',  ( 178.0315741628076012, 287.5935043698759728, -13.06113257055532451 ) ) ;
#57122=CARTESIAN_POINT ( 'NONE',  ( 189.6918891073893008, 290.1382577116506241, 14.45894197730551589 ) ) ;
#57123=CARTESIAN_POINT ( 'NONE',  ( 172.7264208856190919, 290.8582626858774347, 2.771863430787652849 ) ) ;
#57124=CARTESIAN_POINT ( 'NONE',  ( 158.1337577521140929, 257.6225849586518279, -16.81478466335610022 ) ) ;
#57125=CARTESIAN_POINT ( 'NONE',  ( 201.4617167010348737, 281.7050662241970826, -17.43131506460443703 ) ) ;
#57132=CARTESIAN_POINT ( 'NONE',  ( 156.2224770818481545, 267.4677849582849376, -16.91854127892884208 ) ) ;
#57135=ORIENTED_EDGE ( 'NONE', *, *, #44414, .F. ) ;
#57137=CARTESIAN_POINT ( 'NONE',  ( 198.1847055346428590, 286.9842163890704683, 16.95145238430053070 ) ) ;
#57138=CARTESIAN_POINT ( 'NONE',  ( 204.3951397407346064, 276.6242284793436852, 14.79595971842109137 ) ) ;
#57139=CARTESIAN_POINT ( 'NONE',  ( 148.1004780136491377, 274.1294427855589788, -7.811560775291159331 ) ) ;
#57141=CARTESIAN_POINT ( 'NONE',  ( 193.7999837595647250, 294.9755769528473479, 15.24609078262870199 ) ) ;
#57142=CARTESIAN_POINT ( 'NONE',  ( 153.2685960449373681, 269.0240501674685447, -15.70450447371167790 ) ) ;
#57143=CARTESIAN_POINT ( 'NONE',  ( 204.9463377925012253, 275.6695254486514841, -14.15865086131798378 ) ) ;
#57144=CARTESIAN_POINT ( 'NONE',  ( 164.6993295494617939, 245.3793885782390589, 4.576454266300281404 ) ) ;
#57145=CARTESIAN_POINT ( 'NONE',  ( 166.1014715941954591, 265.5448861341674274, 16.58231607936238916 ) ) ;
#57148=CARTESIAN_POINT ( 'NONE',  ( 81.20281187136818346, 223.8149278399160664, 9.188101187500093303 ) ) ;
#57151=ORIENTED_EDGE ( 'NONE', *, *, #25902, .T. ) ;
#57157=CARTESIAN_POINT ( 'NONE',  ( 164.1377787084186934, 249.9599717614572114, 10.21025470079037056 ) ) ;
#57158=CARTESIAN_POINT ( 'NONE',  ( 206.8659638600981623, 272.3446355680395641, -10.26115277030573125 ) ) ;
#57159=CARTESIAN_POINT ( 'NONE',  ( 207.0601855587586329, 271.2283032176189295, -4.679519923957272454 ) ) ;
#57160=CARTESIAN_POINT ( 'NONE',  ( 97.65764163903753570, 221.0643266524160424, 9.188101187500095079 ) ) ;
#57162=EDGE_CURVE ( 'NONE', #41308, #61729, #51392, .T. ) ;
#57166=EDGE_CURVE ( 'NONE', #98884, #76355, #47583, .T. ) ;
#57170=CARTESIAN_POINT ( 'NONE',  ( 136.3040252829181327, 243.3768266524159856, 9.188101187500098632 ) ) ;
#57172=CARTESIAN_POINT ( 'NONE',  ( -1.367124174595798713, 160.0177522451418213, 5.000000000000051514 ) ) ;
#57175=CARTESIAN_POINT ( 'NONE',  ( 157.0858749576330524, 258.5662787524049122, 18.43576942457294976 ) ) ;
#57177=CARTESIAN_POINT ( 'NONE',  ( 160.4962995477943650, 275.9333967852908813, 14.18032076246626794 ) ) ;
#57178=FACE_OUTER_BOUND ( 'NONE', #98167, .T. ) ;
#57181=CARTESIAN_POINT ( 'NONE',  ( 174.5944895219865316, 283.7845549098777838, 13.67518389082495034 ) ) ;
#57185=CARTESIAN_POINT ( 'NONE',  ( 161.1990332043106946, 251.4420796895884394, 14.26998817770995487 ) ) ;
#57189=CARTESIAN_POINT ( 'NONE',  ( 175.9704269209120753, 290.3320350542924757, -6.214979091763118468 ) ) ;
#57190=CARTESIAN_POINT ( 'NONE',  ( 195.8285188278500470, 273.2427770020486832, 15.26130794574777383 ) ) ;
#57194=CARTESIAN_POINT ( 'NONE',  ( 180.7942833579522812, 266.7097690628117448, -16.23795806611159520 ) ) ;
#57196=CARTESIAN_POINT ( 'NONE',  ( 74.41009865654255862, 213.7677522451418497, 10.00000000000009592 ) ) ;
#57198=CARTESIAN_POINT ( 'NONE',  ( 152.7314557461996571, 266.1083540640618708, 17.39314074348802208 ) ) ;
#57199=CARTESIAN_POINT ( 'NONE',  ( 155.3250150347760723, 261.6161776038049425, -18.57420904020362684 ) ) ;
#57201=CARTESIAN_POINT ( 'NONE',  ( 160.8072101477444846, 273.0293901340574507, -14.97921187206499027 ) ) ;
#57204=CARTESIAN_POINT ( 'NONE',  ( 8.781437479894508513, 182.0024278399160949, 9.188101187500095079 ) ) ;
#57208=AXIS2_PLACEMENT_3D ( 'NONE', #86360, #62472, #16890 ) ;
#57210=CARTESIAN_POINT ( 'NONE',  ( 37.46976539259314620, 180.8932355074535678, -2.679491924311248496 ) ) ;
#57212=CARTESIAN_POINT ( 'NONE',  ( 41.04123086662985997, 188.3768266524159856, -9.188101187500093303 ) ) ;
#57215=CARTESIAN_POINT ( 'NONE',  ( 190.9498149295421570, 299.9122141765958531, -5.138500224925297566 ) ) ;
#57218=CARTESIAN_POINT ( 'NONE',  ( 191.5324528500417216, 298.9030556958743432, -8.286652526617016790 ) ) ;
#57220=CARTESIAN_POINT ( 'NONE',  ( 182.5821340850675938, 280.3201940986122054, -16.08842446693554606 ) ) ;
#57222=B_SPLINE_SURFACE_WITH_KNOTS ( 'NONE', 3, 1, ( 
 ( #23703, #31313 ),
 ( #7511, #75957 ),
 ( #62202, #29824 ),
 ( #77937, #23210 ),
 ( #76442, #61707 ),
 ( #30325, #7017 ),
 ( #39397, #54598 ),
 ( #37902, #61213 ),
 ( #92179, #53608 ),
 ( #85581, #70314 ),
 ( #16124, #927 ),
 ( #15105, #72852 ),
 ( #17114, #48012 ),
 ( #88088, #18637 ),
 ( #55107, #10034 ),
 ( #78955, #24715 ),
 ( #87603, #25740 ),
 ( #56102, #1439 ),
 ( #3444, #70829 ),
 ( #56619, #40404 ),
 ( #87093, #71341 ),
 ( #32819, #17630 ),
 ( #72352, #86581 ),
 ( #63220, #94162 ),
 ( #32319, #18129 ),
 ( #49030, #78441 ),
 ( #2956, #48533 ),
 ( #79964, #80471 ),
 ( #10532, #9022 ),
 ( #55598, #9544 ),
 ( #1933, #2443 ),
 ( #49516, #95171 ),
 ( #63724, #33321 ),
 ( #94661, #25217 ) ),
 .UNSPECIFIED., .T., .F., .F.,
 ( 4, 2, 2, 2, 2, 2, 2, 2, 2, 2, 2, 2, 2, 2, 2, 2, 4 ),
 ( 2, 2 ),
 ( 0.000000000000000000, 0.06250000000000000000, 0.1250000000000000000, 0.1875000000000000000, 0.2500000000000000000, 0.3125000000000000000, 0.3750000000000000000, 0.4375000000000000000, 0.5000000000000000000, 0.5625000000000000000, 0.6250000000000000000, 0.6875000000000000000, 0.7500000000000000000, 0.8125000000000000000, 0.8750000000000000000, 0.9375000000000000000, 1.000000000000000000 ),
 ( 0.000000000000000000, 1.000000000000000000 ),
 .UNSPECIFIED. ) ;
#57223=CARTESIAN_POINT ( 'NONE',  ( 107.7317227740038987, 244.5530062829863311, -4.648177544792955347E-16 ) ) ;
#57224=CARTESIAN_POINT ( 'NONE',  ( 83.21237853290490705, 230.3967562850347122, -4.648177544792955347E-16 ) ) ;
#57225=CARTESIAN_POINT ( 'NONE',  ( 84.89261448506459828, 226.4865022471902876, -10.00000000000009415 ) ) ;
#57228=CARTESIAN_POINT ( 'NONE',  ( 45.37135788555205096, 190.8768266524159856, 9.188101187500098632 ) ) ;
#57232=CARTESIAN_POINT ( 'NONE',  ( 198.4522155198218059, 286.9176751754968109, -17.57438352224490075 ) ) ;
#57233=EDGE_CURVE ( 'NONE', #24654, #67131, #59813, .T. ) ;
#57235=EDGE_LOOP ( 'NONE', ( #1486, #3778, #56918, #376 ) ) ;
#57236=CARTESIAN_POINT ( 'NONE',  ( 167.4242128886634760, 285.3674954085350919, 7.916955735753099077 ) ) ;
#57237=CARTESIAN_POINT ( 'NONE',  ( 206.9676408587583296, 272.1685258403992975, 7.544050792475608169 ) ) ;
#57241=CARTESIAN_POINT ( 'NONE',  ( 151.1044726995390306, 278.3667167227523009, 2.833052190833913464 ) ) ;
#57242=CARTESIAN_POINT ( 'NONE',  ( 171.5228814212670159, 255.7221739033098800, 11.23420559966320553 ) ) ;
#57246=CARTESIAN_POINT ( 'NONE',  ( 171.6147572926790303, 252.5492226098082824, 8.631356844989948485 ) ) ;
#57251=CARTESIAN_POINT ( 'NONE',  ( 166.8885992513889960, 261.3854899355708881, 16.67823075215012452 ) ) ;
#57252=ADVANCED_FACE ( 'NONE', ( #6489 ), #74417, .T. ) ;
#57253=CARTESIAN_POINT ( 'NONE',  ( 177.9925615710933755, 254.8251403409008731, -7.350624415798725053 ) ) ;
#57257=CARTESIAN_POINT ( 'NONE',  ( 207.7320178805681508, 270.8445860024863237, -5.379955943374661764 ) ) ;
#57258=DIRECTION ( 'NONE',  ( -0.8660254037844387076, -0.4999999999999998890, -0.000000000000000000 ) ) ;
#57259=CARTESIAN_POINT ( 'NONE',  ( 196.2630260332681189, 290.7094625936034049, -17.43112004684450866 ) ) ;
#57262=CARTESIAN_POINT ( 'NONE',  ( 173.4586948132588873, 285.6886373276996096, -12.44553698290859600 ) ) ;
#57265=CARTESIAN_POINT ( 'NONE',  ( 157.4893260420801653, 257.8674809757739013, -18.30842125257398223 ) ) ;
#57266=B_SPLINE_CURVE_WITH_KNOTS ( 'NONE', 3,
 ( #32092, #9830, #16897, #70093, #94443, #64005, #2730, #704, #63005, #71126, #55875, #86871, #17404, #33617, #79259, #40691, #71631, #2226, #64513, #94945, #87877, #73614, #43688, #5202, #66985, #74121, #58389, #72637 ),
 .UNSPECIFIED., .F., .F.,
 ( 4, 2, 2, 2, 2, 2, 2, 2, 2, 2, 2, 2, 2, 4 ),
 ( 0.0004012327469206063211, 0.001481470891302587214, 0.002561709035684567835, 0.003101828107875521066, 0.003236857875923203863, 0.003304372759947044828, 0.003338130201959010630, 0.003371887643970976865, 0.003439402527995009083, 0.003506917412019041301, 0.003641947180067237576, 0.004182066252259748589, 0.004452125788356024912, 0.004722185324452301235 ),
 .UNSPECIFIED. ) ;
#57267=CARTESIAN_POINT ( 'NONE',  ( 120.7695210546522446, 240.5333772461660544, 9.188101187500095079 ) ) ;
#57269=FACE_OUTER_BOUND ( 'NONE', #81858, .T. ) ;
#57270=EDGE_LOOP ( 'NONE', ( #13584, #27840, #48956, #21000 ) ) ;
#57271=CARTESIAN_POINT ( 'NONE',  ( 164.3053959849042087, 246.0617015268593661, -7.251939739328854273 ) ) ;
#57276=CARTESIAN_POINT ( 'NONE',  ( 71.75763553740291911, 221.4244531367911293, -4.594050593750046652 ) ) ;
#57278=( BOUNDED_CURVE ( )  B_SPLINE_CURVE ( 2, ( #1041, #16732, #78048, #1553, #23321, #32927, #54209, #23822, #71951 ),
 .UNSPECIFIED., .F., .T. ) 
 B_SPLINE_CURVE_WITH_KNOTS ( ( 3, 2, 2, 2, 3 ),
 ( 0.1411290322580645296, 0.1424731182795699047, 0.1451612903225806550, 0.1478494623655914053, 0.1491935483870967805 ),
 .UNSPECIFIED. ) 
 CURVE ( )  GEOMETRIC_REPRESENTATION_ITEM ( )  RATIONAL_B_SPLINE_CURVE ( ( 0.9330127018922194093, 0.9330127018922200755, 1.000000000000000000, 0.8660254037844387076, 1.000000000000000000, 0.8660254037844387076, 1.000000000000000000, 0.9330127018922194093, 0.9330127018922194093 ) ) 
 REPRESENTATION_ITEM ( '' )  );
#57279=CARTESIAN_POINT ( 'NONE',  ( 151.4281781455628675, 268.3656970847310390, 15.24742929158552585 ) ) ;
#57280=CARTESIAN_POINT ( 'NONE',  ( 198.7564336180209068, 286.3907539728338634, 17.89468790901915796 ) ) ;
#57281=CARTESIAN_POINT ( 'NONE',  ( 175.6467143226808503, 278.3879956775477922, 15.52796216301298315 ) ) ;
#57284=EDGE_CURVE ( 'NONE', #64387, #48833, #54576, .T. ) ;
#57286=CARTESIAN_POINT ( 'NONE',  ( 171.0076677319804332, 284.3901048210457247, 12.34237328981812176 ) ) ;
#57287=ORIENTED_EDGE ( 'NONE', *, *, #98412, .F. ) ;
#57290=CARTESIAN_POINT ( 'NONE',  ( 160.6728723076546430, 258.4027085289857837, -16.77127213560359920 ) ) ;
#57291=CARTESIAN_POINT ( 'NONE',  ( 70.67536410627003818, 221.6115022471903160, -5.000000000000047962 ) ) ;
#57294=EDGE_CURVE ( 'NONE', #81147, #73927, #35606, .T. ) ;
#57295=CARTESIAN_POINT ( 'NONE',  ( 190.7805732161387766, 300.2053494229706985, 4.237982805666590025 ) ) ;
#57296=CARTESIAN_POINT ( 'NONE',  ( 177.0083656731012525, 269.8104889733541540, 16.33643522331352216 ) ) ;
#57297=CARTESIAN_POINT ( 'NONE',  ( 164.9171241593586217, 245.0021572482830550, 1.622680932994367220 ) ) ;
#57298=CARTESIAN_POINT ( 'NONE',  ( 153.8341890703302113, 264.8936564568936660, -16.55105041955311407 ) ) ;
#57300=CARTESIAN_POINT ( 'NONE',  ( 207.8302079587528794, 270.6745157982714431, 3.572475529330238153 ) ) ;
#57302=CARTESIAN_POINT ( 'NONE',  ( 125.9656734773588767, 243.5333772461660544, 9.188101187500095079 ) ) ;
#57306=EDGE_CURVE ( 'NONE', #41965, #33184, #86444, .T. ) ;
#57309=CARTESIAN_POINT ( 'NONE',  ( -1.565588326081831072, 163.2365022471902307, 10.00000000000009948 ) ) ;
#57310=CARTESIAN_POINT ( 'NONE',  ( 177.8439380257527489, 255.3043160970806582, 4.874347355181736674 ) ) ;
#57313=CARTESIAN_POINT ( 'NONE',  ( 157.9403153459281839, 276.0785681647408865, -12.83070520789915037 ) ) ;
#57315=CARTESIAN_POINT ( 'NONE',  ( 182.1256972723869296, 260.2463563092551340, 10.61513437760372192 ) ) ;
#57316=CARTESIAN_POINT ( 'NONE',  ( 164.3231499090067302, 246.0309508282801971, -1.360008376207661573 ) ) ;
#57317=CARTESIAN_POINT ( 'NONE',  ( 132.6770232609232778, 259.6589784336661637, -6.496448406907676862E-16 ) ) ;
#57320=CARTESIAN_POINT ( 'NONE',  ( 53.24634253151052832, 210.7369531367911293, -4.594050593750048428 ) ) ;
#57321=CARTESIAN_POINT ( 'NONE',  ( 205.3708847852691406, 274.9341884869767227, -13.70973585089674174 ) ) ;
#57322=CARTESIAN_POINT ( 'NONE',  ( 153.1198285439165545, 279.2890930352092482, 3.903594709581249322 ) ) ;
#57324=CARTESIAN_POINT ( 'NONE',  ( 148.9230895364621574, 272.7046378331555161, 12.20434325797056019 ) ) ;
#57325=CARTESIAN_POINT ( 'NONE',  ( 155.4143072506629721, 279.7256007574335968, -1.410841605574949531 ) ) ;
#57326=CARTESIAN_POINT ( 'NONE',  ( 172.3432469182100988, 287.9044152303682154, -8.453389800301932766 ) ) ;
#57327=CARTESIAN_POINT ( 'NONE',  ( 159.2554912534056939, 254.8083930951974878, 16.49944922174842432 ) ) ;
#57328=CARTESIAN_POINT ( 'NONE',  ( 193.5827109575123188, 288.5416519977895291, 16.06052787264825810 ) ) ;
#57329=CARTESIAN_POINT ( 'NONE',  ( 135.4648896233454991, 249.0177522451418497, -10.00000000000009592 ) ) ;
#57331=EDGE_LOOP ( 'NONE', ( #3282, #26382, #72690, #79780, #90972 ) ) ;
#57334=CARTESIAN_POINT ( 'NONE',  ( 147.6121581866023007, 274.9752375363476631, 8.700660424766859080 ) ) ;
#57335=CARTESIAN_POINT ( 'NONE',  ( -14.30363896367569509, 171.7369531367911293, -4.594050593750048428 ) ) ;
#57336=CARTESIAN_POINT ( 'NONE',  ( 44.64073572505018461, 187.3923013555410080, 4.594050593750050204 ) ) ;
#57337=CARTESIAN_POINT ( 'NONE',  ( 175.5279092779543646, 256.8636307276551634, -10.65721348558485282 ) ) ;
#57340=CARTESIAN_POINT ( 'NONE',  ( 157.3661765229227285, 258.0807821998820373, -18.27254492731150748 ) ) ;
#57342=CARTESIAN_POINT ( 'NONE',  ( 190.3625087333586521, 300.9294583479858147, -4.271886578030237303 ) ) ;
#57344=CARTESIAN_POINT ( 'NONE',  ( 171.0951295267471721, 257.9025284764553021, 14.56267897235280984 ) ) ;
#57345=CARTESIAN_POINT ( 'NONE',  ( 48.42933654300934876, 208.7677522451419350, -5.000000000000047962 ) ) ;
#57346=CARTESIAN_POINT ( 'NONE',  ( 180.8196955730123818, 256.2390112858561793, 1.639671592817103063 ) ) ;
#57347=CARTESIAN_POINT ( 'NONE',  ( 205.3708847852691406, 274.9341884869767227, -13.70973585089674174 ) ) ;
#57348=CARTESIAN_POINT ( 'NONE',  ( 162.2336410148055279, 251.8862672885301492, -14.09881826716025799 ) ) ;
#57350=CARTESIAN_POINT ( 'NONE',  ( 50.39593590098449738, 193.2365022471902023, 10.00000000000009592 ) ) ;
#57351=CARTESIAN_POINT ( 'NONE',  ( 181.3600705323845261, 292.3670172205969493, 9.011603952510858662 ) ) ;
#57352=CARTESIAN_POINT ( 'NONE',  ( 49.43738778531180600, 210.8967562850346837, -4.648177544792955347E-16 ) ) ;
#57353=CARTESIAN_POINT ( 'NONE',  ( 5.777845730223497789, 164.9548013555410080, -4.594050593750042211 ) ) ;
#57355=CARTESIAN_POINT ( 'NONE',  ( 164.2487865911519975, 246.9563108291715992, 5.899911436263182374 ) ) ;
#57356=CARTESIAN_POINT ( 'NONE',  ( 152.8107382695299918, 265.9710327055011589, 16.32045346488711246 ) ) ;
#57360=CARTESIAN_POINT ( 'NONE',  ( 164.9335952247126045, 244.9736285262353306, -1.661461410667423255 ) ) ;
#57362=CARTESIAN_POINT ( 'NONE',  ( 196.3286486926436680, 290.5958008134369948, -16.58330917766970458 ) ) ;
#57366=CARTESIAN_POINT ( 'NONE',  ( 153.2953991261116187, 277.6583650081004748, -5.430105486410409021 ) ) ;
#57368=CARTESIAN_POINT ( 'NONE',  ( 157.4627203480516755, 258.4629190429250798, 16.86169483958236626 ) ) ;
#57369=CARTESIAN_POINT ( 'NONE',  ( 153.2427285380101978, 277.7181708921816607, -5.112331264339823989 ) ) ;
#57371=CARTESIAN_POINT ( 'NONE',  ( 206.6912923161529818, 272.6471755567893638, -9.325620632947922317 ) ) ;
#57372=CARTESIAN_POINT ( 'NONE',  ( 165.0391502558331069, 249.6778246878102436, -10.74756611015070717 ) ) ;
#57374=ORIENTED_EDGE ( 'NONE', *, *, #53633, .T. ) ;
#57375=CARTESIAN_POINT ( 'NONE',  ( 152.7531861616124615, 266.0707158804971186, 17.45453282433162556 ) ) ;
#57376=CARTESIAN_POINT ( 'NONE',  ( 164.4858674010174298, 245.7491158648375347, -2.958464974013825355 ) ) ;
#57378=EDGE_CURVE ( 'NONE', #28585, #49558, #50136, .T. ) ;
#57382=DIRECTION ( 'NONE',  ( -0.8660254037844387076, -0.4999999999999998890, -0.000000000000000000 ) ) ;
#57387=CARTESIAN_POINT ( 'NONE',  ( 174.3627903489640687, 262.5166068422508943, 14.67416242571188256 ) ) ;
#57394=CARTESIAN_POINT ( 'NONE',  ( 174.2647729094104818, 267.6455815624914862, 16.44362021030165977 ) ) ;
#57395=CARTESIAN_POINT ( 'NONE',  ( 169.1871453744360849, 276.0921898949916908, -15.50345989341305497 ) ) ;
#57398=CARTESIAN_POINT ( 'NONE',  ( 171.0009588779175829, 254.8957903787501493, -11.39820321899803623 ) ) ;
#57400=CARTESIAN_POINT ( 'NONE',  ( 156.9694903541507074, 266.1758412851487492, -17.34135443527054576 ) ) ;
#57402=CARTESIAN_POINT ( 'NONE',  ( 157.0523007431125961, 269.6879238887856332, 16.04707504889739056 ) ) ;
#57404=ADVANCED_FACE ( 'NONE', ( #85010 ), #65103, .F. ) ;
#57405=CARTESIAN_POINT ( 'NONE',  ( 193.9130084035158745, 294.7798125270166452, 13.46593982140802837 ) ) ;
#57406=CARTESIAN_POINT ( 'NONE',  ( 180.4099482243281045, 291.1497967234276416, -9.622827375937299976 ) ) ;
#57407=CYLINDRICAL_SURFACE ( 'NONE', #78679, 10.00000000000010658 ) ;
#57408=CARTESIAN_POINT ( 'NONE',  ( 199.6570654737131747, 281.0878073294180695, -17.28888823238446193 ) ) ;
#57409=CARTESIAN_POINT ( 'NONE',  ( 176.0858336914031383, 290.3330534276880144, 6.126020769380866149 ) ) ;
#57410=CARTESIAN_POINT ( 'NONE',  ( 197.5632903914970768, 288.4573386618801010, -18.12045497471262578 ) ) ;
#57411=EDGE_LOOP ( 'NONE', ( #17931, #63577, #89926, #14430 ) ) ;
#57412=CARTESIAN_POINT ( 'NONE',  ( 93.82350145804369390, 231.6427522451419065, -10.00000000000009592 ) ) ;
#57414=CARTESIAN_POINT ( 'NONE',  ( 164.5813345449211624, 245.5837619211427523, 1.447064457712487373 ) ) ;
#57415=CARTESIAN_POINT ( 'NONE',  ( 164.2813349609167517, 246.1033764428878214, 1.949810150281061638 ) ) ;
#57417=VERTEX_POINT ( 'NONE', #93440 ) ;
#57419=CARTESIAN_POINT ( 'NONE',  ( 190.3549927569640943, 300.9424764009692126, 6.306669742828282743 ) ) ;
#57421=EDGE_CURVE ( 'NONE', #30831, #80515, #61976, .T. ) ;
#57425=CARTESIAN_POINT ( 'NONE',  ( 198.8384730411855514, 286.2486575236893032, -17.11322556960806551 ) ) ;
#57426=CARTESIAN_POINT ( 'NONE',  ( 190.6136768402189716, 300.4944224256624921, -0.6663190606136376593 ) ) ;
#57428=CYLINDRICAL_SURFACE ( 'NONE', #5754, 17.82106496071139645 ) ;
#57431=CARTESIAN_POINT ( 'NONE',  ( -9.864998445682774175, 175.1115022471903160, -5.000000000000047962 ) ) ;
#57432=CARTESIAN_POINT ( 'NONE',  ( 30.74798454907712397, 181.8927522451418213, 10.00000000000009592 ) ) ;
#57433=CARTESIAN_POINT ( 'NONE',  ( 100.0117143358702236, 237.7369531367911009, -4.594050593750048428 ) ) ;
#57435=CARTESIAN_POINT ( 'NONE',  ( 168.2322000736707537, 260.5619311436532826, 16.64139255606118439 ) ) ;
#57437=CARTESIAN_POINT ( 'NONE',  ( 162.5429104506708597, 249.1144160197565043, 10.44355587256373674 ) ) ;
#57438=EDGE_CURVE ( 'NONE', #84087, #99795, #54973, .T. ) ;
#57439=CARTESIAN_POINT ( 'NONE',  ( 15.76359375002403596, 192.1589784336661637, -6.496448406907675876E-16 ) ) ;
#57440=CARTESIAN_POINT ( 'NONE',  ( 161.8016137473484548, 250.3983795733946636, 14.25000412375400316 ) ) ;
#57441=ORIENTED_EDGE ( 'NONE', *, *, #28208, .F. ) ;
#57443=CARTESIAN_POINT ( 'NONE',  ( 185.3693644285349365, 260.1071722789047271, -5.798844428750127733 ) ) ;
#57445=CARTESIAN_POINT ( 'NONE',  ( 146.8729474948188454, 276.2555880120147549, 3.934020695290606273 ) ) ;
#57446=DIRECTION ( 'NONE',  ( -0.8660254037844387076, -0.4999999999999998890, -0.000000000000000000 ) ) ;
#57448=CARTESIAN_POINT ( 'NONE',  ( 161.1093323826042933, 251.5974460702646809, -13.93502574894237078 ) ) ;
#57449=DIRECTION ( 'NONE',  ( 0.5000000000000001110, -0.8660254037844385966, 0.000000000000000000 ) ) ;
#57451=CARTESIAN_POINT ( 'NONE',  ( 45.07374842694240868, 187.6423013555410080, -4.594050593750043987 ) ) ;
#57452=CARTESIAN_POINT ( 'NONE',  ( 88.77168660263453148, 215.3927522451418213, -10.00000000000009059 ) ) ;
#57453=ADVANCED_FACE ( 'NONE', ( #46802 ), #42450, .F. ) ;
#57455=CARTESIAN_POINT ( 'NONE',  ( 179.2638961323747537, 258.2260800035196553, -10.18064271055803616 ) ) ;
#57456=CARTESIAN_POINT ( 'NONE',  ( -0.04102277327696322862, 170.7833772461660828, -9.188101187500095079 ) ) ;
#57458=CARTESIAN_POINT ( 'NONE',  ( 150.9363692955544991, 269.2175350005573478, -14.27857383982596140 ) ) ;
#57460=CARTESIAN_POINT ( 'NONE',  ( 192.6170194583582429, 297.0245312260774995, -11.90166228306590490 ) ) ;
#57462=CARTESIAN_POINT ( 'NONE',  ( 163.7136804588959649, 247.0865828815331042, 6.783386239354816105 ) ) ;
#57463=CARTESIAN_POINT ( 'NONE',  ( 146.6138605399200117, 276.7043397814778132, -0.5394499176159462950 ) ) ;
#57464=CARTESIAN_POINT ( 'NONE',  ( 206.9377610035629118, 272.2202792677204002, 7.440532334334675646 ) ) ;
#57465=ORIENTED_EDGE ( 'NONE', *, *, #87323, .T. ) ;
#57466=CARTESIAN_POINT ( 'NONE',  ( -2.503782513514959174, 159.3615022471902023, 5.000000000000051514 ) ) ;
#57469=CARTESIAN_POINT ( 'NONE',  ( 129.8627877943888791, 245.7833772461660544, -9.188101187500095079 ) ) ;
#57472=DIRECTION ( 'NONE',  ( -0.8660254037844387076, -0.4999999999999998890, -0.000000000000000000 ) ) ;
#57474=CARTESIAN_POINT ( 'NONE',  ( 185.6255372557312455, 288.0586212204385106, 14.85957563350848254 ) ) ;
#57475=CARTESIAN_POINT ( 'NONE',  ( 190.5723142641005552, 300.5660645090316052, -7.285051322221389292 ) ) ;
#57477=CARTESIAN_POINT ( 'NONE',  ( 191.5451565139252068, 298.8810523045859213, 7.782291334092181323 ) ) ;
#57478=CARTESIAN_POINT ( 'NONE',  ( 197.0184425104562820, 289.4010428742387262, -16.90752553128928426 ) ) ;
#57479=CARTESIAN_POINT ( 'NONE',  ( 190.6149048745654966, 300.0785874667154758, 3.592099452960924477 ) ) ;
#57480=CARTESIAN_POINT ( 'NONE',  ( 175.0221218187403451, 292.3615283621688832, -1.152100040113013479 ) ) ;
#57481=ORIENTED_EDGE ( 'NONE', *, *, #99481, .F. ) ;
#57484=CARTESIAN_POINT ( 'NONE',  ( 168.8129333540870221, 271.8871668449080516, -17.12755824114822900 ) ) ;
#57488=CARTESIAN_POINT ( 'NONE',  ( 200.2688005423887603, 272.3943678420544074, 12.70188190611125556 ) ) ;
#57491=EDGE_CURVE ( 'NONE', #39184, #21534, #41704, .T. ) ;
#57493=CARTESIAN_POINT ( 'NONE',  ( 153.4578721839791342, 264.8501638863745029, 16.85421393845643223 ) ) ;
#57495=CARTESIAN_POINT ( 'NONE',  ( 190.7685680519976188, 280.8244985282360631, 16.64107897673111580 ) ) ;
#57496=EDGE_CURVE ( 'NONE', #4766, #3950, #83706, .T. ) ;
#57498=CARTESIAN_POINT ( 'NONE',  ( 173.9239121147568881, 272.8349737613822867, -16.35791196226779931 ) ) ;
#57499=VERTEX_POINT ( 'NONE', #74496 ) ;
#57501=CARTESIAN_POINT ( 'NONE',  ( 164.5514333943684733, 280.2750504504191440, 12.59899363382133686 ) ) ;
#57502=EDGE_CURVE ( 'NONE', #31691, #93599, #63418, .T. ) ;
#57503=CARTESIAN_POINT ( 'NONE',  ( 147.7112127936102866, 274.8036699242858276, -9.124700685424272706 ) ) ;
#57509=B_SPLINE_CURVE_WITH_KNOTS ( 'NONE', 3,
 ( #28669, #44363, #5877, #21579, #92021, #75794, #84404, #14949, #37751, #7874, #75296, #36763, #83915, #91016, #92498, #45838, #30164, #98601, #68657, #22067, #76761, #29185, #6380, #15440, #52464, #46339, #7356, #60052, #38240, #69155, #45358, #76290, #83408, #100084, #13979, #44854, #90530, #29670, #61046, #61552, #6862, #99088, #84899, #21101, #23043, #53939, #77262, #38750 ),
 .UNSPECIFIED., .F., .F.,
 ( 4, 2, 2, 2, 2, 2, 2, 2, 2, 2, 2, 2, 2, 2, 2, 2, 2, 2, 2, 2, 2, 2, 2, 4 ),
 ( 0.003026550417145748746, 0.003224528412346372268, 0.003422506407546995789, 0.003521495405147307550, 0.003620484402747619311, 0.003818462397948246302, 0.004214418388349643399, 0.004610374378751041363, 0.005402286359553663819, 0.006194198340356286275, 0.006986110321158909599, 0.007778022301961532055, 0.007877011299561914939, 0.007926505798362145847, 0.007976000297162375019, 0.008025494795962605926, 0.008074989294762836833, 0.008173978292363319464, 0.008371956287564218807, 0.008569934282765118150, 0.008767912277966019227, 0.008965890273166920305, 0.009163868268367819647, 0.009361846263568718990 ),
 .UNSPECIFIED. ) ;
#57510=B_SPLINE_CURVE_WITH_KNOTS ( 'NONE', 3,
 ( #45626, #92776, #85706, #78056 ),
 .UNSPECIFIED., .F., .F.,
 ( 4, 4 ),
 ( 0.001468722747720561895, 0.009396689447536171053 ),
 .UNSPECIFIED. ) ;
#57511=ORIENTED_EDGE ( 'NONE', *, *, #70785, .T. ) ;
#57514=CARTESIAN_POINT ( 'NONE',  ( 185.0696649060035668, 259.9978788641606684, -6.171662045453295775 ) ) ;
#57515=ORIENTED_EDGE ( 'NONE', *, *, #8917, .T. ) ;
#57516=EDGE_LOOP ( 'NONE', ( #57924, #89693, #48684, #68954 ) ) ;
#57518=ORIENTED_EDGE ( 'NONE', *, *, #24922, .T. ) ;
#57520=VERTEX_POINT ( 'NONE', #3589 ) ;
#57522=CARTESIAN_POINT ( 'NONE',  ( 205.5791761573774181, 272.5734172477073116, 10.13670412909801044 ) ) ;
#57524=CARTESIAN_POINT ( 'NONE',  ( 182.8809842375080734, 280.3743175483600112, -16.11093289984563981 ) ) ;
#57526=CARTESIAN_POINT ( 'NONE',  ( 162.4754228937684957, 255.5738001540079836, -14.97516694854825658 ) ) ;
#57527=DIRECTION ( 'NONE',  ( -0.8660254037844387076, -0.4999999999999998890, -0.000000000000000000 ) ) ;
#57528=CARTESIAN_POINT ( 'NONE',  ( 147.5540328368684300, 275.0759135952944234, -4.750028533202499403 ) ) ;
#57532=CARTESIAN_POINT ( 'NONE',  ( 142.5284093247362591, 253.0958772461660544, -9.188101187500095079 ) ) ;
#57538=CARTESIAN_POINT ( 'NONE',  ( 3.125382611083894702, 162.6115022471902023, -5.000000000000041744 ) ) ;
#57539=CARTESIAN_POINT ( 'NONE',  ( 181.4954090331713417, 255.0423029034424189, 0.9094182891644410072 ) ) ;
#57541=CARTESIAN_POINT ( 'NONE',  ( 157.3462768699361902, 280.0432704934171397, -6.946531866745294437 ) ) ;
#57542=CARTESIAN_POINT ( 'NONE',  ( 173.8469137325424185, 256.4471593116459189, -12.44389045026504270 ) ) ;
#57545=CARTESIAN_POINT ( 'NONE',  ( 192.7433141272525745, 292.4329090757873360, -14.35978368495236168 ) ) ;
#57549=B_SPLINE_CURVE_WITH_KNOTS ( 'NONE', 3,
 ( #67958, #98878, #68444, #20378 ),
 .UNSPECIFIED., .F., .F.,
 ( 4, 4 ),
 ( 0.01007977251148702881, 0.01610653884049561071 ),
 .UNSPECIFIED. ) ;
#57550=CARTESIAN_POINT ( 'NONE',  ( 147.7112127936102866, 274.8036699242858276, -9.124700685424272706 ) ) ;
#57552=EDGE_LOOP ( 'NONE', ( #99784, #21401, #4582, #69206, #99441 ) ) ;
#57554=CARTESIAN_POINT ( 'NONE',  ( 201.2129524287560969, 267.2802673471600770, -2.216931291613017052 ) ) ;
#57555=FACE_OUTER_BOUND ( 'NONE', #77829, .T. ) ;
#57556=CARTESIAN_POINT ( 'NONE',  ( 190.7805732161387766, 300.2053494229706985, 4.237982805666590025 ) ) ;
#57558=CARTESIAN_POINT ( 'NONE',  ( 163.0309151244508712, 248.2691671304387739, 11.27270415168660200 ) ) ;
#57559=CARTESIAN_POINT ( 'NONE',  ( 156.5497824763685912, 272.6770023486104719, 14.78669166138748814 ) ) ;
#57561=CARTESIAN_POINT ( 'NONE',  ( 203.9077188555663156, 269.1475184353535042, 5.568207685932024198 ) ) ;
#57563=AXIS2_PLACEMENT_3D ( 'NONE', #28273, #50088, #73401 ) ;
#57564=CARTESIAN_POINT ( 'NONE',  ( 6.860117161356328097, 174.7677522451418781, 10.00000000000009592 ) ) ;
#57565=CARTESIAN_POINT ( 'NONE',  ( 189.8874520319352541, 274.0679647338298537, -15.62099291552114799 ) ) ;
#57567=VECTOR ( 'NONE', #1954, 1000.000000000000000 ) ;
#57571=CARTESIAN_POINT ( 'NONE',  ( 174.4665098196985298, 288.5002641398569949, -10.08633113632384237 ) ) ;
#57573=CARTESIAN_POINT ( 'NONE',  ( 1.609577830863368586, 180.9244531367911577, -4.594050593750046652 ) ) ;
#57574=CARTESIAN_POINT ( 'NONE',  ( 108.2124997955428967, 221.0327760586659451, 1.948934522072303157E-15 ) ) ;
#57575=CARTESIAN_POINT ( 'NONE',  ( 202.7973612924478743, 279.3916619310153919, -15.54732529288344089 ) ) ;
#57577=CARTESIAN_POINT ( 'NONE',  ( 182.4824444819098801, 257.3791432140518509, -2.310616456812910169 ) ) ;
#57579=CYLINDRICAL_SURFACE ( 'NONE', #38277, 17.82106496071139645 ) ;
#57581=CARTESIAN_POINT ( 'NONE',  ( 152.6809499003229860, 273.9044486092186048, 12.24870461040242553 ) ) ;
#57582=CARTESIAN_POINT ( 'NONE',  ( 148.3025927079438304, 273.7793698660844939, -8.046026357031887954 ) ) ;
#57583=CARTESIAN_POINT ( 'NONE',  ( 181.7688134247665630, 291.5467564283949855, 9.356705366744733965 ) ) ;
#57584=CARTESIAN_POINT ( 'NONE',  ( 205.5941538711272472, 274.5474750865108717, -13.11650762359312772 ) ) ;
#57586=CARTESIAN_POINT ( 'NONE',  ( 166.1724940190044606, 253.7130649904839572, -13.33068584944167512 ) ) ;
#57589=CARTESIAN_POINT ( 'NONE',  ( 81.04025856027610075, 229.8464784336661353, 1.353441290958777327E-15 ) ) ;
#57590=CARTESIAN_POINT ( 'NONE',  ( 207.8792014703394671, 270.5896565469619759, -5.780233892547864905 ) ) ;
#57592=CARTESIAN_POINT ( 'NONE',  ( 163.5110577551225788, 257.9154526713028304, 15.56383249676774128 ) ) ;
#57593=DIRECTION ( 'NONE',  ( -0.8660254037844387076, -0.4999999999999998890, -0.000000000000000000 ) ) ;
#57594=CARTESIAN_POINT ( 'NONE',  ( 151.7329441859792212, 267.8378268183080309, 16.45705841208969389 ) ) ;
#57597=VECTOR ( 'NONE', #4767, 1000.000000000000000 ) ;
#57603=CARTESIAN_POINT ( 'NONE',  ( 69.26781250152264136, 219.9869531367911293, 4.594050593750046652 ) ) ;
#57604=CARTESIAN_POINT ( 'NONE',  ( 172.2702976754117401, 289.2103317004583118, -1.060902075591837468 ) ) ;
#57605=CARTESIAN_POINT ( 'NONE',  ( 146.9700173529739970, 276.0874580858064746, -5.099093031535578469 ) ) ;
#57606=CARTESIAN_POINT ( 'NONE',  ( 188.0806836029928490, 285.9827684710060112, -16.28010878645887871 ) ) ;
#57612=CARTESIAN_POINT ( 'NONE',  ( 134.4004000680750437, 241.7365022471901739, -10.00000000000009059 ) ) ;
#57613=CARTESIAN_POINT ( 'NONE',  ( 205.2941531242069857, 275.0670916224857478, -13.92605142593109058 ) ) ;
#57616=CARTESIAN_POINT ( 'NONE',  ( 168.2388598609233554, 248.3799976336047166, -1.878115610807055136 ) ) ;
#57617=VERTEX_POINT ( 'NONE', #99276 ) ;
#57618=FACE_OUTER_BOUND ( 'NONE', #60611, .T. ) ;
#57619=CARTESIAN_POINT ( 'NONE',  ( 180.3910019823692323, 289.3959781800792257, -12.70720770915142062 ) ) ;
#57620=CARTESIAN_POINT ( 'NONE',  ( 164.8489450237687493, 247.1202469751449939, -7.123750760659631531 ) ) ;
#57622=EDGE_LOOP ( 'NONE', ( #87915, #80484, #47185, #83728, #56901 ) ) ;
#57624=EDGE_LOOP ( 'NONE', ( #15884, #83113, #23724, #45165 ) ) ;
#57625=CARTESIAN_POINT ( 'NONE',  ( 189.1366665130657623, 290.3664947348045757, 14.33938321420245110 ) ) ;
#57626=CARTESIAN_POINT ( 'NONE',  ( 167.6010540021560189, 247.4270797612363708, 3.638657435017179864 ) ) ;
#57627=CARTESIAN_POINT ( 'NONE',  ( 148.5637841791828464, 247.3923013555409796, 4.594050593750050204 ) ) ;
#57633=CARTESIAN_POINT ( 'NONE',  ( 164.7481050786816468, 274.5153366401211770, 14.74424062371369004 ) ) ;
#57634=CYLINDRICAL_SURFACE ( 'NONE', #1212, 10.00000000000010658 ) ;
#57638=CARTESIAN_POINT ( 'NONE',  ( 185.7832802462722555, 297.7360824256689966, 1.038627234575328240 ) ) ;
#57639=CARTESIAN_POINT ( 'NONE',  ( 164.0777181605478745, 246.4560510864015441, 5.763760713451748785 ) ) ;
#57644=CARTESIAN_POINT ( 'NONE',  ( 205.2391015854675516, 275.1624436846170738, -14.01434138479280911 ) ) ;
#57645=CARTESIAN_POINT ( 'NONE',  ( 207.7489713718107396, 270.8152216942889368, -5.185099786540344979 ) ) ;
#57646=CARTESIAN_POINT ( 'NONE',  ( 169.8538121856582563, 267.4705051540672116, 17.20835523141332146 ) ) ;
#57648=CARTESIAN_POINT ( 'NONE',  ( 101.4736528484039724, 220.2048013555409796, 4.594050593750051981 ) ) ;
#57652=CARTESIAN_POINT ( 'NONE',  ( 166.2874581756877035, 279.2881603620531337, -13.76640555504497954 ) ) ;
#57654=ORIENTED_EDGE ( 'NONE', *, *, #8315, .T. ) ;
#57657=CARTESIAN_POINT ( 'NONE',  ( 163.2352853045945267, 249.3765732455295563, 10.26252278998509659 ) ) ;
#57658=CARTESIAN_POINT ( 'NONE',  ( 159.6962080797732710, 254.0450491601782232, -15.33973334987084947 ) ) ;
#57659=CARTESIAN_POINT ( 'NONE',  ( 207.0998140485927479, 271.3089257990250758, -4.582213832299882661 ) ) ;
#57660=CARTESIAN_POINT ( 'NONE',  ( 91.83912023130210400, 214.6423013555409796, -4.594050593750043987 ) ) ;
#57662=VERTEX_POINT ( 'NONE', #6568 ) ;
#57664=CARTESIAN_POINT ( 'NONE',  ( 208.2912792141756029, 269.8759169579697641, -2.198672330625011995 ) ) ;
#57667=CARTESIAN_POINT ( 'NONE',  ( 153.6201142527220895, 265.1962041066475990, 16.40937927818958642 ) ) ;
#57669=ADVANCED_FACE ( 'NONE', ( #13669 ), #27115, .F. ) ;
#57671=CARTESIAN_POINT ( 'NONE',  ( 135.2750994722765654, 261.1589784336661637, -6.496448406907675876E-16 ) ) ;
#57672=DIRECTION ( 'NONE',  ( 0.4999999999999992784, -0.8660254037844390407, 0.000000000000000000 ) ) ;
#57673=CARTESIAN_POINT ( 'NONE',  ( -13.92449252947024263, 172.7677522451419350, -5.000000000000047962 ) ) ;
#57677=CARTESIAN_POINT ( 'NONE',  ( 157.1320038828994257, 274.0846122766332087, 13.24865132448945104 ) ) ;
#57678=CYLINDRICAL_SURFACE ( 'NONE', #9612, 10.00000000000010658 ) ;
#57679=CARTESIAN_POINT ( 'NONE',  ( 189.4938711747170146, 269.6765502774059087, 15.12816668017716459 ) ) ;
#57680=CARTESIAN_POINT ( 'NONE',  ( 167.4011299790239775, 281.5488363183706042, 12.98604958840868662 ) ) ;
#57684=CARTESIAN_POINT ( 'NONE',  ( 195.8015466934768654, 279.9124873149544896, -16.84388544808167154 ) ) ;
#57688=CARTESIAN_POINT ( 'NONE',  ( 167.7122741723079002, 249.7662244187599185, 7.851770579763321933 ) ) ;
#57690=CARTESIAN_POINT ( 'NONE',  ( 207.6875671281972870, 270.9215769640275653, -2.211577121115235300 ) ) ;
#57692=CARTESIAN_POINT ( 'NONE',  ( 162.9298729957551473, 248.4441772310448755, -10.24417153209544651 ) ) ;
#57693=VECTOR ( 'NONE', #13463, 1000.000000000000000 ) ;
#57695=CARTESIAN_POINT ( 'NONE',  ( 185.2999266589457932, 266.4615743673832071, 13.16452756711701966 ) ) ;
#57696=CARTESIAN_POINT ( 'NONE',  ( 184.7144364183202185, 266.1639934807288341, -14.90341959938623617 ) ) ;
#57699=CARTESIAN_POINT ( 'NONE',  ( 203.2369479875374623, 278.6302754407888074, -16.66242713208754367 ) ) ;
#57700=CARTESIAN_POINT ( 'NONE',  ( 157.6996016306053150, 271.0617617641458423, -14.71839889293659986 ) ) ;
#57703=CARTESIAN_POINT ( 'NONE',  ( 17.63104780087548562, 190.1744531367911293, 4.594050593750047540 ) ) ;
#57704=CARTESIAN_POINT ( 'NONE',  ( 90.45192255479418009, 211.4824982072973683, 3.021315404115420679E-15 ) ) ;
#57707=CARTESIAN_POINT ( 'NONE',  ( 192.7619763870382315, 275.9402076810760036, 17.00737747304665959 ) ) ;
#57709=CARTESIAN_POINT ( 'NONE',  ( 34.97905304013878691, 184.8768266524160140, 9.188101187500096856 ) ) ;
#57711=CARTESIAN_POINT ( 'NONE',  ( 147.5492216329511166, 275.0842468449245644, 4.751613690710122739 ) ) ;
#57713=CARTESIAN_POINT ( 'NONE',  ( 199.8627835468920466, 267.3049400163769178, -6.768725752350158054 ) ) ;
#57714=CARTESIAN_POINT ( 'NONE',  ( 177.7927449247031859, 293.7502563218264413, 2.765845172227290760 ) ) ;
#57715=CARTESIAN_POINT ( 'NONE',  ( 179.3005203053959633, 278.5776234110656446, -17.15738409824242083 ) ) ;
#57716=CARTESIAN_POINT ( 'NONE',  ( 160.4478367305730444, 269.5427765943644545, 17.02708557859721239 ) ) ;
#57719=CARTESIAN_POINT ( 'NONE',  ( 166.3765111647684023, 257.7471643095800573, -15.10258006359619465 ) ) ;
#57721=CARTESIAN_POINT ( 'NONE',  ( 81.06766895168334486, 217.6115022471902591, 10.00000000000009592 ) ) ;
#57723=CARTESIAN_POINT ( 'NONE',  ( 185.2419368458229769, 261.1426024236396870, -10.52247972935524345 ) ) ;
#57724=CARTESIAN_POINT ( 'NONE',  ( 48.05019010880389629, 207.7369531367911293, -4.594050593750048428 ) ) ;
#57727=CARTESIAN_POINT ( 'NONE',  ( 147.2494378675467033, 275.6034875578896504, 3.639370109197119341 ) ) ;
#57730=ORIENTED_EDGE ( 'NONE', *, *, #4586, .F. ) ;
#57731=CARTESIAN_POINT ( 'NONE',  ( 170.6096849177089894, 286.1922839665126048, 7.471123016262505523 ) ) ;
#57732=CARTESIAN_POINT ( 'NONE',  ( 164.5867587387928950, 245.5743669417666126, -3.022048486790635202 ) ) ;
#57735=CARTESIAN_POINT ( 'NONE',  ( 188.5767478252478213, 265.3039102131422737, 10.74219168877824160 ) ) ;
#57738=CARTESIAN_POINT ( 'NONE',  ( 174.0983890414937321, 257.0653133237892121, 11.33330784449225703 ) ) ;
#57742=EDGE_CURVE ( 'NONE', #62454, #28585, #39158, .T. ) ;
#57743=DIRECTION ( 'NONE',  ( -0.4330127018922184656, -0.2499999999999943934, 0.8660254037844407060 ) ) ;
#57744=CARTESIAN_POINT ( 'NONE',  ( 174.7807705099663451, 255.1531767004597953, 8.228258982011636746 ) ) ;
#57746=B_SPLINE_CURVE_WITH_KNOTS ( 'NONE', 3,
 ( #57368, #88342, #18899, #49778, #11310, #70572, #32066, #62978, #97886, #88847, #11798, #42167, #43147, #42653, #65475, #89338, #19411, #44149, #13288, #75083, #74088, #74600, #73587, #96417 ),
 .UNSPECIFIED., .F., .F.,
 ( 4, 2, 2, 2, 2, 2, 2, 2, 2, 2, 2, 4 ),
 ( 0.0002774176761712133306, 0.001899884551711553300, 0.002102692911154076423, 0.002153395001014668606, 0.002204097090875261223, 0.002229448135805543654, 0.002254799180735826518, 0.002305501270596266913, 0.002711117989480261482, 0.003116734708364256919, 0.003319543067806199777, 0.003522351427248143069 ),
 .UNSPECIFIED. ) ;
#57749=CARTESIAN_POINT ( 'NONE',  ( 164.7396270603856294, 269.0037874151494179, 17.61975801440670608 ) ) ;
#57753=ORIENTED_EDGE ( 'NONE', *, *, #28094, .T. ) ;
#57754=CIRCLE ( 'NONE', #91775, 17.82106496071138935 ) ;
#57755=CARTESIAN_POINT ( 'NONE',  ( 207.8570869662935365, 270.6279599915536664, -5.669188455878507504 ) ) ;
#57756=CARTESIAN_POINT ( 'NONE',  ( 151.0052876815146590, 270.5891121319239687, -13.76719987110444876 ) ) ;
#57757=DIRECTION ( 'NONE',  ( -0.8660254037844359321, -0.5000000000000051070, -0.000000000000000000 ) ) ;
#57760=CARTESIAN_POINT ( 'NONE',  ( 197.9598023461055902, 287.7705598106892921, 18.23120408239484291 ) ) ;
#57763=CARTESIAN_POINT ( 'NONE',  ( 157.0887340267001946, 258.5613266995183039, -17.61824281915036394 ) ) ;
#57764=CARTESIAN_POINT ( 'NONE',  ( 112.7044859340271614, 242.0024278399160949, 9.188101187500095079 ) ) ;
#57765=CARTESIAN_POINT ( 'NONE',  ( 181.8559320684326224, 273.7276056269956257, 17.73031764801637067 ) ) ;
#57766=CARTESIAN_POINT ( 'NONE',  ( 74.86346528667428402, 202.4824982072973967, 3.021315404115420679E-15 ) ) ;
#57767=ORIENTED_EDGE ( 'NONE', *, *, #84708, .T. ) ;
#57768=AXIS2_PLACEMENT_3D ( 'NONE', #12177, #57757, #43557 ) ;
#57769=CARTESIAN_POINT ( 'NONE',  ( 201.2806641633649747, 280.3747929596665927, 16.67906474368300707 ) ) ;
#57770=B_SPLINE_CURVE_WITH_KNOTS ( 'NONE', 3,
 ( #88623, #35354, #58153, #19192, #97198, #82993, #27765, #36345, #59636, #19684, #28249, #89613, #12070, #81020, #20175, #75373, #13078, #82000, #42928, #90608, #59124, #73867, #51042, #43449, #34844, #11581, #42439, #74390, #97684, #73375, #43939, #74878, #98177, #67247, #21175, #44441, #5955, #67756, #75881, #76840, #61631, #7437, #92585, #69238, #29752, #54515, #100168, #85493, #29261, #38330, #8447, #92106, #23127, #6459, #54022, #6941 ),
 .UNSPECIFIED., .F., .F.,
 ( 4, 2, 2, 2, 2, 2, 2, 2, 2, 2, 2, 2, 2, 2, 2, 2, 2, 2, 2, 2, 2, 2, 2, 2, 2, 2, 2, 4 ),
 ( 0.0007988174167732828290, 0.001285921168468543568, 0.001773024920163804525, 0.002016576796011434677, 0.002260128671859065481, 0.002381904609782880666, 0.002503680547706696284, 0.002625456485630511469, 0.002747232423554327087, 0.002990784299402038555, 0.003234336175249749590, 0.003721439926945132627, 0.004695647430335955080, 0.005669854933726776666, 0.006156958685422224756, 0.006400510561269988699, 0.006644062437117751775, 0.006704950406079751742, 0.006765838375041750841, 0.006826726344003750807, 0.006887614312965749039, 0.007009390250889750706, 0.007131166188813752374, 0.007374718064661747903, 0.007618269940509743432, 0.007861821816357739828, 0.008105373692205734490, 0.008592477443901725548 ),
 .UNSPECIFIED. ) ;
#57775=CARTESIAN_POINT ( 'NONE',  ( 65.45180129215621889, 220.8464784336661637, 1.353441290958777525E-15 ) ) ;
#57778=FACE_OUTER_BOUND ( 'NONE', #14160, .T. ) ;
#57779=CARTESIAN_POINT ( 'NONE',  ( 173.2412943989675398, 277.7050541934257240, 16.79641741871846250 ) ) ;
#57780=VERTEX_POINT ( 'NONE', #18670 ) ;
#57781=CARTESIAN_POINT ( 'NONE',  ( 180.3268137483904354, 258.1330830615356149, 10.30874540274224849 ) ) ;
#57783=CARTESIAN_POINT ( 'NONE',  ( 155.6281496932864457, 261.0911329737299980, -18.07904265579665548 ) ) ;
#57784=EDGE_LOOP ( 'NONE', ( #65663, #29486, #61482, #54155, #22158 ) ) ;
#57787=CARTESIAN_POINT ( 'NONE',  ( 207.1019571622349815, 271.9358831784929293, -5.989975140547304733 ) ) ;
#57788=CARTESIAN_POINT ( 'NONE',  ( 146.9129474150286683, 276.1863061179126930, -5.016087650759920358 ) ) ;
#57790=CARTESIAN_POINT ( 'NONE',  ( 205.7576124508049418, 274.2643565215761328, 10.88614016733041545 ) ) ;
#57792=CARTESIAN_POINT ( 'NONE',  ( 152.4046781316253316, 270.1998585947901006, -14.67976713775933639 ) ) ;
#57794=CARTESIAN_POINT ( 'NONE',  ( 167.2323824317113008, 256.3428130233486968, 13.71918974570849237 ) ) ;
#57795=CARTESIAN_POINT ( 'NONE',  ( 208.2175703429120688, 270.0035844679667889, 2.257951022351344150 ) ) ;
#57796=CARTESIAN_POINT ( 'NONE',  ( 124.8288415870092933, 249.0024278399161517, -9.188101187500093303 ) ) ;
#57797=VERTEX_POINT ( 'NONE', #50056 ) ;
#57804=CARTESIAN_POINT ( 'NONE',  ( 177.2585349158682959, 253.1952230001477915, 4.378219909316201530 ) ) ;
#57805=VERTEX_POINT ( 'NONE', #35348 ) ;
#57806=CARTESIAN_POINT ( 'NONE',  ( 177.1394999532559211, 267.7181704969479483, -17.21589890951720037 ) ) ;
#57807=CARTESIAN_POINT ( 'NONE',  ( 155.1068683166927826, 274.9036901648098592, 12.61603981672170072 ) ) ;
#57809=CARTESIAN_POINT ( 'NONE',  ( 207.1181895030469491, 269.9077679394811753, 1.745611964362854929 ) ) ;
#57810=CARTESIAN_POINT ( 'NONE',  ( 165.0803978706131545, 244.7193588848498678, -1.793249961207334486 ) ) ;
#57813=DIRECTION ( 'NONE',  ( -0.8660254037844387076, -0.4999999999999998890, -0.000000000000000000 ) ) ;
#57814=CARTESIAN_POINT ( 'NONE',  ( 155.0584575552912554, 280.8822639477641587, 1.046265068571241796 ) ) ;
#57816=AXIS2_PLACEMENT_3D ( 'NONE', #7423, #77335, #69225 ) ;
#57819=B_SPLINE_SURFACE_WITH_KNOTS ( 'NONE', 3, 1, ( 
 ( #89986, #42826 ),
 ( #73760, #95612 ),
 ( #4352, #28145 ),
 ( #59017, #20563 ),
 ( #26161, #57038 ),
 ( #18569, #49448 ),
 ( #80402, #10972 ),
 ( #41844, #72792 ),
 ( #3382, #23017 ),
 ( #5845, #75261 ),
 ( #30132, #83378 ),
 ( #98570, #99060 ),
 ( #36731, #53424 ),
 ( #67140, #98062 ),
 ( #45809, #67636 ),
 ( #61526, #14921 ),
 ( #52431, #37234 ),
 ( #84374, #6833 ),
 ( #76734, #44825 ),
 ( #84869, #21549 ),
 ( #7328, #92470 ),
 ( #14446, #90500 ),
 ( #100052, #29153 ),
 ( #29642, #13944 ),
 ( #60024, #91987 ),
 ( #28638, #90988 ),
 ( #61015, #45327 ),
 ( #75760, #15412 ),
 ( #68132, #6346 ),
 ( #38208, #37718 ),
 ( #68628, #74774 ),
 ( #44329, #76261 ),
 ( #69126, #60515 ),
 ( #53910, #5353 ) ),
 .UNSPECIFIED., .T., .F., .F.,
 ( 4, 2, 2, 2, 2, 2, 2, 2, 2, 2, 2, 2, 2, 2, 2, 2, 4 ),
 ( 2, 2 ),
 ( 0.000000000000000000, 0.06250000000000000000, 0.1250000000000000000, 0.1875000000000000000, 0.2500000000000000000, 0.3125000000000000000, 0.3750000000000000000, 0.4375000000000000000, 0.5000000000000000000, 0.5625000000000000000, 0.6250000000000000000, 0.6875000000000000000, 0.7500000000000000000, 0.8125000000000000000, 0.8750000000000000000, 0.9375000000000000000, 1.000000000000000000 ),
 ( 0.000000000000000000, 1.000000000000000000 ),
 .UNSPECIFIED. ) ;
#57821=EDGE_CURVE ( 'NONE', #28867, #24384, #28419, .T. ) ;
#57823=CARTESIAN_POINT ( 'NONE',  ( 154.8891180328150199, 280.6470120869327616, -0.9323348256675227930 ) ) ;
#57824=CARTESIAN_POINT ( 'NONE',  ( 169.5939356907569788, 285.2851384293307433, -7.966250160088273802 ) ) ;
#57826=CARTESIAN_POINT ( 'NONE',  ( 193.4739544967976883, 288.6957167552757255, 16.02685211616793381 ) ) ;
#57827=CARTESIAN_POINT ( 'NONE',  ( 132.9389821956409037, 240.8927522451417929, -10.00000000000009059 ) ) ;
#57830=CARTESIAN_POINT ( 'NONE',  ( 157.6335212189247557, 257.6177276032722716, 16.76495363836117036 ) ) ;
#57831=CARTESIAN_POINT ( 'NONE',  ( 190.5893431400089923, 300.5365696307625853, -0.3099240395267599535 ) ) ;
#57832=CARTESIAN_POINT ( 'NONE',  ( -5.047471817081990331, 158.7048013555409796, 4.594050593750051981 ) ) ;
#57833=CARTESIAN_POINT ( 'NONE',  ( 36.49425040099653472, 198.0024278399160949, -9.188101187500093303 ) ) ;
#57834=CARTESIAN_POINT ( 'NONE',  ( 175.4085403292222338, 256.6757290962687534, -10.74039065239221102 ) ) ;
#57838=CARTESIAN_POINT ( 'NONE',  ( 205.3465787480556344, 274.9762877783610406, -13.79319041940166279 ) ) ;
#57840=CARTESIAN_POINT ( 'NONE',  ( 147.4963928429778264, 275.1757489932608109, 4.929816573182678852 ) ) ;
#57843=CARTESIAN_POINT ( 'NONE',  ( 74.41009865654255862, 213.7677522451418497, 10.00000000000009592 ) ) ;
#57846=DIRECTION ( 'NONE',  ( -0.8660254037844387076, -0.4999999999999998890, -0.000000000000000000 ) ) ;
#57847=ADVANCED_FACE ( 'NONE', ( #68234 ), #5454, .T. ) ;
#57848=CARTESIAN_POINT ( 'NONE',  ( 180.0741617902815221, 294.2070188947237739, 1.027227668438557506 ) ) ;
#57849=CARTESIAN_POINT ( 'NONE',  ( 42.09652578138363310, 185.1115022471902023, -5.000000000000041744 ) ) ;
#57851=B_SPLINE_CURVE_WITH_KNOTS ( 'NONE', 3,
 ( #39741, #32673, #15455, #1285, #32169, #85944, #78794, #63573, #86438, #77277, #77799, #7369, #23060, #275, #92512, #45853, #31655, #54447, #38765, #16472, #46353, #63073, #94016, #62051, #7888, #39249, #46873, #54965, #8382, #24568, #47367, #78290, #70160, #769, #16965, #47855, #9380, #71198, #84419, #76776, #69168, #100100, #30684, #61564, #11893, #17994 ),
 .UNSPECIFIED., .F., .F.,
 ( 4, 2, 2, 2, 2, 2, 2, 2, 2, 2, 2, 2, 2, 2, 2, 2, 2, 2, 2, 2, 2, 2, 4 ),
 ( 0.0009592261741756381941, 0.001443980160452349847, 0.001928734146729061717, 0.002171111139867377103, 0.002413488133005692489, 0.002534676629574850616, 0.002655865126144008742, 0.002777053622713166435, 0.002898242119282324562, 0.003140619112420641248, 0.003382996105558959236, 0.003867750091835591743, 0.004837258064388857623, 0.005806766036942124370, 0.006291520023218749071, 0.006776274009495372903, 0.006897462506064565291, 0.006958056754349161918, 0.007018651002633757678, 0.007261027995772108626, 0.007745781982048733326, 0.008230535968325358026, 0.008715289954601980124 ),
 .UNSPECIFIED. ) ;
#57852=CARTESIAN_POINT ( 'NONE',  ( 163.3543347837650686, 247.7089878483399730, 10.92686688779373405 ) ) ;
#57853=CARTESIAN_POINT ( 'NONE',  ( 3.179769518870181777, 163.4548013555410080, -4.594050593750042211 ) ) ;
#57855=CARTESIAN_POINT ( 'NONE',  ( 162.0143583332327921, 251.6182954191690726, 13.01856005289551277 ) ) ;
#57856=CARTESIAN_POINT ( 'NONE',  ( 153.3920560952016956, 264.9641606960921649, 16.50453917291963535 ) ) ;
#57858=DIRECTION ( 'NONE',  ( -0.8660254037844387076, -0.4999999999999998890, -0.000000000000000000 ) ) ;
#57859=CARTESIAN_POINT ( 'NONE',  ( 179.4673683373077893, 277.3829114355249317, 16.47530701906485717 ) ) ;
#57861=CARTESIAN_POINT ( 'NONE',  ( 154.8679462054080318, 262.4078440388265676, 17.98338675682672871 ) ) ;
#57863=CARTESIAN_POINT ( 'NONE',  ( 145.5865615336240353, 244.8615022471901739, 5.000000000000051514 ) ) ;
#57869=EDGE_CURVE ( 'NONE', #61372, #17056, #22137, .T. ) ;
#57870=CARTESIAN_POINT ( 'NONE',  ( 153.1651950822421213, 277.6376015683730998, -5.200947853335143201 ) ) ;
#57871=ORIENTED_EDGE ( 'NONE', *, *, #8317, .T. ) ;
#57872=CARTESIAN_POINT ( 'NONE',  ( 105.6772241758911264, 238.4865022471902876, -10.00000000000009592 ) ) ;
#57876=( BOUNDED_CURVE ( )  B_SPLINE_CURVE ( 2, ( #55338, #40641, #25976, #78171, #87342, #33055, #56846, #85828, #2675 ),
 .UNSPECIFIED., .F., .T. ) 
 B_SPLINE_CURVE_WITH_KNOTS ( ( 3, 2, 2, 2, 3 ),
 ( 0.8508064516129032473, 0.8521505376344086224, 0.8548387096774193727, 0.8575268817204301230, 0.8588709677419354982 ),
 .UNSPECIFIED. ) 
 CURVE ( )  GEOMETRIC_REPRESENTATION_ITEM ( )  RATIONAL_B_SPLINE_CURVE ( ( 0.9330127018922194093, 0.9330127018922194093, 1.000000000000000000, 0.8660254037844387076, 1.000000000000000000, 0.8660254037844387076, 1.000000000000000000, 0.9330127018922194093, 0.9330127018922194093 ) ) 
 REPRESENTATION_ITEM ( '' )  );
#57877=CARTESIAN_POINT ( 'NONE',  ( 153.4389798490260262, 264.8828863703868137, 16.68923469758090761 ) ) ;
#57878=CARTESIAN_POINT ( 'NONE',  ( 164.4440639631384045, 245.8215215431751233, -2.910115319305802029 ) ) ;
#57880=CARTESIAN_POINT ( 'NONE',  ( 125.2349645446897455, 233.1115022471901739, -5.000000000000041744 ) ) ;
#57882=ORIENTED_EDGE ( 'NONE', *, *, #70803, .T. ) ;
#57883=CARTESIAN_POINT ( 'NONE',  ( 164.5368030896599691, 246.5300180790061404, -4.380742116717776469 ) ) ;
#57884=CARTESIAN_POINT ( 'NONE',  ( 204.7235752877335244, 276.0553614249301972, 14.82397698933823271 ) ) ;
#57885=CARTESIAN_POINT ( 'NONE',  ( 192.0331311261993790, 298.0358554833232461, 11.82583305898340953 ) ) ;
#57888=CARTESIAN_POINT ( 'NONE',  ( 193.4764931876557341, 292.8054267365567966, 15.43080237163636070 ) ) ;
#57889=CARTESIAN_POINT ( 'NONE',  ( 178.1396926282777997, 263.7657380533013907, 15.23609645299708326 ) ) ;
#57890=B_SPLINE_CURVE_WITH_KNOTS ( 'NONE', 3,
 ( #91894, #69037, #78157, #8253, #1155, #16344, #7237, #30551, #9252, #32029, #85816, #93382, #8745, #39118 ),
 .UNSPECIFIED., .F., .F.,
 ( 4, 2, 2, 2, 2, 2, 4 ),
 ( 0.001181140099763508013, 0.001412183555258165199, 0.001643227010752822386, 0.001874270466247479790, 0.002105313921742136760, 0.002567400832731370035, 0.003029487743720602876 ),
 .UNSPECIFIED. ) ;
#57897=CARTESIAN_POINT ( 'NONE',  ( 200.8551880497955437, 282.7556046643899776, 18.00894873733387058 ) ) ;
#57898=CARTESIAN_POINT ( 'NONE',  ( 166.2168471871404734, 273.8149888340271900, -15.47012930002172837 ) ) ;
#57902=CARTESIAN_POINT ( 'NONE',  ( 190.0259678364800493, 301.5123642802043946, 4.004183174499006626 ) ) ;
#57903=CARTESIAN_POINT ( 'NONE',  ( 203.0398866899141126, 278.9715956204779559, 16.57839218037009132 ) ) ;
#57905=CARTESIAN_POINT ( 'NONE',  ( 156.8156315612123137, 266.4525211182331077, -16.29134938265778842 ) ) ;
#57907=CARTESIAN_POINT ( 'NONE',  ( 157.1309033697166910, 269.5518756982808668, 15.81807010761959731 ) ) ;
#57910=CARTESIAN_POINT ( 'NONE',  ( 159.0726324473315003, 259.5960639973407638, 16.73037245408614027 ) ) ;
#57911=CARTESIAN_POINT ( 'NONE',  ( 193.6284877719895974, 295.2726167166218829, 14.91976605476162021 ) ) ;
#57913=CARTESIAN_POINT ( 'NONE',  ( 138.2253456014563255, 250.6115022471902591, 10.00000000000009592 ) ) ;
#57915=CARTESIAN_POINT ( 'NONE',  ( 164.5329775610532010, 278.6465748849269062, -13.92721442706176482 ) ) ;
#57916=CARTESIAN_POINT ( 'NONE',  ( 158.7792683104916307, 255.6332354280542063, -16.04672224821257487 ) ) ;
#57918=ORIENTED_EDGE ( 'NONE', *, *, #27159, .F. ) ;
#57921=CARTESIAN_POINT ( 'NONE',  ( 106.5950644350847369, 243.8967562850346837, -4.648177544792955347E-16 ) ) ;
#57922=CARTESIAN_POINT ( 'NONE',  ( 0.9806730298622799991, 159.8262482093458061, 3.021315404115420679E-15 ) ) ;
#57924=ORIENTED_EDGE ( 'NONE', *, *, #62513, .T. ) ;
#57925=CARTESIAN_POINT ( 'NONE',  ( 187.1732433188570894, 276.9074010399757526, 16.80578958361036257 ) ) ;
#57926=CARTESIAN_POINT ( 'NONE',  ( 171.4502695138348543, 259.7973668612793290, -14.48892546229642520 ) ) ;
#57927=CARTESIAN_POINT ( 'NONE',  ( 163.5859548838263038, 247.8737923133996901, 8.124920029444005820 ) ) ;
#57930=CARTESIAN_POINT ( 'NONE',  ( 159.9421317827104758, 253.6190968119055356, -14.98049406679499640 ) ) ;
#57932=ORIENTED_EDGE ( 'NONE', *, *, #33652, .T. ) ;
#57933=CARTESIAN_POINT ( 'NONE',  ( 167.4864847214653594, 252.8241918798602228, -12.40380003664212616 ) ) ;
#57935=FACE_OUTER_BOUND ( 'NONE', #99892, .T. ) ;
#57936=CARTESIAN_POINT ( 'NONE',  ( 164.9404048476745004, 244.9618339132846074, -2.801285734921658666 ) ) ;
#57937=CARTESIAN_POINT ( 'NONE',  ( 32.84087927488948822, 189.7677522451418497, 10.00000000000009592 ) ) ;
#57938=CARTESIAN_POINT ( 'NONE',  ( 105.1271107466783121, 225.3768266524160140, 9.188101187500096856 ) ) ;
#57939=ADVANCED_FACE ( 'NONE', ( #68733 ), #60617, .T. ) ;
#57940=CARTESIAN_POINT ( 'NONE',  ( 170.8865616681041786, 262.8912071418242817, 16.88624067591380040 ) ) ;
#57941=CARTESIAN_POINT ( 'NONE',  ( 162.6515360750312027, 249.5066621596292293, -10.92528266655622815 ) ) ;
#57943=CARTESIAN_POINT ( 'NONE',  ( 207.8833583980453739, 270.5824565369721313, 1.564926904161892285 ) ) ;
#57944=CARTESIAN_POINT ( 'NONE',  ( 19.87790860953014160, 170.0327760586659736, 1.948934522072303157E-15 ) ) ;
#57945=CARTESIAN_POINT ( 'NONE',  ( 174.8250621633554260, 255.6858076512632465, 11.15776497395374101 ) ) ;
#57948=CARTESIAN_POINT ( 'NONE',  ( 147.5268811534417637, 275.7712507861047584, -0.5032726463638115266 ) ) ;
#57950=DIRECTION ( 'NONE',  ( -0.8660254037844387076, -0.4999999999999998890, -0.000000000000000000 ) ) ;
#57951=EDGE_CURVE ( 'NONE', #13801, #62993, #49960, .T. ) ;
#57952=CARTESIAN_POINT ( 'NONE',  ( 190.4976253092930278, 300.6954295735222900, -5.764807383508308902 ) ) ;
#57953=CARTESIAN_POINT ( 'NONE',  ( 148.1846401255833996, 275.9836697316168284, -5.368268268079755323 ) ) ;
#57954=CARTESIAN_POINT ( 'NONE',  ( 207.1211793645798878, 271.9025893473983047, -6.294110402770905388 ) ) ;
#57956=CARTESIAN_POINT ( 'NONE',  ( 37.98264478980979675, 201.9244531367911293, -4.594050593750046652 ) ) ;
#57957=CARTESIAN_POINT ( 'NONE',  ( 100.3908607700757472, 218.7677522451417644, -5.000000000000041744 ) ) ;
#57958=CIRCLE ( 'NONE', #23955, 17.82106496071138224 ) ;
#57962=CARTESIAN_POINT ( 'NONE',  ( 179.0719375569688623, 258.5579859881011657, -10.02328217832856438 ) ) ;
#57964=CARTESIAN_POINT ( 'NONE',  ( 8.700681467995980967, 166.6423013555410080, -4.594050593750043987 ) ) ;
#57967=CARTESIAN_POINT ( 'NONE',  ( 198.5511052797322975, 286.7463930869835167, -17.24711022262289006 ) ) ;
#57969=CARTESIAN_POINT ( 'NONE',  ( 146.7842303614460207, 276.4092505945183689, -4.491116827832889236 ) ) ;
#57970=B_SPLINE_CURVE_WITH_KNOTS ( 'NONE', 3,
 ( #39480, #61795, #54684, #31893 ),
 .UNSPECIFIED., .F., .F.,
 ( 4, 4 ),
 ( 0.01044120455681045272, 0.01649765149563178768 ),
 .UNSPECIFIED. ) ;
#57972=CARTESIAN_POINT ( 'NONE',  ( 203.6934353594241713, 276.2490116884532654, 13.33169628994285993 ) ) ;
#57974=CARTESIAN_POINT ( 'NONE',  ( 164.2953672501826929, 246.0790718049323687, -2.576662677987826111 ) ) ;
#57976=ADVANCED_FACE ( 'NONE', ( #99656 ), #14225, .F. ) ;
#57978=CARTESIAN_POINT ( 'NONE',  ( -9.431985743790550103, 175.3615022471903160, 5.000000000000046185 ) ) ;
#57980=CARTESIAN_POINT ( 'NONE',  ( 129.3218690127885964, 233.2202760586659736, -5.415160957724236172E-17 ) ) ;
#57983=CARTESIAN_POINT ( 'NONE',  ( 43.73836560584370403, 189.3927522451417929, 10.00000000000009948 ) ) ;
#57985=CARTESIAN_POINT ( 'NONE',  ( 196.0727848089514964, 291.0389700598140621, 17.56388901715066808 ) ) ;
#57988=CARTESIAN_POINT ( 'NONE',  ( 150.2569279433535883, 270.3943619433326830, -14.69852926823082839 ) ) ;
#57989=ORIENTED_EDGE ( 'NONE', *, *, #85701, .F. ) ;
#57990=CARTESIAN_POINT ( 'NONE',  ( 150.6453220160077251, 269.7216436761371483, 14.94145576020818034 ) ) ;
#57991=CARTESIAN_POINT ( 'NONE',  ( 208.0000668123412595, 270.3803116337406891, -0.2337639243167183301 ) ) ;
#57992=CARTESIAN_POINT ( 'NONE',  ( 189.6738045434663320, 300.1223289962524063, 4.832295392723879424 ) ) ;
#57993=CARTESIAN_POINT ( 'NONE',  ( 172.4614876683343425, 267.8189099582538120, -16.31738736074272467 ) ) ;
#57996=LINE ( 'NONE', #11918, #13410 ) ;
#58001=CARTESIAN_POINT ( 'NONE',  ( 182.0170707230944060, 295.5524055634063529, 4.928801494141618278 ) ) ;
#58003=CARTESIAN_POINT ( 'NONE',  ( 150.7797507404552846, 277.9900660939502473, -8.190901894163754267E-05 ) ) ;
#58005=ORIENTED_EDGE ( 'NONE', *, *, #24461, .F. ) ;
#58006=CARTESIAN_POINT ( 'NONE',  ( 194.3983564485891975, 282.9291968243864517, 17.33109156482955626 ) ) ;
#58009=ORIENTED_EDGE ( 'NONE', *, *, #20721, .F. ) ;
#58010=CARTESIAN_POINT ( 'NONE',  ( 161.5515493166768977, 252.8315038724842623, 14.92355679770252053 ) ) ;
#58011=CARTESIAN_POINT ( 'NONE',  ( 196.4164021072083983, 270.5621661862001019, 13.33908636140236936 ) ) ;
#58012=CARTESIAN_POINT ( 'NONE',  ( 159.7180752573169684, 264.1341207546815895, -17.45630029751305656 ) ) ;
#58013=ORIENTED_EDGE ( 'NONE', *, *, #13054, .T. ) ;
#58015=CARTESIAN_POINT ( 'NONE',  ( 184.8456707333363909, 292.0357465481239387, 12.28532852304464207 ) ) ;
#58016=B_SPLINE_CURVE_WITH_KNOTS ( 'NONE', 3,
 ( #27341, #72962, #10648, #49627 ),
 .UNSPECIFIED., .F., .F.,
 ( 4, 4 ),
 ( 0.01255948763041959439, 0.01883562040667947218 ),
 .UNSPECIFIED. ) ;
#58020=ORIENTED_EDGE ( 'NONE', *, *, #90808, .T. ) ;
#58021=CARTESIAN_POINT ( 'NONE',  ( 87.26533679362427165, 215.0643266524160140, 9.188101187500095079 ) ) ;
#58023=CARTESIAN_POINT ( 'NONE',  ( 185.4243904228094095, 269.9367370257660355, 16.45094022865727368 ) ) ;
#58024=CARTESIAN_POINT ( 'NONE',  ( 185.2398828118039660, 259.7113007520022734, -6.730862835317267034 ) ) ;
#58026=ORIENTED_EDGE ( 'NONE', *, *, #43789, .F. ) ;
#58027=CARTESIAN_POINT ( 'NONE',  ( 175.0695970114038005, 258.6570182761398655, 12.72039775904022996 ) ) ;
#58029=CARTESIAN_POINT ( 'NONE',  ( 181.9559929377375056, 291.6402902057536721, -11.43735378946719372 ) ) ;
#58032=CARTESIAN_POINT ( 'NONE',  ( 202.9490938173916561, 279.1288534886517709, -16.56031645010252973 ) ) ;
#58034=CARTESIAN_POINT ( 'NONE',  ( 207.3202802199240296, 271.5577365501114286, -6.820371601869826605 ) ) ;
#58037=CARTESIAN_POINT ( 'NONE',  ( 161.7372449923526005, 277.0660816109730717, -12.77480613138230581 ) ) ;
#58038=CARTESIAN_POINT ( 'NONE',  ( 200.6985908945154335, 283.0268388936558495, -17.74173253065502820 ) ) ;
#58042=CARTESIAN_POINT ( 'NONE',  ( 0.1899651733832354861, 182.4637435831425307, 2.679491924311264039 ) ) ;
#58043=CARTESIAN_POINT ( 'NONE',  ( 139.9303331133829715, 251.5958772461660544, -9.188101187500095079 ) ) ;
#58047=EDGE_LOOP ( 'NONE', ( #33657, #29010, #5061, #56627 ) ) ;
#58050=ORIENTED_EDGE ( 'NONE', *, *, #11399, .T. ) ;
#58054=CARTESIAN_POINT ( 'NONE',  ( 155.4334144234936446, 278.1011161893850954, 7.188626922287153498 ) ) ;
#58055=CARTESIAN_POINT ( 'NONE',  ( 165.5206796362886053, 246.9121039173171539, -1.897138224611882640 ) ) ;
#58056=CARTESIAN_POINT ( 'NONE',  ( 171.1951747928532086, 280.5720821316805313, 13.82413286205249214 ) ) ;
#58057=CARTESIAN_POINT ( 'NONE',  ( 168.0789332142355761, 252.9049754911962964, 11.87642061956828421 ) ) ;
#58064=CARTESIAN_POINT ( 'NONE',  ( 163.8880225243198083, 277.8562197680003010, 13.11111227161160997 ) ) ;
#58065=CARTESIAN_POINT ( 'NONE',  ( 200.9648348225670986, 267.8090230095998550, -2.831290352090367612 ) ) ;
#58066=CARTESIAN_POINT ( 'NONE',  ( 163.8376739375615614, 246.8718198766768808, -7.388296869948213441 ) ) ;
#58067=CARTESIAN_POINT ( 'NONE',  ( 190.0445576990143195, 301.4801656937889902, 4.140328216824785912 ) ) ;
#58068=CARTESIAN_POINT ( 'NONE',  ( 164.5368361882794943, 274.3627312642749416, 14.76381770633092216 ) ) ;
#58069=CARTESIAN_POINT ( 'NONE',  ( 160.9899226891051569, 282.1625248316790362, -7.707013335689073763 ) ) ;
#58072=CARTESIAN_POINT ( 'NONE',  ( 200.8804270585581833, 268.5305093043455145, 6.050783656218224671 ) ) ;
#58074=B_SPLINE_SURFACE_WITH_KNOTS ( 'NONE', 3, 1, ( 
 ( #58391, #96452 ),
 ( #27018, #88882 ),
 ( #57902, #4198 ),
 ( #97426, #81744 ),
 ( #50794, #74123 ),
 ( #4719, #66500 ),
 ( #58875, #89844 ),
 ( #53765, #8192 ),
 ( #29985, #54258 ),
 ( #93320, #13792 ),
 ( #62363, #97 ),
 ( #7686, #587 ),
 ( #39061, #60865 ),
 ( #22879, #69973 ),
 ( #91827, #14296 ),
 ( #45668, #53285 ),
 ( #31472, #15266 ),
 ( #98911, #29492 ),
 ( #37087, #46681 ),
 ( #52773, #68478 ),
 ( #84237, #99900 ),
 ( #52285, #14786 ),
 ( #85229, #60368 ),
 ( #44671, #30980 ),
 ( #61867, #21886 ),
 ( #83733, #46161 ),
 ( #91326, #45182 ),
 ( #6192, #83226 ),
 ( #76592, #22389 ),
 ( #76121, #75604 ),
 ( #6694, #23372 ),
 ( #67991, #7178 ),
 ( #77607, #30487 ),
 ( #37571, #99408 ) ),
 .UNSPECIFIED., .T., .F., .F.,
 ( 4, 2, 2, 2, 2, 2, 2, 2, 2, 2, 2, 2, 2, 2, 2, 2, 4 ),
 ( 2, 2 ),
 ( 0.000000000000000000, 0.06250000000000000000, 0.1250000000000000000, 0.1875000000000000000, 0.2500000000000000000, 0.3125000000000000000, 0.3750000000000000000, 0.4375000000000000000, 0.5000000000000000000, 0.5625000000000000000, 0.6250000000000000000, 0.6875000000000000000, 0.7500000000000000000, 0.8125000000000000000, 0.8750000000000000000, 0.9375000000000000000, 1.000000000000000000 ),
 ( 0.000000000000000000, 1.000000000000000000 ),
 .UNSPECIFIED. ) ;
#58076=CARTESIAN_POINT ( 'NONE',  ( 190.2656474672665468, 273.4017421308091684, -16.11817620543089191 ) ) ;
#58079=CYLINDRICAL_SURFACE ( 'NONE', #64713, 10.00000000000010658 ) ;
#58083=CARTESIAN_POINT ( 'NONE',  ( 9.052243966459650792, 176.0333772461660828, 9.188101187500095079 ) ) ;
#58084=CARTESIAN_POINT ( 'NONE',  ( 110.0524566828198232, 234.3458772461660544, 9.188101187500095079 ) ) ;
#58085=CARTESIAN_POINT ( 'NONE',  ( 155.3513572141771704, 261.5705516107003064, -17.00592413546589299 ) ) ;
#58087=CARTESIAN_POINT ( 'NONE',  ( 180.1973933060313868, 254.8900073420350907, -2.451664709510168016 ) ) ;
#58089=FACE_OUTER_BOUND ( 'NONE', #86595, .T. ) ;
#58090=DIRECTION ( 'NONE',  ( 0.4999999999999992784, -0.8660254037844390407, 0.000000000000000000 ) ) ;
#58091=CARTESIAN_POINT ( 'NONE',  ( 147.9500839974939197, 274.3899328626944225, -9.375093207164509224 ) ) ;
#58096=CARTESIAN_POINT ( 'NONE',  ( 173.1833993531181193, 264.1544810417100848, -15.45454764063065234 ) ) ;
#58097=CARTESIAN_POINT ( 'NONE',  ( 70.64795371486285092, 223.8464784336661637, 1.353441290958777327E-15 ) ) ;
#58098=CARTESIAN_POINT ( 'NONE',  ( 207.1211793645798878, 271.9025893473983047, -6.294110402770905388 ) ) ;
#58099=DIRECTION ( 'NONE',  ( -0.8660254037844387076, -0.4999999999999998890, -0.000000000000000000 ) ) ;
#58102=CARTESIAN_POINT ( 'NONE',  ( 157.7861133721078772, 257.3534302411229646, 18.03837896619386783 ) ) ;
#58104=CARTESIAN_POINT ( 'NONE',  ( 198.7829547491859330, 286.3448180261817129, -18.59838968157616179 ) ) ;
#58105=CARTESIAN_POINT ( 'NONE',  ( 196.8708119716154954, 268.3476497963631573, -11.07389558091716708 ) ) ;
#58112=CARTESIAN_POINT ( 'NONE',  ( 173.1286500857816293, 289.7119308821054346, -0.9330850667108907537 ) ) ;
#58114=CARTESIAN_POINT ( 'NONE',  ( 191.7217873212802601, 287.9217275298282743, -15.84537559439743326 ) ) ;
#58117=DIRECTION ( 'NONE',  ( -0.8660254037844387076, -0.4999999999999998890, -0.000000000000000000 ) ) ;
#58118=VECTOR ( 'NONE', #40933, 1000.000000000000000 ) ;
#58119=CARTESIAN_POINT ( 'NONE',  ( 122.6368883333364295, 231.6115022471901739, -5.000000000000041744 ) ) ;
#58120=CARTESIAN_POINT ( 'NONE',  ( 157.3198323354746435, 258.1610526871778006, -16.77630483474704093 ) ) ;
#58123=CARTESIAN_POINT ( 'NONE',  ( 166.1868863523491484, 247.3274724192857548, -1.867640438089152033 ) ) ;
#58125=CARTESIAN_POINT ( 'NONE',  ( 202.7865629936218284, 279.4103651332174536, 17.10878160033216133 ) ) ;
#58131=CARTESIAN_POINT ( 'NONE',  ( 205.7209699951682182, 274.3278231164531462, 10.82489695893654158 ) ) ;
#58134=CARTESIAN_POINT ( 'NONE',  ( 195.0052008962354648, 274.1277100424396167, 15.91609426908852498 ) ) ;
#58139=CARTESIAN_POINT ( 'NONE',  ( 164.5161215291067549, 274.6587578575884550, 14.67424033123101879 ) ) ;
#58140=CARTESIAN_POINT ( 'NONE',  ( 170.9811431790156462, 280.9458665424763240, 14.82329785628973440 ) ) ;
#58143=CARTESIAN_POINT ( 'NONE',  ( 182.7859092779136745, 296.3208846843115225, 0.2810723611678059286 ) ) ;
#58145=CARTESIAN_POINT ( 'NONE',  ( 165.3416878791837803, 273.7316169911477459, -15.20817556363227574 ) ) ;
#58147=CARTESIAN_POINT ( 'NONE',  ( 201.3405586841460035, 274.8867726572458423, -14.10034985609714298 ) ) ;
#58148=CARTESIAN_POINT ( 'NONE',  ( 147.5531173542960062, 275.8601889253673676, 0.6003615892798087605 ) ) ;
#58150=B_SPLINE_CURVE_WITH_KNOTS ( 'NONE', 3,
 ( #59193, #57714, #19264, #50131, #33954, #97262, #81083, #4524, #89679, #20240, #11649, #42509, #73445, #12647, #74456, #5036, #64841, #66819, #97747, #28315, #90169, #20742, #41520, #51629, #10645, #3068, #84563, #28829, #45008, #74943, #14127, #7508, #67315, #44507, #84074, #6020, #21234, #37899, #21722, #30322, #52113, #98243, #83563, #60196, #53117, #38405, #99235, #61704, #5527, #6530 ),
 .UNSPECIFIED., .F., .F.,
 ( 4, 2, 2, 2, 2, 2, 2, 2, 2, 2, 2, 2, 2, 2, 2, 2, 2, 2, 2, 2, 2, 2, 2, 2, 4 ),
 ( 0.0003069541420656791151, 0.0007786567417661697209, 0.001250359341466660218, 0.001368284991391783764, 0.001486210641316906660, 0.001604136291242029989, 0.001722061941167153318, 0.001957913241017399976, 0.002193764540867646634, 0.002665467140568139950, 0.003137169740268633700, 0.004080574939669620767, 0.005023980139070607399, 0.005495682738771066021, 0.005731534038621340435, 0.005849459688546477208, 0.005908422513509046028, 0.005967385338471614849, 0.006026348163434183669, 0.006085310988396752489, 0.006203236638321890997, 0.006439087938172168013, 0.006910790537872688218, 0.007382493137573210157, 0.007854195737273732963 ),
 .UNSPECIFIED. ) ;
#58151=LINE ( 'NONE', #11579, #54336 ) ;
#58153=CARTESIAN_POINT ( 'NONE',  ( 181.2447728743449318, 255.8601296356839327, 5.264276447811296222 ) ) ;
#58154=CARTESIAN_POINT ( 'NONE',  ( 93.32716752435031538, 230.8149278399160949, -9.188101187500095079 ) ) ;
#58155=VERTEX_POINT ( 'NONE', #12961 ) ;
#58157=CARTESIAN_POINT ( 'NONE',  ( 166.8362749997322965, 278.2767805360451803, -13.32482071573584648 ) ) ;
#58158=EDGE_LOOP ( 'NONE', ( #29035, #76035, #21093, #17784 ) ) ;
#58162=CARTESIAN_POINT ( 'NONE',  ( 195.7291850945597957, 291.6341022226063160, 17.08310330964873813 ) ) ;
#58163=CARTESIAN_POINT ( 'NONE',  ( 166.0506673010352472, 274.1027903476490337, -16.62009509085023851 ) ) ;
#58164=CARTESIAN_POINT ( 'NONE',  ( 163.1177074157340030, 248.1188384722309195, 11.53923137679231026 ) ) ;
#58165=CARTESIAN_POINT ( 'NONE',  ( 101.7984123748231298, 220.3923013555410080, 4.594050593750050204 ) ) ;
#58167=( BOUNDED_CURVE ( )  B_SPLINE_CURVE ( 2, ( #74585, #5164, #36043, #97874, #20878, #5652, #51767, #75072, #90805 ),
 .UNSPECIFIED., .F., .T. ) 
 B_SPLINE_CURVE_WITH_KNOTS ( ( 3, 2, 2, 2, 3 ),
 ( 0.1330645161290322509, 0.1344086021505376261, 0.1370967741935483764, 0.1397849462365591267, 0.1411290322580645296 ),
 .UNSPECIFIED. ) 
 CURVE ( )  GEOMETRIC_REPRESENTATION_ITEM ( )  RATIONAL_B_SPLINE_CURVE ( ( 0.9330127018922194093, 0.9330127018922194093, 1.000000000000000000, 0.8660254037844387076, 1.000000000000000000, 0.8660254037844387076, 1.000000000000000000, 0.9330127018922187432, 0.9330127018922194093 ) ) 
 REPRESENTATION_ITEM ( '' )  );
#58170=VERTEX_POINT ( 'NONE', #38196 ) ;
#58172=CARTESIAN_POINT ( 'NONE',  ( 194.0048607262993698, 265.9479453833899925, -7.746409940373651715 ) ) ;
#58175=CARTESIAN_POINT ( 'NONE',  ( 138.9021014942714487, 244.8768266524159856, 9.188101187500098632 ) ) ;
#58176=DIRECTION ( 'NONE',  ( -0.8660254037844387076, -0.4999999999999998890, -0.000000000000000000 ) ) ;
#58177=CARTESIAN_POINT ( 'NONE',  ( -8.223158621222619757, 159.3927522451418213, 10.00000000000009592 ) ) ;
#58178=CARTESIAN_POINT ( 'NONE',  ( 156.2745578679571565, 265.5782693780779482, -17.38162733845839369 ) ) ;
#58179=VECTOR ( 'NONE', #25072, 1000.000000000000000 ) ;
#58181=CARTESIAN_POINT ( 'NONE',  ( 156.9196333786560160, 258.8542176135235877, 18.37000459710097644 ) ) ;
#58184=CARTESIAN_POINT ( 'NONE',  ( 170.5373622343556690, 269.7751423367952270, 17.81562764448176850 ) ) ;
#58185=CARTESIAN_POINT ( 'NONE',  ( 165.8206990081297931, 283.8978799598649516, 9.576760697357309837 ) ) ;
#58188=CARTESIAN_POINT ( 'NONE',  ( 199.0694199359834045, 281.8589904182013015, -16.59703209974210836 ) ) ;
#58189=ADVANCED_FACE ( 'NONE', ( #59003 ), #52919, .T. ) ;
#58190=DIRECTION ( 'NONE',  ( -0.8660254037844387076, -0.4999999999999998890, -0.000000000000000000 ) ) ;
#58193=DIRECTION ( 'NONE',  ( 0.4999999999999998890, -0.8660254037844385966, 0.000000000000000000 ) ) ;
#58195=CARTESIAN_POINT ( 'NONE',  ( 167.5939664823378337, 249.9752123500401524, 7.239111559830059939 ) ) ;
#58197=CARTESIAN_POINT ( 'NONE',  ( 163.3473224498206093, 247.7211335670114352, -10.00320358166632850 ) ) ;
#58198=DIRECTION ( 'NONE',  ( -0.8660254037844387076, -0.4999999999999998890, -0.000000000000000000 ) ) ;
#58202=CARTESIAN_POINT ( 'NONE',  ( 185.2385187869343213, 266.4459329430754906, 13.17615627545476720 ) ) ;
#58206=CARTESIAN_POINT ( 'NONE',  ( 192.1883190596398094, 297.7670620978826150, 12.41391288785556668 ) ) ;
#58208=CARTESIAN_POINT ( 'NONE',  ( 157.6042236584425780, 270.9851239571572705, -14.73351287006370391 ) ) ;
#58210=CARTESIAN_POINT ( 'NONE',  ( 13.97758990260114231, 185.0024278399160949, 9.188101187500095079 ) ) ;
#58211=CARTESIAN_POINT ( 'NONE',  ( 207.0684042065635992, 270.3832170946865858, 3.383249001289787117 ) ) ;
#58214=CARTESIAN_POINT ( 'NONE',  ( 29.10614472461697133, 197.6115022471903160, -5.000000000000047962 ) ) ;
#58216=CARTESIAN_POINT ( 'NONE',  ( 38.76756708593069334, 199.3149278399161517, -9.188101187500095079 ) ) ;
#58217=CARTESIAN_POINT ( 'NONE',  ( 200.8828793852583203, 282.7076418644388696, 17.90302398138411633 ) ) ;
#58218=CARTESIAN_POINT ( 'NONE',  ( 190.9441801652054096, 299.9219738747156043, -4.765040093794296716 ) ) ;
#58221=CARTESIAN_POINT ( 'NONE',  ( 146.8637854207107409, 276.2714571898724216, 0.7988785540157756770 ) ) ;
#58222=CARTESIAN_POINT ( 'NONE',  ( 178.9700315119640663, 278.3247164859652685, -16.90640454279861160 ) ) ;
#58224=CARTESIAN_POINT ( 'NONE',  ( 166.8083734521890449, 257.5796782931630560, -15.79284703031436798 ) ) ;
#58226=CARTESIAN_POINT ( 'NONE',  ( 86.26382137438996267, 220.6115022471902591, 10.00000000000009592 ) ) ;
#58229=ORIENTED_EDGE ( 'NONE', *, *, #64953, .F. ) ;
#58230=CARTESIAN_POINT ( 'NONE',  ( 41.74435586355720318, 207.1589784336661637, -6.496448406907675876E-16 ) ) ;
#58231=ORIENTED_EDGE ( 'NONE', *, *, #83285, .T. ) ;
#58233=CARTESIAN_POINT ( 'NONE',  ( 150.6815632051821581, 269.6588720951601772, -14.68790257316217307 ) ) ;
#58237=CARTESIAN_POINT ( 'NONE',  ( 167.3858196111910388, 285.2936306680765028, 7.894013122999995247 ) ) ;
#58238=CARTESIAN_POINT ( 'NONE',  ( 164.9335952247126045, 244.9736285262353306, -1.661461410667423255 ) ) ;
#58241=CARTESIAN_POINT ( 'NONE',  ( 187.1111986486765488, 263.3028977142639633, 11.61052883540825142 ) ) ;
#58244=CARTESIAN_POINT ( 'NONE',  ( 171.3908936290850988, 255.6478991229282940, 12.28342243807102996 ) ) ;
#58245=ORIENTED_EDGE ( 'NONE', *, *, #39446, .F. ) ;
#58248=CARTESIAN_POINT ( 'NONE',  ( 174.8768402572162302, 255.1920038171627709, 8.200017817996553049 ) ) ;
#58249=CARTESIAN_POINT ( 'NONE',  ( 170.2148221929604119, 256.7370173464272511, -14.26952246837105598 ) ) ;
#58252=CARTESIAN_POINT ( 'NONE',  ( 150.6655900823359389, 269.6865383554857090, 15.31288044136207205 ) ) ;
#58254=EDGE_CURVE ( 'NONE', #28329, #22379, #426, .T. ) ;
#58255=AXIS2_PLACEMENT_3D ( 'NONE', #56695, #24304, #80040 ) ;
#58257=CARTESIAN_POINT ( 'NONE',  ( 207.7296438747196134, 270.8486979012336633, -6.692930657757584001 ) ) ;
#58259=CARTESIAN_POINT ( 'NONE',  ( 148.9831146496684084, 272.6006712873522133, -12.63706091291043343 ) ) ;
#58262=CARTESIAN_POINT ( 'NONE',  ( 171.5146026185341839, 284.8826077422594949, -12.15938192449176114 ) ) ;
#58266=CARTESIAN_POINT ( 'NONE',  ( 197.9919592856120687, 286.7924423995140728, 16.94645048433601531 ) ) ;
#58267=B_SPLINE_CURVE_WITH_KNOTS ( 'NONE', 3,
 ( #58011, #88992, #84342, #30101 ),
 .UNSPECIFIED., .F., .F.,
 ( 4, 4 ),
 ( 0.007886306542003318140, 0.01295349318365762899 ),
 .UNSPECIFIED. ) ;
#58268=CARTESIAN_POINT ( 'NONE',  ( 104.4229444624559591, 243.3464784336661637, 1.353441290958777525E-15 ) ) ;
#58269=CARTESIAN_POINT ( 'NONE',  ( 122.9742295596836925, 230.2592609112380160, 2.679491924311254714 ) ) ;
#58270=DIRECTION ( 'NONE',  ( -0.8660254037844387076, -0.4999999999999998890, -0.000000000000000000 ) ) ;
#58272=ORIENTED_EDGE ( 'NONE', *, *, #65624, .T. ) ;
#58273=CARTESIAN_POINT ( 'NONE',  ( 163.7423057141168385, 247.0370024851108610, -6.909410042141566066 ) ) ;
#58277=CARTESIAN_POINT ( 'NONE',  ( 194.9396225458042409, 291.6968222089742540, -15.91036236140263505 ) ) ;
#58278=CARTESIAN_POINT ( 'NONE',  ( 80.33713356334875755, 211.0643266524159856, -9.188101187500093303 ) ) ;
#58279=CARTESIAN_POINT ( 'NONE',  ( -5.676897265278508797, 155.9824982072973683, -6.972266317189433020E-16 ) ) ;
#58280=CARTESIAN_POINT ( 'NONE',  ( 191.4484954869714954, 299.0484741143815199, 8.684991747358081327 ) ) ;
#58282=CARTESIAN_POINT ( 'NONE',  ( 175.5122396641868079, 278.4443030880159426, 15.47154450738855225 ) ) ;
#58288=CARTESIAN_POINT ( 'NONE',  ( 194.7230684019799867, 293.3767474524976251, 15.79132110000472444 ) ) ;
#58290=CARTESIAN_POINT ( 'NONE',  ( 161.6923300915171922, 250.5876644177310482, -14.43081872899884566 ) ) ;
#58293=CARTESIAN_POINT ( 'NONE',  ( 176.9285354572846245, 269.9431028654713032, 17.13598235524080238 ) ) ;
#58296=CARTESIAN_POINT ( 'NONE',  ( 203.2757866645317222, 269.5093088776978334, -7.514607224931010521 ) ) ;
#58297=CARTESIAN_POINT ( 'NONE',  ( 119.4704829489755724, 239.7833772461660544, -9.188101187500095079 ) ) ;
#58298=ORIENTED_EDGE ( 'NONE', *, *, #63555, .F. ) ;
#58300=CARTESIAN_POINT ( 'NONE',  ( 81.86698606425520097, 229.6199935810941213, 2.679491924311251605 ) ) ;
#58301=EDGE_CURVE ( 'NONE', #87041, #79979, #52999, .T. ) ;
#58302=CARTESIAN_POINT ( 'NONE',  ( 155.2193237801463113, 261.7992402267395846, -18.58295809893692407 ) ) ;
#58303=CARTESIAN_POINT ( 'NONE',  ( 204.9780665305064531, 275.6145696623662502, 14.10615427165218883 ) ) ;
#58304=CARTESIAN_POINT ( 'NONE',  ( -9.431985743790550103, 175.3615022471903160, 5.000000000000046185 ) ) ;
#58305=CARTESIAN_POINT ( 'NONE',  ( 181.0465414429574480, 255.4906575730030340, -4.757053701627741660 ) ) ;
#58308=CARTESIAN_POINT ( 'NONE',  ( 167.5331536921724194, 249.1563084341292154, -5.485378542569181448 ) ) ;
#58310=CARTESIAN_POINT ( 'NONE',  ( 206.6672608846700427, 272.6887992170966299, -10.88770374553082121 ) ) ;
#58311=ADVANCED_FACE ( 'NONE', ( #96588 ), #36586, .T. ) ;
#58313=EDGE_CURVE ( 'NONE', #4228, #43534, #24651, .T. ) ;
#58314=CARTESIAN_POINT ( 'NONE',  ( 147.3154503175461514, 275.4891506405583073, 3.671329888160011823 ) ) ;
#58316=EDGE_CURVE ( 'NONE', #53063, #57662, #5282, .T. ) ;
#58317=CARTESIAN_POINT ( 'NONE',  ( 170.7054206766590880, 250.3903097054384546, 3.971403188103841408 ) ) ;
#58319=CARTESIAN_POINT ( 'NONE',  ( 190.0340467409721441, 301.4983712071542641, 4.077645795029533282 ) ) ;
#58321=CARTESIAN_POINT ( 'NONE',  ( 169.4000131232833155, 285.1406234409721492, -8.020725679492032967 ) ) ;
#58322=CARTESIAN_POINT ( 'NONE',  ( 198.2114954873088948, 287.3346145022089786, 18.52864136173620935 ) ) ;
#58324=CARTESIAN_POINT ( 'NONE',  ( 157.3983369238794410, 271.2561898657742745, -14.62425919491228044 ) ) ;
#58325=CARTESIAN_POINT ( 'NONE',  ( 136.7639277290220718, 259.7677522451419350, -5.000000000000047962 ) ) ;
#58326=CARTESIAN_POINT ( 'NONE',  ( 173.0666269367678751, 283.8557712307529073, -12.24563893785450297 ) ) ;
#58328=CARTESIAN_POINT ( 'NONE',  ( 157.8360072705708603, 257.2670114739976839, 17.12122855844125269 ) ) ;
#58329=CARTESIAN_POINT ( 'NONE',  ( 147.8465295590381743, 274.5692944114487091, 9.322947948439978205 ) ) ;
#58330=CARTESIAN_POINT ( 'NONE',  ( -1.664820405372784862, 169.8458772461660544, 9.188101187500095079 ) ) ;
#58331=CARTESIAN_POINT ( 'NONE',  ( 45.42531092540608029, 197.0333772461660828, 9.188101187500095079 ) ) ;
#58332=CARTESIAN_POINT ( 'NONE',  ( 178.2615612386009047, 258.9310810631866389, -10.32181247301958571 ) ) ;
#58335=DIRECTION ( 'NONE',  ( 0.4999999999999992784, -0.8660254037844390407, 0.000000000000000000 ) ) ;
#58339=CARTESIAN_POINT ( 'NONE',  ( 171.3032759856405107, 258.3952365426850974, 14.09859993956650648 ) ) ;
#58340=CARTESIAN_POINT ( 'NONE',  ( 61.85273030166814578, 216.5177522451419065, 5.000000000000046185 ) ) ;
#58343=CARTESIAN_POINT ( 'NONE',  ( 162.2150750494025431, 251.9152425808378553, -13.05861332114117168 ) ) ;
#58344=CARTESIAN_POINT ( 'NONE',  ( 40.00363105557123333, 187.2365022471902023, 10.00000000000009592 ) ) ;
#58346=CARTESIAN_POINT ( 'NONE',  ( 163.4216610345155800, 247.5923753613567442, 10.58669027323842826 ) ) ;
#58347=CARTESIAN_POINT ( 'NONE',  ( -3.478321416370212305, 177.9869531367911293, 4.594050593750046652 ) ) ;
#58348=CARTESIAN_POINT ( 'NONE',  ( 165.7591614932538278, 285.0852518727915594, 4.131734285391062578 ) ) ;
#58352=CARTESIAN_POINT ( 'NONE',  ( 207.6628070930962906, 270.9644626028195376, 7.378217122120054761 ) ) ;
#58353=CARTESIAN_POINT ( 'NONE',  ( 154.8989000222956349, 262.3542304552891551, 17.41779271305265908 ) ) ;
#58354=CARTESIAN_POINT ( 'NONE',  ( 196.3507576896697344, 290.5575069072837664, -17.68249398312240928 ) ) ;
#58358=CARTESIAN_POINT ( 'NONE',  ( 165.4299515451023410, 285.6795224695716229, -0.1515405553588986542 ) ) ;
#58362=CARTESIAN_POINT ( 'NONE',  ( 193.7118145980225279, 295.1282904202991517, 14.61271143546694162 ) ) ;
#58368=ORIENTED_EDGE ( 'NONE', *, *, #6025, .T. ) ;
#58369=CARTESIAN_POINT ( 'NONE',  ( 152.3564455502385044, 267.3888446593566641, 15.42595238024932414 ) ) ;
#58373=EDGE_LOOP ( 'NONE', ( #37741, #69256, #64107, #77981 ) ) ;
#58376=CARTESIAN_POINT ( 'NONE',  ( 204.2129321040862919, 276.9398213635460024, 14.41515352680879758 ) ) ;
#58377=CARTESIAN_POINT ( 'NONE',  ( 192.0963028965829551, 297.9264387674147656, 11.34530024772836754 ) ) ;
#58380=CARTESIAN_POINT ( 'NONE',  ( 168.4954155832338074, 247.6751246288074526, 2.275130870958896434 ) ) ;
#58382=EDGE_CURVE ( 'NONE', #22391, #47320, #82665, .T. ) ;
#58384=CARTESIAN_POINT ( 'NONE',  ( 78.23504418992378362, 222.6427522451419065, -10.00000000000009592 ) ) ;
#58387=CARTESIAN_POINT ( 'NONE',  ( 177.6900565734887323, 268.6111475138295646, 16.75654593232756540 ) ) ;
#58388=CARTESIAN_POINT ( 'NONE',  ( 166.4818116705677653, 274.3668896485694404, -15.18083394624400562 ) ) ;
#58389=CARTESIAN_POINT ( 'NONE',  ( 150.8884397357406328, 275.9708103743298580, -8.379586308329308508 ) ) ;
#58390=ORIENTED_EDGE ( 'NONE', *, *, #55901, .F. ) ;
#58391=CARTESIAN_POINT ( 'NONE',  ( 190.0445576990143195, 301.4801656937889902, 4.140328216824785912 ) ) ;
#58392=CARTESIAN_POINT ( 'NONE',  ( 200.7812400522830956, 279.0213764812114050, 16.52495314239560287 ) ) ;
#58393=ORIENTED_EDGE ( 'NONE', *, *, #76233, .F. ) ;
#58395=DIRECTION ( 'NONE',  ( -0.4999999999999987788, 0.8660254037844392627, 0.000000000000000000 ) ) ;
#58398=AXIS2_PLACEMENT_3D ( 'NONE', #20519, #81356, #59981 ) ;
#58399=ORIENTED_EDGE ( 'NONE', *, *, #59171, .T. ) ;
#58400=CARTESIAN_POINT ( 'NONE',  ( 159.1259971461353473, 259.5205376126884858, 16.70218726448308999 ) ) ;
#58401=CYLINDRICAL_SURFACE ( 'NONE', #69391, 17.82106496071139645 ) ;
#58402=CARTESIAN_POINT ( 'NONE',  ( 193.9583149726292959, 294.7013392473955946, 13.54389207180881805 ) ) ;
#58403=CARTESIAN_POINT ( 'NONE',  ( 188.5999732098899528, 298.6034004545671223, -4.739567632090335714 ) ) ;
#58404=CARTESIAN_POINT ( 'NONE',  ( 132.5758265486178971, 258.8967562850347122, -4.648177544792955347E-16 ) ) ;
#58406=CARTESIAN_POINT ( 'NONE',  ( 178.0302064638906074, 292.4640037680099454, 7.106335582765731296 ) ) ;
#58407=CARTESIAN_POINT ( 'NONE',  ( 158.3871229378075611, 256.3124511374962253, -17.26248367166835607 ) ) ;
#58408=ORIENTED_EDGE ( 'NONE', *, *, #13718, .F. ) ;
#58413=ORIENTED_EDGE ( 'NONE', *, *, #17631, .T. ) ;
#58415=CARTESIAN_POINT ( 'NONE',  ( 190.4191603088290776, 300.8313349409419288, 6.519931150822659838 ) ) ;
#58418=CARTESIAN_POINT ( 'NONE',  ( -22.42236680055709641, 157.8615022471902591, 0.000000000000000000 ) ) ;
#58419=CARTESIAN_POINT ( 'NONE',  ( 177.9714937548455680, 255.7189482022137383, 8.882064279750110813 ) ) ;
#58420=CARTESIAN_POINT ( 'NONE',  ( 160.0245045302084179, 253.4764230280800916, -16.06816193402951853 ) ) ;
#58421=CARTESIAN_POINT ( 'NONE',  ( 190.1563334688368911, 301.2865643814013765, -1.454600626587476686 ) ) ;
#58422=ORIENTED_EDGE ( 'NONE', *, *, #63334, .T. ) ;
#58426=CARTESIAN_POINT ( 'NONE',  ( 164.3774690880109119, 245.9368672504194819, -2.805681983503304000 ) ) ;
#58427=CARTESIAN_POINT ( 'NONE',  ( 29.80979036164399432, 178.0177522451417929, 5.000000000000051514 ) ) ;
#58428=CARTESIAN_POINT ( 'NONE',  ( 101.9874215621947116, 235.8149278399160949, 9.188101187500093303 ) ) ;
#58431=CARTESIAN_POINT ( 'NONE',  ( 164.0889469084813186, 280.5819020075147705, -11.59149887344287677 ) ) ;
#58432=CARTESIAN_POINT ( 'NONE',  ( 195.6974783896144174, 291.6890198465123945, 16.70600479393688431 ) ) ;
#58433=CARTESIAN_POINT ( 'NONE',  ( 165.0952264510788154, 281.4963861521250124, -11.84807672454148886 ) ) ;
#58434=CARTESIAN_POINT ( 'NONE',  ( 21.44705901024191874, 189.3149278399161233, 9.188101187500093303 ) ) ;
#58435=CARTESIAN_POINT ( 'NONE',  ( 153.1198285439165545, 279.2890930352092482, 3.903594709581249322 ) ) ;
#58437=VERTEX_POINT ( 'NONE', #39064 ) ;
#58445=( BOUNDED_CURVE ( )  B_SPLINE_CURVE ( 2, ( #14200, #28393, #52678, #36990, #91726, #74530, #44576, #6095, #90248 ),
 .UNSPECIFIED., .F., .T. ) 
 B_SPLINE_CURVE_WITH_KNOTS ( ( 3, 2, 2, 2, 3 ),
 ( 0.3427419354838709964, 0.3440860215053763715, 0.3467741935483871218, 0.3494623655913978721, 0.3508064516129032473 ),
 .UNSPECIFIED. ) 
 CURVE ( )  GEOMETRIC_REPRESENTATION_ITEM ( )  RATIONAL_B_SPLINE_CURVE ( ( 0.9330127018922194093, 0.9330127018922207416, 1.000000000000000000, 0.8660254037844387076, 1.000000000000000000, 0.8660254037844387076, 1.000000000000000000, 0.9330127018922194093, 0.9330127018922194093 ) ) 
 REPRESENTATION_ITEM ( '' )  );
#58447=CYLINDRICAL_SURFACE ( 'NONE', #67724, 17.82106496071139645 ) ;
#58448=CARTESIAN_POINT ( 'NONE',  ( 43.17879721251643588, 204.9244531367911293, -4.594050593750046652 ) ) ;
#58449=CARTESIAN_POINT ( 'NONE',  ( 83.57553417992782840, 232.3927522451419350, 2.944929066748280225E-16 ) ) ;
#58450=VERTEX_POINT ( 'NONE', #39561 ) ;
#58451=CARTESIAN_POINT ( 'NONE',  ( 194.7794102799644520, 266.3152794235413126, -7.644990388705906526 ) ) ;
#58452=CARTESIAN_POINT ( 'NONE',  ( 179.5827521140122087, 259.6898873773316723, -10.31498942205267078 ) ) ;
#58453=CARTESIAN_POINT ( 'NONE',  ( 1.528821818964843482, 165.5643266524160140, 9.188101187500095079 ) ) ;
#58454=CARTESIAN_POINT ( 'NONE',  ( 198.6363782946250183, 286.5986958926748116, -18.50260615857378355 ) ) ;
#58456=CARTESIAN_POINT ( 'NONE',  ( 146.9978162861947908, 276.0393089210717790, -5.134868500856280882 ) ) ;
#58457=CARTESIAN_POINT ( 'NONE',  ( 163.7423057141168385, 247.0370024851108610, -6.909410042141566066 ) ) ;
#58458=CARTESIAN_POINT ( 'NONE',  ( 203.8087165842311776, 276.3139229654213409, 13.33924813713301738 ) ) ;
#58460=CARTESIAN_POINT ( 'NONE',  ( 207.6628070930962906, 270.9644626028195376, 7.378217122120054761 ) ) ;
#58462=ORIENTED_EDGE ( 'NONE', *, *, #48245, .F. ) ;
#58464=CARTESIAN_POINT ( 'NONE',  ( -2.070769811622737766, 159.6115022471902023, -5.000000000000041744 ) ) ;
#58466=CARTESIAN_POINT ( 'NONE',  ( 123.7191597644692393, 251.4244531367911293, -4.594050593750046652 ) ) ;
#58468=CARTESIAN_POINT ( 'NONE',  ( 164.4939982559556029, 245.7350328109756390, 0.9880945281613151554 ) ) ;
#58469=CARTESIAN_POINT ( 'NONE',  ( 178.3571982967953602, 292.6181790745828835, -7.174879954037646002 ) ) ;
#58470=CARTESIAN_POINT ( 'NONE',  ( 157.7365441389748923, 257.4392866714015895, 18.13124212464487073 ) ) ;
#58473=ORIENTED_EDGE ( 'NONE', *, *, #79542, .F. ) ;
#58474=CARTESIAN_POINT ( 'NONE',  ( 151.3883635558152321, 268.4346579770563608, 15.44343517165679103 ) ) ;
#58475=FACE_OUTER_BOUND ( 'NONE', #35370, .T. ) ;
#58476=CARTESIAN_POINT ( 'NONE',  ( 190.6456776865061613, 300.0543483028657192, 3.690611039747805577 ) ) ;
#58477=CARTESIAN_POINT ( 'NONE',  ( 172.9246534260911972, 268.4856987155242791, -16.42706699595391484 ) ) ;
#58484=CARTESIAN_POINT ( 'NONE',  ( 197.4664967616869831, 271.4698837146752908, 12.07595270249984232 ) ) ;
#58486=CARTESIAN_POINT ( 'NONE',  ( 185.8122340750109913, 296.6774856835382934, 4.673344314135899680 ) ) ;
#58488=CARTESIAN_POINT ( 'NONE',  ( 148.4946753614456725, 273.9075993938183160, -8.034288511620331974 ) ) ;
#58490=CARTESIAN_POINT ( 'NONE',  ( 194.4892283647733109, 282.9810723741138645, 17.41623236043902523 ) ) ;
#58494=CYLINDRICAL_SURFACE ( 'NONE', #70851, 17.82106496071139645 ) ;
#58495=CARTESIAN_POINT ( 'NONE',  ( 194.3011251241114508, 294.1075746476782342, -14.76047579547631905 ) ) ;
#58496=CARTESIAN_POINT ( 'NONE',  ( 159.6022460529178488, 264.0598611018144766, -17.33694791066348273 ) ) ;
#58497=ORIENTED_EDGE ( 'NONE', *, *, #26525, .T. ) ;
#58504=CARTESIAN_POINT ( 'NONE',  ( 89.32180003184730310, 228.5024278399160949, 9.188101187500095079 ) ) ;
#58505=CARTESIAN_POINT ( 'NONE',  ( 202.9667708310126386, 279.0982360029344136, 16.24681954556558949 ) ) ;
#58507=CARTESIAN_POINT ( 'NONE',  ( 182.0653602573277396, 257.7337868896066198, -5.961595716692482227 ) ) ;
#58509=ADVANCED_FACE ( 'NONE', ( #19324 ), #66386, .T. ) ;
#58514=CARTESIAN_POINT ( 'NONE',  ( 192.6361035247282985, 294.0892689374524593, 14.43747539422717630 ) ) ;
#58516=CARTESIAN_POINT ( 'NONE',  ( 148.8636819117637629, 274.0699646975406836, 8.926834414297511344 ) ) ;
#58518=VERTEX_POINT ( 'NONE', #58279 ) ;
#58519=FACE_OUTER_BOUND ( 'NONE', #70515, .T. ) ;
#58521=CARTESIAN_POINT ( 'NONE',  ( 189.9342510962733002, 301.6712223341471031, 2.454586110798282039 ) ) ;
#58522=CARTESIAN_POINT ( 'NONE',  ( 172.6012549852709412, 290.2025030293380610, -5.021894074213228087 ) ) ;
#58525=CARTESIAN_POINT ( 'NONE',  ( 148.6720373546558847, 247.4548013555409796, -4.594050593750042211 ) ) ;
#58526=CARTESIAN_POINT ( 'NONE',  ( 167.6713749921846102, 266.7905464791912777, -17.76959288544986393 ) ) ;
#58530=ORIENTED_EDGE ( 'NONE', *, *, #15190, .T. ) ;
#58532=CARTESIAN_POINT ( 'NONE',  ( 203.5888533553347202, 271.6823068233347271, 9.589978014565568643 ) ) ;
#58535=FACE_OUTER_BOUND ( 'NONE', #75754, .T. ) ;
#58537=CARTESIAN_POINT ( 'NONE',  ( 156.6830332884052552, 279.5358271113678938, 7.481028761613042199 ) ) ;
#58538=CARTESIAN_POINT ( 'NONE',  ( 179.0685761320505947, 258.5468394390073286, -11.57600102548048149 ) ) ;
#58539=CARTESIAN_POINT ( 'NONE',  ( 192.7113383204448667, 292.2246753303537616, -14.48311065252534391 ) ) ;
#58546=ORIENTED_EDGE ( 'NONE', *, *, #54687, .T. ) ;
#58547=CARTESIAN_POINT ( 'NONE',  ( 161.8699203163502034, 276.4193623153122417, 12.82305117122160887 ) ) ;
#58549=EDGE_CURVE ( 'NONE', #54504, #11091, #59621, .T. ) ;
#58552=CARTESIAN_POINT ( 'NONE',  ( 190.8138402884741254, 300.1477291634665789, 4.037153726988762514 ) ) ;
#58555=CARTESIAN_POINT ( 'NONE',  ( 151.2546443255573934, 275.3395117651207897, -9.775857568146751220 ) ) ;
#58556=CARTESIAN_POINT ( 'NONE',  ( 200.6684024474820944, 268.3695016763517742, 6.063491142324016536 ) ) ;
#58557=ORIENTED_EDGE ( 'NONE', *, *, #94579, .F. ) ;
#58559=EDGE_LOOP ( 'NONE', ( #57882, #80523, #96057, #35342 ) ) ;
#58561=EDGE_CURVE ( 'NONE', #6222, #3083, #79055, .T. ) ;
#58563=EDGE_CURVE ( 'NONE', #16138, #64801, #16434, .T. ) ;
#58565=CARTESIAN_POINT ( 'NONE',  ( 153.1314981037513121, 265.4154603756023789, 17.73969815997475408 ) ) ;
#58567=CARTESIAN_POINT ( 'NONE',  ( 2.394847222749282079, 166.0643266524160140, -9.188101187500093303 ) ) ;
#58568=CARTESIAN_POINT ( 'NONE',  ( 110.8105760068962127, 222.5327760586659736, 1.948934522072303157E-15 ) ) ;
#58569=CARTESIAN_POINT ( 'NONE',  ( 186.1630411436486554, 296.9614825196608194, -7.488375694256206749 ) ) ;
#58570=CARTESIAN_POINT ( 'NONE',  ( -12.91644128716779072, 174.8967562850347406, 1.347971487989956912E-14 ) ) ;
#58571=B_SPLINE_CURVE_WITH_KNOTS ( 'NONE', 3,
 ( #49006, #71818, #94135, #11019, #79940, #48507, #72829, #40872, #31777, #2415, #41383, #39866, #72323, #9514, #95656, #26205, #78926, #40377, #71315, #63698, #62680, #24200, #86067, #16593, #47489, #78414, #34296, #26698, #96140, #88557, #19123, #42376, #57583, #65195, #49997, #80954, #11520, #3422, #53204, #85663, #46584, #22806, #60776, #62280, #92735, #69403, #83653, #7600 ),
 .UNSPECIFIED., .F., .F.,
 ( 4, 2, 2, 2, 2, 2, 2, 2, 2, 2, 2, 2, 2, 2, 2, 2, 2, 2, 2, 2, 2, 2, 2, 4 ),
 ( 0.001558436884926003851, 0.002019628477514530829, 0.002480820070103058241, 0.002711415866397258196, 0.002826713764544444910, 0.002942011662691631189, 0.003057309560838817469, 0.003172607458986004183, 0.003403203255280448300, 0.003864394847869302707, 0.004325586440458157114, 0.005247969625635865928, 0.006170352810813574743, 0.006631544403402352822, 0.007092735995991130034, 0.007208033894138404785, 0.007265682843212073819, 0.007323331792285742853, 0.007438629690433081788, 0.007553927588580421591, 0.008015119181169766058, 0.008476310773759109657, 0.008706906570053764977, 0.008937502366348420296 ),
 .UNSPECIFIED. ) ;
#58573=DIRECTION ( 'NONE',  ( -0.8660254037844387076, -0.4999999999999998890, -0.000000000000000000 ) ) ;
#58575=CARTESIAN_POINT ( 'NONE',  ( 194.9220242159064185, 293.0321458743159724, -14.92681063007793263 ) ) ;
#58579=CARTESIAN_POINT ( 'NONE',  ( 176.0835288146691369, 265.6135182482621531, -15.96225161722567698 ) ) ;
#58581=CARTESIAN_POINT ( 'NONE',  ( 82.06918437091763963, 212.0643266524160140, 9.188101187500095079 ) ) ;
#58582=FACE_OUTER_BOUND ( 'NONE', #12476, .T. ) ;
#58584=CARTESIAN_POINT ( 'NONE',  ( 157.1338510812060747, 258.4831816688264325, 17.88958125218800888 ) ) ;
#58587=CARTESIAN_POINT ( 'NONE',  ( 204.6350011963004647, 275.7068757420208271, -12.64342396695018245 ) ) ;
#58589=CARTESIAN_POINT ( 'NONE',  ( 147.5118896528469179, 275.1489077312122049, -3.975523961781759930 ) ) ;
#58590=CARTESIAN_POINT ( 'NONE',  ( 134.4004000680750437, 241.7365022471901739, -10.00000000000009237 ) ) ;
#58591=EDGE_LOOP ( 'NONE', ( #20438, #33945, #35361, #13057 ) ) ;
#58595=CARTESIAN_POINT ( 'NONE',  ( 54.74956561180287196, 213.9637435831425307, 2.679491924311251605 ) ) ;
#58596=ORIENTED_EDGE ( 'NONE', *, *, #7089, .T. ) ;
#58598=CARTESIAN_POINT ( 'NONE',  ( 157.6629252921874240, 268.6179840388248863, 15.76425181776533790 ) ) ;
#58600=CARTESIAN_POINT ( 'NONE',  ( 129.9259354818553618, 252.4865022471903160, 10.00000000000009237 ) ) ;
#58601=CARTESIAN_POINT ( 'NONE',  ( 157.8820657059571033, 257.1872359237914338, -17.60412210594719440 ) ) ;
#58605=CARTESIAN_POINT ( 'NONE',  ( 166.6303123248438851, 247.5856509766914257, -1.864895467279636954 ) ) ;
#58607=CYLINDRICAL_SURFACE ( 'NONE', #20779, 10.00000000000010658 ) ;
#58614=CARTESIAN_POINT ( 'NONE',  ( 205.6265063320869899, 274.4914389803786321, 12.09149883072402432 ) ) ;
#58621=CARTESIAN_POINT ( 'NONE',  ( 61.87308422990769685, 194.9824982072973683, 3.021315404115420679E-15 ) ) ;
#58624=ADVANCED_FACE ( 'NONE', ( #68372 ), #12586, .F. ) ;
#58625=ORIENTED_EDGE ( 'NONE', *, *, #20019, .F. ) ;
#58626=ORIENTED_EDGE ( 'NONE', *, *, #95172, .T. ) ;
#58629=CARTESIAN_POINT ( 'NONE',  ( 204.5730103890532519, 276.3161474792809145, 14.88139715235883109 ) ) ;
#58630=CARTESIAN_POINT ( 'NONE',  ( 147.8505793332463725, 274.5622799967613332, -9.317516487097901035 ) ) ;
#58632=CARTESIAN_POINT ( 'NONE',  ( 156.6812872898450735, 261.2670451491295012, 0.000000000000000000 ) ) ;
#58633=CARTESIAN_POINT ( 'NONE',  ( 147.7487589314264653, 276.5474923016458888, 0.9592504414694114079 ) ) ;
#58635=CARTESIAN_POINT ( 'NONE',  ( 181.3346534254663140, 271.3440730695800767, -17.45372068697093226 ) ) ;
#58638=VERTEX_POINT ( 'NONE', #10083 ) ;
#58641=CARTESIAN_POINT ( 'NONE',  ( 166.1101521600732269, 277.8106941408184412, -13.38614590722673903 ) ) ;
#58643=CIRCLE ( 'NONE', #87873, 17.82106496071138224 ) ;
#58650=CARTESIAN_POINT ( 'NONE',  ( 195.6974783896144174, 291.6890198465123945, 16.70600479393688431 ) ) ;
#58651=CARTESIAN_POINT ( 'NONE',  ( 160.5099781893591455, 258.1706592185460067, -17.21824937912870013 ) ) ;
#58652=DIRECTION ( 'NONE',  ( -0.9659258262890649815, 0.2588190451025335070, 8.659560562355099259E-17 ) ) ;
#58653=ORIENTED_EDGE ( 'NONE', *, *, #41874, .F. ) ;
#58654=ORIENTED_EDGE ( 'NONE', *, *, #28918, .T. ) ;
#58659=CARTESIAN_POINT ( 'NONE',  ( 165.9969153545198708, 246.1123342570000716, -1.176638740111072723 ) ) ;
#58660=CARTESIAN_POINT ( 'NONE',  ( 153.3625104204072613, 266.6599839071155884, 16.46888835387834860 ) ) ;
#58662=CARTESIAN_POINT ( 'NONE',  ( 131.1078728602114722, 240.3768266524160424, 9.188101187500098632 ) ) ;
#58666=CARTESIAN_POINT ( 'NONE',  ( 205.0722772166587902, 275.4513919673344731, 14.18415804594472185 ) ) ;
#58671=CARTESIAN_POINT ( 'NONE',  ( 178.4342578914419732, 285.3753072366883430, 13.06730828328389649 ) ) ;
#58673=CARTESIAN_POINT ( 'NONE',  ( 195.4363368379034966, 279.6451395730842364, -17.08598955341190262 ) ) ;
#58674=CARTESIAN_POINT ( 'NONE',  ( 157.0239713899953244, 269.7369771206523978, 16.31777668093047851 ) ) ;
#58676=CARTESIAN_POINT ( 'NONE',  ( -22.42236680055709641, 157.8615022471902591, 0.000000000000000000 ) ) ;
#58679=CARTESIAN_POINT ( 'NONE',  ( 207.8136982414359579, 270.7031114674828700, -0.9536989003868096004 ) ) ;
#58690=CARTESIAN_POINT ( 'NONE',  ( 161.1093323826042933, 251.5974460702646809, -13.93502574894237078 ) ) ;
#58691=CARTESIAN_POINT ( 'NONE',  ( 13.46382118881039602, 169.3923013555410080, 4.594050593750050204 ) ) ;
#58698=CARTESIAN_POINT ( 'NONE',  ( 46.91405240998433612, 188.7048013555409796, 4.594050593750051981 ) ) ;
#58701=CARTESIAN_POINT ( 'NONE',  ( 171.2125587931870427, 286.8147667620277161, 7.172632356338288773 ) ) ;
#58702=CARTESIAN_POINT ( 'NONE',  ( 146.8729474948188454, 276.2555880120147549, 3.934020695290606273 ) ) ;
#58704=CARTESIAN_POINT ( 'NONE',  ( 198.1292909865887566, 287.0949182644739039, 16.93298125210290550 ) ) ;
#58705=CARTESIAN_POINT ( 'NONE',  ( 146.5689048584090699, 276.7822053059436485, -0.4306668706573002492 ) ) ;
#58706=CARTESIAN_POINT ( 'NONE',  ( 179.3320168101770378, 276.6075631236466847, 16.30429811271319451 ) ) ;
#58707=CARTESIAN_POINT ( 'NONE',  ( 179.1186523009620544, 278.4480982664924795, -17.05943142709577387 ) ) ;
#58708=CARTESIAN_POINT ( 'NONE',  ( 148.4572820722141557, 276.8246940256113930, 2.891641560416912338 ) ) ;
#58709=CARTESIAN_POINT ( 'NONE',  ( 119.0307608796806278, 227.9824982072973683, 3.021315404115420679E-15 ) ) ;
#58711=DIRECTION ( 'NONE',  ( -0.8660254037844387076, -0.4999999999999998890, -0.000000000000000000 ) ) ;
#58712=CARTESIAN_POINT ( 'NONE',  ( 89.29491028763546012, 232.3615022471903160, 5.000000000000046185 ) ) ;
#58714=CARTESIAN_POINT ( 'NONE',  ( 161.6164657043237014, 267.7223936679948224, -17.07498630821350005 ) ) ;
#58716=CARTESIAN_POINT ( 'NONE',  ( 65.88516108981343677, 208.8458772461660544, 9.188101187500095079 ) ) ;
#58724=CARTESIAN_POINT ( 'NONE',  ( 164.8329445879545290, 245.1479605429143760, -2.955380775890217304 ) ) ;
#58729=CARTESIAN_POINT ( 'NONE',  ( 172.0805575621569687, 256.0411262410343625, 11.22366668844141202 ) ) ;
#58730=ORIENTED_EDGE ( 'NONE', *, *, #28700, .T. ) ;
#58733=CARTESIAN_POINT ( 'NONE',  ( 16.56913029798217352, 168.8262482093458061, 3.021315404115420679E-15 ) ) ;
#58737=CARTESIAN_POINT ( 'NONE',  ( 151.2057546125658973, 268.7509459446807227, 15.78031848731319187 ) ) ;
#58738=CARTESIAN_POINT ( 'NONE',  ( 159.6288139302610887, 254.1617792512662675, -15.32287760493869477 ) ) ;
#58739=B_SPLINE_CURVE_WITH_KNOTS ( 'NONE', 3,
 ( #78248, #71155, #8828, #63529 ),
 .UNSPECIFIED., .F., .F.,
 ( 4, 4 ),
 ( 0.000000000000000000, 0.004615008360511261773 ),
 .UNSPECIFIED. ) ;
#58742=ORIENTED_EDGE ( 'NONE', *, *, #81639, .T. ) ;
#58743=CARTESIAN_POINT ( 'NONE',  ( 207.4541616930702617, 271.3258470364304458, -6.834942797545373594 ) ) ;
#58745=CARTESIAN_POINT ( 'NONE',  ( 148.9322735291567597, 272.6887306911919495, -12.40988026045598858 ) ) ;
#58749=CARTESIAN_POINT ( 'NONE',  ( 159.2077906806335932, 254.8910129107889588, 16.14624949541834553 ) ) ;
#58753=CARTESIAN_POINT ( 'NONE',  ( 121.5276403787286341, 228.7202760586659736, -5.415160957724236172E-17 ) ) ;
#58755=CYLINDRICAL_SURFACE ( 'NONE', #15686, 10.00000000000010658 ) ;
#58756=CARTESIAN_POINT ( 'NONE',  ( 107.4814437671086580, 242.8615022471903160, 5.000000000000046185 ) ) ;
#58758=CARTESIAN_POINT ( 'NONE',  ( 207.5570596878370679, 271.1476224814971374, 2.444960520848353358 ) ) ;
#58763=CARTESIAN_POINT ( 'NONE',  ( 68.53719034102077501, 216.5024278399160664, 9.188101187500095079 ) ) ;
#58766=CARTESIAN_POINT ( 'NONE',  ( 198.6455782124543248, 286.5827611675690605, 17.19551065434971093 ) ) ;
#58768=ORIENTED_EDGE ( 'NONE', *, *, #50081, .T. ) ;
#58770=CARTESIAN_POINT ( 'NONE',  ( 201.4520623681621316, 281.7217880192456505, -17.56577389517433119 ) ) ;
#58771=CARTESIAN_POINT ( 'NONE',  ( 155.4661767250933622, 261.3716783840932294, -17.10192542004562810 ) ) ;
#58773=CARTESIAN_POINT ( 'NONE',  ( 185.4867332780130766, 297.4061142773095412, 5.671143563000668131 ) ) ;
#58774=CARTESIAN_POINT ( 'NONE',  ( 161.3145230519951951, 251.2420454056404822, -14.44869077440025151 ) ) ;
#58775=CARTESIAN_POINT ( 'NONE',  ( 146.9422184197532317, 276.1356072505412840, -5.063317562214876943 ) ) ;
#58776=CARTESIAN_POINT ( 'NONE',  ( 59.32682287396359300, 198.3927522451418213, 10.00000000000009948 ) ) ;
#58777=CARTESIAN_POINT ( 'NONE',  ( 164.9103019330012216, 245.0139736909548560, 2.841678961959298810 ) ) ;
#58779=CARTESIAN_POINT ( 'NONE',  ( 208.1757572214753793, 270.0760069187178374, 2.172546422564154867 ) ) ;
#58780=B_SPLINE_CURVE_WITH_KNOTS ( 'NONE', 3,
 ( #11951, #28128, #67622, #66133 ),
 .UNSPECIFIED., .F., .F.,
 ( 4, 4 ),
 ( 0.04223839839039728733, 0.04887120950165271815 ),
 .UNSPECIFIED. ) ;
#58781=CARTESIAN_POINT ( 'NONE',  ( 126.3172359758225554, 252.9244531367911293, -4.594050593750046652 ) ) ;
#58785=CARTESIAN_POINT ( 'NONE',  ( 203.2732885619977026, 278.5673317194472247, -16.64305493556850024 ) ) ;
#58788=DIRECTION ( 'NONE',  ( 0.4999999999999998890, -0.8660254037844385966, 0.000000000000000000 ) ) ;
#58795=CARTESIAN_POINT ( 'NONE',  ( 38.03703169759616287, 182.7677522451417929, -5.000000000000041744 ) ) ;
#58796=CARTESIAN_POINT ( 'NONE',  ( 202.6334567748964730, 267.3808444593984746, 0.8764476327814421097 ) ) ;
#58797=CARTESIAN_POINT ( 'NONE',  ( 196.2953682204578456, 263.5854184417236752, 0.8810977108677261471 ) ) ;
#58799=CARTESIAN_POINT ( 'NONE',  ( 147.4317198359019301, 275.2877659273946733, 3.797273160043843188 ) ) ;
#58801=ADVANCED_FACE ( 'NONE', ( #66273 ), #82525, .T. ) ;
#58802=CARTESIAN_POINT ( 'NONE',  ( 204.6475128369918082, 276.1871054541632020, -13.72068618491070779 ) ) ;
#58803=CARTESIAN_POINT ( 'NONE',  ( 170.6625046707854665, 250.4727288339191773, 3.630827311776036570 ) ) ;
#58805=CARTESIAN_POINT ( 'NONE',  ( 190.0226014859668453, 301.5181949703289774, 3.835066345245774500 ) ) ;
#58808=CARTESIAN_POINT ( 'NONE',  ( 203.1044072055706806, 278.8598428092302584, -16.67109798570195878 ) ) ;
#58810=CARTESIAN_POINT ( 'NONE',  ( 132.9389821956408184, 260.8927522451419918, 2.944929066748280225E-16 ) ) ;
#58811=CARTESIAN_POINT ( 'NONE',  ( 175.4000927154525584, 286.5048389028432894, -12.54572841542827710 ) ) ;
#58812=ORIENTED_EDGE ( 'NONE', *, *, #6405, .T. ) ;
#58814=CARTESIAN_POINT ( 'NONE',  ( 196.2255671652529259, 290.7743432561995860, 16.01325193769018185 ) ) ;
#58815=CARTESIAN_POINT ( 'NONE',  ( 151.4376533647338476, 268.3492855237141725, -15.16853828792834236 ) ) ;
#58816=CARTESIAN_POINT ( 'NONE',  ( -2.963858511049441979, 169.0958772461660544, -9.188101187500095079 ) ) ;
#58817=CARTESIAN_POINT ( 'NONE',  ( 54.00411475982191689, 211.1744531367911293, 4.594050593750047540 ) ) ;
#58818=CARTESIAN_POINT ( 'NONE',  ( 178.9106358762607272, 258.8247338180944439, -11.56834183610952316 ) ) ;
#58821=CARTESIAN_POINT ( 'NONE',  ( 205.2391015854675516, 275.1624436846170738, -14.01434138479280911 ) ) ;
#58824=CARTESIAN_POINT ( 'NONE',  ( 167.9782759209660128, 256.7986816940351105, 13.70024866366997962 ) ) ;
#58825=CARTESIAN_POINT ( 'NONE',  ( 62.79092448910127189, 220.3927522451419350, 2.944929066748280225E-16 ) ) ;
#58826=CARTESIAN_POINT ( 'NONE',  ( 179.4461805389133531, 254.8738420869291019, -4.069619891950734036 ) ) ;
#58827=CARTESIAN_POINT ( 'NONE',  ( 198.4383541551818553, 286.9416837633153250, 16.97133247567711578 ) ) ;
#58828=CARTESIAN_POINT ( 'NONE',  ( 55.59208832369112230, 196.2365022471902023, 10.00000000000009592 ) ) ;
#58829=DIRECTION ( 'NONE',  ( -0.8660254037844387076, -0.4999999999999998890, -0.000000000000000000 ) ) ;
#58830=CARTESIAN_POINT ( 'NONE',  ( 147.6220714307702622, 274.9580672937808572, 8.392894244419288441 ) ) ;
#58831=CARTESIAN_POINT ( 'NONE',  ( 16.25090658753528317, 186.3149278399161233, 9.188101187500093303 ) ) ;
#58835=CARTESIAN_POINT ( 'NONE',  ( 159.8896510172052103, 272.0516993742419345, 16.05765770493651701 ) ) ;
#58836=CARTESIAN_POINT ( 'NONE',  ( 181.2600193737777374, 277.7392251741971450, 16.38192420661602711 ) ) ;
#58840=CARTESIAN_POINT ( 'NONE',  ( 164.9538401224995425, 286.5040288536138746, -0.08628193082933090230 ) ) ;
#58841=DIRECTION ( 'NONE',  ( -0.8660254037844387076, -0.4999999999999998890, -0.000000000000000000 ) ) ;
#58842=CARTESIAN_POINT ( 'NONE',  ( 183.6964659824695332, 271.1858650112955615, -17.13366558732818135 ) ) ;
#58849=CARTESIAN_POINT ( 'NONE',  ( 192.7693357657653053, 296.7607116428271183, 12.22606306887835714 ) ) ;
#58852=CARTESIAN_POINT ( 'NONE',  ( 202.7754741559590173, 279.4295715634463022, -15.65855077192107636 ) ) ;
#58853=AXIS2_PLACEMENT_3D ( 'NONE', #18784, #50654, #80620 ) ;
#58856=CYLINDRICAL_SURFACE ( 'NONE', #55132, 10.00000000000010658 ) ;
#58857=CARTESIAN_POINT ( 'NONE',  ( 163.9587364689194260, 246.6621334214722481, 5.816126667419880825 ) ) ;
#58858=CARTESIAN_POINT ( 'NONE',  ( 152.8107382695299918, 265.9710327055011589, 16.32045346488711246 ) ) ;
#58862=CARTESIAN_POINT ( 'NONE',  ( 174.8371417102094370, 262.4333147357459666, 14.35597617782233471 ) ) ;
#58866=CARTESIAN_POINT ( 'NONE',  ( 164.5139018292655919, 259.6662038739244736, -17.01387605652571366 ) ) ;
#58868=CARTESIAN_POINT ( 'NONE',  ( 149.7200635338602410, 271.3242383773507527, -12.12223662813266500 ) ) ;
#58870=DIRECTION ( 'NONE',  ( 0.5000000000000048850, -0.8660254037844358210, 0.000000000000000000 ) ) ;
#58871=CARTESIAN_POINT ( 'NONE',  ( 164.2545401858843945, 246.1497863546213978, 2.275217130759496609 ) ) ;
#58875=CARTESIAN_POINT ( 'NONE',  ( 190.0896302098338424, 301.4020978150248311, 3.433521196325825642 ) ) ;
#58876=CARTESIAN_POINT ( 'NONE',  ( 172.1455357562699362, 263.5618832647229510, -15.46582821167986488 ) ) ;
#58879=ORIENTED_EDGE ( 'NONE', *, *, #1124, .F. ) ;
#58880=CARTESIAN_POINT ( 'NONE',  ( 157.7063754007213845, 268.8955880366740416, 15.63381455156026867 ) ) ;
#58881=ORIENTED_EDGE ( 'NONE', *, *, #13818, .F. ) ;
#58882=CARTESIAN_POINT ( 'NONE',  ( 156.5028614784543208, 266.9798413144324059, -16.21780324415792762 ) ) ;
#58884=CARTESIAN_POINT ( 'NONE',  ( -7.720288864461156919, 177.8967562850347122, -4.648177544792955347E-16 ) ) ;
#58886=CARTESIAN_POINT ( 'NONE',  ( 192.7693357657653053, 296.7607116428271183, 12.22606306887835714 ) ) ;
#58888=CARTESIAN_POINT ( 'NONE',  ( 158.7310127332570460, 255.7168165395733581, -16.04306221441551017 ) ) ;
#58891=CARTESIAN_POINT ( 'NONE',  ( 165.0538309624641613, 244.7653741195639157, 2.311334310144196547 ) ) ;
#58894=CARTESIAN_POINT ( 'NONE',  ( 190.4556184745922280, 300.2183394804145564, 2.916409228186030322 ) ) ;
#58895=B_SPLINE_CURVE_WITH_KNOTS ( 'NONE', 3,
 ( #86049, #48990, #56055, #71299 ),
 .UNSPECIFIED., .F., .F.,
 ( 4, 4 ),
 ( 0.01127661141674762141, 0.01717785629562665339 ),
 .UNSPECIFIED. ) ;
#58896=CARTESIAN_POINT ( 'NONE',  ( 176.5821120313724464, 290.0546866683789062, -9.551980326619117889 ) ) ;
#58897=ORIENTED_EDGE ( 'NONE', *, *, #9246, .T. ) ;
#58899=CARTESIAN_POINT ( 'NONE',  ( 197.8666518381295987, 272.7614078478216015, 14.30677244657330860 ) ) ;
#58900=CARTESIAN_POINT ( 'NONE',  ( 193.8003511027313550, 288.1208047801705447, 17.19107869180001913 ) ) ;
#58901=CARTESIAN_POINT ( 'NONE',  ( 198.7680848198567674, 286.3705734992850580, -17.20718207227004015 ) ) ;
#58902=CARTESIAN_POINT ( 'NONE',  ( 102.1896198688571644, 218.2592609112380160, 2.679491924311254714 ) ) ;
#58904=CARTESIAN_POINT ( 'NONE',  ( 170.5267406923843510, 255.5323226702545583, -11.62603975033689352 ) ) ;
#58906=B_SPLINE_CURVE_WITH_KNOTS ( 'NONE', 3,
 ( #2818, #56975, #87961, #49891, #86955, #25600, #56486, #18505, #87474, #65088, #26600, #57474, #88457, #19016, #51890, #5778, #52374, #74214, #36666, #29580, #12403, #67574, #82831, #75693, #21009, #35686, #98506, #13399, #44271, #89924, #50879, #51375, #4804, #75201, #82343, #12911, #42764, #59456, #66587, #59962, #83317, #37174, #43268, #97997, #60457, #67074 ),
 .UNSPECIFIED., .F., .F.,
 ( 4, 2, 2, 2, 2, 2, 2, 2, 2, 2, 2, 2, 2, 2, 2, 2, 2, 2, 2, 2, 2, 2, 4 ),
 ( 0.002536418406735530592, 0.002949603472297969257, 0.003156196005079241716, 0.003259492271469948202, 0.003362788537860654688, 0.003466084804251361607, 0.003569381070642068526, 0.003775973603423508820, 0.004189158668986388973, 0.005015528800112283719, 0.005841898931238180201, 0.006668269062364074948, 0.007081454127926947728, 0.007494639193489818774, 0.007597935459880630210, 0.007649583593076001234, 0.007701231726271372258, 0.007804527992662112570, 0.007907824259052854618, 0.008321009324615878319, 0.008734194390178900286, 0.008940786922960408667, 0.009147379455741920518 ),
 .UNSPECIFIED. ) ;
#58907=CARTESIAN_POINT ( 'NONE',  ( 201.3505934466285510, 281.8975373467312693, -16.83770227898004279 ) ) ;
#58908=CARTESIAN_POINT ( 'NONE',  ( 155.3874097416376969, 262.7157056314985653, 17.32087637530853641 ) ) ;
#58909=CARTESIAN_POINT ( 'NONE',  ( 26.41785753015485128, 199.3927522451419634, 2.944929066748280225E-16 ) ) ;
#58910=CARTESIAN_POINT ( 'NONE',  ( 112.3797264076079756, 241.8149278399160949, 9.188101187500093303 ) ) ;
#58912=CARTESIAN_POINT ( 'NONE',  ( 164.1420675163463159, 280.3382853379264930, -11.37976142735245588 ) ) ;
#58914=CARTESIAN_POINT ( 'NONE',  ( 33.95012722949724093, 202.6589784336661637, -6.496448406907675876E-16 ) ) ;
#58916=CARTESIAN_POINT ( 'NONE',  ( 200.7523954295751594, 282.9336467052548869, 18.23634913067694185 ) ) ;
#58917=VERTEX_POINT ( 'NONE', #18683 ) ;
#58919=CARTESIAN_POINT ( 'NONE',  ( 190.3268461984029614, 299.2279209427761657, 7.463966244697216368 ) ) ;
#58920=CARTESIAN_POINT ( 'NONE',  ( 185.8237621104296409, 258.7144012905565660, -5.701851391998975949 ) ) ;
#58921=CARTESIAN_POINT ( 'NONE',  ( 20.28351092001508960, 192.5177522451419350, 5.000000000000046185 ) ) ;
#58922=CARTESIAN_POINT ( 'NONE',  ( 101.6898988757523625, 229.5177522451418781, -10.00000000000009592 ) ) ;
#58925=FACE_OUTER_BOUND ( 'NONE', #1847, .T. ) ;
#58926=CARTESIAN_POINT ( 'NONE',  ( 96.56591523669446531, 219.8927522451417929, -10.00000000000009059 ) ) ;
#58928=EDGE_CURVE ( 'NONE', #84360, #65090, #18575, .T. ) ;
#58929=CARTESIAN_POINT ( 'NONE',  ( 194.8412596780180763, 266.4128482819364194, -7.732926466646180330 ) ) ;
#58930=CARTESIAN_POINT ( 'NONE',  ( 202.6560281492536717, 279.6364581158209717, 17.15553667345918853 ) ) ;
#58931=CARTESIAN_POINT ( 'NONE',  ( 162.6341128535665064, 248.9564488241690299, -10.63508949045170660 ) ) ;
#58932=CARTESIAN_POINT ( 'NONE',  ( 15.03297158952216961, 188.6744531367911293, 4.594050593750047540 ) ) ;
#58933=CARTESIAN_POINT ( 'NONE',  ( 150.8168331730346949, 269.4245776381016526, -15.71017957295074652 ) ) ;
#58937=CARTESIAN_POINT ( 'NONE',  ( 50.97302584657637681, 209.4244531367911577, -4.594050593750046652 ) ) ;
#58938=CARTESIAN_POINT ( 'NONE',  ( 164.2090401137261892, 246.2285947913476889, -5.787448100099915393 ) ) ;
#58941=CARTESIAN_POINT ( 'NONE',  ( 165.0387478276132072, 244.7914988754632191, -2.473354058663827626 ) ) ;
#58942=EDGE_CURVE ( 'NONE', #4112, #44171, #6535, .T. ) ;
#58943=ORIENTED_EDGE ( 'NONE', *, *, #15160, .T. ) ;
#58944=CARTESIAN_POINT ( 'NONE',  ( 10.91961124514384274, 167.1115022471901739, -5.000000000000041744 ) ) ;
#58946=CARTESIAN_POINT ( 'NONE',  ( 131.4326323866306439, 240.5643266524160140, 9.188101187500095079 ) ) ;
#58948=CARTESIAN_POINT ( 'NONE',  ( 206.9515461683482442, 272.1964026619218089, -8.225306050385031043 ) ) ;
#58949=CARTESIAN_POINT ( 'NONE',  ( 188.6377010289637326, 260.8445305228526649, 6.834932301962454382 ) ) ;
#58951=CARTESIAN_POINT ( 'NONE',  ( 196.2048238403250764, 290.8102717488927169, 17.53926796892840656 ) ) ;
#58955=CARTESIAN_POINT ( 'NONE',  ( 150.6533415055477008, 269.7077535128032082, 14.84621632544246062 ) ) ;
#58956=CARTESIAN_POINT ( 'NONE',  ( 207.6123412471599181, 271.0518720120282978, -1.072722343106485843 ) ) ;
#58957=CARTESIAN_POINT ( 'NONE',  ( 178.6423073663378602, 290.9544255387157818, 10.03153667033594765 ) ) ;
#58958=CARTESIAN_POINT ( 'NONE',  ( 171.9228082726160096, 267.5004681726649096, -16.35366899046682221 ) ) ;
#58959=CARTESIAN_POINT ( 'NONE',  ( 194.2019594945463723, 271.1902707947111253, -13.60880440021994531 ) ) ;
#58961=DIRECTION ( 'NONE',  ( 0.5000000000000003331, -0.8660254037844384856, 0.000000000000000000 ) ) ;
#58967=CARTESIAN_POINT ( 'NONE',  ( 196.2073114852891536, 270.9366426346837784, 12.15079365960697544 ) ) ;
#58968=CARTESIAN_POINT ( 'NONE',  ( 181.9118032920808616, 295.3731262585166064, 4.899329891614067733 ) ) ;
#58970=CARTESIAN_POINT ( 'NONE',  ( 150.8122822842734934, 278.1341709827950126, -0.0002939758904230073302 ) ) ;
#58972=B_SPLINE_CURVE_WITH_KNOTS ( 'NONE', 3,
 ( #30606, #45297, #14891, #60987 ),
 .UNSPECIFIED., .F., .F.,
 ( 4, 4 ),
 ( 0.009279588375480398582, 0.01508950711662758459 ),
 .UNSPECIFIED. ) ;
#58974=CARTESIAN_POINT ( 'NONE',  ( 95.64807497750081211, 214.4824982072973683, 3.021315404115420679E-15 ) ) ;
#58975=VERTEX_POINT ( 'NONE', #99672 ) ;
#58978=CARTESIAN_POINT ( 'NONE',  ( 159.0121568112382988, 263.7050002963263182, -17.11747536930247549 ) ) ;
#58979=ORIENTED_EDGE ( 'NONE', *, *, #89920, .T. ) ;
#58980=CARTESIAN_POINT ( 'NONE',  ( 191.1000148935602567, 299.6520602076213891, -9.462302242170249400 ) ) ;
#58982=CARTESIAN_POINT ( 'NONE',  ( 184.8121857201937530, 292.0935771287341254, 12.40013839118309491 ) ) ;
#58983=CARTESIAN_POINT ( 'NONE',  ( 164.4272222519600746, 245.8506922426221593, 7.021336339662529902 ) ) ;
#58984=CARTESIAN_POINT ( 'NONE',  ( 160.9738207889920716, 284.1303138127853458, -2.465274816821101833 ) ) ;
#58985=CARTESIAN_POINT ( 'NONE',  ( -22.42236680055709641, 157.8615022471902591, 0.000000000000000000 ) ) ;
#58986=ORIENTED_EDGE ( 'NONE', *, *, #46022, .F. ) ;
#58987=CARTESIAN_POINT ( 'NONE',  ( 86.64296780859545777, 211.6423013555409796, -4.594050593750043987 ) ) ;
#58988=CARTESIAN_POINT ( 'NONE',  ( 155.2816187818737603, 261.6913421186901587, 18.56800597028529509 ) ) ;
#58989=CARTESIAN_POINT ( 'NONE',  ( 181.1203783733027421, 271.7167412992034201, -16.96219288225206157 ) ) ;
#58990=CARTESIAN_POINT ( 'NONE',  ( 184.6166050049803289, 259.6725624253173237, -5.813182908278067273 ) ) ;
#58992=ORIENTED_EDGE ( 'NONE', *, *, #46941, .T. ) ;
#58993=ORIENTED_EDGE ( 'NONE', *, *, #28974, .T. ) ;
#58996=CARTESIAN_POINT ( 'NONE',  ( 137.5794118583994532, 267.3524639162450853, 0.000000000000000000 ) ) ;
#58998=ORIENTED_EDGE ( 'NONE', *, *, #64431, .T. ) ;
#58999=CARTESIAN_POINT ( 'NONE',  ( 202.5128468779458331, 267.1751508879428343, 0.8823122286173835649 ) ) ;
#59000=CARTESIAN_POINT ( 'NONE',  ( 155.6048174803203210, 261.1315455520403361, -17.38645169541727498 ) ) ;
#59001=ORIENTED_EDGE ( 'NONE', *, *, #95434, .T. ) ;
#59002=CARTESIAN_POINT ( 'NONE',  ( 164.9264240583707419, 244.9860493506886030, 2.333010560622383434 ) ) ;
#59003=FACE_OUTER_BOUND ( 'NONE', #36917, .T. ) ;
#59008=FACE_OUTER_BOUND ( 'NONE', #34585, .T. ) ;
#59013=CARTESIAN_POINT ( 'NONE',  ( 166.8837065285814845, 246.9778330270648041, 3.492974035202267125 ) ) ;
#59014=CARTESIAN_POINT ( 'NONE',  ( 199.9790510050489445, 270.1949291182149295, 9.285085457420754196 ) ) ;
#59015=B_SPLINE_CURVE_WITH_KNOTS ( 'NONE', 3,
 ( #20576, #61031, #44840, #83392, #60532, #5367, #74789, #67654, #45342, #13475, #84387, #98074, #52948, #13961, #98585, #28652, #43349, #59534, #91485, #22048, #53436, #74297, #83897, #4880, #90514, #35762, #52447, #29168, #66658, #21086, #99563, #44346, #60036, #6847, #37733, #68642, #97589, #21564, #92003, #28160, #25041, #62022, #1255, #40227, #55918, #32137, #38223, #93485, #46322, #14933 ),
 .UNSPECIFIED., .F., .F.,
 ( 4, 2, 2, 2, 2, 2, 2, 2, 2, 2, 2, 2, 2, 2, 2, 2, 2, 2, 2, 2, 2, 2, 2, 2, 4 ),
 ( 0.0002342349665180101781, 0.001258123135262355667, 0.001770067219634560490, 0.002026039261820688272, 0.002154025282913752271, 0.002282011304006816271, 0.002409997325099880270, 0.002537983346192944269, 0.002793955388379072268, 0.003305899472751457503, 0.004329787641496161618, 0.005353675810240866167, 0.005865619894613221912, 0.006121591936799440983, 0.006377563978985659188, 0.006441556989532238459, 0.006505550000078817729, 0.006569543010625396133, 0.006633536021171974537, 0.006889508063358473766, 0.007401452147731471358, 0.007657424189917910740, 0.007913396232104349254, 0.008169368274290789503, 0.008425340316477228017 ),
 .UNSPECIFIED. ) ;
#59016=CARTESIAN_POINT ( 'NONE',  ( -4.668846022976141263, 178.1115022471903160, -5.000000000000047962 ) ) ;
#59017=CARTESIAN_POINT ( 'NONE',  ( 202.7041331321765938, 279.5531378413010657, 17.14708438049711248 ) ) ;
#59018=CARTESIAN_POINT ( 'NONE',  ( 198.2505066714982149, 285.2670451491296149, 0.000000000000000000 ) ) ;
#59019=CARTESIAN_POINT ( 'NONE',  ( 158.6703588719639697, 280.1886327639391538, -6.711918335171482397 ) ) ;
#59021=CARTESIAN_POINT ( 'NONE',  ( 192.8135389063894820, 292.0478606184409500, -14.85096288738734671 ) ) ;
#59024=( BOUNDED_CURVE ( )  B_SPLINE_CURVE ( 2, ( #17336, #1151, #148, #77138, #93888, #31527, #62418, #55321, #40121 ),
 .UNSPECIFIED., .F., .T. ) 
 B_SPLINE_CURVE_WITH_KNOTS ( ( 3, 2, 2, 2, 3 ),
 ( 0.1572580645161290314, 0.1586021505376344065, 0.1612903225806451568, 0.1639784946236559071, 0.1653225806451612823 ),
 .UNSPECIFIED. ) 
 CURVE ( )  GEOMETRIC_REPRESENTATION_ITEM ( )  RATIONAL_B_SPLINE_CURVE ( ( 0.9330127018922194093, 0.9330127018922194093, 1.000000000000000000, 0.8660254037844387076, 1.000000000000000000, 0.8660254037844387076, 1.000000000000000000, 0.9330127018922194093, 0.9330127018922194093 ) ) 
 REPRESENTATION_ITEM ( '' )  );
#59026=CARTESIAN_POINT ( 'NONE',  ( 155.5450908721997791, 261.2349950718688660, -18.53705729126367530 ) ) ;
#59028=EDGE_LOOP ( 'NONE', ( #64497, #16200, #13581 ) ) ;
#59029=CARTESIAN_POINT ( 'NONE',  ( 163.4341025207368716, 282.8476932499685859, 9.116081536633066307 ) ) ;
#59032=CARTESIAN_POINT ( 'NONE',  ( 148.9230895364621574, 272.7046378331555161, 12.20434325797056019 ) ) ;
#59033=CARTESIAN_POINT ( 'NONE',  ( 164.4537261901595286, 274.3242769609400398, 14.76238940331070815 ) ) ;
#59038=CARTESIAN_POINT ( 'NONE',  ( -22.42236680055709641, 157.8615022471902591, 0.000000000000000000 ) ) ;
#59040=ORIENTED_EDGE ( 'NONE', *, *, #65121, .T. ) ;
#59042=CARTESIAN_POINT ( 'NONE',  ( 187.4955502139596888, 283.9325251962030734, -17.32086278988823125 ) ) ;
#59044=LINE ( 'NONE', #7225, #16021 ) ;
#59045=CARTESIAN_POINT ( 'NONE',  ( 175.2000473418449360, 291.7498890306831072, 3.463214443597544268 ) ) ;
#59048=CARTESIAN_POINT ( 'NONE',  ( 4.992923434102598534, 167.5643266524160140, -9.188101187500093303 ) ) ;
#59049=CARTESIAN_POINT ( 'NONE',  ( 100.4447270377624477, 237.9869531367911293, 4.594050593750046652 ) ) ;
#59051=CARTESIAN_POINT ( 'NONE',  ( 179.9270665230947657, 255.1929127066956937, -2.395391053091963762 ) ) ;
#59055=CARTESIAN_POINT ( 'NONE',  ( 155.2695601165254402, 261.7122283397445131, 16.98599069618989077 ) ) ;
#59056=CARTESIAN_POINT ( 'NONE',  ( 181.1390047055053287, 273.3328751412228144, 17.56653892176710130 ) ) ;
#59057=CARTESIAN_POINT ( 'NONE',  ( 148.3625667886952044, 273.6754917110858401, -8.960758510948144462 ) ) ;
#59060=CARTESIAN_POINT ( 'NONE',  ( 193.9296649147714788, 265.9040112472643500, 7.816750032855302344 ) ) ;
#59062=CARTESIAN_POINT ( 'NONE',  ( 58.31645990288170367, 211.1427522451419065, 10.00000000000009415 ) ) ;
#59064=VECTOR ( 'NONE', #34601, 1000.000000000000000 ) ;
#59065=CARTESIAN_POINT ( 'NONE',  ( 42.77981749017101976, 207.0530062829863311, -4.648177544792955347E-16 ) ) ;
#59067=CARTESIAN_POINT ( 'NONE',  ( 81.01380268399661588, 208.3923013555409796, 4.594050593750050204 ) ) ;
#59068=CARTESIAN_POINT ( 'NONE',  ( 161.8839333999304415, 250.2557977526613229, -13.90128376743482441 ) ) ;
#59069=( GEOMETRIC_REPRESENTATION_CONTEXT ( 3 ) GLOBAL_UNCERTAINTY_ASSIGNED_CONTEXT ( ( #32145 ) ) GLOBAL_UNIT_ASSIGNED_CONTEXT ( ( #88338, #72606, #94414 ) ) REPRESENTATION_CONTEXT ( 'NONE', 'WORKASPACE' ) );
#59070=CARTESIAN_POINT ( 'NONE',  ( 158.1254202985194581, 258.8215446263105832, -16.98779281373658989 ) ) ;
#59071=CARTESIAN_POINT ( 'NONE',  ( 157.5710319558766344, 257.7259621817996162, 18.28704422422941533 ) ) ;
#59072=CARTESIAN_POINT ( 'NONE',  ( 152.4345947225712621, 266.6225324397728400, 16.69537593800771091 ) ) ;
#59075=CARTESIAN_POINT ( 'NONE',  ( 173.1907548464488116, 268.0754673152154055, -16.28899667295896947 ) ) ;
#59077=CARTESIAN_POINT ( 'NONE',  ( 147.2089949622447875, 275.6735367246781720, -3.633014386235353221 ) ) ;
#59078=DIRECTION ( 'NONE',  ( -0.8660254037844387076, -0.4999999999999998890, -0.000000000000000000 ) ) ;
#59082=CARTESIAN_POINT ( 'NONE',  ( 147.0456760057551833, 275.9564134551570760, -3.678503029046952033 ) ) ;
#59083=CARTESIAN_POINT ( 'NONE',  ( 188.4945086955212901, 286.1460090028926402, -16.09362256013984194 ) ) ;
#59084=EDGE_CURVE ( 'NONE', #87476, #57035, #47609, .T. ) ;
#59088=CARTESIAN_POINT ( 'NONE',  ( 153.9489233572929834, 266.9981809298170106, 16.25793775942264219 ) ) ;
#59090=CARTESIAN_POINT ( 'NONE',  ( 146.0195742355162452, 245.1115022471902023, -5.000000000000041744 ) ) ;
#59091=CARTESIAN_POINT ( 'NONE',  ( 204.6149525604204769, 276.2435015074934199, -13.22810747389629960 ) ) ;
#59094=CARTESIAN_POINT ( 'NONE',  ( 88.62734903533704767, 228.6427522451418781, -10.00000000000009592 ) ) ;
#59095=ORIENTED_EDGE ( 'NONE', *, *, #37040, .F. ) ;
#59103=CARTESIAN_POINT ( 'NONE',  ( 206.0686240106620915, 273.7256686981625080, 10.79590858600826309 ) ) ;
#59104=CARTESIAN_POINT ( 'NONE',  ( 158.7005503356804752, 257.5255643194142863, -17.18125617848118480 ) ) ;
#59105=CARTESIAN_POINT ( 'NONE',  ( 153.7116827962181560, 264.4105510104763539, -18.11656053488752605 ) ) ;
#59106=CARTESIAN_POINT ( 'NONE',  ( 153.3544108199959908, 265.0293642254135307, -17.49105661178601423 ) ) ;
#59111=CARTESIAN_POINT ( 'NONE',  ( 166.1866365242245536, 275.3519730907532335, 14.78294132260052152 ) ) ;
#59113=ORIENTED_EDGE ( 'NONE', *, *, #24417, .F. ) ;
#59116=CARTESIAN_POINT ( 'NONE',  ( -27.42236680055714260, 166.5217562850347406, 1.224646799147364892E-15 ) ) ;
#59117=CARTESIAN_POINT ( 'NONE',  ( 194.2900850603946310, 294.1266965989547657, -15.88613936555681505 ) ) ;
#59122=CARTESIAN_POINT ( 'NONE',  ( 167.7492589498101268, 287.2853069970565230, -4.990612205622849906 ) ) ;
#59123=CARTESIAN_POINT ( 'NONE',  ( 167.0261895629188302, 265.8937476829661364, 16.54818857680643163 ) ) ;
#59124=CARTESIAN_POINT ( 'NONE',  ( 181.3894115369784572, 256.9812711509448491, 4.984939519295573440 ) ) ;
#59125=CARTESIAN_POINT ( 'NONE',  ( 89.61940949045693117, 231.7369531367911009, -4.594050593750048428 ) ) ;
#59127=CARTESIAN_POINT ( 'NONE',  ( 148.2529106943155455, 274.6458799743566033, -6.824415188474639571 ) ) ;
#59128=CARTESIAN_POINT ( 'NONE',  ( 189.7493380202622291, 294.8126471784881915, -12.68491631734921299 ) ) ;
#59129=CARTESIAN_POINT ( 'NONE',  ( 166.7606291933738021, 278.4628371803321443, -13.23787148276527681 ) ) ;
#59130=VERTEX_POINT ( 'NONE', #40334 ) ;
#59132=ORIENTED_EDGE ( 'NONE', *, *, #78233, .T. ) ;
#59134=CARTESIAN_POINT ( 'NONE',  ( 178.0175832155955220, 292.6799449813070169, -2.666636303287813092 ) ) ;
#59135=CARTESIAN_POINT ( 'NONE',  ( 157.0848929289108469, 258.5679796760466047, 17.57466231005294688 ) ) ;
#59136=CARTESIAN_POINT ( 'NONE',  ( 175.0125019719911847, 292.0719086349095051, 3.303583340955516423 ) ) ;
#59139=AXIS2_PLACEMENT_3D ( 'NONE', #32816, #16121, #94159 ) ;
#59141=CARTESIAN_POINT ( 'NONE',  ( 208.3764315856425640, 269.7284287242038658, -1.833640725398759441 ) ) ;
#59143=ADVANCED_FACE ( 'NONE', ( #58475 ), #20924, .F. ) ;
#59144=CARTESIAN_POINT ( 'NONE',  ( 191.7288270367013467, 263.6483701492742284, -8.196354403749188222 ) ) ;
#59145=CARTESIAN_POINT ( 'NONE',  ( -22.42236680055709641, 157.8615022471902591, 0.000000000000000000 ) ) ;
#59147=CARTESIAN_POINT ( 'NONE',  ( 133.7867050834633460, 257.2369531367911009, -4.594050593750048428 ) ) ;
#59149=DIRECTION ( 'NONE',  ( -0.8660254037844387076, -0.4999999999999998890, -0.000000000000000000 ) ) ;
#59150=ORIENTED_EDGE ( 'NONE', *, *, #91521, .F. ) ;
#59151=B_SPLINE_CURVE_WITH_KNOTS ( 'NONE', 3,
 ( #39805, #86007, #9955, #86501, #47430, #78357, #32234, #338, #94080, #63135, #24633, #32733, #78861, #40814, #71761, #31229, #62115, #55513 ),
 .UNSPECIFIED., .F., .F.,
 ( 4, 2, 2, 2, 2, 2, 2, 2, 4 ),
 ( 0.003355772174813248000, 0.003464747999639208008, 0.003573723824465168016, 0.003682699649291128023, 0.003791675474117088031, 0.004009627123769074833, 0.004227578773421060768, 0.005099385372029013180, 0.006842998569244833004 ),
 .UNSPECIFIED. ) ;
#59155=CARTESIAN_POINT ( 'NONE',  ( 192.7653315510534924, 271.1824743346560922, 14.22424966267575819 ) ) ;
#59156=CARTESIAN_POINT ( 'NONE',  ( 167.1866462610758788, 284.4963469294596621, 9.835208695640710985 ) ) ;
#59159=CARTESIAN_POINT ( 'NONE',  ( 136.3105610988903607, 261.0530062829863027, -4.648177544792955347E-16 ) ) ;
#59160=CARTESIAN_POINT ( 'NONE',  ( 183.3811779399601960, 287.6651436968118674, 15.08102091061752859 ) ) ;
#59162=CARTESIAN_POINT ( 'NONE',  ( 70.72975101405640430, 202.4548013555409796, -4.594050593750042211 ) ) ;
#59165=CARTESIAN_POINT ( 'NONE',  ( 162.6341128535665064, 248.9564488241690299, -10.63508949045170660 ) ) ;
#59171=EDGE_CURVE ( 'NONE', #93728, #2250, #14766, .T. ) ;
#59173=B_SPLINE_CURVE_WITH_KNOTS ( 'NONE', 3,
 ( #49653, #28345, #58249, #36439 ),
 .UNSPECIFIED., .F., .F.,
 ( 4, 4 ),
 ( 0.004312638717203288660, 0.01230371896665270748 ),
 .UNSPECIFIED. ) ;
#59179=CARTESIAN_POINT ( 'NONE',  ( 9.403806464923315289, 185.4244531367911293, -4.594050593750046652 ) ) ;
#59181=ORIENTED_EDGE ( 'NONE', *, *, #33966, .F. ) ;
#59182=CARTESIAN_POINT ( 'NONE',  ( 157.8849654228661166, 257.1822134667773980, 17.43614750057631468 ) ) ;
#59183=CARTESIAN_POINT ( 'NONE',  ( 199.2604132571903790, 277.9333477773519121, 15.74201777144865844 ) ) ;
#59184=CARTESIAN_POINT ( 'NONE',  ( 28.65277809448527080, 198.8967562850347122, -4.648177544792955347E-16 ) ) ;
#59185=CARTESIAN_POINT ( 'NONE',  ( 208.3057440179679531, 269.8508631828800617, 2.969924427282375046 ) ) ;
#59187=CARTESIAN_POINT ( 'NONE',  ( 57.30635725539759306, 194.7048013555409796, 4.594050593750051981 ) ) ;
#59188=CARTESIAN_POINT ( 'NONE',  ( 161.8948331661419218, 250.2369188037922356, 13.64419044796309777 ) ) ;
#59189=CARTESIAN_POINT ( 'NONE',  ( 198.9832789858017463, 285.9978462703757600, -18.55676541969546278 ) ) ;
#59190=CARTESIAN_POINT ( 'NONE',  ( 190.8683709797118411, 300.0532792356709706, -4.461919767133968762 ) ) ;
#59192=CARTESIAN_POINT ( 'NONE',  ( 159.8822213732012756, 255.7228646850775533, -16.63148941946954196 ) ) ;
#59193=CARTESIAN_POINT ( 'NONE',  ( 177.6444986370304946, 293.6980009803469329, 2.770296639708824227 ) ) ;
#59198=AXIS2_PLACEMENT_3D ( 'NONE', #903, #62684, #71319 ) ;
#59200=CARTESIAN_POINT ( 'NONE',  ( 97.08913892169542237, 236.8615022471903160, 5.000000000000046185 ) ) ;
#59203=CARTESIAN_POINT ( 'NONE',  ( 164.9009427471078766, 270.4319544559331234, -17.40525121274953335 ) ) ;
#59205=CARTESIAN_POINT ( 'NONE',  ( 67.69866210081085001, 200.7048013555409796, 4.594050593750051981 ) ) ;
#59207=CARTESIAN_POINT ( 'NONE',  ( 166.3615356672940777, 265.0576312756302286, 16.62332830971679698 ) ) ;
#59208=CARTESIAN_POINT ( 'NONE',  ( 147.5492216329511166, 275.0842468449245644, 4.751613690710122739 ) ) ;
#59209=CARTESIAN_POINT ( 'NONE',  ( 173.5247214620460738, 266.5572136672606689, 17.40638611211905484 ) ) ;
#59210=ORIENTED_EDGE ( 'NONE', *, *, #31427, .T. ) ;
#59212=CARTESIAN_POINT ( 'NONE',  ( 207.6508796976096107, 270.9851214578045528, 6.713685698622268383 ) ) ;
#59216=CARTESIAN_POINT ( 'NONE',  ( 189.7373781100581027, 264.4670991245342293, 10.92349686411582788 ) ) ;
#59217=CARTESIAN_POINT ( 'NONE',  ( 149.2923684163597784, 272.0650280510108701, -12.99082738998495756 ) ) ;
#59218=CARTESIAN_POINT ( 'NONE',  ( 204.3646970165318351, 276.6769568243839217, 14.33703115251539018 ) ) ;
#59222=CARTESIAN_POINT ( 'NONE',  ( 174.9566398689986499, 255.1230660018185574, 8.075064970304348222 ) ) ;
#59224=EDGE_CURVE ( 'NONE', #15171, #92056, #2865, .T. ) ;
#59226=CARTESIAN_POINT ( 'NONE',  ( 182.1243482512361709, 283.9946157055692879, 14.95652526196643883 ) ) ;
#59227=CARTESIAN_POINT ( 'NONE',  ( 191.2729698983822288, 299.3524933518466469, 8.871011392605806734 ) ) ;
#59228=CARTESIAN_POINT ( 'NONE',  ( 159.5221561062548972, 254.3465160214695118, -16.91023001054109542 ) ) ;
#59231=CARTESIAN_POINT ( 'NONE',  ( 161.4816992964961742, 250.9524876563463067, -12.92750327687364198 ) ) ;
#59233=CARTESIAN_POINT ( 'NONE',  ( 196.7130436017243653, 289.9300093007386749, -16.33278734947153765 ) ) ;
#59234=ORIENTED_EDGE ( 'NONE', *, *, #64057, .F. ) ;
#59237=DIRECTION ( 'NONE',  ( -0.4999999999999987788, 0.8660254037844392627, 0.000000000000000000 ) ) ;
#59238=CARTESIAN_POINT ( 'NONE',  ( 161.4611533925282458, 263.2350952187405255, -17.14425122640257726 ) ) ;
#59239=CARTESIAN_POINT ( 'NONE',  ( 123.3675972660055749, 242.0333772461660544, 9.188101187500095079 ) ) ;
#59240=CARTESIAN_POINT ( 'NONE',  ( 190.8623743139412454, 300.0636657654615647, 8.577953960666059530 ) ) ;
#59242=CARTESIAN_POINT ( 'NONE',  ( 170.5590276664972862, 263.8138381775597736, 15.82950496912112470 ) ) ;
#59243=CARTESIAN_POINT ( 'NONE',  ( 28.87159617421078295, 194.1427522451419350, -10.00000000000009592 ) ) ;
#59245=EDGE_LOOP ( 'NONE', ( #4204, #52015, #45798, #42935 ) ) ;
#59247=AXIS2_PLACEMENT_3D ( 'NONE', #13343, #20954, #44207 ) ;
#59249=VERTEX_POINT ( 'NONE', #72793 ) ;
#59250=CARTESIAN_POINT ( 'NONE',  ( 198.6012358295098750, 286.6595644277572887, 18.21911298807435386 ) ) ;
#59252=CARTESIAN_POINT ( 'NONE',  ( 85.15457341978220995, 207.7202760586659167, -5.415160957724236172E-17 ) ) ;
#59253=CARTESIAN_POINT ( 'NONE',  ( 173.8612121445452203, 290.1417140779839201, 6.947705100246971632 ) ) ;
#59255=CARTESIAN_POINT ( 'NONE',  ( 198.1857676047573307, 287.3791765019590798, 18.47549341984830562 ) ) ;
#59257=CARTESIAN_POINT ( 'NONE',  ( 171.9727612249948550, 276.6547058738756277, 16.01864781142220195 ) ) ;
#59258=ORIENTED_EDGE ( 'NONE', *, *, #38471, .F. ) ;
#59261=CARTESIAN_POINT ( 'NONE',  ( 201.4214977800931763, 281.7747274386935601, -17.04225209925078133 ) ) ;
#59265=EDGE_CURVE ( 'NONE', #40206, #13906, #64123, .T. ) ;
#59269=CARTESIAN_POINT ( 'NONE',  ( 206.4537138826727301, 273.0586734743599209, 11.45643784582899016 ) ) ;
#59272=CARTESIAN_POINT ( 'NONE',  ( 9.911560002841389050, 164.9824982072973967, 3.021315404115420679E-15 ) ) ;
#59273=CARTESIAN_POINT ( 'NONE',  ( 143.8006444583684242, 244.6423013555409796, -4.594050593750043987 ) ) ;
#59274=VERTEX_POINT ( 'NONE', #20564 ) ;
#59276=CARTESIAN_POINT ( 'NONE',  ( -3.369807917299440181, 168.8615022471902591, -10.00000000000009592 ) ) ;
#59278=CARTESIAN_POINT ( 'NONE',  ( 155.6308784268266265, 261.7459045956564978, -16.98888936756683066 ) ) ;
#59279=CONICAL_SURFACE ( 'NONE', #2709, 16.82106496071143908, 0.7853981633974241872 ) ;
#59280=CARTESIAN_POINT ( 'NONE',  ( 204.4325665793906524, 276.5594032932251594, 13.33817701435311598 ) ) ;
#59283=VERTEX_POINT ( 'NONE', #2883 ) ;
#59285=CARTESIAN_POINT ( 'NONE',  ( 182.3579730533000998, 275.1687724611243766, -17.70355169473433676 ) ) ;
#59287=CARTESIAN_POINT ( 'NONE',  ( 205.9447606851647947, 273.9402062711180861, -10.75123264850128102 ) ) ;
#59288=CARTESIAN_POINT ( 'NONE',  ( 200.9728293662470833, 267.3697413902040125, 0.8356558750402847124 ) ) ;
#59289=CARTESIAN_POINT ( 'NONE',  ( 190.2287563641723978, 301.1611242470490311, -4.521471513871881953 ) ) ;
#59290=CARTESIAN_POINT ( 'NONE',  ( 182.8870023055169156, 280.6774797787840612, 16.96697556416149411 ) ) ;
#59291=CARTESIAN_POINT ( 'NONE',  ( 157.0887340267001946, 258.5613266995183039, -17.61824281915036394 ) ) ;
#59292=CARTESIAN_POINT ( 'NONE',  ( 196.3186127241907570, 270.7072474025165434, 11.90743844834340059 ) ) ;
#59293=EDGE_CURVE ( 'NONE', #57780, #80596, #74006, .T. ) ;
#59295=CARTESIAN_POINT ( 'NONE',  ( 149.7166446726674565, 271.3301600186404698, 12.26048591517335495 ) ) ;
#59298=CARTESIAN_POINT ( 'NONE',  ( 197.9002057575219453, 287.8737841300738296, 18.01270164875645818 ) ) ;
#59300=CARTESIAN_POINT ( 'NONE',  ( 207.1811000426777980, 271.7988036885084853, 5.430390748498256315 ) ) ;
#59301=CARTESIAN_POINT ( 'NONE',  ( 132.7946446283434341, 254.1427522451419065, -10.00000000000009415 ) ) ;
#59303=CARTESIAN_POINT ( 'NONE',  ( 172.2205269341238250, 283.6848208328027567, -12.54202715120148959 ) ) ;
#59304=ORIENTED_EDGE ( 'NONE', *, *, #20347, .T. ) ;
#59305=ADVANCED_FACE ( 'NONE', ( #38209 ), #50557, .F. ) ;
#59306=B_SPLINE_CURVE_WITH_KNOTS ( 'NONE', 3,
 ( #24179, #25169, #8974, #39352, #48484, #54548, #30785, #61666, #56051, #31754, #55061, #46976, #100200, #7989, #9488, #16572 ),
 .UNSPECIFIED., .F., .F.,
 ( 4, 2, 2, 2, 2, 2, 2, 4 ),
 ( 0.000000000000000000, 0.0003786681000627616523, 0.0007573362001255233046, 0.001136004300188284740, 0.001514672400251046609, 0.001893340500313808262, 0.002272008600376569480, 0.003029344800502104494 ),
 .UNSPECIFIED. ) ;
#59308=CARTESIAN_POINT ( 'NONE',  ( 198.4427928769277969, 286.9339956717308837, -17.97122743692687763 ) ) ;
#59309=CARTESIAN_POINT ( 'NONE',  ( 6.887527552763561545, 162.5327760586659736, 1.948934522072302763E-15 ) ) ;
#59311=CARTESIAN_POINT ( 'NONE',  ( 178.4620001282691248, 259.0559472856667185, -10.32065242460678789 ) ) ;
#59314=CARTESIAN_POINT ( 'NONE',  ( 204.7519188734507622, 276.0062688943993408, -12.76027478560537531 ) ) ;
#59317=CARTESIAN_POINT ( 'NONE',  ( 168.3523909146705080, 257.0143146618579522, 13.69849197686756526 ) ) ;
#59318=CARTESIAN_POINT ( 'NONE',  ( 64.45080651302146180, 218.0177522451419065, 5.000000000000046185 ) ) ;
#59320=CARTESIAN_POINT ( 'NONE',  ( 198.7076130252130497, 286.4753137200327728, 17.36142183403824291 ) ) ;
#59321=CARTESIAN_POINT ( 'NONE',  ( 51.26196130476884605, 213.7365022471903160, 2.944929066748280225E-16 ) ) ;
#59325=CARTESIAN_POINT ( 'NONE',  ( 6.913983429043053519, 183.9869531367911009, 4.594050593750046652 ) ) ;
#59327=CARTESIAN_POINT ( 'NONE',  ( 152.8522706834672533, 265.8990964544007056, 17.63080661522264947 ) ) ;
#59329=CARTESIAN_POINT ( 'NONE',  ( 133.7124848875370731, 259.5530062829863596, -4.648177544792955347E-16 ) ) ;
#59330=CARTESIAN_POINT ( 'NONE',  ( 179.4408063581041688, 277.4340371255875652, 17.62723233342114071 ) ) ;
#59331=CARTESIAN_POINT ( 'NONE',  ( 185.2668547008559301, 266.6439737122302631, 14.32305106529361893 ) ) ;
#59333=CARTESIAN_POINT ( 'NONE',  ( 160.8582016657742031, 280.1240471360480910, 9.077153339507843199 ) ) ;
#59337=DIRECTION ( 'NONE',  ( 0.4999999999999992784, -0.8660254037844390407, 0.000000000000000000 ) ) ;
#59338=CARTESIAN_POINT ( 'NONE',  ( 187.4908492809263691, 258.5206764845227099, -1.234691217589329870 ) ) ;
#59340=CARTESIAN_POINT ( 'NONE',  ( 194.3252252352508265, 294.0658320307167628, 14.07225870721148731 ) ) ;
#59342=AXIS2_PLACEMENT_3D ( 'NONE', #29891, #99806, #38477 ) ;
#59343=CARTESIAN_POINT ( 'NONE',  ( 181.7253891428028396, 289.6325948940144599, 12.87432269931904649 ) ) ;
#59344=CARTESIAN_POINT ( 'NONE',  ( 156.6168467568483891, 276.9391697405689001, 11.51099842983860633 ) ) ;
#59345=CARTESIAN_POINT ( 'NONE',  ( 159.3995226465659982, 254.5589234043588078, -16.81133486613867234 ) ) ;
#59346=DIRECTION ( 'NONE',  ( -0.8660254037844387076, -0.4999999999999998890, -0.000000000000000000 ) ) ;
#59348=CARTESIAN_POINT ( 'NONE',  ( 196.5932062138799949, 289.3313561647224219, -16.66630370796737282 ) ) ;
#59352=CARTESIAN_POINT ( 'NONE',  ( 203.0862352702880003, 278.8913175244117610, -15.09542727681365015 ) ) ;
#59354=ORIENTED_EDGE ( 'NONE', *, *, #11853, .T. ) ;
#59355=CARTESIAN_POINT ( 'NONE',  ( 159.6554334375900055, 278.4301001067392463, -9.783717483729949649 ) ) ;
#59356=CARTESIAN_POINT ( 'NONE',  ( 164.0777181605478745, 246.4560510864015441, 5.763760713451748785 ) ) ;
#59357=CARTESIAN_POINT ( 'NONE',  ( 192.0645969571214096, 297.9813550654635605, 11.46542907566974812 ) ) ;
#59358=ORIENTED_EDGE ( 'NONE', *, *, #12881, .T. ) ;
#59359=CARTESIAN_POINT ( 'NONE',  ( 190.7851866479434761, 300.1973587246873194, 7.931162401707728016 ) ) ;
#59361=CARTESIAN_POINT ( 'NONE',  ( 177.4308907843801535, 263.7877129026015268, 14.57181058525106643 ) ) ;
#59364=ADVANCED_FACE ( 'NONE', ( #10349 ), #74153, .T. ) ;
#59367=CARTESIAN_POINT ( 'NONE',  ( 164.8616299252405213, 245.0982760813026857, 1.544363874765093625 ) ) ;
#59370=CARTESIAN_POINT ( 'NONE',  ( 174.4235015103839430, 277.1789894570474644, -15.65561870163843139 ) ) ;
#59371=CARTESIAN_POINT ( 'NONE',  ( 170.6146014438598399, 262.6168579639755762, -15.59251864883664496 ) ) ;
#59374=CARTESIAN_POINT ( 'NONE',  ( 193.2140586456748679, 295.9904290195353269, -12.67640480829088823 ) ) ;
#59376=CARTESIAN_POINT ( 'NONE',  ( 157.6447300738524007, 268.8659721402340210, 15.63426755860266049 ) ) ;
#59377=ORIENTED_EDGE ( 'NONE', *, *, #33382, .F. ) ;
#59379=CARTESIAN_POINT ( 'NONE',  ( 168.9258527264130976, 272.6118975377002016, 16.11663601824622560 ) ) ;
#59380=CARTESIAN_POINT ( 'NONE',  ( 190.7569505155522904, 300.2462651405980978, -5.670926626284815697 ) ) ;
#59381=CARTESIAN_POINT ( 'NONE',  ( 188.6309741990370981, 298.5980790689797004, -4.273843755561794744 ) ) ;
#59383=FACE_OUTER_BOUND ( 'NONE', #87108, .T. ) ;
#59384=CARTESIAN_POINT ( 'NONE',  ( 191.0852157684255133, 299.6776930442621278, 8.737980942128526607 ) ) ;
#59385=CARTESIAN_POINT ( 'NONE',  ( 146.5157004908022031, 276.8743579738231233, -0.1877253132609108255 ) ) ;
#59390=CARTESIAN_POINT ( 'NONE',  ( 196.3286486926436680, 290.5958008134369948, -16.58330917766970458 ) ) ;
#59391=CARTESIAN_POINT ( 'NONE',  ( 164.5813345449211624, 245.5837619211427523, 1.447064457712487373 ) ) ;
#59393=ORIENTED_EDGE ( 'NONE', *, *, #17792, .F. ) ;
#59394=CARTESIAN_POINT ( 'NONE',  ( 171.4377615637976646, 289.1140544575544595, 4.296774136842674174 ) ) ;
#59395=CARTESIAN_POINT ( 'NONE',  ( 176.6326841078148107, 289.9666541282182948, -9.329455955297444092 ) ) ;
#59398=CARTESIAN_POINT ( 'NONE',  ( 190.3115065349328177, 301.0177967469567761, -3.259545964094417769 ) ) ;
#59400=CARTESIAN_POINT ( 'NONE',  ( 202.8915528389443068, 277.8823096497555412, 15.16837591707065869 ) ) ;
#59402=CARTESIAN_POINT ( 'NONE',  ( 160.1334858203248643, 253.2876618965237867, -16.18833947189418510 ) ) ;
#59403=CARTESIAN_POINT ( 'NONE',  ( 189.9981042791225150, 301.5606253772268133, -1.333257489390088368 ) ) ;
#59405=CARTESIAN_POINT ( 'NONE',  ( 170.7953178271928039, 255.2457615276028093, -12.92277808742838374 ) ) ;
#59407=CARTESIAN_POINT ( 'NONE',  ( 193.8354046899084153, 268.4885937380259406, 12.87375928640720524 ) ) ;
#59408=CARTESIAN_POINT ( 'NONE',  ( 164.2578067403839555, 246.1441285162624126, -2.322300236470859591 ) ) ;
#59409=CARTESIAN_POINT ( 'NONE',  ( 39.40823858692152015, 186.8927522451417929, -10.00000000000009059 ) ) ;
#59410=CARTESIAN_POINT ( 'NONE',  ( 122.6912752411227103, 232.4548013555409796, -4.594050593750042211 ) ) ;
#59411=CARTESIAN_POINT ( 'NONE',  ( 199.0773057068961123, 285.8349872121713702, -17.17316764978006560 ) ) ;
#59413=CARTESIAN_POINT ( 'NONE',  ( -22.42236680055709641, 157.8615022471902591, 0.000000000000000000 ) ) ;
#59414=CARTESIAN_POINT ( 'NONE',  ( 208.2161171980831682, 270.0061013886409569, 2.944709006235987747 ) ) ;
#59415=CARTESIAN_POINT ( 'NONE',  ( 29.51209413086700906, 187.8458772461660544, 9.188101187500095079 ) ) ;
#59419=CARTESIAN_POINT ( 'NONE',  ( 174.5508403973756515, 260.3590064504865040, -14.93617697178709314 ) ) ;
#59420=CARTESIAN_POINT ( 'NONE',  ( 181.2785360512119155, 267.7684897940154656, 14.99012931819231653 ) ) ;
#59421=EDGE_CURVE ( 'NONE', #13195, #64017, #57107, .T. ) ;
#59423=CARTESIAN_POINT ( 'NONE',  ( 105.5870131927823792, 221.7677522451417929, -5.000000000000041744 ) ) ;
#59426=CARTESIAN_POINT ( 'NONE',  ( 179.2989983647532881, 287.9912263975500650, -12.74886096560045878 ) ) ;
#59427=CARTESIAN_POINT ( 'NONE',  ( 164.1030008762014063, 250.1404465237781949, 10.60968069481521781 ) ) ;
#59429=CARTESIAN_POINT ( 'NONE',  ( 101.7620676594010973, 222.8927522451418213, -10.00000000000009059 ) ) ;
#59431=CARTESIAN_POINT ( 'NONE',  ( 198.7756665828275686, 267.6177563492644254, -8.240796915055890182 ) ) ;
#59432=ADVANCED_FACE ( 'NONE', ( #66528 ), #41725, .T. ) ;
#59433=CARTESIAN_POINT ( 'NONE',  ( 156.6246755477763202, 280.3786321986610233, -1.584460325695541849 ) ) ;
#59435=CARTESIAN_POINT ( 'NONE',  ( 19.44454881187291662, 182.0333772461660544, 9.188101187500095079 ) ) ;
#59440=CARTESIAN_POINT ( 'NONE',  ( 59.55252387252222945, 199.0643266524159856, -9.188101187500093303 ) ) ;
#59441=CARTESIAN_POINT ( 'NONE',  ( 207.7655736232174206, 270.7864657513322300, 3.530742899761726949 ) ) ;
#59442=CARTESIAN_POINT ( 'NONE',  ( 164.2712161151136172, 246.1209027979328710, 7.276091357954241445 ) ) ;
#59444=CARTESIAN_POINT ( 'NONE',  ( 149.0155189933042266, 277.2682270220686291, -2.168681601895305011 ) ) ;
#59446=CARTESIAN_POINT ( 'NONE',  ( 208.3132655666949233, 269.8378354783333180, 2.688523655043302707 ) ) ;
#59447=CARTESIAN_POINT ( 'NONE',  ( 21.31191609055711211, 173.1115022471901739, -5.000000000000041744 ) ) ;
#59450=CARTESIAN_POINT ( 'NONE',  ( 145.2890388471816721, 248.5643266524159856, -9.188101187500093303 ) ) ;
#59452=CARTESIAN_POINT ( 'NONE',  ( 165.0094001503442485, 244.8423305435771624, 1.224072641870707301 ) ) ;
#59456=CARTESIAN_POINT ( 'NONE',  ( 189.5229297568409663, 289.6899146468908270, 14.72468552167156908 ) ) ;
#59458=ORIENTED_EDGE ( 'NONE', *, *, #26141, .T. ) ;
#59459=CARTESIAN_POINT ( 'NONE',  ( 150.7254409736883645, 269.5828735707850683, 14.54962197351449049 ) ) ;
#59460=CARTESIAN_POINT ( 'NONE',  ( 163.3401907624258627, 247.7334860119229063, 8.055311219927849820 ) ) ;
#59461=CARTESIAN_POINT ( 'NONE',  ( 187.4171132689631634, 261.5282790321019206, -9.397869408254909018 ) ) ;
#59462=CARTESIAN_POINT ( 'NONE',  ( 173.0074926688108405, 268.3266801289679506, -16.33672149581441246 ) ) ;
#59463=CARTESIAN_POINT ( 'NONE',  ( 197.3443253216253481, 273.2483388696968518, -14.62721317763432971 ) ) ;
#59467=CARTESIAN_POINT ( 'NONE',  ( 170.8306833669449247, 284.5486215507588099, -11.65048194455012620 ) ) ;
#59469=B_SPLINE_SURFACE_WITH_KNOTS ( 'NONE', 3, 1, ( 
 ( #40151, #31059 ),
 ( #53848, #39144 ),
 ( #16866, #94409 ),
 ( #7773, #47752 ),
 ( #9795, #77169 ),
 ( #78185, #24962 ),
 ( #46769, #15861 ),
 ( #672, #9278 ),
 ( #84808, #77694 ),
 ( #31555, #1181 ),
 ( #8277, #70056 ),
 ( #71093, #40655 ),
 ( #15348, #62967 ),
 ( #79221, #85315 ),
 ( #93412, #23961 ),
 ( #61949, #24470 ),
 ( #55840, #86835 ),
 ( #2188, #17369 ),
 ( #23452, #46244 ),
 ( #71593, #38665 ),
 ( #62444, #69568 ),
 ( #176, #54863 ),
 ( #92900, #54344 ),
 ( #85843, #47263 ),
 ( #18383, #66461 ),
 ( #35560, #18889 ),
 ( #95437, #19882 ),
 ( #25989, #41658 ),
 ( #87844, #27483 ),
 ( #49278, #34090 ),
 ( #73576, #10281 ),
 ( #64979, #41151 ),
 ( #42158, #96912 ),
 ( #3686, #26976 ) ),
 .UNSPECIFIED., .T., .F., .F.,
 ( 4, 2, 2, 2, 2, 2, 2, 2, 2, 2, 2, 2, 2, 2, 2, 2, 4 ),
 ( 2, 2 ),
 ( 0.000000000000000000, 0.06250000000000000000, 0.1250000000000000000, 0.1875000000000000000, 0.2500000000000000000, 0.3125000000000000000, 0.3750000000000000000, 0.4375000000000000000, 0.5000000000000000000, 0.5625000000000000000, 0.6250000000000000000, 0.6875000000000000000, 0.7500000000000000000, 0.8125000000000000000, 0.8750000000000000000, 0.9375000000000000000, 1.000000000000000000 ),
 ( 0.000000000000000000, 1.000000000000000000 ),
 .UNSPECIFIED. ) ;
#59472=CARTESIAN_POINT ( 'NONE',  ( 185.7378568990949645, 296.6331975062905144, 4.666997342915078839 ) ) ;
#59475=CARTESIAN_POINT ( 'NONE',  ( 153.3544108199959908, 265.0293642254135307, -17.49105661178601423 ) ) ;
#59482=CARTESIAN_POINT ( 'NONE',  ( 156.8307661425255048, 262.4341872189889386, -16.93460929011386540 ) ) ;
#59484=CARTESIAN_POINT ( 'NONE',  ( 147.2937583206075942, 275.5267222813735088, 0.1877253132609109920 ) ) ;
#59485=CARTESIAN_POINT ( 'NONE',  ( 205.1818214405880951, 273.2280494462991101, -9.772995860142792424 ) ) ;
#59487=CARTESIAN_POINT ( 'NONE',  ( 204.1793240545508752, 276.9980322128846524, 14.17550310845996187 ) ) ;
#59488=CARTESIAN_POINT ( 'NONE',  ( 157.7632566947985708, 282.3764601569879460, -1.694678876849560645 ) ) ;
#59490=DIRECTION ( 'NONE',  ( 0.4999999999999992784, -0.8660254037844390407, 0.000000000000000000 ) ) ;
#59492=CARTESIAN_POINT ( 'NONE',  ( 89.59260651841245249, 222.5333772461660544, 9.188101187500095079 ) ) ;
#59493=CARTESIAN_POINT ( 'NONE',  ( 174.3282188611405559, 255.0574352009110157, -10.77860568660477902 ) ) ;
#59496=CARTESIAN_POINT ( 'NONE',  ( 178.0813752549872504, 269.0315758126946548, -16.95330150772717204 ) ) ;
#59501=VERTEX_POINT ( 'NONE', #11851 ) ;
#59502=CARTESIAN_POINT ( 'NONE',  ( -22.42236680055709641, 157.8615022471902591, 0.000000000000000000 ) ) ;
#59504=EDGE_CURVE ( 'NONE', #76998, #4619, #60677, .T. ) ;
#59507=CARTESIAN_POINT ( 'NONE',  ( 164.9546295582813400, 248.3711573621226023, -9.130659607263403643 ) ) ;
#59513=CARTESIAN_POINT ( 'NONE',  ( 165.4931806181214995, 265.5848062394981639, -16.61349363679761026 ) ) ;
#59514=EDGE_LOOP ( 'NONE', ( #64727, #74632, #93980, #17934 ) ) ;
#59518=CARTESIAN_POINT ( 'NONE',  ( 167.2093226243390802, 283.7324425667255241, 9.043444139037532636 ) ) ;
#59519=CARTESIAN_POINT ( 'NONE',  ( 199.9158715130028838, 270.2492972290452826, 9.939794670651632913 ) ) ;
#59521=DIRECTION ( 'NONE',  ( 0.4999999999999995559, -0.8660254037844389297, 0.000000000000000000 ) ) ;
#59522=CARTESIAN_POINT ( 'NONE',  ( 206.8317058779879574, 272.4039721336197317, -10.41591514895975834 ) ) ;
#59523=CARTESIAN_POINT ( 'NONE',  ( 149.0752043596417593, 276.3754483912217097, -5.522432154670898541 ) ) ;
#59525=CARTESIAN_POINT ( 'NONE',  ( 158.6496056213609904, 257.8578177934796258, 17.38082990300775776 ) ) ;
#59526=DIRECTION ( 'NONE',  ( -0.8660254037844392627, -0.4999999999999987232, 0.000000000000000000 ) ) ;
#59529=CARTESIAN_POINT ( 'NONE',  ( 147.7395812515338491, 275.4447818272566337, 3.760927250875937489 ) ) ;
#59533=CARTESIAN_POINT ( 'NONE',  ( 160.9531570974293402, 275.8817019889240214, 12.81199482524368882 ) ) ;
#59534=CARTESIAN_POINT ( 'NONE',  ( 171.9666747079280071, 279.8309318510848698, -14.47863982768428137 ) ) ;
#59535=CARTESIAN_POINT ( 'NONE',  ( 164.0970344217799948, 246.4225943405349710, -8.491506243827155131 ) ) ;
#59538=CARTESIAN_POINT ( 'NONE',  ( 160.9791900386504722, 272.6641784107281410, 15.33525930436291951 ) ) ;
#59539=CARTESIAN_POINT ( 'NONE',  ( -8.160010933756074891, 166.0958772461660544, -9.188101187500095079 ) ) ;
#59541=CARTESIAN_POINT ( 'NONE',  ( 16.91508078042228647, 192.1199935810941213, 2.679491924311251605 ) ) ;
#59543=AXIS2_PLACEMENT_3D ( 'NONE', #31860, #62252, #54150 ) ;
#59544=ORIENTED_EDGE ( 'NONE', *, *, #56489, .T. ) ;
#59545=CARTESIAN_POINT ( 'NONE',  ( 13.97105408662886461, 167.3262482093458061, -5.229199737892075682E-14 ) ) ;
#59550=DIRECTION ( 'NONE',  ( -0.8660254037844387076, -0.4999999999999998890, -0.000000000000000000 ) ) ;
#59551=AXIS2_PLACEMENT_3D ( 'NONE', #51625, #21230, #52601 ) ;
#59553=CARTESIAN_POINT ( 'NONE',  ( 172.3741624485570867, 252.4865239976215037, 8.880853820034850798 ) ) ;
#59554=CARTESIAN_POINT ( 'NONE',  ( 3.504529045289348055, 163.6423013555410080, -4.594050593750043987 ) ) ;
#59555=CARTESIAN_POINT ( 'NONE',  ( 108.9156247924702114, 239.8149278399160949, -9.188101187500095079 ) ) ;
#59556=CARTESIAN_POINT ( 'NONE',  ( 36.90037335867692292, 202.1115022471903160, -5.000000000000047962 ) ) ;
#59557=CARTESIAN_POINT ( 'NONE',  ( 183.1379727938016799, 294.1415918804704575, -7.857043814308706686 ) ) ;
#59560=CIRCLE ( 'NONE', #62814, 17.82106496071138935 ) ;
#59561=EDGE_CURVE ( 'NONE', #86137, #94561, #2670, .T. ) ;
#59563=CARTESIAN_POINT ( 'NONE',  ( 69.66731286396763778, 199.4824982072973967, 3.021315404115420679E-15 ) ) ;
#59565=CARTESIAN_POINT ( 'NONE',  ( 207.8996209429610360, 270.5542889829179103, -5.987818313449536411 ) ) ;
#59566=CARTESIAN_POINT ( 'NONE',  ( 148.1632261683078013, 274.0207597936089883, -7.853210555358286271 ) ) ;
#59568=CARTESIAN_POINT ( 'NONE',  ( 190.4356836585210431, 300.3996184492839916, -0.5836641476860114919 ) ) ;
#59569=CARTESIAN_POINT ( 'NONE',  ( 46.72328617017402053, 209.3297689869269504, -2.679491924311201423 ) ) ;
#59570=CARTESIAN_POINT ( 'NONE',  ( 162.7494290383994553, 250.9923089725520242, -12.89632743124666803 ) ) ;
#59571=DIRECTION ( 'NONE',  ( 0.4999999999999998890, -0.8660254037844385966, 0.000000000000000000 ) ) ;
#59572=AXIS2_PLACEMENT_3D ( 'NONE', #78153, #38115, #78657 ) ;
#59573=CARTESIAN_POINT ( 'NONE',  ( 175.8807902318873744, 265.5460882003382039, -15.84645557839000496 ) ) ;
#59574=CARTESIAN_POINT ( 'NONE',  ( 97.65764163903753570, 221.0643266524160424, 9.188101187500095079 ) ) ;
#59576=CARTESIAN_POINT ( 'NONE',  ( 150.6487462746963502, 269.7157126861102370, 15.18501655901553704 ) ) ;
#59578=CARTESIAN_POINT ( 'NONE',  ( 157.2744851780909414, 258.2395962677452985, 18.17792129701959070 ) ) ;
#59579=CARTESIAN_POINT ( 'NONE',  ( 200.3578380681407793, 283.6170401017593576, 17.20245520226215774 ) ) ;
#59580=CARTESIAN_POINT ( 'NONE',  ( 196.3322077676189394, 290.5896363147520560, 17.46901783180497603 ) ) ;
#59581=CARTESIAN_POINT ( 'NONE',  ( 151.4376533647338476, 268.3492855237141725, -15.16853828792834236 ) ) ;
#59585=CARTESIAN_POINT ( 'NONE',  ( 192.6789561813392595, 296.9172536750198219, -11.84591848451790952 ) ) ;
#59590=CARTESIAN_POINT ( 'NONE',  ( 146.9422184197532317, 276.1356072505412840, -5.063317562214876943 ) ) ;
#59594=CARTESIAN_POINT ( 'NONE',  ( 159.5573297132660002, 254.2855935470410031, 16.91607698584599007 ) ) ;
#59595=CARTESIAN_POINT ( 'NONE',  ( 154.0583916588297768, 267.0402830145829967, 16.21101371575731065 ) ) ;
#59597=CARTESIAN_POINT ( 'NONE',  ( 133.4622058806418750, 257.8615022471902876, 5.000000000000046185 ) ) ;
#59598=EDGE_LOOP ( 'NONE', ( #4332, #76928, #35412, #46442 ) ) ;
#59605=CARTESIAN_POINT ( 'NONE',  ( 181.8498033080804248, 291.5435437066161626, -11.41179615309663120 ) ) ;
#59607=AXIS2_PLACEMENT_3D ( 'NONE', #70326, #32332, #23717 ) ;
#59609=CARTESIAN_POINT ( 'NONE',  ( 158.6518137166425788, 255.8539932602588181, 16.06016111216393583 ) ) ;
#59610=CARTESIAN_POINT ( 'NONE',  ( 190.7226089735735570, 278.2851069703174289, -16.65597922127235719 ) ) ;
#59612=CARTESIAN_POINT ( 'NONE',  ( 201.0732166862245549, 282.3779679885897167, -18.18766936363638820 ) ) ;
#59614=EDGE_CURVE ( 'NONE', #16011, #10482, #25741, .T. ) ;
#59618=EDGE_CURVE ( 'NONE', #97695, #97906, #37721, .T. ) ;
#59621=B_SPLINE_CURVE_WITH_KNOTS ( 'NONE', 3,
 ( #43058, #81140, #59253, #12707 ),
 .UNSPECIFIED., .F., .F.,
 ( 4, 4 ),
 ( 0.01172910784184959775, 0.01779018763767279548 ),
 .UNSPECIFIED. ) ;
#59624=CARTESIAN_POINT ( 'NONE',  ( 182.9391731548801943, 296.0526933300616861, 0.3971291663347272238 ) ) ;
#59626=( BOUNDED_CURVE ( )  B_SPLINE_CURVE ( 2, ( #49759, #79207, #25456, #2677, #63460, #18372, #56344, #41645, #55827 ),
 .UNSPECIFIED., .F., .T. ) 
 B_SPLINE_CURVE_WITH_KNOTS ( ( 3, 2, 2, 2, 3 ),
 ( 0.09274193548387096864, 0.09408602150537634379, 0.09677419354838709409, 0.09946236559139784439, 0.1008064516129032334 ),
 .UNSPECIFIED. ) 
 CURVE ( )  GEOMETRIC_REPRESENTATION_ITEM ( )  RATIONAL_B_SPLINE_CURVE ( ( 0.9330127018922194093, 0.9330127018922194093, 1.000000000000000000, 0.8660254037844387076, 1.000000000000000000, 0.8660254037844387076, 1.000000000000000000, 0.9330127018922189652, 0.9330127018922192983 ) ) 
 REPRESENTATION_ITEM ( '' )  );
#59627=CARTESIAN_POINT ( 'NONE',  ( 174.4196659502841271, 257.0085290835094156, -12.24909860563172259 ) ) ;
#59628=CARTESIAN_POINT ( 'NONE',  ( 162.2331215717501607, 272.2958999960979440, -15.94685713422084739 ) ) ;
#59629=CARTESIAN_POINT ( 'NONE',  ( 165.0817809681736037, 244.7169632896033136, -1.727194264083430131 ) ) ;
#59631=CARTESIAN_POINT ( 'NONE',  ( 203.4435754520237651, 276.2723861740593634, 14.48166091637323483 ) ) ;
#59633=CARTESIAN_POINT ( 'NONE',  ( 170.6833767652849758, 288.4039556261358825, -4.055045876719096221 ) ) ;
#59635=CARTESIAN_POINT ( 'NONE',  ( 165.8447336379009300, 265.9679405602628890, 17.68066565608797092 ) ) ;
#59636=CARTESIAN_POINT ( 'NONE',  ( 181.9564058445976400, 256.6289831591705592, 5.167692713115564551 ) ) ;
#59637=CARTESIAN_POINT ( 'NONE',  ( 115.5194155920915620, 231.3768266524159856, 9.188101187500098632 ) ) ;
#59638=B_SPLINE_CURVE_WITH_KNOTS ( 'NONE', 3,
 ( #25403, #71529, #10718, #54799 ),
 .UNSPECIFIED., .F., .F.,
 ( 4, 4 ),
 ( 0.008498457973065165830, 0.01488670130818619056 ),
 .UNSPECIFIED. ) ;
#59642=CARTESIAN_POINT ( 'NONE',  ( 188.2915414428695726, 273.5140509337351773, 15.65656605059880313 ) ) ;
#59643=VERTEX_POINT ( 'NONE', #99435 ) ;
#59645=VERTEX_POINT ( 'NONE', #97456 ) ;
#59647=EDGE_CURVE ( 'NONE', #26502, #72620, #95753, .T. ) ;
#59649=CARTESIAN_POINT ( 'NONE',  ( 196.4982648257524147, 290.3020170531091821, 16.69353242256149628 ) ) ;
#59650=CARTESIAN_POINT ( 'NONE',  ( 206.4640281786353171, 273.0408085897082060, -10.81921452789957883 ) ) ;
#59651=DIRECTION ( 'NONE',  ( -0.8660254037844387076, -0.4999999999999998890, -0.000000000000000000 ) ) ;
#59654=ORIENTED_EDGE ( 'NONE', *, *, #87942, .F. ) ;
#59657=CARTESIAN_POINT ( 'NONE',  ( 194.6804144021959928, 266.4464820258078817, -8.228719024875283949 ) ) ;
#59658=CARTESIAN_POINT ( 'NONE',  ( -2.962795650140754855, 157.5494855054052152, -2.679491924311252493 ) ) ;
#59660=CARTESIAN_POINT ( 'NONE',  ( 184.3888951012362440, 288.9016753704191274, -13.18852512495808860 ) ) ;
#59662=CARTESIAN_POINT ( 'NONE',  ( 169.7943624855302858, 249.0057814370864833, -4.764873173913280802 ) ) ;
#59664=CARTESIAN_POINT ( 'NONE',  ( 64.01779381112929457, 207.7677522451418497, 10.00000000000009592 ) ) ;
#59668=CARTESIAN_POINT ( 'NONE',  ( 173.2640478233614374, 251.6539192559667413, -0.3386657152870858334 ) ) ;
#59672=CARTESIAN_POINT ( 'NONE',  ( 126.5340026503663466, 243.8615022471902591, -10.00000000000009592 ) ) ;
#59673=EDGE_CURVE ( 'NONE', #58450, #61729, #93400, .T. ) ;
#59675=CARTESIAN_POINT ( 'NONE',  ( 206.5092799326709780, 271.9210634963550888, 7.392161875056491915 ) ) ;
#59677=CARTESIAN_POINT ( 'NONE',  ( 64.58612298413676456, 208.0958772461660544, -9.188101187500095079 ) ) ;
#59678=CARTESIAN_POINT ( 'NONE',  ( 159.2102594322688844, 254.8867369075254885, -16.13039487917589199 ) ) ;
#59680=CARTESIAN_POINT ( 'NONE',  ( 178.1650032105745538, 292.9353035937096479, -5.923887690835723419 ) ) ;
#59686=AXIS2_PLACEMENT_3D ( 'NONE', #99189, #82025, #14078 ) ;
#59687=CARTESIAN_POINT ( 'NONE',  ( 207.4218731373931632, 271.3817724553659332, -5.249531240730909154 ) ) ;
#59690=CARTESIAN_POINT ( 'NONE',  ( 185.8045553127517451, 265.6963936551481424, 13.19588143967888350 ) ) ;
#59696=CARTESIAN_POINT ( 'NONE',  ( 157.6394123119580968, 270.8627004967905805, -14.82514603415767063 ) ) ;
#59699=CARTESIAN_POINT ( 'NONE',  ( 27.50958393249801404, 180.5643266524160424, 9.188101187500095079 ) ) ;
#59700=CARTESIAN_POINT ( 'NONE',  ( 196.0034224882197975, 291.1591091234520263, 17.53794140922627776 ) ) ;
#59701=B_SPLINE_CURVE_WITH_KNOTS ( 'NONE', 3,
 ( #98916, #20421, #44675, #52778 ),
 .UNSPECIFIED., .F., .F.,
 ( 4, 4 ),
 ( 0.007301977675103129943, 0.01234114840196185066 ),
 .UNSPECIFIED. ) ;
#59702=CARTESIAN_POINT ( 'NONE',  ( 200.1719577690460881, 277.9335415779574419, 15.23757986191821345 ) ) ;
#59703=CARTESIAN_POINT ( 'NONE',  ( 164.6150166221017912, 248.5083581723461350, -9.597476261921807250 ) ) ;
#59705=CARTESIAN_POINT ( 'NONE',  ( 54.03161192339643293, 195.8768266524159856, -9.188101187500093303 ) ) ;
#59708=CARTESIAN_POINT ( 'NONE',  ( 170.6125138170483524, 287.8455895967342144, 7.516220978703161748 ) ) ;
#59711=CARTESIAN_POINT ( 'NONE',  ( 180.3600075739701651, 254.8198211655269176, -3.768796009823502047 ) ) ;
#59716=B_SPLINE_SURFACE_WITH_KNOTS ( 'NONE', 3, 1, ( 
 ( #54254, #54767 ),
 ( #30483, #78600 ),
 ( #85749, #30975 ),
 ( #62872, #93830 ),
 ( #15770, #46676 ),
 ( #77603, #76589 ),
 ( #45665, #84723 ),
 ( #47172, #8188 ),
 ( #92329, #7174 ),
 ( #78093, #38060 ),
 ( #39056, #8684 ),
 ( #68974, #15263 ),
 ( #46158, #77077 ),
 ( #38572, #76897 ),
 ( #53105, #22208 ),
 ( #60682, #7001 ),
 ( #84060, #90667 ),
 ( #36903, #22714 ),
 ( #92164, #15091 ),
 ( #82571, #99223 ),
 ( #14116, #67304 ),
 ( #98231, #35907 ),
 ( #37887, #59182 ),
 ( #29809, #6009 ),
 ( #13133, #61195 ),
 ( #44994, #14616 ),
 ( #52103, #6518 ),
 ( #83551, #45494 ),
 ( #67815, #91146 ),
 ( #76428, #53594 ),
 ( #36399, #28816 ),
 ( #5515, #91641 ),
 ( #68796, #68300 ),
 ( #59700, #43991 ) ),
 .UNSPECIFIED., .T., .F., .F.,
 ( 4, 2, 2, 2, 2, 2, 2, 2, 2, 2, 2, 2, 2, 2, 2, 2, 4 ),
 ( 2, 2 ),
 ( 0.000000000000000000, 0.06250000000000000000, 0.1250000000000000000, 0.1875000000000000000, 0.2500000000000000000, 0.3125000000000000000, 0.3750000000000000000, 0.4375000000000000000, 0.5000000000000000000, 0.5625000000000000000, 0.6250000000000000000, 0.6875000000000000000, 0.7500000000000000000, 0.8125000000000000000, 0.8750000000000000000, 0.9375000000000000000, 1.000000000000000000 ),
 ( 0.000000000000000000, 1.000000000000000000 ),
 .UNSPECIFIED. ) ;
#59717=CARTESIAN_POINT ( 'NONE',  ( 163.2851116495353665, 256.0038574147548616, -14.89960205689385120 ) ) ;
#59718=CYLINDRICAL_SURFACE ( 'NONE', #54185, 10.00000000000010658 ) ;
#59719=CARTESIAN_POINT ( 'NONE',  ( 90.08876690777121610, 229.4865022471902876, -10.00000000000009415 ) ) ;
#59720=CARTESIAN_POINT ( 'NONE',  ( 200.4403816905005158, 283.4740703539914648, 16.81798557643505987 ) ) ;
#59721=CARTESIAN_POINT ( 'NONE',  ( 164.9043417134678577, 286.5925546497160212, 0.04530247668140159611 ) ) ;
#59722=EDGE_LOOP ( 'NONE', ( #43186, #13320, #45879, #99664 ) ) ;
#59723=CARTESIAN_POINT ( 'NONE',  ( 53.67935523340274528, 210.9869531367911009, 4.594050593750046652 ) ) ;
#59724=ORIENTED_EDGE ( 'NONE', *, *, #9240, .T. ) ;
#59725=CARTESIAN_POINT ( 'NONE',  ( 164.4943844331201603, 264.4168344445729417, 16.69252833053101526 ) ) ;
#59726=CARTESIAN_POINT ( 'NONE',  ( 190.8683709797118411, 300.0532792356709706, -4.461919767133968762 ) ) ;
#59734=CARTESIAN_POINT ( 'NONE',  ( 204.9134960529544287, 275.7264090101555212, 14.56629498631681408 ) ) ;
#59738=CARTESIAN_POINT ( 'NONE',  ( 175.5824964429158399, 254.0579991535531406, 8.209342937837284637 ) ) ;
#59742=CARTESIAN_POINT ( 'NONE',  ( 167.0738366597983031, 261.5866074660107188, 16.40510134541907661 ) ) ;
#59743=CARTESIAN_POINT ( 'NONE',  ( 206.1405152101578437, 273.6011494880188479, -9.618815605734603480 ) ) ;
#59744=VERTEX_POINT ( 'NONE', #39090 ) ;
#59745=CARTESIAN_POINT ( 'NONE',  ( 159.7553372911454233, 283.1775518570184431, -3.360441317989244947 ) ) ;
#59746=CARTESIAN_POINT ( 'NONE',  ( 61.41971759977600698, 196.2677522451418213, -5.000000000000041744 ) ) ;
#59747=CARTESIAN_POINT ( 'NONE',  ( 207.6067494229581314, 271.0615573356529353, -1.924113146155245868 ) ) ;
#59749=CARTESIAN_POINT ( 'NONE',  ( 198.3150362131025588, 287.1552767044814800, 18.53472937702030521 ) ) ;
#59751=CARTESIAN_POINT ( 'NONE',  ( 162.1286899612119612, 263.6308679106482487, -16.92993415948811986 ) ) ;
#59752=CARTESIAN_POINT ( 'NONE',  ( 128.2121871902485566, 235.6423013555409796, -4.594050593750043987 ) ) ;
#59756=VERTEX_POINT ( 'NONE', #80533 ) ;
#59759=VERTEX_POINT ( 'NONE', #69003 ) ;
#59762=VERTEX_POINT ( 'NONE', #99931 ) ;
#59764=CARTESIAN_POINT ( 'NONE',  ( 81.69914580506154778, 224.6427522451419065, 10.00000000000009415 ) ) ;
#59766=CARTESIAN_POINT ( 'NONE',  ( 195.3630008912252549, 285.3603474548959298, 16.99413665511329086 ) ) ;
#59767=EDGE_CURVE ( 'NONE', #12230, #52681, #30516, .T. ) ;
#59770=CARTESIAN_POINT ( 'NONE',  ( 194.1153812227096864, 294.4292925221022870, 15.54001482840963710 ) ) ;
#59772=EDGE_CURVE ( 'NONE', #13298, #22379, #8666, .T. ) ;
#59781=CARTESIAN_POINT ( 'NONE',  ( 164.1943448329197395, 246.6690389504045413, 4.590013871137070822 ) ) ;
#59783=CARTESIAN_POINT ( 'NONE',  ( 193.6564271169084464, 262.6014873983580742, -4.146719891036213745 ) ) ;
#59784=AXIS2_PLACEMENT_3D ( 'NONE', #39863, #77407, #8499 ) ;
#59785=CARTESIAN_POINT ( 'NONE',  ( 195.1154436510188077, 279.2972436967689873, 16.36790060704208116 ) ) ;
#59786=CARTESIAN_POINT ( 'NONE',  ( 164.4678285797544106, 245.7803600197737524, -6.875991496205872799 ) ) ;
#59787=CARTESIAN_POINT ( 'NONE',  ( 130.4037065759891334, 258.3464784336661637, 1.353441290958777327E-15 ) ) ;
#59788=ORIENTED_EDGE ( 'NONE', *, *, #62772, .T. ) ;
#59789=CARTESIAN_POINT ( 'NONE',  ( -0.6995629222973920314, 163.7365022471902023, -10.00000000000009237 ) ) ;
#59790=CARTESIAN_POINT ( 'NONE',  ( 183.8210692855788864, 257.9504670327482927, 6.873620218444065344 ) ) ;
#59793=CARTESIAN_POINT ( 'NONE',  ( 185.8492146212669240, 258.6745004276652935, -5.862532207920108540 ) ) ;
#59794=ORIENTED_EDGE ( 'NONE', *, *, #83368, .F. ) ;
#59797=ADVANCED_FACE ( 'NONE', ( #12602 ), #27790, .T. ) ;
#59798=CARTESIAN_POINT ( 'NONE',  ( 167.6136624610167019, 249.2005778497498341, -6.016629856180416347 ) ) ;
#59802=CARTESIAN_POINT ( 'NONE',  ( 147.5693121967435957, 275.0494489676833041, 4.210973343677100189 ) ) ;
#59803=ADVANCED_FACE ( 'NONE', ( #23652 ), #52562, .T. ) ;
#59804=CARTESIAN_POINT ( 'NONE',  ( 186.5492813281628912, 282.5551454570558008, 16.18981372509010797 ) ) ;
#59805=CARTESIAN_POINT ( 'NONE',  ( 205.0520875136525376, 275.4863615587311756, -14.16385635411862509 ) ) ;
#59806=CARTESIAN_POINT ( 'NONE',  ( 194.3107701606939486, 269.6703757554475942, 12.05248313980574615 ) ) ;
#59810=CARTESIAN_POINT ( 'NONE',  ( 190.1190668544949460, 301.3511120508678118, 4.410340539513557090 ) ) ;
#59811=CARTESIAN_POINT ( 'NONE',  ( 172.0910100529608258, 260.0785035667472584, 15.53398388876759206 ) ) ;
#59813=B_SPLINE_CURVE_WITH_KNOTS ( 'NONE', 3,
 ( #69394, #24298, #30394, #92249, #22799, #53678, #15173, #46074, #76986, #1999, #87168, #87670, #57677, #88656, #2510, #96734, #32885, #79543, #48603, #71409, #3515, #10100, #71909, #65291, #80539, #63788, #33393, #19221, #34392, #88156, #18205, #56687, #89166, #49098, #41474, #3026, #11611, #41988, #96232, #64295, #11118, #48085, #50092, #33915, #9615, #80033, #26301, #57177 ),
 .UNSPECIFIED., .F., .F.,
 ( 4, 2, 2, 2, 2, 2, 2, 2, 2, 2, 2, 2, 2, 2, 2, 2, 2, 2, 2, 2, 2, 2, 2, 4 ),
 ( 0.0007190175845426069901, 0.0009287040927872296453, 0.001138390601031852301, 0.001243233855154209436, 0.001348077109276566788, 0.001557763617521332015, 0.001977136634010862037, 0.002396509650500392493, 0.003235255683479394857, 0.004074001716458396788, 0.004912747749437398719, 0.005332120765926939149, 0.005541807274171669899, 0.005646650528294073004, 0.005699072155355274123, 0.005751493782416475242, 0.005856337036538874011, 0.005961180290661273647, 0.006170866798906022611, 0.006590239815395467632, 0.006799926323640210525, 0.007009612831884953418, 0.007219299340129695444, 0.007428985848374438337 ),
 .UNSPECIFIED. ) ;
#59814=CARTESIAN_POINT ( 'NONE',  ( 197.9952413503812352, 287.7091776547143809, 17.17611241386010690 ) ) ;
#59815=CARTESIAN_POINT ( 'NONE',  ( 161.3042361785515197, 251.2598627930960333, 13.07175971676398341 ) ) ;
#59816=CARTESIAN_POINT ( 'NONE',  ( -3.667330603741788320, 162.5643266524160140, 9.188101187500095079 ) ) ;
#59817=CARTESIAN_POINT ( 'NONE',  ( 175.7917838780750799, 285.8274689740071608, -11.81341207233009705 ) ) ;
#59819=CIRCLE ( 'NONE', #85796, 17.82106496071138224 ) ;
#59822=CARTESIAN_POINT ( 'NONE',  ( 198.8570476668614049, 286.2164853282868080, -17.01721544293231858 ) ) ;
#59823=B_SPLINE_CURVE_WITH_KNOTS ( 'NONE', 3,
 ( #2284, #31144, #77781, #70657 ),
 .UNSPECIFIED., .F., .F.,
 ( 4, 4 ),
 ( 0.01157169839800022484, 0.01758127579506474358 ),
 .UNSPECIFIED. ) ;
#59824=CARTESIAN_POINT ( 'NONE',  ( 6.480970727150832111, 183.7369531367911009, -4.594050593750048428 ) ) ;
#59825=CARTESIAN_POINT ( 'NONE',  ( 181.7611970338358560, 276.1868128385311252, -16.62830721219069119 ) ) ;
#59828=CARTESIAN_POINT ( 'NONE',  ( 170.2912665166379611, 270.8011127091891126, -16.89563538064900428 ) ) ;
#59830=CARTESIAN_POINT ( 'NONE',  ( -22.42236680055709641, 157.8615022471902591, 0.000000000000000000 ) ) ;
#59831=CARTESIAN_POINT ( 'NONE',  ( 21.22170510744830096, 176.3927522451418213, -10.00000000000009237 ) ) ;
#59832=CARTESIAN_POINT ( 'NONE',  ( 75.78130554586795142, 207.8927522451417929, -10.00000000000009059 ) ) ;
#59833=CARTESIAN_POINT ( 'NONE',  ( 176.7457436420401677, 254.2668712825680188, -3.870637407069959401 ) ) ;
#59834=CARTESIAN_POINT ( 'NONE',  ( 198.5386315514599858, 286.7679982181109608, 17.03868888912368718 ) ) ;
#59835=EDGE_CURVE ( 'NONE', #95312, #8176, #38982, .T. ) ;
#59836=AXIS2_PLACEMENT_3D ( 'NONE', #54958, #95016, #17467 ) ;
#59837=CARTESIAN_POINT ( 'NONE',  ( 60.28305926085685229, 195.6115022471902023, -5.000000000000041744 ) ) ;
#59839=CARTESIAN_POINT ( 'NONE',  ( 119.0307608796806278, 227.9824982072973683, 3.021315404115420679E-15 ) ) ;
#59840=CARTESIAN_POINT ( 'NONE',  ( 17.65854496445001232, 174.8768266524159856, -9.188101187500091527 ) ) ;
#59841=CARTESIAN_POINT ( 'NONE',  ( 167.7210762313646910, 287.2684685992639402, 4.983143766097549943 ) ) ;
#59842=EDGE_CURVE ( 'NONE', #18980, #13449, #77584, .T. ) ;
#59843=CARTESIAN_POINT ( 'NONE',  ( 192.6797324865049745, 296.9159090750308110, 12.42053959885222625 ) ) ;
#59845=CARTESIAN_POINT ( 'NONE',  ( 165.9969153545198708, 246.1123342570000716, -1.176638740111072723 ) ) ;
#59846=CARTESIAN_POINT ( 'NONE',  ( 207.4764081617721843, 271.2873150223495600, 6.359972247200924578 ) ) ;
#59847=CARTESIAN_POINT ( 'NONE',  ( 186.8874022707183826, 267.3628004192088383, 13.25673146551773129 ) ) ;
#59848=CARTESIAN_POINT ( 'NONE',  ( 153.2978239650968533, 265.5538651647430584, -16.15457164513478006 ) ) ;
#59849=CARTESIAN_POINT ( 'NONE',  ( 160.1502792044530850, 280.1323723417889369, 9.307031849721941086 ) ) ;
#59852=CARTESIAN_POINT ( 'NONE',  ( -22.42236680055709641, 157.8615022471902591, 0.000000000000000000 ) ) ;
#59853=AXIS2_PLACEMENT_3D ( 'NONE', #34779, #27202, #58090 ) ;
#59855=CARTESIAN_POINT ( 'NONE',  ( 194.3799873100184641, 293.9709813348915191, 15.33105633561973669 ) ) ;
#59857=CARTESIAN_POINT ( 'NONE',  ( 183.4752222048318515, 289.9104771362203792, 12.19711425367773394 ) ) ;
#59858=CARTESIAN_POINT ( 'NONE',  ( 174.5885488454506174, 256.4458599265808516, 12.05082362884263425 ) ) ;
#59864=CARTESIAN_POINT ( 'NONE',  ( 203.1705638993064156, 278.7452560544191442, -15.08126533799095093 ) ) ;
#59869=CARTESIAN_POINT ( 'NONE',  ( 152.6992418905140028, 266.1641500988167763, 17.27767170937316621 ) ) ;
#59871=CARTESIAN_POINT ( 'NONE',  ( 190.7779368023172708, 300.2099158256590385, 8.142228434510803581 ) ) ;
#59874=EDGE_LOOP ( 'NONE', ( #34649, #1947, #76716, #42217 ) ) ;
#59881=VERTEX_POINT ( 'NONE', #44845 ) ;
#59882=CARTESIAN_POINT ( 'NONE',  ( 177.5916152172162299, 279.2165670549423453, -16.08229183096581139 ) ) ;
#59883=CARTESIAN_POINT ( 'NONE',  ( 172.1850212007017262, 264.1675647692185294, -16.02513241725109339 ) ) ;
#59884=VERTEX_POINT ( 'NONE', #99077 ) ;
#59885=EDGE_CURVE ( 'NONE', #1543, #39441, #85735, .T. ) ;
#59886=CARTESIAN_POINT ( 'NONE',  ( 158.5760999176972632, 274.9853568892722819, -13.72891502304694633 ) ) ;
#59891=CARTESIAN_POINT ( 'NONE',  ( 156.6755709933906076, 266.6679220207594767, -16.20175030095106905 ) ) ;
#59892=CARTESIAN_POINT ( 'NONE',  ( 147.2494378675467033, 275.6034875578896504, 3.639370109197119341 ) ) ;
#59893=CARTESIAN_POINT ( 'NONE',  ( 206.9942764641839688, 270.1223916185117560, -3.431663675821580828 ) ) ;
#59894=CARTESIAN_POINT ( 'NONE',  ( 190.0607312434325138, 301.4521522931182176, 3.538147641957853473 ) ) ;
#59895=CARTESIAN_POINT ( 'NONE',  ( 192.6470966816805230, 296.9724359471326807, 11.11268290051284424 ) ) ;
#59897=CARTESIAN_POINT ( 'NONE',  ( 191.8398273019305691, 298.3706675282543301, 9.207119386290592900 ) ) ;
#59898=CARTESIAN_POINT ( 'NONE',  ( 147.0660117096331874, 275.9211909828330249, -0.7354350123930680772 ) ) ;
#59899=ORIENTED_EDGE ( 'NONE', *, *, #64637, .T. ) ;
#59901=CARTESIAN_POINT ( 'NONE',  ( 164.9103019330012216, 245.0139736909548560, 2.841678961959298810 ) ) ;
#59903=CARTESIAN_POINT ( 'NONE',  ( -17.42236680055705023, 149.2012482093457777, 0.000000000000000000 ) ) ;
#59904=CARTESIAN_POINT ( 'NONE',  ( 168.0314348872740311, 286.7485367448098827, 3.530950783189123587 ) ) ;
#59906=VERTEX_POINT ( 'NONE', #84392 ) ;
#59907=CARTESIAN_POINT ( 'NONE',  ( 149.1183742800849643, 272.3663947352575860, -12.92061183374618238 ) ) ;
#59909=CARTESIAN_POINT ( 'NONE',  ( 148.9047129658783319, 273.1746572624253986, 9.419085927755277865 ) ) ;
#59911=CARTESIAN_POINT ( 'NONE',  ( 182.4816129607276025, 284.1573356931687044, -15.00314700627625975 ) ) ;
#59915=CARTESIAN_POINT ( 'NONE',  ( 163.4139553296302267, 247.6057220337265505, -10.31482883765270842 ) ) ;
#59917=EDGE_CURVE ( 'NONE', #82871, #68558, #64970, .T. ) ;
#59918=CARTESIAN_POINT ( 'NONE',  ( 155.3072241301414067, 262.2133070116863109, 17.03827534033916535 ) ) ;
#59919=CARTESIAN_POINT ( 'NONE',  ( 56.22356517706937495, 193.2677522451418213, -5.000000000000041744 ) ) ;
#59920=CARTESIAN_POINT ( 'NONE',  ( 112.6505328941731108, 235.8458772461660544, 9.188101187500095079 ) ) ;
#59921=CARTESIAN_POINT ( 'NONE',  ( 199.0756812798354645, 285.8378008023734083, -18.45377816087746936 ) ) ;
#59924=CARTESIAN_POINT ( 'NONE',  ( 33.92367135321775606, 181.2048013555409796, 4.594050593750051981 ) ) ;
#59927=CARTESIAN_POINT ( 'NONE',  ( 195.1474640768281290, 265.6393084148356252, -8.887799905196541062 ) ) ;
#59928=CARTESIAN_POINT ( 'NONE',  ( 181.5271692362856015, 267.5257140134757492, 14.92964428755297135 ) ) ;
#59929=( BOUNDED_SURFACE ( )  B_SPLINE_SURFACE ( 1, 2, ( 
 ( #89052, #90518, #5371, #12993, #37737, #44350, #29172, #82907, #75781, #52451, #38227, #22555, #7345, #76277, #22052, #91489, #51461, #52952, #60536, #14464, #45828, #69143, #45346, #100072, #59539, #53440, #74793, #30659, #6851, #30150, #61542, #67157, #51967, #36254, #76751, #21090, #13479, #68647, #75281, #13965, #68150, #99567, #61035, #84391, #5865, #36750, #92008, #92485, #83902, #82427, #14937, #67659, #98078, #43852, #28656, #98589, #60040, #91006, #6367, #83396, #21568, #44844, #37251, #99076, #29659, #63048, #23032, #93992, #32140, #86409, #17450, #79306, #16940, #40733, #31132, #94485, #46326, #9875, #47826, #1769, #71678, #38738, #23530, #7859, #48358, #62025, #54421, #40230, #85398, #85918, #39715, #78765, #9352, #55920, #92976, #8355, #63544, #2269, #24542, #33151, #55422, #15945, #71172, #53925, #32648, #64051, #86913, #16444, #8845, #25044, #1258, #39224, #84888, #15428, #77251, #47340, #69644, #252, #62527, #46848, #77770, #70131, #744, #31628, #93488, #24046, #54941, #78264, #70643, #57944, #73174, #27062, #74170, #26563, #64558, #88927, #42235, #4762, #96492, #72686, #56446, #66051, #34646, #65546, #96999, #96003, #3278, #41741, #18976, #80295, #49850, #81295, #48867, #11868, #10365, #87439, #3764, #80812, #17972, #57439, #42724, #79800, #41233, #19487, #50343, #73662, #72172, #2778, #4240, #95517, #35644, #33666, #11385, #58434, #35140, #26063, #94995, #88416, #34161, #43228, #56940, #25558, #87926, #27568, #10866, #89409, #18468, #49355, #19960, #50837, #65053, #81787, #12362, #28532, #84281, #68036, #6235, #98957, #59415, #82301, #59924, #37619, #75162, #7223, #5250, #76165, #5737, #45228, #99453, #36624, #67033, #29541, #60413, #76638, #83271, #29056, #91880, #91369, #21932, #52822, #30029, #45715, #83778, #60913, #68530, #66545, #13839, #22433, #37129, #98462, #43730, #53325, #67533, #14339, #90894, #13359, #6742, #14826, #97473, #28039, #89885, #44715, #90395, #58914, #20459, #51333, #21444, #12871, #74673, #36130, #20970, #52330, #51852, #82793, #44224, #75649, #94371, #22921, #63433, #79177, #92862, #54820, #46725, #139, #38107, #31515, #39105, #78146, #32539, #69020, #55309, #17325, #31022, #85800, #40113, #92373, #1140, #8732, #9233, #30534, #47712, #24926, #24434, #61914, #23416, #48231, #15821, #71052, #46207, #99950, #61421, #54306, #1654, #39604, #7731, #32017, #69528, #62926, #70524, #77124, #85274, #84772, #53808, #15308, #55800, #38619, #77653, #8239, #86792, #70019, #635, #62409, #93365, #23922, #16330, #47224, #93877, #86291, #16825, #78650, #49725, #5499, #9756, #28286, #90650, #72045, #57320, #13116, #63927, #74427, #80682, #82551, #2146, #20710, #36382, #97718, #33536, #2649, #21208, #87806, #43975, #17847, #52088, #40616, #64435, #74917, #11257, #79679, #5011, #41111, #35891, #43483, #48748, #95395, #56319, #94866, #71550, #67286, #10741, #18348, #59677, #10242, #33027, #25950, #98213, #56823, #66793, #25424, #87313, #72561, #59162, #49241, #80176, #90136, #41616, #28797, #51597, #3164, #34050, #64939, #95883, #26444, #88292, #18846, #23666, #21696, #92624, #91622, #61674, #15565, #22192, #83533, #15074, #45963, #93114, #99702, #45477, #8001, #76880, #7476, #69284, #46468, #62165, #84530, #77398, #85021, #83034, #30290, #38876, #53575, #14598, #60167, #54066, #53086, #30795, #84040, #29791, #100209, #69780, #13605, #23174, #5993, #61178, #14097, #44478, #22698, #38371, #76411, #98721, #389, #75409, #31277, #6984, #92145, #68284, #36887, #67796, #29305, #37869, #91132, #52579, #68779, #44979, #75920, #6501, #37378, #99205, #60663, #87053, #95135, #94126, #78403, #17588, #32777, #48494, #64694, #86547, #24188, #79435, #1897, #95646, #56060, #32279, #16083, #25700, #94623, #25180, #56580, #55563, #63183, #1400, #78914, #39855, #9500, #40862, #8491, #71809, #70275, #46989, #63686, #40366, #77905, #17078, #2406, #39361, #886, #10000, #33284, #64186, #31765, #62669, #87567, #55071, #54558, #93621, #71305, #48994, #79930, #86057, #85542, #2918, #10490, #16583, #47479, #8984, #41372, #70790, #24681, #47968, #72311, #27195, #13006, #97610, #82443, #50972, #97133, #66187, #26193, #27700, #35281, #89540, #20593, #43866, #20101, #74808, #34287, #28178, #49480, #5386, #81924, #4898, #36272, #41883, #26686, #11010, #51476, #65184, #57574, #43369, #88547, #89064, #42856, #12500, #74316, #59049, #96132, #11512, #66676, #67171, #58568, #57072, #35782, #19113, #90021, #88053, #18601, #80436, #72821, #19616, #11999, #3413, #49989, #80944, #42366, #73300, #3891, #34773, #65674, #73792, #96629, #58084, #50474, #81427, #4381, #14951, #36765, #51981, #59555, #84406, #91018, #75796, #29187, #22071, #99090, #84901, #69157, #53943, #22569, #68659, #37754, #98094, #99582, #6864, #61050, #92500, #15442, #92023, #46341, #5879, #100087, #82920, #77264, #53455, #76763, #7876, #13496, #98604, #44366, #23045, #67675, #60055, #45841, #21581, #60549, #14479, #7358, #38242, #30674, #52466, #83411, #61554, #38753, #30166, #28672, #90532, #13981, #75298, #44856, #6382, #37265, #68164, #91506, #83917, #29674, #76292, #52966, #45360, #85410, #46862, #23544, #77784, #15959, #92990, #8371, #265, #69656, #31146, #62037, #54435, #97220, #4997, #3984, #88649, #27789, #42953, #58662, #43961, #96728, #34386, #89634, #12091, #74899, #66287, #42464, #26295, #35874, #4482, #35376, #66778, #65770, #73398, #11605, #89160, #50085, #19706, #51066, #18698, #82026, #80532, #57170, #73893, #50572, #88150, #27293, #12601, #49579, #11112, #20196, #43468, #34870, #74412, #58175, #81522, #97703, #90117, #5484, #28271, #41981, #59147, #96225, #64797, #20691, #51580, #82537, #72918, #13101, #95742, #3509, #65284, #26789, #81042, #57671, #19215, #55094, #84065, #24213, #41264, #53597, #15591, #7498, #61199, #99226, #92647, #100229, #38898, #93648, #29813, #16110, #79827, #92167, #46492, #912, #53109, #62189, #69802, #70301, #91644, #8515, #86081, #85566, #22718, #84555, #10395, #76900, #31790 ),
 ( #54584, #38396, #60686, #76431, #62692, #22211, #93140, #18001, #31301, #39384, #69308, #15094, #23689, #77426, #47009, #14619, #30815, #68799, #77923, #8025, #45498, #412, #61695, #7004, #48893, #37891, #99727, #30313, #23196, #54088, #45984, #85042, #57466, #27095, #58464, #26094, #89436, #87953, #33700, #81328, #57978, #64593, #3793, #19990, #95545, #56968, #11898, #97029, #35172, #18498, #49384, #65081, #82334, #49883, #74206, #80329, #12903, #72207, #26593, #43261, #73689, #41773, #66083, #3310, #27598, #4273, #10896, #96031, #72719, #34189, #2811, #66578, #73199, #80842, #20495, #88450, #19009, #11412, #4796, #42266, #42757, #34675, #65577, #96525, #50870, #88960, #19515, #81820, #50375, #89915, #12395, #35677, #97502, #28071, #58944, #51367, #14858, #52363, #84802, #82823, #53361, #83309, #22467, #76669, #13871, #44261, #76195, #6771, #53842, #60448, #6271, #69057, #37650, #68560, #30064, #7257, #22953, #45260, #38140, #45745, #43762, #91402, #99985, #14377, #75684, #21001, #30570, #44751, #91911, #37166, #90926, #60953, #61455, #74706, #84311, #67065, #21967, #75194, #5283, #83810, #99486, #68064, #59447, #92405, #36161, #97989, #98988, #90429, #29088, #5769, #28568, #51882, #13390, #36658, #67564, #98498, #52860, #29571, #59954, #21476, #8765, #16364, #55343, #9786, #15342, #32567, #94898, #77688, #62959, #17357, #69562, #78681, #86320, #86825, #7764, #24954, #40646, #1683, #39136, #47255, #85309, #9270, #93909, #25460, #16857, #93403, #77164, #48264, #47744, #40142, #79212, #78176, #23952, #62438, #39634, #664, #70556, #63464, #169, #94400, #31053, #38659, #24463, #1172, #61942, #32046, #55830, #92894, #23447, #71084, #71584, #2179, #54337, #15855, #33061, #46762, #56349, #8271, #63956, #46238, #70049, #31549, #54856, #85834, #4150, #25980, #41142, #48777, #73567, #80207, #64971, #18375, #11290, #88326, #74071, #58344, #43130, #11777, #57849, #26968, #87350, #88829, #96399, #50253, #81697, #4661, #81206, #35553, #95427, #89320, #10272, #66454, #42638, #65953, #97379, #2681, #87836, #72080, #12270, #56850, #49271, #35047, #10775, #49761, #3678, #96905, #27476, #19874, #41649, #72591, #50743, #27946, #19394, #17879, #79709, #3197, #33571, #64465, #34081, #95914, #26474, #80715, #73084, #57350, #65457, #18881, #42149, #34557, #37526, #83184, #60815, #14248, #98369, #99853, #36038, #29941, #51239, #52726, #45622, #91278, #99361, #28958, #82704, #21844, #37038, #83688, #38017, #58828, #13271, #91777, #60322, #28441, #45135, #90301, #76075, #6652, #66939, #51762, #5159, #12776, #89792, #53238, #59837, #36536, #7130, #97869, #20366, #59321, #22341, #75067, #98867, #68928, #43642, #21355, #68432, #20871, #67441, #84193, #44133, #76551, #14740, #29445, #82205, #5646, #74580, #52240, #90800, #13744, #44624, #75558, #6144, #67949, #9142, #63339, #69926, #30935, #62827, #93784, #40524, #47129, #93270, #55706, #24344, #55218, #16737, #94277, #9662, #31924, #24832, #32443, #71459, #78052, #86696, #1045, #62317, #7637, #1558, #543, #78557, #31425, #77556, #47627, #17229, #30437, #40017, #53720, #8641, #61820, #61326, #70435, #86199, #23826, #46115, #48136, #92287, #70955, #39018, #77031, #15728, #92771, #79081, #22836, #15220, #84680, #38528, #85180, #39510, #54720, #23326, #69435, #85702, #16238, #52, #54213, #46630, #8145, #81575, #64339, #49631, #4035, #56224, #65338, #42033, #73452, #94774, #11656, #27345, #88700, #25858, #95302, #12146, #80084, #34924, #10151, #43008, #81090, #26349, #65820, #57721, #41527, #2050, #79587, #96785, #25334, #96276, #89207, #34439, #42517, #72470, #56735, #26846, #80588, #19271, #32932, #33963, #71955, #50137, #11165, #63836, #3558, #10651, #87218, #58226, #72969, #19755, #50623, #3075, #64848, #49149, #57225, #87717, #88201, #17753, #48654, #41017, #2558, #33441, #18253, #18752, #95795, #5534, #91164, #35432, #27835, #13640, #98756, #36922, #66335, #89688, #83571, #74463, #84081, #82084, #59719, #37412, #44513, #58712, #14632, #22224, #21729, #12656, #20246, #97268, #60203, #66826, #51638, #5044, #98249, #74950, #60700, #45018, #29828, #29339, #75444, #6028, #73946, #67836, #83069, #52613, #68318, #91661, #14132, #53124, #43525, #75961, #51122, #4532, #6537, #99243, #35924, #97754, #28324, #59200, #90176, #20751, #82588, #13153, #44007, #36418, #90685, #67325, #28839, #21242, #52119, #30828, #86096, #1443, #85585, #55600, #47024, #7517, #16126, #45513, #931, #94166, #78445, #38912, #31316, #55108, #23707, #61714, #9026, #39402, #77941, #8530, #38410, #61217, #69818, #16621, #54103, #86585, #84569, #47518, #85060, #24230, #39899, #15608, #45999, #70317, #31806, #76444, #62205, #8040, #70831, #62707, #93666, #32323, #63224, #24717, #7020, #37905, #68815, #99742, #93157, #30327, #92181, #77444, #22734, #53612, #46506, #15107, #429, #92660, #76918, #69325, #100246, #23213, #54601, #95689, #48535, #58119, #57111, #41923, #49036, #32820, #34810, #96665, #80475, #25744, #63727, #2447, #17636, #50028, #73340, #1934, #42405, #17120, #71849, #33855, #56624, #79474, #48015, #10537, #18135, #88093, #11547, #78959, #34327, #27234, #10038, #64738, #19153, #71343, #11045, #18642, #88591, #9548, #26728, #3927, #3447, #40901, #33327, #40410, #95175, #80981, #25221, #94663, #56108, #64225, #65711, #49522, #87097, #72859, #87607, #65224, #96167, #79969, #41412, #72357, #2961, #26236, #57612, #90064, #66715, #37306, #27732, #89100, #58600, #91061, #4941, #28723, #99132, #73831, #51518, #90576, #20138, #97649, #75337, #51010, #6429, #21143, #35820, #5920, #14021, #29717, #36809, #12038, #67215, #81961, #19650, #59597, #13536, #20633, #4420, #68206, #50512, #52022, #28216, #35316, #74356, #89575, #21625, #44900, #66229, #75841, #81463, #43409, #5428, #59090, #12536, #42891, #82483, #13047, #82962, #83455, #97165, #67721, #43908, #74847, #36310, #52507, #98138, #44406, #98646, #60096, #29229, #70192, #85977, #46906, #84456, #53501, #70704, #38294, #62587, #68703 ) ),
 .UNSPECIFIED., .F., .F., .T. ) 
 B_SPLINE_SURFACE_WITH_KNOTS ( ( 2, 2 ),
 ( 3, 2, 2, 2, 2, 2, 2, 2, 2, 2, 2, 2, 2, 2, 2, 2, 2, 2, 2, 2, 2, 2, 2, 2, 2, 2, 2, 2, 2, 2, 2, 2, 2, 2, 2, 2, 2, 2, 2, 2, 2, 2, 2, 2, 2, 2, 2, 2, 2, 2, 2, 2, 2, 2, 2, 2, 2, 2, 2, 2, 2, 2, 2, 2, 2, 2, 2, 2, 2, 2, 2, 2, 2, 2, 2, 2, 2, 2, 2, 2, 2, 2, 2, 2, 2, 2, 2, 2, 2, 2, 2, 2, 2, 2, 2, 2, 2, 2, 2, 2, 2, 2, 2, 2, 2, 2, 2, 2, 2, 2, 2, 2, 2, 2, 2, 2, 2, 2, 2, 2, 2, 2, 2, 2, 2, 2, 2, 2, 2, 2, 2, 2, 2, 2, 2, 2, 2, 2, 2, 2, 2, 2, 2, 2, 2, 2, 2, 2, 2, 2, 2, 2, 2, 2, 2, 2, 2, 2, 2, 2, 2, 2, 2, 2, 2, 2, 2, 2, 2, 2, 2, 2, 2, 2, 2, 2, 2, 2, 2, 2, 2, 2, 2, 2, 2, 2, 2, 2, 2, 2, 2, 2, 2, 2, 2, 2, 2, 2, 2, 2, 2, 2, 2, 2, 2, 2, 2, 2, 2, 2, 2, 2, 2, 2, 2, 2, 2, 2, 2, 2, 2, 2, 2, 2, 2, 2, 2, 2, 2, 2, 2, 2, 2, 2, 2, 2, 2, 2, 2, 2, 2, 2, 2, 2, 2, 2, 2, 2, 2, 2, 2, 2, 2, 2, 2, 2, 2, 2, 2, 2, 2, 2, 2, 2, 2, 2, 2, 2, 2, 2, 2, 2, 2, 2, 2, 2, 2, 2, 2, 2, 2, 2, 2, 2, 2, 2, 2, 2, 2, 2, 2, 2, 2, 2, 2, 2, 2, 2, 2, 2, 2, 2, 2, 2, 2, 2, 2, 2, 2, 2, 2, 2, 2, 2, 2, 2, 2, 2, 2, 2, 2, 2, 2, 2, 2, 2, 2, 2, 2, 2, 2, 2, 2, 2, 2, 2, 2, 2, 2, 2, 2, 2, 2, 2, 2, 2, 2, 2, 2, 2, 2, 2, 2, 2, 2, 2, 2, 2, 2, 2, 2, 2, 2, 2, 2, 2, 2, 2, 2, 2, 2, 2, 3 ),
 ( 0.000000000000000000, 1.000000000000000000 ),
 ( 0.000000000000000000, 0.002688172043010752903, 0.005376344086021505805, 0.008064516129032257841, 0.01075268817204301161, 0.01344086021505376365, 0.01612903225806451568, 0.01881720430107526945, 0.02150537634408602322, 0.02419354838709677352, 0.02688172043010752729, 0.02956989247311828106, 0.03225806451612903136, 0.03494623655913978166, 0.03763440860215053890, 0.04032258064516128920, 0.04301075268817204644, 0.04569892473118279674, 0.04838709677419354704, 0.05107526881720430428, 0.05376344086021505458, 0.05645161290322580488, 0.05913978494623656212, 0.06182795698924731242, 0.06451612903225806273, 0.06720430107526881303, 0.06989247311827956333, 0.07258064516129032751, 0.07526881720430107781, 0.07795698924731182811, 0.08064516129032257841, 0.08333333333333332871, 0.08602150537634409289, 0.08870967741935484319, 0.09139784946236559349, 0.09408602150537634379, 0.09677419354838709409, 0.09946236559139784439, 0.1021505376344086086, 0.1048387096774193589, 0.1075268817204301092, 0.1102150537634408595, 0.1129032258064516098, 0.1155913978494623601, 0.1182795698924731242, 0.1209677419354838745, 0.1236559139784946248, 0.1263440860215053752, 0.1290322580645161255, 0.1317204301075268758, 0.1344086021505376261, 0.1370967741935483764, 0.1397849462365591267, 0.1424731182795699047, 0.1451612903225806550, 0.1478494623655914053, 0.1505376344086021556, 0.1532258064516129059, 0.1559139784946236562, 0.1586021505376344065, 0.1612903225806451568, 0.1639784946236559071, 0.1666666666666666574, 0.1693548387096774077, 0.1720430107526881858, 0.1747311827956989361, 0.1774193548387096864, 0.1801075268817204367, 0.1827956989247311870, 0.1854838709677419373, 0.1881720430107526876, 0.1908602150537634379, 0.1935483870967741882, 0.1962365591397849385, 0.1989247311827956888, 0.2016129032258064391, 0.2043010752688172171, 0.2069892473118279674, 0.2096774193548387177, 0.2123655913978494680, 0.2150537634408602183, 0.2177419354838709686, 0.2204301075268817189, 0.2231182795698924692, 0.2258064516129032195, 0.2284946236559139698, 0.2311827956989247201, 0.2338709677419354704, 0.2365591397849462485, 0.2392473118279569988, 0.2419354838709677491, 0.2446236559139784994, 0.2473118279569892497, 0.2500000000000000000, 0.2526881720430107503, 0.2553763440860215006, 0.2580645161290322509, 0.2607526881720430012, 0.2634408602150537515, 0.2661290322580645018, 0.2688172043010752521, 0.2715053763440860024, 0.2741935483870967527, 0.2768817204301075030, 0.2795698924731182533, 0.2822580645161290591, 0.2849462365591398094, 0.2876344086021505597, 0.2903225806451613100, 0.2930107526881720603, 0.2956989247311828106, 0.2983870967741935609, 0.3010752688172043112, 0.3037634408602150615, 0.3064516129032258118, 0.3091397849462365621, 0.3118279569892473124, 0.3145161290322580627, 0.3172043010752688130, 0.3198924731182795633, 0.3225806451612903136, 0.3252688172043010639, 0.3279569892473118142, 0.3306451612903225645, 0.3333333333333333148, 0.3360215053763440651, 0.3387096774193548154, 0.3413978494623655657, 0.3440860215053763715, 0.3467741935483871218, 0.3494623655913978721, 0.3521505376344086224, 0.3548387096774193727, 0.3575268817204301230, 0.3602150537634408733, 0.3629032258064516236, 0.3655913978494623739, 0.3682795698924731242, 0.3709677419354838745, 0.3736559139784946248, 0.3763440860215053752, 0.3790322580645161255, 0.3817204301075268758, 0.3844086021505376261, 0.3870967741935483764, 0.3897849462365591267, 0.3924731182795698770, 0.3951612903225806273, 0.3978494623655913776, 0.4005376344086021279, 0.4032258064516128782, 0.4059139784946236285, 0.4086021505376344343, 0.4112903225806451846, 0.4139784946236559349, 0.4166666666666666852, 0.4193548387096774355, 0.4220430107526881858, 0.4247311827956989361, 0.4274193548387096864, 0.4301075268817204367, 0.4327956989247311870, 0.4354838709677419373, 0.4381720430107526876, 0.4408602150537634379, 0.4435483870967741882, 0.4462365591397849385, 0.4489247311827956888, 0.4516129032258064391, 0.4543010752688171894, 0.4569892473118279397, 0.4596774193548386900, 0.4623655913978494403, 0.4650537634408601906, 0.4677419354838709409, 0.4704301075268817467, 0.4731182795698924970, 0.4758064516129032473, 0.4784946236559139976, 0.4811827956989247479, 0.4838709677419354982, 0.4865591397849462485, 0.4892473118279569988, 0.4919354838709677491, 0.4946236559139784994, 0.4973118279569892497, 0.5000000000000000000, 0.5026881720430107503, 0.5053763440860215006, 0.5080645161290322509, 0.5107526881720430012, 0.5134408602150537515, 0.5161290322580645018, 0.5188172043010752521, 0.5215053763440860024, 0.5241935483870967527, 0.5268817204301075030, 0.5295698924731182533, 0.5322580645161290036, 0.5349462365591397539, 0.5376344086021505042, 0.5403225806451612545, 0.5430107526881720048, 0.5456989247311827551, 0.5483870967741935054, 0.5510752688172042557, 0.5537634408602150060, 0.5564516129032257563, 0.5591397849462365066, 0.5618279569892472569, 0.5645161290322581182, 0.5672043010752688685, 0.5698924731182796188, 0.5725806451612903691, 0.5752688172043011194, 0.5779569892473118697, 0.5806451612903226200, 0.5833333333333333703, 0.5860215053763441206, 0.5887096774193548709, 0.5913978494623656212, 0.5940860215053763715, 0.5967741935483871218, 0.5994623655913978721, 0.6021505376344086224, 0.6048387096774193727, 0.6075268817204301230, 0.6102150537634408733, 0.6129032258064516236, 0.6155913978494623739, 0.6182795698924731242, 0.6209677419354838745, 0.6236559139784946248, 0.6263440860215053752, 0.6290322580645161255, 0.6317204301075268758, 0.6344086021505376261, 0.6370967741935483764, 0.6397849462365591267, 0.6424731182795698770, 0.6451612903225806273, 0.6478494623655913776, 0.6505376344086021279, 0.6532258064516128782, 0.6559139784946236285, 0.6586021505376343788, 0.6612903225806451291, 0.6639784946236558794, 0.6666666666666666297, 0.6693548387096773800, 0.6720430107526881303, 0.6747311827956988806, 0.6774193548387096309, 0.6801075268817203812, 0.6827956989247311315, 0.6854838709677418818, 0.6881720430107527431, 0.6908602150537634934, 0.6935483870967742437, 0.6962365591397849940, 0.6989247311827957443, 0.7016129032258064946, 0.7043010752688172449, 0.7069892473118279952, 0.7096774193548387455, 0.7123655913978494958, 0.7150537634408602461, 0.7177419354838709964, 0.7204301075268817467, 0.7231182795698924970, 0.7258064516129032473, 0.7284946236559139976, 0.7311827956989247479, 0.7338709677419354982, 0.7365591397849462485, 0.7392473118279569988, 0.7419354838709677491, 0.7446236559139784994, 0.7473118279569892497, 0.7500000000000000000, 0.7526881720430107503, 0.7553763440860215006, 0.7580645161290322509, 0.7607526881720430012, 0.7634408602150537515, 0.7661290322580645018, 0.7688172043010752521, 0.7715053763440860024, 0.7741935483870967527, 0.7768817204301075030, 0.7795698924731182533, 0.7822580645161290036, 0.7849462365591397539, 0.7876344086021505042, 0.7903225806451612545, 0.7930107526881720048, 0.7956989247311827551, 0.7983870967741935054, 0.8010752688172042557, 0.8037634408602150060, 0.8064516129032257563, 0.8091397849462365066, 0.8118279569892472569, 0.8145161290322581182, 0.8172043010752688685, 0.8198924731182796188, 0.8225806451612903691, 0.8252688172043011194, 0.8279569892473118697, 0.8306451612903226200, 0.8333333333333333703, 0.8360215053763441206, 0.8387096774193548709, 0.8413978494623656212, 0.8440860215053763715, 0.8467741935483871218, 0.8494623655913978721, 0.8521505376344086224, 0.8548387096774193727, 0.8575268817204301230, 0.8602150537634408733, 0.8629032258064516236, 0.8655913978494623739, 0.8682795698924731242, 0.8709677419354838745, 0.8736559139784946248, 0.8763440860215053752, 0.8790322580645161255, 0.8817204301075268758, 0.8844086021505376261, 0.8870967741935483764, 0.8897849462365591267, 0.8924731182795698770, 0.8951612903225806273, 0.8978494623655913776, 0.9005376344086021279, 0.9032258064516128782, 0.9059139784946236285, 0.9086021505376343788, 0.9112903225806451291, 0.9139784946236558794, 0.9166666666666666297, 0.9193548387096773800, 0.9220430107526881303, 0.9247311827956988806, 0.9274193548387096309, 0.9301075268817203812, 0.9327956989247311315, 0.9354838709677418818, 0.9381720430107527431, 0.9408602150537634934, 0.9435483870967742437, 0.9462365591397849940, 0.9489247311827957443, 0.9516129032258064946, 0.9543010752688172449, 0.9569892473118279952, 0.9596774193548387455, 0.9623655913978494958, 0.9650537634408602461, 0.9677419354838709964, 0.9704301075268817467, 0.9731182795698924970, 0.9758064516129032473, 0.9784946236559139976, 0.9811827956989247479, 0.9838709677419354982, 0.9865591397849462485, 0.9892473118279569988, 0.9919354838709677491, 0.9946236559139784994, 0.9973118279569892497, 1.000000000000000000 ),
 .UNSPECIFIED. ) 
 GEOMETRIC_REPRESENTATION_ITEM ( )  RATIONAL_B_SPLINE_SURFACE ( (
 ( 1.000000000000000000, 0.8660254037844387076, 1.000000000000000000, 0.8660254037844387076, 1.000000000000000000, 0.8660254037844387076, 1.000000000000000000, 0.8660254037844387076, 1.000000000000000000, 0.8660254037844387076, 1.000000000000000000, 0.8660254037844387076, 1.000000000000000000, 0.8660254037844387076, 1.000000000000000000, 0.8660254037844387076, 1.000000000000000000, 0.8660254037844387076, 1.000000000000000000, 0.8660254037844387076, 1.000000000000000000, 0.8660254037844387076, 1.000000000000000000, 0.8660254037844387076, 1.000000000000000000, 0.8660254037844387076, 1.000000000000000000, 0.8660254037844387076, 1.000000000000000000, 0.8660254037844387076, 1.000000000000000000, 0.8660254037844387076, 1.000000000000000000, 0.8660254037844387076, 1.000000000000000000, 0.8660254037844387076, 1.000000000000000000, 0.8660254037844387076, 1.000000000000000000, 0.8660254037844387076, 1.000000000000000000, 0.8660254037844387076, 1.000000000000000000, 0.8660254037844387076, 1.000000000000000000, 0.8660254037844387076, 1.000000000000000000, 0.8660254037844387076, 1.000000000000000000, 0.8660254037844387076, 1.000000000000000000, 0.8660254037844387076, 1.000000000000000000, 0.8660254037844387076, 1.000000000000000000, 0.8660254037844387076, 1.000000000000000000, 0.8660254037844387076, 1.000000000000000000, 0.8660254037844387076, 1.000000000000000000, 0.8660254037844387076, 1.000000000000000000, 0.8660254037844387076, 1.000000000000000000, 0.8660254037844387076, 1.000000000000000000, 0.8660254037844387076, 1.000000000000000000, 0.8660254037844387076, 1.000000000000000000, 0.8660254037844387076, 1.000000000000000000, 0.8660254037844387076, 1.000000000000000000, 0.8660254037844387076, 1.000000000000000000, 0.8660254037844387076, 1.000000000000000000, 0.8660254037844387076, 1.000000000000000000, 0.8660254037844387076, 1.000000000000000000, 0.8660254037844387076, 1.000000000000000000, 0.8660254037844387076, 1.000000000000000000, 0.8660254037844387076, 1.000000000000000000, 0.8660254037844387076, 1.000000000000000000, 0.8660254037844387076, 1.000000000000000000, 0.8660254037844387076, 1.000000000000000000, 0.8660254037844387076, 1.000000000000000000, 0.8660254037844387076, 1.000000000000000000, 0.8660254037844387076, 1.000000000000000000, 0.8660254037844387076, 1.000000000000000000, 0.8660254037844387076, 1.000000000000000000, 0.8660254037844387076, 1.000000000000000000, 0.8660254037844387076, 1.000000000000000000, 0.8660254037844387076, 1.000000000000000000, 0.8660254037844387076, 1.000000000000000000, 0.8660254037844387076, 1.000000000000000000, 0.8660254037844387076, 1.000000000000000000, 0.8660254037844387076, 1.000000000000000000, 0.8660254037844387076, 1.000000000000000000, 0.8660254037844387076, 1.000000000000000000, 0.8660254037844387076, 1.000000000000000000, 0.8660254037844387076, 1.000000000000000000, 0.8660254037844387076, 1.000000000000000000, 0.8660254037844387076, 1.000000000000000000, 0.8660254037844387076, 1.000000000000000000, 0.8660254037844387076, 1.000000000000000000, 0.8660254037844387076, 1.000000000000000000, 0.8660254037844387076, 1.000000000000000000, 0.8660254037844387076, 1.000000000000000000, 0.8660254037844387076, 1.000000000000000000, 0.8660254037844387076, 1.000000000000000000, 0.8660254037844387076, 1.000000000000000000, 0.8660254037844387076, 1.000000000000000000, 0.8660254037844387076, 1.000000000000000000, 0.8660254037844387076, 1.000000000000000000, 0.8660254037844387076, 1.000000000000000000, 0.8660254037844387076, 1.000000000000000000, 0.8660254037844387076, 1.000000000000000000, 0.8660254037844387076, 1.000000000000000000, 0.8660254037844387076, 1.000000000000000000, 0.8660254037844387076, 1.000000000000000000, 0.8660254037844387076, 1.000000000000000000, 0.8660254037844387076, 1.000000000000000000, 0.8660254037844387076, 1.000000000000000000, 0.8660254037844387076, 1.000000000000000000, 0.8660254037844387076, 1.000000000000000000, 0.8660254037844387076, 1.000000000000000000, 0.8660254037844387076, 1.000000000000000000, 0.8660254037844387076, 1.000000000000000000, 0.8660254037844387076, 1.000000000000000000, 0.8660254037844387076, 1.000000000000000000, 0.8660254037844387076, 1.000000000000000000, 0.8660254037844387076, 1.000000000000000000, 0.8660254037844387076, 1.000000000000000000, 0.8660254037844387076, 1.000000000000000000, 0.8660254037844387076, 1.000000000000000000, 0.8660254037844387076, 1.000000000000000000, 0.8660254037844387076, 1.000000000000000000, 0.8660254037844387076, 1.000000000000000000, 0.8660254037844387076, 1.000000000000000000, 0.8660254037844387076, 1.000000000000000000, 0.8660254037844387076, 1.000000000000000000, 0.8660254037844387076, 1.000000000000000000, 0.8660254037844387076, 1.000000000000000000, 0.8660254037844387076, 1.000000000000000000, 0.8660254037844387076, 1.000000000000000000, 0.8660254037844387076, 1.000000000000000000, 0.8660254037844387076, 1.000000000000000000, 0.8660254037844387076, 1.000000000000000000, 0.8660254037844387076, 1.000000000000000000, 0.8660254037844387076, 1.000000000000000000, 0.8660254037844387076, 1.000000000000000000, 0.8660254037844387076, 1.000000000000000000, 0.8660254037844387076, 1.000000000000000000, 0.8660254037844387076, 1.000000000000000000, 0.8660254037844387076, 1.000000000000000000, 0.8660254037844387076, 1.000000000000000000, 0.8660254037844387076, 1.000000000000000000, 0.8660254037844387076, 1.000000000000000000, 0.8660254037844387076, 1.000000000000000000, 0.8660254037844387076, 1.000000000000000000, 0.8660254037844387076, 1.000000000000000000, 0.8660254037844387076, 1.000000000000000000, 0.8660254037844387076, 1.000000000000000000, 0.8660254037844387076, 1.000000000000000000, 0.8660254037844387076, 1.000000000000000000, 0.8660254037844387076, 1.000000000000000000, 0.8660254037844387076, 1.000000000000000000, 0.8660254037844387076, 1.000000000000000000, 0.8660254037844387076, 1.000000000000000000, 0.8660254037844387076, 1.000000000000000000, 0.8660254037844387076, 1.000000000000000000, 0.8660254037844387076, 1.000000000000000000, 0.8660254037844387076, 1.000000000000000000, 0.8660254037844387076, 1.000000000000000000, 0.8660254037844387076, 1.000000000000000000, 0.8660254037844387076, 1.000000000000000000, 0.8660254037844387076, 1.000000000000000000, 0.8660254037844387076, 1.000000000000000000, 0.8660254037844387076, 1.000000000000000000, 0.8660254037844387076, 1.000000000000000000, 0.8660254037844387076, 1.000000000000000000, 0.8660254037844387076, 1.000000000000000000, 0.8660254037844387076, 1.000000000000000000, 0.8660254037844387076, 1.000000000000000000, 0.8660254037844387076, 1.000000000000000000, 0.8660254037844387076, 1.000000000000000000, 0.8660254037844387076, 1.000000000000000000, 0.8660254037844387076, 1.000000000000000000, 0.8660254037844387076, 1.000000000000000000, 0.8660254037844387076, 1.000000000000000000, 0.8660254037844387076, 1.000000000000000000, 0.8660254037844387076, 1.000000000000000000, 0.8660254037844387076, 1.000000000000000000, 0.8660254037844387076, 1.000000000000000000, 0.8660254037844387076, 1.000000000000000000, 0.8660254037844387076, 1.000000000000000000, 0.8660254037844387076, 1.000000000000000000, 0.8660254037844387076, 1.000000000000000000, 0.8660254037844387076, 1.000000000000000000, 0.8660254037844387076, 1.000000000000000000, 0.8660254037844387076, 1.000000000000000000, 0.8660254037844387076, 1.000000000000000000, 0.8660254037844387076, 1.000000000000000000, 0.8660254037844387076, 1.000000000000000000, 0.8660254037844387076, 1.000000000000000000, 0.8660254037844387076, 1.000000000000000000, 0.8660254037844387076, 1.000000000000000000, 0.8660254037844387076, 1.000000000000000000, 0.8660254037844387076, 1.000000000000000000, 0.8660254037844387076, 1.000000000000000000, 0.8660254037844387076, 1.000000000000000000, 0.8660254037844387076, 1.000000000000000000, 0.8660254037844387076, 1.000000000000000000, 0.8660254037844387076, 1.000000000000000000, 0.8660254037844387076, 1.000000000000000000, 0.8660254037844387076, 1.000000000000000000, 0.8660254037844387076, 1.000000000000000000, 0.8660254037844387076, 1.000000000000000000, 0.8660254037844387076, 1.000000000000000000, 0.8660254037844387076, 1.000000000000000000, 0.8660254037844387076, 1.000000000000000000, 0.8660254037844387076, 1.000000000000000000, 0.8660254037844387076, 1.000000000000000000, 0.8660254037844387076, 1.000000000000000000, 0.8660254037844387076, 1.000000000000000000, 0.8660254037844387076, 1.000000000000000000, 0.8660254037844387076, 1.000000000000000000, 0.8660254037844387076, 1.000000000000000000, 0.8660254037844387076, 1.000000000000000000, 0.8660254037844387076, 1.000000000000000000, 0.8660254037844387076, 1.000000000000000000, 0.8660254037844387076, 1.000000000000000000, 0.8660254037844387076, 1.000000000000000000, 0.8660254037844387076, 1.000000000000000000, 0.8660254037844387076, 1.000000000000000000, 0.8660254037844387076, 1.000000000000000000, 0.8660254037844387076, 1.000000000000000000, 0.8660254037844387076, 1.000000000000000000, 0.8660254037844387076, 1.000000000000000000, 0.8660254037844387076, 1.000000000000000000, 0.8660254037844387076, 1.000000000000000000, 0.8660254037844387076, 1.000000000000000000, 0.8660254037844387076, 1.000000000000000000, 0.8660254037844387076, 1.000000000000000000, 0.8660254037844387076, 1.000000000000000000, 0.8660254037844387076, 1.000000000000000000, 0.8660254037844387076, 1.000000000000000000, 0.8660254037844387076, 1.000000000000000000, 0.8660254037844387076, 1.000000000000000000, 0.8660254037844387076, 1.000000000000000000, 0.8660254037844387076, 1.000000000000000000, 0.8660254037844387076, 1.000000000000000000, 0.8660254037844387076, 1.000000000000000000, 0.8660254037844387076, 1.000000000000000000, 0.8660254037844387076, 1.000000000000000000, 0.8660254037844387076, 1.000000000000000000, 0.8660254037844387076, 1.000000000000000000, 0.8660254037844387076, 1.000000000000000000, 0.8660254037844387076, 1.000000000000000000, 0.8660254037844387076, 1.000000000000000000, 0.8660254037844387076, 1.000000000000000000, 0.8660254037844387076, 1.000000000000000000, 0.8660254037844387076, 1.000000000000000000, 0.8660254037844387076, 1.000000000000000000, 0.8660254037844387076, 1.000000000000000000, 0.8660254037844387076, 1.000000000000000000, 0.8660254037844387076, 1.000000000000000000, 0.8660254037844387076, 1.000000000000000000, 0.8660254037844387076, 1.000000000000000000, 0.8660254037844387076, 1.000000000000000000, 0.8660254037844387076, 1.000000000000000000, 0.8660254037844387076, 1.000000000000000000, 0.8660254037844387076, 1.000000000000000000, 0.8660254037844387076, 1.000000000000000000, 0.8660254037844387076, 1.000000000000000000, 0.8660254037844387076, 1.000000000000000000, 0.8660254037844387076, 1.000000000000000000, 0.8660254037844387076, 1.000000000000000000, 0.8660254037844387076, 1.000000000000000000, 0.8660254037844387076, 1.000000000000000000, 0.8660254037844387076, 1.000000000000000000, 0.8660254037844387076, 1.000000000000000000, 0.8660254037844387076, 1.000000000000000000, 0.8660254037844387076, 1.000000000000000000, 0.8660254037844387076, 1.000000000000000000, 0.8660254037844387076, 1.000000000000000000, 0.8660254037844387076, 1.000000000000000000, 0.8660254037844387076, 1.000000000000000000, 0.8660254037844387076, 1.000000000000000000, 0.8660254037844387076, 1.000000000000000000, 0.8660254037844387076, 1.000000000000000000, 0.8660254037844387076, 1.000000000000000000, 0.8660254037844387076, 1.000000000000000000, 0.8660254037844387076, 1.000000000000000000, 0.8660254037844387076, 1.000000000000000000, 0.8660254037844387076, 1.000000000000000000, 0.8660254037844387076, 1.000000000000000000, 0.8660254037844387076, 1.000000000000000000, 0.8660254037844387076, 1.000000000000000000, 0.8660254037844387076, 1.000000000000000000, 0.8660254037844387076, 1.000000000000000000, 0.8660254037844387076, 1.000000000000000000, 0.8660254037844387076, 1.000000000000000000, 0.8660254037844387076, 1.000000000000000000, 0.8660254037844387076, 1.000000000000000000, 0.8660254037844387076, 1.000000000000000000, 0.8660254037844387076, 1.000000000000000000, 0.8660254037844387076, 1.000000000000000000, 0.8660254037844387076, 1.000000000000000000, 0.8660254037844387076, 1.000000000000000000, 0.8660254037844387076, 1.000000000000000000, 0.8660254037844387076, 1.000000000000000000, 0.8660254037844387076, 1.000000000000000000, 0.8660254037844387076, 1.000000000000000000, 0.8660254037844387076, 1.000000000000000000, 0.8660254037844387076, 1.000000000000000000, 0.8660254037844387076, 1.000000000000000000, 0.8660254037844387076, 1.000000000000000000, 0.8660254037844387076, 1.000000000000000000, 0.8660254037844387076, 1.000000000000000000, 0.8660254037844387076, 1.000000000000000000, 0.8660254037844387076, 1.000000000000000000, 0.8660254037844387076, 1.000000000000000000, 0.8660254037844387076, 1.000000000000000000, 0.8660254037844387076, 1.000000000000000000, 0.8660254037844387076, 1.000000000000000000, 0.8660254037844387076, 1.000000000000000000, 0.8660254037844387076, 1.000000000000000000, 0.8660254037844387076, 1.000000000000000000, 0.8660254037844387076, 1.000000000000000000, 0.8660254037844387076, 1.000000000000000000, 0.8660254037844387076, 1.000000000000000000, 0.8660254037844387076, 1.000000000000000000, 0.8660254037844387076, 1.000000000000000000, 0.8660254037844387076, 1.000000000000000000, 0.8660254037844387076, 1.000000000000000000, 0.8660254037844387076, 1.000000000000000000, 0.8660254037844387076, 1.000000000000000000, 0.8660254037844387076, 1.000000000000000000, 0.8660254037844387076, 1.000000000000000000, 0.8660254037844387076, 1.000000000000000000, 0.8660254037844387076, 1.000000000000000000, 0.8660254037844387076, 1.000000000000000000, 0.8660254037844387076, 1.000000000000000000, 0.8660254037844387076, 1.000000000000000000, 0.8660254037844387076, 1.000000000000000000, 0.8660254037844387076, 1.000000000000000000, 0.8660254037844387076, 1.000000000000000000, 0.8660254037844387076, 1.000000000000000000, 0.8660254037844387076, 1.000000000000000000, 0.8660254037844387076, 1.000000000000000000, 0.8660254037844387076, 1.000000000000000000, 0.8660254037844387076, 1.000000000000000000, 0.8660254037844387076, 1.000000000000000000, 0.8660254037844387076, 1.000000000000000000, 0.8660254037844387076, 1.000000000000000000, 0.8660254037844387076, 1.000000000000000000, 0.8660254037844387076, 1.000000000000000000, 0.8660254037844387076, 1.000000000000000000, 0.8660254037844387076, 1.000000000000000000, 0.8660254037844387076, 1.000000000000000000, 0.8660254037844387076, 1.000000000000000000, 0.8660254037844387076, 1.000000000000000000, 0.8660254037844387076, 1.000000000000000000, 0.8660254037844387076, 1.000000000000000000, 0.8660254037844387076, 1.000000000000000000, 0.8660254037844387076, 1.000000000000000000, 0.8660254037844387076, 1.000000000000000000, 0.8660254037844387076, 1.000000000000000000, 0.8660254037844387076, 1.000000000000000000, 0.8660254037844387076, 1.000000000000000000, 0.8660254037844387076, 1.000000000000000000, 0.8660254037844387076, 1.000000000000000000, 0.8660254037844387076, 1.000000000000000000, 0.8660254037844387076, 1.000000000000000000, 0.8660254037844387076, 1.000000000000000000, 0.8660254037844387076, 1.000000000000000000, 0.8660254037844387076, 1.000000000000000000, 0.8660254037844387076, 1.000000000000000000, 0.8660254037844387076, 1.000000000000000000, 0.8660254037844387076, 1.000000000000000000, 0.8660254037844387076, 1.000000000000000000, 0.8660254037844387076, 1.000000000000000000, 0.8660254037844387076, 1.000000000000000000, 0.8660254037844387076, 1.000000000000000000, 0.8660254037844387076, 1.000000000000000000, 0.8660254037844387076, 1.000000000000000000, 0.8660254037844387076, 1.000000000000000000, 0.8660254037844387076, 1.000000000000000000, 0.8660254037844387076, 1.000000000000000000, 0.8660254037844387076, 1.000000000000000000, 0.8660254037844387076, 1.000000000000000000, 0.8660254037844387076, 1.000000000000000000, 0.8660254037844387076, 1.000000000000000000, 0.8660254037844387076, 1.000000000000000000, 0.8660254037844387076, 1.000000000000000000, 0.8660254037844387076, 1.000000000000000000, 0.8660254037844387076, 1.000000000000000000, 0.8660254037844387076, 1.000000000000000000, 0.8660254037844387076, 1.000000000000000000, 0.8660254037844387076, 1.000000000000000000, 0.8660254037844387076, 1.000000000000000000, 0.8660254037844387076, 1.000000000000000000, 0.8660254037844387076, 1.000000000000000000, 0.8660254037844387076, 1.000000000000000000, 0.8660254037844387076, 1.000000000000000000, 0.8660254037844387076, 1.000000000000000000, 0.8660254037844387076, 1.000000000000000000, 0.8660254037844387076, 1.000000000000000000, 0.8660254037844387076, 1.000000000000000000),
 ( 1.000000000000000000, 0.8660254037844387076, 1.000000000000000000, 0.8660254037844387076, 1.000000000000000000, 0.8660254037844387076, 1.000000000000000000, 0.8660254037844387076, 1.000000000000000000, 0.8660254037844387076, 1.000000000000000000, 0.8660254037844387076, 1.000000000000000000, 0.8660254037844387076, 1.000000000000000000, 0.8660254037844387076, 1.000000000000000000, 0.8660254037844387076, 1.000000000000000000, 0.8660254037844387076, 1.000000000000000000, 0.8660254037844387076, 1.000000000000000000, 0.8660254037844387076, 1.000000000000000000, 0.8660254037844387076, 1.000000000000000000, 0.8660254037844387076, 1.000000000000000000, 0.8660254037844387076, 1.000000000000000000, 0.8660254037844387076, 1.000000000000000000, 0.8660254037844387076, 1.000000000000000000, 0.8660254037844387076, 1.000000000000000000, 0.8660254037844387076, 1.000000000000000000, 0.8660254037844387076, 1.000000000000000000, 0.8660254037844387076, 1.000000000000000000, 0.8660254037844387076, 1.000000000000000000, 0.8660254037844387076, 1.000000000000000000, 0.8660254037844387076, 1.000000000000000000, 0.8660254037844387076, 1.000000000000000000, 0.8660254037844387076, 1.000000000000000000, 0.8660254037844387076, 1.000000000000000000, 0.8660254037844387076, 1.000000000000000000, 0.8660254037844387076, 1.000000000000000000, 0.8660254037844387076, 1.000000000000000000, 0.8660254037844387076, 1.000000000000000000, 0.8660254037844387076, 1.000000000000000000, 0.8660254037844387076, 1.000000000000000000, 0.8660254037844387076, 1.000000000000000000, 0.8660254037844387076, 1.000000000000000000, 0.8660254037844387076, 1.000000000000000000, 0.8660254037844387076, 1.000000000000000000, 0.8660254037844387076, 1.000000000000000000, 0.8660254037844387076, 1.000000000000000000, 0.8660254037844387076, 1.000000000000000000, 0.8660254037844387076, 1.000000000000000000, 0.8660254037844387076, 1.000000000000000000, 0.8660254037844387076, 1.000000000000000000, 0.8660254037844387076, 1.000000000000000000, 0.8660254037844387076, 1.000000000000000000, 0.8660254037844387076, 1.000000000000000000, 0.8660254037844387076, 1.000000000000000000, 0.8660254037844387076, 1.000000000000000000, 0.8660254037844387076, 1.000000000000000000, 0.8660254037844387076, 1.000000000000000000, 0.8660254037844387076, 1.000000000000000000, 0.8660254037844387076, 1.000000000000000000, 0.8660254037844387076, 1.000000000000000000, 0.8660254037844387076, 1.000000000000000000, 0.8660254037844387076, 1.000000000000000000, 0.8660254037844387076, 1.000000000000000000, 0.8660254037844387076, 1.000000000000000000, 0.8660254037844387076, 1.000000000000000000, 0.8660254037844387076, 1.000000000000000000, 0.8660254037844387076, 1.000000000000000000, 0.8660254037844387076, 1.000000000000000000, 0.8660254037844387076, 1.000000000000000000, 0.8660254037844387076, 1.000000000000000000, 0.8660254037844387076, 1.000000000000000000, 0.8660254037844387076, 1.000000000000000000, 0.8660254037844387076, 1.000000000000000000, 0.8660254037844387076, 1.000000000000000000, 0.8660254037844387076, 1.000000000000000000, 0.8660254037844387076, 1.000000000000000000, 0.8660254037844387076, 1.000000000000000000, 0.8660254037844387076, 1.000000000000000000, 0.8660254037844387076, 1.000000000000000000, 0.8660254037844387076, 1.000000000000000000, 0.8660254037844387076, 1.000000000000000000, 0.8660254037844387076, 1.000000000000000000, 0.8660254037844387076, 1.000000000000000000, 0.8660254037844387076, 1.000000000000000000, 0.8660254037844387076, 1.000000000000000000, 0.8660254037844387076, 1.000000000000000000, 0.8660254037844387076, 1.000000000000000000, 0.8660254037844387076, 1.000000000000000000, 0.8660254037844387076, 1.000000000000000000, 0.8660254037844387076, 1.000000000000000000, 0.8660254037844387076, 1.000000000000000000, 0.8660254037844387076, 1.000000000000000000, 0.8660254037844387076, 1.000000000000000000, 0.8660254037844387076, 1.000000000000000000, 0.8660254037844387076, 1.000000000000000000, 0.8660254037844387076, 1.000000000000000000, 0.8660254037844387076, 1.000000000000000000, 0.8660254037844387076, 1.000000000000000000, 0.8660254037844387076, 1.000000000000000000, 0.8660254037844387076, 1.000000000000000000, 0.8660254037844387076, 1.000000000000000000, 0.8660254037844387076, 1.000000000000000000, 0.8660254037844387076, 1.000000000000000000, 0.8660254037844387076, 1.000000000000000000, 0.8660254037844387076, 1.000000000000000000, 0.8660254037844387076, 1.000000000000000000, 0.8660254037844387076, 1.000000000000000000, 0.8660254037844387076, 1.000000000000000000, 0.8660254037844387076, 1.000000000000000000, 0.8660254037844387076, 1.000000000000000000, 0.8660254037844387076, 1.000000000000000000, 0.8660254037844387076, 1.000000000000000000, 0.8660254037844387076, 1.000000000000000000, 0.8660254037844387076, 1.000000000000000000, 0.8660254037844387076, 1.000000000000000000, 0.8660254037844387076, 1.000000000000000000, 0.8660254037844387076, 1.000000000000000000, 0.8660254037844387076, 1.000000000000000000, 0.8660254037844387076, 1.000000000000000000, 0.8660254037844387076, 1.000000000000000000, 0.8660254037844387076, 1.000000000000000000, 0.8660254037844387076, 1.000000000000000000, 0.8660254037844387076, 1.000000000000000000, 0.8660254037844387076, 1.000000000000000000, 0.8660254037844387076, 1.000000000000000000, 0.8660254037844387076, 1.000000000000000000, 0.8660254037844387076, 1.000000000000000000, 0.8660254037844387076, 1.000000000000000000, 0.8660254037844387076, 1.000000000000000000, 0.8660254037844387076, 1.000000000000000000, 0.8660254037844387076, 1.000000000000000000, 0.8660254037844387076, 1.000000000000000000, 0.8660254037844387076, 1.000000000000000000, 0.8660254037844387076, 1.000000000000000000, 0.8660254037844387076, 1.000000000000000000, 0.8660254037844387076, 1.000000000000000000, 0.8660254037844387076, 1.000000000000000000, 0.8660254037844387076, 1.000000000000000000, 0.8660254037844387076, 1.000000000000000000, 0.8660254037844387076, 1.000000000000000000, 0.8660254037844387076, 1.000000000000000000, 0.8660254037844387076, 1.000000000000000000, 0.8660254037844387076, 1.000000000000000000, 0.8660254037844387076, 1.000000000000000000, 0.8660254037844387076, 1.000000000000000000, 0.8660254037844387076, 1.000000000000000000, 0.8660254037844387076, 1.000000000000000000, 0.8660254037844387076, 1.000000000000000000, 0.8660254037844387076, 1.000000000000000000, 0.8660254037844387076, 1.000000000000000000, 0.8660254037844387076, 1.000000000000000000, 0.8660254037844387076, 1.000000000000000000, 0.8660254037844387076, 1.000000000000000000, 0.8660254037844387076, 1.000000000000000000, 0.8660254037844387076, 1.000000000000000000, 0.8660254037844387076, 1.000000000000000000, 0.8660254037844387076, 1.000000000000000000, 0.8660254037844387076, 1.000000000000000000, 0.8660254037844387076, 1.000000000000000000, 0.8660254037844387076, 1.000000000000000000, 0.8660254037844387076, 1.000000000000000000, 0.8660254037844387076, 1.000000000000000000, 0.8660254037844387076, 1.000000000000000000, 0.8660254037844387076, 1.000000000000000000, 0.8660254037844387076, 1.000000000000000000, 0.8660254037844387076, 1.000000000000000000, 0.8660254037844387076, 1.000000000000000000, 0.8660254037844387076, 1.000000000000000000, 0.8660254037844387076, 1.000000000000000000, 0.8660254037844387076, 1.000000000000000000, 0.8660254037844387076, 1.000000000000000000, 0.8660254037844387076, 1.000000000000000000, 0.8660254037844387076, 1.000000000000000000, 0.8660254037844387076, 1.000000000000000000, 0.8660254037844387076, 1.000000000000000000, 0.8660254037844387076, 1.000000000000000000, 0.8660254037844387076, 1.000000000000000000, 0.8660254037844387076, 1.000000000000000000, 0.8660254037844387076, 1.000000000000000000, 0.8660254037844387076, 1.000000000000000000, 0.8660254037844387076, 1.000000000000000000, 0.8660254037844387076, 1.000000000000000000, 0.8660254037844387076, 1.000000000000000000, 0.8660254037844387076, 1.000000000000000000, 0.8660254037844387076, 1.000000000000000000, 0.8660254037844387076, 1.000000000000000000, 0.8660254037844387076, 1.000000000000000000, 0.8660254037844387076, 1.000000000000000000, 0.8660254037844387076, 1.000000000000000000, 0.8660254037844387076, 1.000000000000000000, 0.8660254037844387076, 1.000000000000000000, 0.8660254037844387076, 1.000000000000000000, 0.8660254037844387076, 1.000000000000000000, 0.8660254037844387076, 1.000000000000000000, 0.8660254037844387076, 1.000000000000000000, 0.8660254037844387076, 1.000000000000000000, 0.8660254037844387076, 1.000000000000000000, 0.8660254037844387076, 1.000000000000000000, 0.8660254037844387076, 1.000000000000000000, 0.8660254037844387076, 1.000000000000000000, 0.8660254037844387076, 1.000000000000000000, 0.8660254037844387076, 1.000000000000000000, 0.8660254037844387076, 1.000000000000000000, 0.8660254037844387076, 1.000000000000000000, 0.8660254037844387076, 1.000000000000000000, 0.8660254037844387076, 1.000000000000000000, 0.8660254037844387076, 1.000000000000000000, 0.8660254037844387076, 1.000000000000000000, 0.8660254037844387076, 1.000000000000000000, 0.8660254037844387076, 1.000000000000000000, 0.8660254037844387076, 1.000000000000000000, 0.8660254037844387076, 1.000000000000000000, 0.8660254037844387076, 1.000000000000000000, 0.8660254037844387076, 1.000000000000000000, 0.8660254037844387076, 1.000000000000000000, 0.8660254037844387076, 1.000000000000000000, 0.8660254037844387076, 1.000000000000000000, 0.8660254037844387076, 1.000000000000000000, 0.8660254037844387076, 1.000000000000000000, 0.8660254037844387076, 1.000000000000000000, 0.8660254037844387076, 1.000000000000000000, 0.8660254037844387076, 1.000000000000000000, 0.8660254037844387076, 1.000000000000000000, 0.8660254037844387076, 1.000000000000000000, 0.8660254037844387076, 1.000000000000000000, 0.8660254037844387076, 1.000000000000000000, 0.8660254037844387076, 1.000000000000000000, 0.8660254037844387076, 1.000000000000000000, 0.8660254037844387076, 1.000000000000000000, 0.8660254037844387076, 1.000000000000000000, 0.8660254037844387076, 1.000000000000000000, 0.8660254037844387076, 1.000000000000000000, 0.8660254037844387076, 1.000000000000000000, 0.8660254037844387076, 1.000000000000000000, 0.8660254037844387076, 1.000000000000000000, 0.8660254037844387076, 1.000000000000000000, 0.8660254037844387076, 1.000000000000000000, 0.8660254037844387076, 1.000000000000000000, 0.8660254037844387076, 1.000000000000000000, 0.8660254037844387076, 1.000000000000000000, 0.8660254037844387076, 1.000000000000000000, 0.8660254037844387076, 1.000000000000000000, 0.8660254037844387076, 1.000000000000000000, 0.8660254037844387076, 1.000000000000000000, 0.8660254037844387076, 1.000000000000000000, 0.8660254037844387076, 1.000000000000000000, 0.8660254037844387076, 1.000000000000000000, 0.8660254037844387076, 1.000000000000000000, 0.8660254037844387076, 1.000000000000000000, 0.8660254037844387076, 1.000000000000000000, 0.8660254037844387076, 1.000000000000000000, 0.8660254037844387076, 1.000000000000000000, 0.8660254037844387076, 1.000000000000000000, 0.8660254037844387076, 1.000000000000000000, 0.8660254037844387076, 1.000000000000000000, 0.8660254037844387076, 1.000000000000000000, 0.8660254037844387076, 1.000000000000000000, 0.8660254037844387076, 1.000000000000000000, 0.8660254037844387076, 1.000000000000000000, 0.8660254037844387076, 1.000000000000000000, 0.8660254037844387076, 1.000000000000000000, 0.8660254037844387076, 1.000000000000000000, 0.8660254037844387076, 1.000000000000000000, 0.8660254037844387076, 1.000000000000000000, 0.8660254037844387076, 1.000000000000000000, 0.8660254037844387076, 1.000000000000000000, 0.8660254037844387076, 1.000000000000000000, 0.8660254037844387076, 1.000000000000000000, 0.8660254037844387076, 1.000000000000000000, 0.8660254037844387076, 1.000000000000000000, 0.8660254037844387076, 1.000000000000000000, 0.8660254037844387076, 1.000000000000000000, 0.8660254037844387076, 1.000000000000000000, 0.8660254037844387076, 1.000000000000000000, 0.8660254037844387076, 1.000000000000000000, 0.8660254037844387076, 1.000000000000000000, 0.8660254037844387076, 1.000000000000000000, 0.8660254037844387076, 1.000000000000000000, 0.8660254037844387076, 1.000000000000000000, 0.8660254037844387076, 1.000000000000000000, 0.8660254037844387076, 1.000000000000000000, 0.8660254037844387076, 1.000000000000000000, 0.8660254037844387076, 1.000000000000000000, 0.8660254037844387076, 1.000000000000000000, 0.8660254037844387076, 1.000000000000000000, 0.8660254037844387076, 1.000000000000000000, 0.8660254037844387076, 1.000000000000000000, 0.8660254037844387076, 1.000000000000000000, 0.8660254037844387076, 1.000000000000000000, 0.8660254037844387076, 1.000000000000000000, 0.8660254037844387076, 1.000000000000000000, 0.8660254037844387076, 1.000000000000000000, 0.8660254037844387076, 1.000000000000000000, 0.8660254037844387076, 1.000000000000000000, 0.8660254037844387076, 1.000000000000000000, 0.8660254037844387076, 1.000000000000000000, 0.8660254037844387076, 1.000000000000000000, 0.8660254037844387076, 1.000000000000000000, 0.8660254037844387076, 1.000000000000000000, 0.8660254037844387076, 1.000000000000000000, 0.8660254037844387076, 1.000000000000000000, 0.8660254037844387076, 1.000000000000000000, 0.8660254037844387076, 1.000000000000000000, 0.8660254037844387076, 1.000000000000000000, 0.8660254037844387076, 1.000000000000000000, 0.8660254037844387076, 1.000000000000000000, 0.8660254037844387076, 1.000000000000000000, 0.8660254037844387076, 1.000000000000000000, 0.8660254037844387076, 1.000000000000000000, 0.8660254037844387076, 1.000000000000000000, 0.8660254037844387076, 1.000000000000000000, 0.8660254037844387076, 1.000000000000000000, 0.8660254037844387076, 1.000000000000000000, 0.8660254037844387076, 1.000000000000000000, 0.8660254037844387076, 1.000000000000000000, 0.8660254037844387076, 1.000000000000000000, 0.8660254037844387076, 1.000000000000000000, 0.8660254037844387076, 1.000000000000000000, 0.8660254037844387076, 1.000000000000000000, 0.8660254037844387076, 1.000000000000000000, 0.8660254037844387076, 1.000000000000000000, 0.8660254037844387076, 1.000000000000000000, 0.8660254037844387076, 1.000000000000000000, 0.8660254037844387076, 1.000000000000000000, 0.8660254037844387076, 1.000000000000000000, 0.8660254037844387076, 1.000000000000000000, 0.8660254037844387076, 1.000000000000000000, 0.8660254037844387076, 1.000000000000000000, 0.8660254037844387076, 1.000000000000000000, 0.8660254037844387076, 1.000000000000000000, 0.8660254037844387076, 1.000000000000000000, 0.8660254037844387076, 1.000000000000000000, 0.8660254037844387076, 1.000000000000000000, 0.8660254037844387076, 1.000000000000000000, 0.8660254037844387076, 1.000000000000000000, 0.8660254037844387076, 1.000000000000000000, 0.8660254037844387076, 1.000000000000000000, 0.8660254037844387076, 1.000000000000000000, 0.8660254037844387076, 1.000000000000000000, 0.8660254037844387076, 1.000000000000000000, 0.8660254037844387076, 1.000000000000000000, 0.8660254037844387076, 1.000000000000000000, 0.8660254037844387076, 1.000000000000000000, 0.8660254037844387076, 1.000000000000000000, 0.8660254037844387076, 1.000000000000000000, 0.8660254037844387076, 1.000000000000000000, 0.8660254037844387076, 1.000000000000000000, 0.8660254037844387076, 1.000000000000000000, 0.8660254037844387076, 1.000000000000000000, 0.8660254037844387076, 1.000000000000000000, 0.8660254037844387076, 1.000000000000000000, 0.8660254037844387076, 1.000000000000000000, 0.8660254037844387076, 1.000000000000000000, 0.8660254037844387076, 1.000000000000000000, 0.8660254037844387076, 1.000000000000000000, 0.8660254037844387076, 1.000000000000000000, 0.8660254037844387076, 1.000000000000000000, 0.8660254037844387076, 1.000000000000000000, 0.8660254037844387076, 1.000000000000000000, 0.8660254037844387076, 1.000000000000000000, 0.8660254037844387076, 1.000000000000000000, 0.8660254037844387076, 1.000000000000000000, 0.8660254037844387076, 1.000000000000000000, 0.8660254037844387076, 1.000000000000000000, 0.8660254037844387076, 1.000000000000000000, 0.8660254037844387076, 1.000000000000000000, 0.8660254037844387076, 1.000000000000000000, 0.8660254037844387076, 1.000000000000000000, 0.8660254037844387076, 1.000000000000000000, 0.8660254037844387076, 1.000000000000000000, 0.8660254037844387076, 1.000000000000000000, 0.8660254037844387076, 1.000000000000000000, 0.8660254037844387076, 1.000000000000000000, 0.8660254037844387076, 1.000000000000000000, 0.8660254037844387076, 1.000000000000000000, 0.8660254037844387076, 1.000000000000000000, 0.8660254037844387076, 1.000000000000000000, 0.8660254037844387076, 1.000000000000000000, 0.8660254037844387076, 1.000000000000000000) ) ) 
 REPRESENTATION_ITEM ( '' )  SURFACE ( )  );
#59930=CARTESIAN_POINT ( 'NONE',  ( 147.5693121967435957, 275.0494489676833041, 4.210973343677100189 ) ) ;
#59935=CARTESIAN_POINT ( 'NONE',  ( 100.3908607700757187, 228.7677522451418497, 10.00000000000009592 ) ) ;
#59938=CARTESIAN_POINT ( 'NONE',  ( 162.6220573360242270, 248.9773295930640131, 10.49878733418918486 ) ) ;
#59941=CARTESIAN_POINT ( 'NONE',  ( 12.94935828348961593, 178.2833772461660544, -9.188101187500095079 ) ) ;
#59943=CARTESIAN_POINT ( 'NONE',  ( 193.3216912985990916, 272.5173147653680417, 14.22613245673542259 ) ) ;
#59944=CARTESIAN_POINT ( 'NONE',  ( 192.4335622838504207, 297.3422883733380786, -12.83044365323471325 ) ) ;
#59946=CARTESIAN_POINT ( 'NONE',  ( 175.0941756799416567, 286.4970703408308736, 10.49273659814999604 ) ) ;
#59947=CARTESIAN_POINT ( 'NONE',  ( 64.36996372895568186, 195.7202760586659167, -5.415160957724236172E-17 ) ) ;
#59948=CARTESIAN_POINT ( 'NONE',  ( 207.6471633721571379, 270.9915583223058206, 2.196965492132801678 ) ) ;
#59949=CARTESIAN_POINT ( 'NONE',  ( 203.9641523903856353, 276.3974457028200504, 13.34757937729907873 ) ) ;
#59952=EDGE_LOOP ( 'NONE', ( #31563, #52957, #99823, #68014, #46416 ) ) ;
#59953=CARTESIAN_POINT ( 'NONE',  ( 164.8638179515183424, 269.0684537314152749, 17.58025323075393587 ) ) ;
#59954=CARTESIAN_POINT ( 'NONE',  ( 16.11576366785039127, 190.1115022471903160, -5.000000000000047962 ) ) ;
#59955=CARTESIAN_POINT ( 'NONE',  ( 207.6932907333322191, 270.9116633891313199, 2.120963121341169710 ) ) ;
#59956=CARTESIAN_POINT ( 'NONE',  ( 142.8531688511554307, 253.2833772461660544, -9.188101187500095079 ) ) ;
#59958=CARTESIAN_POINT ( 'NONE',  ( 164.2980929276580468, 246.0743507930604608, 1.884825537327208478 ) ) ;
#59960=CARTESIAN_POINT ( 'NONE',  ( 176.6558404752379090, 252.2237374370411942, -0.2705739152901737166 ) ) ;
#59962=CARTESIAN_POINT ( 'NONE',  ( 189.5765870809536580, 289.5964489643898219, 15.12308329164838128 ) ) ;
#59966=CARTESIAN_POINT ( 'NONE',  ( 163.9377421930003607, 246.6984965740322480, 8.856459175406742546 ) ) ;
#59967=CARTESIAN_POINT ( 'NONE',  ( 192.7686961758011250, 263.9209412561240811, -8.347089341778378468 ) ) ;
#59968=CARTESIAN_POINT ( 'NONE',  ( 169.1830573458304627, 254.2960580516546827, 12.91860015404840389 ) ) ;
#59969=CARTESIAN_POINT ( 'NONE',  ( 197.2578275771767551, 273.1615466810303587, -13.38357264611757103 ) ) ;
#59970=ORIENTED_EDGE ( 'NONE', *, *, #15181, .T. ) ;
#59971=DIRECTION ( 'NONE',  ( -0.8660254037844387076, -0.4999999999999998890, -0.000000000000000000 ) ) ;
#59972=CARTESIAN_POINT ( 'NONE',  ( 170.1929779583345237, 284.3448978393517450, -11.77788885849169453 ) ) ;
#59975=CARTESIAN_POINT ( 'NONE',  ( 203.2757866645317222, 269.5093088776978334, -7.514607224931010521 ) ) ;
#59976=DIRECTION ( 'NONE',  ( 0.4999999999999992784, -0.8660254037844390407, 0.000000000000000000 ) ) ;
#59981=DIRECTION ( 'NONE',  ( 0.4999999999999992784, -0.8660254037844390407, 0.000000000000000000 ) ) ;
#59985=DIRECTION ( 'NONE',  ( -0.8660254037844387076, -0.4999999999999998890, -0.000000000000000000 ) ) ;
#59989=CARTESIAN_POINT ( 'NONE',  ( 191.7187529716733820, 298.5803744197520473, -8.487597704798396592 ) ) ;
#59991=CARTESIAN_POINT ( 'NONE',  ( 204.8189571845487080, 275.8901551335242175, 13.43702398685204358 ) ) ;
#59994=ORIENTED_EDGE ( 'NONE', *, *, #97722, .F. ) ;
#59995=CARTESIAN_POINT ( 'NONE',  ( 87.34609280552280097, 230.4244531367911009, -4.594050593750046652 ) ) ;
#59996=CARTESIAN_POINT ( 'NONE',  ( 198.7838390185755770, 282.9248331187500298, 17.36760380735526610 ) ) ;
#60000=ORIENTED_EDGE ( 'NONE', *, *, #55161, .T. ) ;
#60002=CARTESIAN_POINT ( 'NONE',  ( 207.1548490022400415, 270.0363760279268490, 1.710376025867456962 ) ) ;
#60005=B_SPLINE_CURVE_WITH_KNOTS ( 'NONE', 3,
 ( #58296, #29402, #31382, #52679 ),
 .UNSPECIFIED., .F., .F.,
 ( 4, 4 ),
 ( 0.003581673450268924204, 0.009034217805257406531 ),
 .UNSPECIFIED. ) ;
#60006=ORIENTED_EDGE ( 'NONE', *, *, #93688, .F. ) ;
#60008=CARTESIAN_POINT ( 'NONE',  ( 203.9697818395143258, 267.9997349688208601, 0.5926888351516317321 ) ) ;
#60010=CARTESIAN_POINT ( 'NONE',  ( 164.6921227768849008, 245.3918710745008127, 2.498195641553966340 ) ) ;
#60012=B_SPLINE_CURVE_WITH_KNOTS ( 'NONE', 3,
 ( #22814, #84651, #7108, #78025 ),
 .UNSPECIFIED., .F., .F.,
 ( 4, 4 ),
 ( 0.03712676085629124101, 0.04575313303586313329 ),
 .UNSPECIFIED. ) ;
#60014=ADVANCED_FACE ( 'NONE', ( #9876 ), #40734, .T. ) ;
#60016=CARTESIAN_POINT ( 'NONE',  ( 164.8146514257492186, 264.9101748124866162, -16.65136860934597252 ) ) ;
#60017=ORIENTED_EDGE ( 'NONE', *, *, #62596, .T. ) ;
#60021=CARTESIAN_POINT ( 'NONE',  ( 164.9015738923758079, 282.0469085907977274, 8.845953399109694359 ) ) ;
#60022=CARTESIAN_POINT ( 'NONE',  ( 206.9022815319215738, 270.8307493124123084, 4.969621876343158107 ) ) ;
#60023=EDGE_LOOP ( 'NONE', ( #39096, #98813, #40072, #62361 ) ) ;
#60024=CARTESIAN_POINT ( 'NONE',  ( 202.9689790241539242, 279.0944113002206564, 15.85114608332523289 ) ) ;
#60025=CARTESIAN_POINT ( 'NONE',  ( 184.9789842570080793, 258.2806869971382184, 2.961155574049133765 ) ) ;
#60026=CARTESIAN_POINT ( 'NONE',  ( 157.9648834242245528, 279.9874070561871804, -6.790362339845969153 ) ) ;
#60028=CARTESIAN_POINT ( 'NONE',  ( 192.7517790942337683, 292.1482192696278162, -14.59390454542270099 ) ) ;
#60030=CARTESIAN_POINT ( 'NONE',  ( 194.6806917771430392, 263.4467307442432684, -0.7818862912174471269 ) ) ;
#60031=ORIENTED_EDGE ( 'NONE', *, *, #40157, .T. ) ;
#60032=CARTESIAN_POINT ( 'NONE',  ( 181.6970786337707864, 271.3723858492330123, -15.97957702204227282 ) ) ;
#60033=CARTESIAN_POINT ( 'NONE',  ( 160.6790552449755864, 275.7503919994865100, 12.80081933329241473 ) ) ;
#60034=CARTESIAN_POINT ( 'NONE',  ( 14.65434579541631521, 169.2677522451417929, -5.000000000000041744 ) ) ;
#60035=CARTESIAN_POINT ( 'NONE',  ( 196.1195291313601672, 269.4854874125175570, -10.82207891638150521 ) ) ;
#60036=CARTESIAN_POINT ( 'NONE',  ( 175.0419018616888991, 281.4530265013858070, -14.15648744962207672 ) ) ;
#60037=CARTESIAN_POINT ( 'NONE',  ( 163.6328441044221620, 247.2265955545804275, -8.943872350901562740 ) ) ;
#60039=CARTESIAN_POINT ( 'NONE',  ( 164.7062239463616606, 274.2877436771660200, 14.86310344068559885 ) ) ;
#60040=CARTESIAN_POINT ( 'NONE',  ( 2.746756816977958593, 163.2048013555410080, 4.594050593750051981 ) ) ;
#60042=CARTESIAN_POINT ( 'NONE',  ( 164.0651280066704771, 248.4778578725967861, 9.975266483072225299 ) ) ;
#60044=EDGE_LOOP ( 'NONE', ( #52554, #72628, #68857, #78076 ) ) ;
#60046=CARTESIAN_POINT ( 'NONE',  ( 127.4000280541508516, 234.3615022471901739, 5.000000000000051514 ) ) ;
#60047=CARTESIAN_POINT ( 'NONE',  ( 171.7465271196784897, 289.8775964799340841, 2.715013937588829140 ) ) ;
#60050=CARTESIAN_POINT ( 'NONE',  ( 203.4435754520237651, 276.2723861740593634, 14.48166091637323483 ) ) ;
#60052=CARTESIAN_POINT ( 'NONE',  ( 150.2121420128144678, 276.5610649638679774, 3.689409684367604303 ) ) ;
#60053=B_SPLINE_CURVE_WITH_KNOTS ( 'NONE', 3,
 ( #39185, #77217, #6820, #14431 ),
 .UNSPECIFIED., .F., .F.,
 ( 4, 4 ),
 ( 0.04707519336486235689, 0.04887066958154942520 ),
 .UNSPECIFIED. ) ;
#60054=CARTESIAN_POINT ( 'NONE',  ( 23.50386934422995822, 190.5024278399160949, -9.188101187500093303 ) ) ;
#60055=CARTESIAN_POINT ( 'NONE',  ( 122.6912752411227103, 232.4548013555409796, -4.594050593750042211 ) ) ;
#60057=CARTESIAN_POINT ( 'NONE',  ( 183.2120991357361106, 257.6510318301264419, -2.908943044801409972 ) ) ;
#60062=CARTESIAN_POINT ( 'NONE',  ( 185.4206969650253711, 260.4038640631882231, 9.453313016594156792 ) ) ;
#60063=CARTESIAN_POINT ( 'NONE',  ( 161.8807657183444064, 250.2612843381103573, -13.52770735624900311 ) ) ;
#60067=CARTESIAN_POINT ( 'NONE',  ( 196.5634515809505842, 266.6633299776104309, 8.168478504490389369 ) ) ;
#60069=CARTESIAN_POINT ( 'NONE',  ( 184.4468480456720840, 268.5537564916724023, -15.62460610151881291 ) ) ;
#60070=CYLINDRICAL_SURFACE ( 'NONE', #62650, 17.82106496071139645 ) ;
#60071=CARTESIAN_POINT ( 'NONE',  ( 188.1412547211656943, 273.5593357346770063, 17.08033167198486879 ) ) ;
#60073=CARTESIAN_POINT ( 'NONE',  ( 102.8537940617441819, 224.0643266524160140, 9.188101187500095079 ) ) ;
#60075=CARTESIAN_POINT ( 'NONE',  ( 191.0170959869219303, 299.7956799668270946, 7.353346939903929069 ) ) ;
#60076=CARTESIAN_POINT ( 'NONE',  ( 159.1113560326100753, 259.2834188555653441, -17.54322067557006903 ) ) ;
#60077=CARTESIAN_POINT ( 'NONE',  ( 157.0935036675524827, 258.5530654392286465, 17.32636058289560665 ) ) ;
#60078=CARTESIAN_POINT ( 'NONE',  ( 151.9298993999875904, 267.4966903808301026, 16.91367899156788468 ) ) ;
#60079=DIRECTION ( 'NONE',  ( 0.5000000000000048850, -0.8660254037844358210, 0.000000000000000000 ) ) ;
#60080=CARTESIAN_POINT ( 'NONE',  ( 198.4860348845112981, 286.8590983175747056, -18.20461732983060088 ) ) ;
#60083=CARTESIAN_POINT ( 'NONE',  ( 193.2100161762185735, 295.9974307820218087, -12.46499585622781758 ) ) ;
#60087=DIRECTION ( 'NONE',  ( -0.8660254037844387076, -0.4999999999999998890, -0.000000000000000000 ) ) ;
#60089=CARTESIAN_POINT ( 'NONE',  ( 196.9319848161575806, 289.5507919934690335, -17.64330560362266453 ) ) ;
#60090=B_SPLINE_CURVE_WITH_KNOTS ( 'NONE', 3,
 ( #61241, #51671, #59745, #13183, #29857, #75989, #44039, #36449, #7546, #75473, #6058, #91689, #45538, #14662, #74979, #67352, #30356, #36952, #20780, #67863, #6566, #46029, #5560, #37931, #98281, #99274, #38438, #37439, #76470, #53154, #7050, #53639, #69352, #100271, #84594, #959, #38940, #77966, #9059, #25250, #48561, #55629, #10063, #70863, #23737, #8561, #79502, #86614, #40928, #458 ),
 .UNSPECIFIED., .F., .F.,
 ( 4, 2, 2, 2, 2, 2, 2, 2, 2, 2, 2, 2, 2, 2, 2, 2, 2, 2, 2, 2, 2, 2, 2, 2, 4 ),
 ( 0.0003281754202554149351, 0.0008006094400505323408, 0.001273043459845649584, 0.001509260469743186088, 0.001627368974692035329, 0.001745477479640884571, 0.001981694489538647890, 0.002217911499436411426, 0.002690345519231964518, 0.003162779539027517611, 0.004107647578618566983, 0.005052515618209615922, 0.005524949638005215852, 0.005761166647903014949, 0.005879275152851915799, 0.005938329405326366224, 0.005997383657800815782, 0.006056437910275266207, 0.006115492162749716631, 0.006233600667698616614, 0.006469817677596420916, 0.006942251697392027784, 0.007414685717187633786, 0.007650902727085504007, 0.007887119736983375096 ),
 .UNSPECIFIED. ) ;
#60093=CARTESIAN_POINT ( 'NONE',  ( 159.7897726928491409, 253.8829904965402875, 16.83923858130328810 ) ) ;
#60094=CARTESIAN_POINT ( 'NONE',  ( 157.7660523726510462, 268.4465589492402842, 16.76385752021615261 ) ) ;
#60096=CARTESIAN_POINT ( 'NONE',  ( 140.8234218128095847, 262.1115022471903444, -5.000000000000047962 ) ) ;
#60099=EDGE_LOOP ( 'NONE', ( #53431, #57518, #85736, #25020, #49179, #80907, #34061, #58413, #80109, #12875, #36441, #36110, #72665, #78379, #28637, #1840, #24867, #74978, #41854, #46695 ) ) ;
#60100=CARTESIAN_POINT ( 'NONE',  ( 195.7229849017213610, 265.1195584955938216, -4.418747677595802337 ) ) ;
#60103=CARTESIAN_POINT ( 'NONE',  ( 185.2143418923794798, 292.5124672671021244, -10.69479488396104827 ) ) ;
#60104=ORIENTED_EDGE ( 'NONE', *, *, #30205, .T. ) ;
#60106=CARTESIAN_POINT ( 'NONE',  ( 206.2356669332361605, 273.4363418692194045, 11.05590195897326922 ) ) ;
#60107=CARTESIAN_POINT ( 'NONE',  ( 190.6061379745418094, 278.8388338309181904, -16.51655004129774795 ) ) ;
#60108=FACE_OUTER_BOUND ( 'NONE', #33198, .T. ) ;
#60109=CARTESIAN_POINT ( 'NONE',  ( 152.7295469705997277, 266.1116601603806657, -17.40211458100010589 ) ) ;
#60115=CARTESIAN_POINT ( 'NONE',  ( 72.84042761573121538, 202.8615022471901739, 5.000000000000051514 ) ) ;
#60116=ORIENTED_EDGE ( 'NONE', *, *, #64577, .T. ) ;
#60119=CARTESIAN_POINT ( 'NONE',  ( 205.2391015854675516, 275.1624436846170738, -14.01434138479280911 ) ) ;
#60120=CARTESIAN_POINT ( 'NONE',  ( 182.5892408154444695, 296.6611350254266313, 0.3217610282793219589 ) ) ;
#60121=CARTESIAN_POINT ( 'NONE',  ( 174.1046625087539894, 257.2888617342148336, -11.85904880942999107 ) ) ;
#60122=CARTESIAN_POINT ( 'NONE',  ( 194.1789525331299728, 294.3191837825503967, -15.34533909744314961 ) ) ;
#60124=CARTESIAN_POINT ( 'NONE',  ( 197.9761018079605606, 272.1676159484598543, -13.70813156040953729 ) ) ;
#60127=CARTESIAN_POINT ( 'NONE',  ( 170.5330744639767033, 287.4519228453978599, -4.620264690464154889 ) ) ;
#60130=CARTESIAN_POINT ( 'NONE',  ( 186.7687816609699212, 286.9689498124462261, -15.64156219619770560 ) ) ;
#60131=B_SPLINE_CURVE_WITH_KNOTS ( 'NONE', 3,
 ( #4072, #37820, #91082, #14046, #45910, #15019, #96822, #84477, #89243, #91568, #27380, #58266, #19793, #76359, #50661, #68729, #60613, #61118 ),
 .UNSPECIFIED., .F., .F.,
 ( 4, 2, 2, 2, 2, 2, 2, 2, 4 ),
 ( 0.0001987964186102976830, 0.0003140683529223511493, 0.0003717043200783778554, 0.0004293402872344046156, 0.0004581582708124750519, 0.0004869762543905454882, 0.0005446122215466848429, 0.0006598841558589985720, 0.001120971893108076763 ),
 .UNSPECIFIED. ) ;
#60132=CARTESIAN_POINT ( 'NONE',  ( 118.1174918034448922, 232.8768266524160140, 9.188101187500098632 ) ) ;
#60134=CARTESIAN_POINT ( 'NONE',  ( 184.0739800145211120, 260.1317561499213298, -9.673630312158074673 ) ) ;
#60137=EDGE_LOOP ( 'NONE', ( #22661, #15368, #82519 ) ) ;
#60140=CARTESIAN_POINT ( 'NONE',  ( 164.4902401177012337, 246.2554029907234678, -2.428734258964198034 ) ) ;
#60141=CARTESIAN_POINT ( 'NONE',  ( 195.9359860111818250, 291.2759125279654882, 17.49638312768267312 ) ) ;
#60145=CARTESIAN_POINT ( 'NONE',  ( 195.5149407638684522, 292.0051842885976043, 15.88854587925930772 ) ) ;
#60150=CARTESIAN_POINT ( 'NONE',  ( 192.7079119722239113, 262.6034417676851263, 4.671215074061198180 ) ) ;
#60151=CARTESIAN_POINT ( 'NONE',  ( 155.5311623832600958, 261.6886619413561448, 17.00987194985870943 ) ) ;
#60155=CARTESIAN_POINT ( 'NONE',  ( 200.7134601498536028, 283.0010845879393742, -16.98649239173277792 ) ) ;
#60157=DIRECTION ( 'NONE',  ( -0.4999999999999987788, 0.8660254037844392627, 0.000000000000000000 ) ) ;
#60161=CARTESIAN_POINT ( 'NONE',  ( 189.0232759416005877, 269.9725822948850578, -14.03890638026795301 ) ) ;
#60165=CARTESIAN_POINT ( 'NONE',  ( 23.57265107556306916, 195.9637435831424739, 2.679491924311251605 ) ) ;
#60167=CARTESIAN_POINT ( 'NONE',  ( 70.32319418844367931, 223.6589784336661921, -6.496448406907675876E-16 ) ) ;
#60168=CARTESIAN_POINT ( 'NONE',  ( 206.1615484827472358, 273.5647187912443314, -9.556459874778100883 ) ) ;
#60170=CARTESIAN_POINT ( 'NONE',  ( 208.3586375946586315, 269.7592488206576604, -1.970210487958146128 ) ) ;
#60173=CARTESIAN_POINT ( 'NONE',  ( 161.2133744761260061, 251.4172398781588811, -14.30368667312104058 ) ) ;
#60176=CARTESIAN_POINT ( 'NONE',  ( 116.1416978049531110, 237.8615022471902307, -10.00000000000009592 ) ) ;
#60182=CARTESIAN_POINT ( 'NONE',  ( 24.64070123457955219, 185.0333772461660544, 9.188101187500095079 ) ) ;
#60183=B_SPLINE_CURVE_WITH_KNOTS ( 'NONE', 3,
 ( #34538, #65436, #98352, #74563, #20854, #27452, #21334, #29429, #13729, #59303, #12759, #20348, #27928, #21825, #4640, #52218, #58326, #83164, #82687, #5627, #98853, #90784, #28941, #36520, #67421, #97362, #28423, #51219, #73549, #82187, #35025, #44606, #13254, #43622, #36021, #4132, #52711, #59817, #35533, #44112, #37023, #66922, #60303, #75540, #6126, #58811, #51745, #67931 ),
 .UNSPECIFIED., .F., .F.,
 ( 4, 2, 2, 2, 2, 2, 2, 2, 2, 2, 2, 2, 2, 2, 2, 2, 2, 2, 2, 2, 2, 2, 2, 4 ),
 ( 0.0004489931541215139068, 0.001462873357728531861, 0.001969813459531987061, 0.002223283510433714770, 0.002350018535884506633, 0.002476753561335297629, 0.002730223612236896968, 0.002983693663138495440, 0.003490633764941693251, 0.004504513968548151323, 0.005518394172154609395, 0.006025334273957838431, 0.006278804324859453383, 0.006532274375761068334, 0.006595641888486466868, 0.006659009401211866269, 0.006722376913937264803, 0.006785744426662664204, 0.007039214477564325126, 0.007546154579367791819, 0.007799624630269523864, 0.008053094681171255043, 0.008306564732072987955, 0.008560034782974719134 ),
 .UNSPECIFIED. ) ;
#60185=CARTESIAN_POINT ( 'NONE',  ( 171.9695299662907360, 276.3046275190319534, -16.98996149290084645 ) ) ;
#60187=CARTESIAN_POINT ( 'NONE',  ( 164.1654149204426858, 248.3041558426086226, -9.671695341034215687 ) ) ;
#60189=CARTESIAN_POINT ( 'NONE',  ( 59.90443346675090908, 196.2048013555409796, 4.594050593750051981 ) ) ;
#60191=CARTESIAN_POINT ( 'NONE',  ( 198.8157103782086210, 286.2880836124806478, -18.60729372713428020 ) ) ;
#60195=CARTESIAN_POINT ( 'NONE',  ( 202.9470114082288319, 270.0688303170933864, -6.543538759376999359 ) ) ;
#60196=CARTESIAN_POINT ( 'NONE',  ( 175.4799100621144134, 291.2742715687741679, 2.018303699312502086 ) ) ;
#60197=CARTESIAN_POINT ( 'NONE',  ( 176.8361213315729117, 275.2114496154293306, 16.59131570778482256 ) ) ;
#60200=DIRECTION ( 'NONE',  ( 0.4999999999999998890, -0.8660254037844385966, 0.000000000000000000 ) ) ;
#60201=EDGE_CURVE ( 'NONE', #14882, #26754, #46668, .T. ) ;
#60203=CARTESIAN_POINT ( 'NONE',  ( 98.02733310912863374, 220.7365022471901739, -10.00000000000009059 ) ) ;
#60204=( BOUNDED_CURVE ( )  B_SPLINE_CURVE ( 2, ( #59159, #82040, #90646, #43972, #90133, #35389, #67792, #43479, #98716 ),
 .UNSPECIFIED., .F., .T. ) 
 B_SPLINE_CURVE_WITH_KNOTS ( ( 3, 2, 2, 2, 3 ),
 ( 0.9556451612903226200, 0.9569892473118279952, 0.9596774193548387455, 0.9623655913978494958, 0.9637096774193548709 ),
 .UNSPECIFIED. ) 
 CURVE ( )  GEOMETRIC_REPRESENTATION_ITEM ( )  RATIONAL_B_SPLINE_CURVE ( ( 0.9330127018922194093, 0.9330127018922194093, 1.000000000000000000, 0.8660254037844387076, 1.000000000000000000, 0.8660254037844387076, 1.000000000000000000, 0.9330127018922194093, 0.9330127018922194093 ) ) 
 REPRESENTATION_ITEM ( '' )  );
#60205=DIRECTION ( 'NONE',  ( 0.4999999999999992784, -0.8660254037844390407, 0.000000000000000000 ) ) ;
#60207=EDGE_LOOP ( 'NONE', ( #16762, #80857, #64283, #39151 ) ) ;
#60208=CARTESIAN_POINT ( 'NONE',  ( 58.44249495421716745, 213.7369531367911293, -4.594050593750048428 ) ) ;
#60210=CARTESIAN_POINT ( 'NONE',  ( 166.2774799739476066, 265.1959323007807257, 16.57056821886706288 ) ) ;
#60211=CARTESIAN_POINT ( 'NONE',  ( 190.7908437487391780, 300.1875603386860689, -4.317984972589949955 ) ) ;
#60216=CARTESIAN_POINT ( 'NONE',  ( 193.5629084239263307, 292.5061527191514870, -15.60167767085171242 ) ) ;
#60218=CARTESIAN_POINT ( 'NONE',  ( 206.6742118400747756, 271.5744752743144659, -6.599374785183829140 ) ) ;
#60219=CARTESIAN_POINT ( 'NONE',  ( 115.9793180381956716, 227.7677522451417929, -5.000000000000041744 ) ) ;
#60225=CARTESIAN_POINT ( 'NONE',  ( 167.9496373820661290, 248.6204696539478789, -6.517719931589019744 ) ) ;
#60229=CARTESIAN_POINT ( 'NONE',  ( 182.6429660890904074, 283.7719756040974062, 15.79391243952982649 ) ) ;
#60230=CARTESIAN_POINT ( 'NONE',  ( 206.6912923161529818, 272.6471755567893638, -9.325620632947922317 ) ) ;
#60235=CARTESIAN_POINT ( 'NONE',  ( 162.7007457333762090, 248.8410372908842021, -10.94671474643812914 ) ) ;
#60236=CARTESIAN_POINT ( 'NONE',  ( 204.9432097630379417, 275.6749433546094679, 13.74700047688257776 ) ) ;
#60237=CARTESIAN_POINT ( 'NONE',  ( 190.0667283601964357, 259.9641452334862493, -5.090329199819447104E-14 ) ) ;
#60239=CARTESIAN_POINT ( 'NONE',  ( 161.0844399624414507, 263.0064568173025350, -17.38383432207021784 ) ) ;
#60240=CARTESIAN_POINT ( 'NONE',  ( 125.2075541532825014, 255.3464784336661353, 1.353441290958777525E-15 ) ) ;
#60241=EDGE_CURVE ( 'NONE', #16392, #33130, #66623, .T. ) ;
#60243=CARTESIAN_POINT ( 'NONE',  ( 81.74442484449845381, 211.8768266524159856, 9.188101187500098632 ) ) ;
#60245=CARTESIAN_POINT ( 'NONE',  ( 174.1398777777984037, 265.6557655336882249, 16.43872977299918503 ) ) ;
#60248=CARTESIAN_POINT ( 'NONE',  ( 160.2539783940571851, 253.8594209733300318, 15.13163501824758228 ) ) ;
#60249=ORIENTED_EDGE ( 'NONE', *, *, #11054, .F. ) ;
#60250=ORIENTED_EDGE ( 'NONE', *, *, #32562, .F. ) ;
#60254=EDGE_CURVE ( 'NONE', #44553, #49678, #40044, .T. ) ;
#60255=CARTESIAN_POINT ( 'NONE',  ( 196.9422331689194152, 286.2628525950418634, 16.90547485990039789 ) ) ;
#60259=CARTESIAN_POINT ( 'NONE',  ( 193.9966098916996771, 294.6350105018939871, 13.97117019253516013 ) ) ;
#60261=CARTESIAN_POINT ( 'NONE',  ( 182.5067194347547854, 257.1923330838238826, -6.222426465989368438 ) ) ;
#60262=ORIENTED_EDGE ( 'NONE', *, *, #89430, .F. ) ;
#60266=B_SPLINE_CURVE_WITH_KNOTS ( 'NONE', 3,
 ( #25459, #87349, #1171, #18374, #79708, #26967, #20365, #75066, #65952, #43129, #52239, #13270, #82204, #12775, #20870, #51761, #5645, #67440, #73083, #57848, #28957, #83183, #34556, #65456, #29940, #76074, #51, #14739, #92770, #91776, #38016, #30436, #53719, #67948, #61325, #84679, #60321, #46629, #69925, #542, #15219, #77030, #38527, #29444, #80083, #2049, #41526, #33962 ),
 .UNSPECIFIED., .F., .F.,
 ( 4, 2, 2, 2, 2, 2, 2, 2, 2, 2, 2, 2, 2, 2, 2, 2, 2, 2, 2, 2, 2, 2, 2, 4 ),
 ( 0.002098688353426452196, 0.002534572199440611722, 0.002752514122447782992, 0.002970456045454953828, 0.003079427006958539680, 0.003188397968462125531, 0.003297368929965711383, 0.003406339891469296801, 0.003624281814476544399, 0.003842223737483791562, 0.004713991429512820117, 0.005585759121541849538, 0.006457526813570877225, 0.006893410659585395839, 0.007329294505599914453, 0.007438265467103608725, 0.007492750947855422033, 0.007547236428607235342, 0.007656207390110858491, 0.007765178351614485108, 0.008201062197628897904, 0.008636946043643310700, 0.008854887966650496281, 0.009072829889657683597 ),
 .UNSPECIFIED. ) ;
#60268=CARTESIAN_POINT ( 'NONE',  ( 173.9990153864150670, 253.4041716863320062, -7.605893656024731442 ) ) ;
#60269=CARTESIAN_POINT ( 'NONE',  ( 186.8006684768011212, 276.5875442340776544, 17.70268152755913604 ) ) ;
#60270=CARTESIAN_POINT ( 'NONE',  ( 196.3507576896697344, 290.5575069072837664, -17.68249398312240928 ) ) ;
#60273=CARTESIAN_POINT ( 'NONE',  ( 140.0928864244750685, 245.5643266524160424, -9.188101187500093303 ) ) ;
#60274=EDGE_LOOP ( 'NONE', ( #38695, #90963, #5177, #53406 ) ) ;
#60276=CARTESIAN_POINT ( 'NONE',  ( 182.9163764445669642, 258.7192441424419371, 6.406310776454488654 ) ) ;
#60277=CARTESIAN_POINT ( 'NONE',  ( 155.9683004480747286, 261.9866473075522322, -16.96465910183697900 ) ) ;
#60280=ORIENTED_EDGE ( 'NONE', *, *, #11007, .T. ) ;
#60282=CARTESIAN_POINT ( 'NONE',  ( 182.1414478339540040, 275.7655165773919634, -16.43324961048260846 ) ) ;
#60283=FACE_OUTER_BOUND ( 'NONE', #52658, .T. ) ;
#60286=CARTESIAN_POINT ( 'NONE',  ( 202.5535515909786000, 267.2301142524262332, 0.8809907921587507573 ) ) ;
#60287=CARTESIAN_POINT ( 'NONE',  ( 198.4976171291946514, 266.2161181449658898, 0.6785798567533030123 ) ) ;
#60288=CARTESIAN_POINT ( 'NONE',  ( 190.9380839614473473, 299.9325328093580652, -5.232187664503159752 ) ) ;
#60289=CARTESIAN_POINT ( 'NONE',  ( 184.2669327163933986, 281.3015570470274724, 16.28411061875366173 ) ) ;
#60290=AXIS2_PLACEMENT_3D ( 'NONE', #64329, #38652, #87707 ) ;
#60291=EDGE_CURVE ( 'NONE', #5719, #21768, #72319, .T. ) ;
#60292=CARTESIAN_POINT ( 'NONE',  ( 193.0780078417625703, 268.7414322461000893, 12.24939826239815055 ) ) ;
#60293=CIRCLE ( 'NONE', #73291, 17.82106496071138935 ) ;
#60298=CARTESIAN_POINT ( 'NONE',  ( 205.3385343418334230, 274.5435030208487319, 11.21992643350996843 ) ) ;
#60300=CARTESIAN_POINT ( 'NONE',  ( 198.6587626159274294, 286.5599251108861267, 17.99840276545888784 ) ) ;
#60301=CARTESIAN_POINT ( 'NONE',  ( 193.0758421513005487, 292.7688076435337621, 15.33214366454828692 ) ) ;
#60302=CARTESIAN_POINT ( 'NONE',  ( 149.3212960838965557, 247.0177522451417644, 5.000000000000051514 ) ) ;
#60303=CARTESIAN_POINT ( 'NONE',  ( 175.4720935967913533, 286.3835187628145036, -12.16069689870089121 ) ) ;
#60304=ORIENTED_EDGE ( 'NONE', *, *, #60787, .F. ) ;
#60309=CARTESIAN_POINT ( 'NONE',  ( 150.6438662863770332, 269.7241650738195631, -14.92510732909997628 ) ) ;
#60310=CARTESIAN_POINT ( 'NONE',  ( -0.2035760843690503918, 176.8149278399160949, -9.188101187500095079 ) ) ;
#60313=CARTESIAN_POINT ( 'NONE',  ( 65.24466313315720356, 215.1427522451419065, -10.00000000000009592 ) ) ;
#60316=B_SPLINE_SURFACE_WITH_KNOTS ( 'NONE', 3, 1, ( 
 ( #84694, #91791 ),
 ( #13759, #62334 ),
 ( #38032, #68448 ),
 ( #61838, #37056 ),
 ( #98881, #37542 ),
 ( #93285, #29955 ),
 ( #92785, #44638 ),
 ( #15235, #85194 ),
 ( #99376, #46646 ),
 ( #15738, #68942 ),
 ( #77571, #22356 ),
 ( #53253, #8159 ),
 ( #67963, #45636 ),
 ( #558, #92302 ),
 ( #45152, #6160 ),
 ( #14754, #52740 ),
 ( #76564, #29461 ),
 ( #30453, #60336 ),
 ( #91293, #61343 ),
 ( #21858, #83702 ),
 ( #6665, #36342 ),
 ( #13567, #76366 ),
 ( #6456, #37334 ),
 ( #91089, #52536 ),
 ( #53037, #30245 ),
 ( #6938, #21654 ),
 ( #28246, #22147 ),
 ( #99160, #90605 ),
 ( #14557, #83487 ),
 ( #92103, #99659 ),
 ( #90094, #4969 ),
 ( #82990, #66745 ),
 ( #61126, #14053 ),
 ( #97680, #67244 ) ),
 .UNSPECIFIED., .T., .F., .F.,
 ( 4, 2, 2, 2, 2, 2, 2, 2, 2, 2, 2, 2, 2, 2, 2, 2, 4 ),
 ( 2, 2 ),
 ( 0.000000000000000000, 0.06250000000000000000, 0.1250000000000000000, 0.1875000000000000000, 0.2500000000000000000, 0.3125000000000000000, 0.3750000000000000000, 0.4375000000000000000, 0.5000000000000000000, 0.5625000000000000000, 0.6250000000000000000, 0.6875000000000000000, 0.7500000000000000000, 0.8125000000000000000, 0.8750000000000000000, 0.9375000000000000000, 1.000000000000000000 ),
 ( 0.000000000000000000, 1.000000000000000000 ),
 .UNSPECIFIED. ) ;
#60319=CARTESIAN_POINT ( 'NONE',  ( 198.6701036545953230, 286.5402818557027445, 17.25253558010639310 ) ) ;
#60321=CARTESIAN_POINT ( 'NONE',  ( 183.1064801743427211, 295.7402259981610655, 1.177175515638812398 ) ) ;
#60322=CARTESIAN_POINT ( 'NONE',  ( 57.68498304950353628, 194.1115022471902023, -5.000000000000041744 ) ) ;
#60324=CARTESIAN_POINT ( 'NONE',  ( 147.8503508990560533, 274.5626756563852950, 7.845851077393495743 ) ) ;
#60325=CARTESIAN_POINT ( 'NONE',  ( 16.79251956066557128, 174.3768266524160140, 9.188101187500098632 ) ) ;
#60326=CARTESIAN_POINT ( 'NONE',  ( 164.3787126659294131, 284.8162412357542621, 4.248981773088212677 ) ) ;
#60327=CARTESIAN_POINT ( 'NONE',  ( 153.0070714074088016, 265.6309737354857248, 17.74442213480098474 ) ) ;
#60329=CARTESIAN_POINT ( 'NONE',  ( 201.2339362457151992, 280.2550766807431160, -16.75742611627472911 ) ) ;
#60330=CYLINDRICAL_SURFACE ( 'NONE', #35329, 17.82106496071139645 ) ;
#60331=CARTESIAN_POINT ( 'NONE',  ( 189.1997833930358013, 268.1800545106789286, 13.86060302672411382 ) ) ;
#60332=CARTESIAN_POINT ( 'NONE',  ( 149.1653648461108617, 275.5304674000249179, 7.618651205328232479 ) ) ;
#60333=CARTESIAN_POINT ( 'NONE',  ( 164.0858594112551430, 281.5537891919451567, 8.872571969112266643 ) ) ;
#60336=CARTESIAN_POINT ( 'NONE',  ( 148.3837145175834280, 273.6388627701866767, 8.841971351370922605 ) ) ;
#60338=CARTESIAN_POINT ( 'NONE',  ( 194.4263876777154394, 293.8906135405502482, 15.23185943445137802 ) ) ;
#60348=CARTESIAN_POINT ( 'NONE',  ( 203.2187760522547819, 278.6617501559703101, -15.08675642319914978 ) ) ;
#60350=ORIENTED_EDGE ( 'NONE', *, *, #62585, .F. ) ;
#60352=CARTESIAN_POINT ( 'NONE',  ( 186.2856400130477539, 271.9584414235993677, -16.42190033998581811 ) ) ;
#60353=CARTESIAN_POINT ( 'NONE',  ( 204.9103773355753617, 275.7318107871104189, 13.62808820451859937 ) ) ;
#60355=CARTESIAN_POINT ( 'NONE',  ( 191.5544531425776427, 298.8649500714207647, 8.366689293739112188 ) ) ;
#60360=CARTESIAN_POINT ( 'NONE',  ( 189.8147415777049218, 301.8782188922952514, -0.5019643756309712934 ) ) ;
#60364=CARTESIAN_POINT ( 'NONE',  ( 206.1215120922853146, 273.6340638536760821, 10.12238414215620885 ) ) ;
#60368=CARTESIAN_POINT ( 'NONE',  ( 149.5633513747893346, 271.5956717990251832, 12.83777201928511325 ) ) ;
#60373=CARTESIAN_POINT ( 'NONE',  ( 84.09875786492884231, 229.3615022471903160, 5.000000000000046185 ) ) ;
#60374=CARTESIAN_POINT ( 'NONE',  ( 180.4054221593022476, 281.2366265252658764, 16.98216568542962435 ) ) ;
#60375=DIRECTION ( 'NONE',  ( -0.8660254037844387076, -0.4999999999999998890, -0.000000000000000000 ) ) ;
#60381=CARTESIAN_POINT ( 'NONE',  ( 190.8957779480239765, 300.0058089740729770, -4.541438514207768229 ) ) ;
#60382=CARTESIAN_POINT ( 'NONE',  ( 148.1634546024981205, 274.0203641339852538, 9.324875965062235039 ) ) ;
#60383=CARTESIAN_POINT ( 'NONE',  ( 175.1455254742422767, 260.8290329488390853, -14.76850912927449322 ) ) ;
#60384=CARTESIAN_POINT ( 'NONE',  ( 152.9489295551198893, 265.7316783776963121, 17.71675637597311237 ) ) ;
#60385=B_SPLINE_CURVE_WITH_KNOTS ( 'NONE', 3,
 ( #32653, #7349, #23036, #53932 ),
 .UNSPECIFIED., .F., .F.,
 ( 4, 4 ),
 ( 0.0005560040454048003873, 0.001053805433886535097 ),
 .UNSPECIFIED. ) ;
#60386=CARTESIAN_POINT ( 'NONE',  ( 147.2637475104381792, 275.5787025293629426, -0.3536082318825462534 ) ) ;
#60387=CARTESIAN_POINT ( 'NONE',  ( 191.0724301404414689, 299.6998384015373063, -9.342134220577969828 ) ) ;
#60388=AXIS2_PLACEMENT_3D ( 'NONE', #35089, #86863, #19435 ) ;
#60392=CARTESIAN_POINT ( 'NONE',  ( 170.9795069520696700, 289.1314490031791706, 4.359428402176874329 ) ) ;
#60395=CARTESIAN_POINT ( 'NONE',  ( 149.1230935109639972, 272.3582207876025336, -11.65754870978959268 ) ) ;
#60397=CARTESIAN_POINT ( 'NONE',  ( 148.9880786965214838, 273.1702080067959173, 9.612489482347704950 ) ) ;
#60400=CARTESIAN_POINT ( 'NONE',  ( 147.9357294667677252, 274.4147956392308174, -9.396937908507679182 ) ) ;
#60401=CARTESIAN_POINT ( 'NONE',  ( 166.0155803056910315, 284.5441077266590355, -8.592831666274795666 ) ) ;
#60403=CARTESIAN_POINT ( 'NONE',  ( 168.3577311645284453, 254.0536616052273473, -11.79086602269251571 ) ) ;
#60404=CARTESIAN_POINT ( 'NONE',  ( 186.7063704226160326, 285.7974574491823319, -16.69995036437973468 ) ) ;
#60406=ADVANCED_FACE ( 'NONE', ( #4069 ), #4569, .T. ) ;
#60407=CARTESIAN_POINT ( 'NONE',  ( 54.99669585504140912, 195.8927522451418213, -10.00000000000009059 ) ) ;
#60408=CARTESIAN_POINT ( 'NONE',  ( 114.9778026189612632, 243.3149278399160664, 9.188101187500093303 ) ) ;
#60409=CARTESIAN_POINT ( 'NONE',  ( 151.2567985338353935, 268.6625352796243646, -15.71756535662528798 ) ) ;
#60412=CARTESIAN_POINT ( 'NONE',  ( 172.8311536199634588, 250.6280622661865607, -4.159570053950042201 ) ) ;
#60413=CARTESIAN_POINT ( 'NONE',  ( 36.52174756457106497, 182.7048013555409796, 4.594050593750051981 ) ) ;
#60414=CARTESIAN_POINT ( 'NONE',  ( 147.6458100276484799, 275.6668707137318393, -2.669052585738262096 ) ) ;
#60415=B_SPLINE_CURVE_WITH_KNOTS ( 'NONE', 3,
 ( #65848, #96303, #19297, #12171 ),
 .UNSPECIFIED., .F., .F.,
 ( 4, 4 ),
 ( 0.04472034873244652015, 0.04887066958154942520 ),
 .UNSPECIFIED. ) ;
#60416=EDGE_LOOP ( 'NONE', ( #3804, #975, #52163, #95478 ) ) ;
#60418=CARTESIAN_POINT ( 'NONE',  ( 181.8935359714662923, 266.9004732347041795, 15.52955990709112122 ) ) ;
#60419=B_SPLINE_CURVE_WITH_KNOTS ( 'NONE', 3,
 ( #53770, #60374, #45187, #98917 ),
 .UNSPECIFIED., .F., .F.,
 ( 4, 4 ),
 ( 0.02807627225634463583, 0.03726733138970944603 ),
 .UNSPECIFIED. ) ;
#60421=CARTESIAN_POINT ( 'NONE',  ( 146.9376205018946848, 276.1435710778808925, 5.066564108429441937 ) ) ;
#60422=CARTESIAN_POINT ( 'NONE',  ( 99.01965388075032592, 234.6427522451419065, -10.00000000000009592 ) ) ;
#60424=CARTESIAN_POINT ( 'NONE',  ( 64.18017357788677657, 207.8615022471902307, -10.00000000000009592 ) ) ;
#60425=CARTESIAN_POINT ( 'NONE',  ( 164.1747640914098554, 250.0330537093315399, 10.26818566766051077 ) ) ;
#60426=CARTESIAN_POINT ( 'NONE',  ( 108.6181021060278198, 243.5177522451419065, 5.000000000000046185 ) ) ;
#60428=CARTESIAN_POINT ( 'NONE',  ( 198.7382248435485792, 267.5558359697628248, -8.259202697554929529 ) ) ;
#60429=EDGE_CURVE ( 'NONE', #39044, #21, #99301, .T. ) ;
#60430=CARTESIAN_POINT ( 'NONE',  ( 155.7386282512242985, 279.8610998479833825, -1.584717933846769400 ) ) ;
#60431=CARTESIAN_POINT ( 'NONE',  ( 163.4218292706009095, 247.5920839679097014, -10.44611490715852042 ) ) ;
#60433=CARTESIAN_POINT ( 'NONE',  ( 16.49491010205593255, 171.1423013555409796, -4.594050593750043987 ) ) ;
#60438=CARTESIAN_POINT ( 'NONE',  ( 174.7685907560459100, 286.3307797320127861, 10.46086992841393482 ) ) ;
#60439=CARTESIAN_POINT ( 'NONE',  ( 61.79834339388186493, 215.6744531367911293, 4.594050593750047540 ) ) ;
#60440=CARTESIAN_POINT ( 'NONE',  ( 163.7038023771459052, 247.1036922210055025, -6.448491958542482472 ) ) ;
#60446=ADVANCED_FACE ( 'NONE', ( #11200 ), #51389, .F. ) ;
#60448=CARTESIAN_POINT ( 'NONE',  ( 6.950328144465094837, 181.4865022471903160, -10.00000000000009415 ) ) ;
#60449=CARTESIAN_POINT ( 'NONE',  ( 207.5290616128274337, 271.1961165699281651, 2.604679844609484984 ) ) ;
#60451=CARTESIAN_POINT ( 'NONE',  ( 141.8249372320439647, 246.5643266524160140, 9.188101187500095079 ) ) ;
#60453=CARTESIAN_POINT ( 'NONE',  ( 164.3691747484889163, 245.9512334678869365, 1.203589100610505724 ) ) ;
#60457=CARTESIAN_POINT ( 'NONE',  ( 189.4564606193425789, 289.8033142756258940, 15.68452023909392956 ) ) ;
#60459=ORIENTED_EDGE ( 'NONE', *, *, #97229, .T. ) ;
#60462=CARTESIAN_POINT ( 'NONE',  ( 155.9200296242932495, 280.3860598674420430, -5.539708607631867565 ) ) ;
#60463=CARTESIAN_POINT ( 'NONE',  ( 197.2238629298283570, 273.4569059118221617, -14.28082208226903305 ) ) ;
#60465=CARTESIAN_POINT ( 'NONE',  ( 206.5287971022838178, 272.9286255231971268, 9.140400389658188018 ) ) ;
#60467=B_SPLINE_CURVE_WITH_KNOTS ( 'NONE', 3,
 ( #8471, #61657, #39342, #70257 ),
 .UNSPECIFIED., .F., .F.,
 ( 4, 4 ),
 ( 0.01270677793150105754, 0.02126268609028184389 ),
 .UNSPECIFIED. ) ;
#60468=CARTESIAN_POINT ( 'NONE',  ( 153.4689407916852701, 266.8309924954582470, 16.62268559038933091 ) ) ;
#60469=CARTESIAN_POINT ( 'NONE',  ( 192.7547114638438188, 293.9047809918118901, -14.59372857566467374 ) ) ;
#60472=CARTESIAN_POINT ( 'NONE',  ( 200.6737073311291795, 283.0699384897140476, -17.61533935526990291 ) ) ;
#60474=CARTESIAN_POINT ( 'NONE',  ( 190.9874095833745002, 280.9743702084771826, 16.64962686899652411 ) ) ;
#60478=CARTESIAN_POINT ( 'NONE',  ( 190.1519139143167081, 301.2942192743771557, 4.481136594690903863 ) ) ;
#60480=CARTESIAN_POINT ( 'NONE',  ( 189.0720163204064477, 297.0724856426199949, 8.110046717386847348 ) ) ;
#60482=CARTESIAN_POINT ( 'NONE',  ( 191.8329718516215223, 298.3825415164982928, -8.871589506312979267 ) ) ;
#60484=CARTESIAN_POINT ( 'NONE',  ( 163.9942050550062049, 246.6007000282974673, 5.791111691696777974 ) ) ;
#60487=CARTESIAN_POINT ( 'NONE',  ( 94.78875894111908451, 225.5333772461660544, 9.188101187500095079 ) ) ;
#60488=CARTESIAN_POINT ( 'NONE',  ( 155.3513056799751553, 261.5706408705564741, 18.59020393050806064 ) ) ;
#60490=CARTESIAN_POINT ( 'NONE',  ( 179.4722142099873565, 269.7276464518548096, -17.35046799866735157 ) ) ;
#60492=VERTEX_POINT ( 'NONE', #60237 ) ;
#60494=VERTEX_POINT ( 'NONE', #28873 ) ;
#60497=ORIENTED_EDGE ( 'NONE', *, *, #85085, .F. ) ;
#60501=CARTESIAN_POINT ( 'NONE',  ( 164.4678285797544106, 245.7803600197737524, -6.875991496205872799 ) ) ;
#60503=CARTESIAN_POINT ( 'NONE',  ( 153.1983976505312626, 265.2995869615763809, -17.69657798691567763 ) ) ;
#60506=CARTESIAN_POINT ( 'NONE',  ( 165.0905872925919198, 264.4194027570436560, -17.26892763788675111 ) ) ;
#60510=ORIENTED_EDGE ( 'NONE', *, *, #2518, .F. ) ;
#60513=CARTESIAN_POINT ( 'NONE',  ( 115.5259514080638468, 249.0530062829863311, -4.648177544792955347E-16 ) ) ;
#60515=CARTESIAN_POINT ( 'NONE',  ( 163.1332433029523372, 248.0919295262283981, 11.24052392390482957 ) ) ;
#60516=CARTESIAN_POINT ( 'NONE',  ( 185.4561098074771621, 258.8772088657420909, 2.911598623360981630 ) ) ;
#60517=CARTESIAN_POINT ( 'NONE',  ( 157.8220056349055369, 279.9582903339057793, -6.810428219376026604 ) ) ;
#60518=CARTESIAN_POINT ( 'NONE',  ( 165.5430083683156681, 246.8960659038277470, -2.170161657073390149 ) ) ;
#60519=( BOUNDED_CURVE ( )  B_SPLINE_CURVE ( 2, ( #95323, #2581, #48676, #43028, #49652, #26370, #97289, #87737, #79608 ),
 .UNSPECIFIED., .F., .T. ) 
 B_SPLINE_CURVE_WITH_KNOTS ( ( 3, 2, 2, 2, 3 ),
 ( 0.2056451612903225923, 0.2069892473118279674, 0.2096774193548387177, 0.2123655913978494680, 0.2137096774193548432 ),
 .UNSPECIFIED. ) 
 CURVE ( )  GEOMETRIC_REPRESENTATION_ITEM ( )  RATIONAL_B_SPLINE_CURVE ( ( 0.9330127018922194093, 0.9330127018922194093, 1.000000000000000000, 0.8660254037844387076, 1.000000000000000000, 0.8660254037844387076, 1.000000000000000000, 0.9330127018922194093, 0.9330127018922194093 ) ) 
 REPRESENTATION_ITEM ( '' )  );
#60520=CARTESIAN_POINT ( 'NONE',  ( -13.19378359325312466, 163.1896272461660544, -9.188101187500095079 ) ) ;
#60522=EDGE_CURVE ( 'NONE', #50774, #59643, #86072, .T. ) ;
#60523=CARTESIAN_POINT ( 'NONE',  ( 161.4396252346964218, 251.0253620690641299, 14.51972485405798885 ) ) ;
#60524=CARTESIAN_POINT ( 'NONE',  ( 157.8800731348900399, 281.1895650486539466, 1.630747533558548401 ) ) ;
#60525=ORIENTED_EDGE ( 'NONE', *, *, #62159, .T. ) ;
#60526=CARTESIAN_POINT ( 'NONE',  ( 181.7865378082156553, 270.5830284917279869, -16.18448056385958722 ) ) ;
#60527=CARTESIAN_POINT ( 'NONE',  ( 142.6123662252853421, 259.5780487066560340, -7.305945665944390655 ) ) ;
#60528=EDGE_CURVE ( 'NONE', #38315, #77337, #20702, .T. ) ;
#60529=CARTESIAN_POINT ( 'NONE',  ( 5.633247839328403117, 167.3927522451417929, -10.00000000000009059 ) ) ;
#60532=CARTESIAN_POINT ( 'NONE',  ( 171.5710534622694752, 280.0502575882814540, -15.14474945027508213 ) ) ;
#60533=CARTESIAN_POINT ( 'NONE',  ( 163.3599243854785641, 247.6993063741778940, -7.900958877154002025 ) ) ;
#60536=CARTESIAN_POINT ( 'NONE',  ( -9.459049039432731121, 165.3458772461660544, 9.188101187500095079 ) ) ;
#60538=CARTESIAN_POINT ( 'NONE',  ( 162.8410080103373048, 248.9638863495861472, 10.02562058800860711 ) ) ;
#60543=CARTESIAN_POINT ( 'NONE',  ( 172.6414858973122080, 289.5474176056248439, 2.599858645979187699 ) ) ;
#60545=CARTESIAN_POINT ( 'NONE',  ( 162.4303591677746681, 249.3093605601900435, -10.83980511239089672 ) ) ;
#60548=CARTESIAN_POINT ( 'NONE',  ( 16.84647260051960060, 180.5333772461660544, 9.188101187500095079 ) ) ;
#60549=CARTESIAN_POINT ( 'NONE',  ( 116.7098534265301595, 244.3149278399160949, -9.188101187500095079 ) ) ;
#60551=CARTESIAN_POINT ( 'NONE',  ( 183.1253468672910287, 257.7788483971966684, -2.448293748885121968 ) ) ;
#60552=CARTESIAN_POINT ( 'NONE',  ( 206.6967779005227328, 272.1534147736609270, -6.959009905159835974 ) ) ;
#60553=CARTESIAN_POINT ( 'NONE',  ( 178.5250536166888935, 283.8345237224107791, -14.80487358518624497 ) ) ;
#60555=CARTESIAN_POINT ( 'NONE',  ( 194.1493756275458793, 294.3704124857528655, 13.94613522129020744 ) ) ;
#60556=CARTESIAN_POINT ( 'NONE',  ( 207.4218731373931632, 271.3817724553659332, -5.249531240730909154 ) ) ;
#60558=CARTESIAN_POINT ( 'NONE',  ( 162.8931802014337791, 249.0911889412991229, -10.32038157250286048 ) ) ;
#60559=CARTESIAN_POINT ( 'NONE',  ( 192.6020418108567469, 265.2366636836216003, 7.811029749084129392 ) ) ;
#60561=CYLINDRICAL_SURFACE ( 'NONE', #62592, 10.00000000000010658 ) ;
#60562=CARTESIAN_POINT ( 'NONE',  ( 183.7010204048396815, 267.9445264290289970, -15.94297069647373633 ) ) ;
#60563=CARTESIAN_POINT ( 'NONE',  ( 53.96283019206333620, 190.4155109091896350, 2.679491924311254714 ) ) ;
#60565=CARTESIAN_POINT ( 'NONE',  ( 183.8043731368310603, 268.5938253857621589, 16.29461355553033997 ) ) ;
#60568=CARTESIAN_POINT ( 'NONE',  ( 95.05956542768421969, 219.5643266524160140, 9.188101187500095079 ) ) ;
#60573=CARTESIAN_POINT ( 'NONE',  ( -22.42236680055709641, 157.8615022471902591, 0.000000000000000000 ) ) ;
#60575=CARTESIAN_POINT ( 'NONE',  ( 201.2481467672282633, 270.6558803864813854, -9.957100446674763461 ) ) ;
#60577=CYLINDRICAL_SURFACE ( 'NONE', #73657, 17.82106496071139645 ) ;
#60579=CARTESIAN_POINT ( 'NONE',  ( 147.5749551500760788, 275.0396750858066639, -4.254929048021584670 ) ) ;
#60580=DIRECTION ( 'NONE',  ( 0.4999999999999998890, -0.8660254037844385966, 0.000000000000000000 ) ) ;
#60581=ORIENTED_EDGE ( 'NONE', *, *, #21783, .F. ) ;
#60584=CARTESIAN_POINT ( 'NONE',  ( 147.3236643320416022, 275.4749235501183193, -5.185334239426818037 ) ) ;
#60586=ORIENTED_EDGE ( 'NONE', *, *, #91303, .T. ) ;
#60588=CARTESIAN_POINT ( 'NONE',  ( 159.6610344727618269, 254.1059716346071866, 15.33388637456589620 ) ) ;
#60590=CARTESIAN_POINT ( 'NONE',  ( 183.2995815306362033, 263.9961729758801994, -13.75453846732532526 ) ) ;
#60591=CARTESIAN_POINT ( 'NONE',  ( 186.6673878995319455, 276.5074556901925007, 17.73048906045012529 ) ) ;
#60594=CARTESIAN_POINT ( 'NONE',  ( 186.5306968903125266, 298.6962994122694681, -3.433113405341845059 ) ) ;
#60595=ORIENTED_EDGE ( 'NONE', *, *, #29949, .F. ) ;
#60599=ORIENTED_EDGE ( 'NONE', *, *, #25802, .F. ) ;
#60600=CARTESIAN_POINT ( 'NONE',  ( 204.3821110352445203, 268.7037507017955136, 3.837584713511939416 ) ) ;
#60601=CARTESIAN_POINT ( 'NONE',  ( 159.4943857219621748, 255.4856773835659851, 16.13974565162016006 ) ) ;
#60602=CARTESIAN_POINT ( 'NONE',  ( 190.7811490393836209, 278.9442883317611290, -16.52517045990749978 ) ) ;
#60604=CARTESIAN_POINT ( 'NONE',  ( 153.1627746953036535, 265.3612877299463548, -17.72069958822647351 ) ) ;
#60609=B_SPLINE_CURVE_WITH_KNOTS ( 'NONE', 3,
 ( #4287, #82349, #59968, #67079 ),
 .UNSPECIFIED., .F., .F.,
 ( 4, 4 ),
 ( 0.002191032057283921405, 0.01012571542419986488 ),
 .UNSPECIFIED. ) ;
#60611=EDGE_LOOP ( 'NONE', ( #85803, #54011, #4467, #1222 ) ) ;
#60613=CARTESIAN_POINT ( 'NONE',  ( 198.1939553405634058, 286.4340473833234455, 17.13778683239836553 ) ) ;
#60614=CARTESIAN_POINT ( 'NONE',  ( 164.2981700896163773, 253.9203781951923133, 14.63367134977796802 ) ) ;
#60615=CARTESIAN_POINT ( 'NONE',  ( 164.4936379324916516, 245.7356569095223051, 6.719479797016231437 ) ) ;
#60616=CARTESIAN_POINT ( 'NONE',  ( 189.6567408476656738, 300.3785186016523312, -3.371745498157157961 ) ) ;
#60617=CYLINDRICAL_SURFACE ( 'NONE', #41720, 10.00000000000010658 ) ;
#60618=CARTESIAN_POINT ( 'NONE',  ( 197.4991444394840130, 272.9982161165312959, -13.25291263813902809 ) ) ;
#60621=CARTESIAN_POINT ( 'NONE',  ( 170.8271762237143321, 287.6167538513918203, -4.615125244751493661 ) ) ;
#60623=CARTESIAN_POINT ( 'NONE',  ( 190.7059995949267659, 300.3345147238140385, 2.121218676196247634E-15 ) ) ;
#60625=CARTESIAN_POINT ( 'NONE',  ( 121.5815934185826421, 234.8768266524159856, -9.188101187500091527 ) ) ;
#60627=CARTESIAN_POINT ( 'NONE',  ( 183.3956148285660390, 260.2657049373422069, -9.373603463087153642 ) ) ;
#60629=CARTESIAN_POINT ( 'NONE',  ( 188.1638898588698510, 273.5466134088359240, 15.69418637652080584 ) ) ;
#60631=ORIENTED_EDGE ( 'NONE', *, *, #9358, .T. ) ;
#60632=CIRCLE ( 'NONE', #62288, 10.00000000000007816 ) ;
#60635=CARTESIAN_POINT ( 'NONE',  ( 147.3848241166324158, 275.3689916958264803, 2.889551403030883758 ) ) ;
#60636=CARTESIAN_POINT ( 'NONE',  ( 159.9770824720811220, 253.5585604421560788, -16.42166711341322483 ) ) ;
#60637=CARTESIAN_POINT ( 'NONE',  ( 17.70578863690133886, 169.4824982072973967, 3.021315404115420679E-15 ) ) ;
#60638=EDGE_LOOP ( 'NONE', ( #98394, #14889, #79994, #34101 ) ) ;
#60641=CARTESIAN_POINT ( 'NONE',  ( 38.03703169759608471, 202.7677522451419350, -5.000000000000047962 ) ) ;
#60643=B_SPLINE_CURVE_WITH_KNOTS ( 'NONE', 3,
 ( #50229, #26940, #19851, #5136 ),
 .UNSPECIFIED., .F., .F.,
 ( 4, 4 ),
 ( 2.841188977517477842E-17, 0.006553300831967987308 ),
 .UNSPECIFIED. ) ;
#60645=CARTESIAN_POINT ( 'NONE',  ( 195.6903230345702411, 265.3535381266730155, 4.357112901190284049 ) ) ;
#60646=CARTESIAN_POINT ( 'NONE',  ( 178.7412395063929011, 273.4583285910464951, -17.81739543535002568 ) ) ;
#60650=CARTESIAN_POINT ( 'NONE',  ( 201.4214977800931763, 281.7747274386935601, -17.04225209925078133 ) ) ;
#60652=CARTESIAN_POINT ( 'NONE',  ( 204.6163864379986705, 276.2410179586759682, 14.66911174422491726 ) ) ;
#60654=CARTESIAN_POINT ( 'NONE',  ( 190.4989056847608424, 264.3463537290907084, -9.383834525416400396 ) ) ;
#60655=CARTESIAN_POINT ( 'NONE',  ( 173.1859566361134739, 251.6088681268793152, -0.2708286262129965816 ) ) ;
#60656=CARTESIAN_POINT ( 'NONE',  ( 189.2760668188215902, 269.4823757547970899, -13.97719911248058366 ) ) ;
#60660=CARTESIAN_POINT ( 'NONE',  ( 168.0462690533684338, 251.4142709888886884, 10.74789308012043954 ) ) ;
#60661=CARTESIAN_POINT ( 'NONE',  ( 189.0446170559639256, 298.4692272884965973, 7.774481545468416854 ) ) ;
#60663=CARTESIAN_POINT ( 'NONE',  ( 78.11742282250361313, 228.1589784336661353, -6.496448406907675876E-16 ) ) ;
#60664=CARTESIAN_POINT ( 'NONE',  ( 206.1405152101578437, 273.6011494880188479, -9.618815605734603480 ) ) ;
#60669=CARTESIAN_POINT ( 'NONE',  ( 207.8844858873204657, 270.5805036682629066, -6.251308616122969397 ) ) ;
#60677=B_SPLINE_CURVE_WITH_KNOTS ( 'NONE', 3,
 ( #65039, #73641, #19945, #56429 ),
 .UNSPECIFIED., .F., .F.,
 ( 4, 4 ),
 ( 0.000000000000000000, 0.003851982118655459045 ),
 .UNSPECIFIED. ) ;
#60679=CARTESIAN_POINT ( 'NONE',  ( 29.05227845693028854, 178.3923013555409796, 4.594050593750050204 ) ) ;
#60680=EDGE_CURVE ( 'NONE', #33648, #45420, #53333, .T. ) ;
#60681=CARTESIAN_POINT ( 'NONE',  ( 59.71473008784930414, 205.2833772461660828, -9.188101187500095079 ) ) ;
#60682=CARTESIAN_POINT ( 'NONE',  ( 196.1241105319816143, 290.9500712997905794, 15.97146679939154268 ) ) ;
#60683=CARTESIAN_POINT ( 'NONE',  ( 199.9978482223838512, 277.8398790452972662, 15.22479436670069930 ) ) ;
#60686=CARTESIAN_POINT ( 'NONE',  ( -17.65922707974272399, 170.6115022471903160, -5.000000000000047962 ) ) ;
#60687=CARTESIAN_POINT ( 'NONE',  ( 48.99766571601688270, 199.0958772461660544, -9.188101187500095079 ) ) ;
#60690=CARTESIAN_POINT ( 'NONE',  ( 151.2964716097791325, 268.5938194963972592, -15.66250187539618111 ) ) ;
#60691=CARTESIAN_POINT ( 'NONE',  ( 149.4456112649506281, 271.7996036513546869, -12.95648166494593667 ) ) ;
#60693=CARTESIAN_POINT ( 'NONE',  ( 157.0887340267001946, 258.5613266995183039, -17.61824281915036394 ) ) ;
#60694=CARTESIAN_POINT ( 'NONE',  ( 158.6775083298138043, 256.2244800708343746, -16.16179708298373896 ) ) ;
#60696=CARTESIAN_POINT ( 'NONE',  ( 179.9209375999747351, 276.5811748711908535, 17.74520275588677265 ) ) ;
#60698=CARTESIAN_POINT ( 'NONE',  ( 149.2163037105164278, 275.3995219928863207, 7.552778309360953735 ) ) ;
#60699=CARTESIAN_POINT ( 'NONE',  ( 168.8244094625508751, 257.0541383169796745, -14.93690306707719628 ) ) ;
#60700=CARTESIAN_POINT ( 'NONE',  ( 93.55286852290896604, 231.4865022471903160, 10.00000000000009237 ) ) ;
#60702=CARTESIAN_POINT ( 'NONE',  ( 194.5231616572618520, 285.4348527426450914, -17.22218120948694775 ) ) ;
#60703=ORIENTED_EDGE ( 'NONE', *, *, #13366, .T. ) ;
#60704=CARTESIAN_POINT ( 'NONE',  ( 58.84905177982988533, 192.5327760586659451, 1.948934522072303157E-15 ) ) ;
#60705=VERTEX_POINT ( 'NONE', #73863 ) ;
#60706=CARTESIAN_POINT ( 'NONE',  ( 166.5905980234743140, 264.6682795497030725, 17.25980299922107264 ) ) ;
#60707=CARTESIAN_POINT ( 'NONE',  ( 146.8195026170398023, 276.3481572557323034, 4.765869558735466249 ) ) ;
#60708=DIRECTION ( 'NONE',  ( -0.8660254037844387076, -0.4999999999999998890, -0.000000000000000000 ) ) ;
#60712=CARTESIAN_POINT ( 'NONE',  ( 147.6512387128590262, 274.9075480792844246, -8.209968531507987777 ) ) ;
#60714=CARTESIAN_POINT ( 'NONE',  ( 204.8109598484962532, 275.9040069258922472, 13.12942483889034762 ) ) ;
#60718=CARTESIAN_POINT ( 'NONE',  ( 175.5341286262602978, 254.1345785787596583, 8.090077792417549318 ) ) ;
#60719=DIRECTION ( 'NONE',  ( 0.4999999999999992784, -0.8660254037844390407, 0.000000000000000000 ) ) ;
#60721=CARTESIAN_POINT ( 'NONE',  ( 189.5534384022301424, 269.0062095459838929, -14.92796778812864922 ) ) ;
#60722=CARTESIAN_POINT ( 'NONE',  ( 160.0081047537594543, 253.5048282741223602, -16.11956848123596941 ) ) ;
#60723=AXIS2_PLACEMENT_3D ( 'NONE', #74864, #97184, #74376 ) ;
#60729=CARTESIAN_POINT ( 'NONE',  ( 163.3723087697842971, 247.6778559913402091, -10.08585062664141319 ) ) ;
#60730=CARTESIAN_POINT ( 'NONE',  ( 204.2133777088835700, 276.9390495533970693, 13.75768580338462144 ) ) ;
#60731=CARTESIAN_POINT ( 'NONE',  ( 198.5612432604688991, 286.7288335892616260, 18.30793681285053509 ) ) ;
#60732=DIRECTION ( 'NONE',  ( -0.8660254037844387076, -0.4999999999999998890, -0.000000000000000000 ) ) ;
#60734=CARTESIAN_POINT ( 'NONE',  ( 139.7141738582018604, 239.2202760586659736, -5.415160957724236172E-17 ) ) ;
#60735=CARTESIAN_POINT ( 'NONE',  ( 159.7100847800667509, 255.0739582339791696, -15.92588830848799475 ) ) ;
#60736=CARTESIAN_POINT ( 'NONE',  ( 180.3268137483904354, 258.1330830615356149, 10.30874540274224849 ) ) ;
#60737=CARTESIAN_POINT ( 'NONE',  ( 70.32319418844367931, 223.6589784336661921, -6.496448406907675876E-16 ) ) ;
#60738=ORIENTED_EDGE ( 'NONE', *, *, #65631, .F. ) ;
#60739=CARTESIAN_POINT ( 'NONE',  ( 173.7695364597527430, 265.5330474293953671, 16.17611066364563044 ) ) ;
#60740=LINE ( 'NONE', #46044, #10838 ) ;
#60741=EDGE_CURVE ( 'NONE', #79661, #76651, #63033, .T. ) ;
#60743=CARTESIAN_POINT ( 'NONE',  ( 169.8069776206597226, 261.6727971985682757, -16.70353856883196286 ) ) ;
#60745=ORIENTED_EDGE ( 'NONE', *, *, #80304, .T. ) ;
#60746=CARTESIAN_POINT ( 'NONE',  ( 90.45192255479418009, 211.4824982072973683, 3.021315404115420679E-15 ) ) ;
#60748=CARTESIAN_POINT ( 'NONE',  ( 1.663964738649737374, 161.7677522451418213, -5.000000000000041744 ) ) ;
#60749=CARTESIAN_POINT ( 'NONE',  ( 146.6138605399200117, 276.7043397814778132, -0.5394499176159462950 ) ) ;
#60750=CARTESIAN_POINT ( 'NONE',  ( 110.0795199784619882, 244.3615022471903160, 5.000000000000046185 ) ) ;
#60751=CARTESIAN_POINT ( 'NONE',  ( 154.9910882912764123, 262.1945556895526579, 18.38052604520346023 ) ) ;
#60757=CARTESIAN_POINT ( 'NONE',  ( 161.8319415995885038, 250.3458501924305608, -12.75194401834632529 ) ) ;
#60765=CARTESIAN_POINT ( 'NONE',  ( 142.3122500695552048, 240.7202760586659736, -5.415160957724236172E-17 ) ) ;
#60768=CARTESIAN_POINT ( 'NONE',  ( 182.3318571492640956, 257.5104630292192383, 6.722139348466238395 ) ) ;
#60770=CARTESIAN_POINT ( 'NONE',  ( 152.7295469705997277, 266.1116601603806657, -17.40211458100010589 ) ) ;
#60775=CARTESIAN_POINT ( 'NONE',  ( 198.3172001563159768, 266.5884540843370587, 4.492955043302433893 ) ) ;
#60776=CARTESIAN_POINT ( 'NONE',  ( 181.7549530557583921, 291.6705231334538553, 10.34832551352762309 ) ) ;
#60779=CARTESIAN_POINT ( 'NONE',  ( 202.5909524705457727, 267.2871136637904215, 0.8794807786250381509 ) ) ;
#60780=ORIENTED_EDGE ( 'NONE', *, *, #5945, .T. ) ;
#60781=CARTESIAN_POINT ( 'NONE',  ( 147.5177358149801421, 275.1387818813681179, 4.867883209065928085 ) ) ;
#60782=CARTESIAN_POINT ( 'NONE',  ( 183.5730992744960020, 281.1681395334279046, 17.34192960090523883 ) ) ;
#60784=CARTESIAN_POINT ( 'NONE',  ( 164.9779129355220562, 244.8968679994381148, -1.771286574179712803 ) ) ;
#60785=CARTESIAN_POINT ( 'NONE',  ( 177.2821372360434395, 264.4767462412605141, -15.52096391193404834 ) ) ;
#60786=CARTESIAN_POINT ( 'NONE',  ( 193.5571956648599325, 268.3914742393835695, 12.81656483086835330 ) ) ;
#60787=EDGE_CURVE ( 'NONE', #53616, #66781, #89643, .T. ) ;
#60788=EDGE_CURVE ( 'NONE', #39182, #39202, #56924, .T. ) ;
#60793=AXIS2_PLACEMENT_3D ( 'NONE', #5746, #99961, #29549 ) ;
#60794=CARTESIAN_POINT ( 'NONE',  ( 159.7897726928491409, 253.8829904965402875, 16.83923858130328810 ) ) ;
#60795=( BOUNDED_CURVE ( )  B_SPLINE_CURVE ( 2, ( #27691, #89532, #73290, #3884, #50963, #81916, #60046, #45352, #84893 ),
 .UNSPECIFIED., .F., .T. ) 
 B_SPLINE_CURVE_WITH_KNOTS ( ( 3, 2, 2, 2, 3 ),
 ( 0.8427419354838709964, 0.8440860215053763715, 0.8467741935483871218, 0.8494623655913978721, 0.8508064516129032473 ),
 .UNSPECIFIED. ) 
 CURVE ( )  GEOMETRIC_REPRESENTATION_ITEM ( )  RATIONAL_B_SPLINE_CURVE ( ( 0.9330127018922194093, 0.9330127018922194093, 1.000000000000000000, 0.8660254037844387076, 1.000000000000000000, 0.8660254037844387076, 1.000000000000000000, 0.9330127018922194093, 0.9330127018922194093 ) ) 
 REPRESENTATION_ITEM ( '' )  );
#60796=CARTESIAN_POINT ( 'NONE',  ( -16.14394294671762253, 170.6744531367911293, 4.594050593750047540 ) ) ;
#60797=DIRECTION ( 'NONE',  ( 0.4999999999999992784, -0.8660254037844390407, 0.000000000000000000 ) ) ;
#60799=PRODUCT_DEFINITION_FORMATION_WITH_SPECIFIED_SOURCE ( 'ANY', '', #43521, .NOT_KNOWN. ) ;
#60800=EDGE_CURVE ( 'NONE', #92056, #81006, #9359, .T. ) ;
#60803=CARTESIAN_POINT ( 'NONE',  ( 151.3124059063077311, 268.5662204852269497, -14.45542936000225609 ) ) ;
#60804=CARTESIAN_POINT ( 'NONE',  ( 10.02652254571713719, 176.5958772461660544, -9.188101187500095079 ) ) ;
#60805=CARTESIAN_POINT ( 'NONE',  ( 172.2317120015379430, 290.4289517053596228, 2.752192634013410633 ) ) ;
#60806=CARTESIAN_POINT ( 'NONE',  ( 179.1290479419255064, 274.0445995950666997, -16.71137309026022422 ) ) ;
#60809=CARTESIAN_POINT ( 'NONE',  ( 171.1784325634547201, 271.3965276148621228, -17.73125513023947875 ) ) ;
#60811=CYLINDRICAL_SURFACE ( 'NONE', #99254, 10.00000000000010658 ) ;
#60813=CARTESIAN_POINT ( 'NONE',  ( 175.7745498293659807, 253.0239432584050974, -3.279651895664616124 ) ) ;
#60814=CARTESIAN_POINT ( 'NONE',  ( 198.7606870255174272, 286.3833868549447743, 17.68329551240030284 ) ) ;
#60815=CARTESIAN_POINT ( 'NONE',  ( 44.69460199273685674, 206.6115022471903160, -5.000000000000047962 ) ) ;
#60816=DIRECTION ( 'NONE',  ( -0.8660254037844387076, -0.4999999999999998890, -0.000000000000000000 ) ) ;
#60817=CARTESIAN_POINT ( 'NONE',  ( 189.8763472015711216, 301.7715148217271803, -0.1184663095182975079 ) ) ;
#60818=CARTESIAN_POINT ( 'NONE',  ( 15.22267496842377099, 179.5958772461660544, -9.188101187500095079 ) ) ;
#60820=CARTESIAN_POINT ( 'NONE',  ( 130.4311169673963775, 246.1115022471902591, 10.00000000000009592 ) ) ;
#60822=CARTESIAN_POINT ( 'NONE',  ( 134.5988642195610225, 258.5177522451419350, 5.000000000000046185 ) ) ;
#60823=B_SPLINE_CURVE_WITH_KNOTS ( 'NONE', 3,
 ( #35013, #18843, #18344, #49722 ),
 .UNSPECIFIED., .F., .F.,
 ( 4, 4 ),
 ( 1.520235486122029408E-16, 0.001720210420923555137 ),
 .UNSPECIFIED. ) ;
#60824=CARTESIAN_POINT ( 'NONE',  ( 207.6900289502458179, 270.9173129631602706, 7.178327969100043227 ) ) ;
#60827=B_SPLINE_CURVE_WITH_KNOTS ( 'NONE', 3,
 ( #26111, #49401, #87484, #25089 ),
 .UNSPECIFIED., .F., .F.,
 ( 4, 4 ),
 ( 0.008475005499723171562, 0.01486344536556217372 ),
 .UNSPECIFIED. ) ;
#60828=CARTESIAN_POINT ( 'NONE',  ( 164.1327037607566410, 281.5579544899051712, 8.906674246401461659 ) ) ;
#60833=AXIS2_PLACEMENT_3D ( 'NONE', #72928, #64806, #62785 ) ;
#60834=CARTESIAN_POINT ( 'NONE',  ( 155.5770330754656072, 261.1796695529068302, 18.26969263326161297 ) ) ;
#60835=VERTEX_POINT ( 'NONE', #50058 ) ;
#60836=CARTESIAN_POINT ( 'NONE',  ( 185.4724630939025758, 290.9233636149379549, 12.26262842363110117 ) ) ;
#60838=CARTESIAN_POINT ( 'NONE',  ( 164.6655030961912871, 284.0863298189144643, -8.309311456134647500 ) ) ;
#60839=CARTESIAN_POINT ( 'NONE',  ( -3.985554314188680003, 180.0530062829863311, 2.649461200531984646E-14 ) ) ;
#60841=ORIENTED_EDGE ( 'NONE', *, *, #44688, .F. ) ;
#60845=CARTESIAN_POINT ( 'NONE',  ( 155.5066938333533528, 261.3015006940112244, -18.40036130547566273 ) ) ;
#60846=ORIENTED_EDGE ( 'NONE', *, *, #34279, .F. ) ;
#60848=CARTESIAN_POINT ( 'NONE',  ( 187.4676533354318906, 272.4601757945604845, -16.88503403312462936 ) ) ;
#60849=CARTESIAN_POINT ( 'NONE',  ( 164.4294002498235159, 245.8469198396639399, 6.098783631055905374 ) ) ;
#60851=CARTESIAN_POINT ( 'NONE',  ( 153.2283961777204695, 265.2476279883323400, -17.66880461074566000 ) ) ;
#60853=DIRECTION ( 'NONE',  ( -0.8660254037844387076, -0.4999999999999998890, -0.000000000000000000 ) ) ;
#60855=ORIENTED_EDGE ( 'NONE', *, *, #53722, .T. ) ;
#60856=CARTESIAN_POINT ( 'NONE',  ( 147.8503508990560533, 274.5626756563852950, 7.845851077393495743 ) ) ;
#60857=CARTESIAN_POINT ( 'NONE',  ( 149.5390997184345281, 271.6376768999995761, -11.52989534384373016 ) ) ;
#60858=CARTESIAN_POINT ( 'NONE',  ( 178.9737876148604130, 272.7588148741942291, 17.78336666879676642 ) ) ;
#60859=EDGE_CURVE ( 'NONE', #18980, #100037, #6073, .T. ) ;
#60861=CARTESIAN_POINT ( 'NONE',  ( 205.8918578537579833, 274.0318366629789466, 11.52627491423194250 ) ) ;
#60862=VECTOR ( 'NONE', #36767, 1000.000000000000000 ) ;
#60865=CARTESIAN_POINT ( 'NONE',  ( 149.6036070299368532, 271.5259469590175740, 11.63513718912356865 ) ) ;
#60866=CARTESIAN_POINT ( 'NONE',  ( 156.2224770818481545, 267.4677849582849376, -16.91854127892884208 ) ) ;
#60868=ORIENTED_EDGE ( 'NONE', *, *, #16976, .T. ) ;
#60870=CARTESIAN_POINT ( 'NONE',  ( 88.86189758574327868, 222.1115022471902591, 10.00000000000009592 ) ) ;
#60873=AXIS2_PLACEMENT_3D ( 'NONE', #49290, #23975, #54874 ) ;
#60874=ORIENTED_EDGE ( 'NONE', *, *, #41095, .T. ) ;
#60875=ORIENTED_EDGE ( 'NONE', *, *, #49202, .F. ) ;
#60877=CARTESIAN_POINT ( 'NONE',  ( 146.8729474948188454, 276.2555880120147549, 3.934020695290606273 ) ) ;
#60878=CARTESIAN_POINT ( 'NONE',  ( 147.7978300115112233, 274.6536445020713018, 7.902890709649431855 ) ) ;
#60879=CARTESIAN_POINT ( 'NONE',  ( 149.0761751337341821, 272.4394858007734683, 11.56094486755886130 ) ) ;
#60880=CARTESIAN_POINT ( 'NONE',  ( 153.4289928607825573, 264.9001843414388873, 17.27358709529985958 ) ) ;
#60881=EDGE_CURVE ( 'NONE', #53329, #86782, #78577, .T. ) ;
#60882=CARTESIAN_POINT ( 'NONE',  ( 147.1288613282876554, 275.8123322500870245, 0.6663123207720744734 ) ) ;
#60883=CARTESIAN_POINT ( 'NONE',  ( 147.2592533090473239, 275.5864867145116932, -0.3770461397900867762 ) ) ;
#60885=FACE_OUTER_BOUND ( 'NONE', #95075, .T. ) ;
#60886=B_SPLINE_CURVE_WITH_KNOTS ( 'NONE', 3,
 ( #6615, #16, #84641, #45589 ),
 .UNSPECIFIED., .F., .F.,
 ( 4, 4 ),
 ( 5.779565477066665081E-15, 0.005039604220546898931 ),
 .UNSPECIFIED. ) ;
#60888=LINE ( 'NONE', #91851, #40145 ) ;
#60890=CARTESIAN_POINT ( 'NONE',  ( 171.5146568604302502, 288.8597905981943654, 4.230659075081162790 ) ) ;
#60892=CARTESIAN_POINT ( 'NONE',  ( 104.3964885861764600, 221.8923013555410080, 4.594050593750050204 ) ) ;
#60893=ORIENTED_EDGE ( 'NONE', *, *, #78407, .F. ) ;
#60894=DIRECTION ( 'NONE',  ( -0.8660254037844387076, -0.4999999999999998890, -0.000000000000000000 ) ) ;
#60896=CARTESIAN_POINT ( 'NONE',  ( 200.3293654959697392, 273.7156512906800572, 13.98704503334941229 ) ) ;
#60897=EDGE_CURVE ( 'NONE', #49659, #66923, #7327, .T. ) ;
#60900=CARTESIAN_POINT ( 'NONE',  ( -17.42236680055705023, 149.2012482093457777, 0.000000000000000000 ) ) ;
#60901=CARTESIAN_POINT ( 'NONE',  ( 189.8305642146623029, 301.8508132811754763, -0.4120780911254784407 ) ) ;
#60904=CARTESIAN_POINT ( 'NONE',  ( 208.2124092825819162, 270.0125236866795149, -2.339659020816897694 ) ) ;
#60905=FACE_OUTER_BOUND ( 'NONE', #57784, .T. ) ;
#60907=CARTESIAN_POINT ( 'NONE',  ( 37.53185021205516847, 199.1427522451419065, 10.00000000000009237 ) ) ;
#60908=CARTESIAN_POINT ( 'NONE',  ( 118.1174918034448922, 232.8768266524160140, 9.188101187500096856 ) ) ;
#60909=CARTESIAN_POINT ( 'NONE',  ( 198.9369963555428740, 286.0780101374919013, -18.58432392708837710 ) ) ;
#60911=CARTESIAN_POINT ( 'NONE',  ( 157.8849654228661166, 257.1822134667773980, 17.43614750057631468 ) ) ;
#60913=CARTESIAN_POINT ( 'NONE',  ( 37.57712925149210292, 186.3768266524160140, 9.188101187500098632 ) ) ;
#60914=VECTOR ( 'NONE', #66392, 1000.000000000000000 ) ;
#60918=CARTESIAN_POINT ( 'NONE',  ( 178.9948746410809690, 264.1102681154287097, -15.56640332105143720 ) ) ;
#60919=CARTESIAN_POINT ( 'NONE',  ( 178.1274316576357819, 265.4983894697847404, 15.93396044624996399 ) ) ;
#60920=EDGE_CURVE ( 'NONE', #16011, #36668, #74993, .T. ) ;
#60921=B_SPLINE_SURFACE_WITH_KNOTS ( 'NONE', 3, 1, ( 
 ( #53073, #83521 ),
 ( #14084, #89638 ),
 ( #90122, #43472 ),
 ( #44466, #84028 ),
 ( #90637, #6974 ),
 ( #20200, #76399 ),
 ( #82541, #37858 ),
 ( #52078, #75398 ),
 ( #75908, #5001 ),
 ( #74416, #5982 ),
 ( #35878, #36877 ),
 ( #97707, #13105 ),
 ( #7467, #99691 ),
 ( #69269, #84518 ),
 ( #54051, #30275 ),
 ( #77385, #38360 ),
 ( #46455, #94116 ),
 ( #78392, #70775 ),
 ( #70264, #377 ),
 ( #92133, #7987 ),
 ( #31751, #23655 ),
 ( #24177, #61164 ),
 ( #85009, #38863 ),
 ( #77893, #47958 ),
 ( #31265, #32269 ),
 ( #15061, #69769 ),
 ( #55060, #62657 ),
 ( #1389, #93608 ),
 ( #8973, #86043 ),
 ( #15553, #23160 ),
 ( #39843, #100198 ),
 ( #40356, #63172 ),
 ( #76869, #62152 ),
 ( #85529, #16571 ) ),
 .UNSPECIFIED., .T., .F., .F.,
 ( 4, 2, 2, 2, 2, 2, 2, 2, 2, 2, 2, 2, 2, 2, 2, 2, 4 ),
 ( 2, 2 ),
 ( 0.000000000000000000, 0.06250000000000000000, 0.1250000000000000000, 0.1875000000000000000, 0.2500000000000000000, 0.3125000000000000000, 0.3750000000000000000, 0.4375000000000000000, 0.5000000000000000000, 0.5625000000000000000, 0.6250000000000000000, 0.6875000000000000000, 0.7500000000000000000, 0.8125000000000000000, 0.8750000000000000000, 0.9375000000000000000, 1.000000000000000000 ),
 ( 0.000000000000000000, 1.000000000000000000 ),
 .UNSPECIFIED. ) ;
#60928=EDGE_CURVE ( 'NONE', #35860, #80312, #97960, .T. ) ;
#60929=CARTESIAN_POINT ( 'NONE',  ( 106.0921946783233096, 225.3927522451418213, 10.00000000000009592 ) ) ;
#60932=CARTESIAN_POINT ( 'NONE',  ( 161.2977680094314223, 251.2710659906439616, -13.03191437619249982 ) ) ;
#60934=CARTESIAN_POINT ( 'NONE',  ( 155.4040338355446522, 279.7651995206167612, -2.031698524654040661 ) ) ;
#60935=CARTESIAN_POINT ( 'NONE',  ( 154.2086446512540761, 265.3719949574480665, 17.07260120196946573 ) ) ;
#60938=CARTESIAN_POINT ( 'NONE',  ( 21.69106252476256458, 174.1423013555409796, -4.594050593750043987 ) ) ;
#60945=CARTESIAN_POINT ( 'NONE',  ( 195.5687578856996822, 275.7294477338082288, -15.46242989827094227 ) ) ;
#60946=CARTESIAN_POINT ( 'NONE',  ( 71.67687952550437558, 206.0643266524160140, 9.188101187500095079 ) ) ;
#60947=CARTESIAN_POINT ( 'NONE',  ( 208.3135187673106543, 269.8373969220020285, 2.829653198597726682 ) ) ;
#60950=CARTESIAN_POINT ( 'NONE',  ( 164.9836323268835940, 244.8869617230113249, -2.696511969808454534 ) ) ;
#60952=CARTESIAN_POINT ( 'NONE',  ( 163.0340262847632289, 267.8216940496866982, 16.48747052884350950 ) ) ;
#60953=CARTESIAN_POINT ( 'NONE',  ( 17.48697055717582316, 174.2365022471902023, -10.00000000000009059 ) ) ;
#60954=CARTESIAN_POINT ( 'NONE',  ( 163.9910908123517288, 246.6060940548019289, -7.333295033952830444 ) ) ;
#60955=CARTESIAN_POINT ( 'NONE',  ( 137.6570164284488271, 250.2833772461660544, -9.188101187500095079 ) ) ;
#60957=CARTESIAN_POINT ( 'NONE',  ( 167.6212268600468462, 262.3307149636390818, -17.03867496724294028 ) ) ;
#60958=LINE ( 'NONE', #5288, #85672 ) ;
#60960=CARTESIAN_POINT ( 'NONE',  ( 203.9914640947099826, 268.0458192746789337, 1.179109546621946114 ) ) ;
#60961=CARTESIAN_POINT ( 'NONE',  ( 170.4623819437503016, 288.8056674672355939, -5.476885062779371260 ) ) ;
#60963=EDGE_LOOP ( 'NONE', ( #90984, #37325, #14469, #7326 ) ) ;
#60964=CARTESIAN_POINT ( 'NONE',  ( 64.58718584504546811, 196.5494855054052152, -2.679491924311248496 ) ) ;
#60966=CARTESIAN_POINT ( 'NONE',  ( 170.8843335314017509, 274.4719442773359219, 17.28596511953734449 ) ) ;
#60970=CARTESIAN_POINT ( 'NONE',  ( 206.7474059308681262, 272.5499839251064031, 9.504501883383504435 ) ) ;
#60971=CARTESIAN_POINT ( 'NONE',  ( -14.42967401501114999, 169.1427522451419065, 10.00000000000009415 ) ) ;
#60973=CARTESIAN_POINT ( 'NONE',  ( 31.27120823407814854, 178.8615022471902023, 5.000000000000051514 ) ) ;
#60974=CARTESIAN_POINT ( 'NONE',  ( 175.8759543544349810, 265.7665519414402979, 16.89567470503287794 ) ) ;
#60975=CARTESIAN_POINT ( 'NONE',  ( 208.0006710756887287, 270.3792650189220126, -0.8737665032493013850 ) ) ;
#60977=VERTEX_POINT ( 'NONE', #39312 ) ;
#60981=VERTEX_POINT ( 'NONE', #1348 ) ;
#60982=CARTESIAN_POINT ( 'NONE',  ( 149.6700657135140489, 271.4108371424580355, 12.58635654151485284 ) ) ;
#60984=CARTESIAN_POINT ( 'NONE',  ( 189.1253271041844073, 297.0913391992372112, 8.133032840077193626 ) ) ;
#60986=CARTESIAN_POINT ( 'NONE',  ( 191.8210230231139803, 298.4032374945642232, -8.800268167321144475 ) ) ;
#60987=CARTESIAN_POINT ( 'NONE',  ( 162.9254136962317148, 277.9293967287522946, 13.77390558128574760 ) ) ;
#60988=CARTESIAN_POINT ( 'NONE',  ( 163.8670932201372352, 246.8208641845333773, 5.912697114930636211 ) ) ;
#60991=ORIENTED_EDGE ( 'NONE', *, *, #65121, .F. ) ;
#60992=CARTESIAN_POINT ( 'NONE',  ( 101.1217432541752856, 223.0643266524159571, -9.188101187500093303 ) ) ;
#60993=CARTESIAN_POINT ( 'NONE',  ( 200.1102648775588193, 284.0458494464393198, 17.54251420653697835 ) ) ;
#60996=ORIENTED_EDGE ( 'NONE', *, *, #21395, .F. ) ;
#61002=CARTESIAN_POINT ( 'NONE',  ( 163.7323023463233937, 247.0543288263758086, -6.244751637846886361 ) ) ;
#61004=CARTESIAN_POINT ( 'NONE',  ( 169.2996641469526367, 281.9763651243665095, 11.69048842974035018 ) ) ;
#61010=CARTESIAN_POINT ( 'NONE',  ( 201.6553334440559695, 279.0490965050211116, -15.83750187978207435 ) ) ;
#61012=CARTESIAN_POINT ( 'NONE',  ( 123.7735466722555771, 232.2677522451417929, -5.000000000000041744 ) ) ;
#61013=ORIENTED_EDGE ( 'NONE', *, *, #49498, .F. ) ;
#61014=CIRCLE ( 'NONE', #41637, 17.82106496071138935 ) ;
#61015=CARTESIAN_POINT ( 'NONE',  ( 203.0507839702407580, 278.9527209772879814, 16.21318481136342626 ) ) ;
#61016=CARTESIAN_POINT ( 'NONE',  ( 188.7366574086433388, 259.9223475325732124, 2.251677873538305175 ) ) ;
#61019=CARTESIAN_POINT ( 'NONE',  ( 182.0925017600785054, 256.7772607896355339, 6.510642260905229683 ) ) ;
#61020=EDGE_CURVE ( 'NONE', #97169, #59501, #59151, .T. ) ;
#61021=CARTESIAN_POINT ( 'NONE',  ( 171.5232944563295234, 255.4040756630877524, 11.03579953863793328 ) ) ;
#61022=CARTESIAN_POINT ( 'NONE',  ( 192.2546761845801200, 262.7471528669759664, -0.7532661484371161453 ) ) ;
#61023=EDGE_LOOP ( 'NONE', ( #82862, #63125, #98040, #15112 ) ) ;
#61024=CARTESIAN_POINT ( 'NONE',  ( 181.8631805538818469, 270.4478486503479076, -17.10574755700200456 ) ) ;
#61028=CARTESIAN_POINT ( 'NONE',  ( 3.035171627975086217, 165.8927522451417929, -10.00000000000009059 ) ) ;
#61030=CARTESIAN_POINT ( 'NONE',  ( 193.9656327198519250, 268.1476455479440801, -10.86522118760852251 ) ) ;
#61031=CARTESIAN_POINT ( 'NONE',  ( 172.3697519336014921, 280.6551101671673223, -15.35839400997692650 ) ) ;
#61032=CARTESIAN_POINT ( 'NONE',  ( 163.4595051773099215, 247.5268273832681132, -8.749824153777744584 ) ) ;
#61034=CARTESIAN_POINT ( 'NONE',  ( 162.5256129416874558, 250.7632698397880233, -12.89907038147651619 ) ) ;
#61035=CARTESIAN_POINT ( 'NONE',  ( -4.262896616726100874, 168.3458772461660544, 9.188101187500095079 ) ) ;
#61037=CARTESIAN_POINT ( 'NONE',  ( 58.36827475829091583, 216.0530062829863311, -4.648177544792955347E-16 ) ) ;
#61039=VERTEX_POINT ( 'NONE', #9443 ) ;
#61043=CARTESIAN_POINT ( 'NONE',  ( 193.5005633302724277, 262.8551920378705518, -5.236817587991198231 ) ) ;
#61044=CARTESIAN_POINT ( 'NONE',  ( 202.2805801041352254, 280.2867532055686297, -17.40773220476747696 ) ) ;
#61045=CARTESIAN_POINT ( 'NONE',  ( 198.8683739244561082, 276.4215138120039796, -15.93986209720707414 ) ) ;
#61046=CARTESIAN_POINT ( 'NONE',  ( 150.0128543151502072, 276.7587017117480173, 3.258831262238442772 ) ) ;
#61047=EDGE_CURVE ( 'NONE', #97906, #40669, #4315, .T. ) ;
#61048=B_SPLINE_CURVE_WITH_KNOTS ( 'NONE', 3,
 ( #25952, #2651, #4122, #88294 ),
 .UNSPECIFIED., .F., .F.,
 ( 4, 4 ),
 ( 0.01040196219446366636, 0.01876899884930364679 ),
 .UNSPECIFIED. ) ;
#61049=CARTESIAN_POINT ( 'NONE',  ( 19.09298631340924501, 172.6423013555409796, -4.594050593750043987 ) ) ;
#61050=CARTESIAN_POINT ( 'NONE',  ( 112.3797264076079756, 241.8149278399160949, 9.188101187500093303 ) ) ;
#61051=CARTESIAN_POINT ( 'NONE',  ( 181.3848234261387802, 294.5949326645637711, -6.610599456467063817 ) ) ;
#61052=CARTESIAN_POINT ( 'NONE',  ( 183.4174296676025904, 257.2981747246719806, -3.184370871148272109 ) ) ;
#61053=CARTESIAN_POINT ( 'NONE',  ( 149.9951969083232370, 271.6664457055391040, -11.69466652306437560 ) ) ;
#61058=CARTESIAN_POINT ( 'NONE',  ( 195.8449251089225811, 291.4336346372613775, 16.14492769602857081 ) ) ;
#61061=CARTESIAN_POINT ( 'NONE',  ( 207.5462191418491500, 271.1663988579299485, -5.239401497773396699 ) ) ;
#61062=CARTESIAN_POINT ( 'NONE',  ( 189.2296340506370029, 284.2231390282569237, 16.49936049877286592 ) ) ;
#61064=CARTESIAN_POINT ( 'NONE',  ( 168.0319076612829861, 278.6233240676867240, 14.86836655933751317 ) ) ;
#61065=CARTESIAN_POINT ( 'NONE',  ( 189.2051289032725947, 299.6734310816647167, -0.5827320972813355704 ) ) ;
#61068=CARTESIAN_POINT ( 'NONE',  ( 184.3466702497243830, 268.6818309632849946, -15.29285969151670521 ) ) ;
#61069=VERTEX_POINT ( 'NONE', #47922 ) ;
#61070=CARTESIAN_POINT ( 'NONE',  ( 166.5497620933320775, 284.9599651698292178, -8.643830016708903941 ) ) ;
#61071=CARTESIAN_POINT ( 'NONE',  ( 181.4153963986084079, 267.9065476240749604, 15.01311212035915332 ) ) ;
#61072=CARTESIAN_POINT ( 'NONE',  ( 99.71410487726056715, 234.5024278399160949, 9.188101187500095079 ) ) ;
#61073=CARTESIAN_POINT ( 'NONE',  ( 207.8431546909062320, 270.6520914003897360, -6.441273666418043220 ) ) ;
#61074=CARTESIAN_POINT ( 'NONE',  ( 151.3589047706063582, 268.4856820897672378, 14.56544807350869419 ) ) ;
#61076=AXIS2_PLACEMENT_3D ( 'NONE', #1586, #32956, #65360 ) ;
#61078=CARTESIAN_POINT ( 'NONE',  ( 191.6900977084123951, 277.0292895703833551, 16.71431191694982843 ) ) ;
#61079=CARTESIAN_POINT ( 'NONE',  ( 201.9158970844873977, 271.2653056115948402, -9.820632838803758702 ) ) ;
#61080=CARTESIAN_POINT ( 'NONE',  ( 198.4427928769277969, 286.9339956717308837, -17.97122743692687763 ) ) ;
#61084=CARTESIAN_POINT ( 'NONE',  ( 174.4279836968870541, 287.7471250269960592, -10.96444086789414030 ) ) ;
#61089=CARTESIAN_POINT ( 'NONE',  ( 192.8607783413999073, 296.6023284558532396, -11.80574095728561446 ) ) ;
#61090=CARTESIAN_POINT ( 'NONE',  ( 196.4783028304046013, 290.3365922432724346, -16.37291435488387492 ) ) ;
#61093=CARTESIAN_POINT ( 'NONE',  ( 183.4250023545107524, 264.1063932265387280, -13.71376836473408645 ) ) ;
#61094=CARTESIAN_POINT ( 'NONE',  ( 169.3341204084158846, 252.1170729295009778, -8.741246645408743632 ) ) ;
#61098=CARTESIAN_POINT ( 'NONE',  ( 187.2681015796103736, 278.8103706783136317, 17.45891525344013218 ) ) ;
#61101=CARTESIAN_POINT ( 'NONE',  ( 168.2356071464602962, 248.8554872198452301, 6.669745218284529820 ) ) ;
#61103=FACE_OUTER_BOUND ( 'NONE', #100185, .T. ) ;
#61104=EDGE_LOOP ( 'NONE', ( #97651, #32978, #79110, #60280 ) ) ;
#61107=CARTESIAN_POINT ( 'NONE',  ( 190.5068628727836710, 278.6829438244865855, -16.50779966355658601 ) ) ;
#61108=CARTESIAN_POINT ( 'NONE',  ( 153.5862473704880244, 264.6278115409098746, -16.56056475222486668 ) ) ;
#61109=CARTESIAN_POINT ( 'NONE',  ( 200.8665851640556070, 282.7358642834317948, -16.69422397739980823 ) ) ;
#61113=( BOUNDED_CURVE ( )  B_SPLINE_CURVE ( 2, ( #91434, #97532, #5802, #73718, #35205, #35707, #66605, #28101, #58974 ),
 .UNSPECIFIED., .F., .T. ) 
 B_SPLINE_CURVE_WITH_KNOTS ( ( 3, 2, 2, 2, 3 ),
 ( 0.6330645161290322509, 0.6344086021505376261, 0.6370967741935483764, 0.6397849462365591267, 0.6411290322580645018 ),
 .UNSPECIFIED. ) 
 CURVE ( )  GEOMETRIC_REPRESENTATION_ITEM ( )  RATIONAL_B_SPLINE_CURVE ( ( 0.9330127018922194093, 0.9330127018922194093, 1.000000000000000000, 0.8660254037844387076, 1.000000000000000000, 0.8660254037844387076, 1.000000000000000000, 0.9330127018922194093, 0.9330127018922194093 ) ) 
 REPRESENTATION_ITEM ( '' )  );
#61115=CARTESIAN_POINT ( 'NONE',  ( 196.1831030080164169, 290.3823853032309898, 16.15582348271726332 ) ) ;
#61118=CARTESIAN_POINT ( 'NONE',  ( 198.2391837281077756, 286.3575794386269422, 17.25947343406376078 ) ) ;
#61122=CARTESIAN_POINT ( 'NONE',  ( 164.4811395904728784, 246.2125872648383620, 1.945510398998699042 ) ) ;
#61124=CARTESIAN_POINT ( 'NONE',  ( 197.6875078399188794, 272.6683531706096915, -13.23822772498251155 ) ) ;
#61126=CARTESIAN_POINT ( 'NONE',  ( 189.8171280724701546, 301.8740853621098950, -0.4360232994423257624 ) ) ;
#61128=CARTESIAN_POINT ( 'NONE',  ( 171.6228816214248809, 250.6675204659138956, -5.726922243694214210 ) ) ;
#61130=ADVANCED_FACE ( 'NONE', ( #62619 ), #90274, .F. ) ;
#61131=CARTESIAN_POINT ( 'NONE',  ( 183.4234925895679567, 284.6666860932168674, -15.01880897167392703 ) ) ;
#61132=CARTESIAN_POINT ( 'NONE',  ( 110.0524566828198232, 234.3458772461660544, 9.188101187500095079 ) ) ;
#61133=ORIENTED_EDGE ( 'NONE', *, *, #84637, .T. ) ;
#61141=CARTESIAN_POINT ( 'NONE',  ( 180.2423226582527604, 295.0003840256651415, -2.029293836717157351 ) ) ;
#61142=CARTESIAN_POINT ( 'NONE',  ( 204.9090237380674182, 269.5176180222230755, 5.449509932175979010 ) ) ;
#61143=CARTESIAN_POINT ( 'NONE',  ( 190.4356836585210431, 300.3996184492839916, -0.5836641476860114919 ) ) ;
#61144=ADVANCED_FACE ( 'NONE', ( #86726 ), #37681, .T. ) ;
#61147=CARTESIAN_POINT ( 'NONE',  ( 148.5647453719543591, 273.3253081326787992, 9.005903527242661966 ) ) ;
#61148=EDGE_CURVE ( 'NONE', #68725, #63243, #60415, .T. ) ;
#61149=VECTOR ( 'NONE', #10266, 1000.000000000000000 ) ;
#61153=ORIENTED_EDGE ( 'NONE', *, *, #97284, .T. ) ;
#61154=CARTESIAN_POINT ( 'NONE',  ( 188.3408396332539212, 265.5067415902187804, -11.62187238349581975 ) ) ;
#61156=B_SPLINE_CURVE_WITH_KNOTS ( 'NONE', 3,
 ( #68935, #9671, #86205, #61830 ),
 .UNSPECIFIED., .F., .F.,
 ( 4, 4 ),
 ( 0.04659044411497612059, 0.04887120950165271815 ),
 .UNSPECIFIED. ) ;
#61157=CARTESIAN_POINT ( 'NONE',  ( 195.2523433541918791, 265.1293616091613217, 4.413780863583922631 ) ) ;
#61158=CARTESIAN_POINT ( 'NONE',  ( 187.9334280069057570, 258.7324837002516347, 0.4517059538649245143 ) ) ;
#61159=CARTESIAN_POINT ( 'NONE',  ( 202.7865629936218284, 279.4103651332174536, 17.10878160033216133 ) ) ;
#61160=CARTESIAN_POINT ( 'NONE',  ( 187.1742838492968986, 290.8334520998986363, -13.54031411274703522 ) ) ;
#61161=CARTESIAN_POINT ( 'NONE',  ( 160.7349768583320042, 281.5384896374872596, 5.620271226638340778 ) ) ;
#61162=FACE_OUTER_BOUND ( 'NONE', #47653, .T. ) ;
#61164=CARTESIAN_POINT ( 'NONE',  ( 147.3023124603499809, 275.5119060767245287, 5.196938859334171212 ) ) ;
#61165=B_SPLINE_SURFACE_WITH_KNOTS ( 'NONE', 3, 1, ( 
 ( #62147, #76393 ),
 ( #30269, #15548 ),
 ( #61159, #57558 ),
 ( #64681, #88039 ),
 ( #48979, #47952 ),
 ( #72297, #33797 ),
 ( #72808, #80421 ),
 ( #18588, #79419 ),
 ( #26179, #64172 ),
 ( #94607, #65166 ),
 ( #95631, #49466 ),
 ( #41866, #17570 ),
 ( #19096, #3397 ),
 ( #34272, #71288 ),
 ( #48477, #1881 ),
 ( #40845, #33269 ),
 ( #25162, #95120 ),
 ( #96618, #11500 ),
 ( #3876, #9480 ),
 ( #63668, #41355 ),
 ( #57057, #56565 ),
 ( #78895, #40351 ),
 ( #79916, #2904 ),
 ( #17061, #56045 ),
 ( #10994, #26672 ),
 ( #32762, #87037 ),
 ( #88534, #96118 ),
 ( #49974, #80931 ),
 ( #42352, #9985 ),
 ( #71791, #2389 ),
 ( #73283, #10478 ),
 ( #25685, #87551 ),
 ( #18084, #55547 ),
 ( #65659, #34759 ) ),
 .UNSPECIFIED., .T., .F., .F.,
 ( 4, 2, 2, 2, 2, 2, 2, 2, 2, 2, 2, 2, 2, 2, 2, 2, 4 ),
 ( 2, 2 ),
 ( 0.000000000000000000, 0.06250000000000000000, 0.1250000000000000000, 0.1875000000000000000, 0.2500000000000000000, 0.3125000000000000000, 0.3750000000000000000, 0.4375000000000000000, 0.5000000000000000000, 0.5625000000000000000, 0.6250000000000000000, 0.6875000000000000000, 0.7500000000000000000, 0.8125000000000000000, 0.8750000000000000000, 0.9375000000000000000, 1.000000000000000000 ),
 ( 0.000000000000000000, 1.000000000000000000 ),
 .UNSPECIFIED. ) ;
#61169=CARTESIAN_POINT ( 'NONE',  ( 192.3395334592007941, 271.2003706416659838, -15.16840763204049658 ) ) ;
#61170=CARTESIAN_POINT ( 'NONE',  ( 172.2467550100553808, 258.4300157609564508, -14.58559033337875377 ) ) ;
#61173=CARTESIAN_POINT ( 'NONE',  ( 194.4904290197884507, 293.7796906822950973, 14.50206953321744940 ) ) ;
#61174=CARTESIAN_POINT ( 'NONE',  ( 33.86928444543146810, 180.3615022471902023, 5.000000000000051514 ) ) ;
#61178=CARTESIAN_POINT ( 'NONE',  ( 74.03095222233704931, 222.7369531367911293, -4.594050593750048428 ) ) ;
#61179=CARTESIAN_POINT ( 'NONE',  ( 206.3423291502491566, 273.2515974901050413, -10.76717883871977577 ) ) ;
#61180=CARTESIAN_POINT ( 'NONE',  ( 192.6247335881259630, 297.0111699613833594, -13.30158778996737290 ) ) ;
#61181=CARTESIAN_POINT ( 'NONE',  ( 163.4222916751007801, 247.5912830598222172, -10.52132777929285012 ) ) ;
#61183=CARTESIAN_POINT ( 'NONE',  ( 207.8570869662935365, 270.6279599915536664, -5.669188455878507504 ) ) ;
#61187=CARTESIAN_POINT ( 'NONE',  ( 191.4155626767636704, 260.8708449615334075, 2.063941295486333427 ) ) ;
#61189=CARTESIAN_POINT ( 'NONE',  ( 205.3054132066514796, 275.0475885875939639, -12.25171873544422141 ) ) ;
#61190=CARTESIAN_POINT ( 'NONE',  ( 157.8740713127050981, 257.2010826190796706, 17.31862062017425075 ) ) ;
#61192=CARTESIAN_POINT ( 'NONE',  ( 33.19304919271588972, 177.7202760586659736, -5.415160957724236172E-17 ) ) ;
#61194=CARTESIAN_POINT ( 'NONE',  ( 44.66719160132967659, 208.8464784336661353, 1.353441290958777327E-15 ) ) ;
#61195=CARTESIAN_POINT ( 'NONE',  ( 157.8562613713738472, 257.2319303423452652, 17.81420683562559404 ) ) ;
#61199=CARTESIAN_POINT ( 'NONE',  ( 142.5284093247362591, 253.0958772461660544, -9.188101187500095079 ) ) ;
#61200=CARTESIAN_POINT ( 'NONE',  ( 52.62397354648171444, 207.3149278399161233, 9.188101187500093303 ) ) ;
#61202=EDGE_CURVE ( 'NONE', #41077, #34164, #24196, .T. ) ;
#61204=CARTESIAN_POINT ( 'NONE',  ( -12.96825614257699399, 169.9865022471903160, 10.00000000000009415 ) ) ;
#61205=CARTESIAN_POINT ( 'NONE',  ( 149.7072529793668707, 271.3464269086063041, -11.98883662638834657 ) ) ;
#61207=CARTESIAN_POINT ( 'NONE',  ( 205.0520875136525376, 275.4863615587311756, -14.16385635411862509 ) ) ;
#61210=AXIS2_PLACEMENT_3D ( 'NONE', #37842, #851, #39330 ) ;
#61211=CARTESIAN_POINT ( 'NONE',  ( 198.1300353965528984, 287.4757075181870505, 18.48278456664528946 ) ) ;
#61213=CARTESIAN_POINT ( 'NONE',  ( 153.3133634134964609, 265.1004604189892575, 17.35325068284992867 ) ) ;
#61217=CARTESIAN_POINT ( 'NONE',  ( 104.4503548538631463, 241.1115022471902876, -5.000000000000047962 ) ) ;
#61218=CYLINDRICAL_SURFACE ( 'NONE', #39327, 10.00000000000010658 ) ;
#61219=CARTESIAN_POINT ( 'NONE',  ( 193.3529349556220325, 284.7064891731757825, -16.83000617485832962 ) ) ;
#61220=ORIENTED_EDGE ( 'NONE', *, *, #77788, .F. ) ;
#61223=CARTESIAN_POINT ( 'NONE',  ( 206.0870578475358172, 273.6937403561189512, -10.07771901274806581 ) ) ;
#61224=CARTESIAN_POINT ( 'NONE',  ( 190.1526130375667094, 278.5908336017399165, -16.50440980714951777 ) ) ;
#61225=CARTESIAN_POINT ( 'NONE',  ( 192.3713340522295709, 271.8780416168410170, 15.57788208939756380 ) ) ;
#61228=CARTESIAN_POINT ( 'NONE',  ( 194.8708600166808651, 293.1207648669033006, -14.79199694356877970 ) ) ;
#61229=CARTESIAN_POINT ( 'NONE',  ( 175.7622132985686392, 274.0430017844784629, -17.75579533532145504 ) ) ;
#61234=CARTESIAN_POINT ( 'NONE',  ( 172.4831635826484444, 290.8796410925290843, -1.652085212636280609 ) ) ;
#61235=DIRECTION ( 'NONE',  ( -0.8660254037844387076, -0.4999999999999998890, -0.000000000000000000 ) ) ;
#61237=CARTESIAN_POINT ( 'NONE',  ( 198.4160757083882345, 267.1808215963346242, -8.346050686629251203 ) ) ;
#61239=VERTEX_POINT ( 'NONE', #48682 ) ;
#61240=CARTESIAN_POINT ( 'NONE',  ( 174.7533417775181306, 286.2318505546784877, 11.43544241327690258 ) ) ;
#61241=CARTESIAN_POINT ( 'NONE',  ( 159.9924463476198753, 283.3850188831759169, -3.371971149216307140 ) ) ;
#61243=CARTESIAN_POINT ( 'NONE',  ( 162.6541320028305506, 248.9217746405196294, -10.16950121496441817 ) ) ;
#61244=CARTESIAN_POINT ( 'NONE',  ( 204.5831314780710954, 276.2986172388744421, 13.28075685133257089 ) ) ;
#61245=CARTESIAN_POINT ( 'NONE',  ( 188.6535065314160704, 295.1378203055187441, -11.17103305312315520 ) ) ;
#61246=CARTESIAN_POINT ( 'NONE',  ( 161.0164413264604661, 262.9588007402923040, -17.56398238099813014 ) ) ;
#61247=CARTESIAN_POINT ( 'NONE',  ( 129.8627877943888791, 245.7833772461660544, -9.188101187500095079 ) ) ;
#61248=CARTESIAN_POINT ( 'NONE',  ( 202.9785155578410354, 267.9986174989653591, 2.523388936575725161 ) ) ;
#61249=CARTESIAN_POINT ( 'NONE',  ( 195.6979370051232934, 290.6267181618097766, -16.31163916660881341 ) ) ;
#61250=CARTESIAN_POINT ( 'NONE',  ( 67.72511797709034909, 222.1589784336661637, -6.496448406907675876E-16 ) ) ;
#61257=ORIENTED_EDGE ( 'NONE', *, *, #86975, .T. ) ;
#61260=CARTESIAN_POINT ( 'NONE',  ( 194.2695434292520247, 284.8040030035346604, 17.71845281746924883 ) ) ;
#61263=CARTESIAN_POINT ( 'NONE',  ( 155.6559071247401960, 261.0430556921643870, 17.79853447468815375 ) ) ;
#61266=CARTESIAN_POINT ( 'NONE',  ( 76.60222546164588664, 215.0333772461660544, 9.188101187500095079 ) ) ;
#61267=EDGE_LOOP ( 'NONE', ( #28985, #4443, #30115, #77751 ) ) ;
#61269=CARTESIAN_POINT ( 'NONE',  ( 161.6539040693529046, 250.6542202404525312, -12.66790845110597807 ) ) ;
#61270=ADVANCED_FACE ( 'NONE', ( #64877 ), #97294, .T. ) ;
#61271=EDGE_LOOP ( 'NONE', ( #46331, #29152, #83387, #43815 ) ) ;
#61276=B_SPLINE_CURVE_WITH_KNOTS ( 'NONE', 3,
 ( #40538, #55721, #92783, #23337 ),
 .UNSPECIFIED., .F., .F.,
 ( 4, 4 ),
 ( 0.04233433915237033024, 0.04887066958154941132 ),
 .UNSPECIFIED. ) ;
#61279=CARTESIAN_POINT ( 'NONE',  ( 164.3493441216711517, 245.9855811210807417, 1.722120810491653664 ) ) ;
#61280=CARTESIAN_POINT ( 'NONE',  ( 161.5504232052330167, 284.0438539892405743, 0.5273125768649428169 ) ) ;
#61281=CARTESIAN_POINT ( 'NONE',  ( 198.1297952544482541, 280.7479725296748825, 16.71566180775300481 ) ) ;
#61282=CARTESIAN_POINT ( 'NONE',  ( 147.4771028564622100, 275.6046161191591182, 9.141179566768406735E-14 ) ) ;
#61286=CARTESIAN_POINT ( 'NONE',  ( 185.3162954522941561, 260.2450069084709412, 6.201801027297742408 ) ) ;
#61288=CARTESIAN_POINT ( 'NONE',  ( 201.4066285247549786, 281.8004817444100354, -17.79749223817309201 ) ) ;
#61291=ORIENTED_EDGE ( 'NONE', *, *, #78890, .T. ) ;
#61292=CARTESIAN_POINT ( 'NONE',  ( 195.7397332151493003, 265.3334278097593710, 5.020291378112107239 ) ) ;
#61294=CARTESIAN_POINT ( 'NONE',  ( 87.73782093965644435, 209.9155109091896065, 2.679491924311254714 ) ) ;
#61298=CARTESIAN_POINT ( 'NONE',  ( 198.5033866919546881, 266.2084897167371196, 0.6426914612636319690 ) ) ;
#61299=ORIENTED_EDGE ( 'NONE', *, *, #14221, .F. ) ;
#61300=CARTESIAN_POINT ( 'NONE',  ( 147.4368675721658519, 275.2788497866417288, 5.050119523016719292 ) ) ;
#61301=CARTESIAN_POINT ( 'NONE',  ( 183.7271510445999070, 281.0151571664360404, 16.38277545986319694 ) ) ;
#61303=CARTESIAN_POINT ( 'NONE',  ( 206.9377610035629118, 272.2202792677204002, 7.440532334334675646 ) ) ;
#61304=CARTESIAN_POINT ( 'NONE',  ( 155.2419697281468416, 261.7600162942170527, 18.58580762350309357 ) ) ;
#61307=CARTESIAN_POINT ( 'NONE',  ( 19.85049821812286908, 192.2677522451419350, -5.000000000000047962 ) ) ;
#61308=CARTESIAN_POINT ( 'NONE',  ( 163.6469966371277849, 283.9424131525427697, -3.116750258215220448 ) ) ;
#61310=CARTESIAN_POINT ( 'NONE',  ( 198.2414483977475754, 287.2827345394944700, 16.94931984969033678 ) ) ;
#61311=CARTESIAN_POINT ( 'NONE',  ( 141.9600801517287323, 262.7677522451419350, -5.000000000000047962 ) ) ;
#61317=CARTESIAN_POINT ( 'NONE',  ( 17.27983239817682559, 168.5327760586659451, 1.948934522072302763E-15 ) ) ;
#61319=CARTESIAN_POINT ( 'NONE',  ( 178.5822171558442619, 273.7261340967344836, -16.93785058890262007 ) ) ;
#61321=CARTESIAN_POINT ( 'NONE',  ( 130.8844835975280887, 234.8262482093457493, 3.021315404115420679E-15 ) ) ;
#61322=CARTESIAN_POINT ( 'NONE',  ( 182.1439385020048860, 290.0253507885926183, 13.01467259685074573 ) ) ;
#61323=DIRECTION ( 'NONE',  ( 0.5000000000000048850, -0.8660254037844358210, 0.000000000000000000 ) ) ;
#61324=CARTESIAN_POINT ( 'NONE',  ( 187.4995632756286739, 259.3762926903145285, -0.7801709818681489272 ) ) ;
#61325=CARTESIAN_POINT ( 'NONE',  ( 183.1000404951680878, 295.7276604254721519, 1.087596103637166189 ) ) ;
#61326=CARTESIAN_POINT ( 'NONE',  ( 65.91222438545561602, 218.8615022471903160, 5.000000000000046185 ) ) ;
#61328=CARTESIAN_POINT ( 'NONE',  ( 148.2267527339363369, 273.9107285543102535, 7.913369084260907016 ) ) ;
#61330=CARTESIAN_POINT ( 'NONE',  ( 32.89474554257621719, 198.9869531367911293, 4.594050593750046652 ) ) ;
#61336=AXIS2_PLACEMENT_3D ( 'NONE', #6575, #83605, #58870 ) ;
#61337=CARTESIAN_POINT ( 'NONE',  ( 164.4440639631384045, 245.8215215431751233, -2.910115319305802029 ) ) ;
#61338=CARTESIAN_POINT ( 'NONE',  ( 188.8123461939931076, 268.1836859051376223, 13.59473602984847140 ) ) ;
#61339=CARTESIAN_POINT ( 'NONE',  ( 202.8965239598698247, 278.6747210883311823, -15.08919433053647374 ) ) ;
#61340=CARTESIAN_POINT ( 'NONE',  ( 161.2976129585435956, 280.2619845096857034, 9.013726905557600588 ) ) ;
#61343=CARTESIAN_POINT ( 'NONE',  ( 148.3707431749605234, 273.6613297946520902, 8.912574527564540716 ) ) ;
#61345=CARTESIAN_POINT ( 'NONE',  ( 155.2098048002210930, 261.8157275836062468, 16.98811268941991059 ) ) ;
#61350=B_SPLINE_CURVE_WITH_KNOTS ( 'NONE', 3,
 ( #41203, #56909, #72143, #64023, #1743, #26039, #63520, #64529, #2243, #79772, #94459, #33122, #15915, #9849, #95487, #46821, #77744, #70107, #716, #24016, #80780, #57409, #80269, #34616, #5221, #19934, #11838, #26536, #20431, #89380, #66515, #74645, #42697, #67002, #27537, #97440, #88390, #18944, #49822, #19457, #88895, #28010, #12331, #58406 ),
 .UNSPECIFIED., .F., .F.,
 ( 4, 2, 2, 2, 2, 2, 2, 2, 2, 2, 2, 2, 2, 2, 2, 2, 2, 2, 2, 2, 2, 4 ),
 ( 0.001113145019558975379, 0.001593043127414757280, 0.002072941235270539181, 0.002312890289198457454, 0.002552839343126374859, 0.002672813870090334429, 0.002792788397054293131, 0.002912762924018251834, 0.003032737450982210536, 0.003512635558838129047, 0.003992533666694047557, 0.004952329882406020754, 0.005912126098117993951, 0.006392024205973977947, 0.006871922313829961944, 0.006991896840793983096, 0.007051884104275961580, 0.007111871367757939197, 0.007351820421685926858, 0.007831718529541909987, 0.008311616637397895718, 0.008791514745253877980 ),
 .UNSPECIFIED. ) ;
#61352=CARTESIAN_POINT ( 'NONE',  ( 148.6890168490380688, 273.7113373112761678, -8.655580785000621447 ) ) ;
#61358=CARTESIAN_POINT ( 'NONE',  ( 181.2250113611592042, 257.6047676075520485, -7.592445647342843884 ) ) ;
#61362=CARTESIAN_POINT ( 'NONE',  ( 202.4568751826897426, 279.4272769738290094, 15.52666735877811455 ) ) ;
#61365=CARTESIAN_POINT ( 'NONE',  ( 151.4361976351029000, 268.3518069213970421, 15.15218985681980612 ) ) ;
#61366=DIRECTION ( 'NONE',  ( 0.4999999999999998890, -0.8660254037844385966, 0.000000000000000000 ) ) ;
#61369=CARTESIAN_POINT ( 'NONE',  ( 148.3707431749605234, 273.6613297946520902, 8.912574527564540716 ) ) ;
#61371=CARTESIAN_POINT ( 'NONE',  ( 176.0994133278866229, 271.7662213919938381, 17.81274505597714253 ) ) ;
#61372=VERTEX_POINT ( 'NONE', #26376 ) ;
#61375=ORIENTED_EDGE ( 'NONE', *, *, #5206, .T. ) ;
#61377=CARTESIAN_POINT ( 'NONE',  ( 166.7959447105422157, 276.3626885415273478, 15.91653206054683523 ) ) ;
#61379=ORIENTED_EDGE ( 'NONE', *, *, #46720, .T. ) ;
#61380=CARTESIAN_POINT ( 'NONE',  ( 172.4419760422836134, 290.9306500000749907, -0.6531725299933459628 ) ) ;
#61381=CARTESIAN_POINT ( 'NONE',  ( 150.6453220160077251, 269.7216436761371483, 14.94145576020818034 ) ) ;
#61386=CARTESIAN_POINT ( 'NONE',  ( 190.5586441464129450, 299.4817191808413668, 6.393230458720348786 ) ) ;
#61388=CARTESIAN_POINT ( 'NONE',  ( 148.3930300673291640, 273.6227277647267897, 8.375036249079425232 ) ) ;
#61389=CARTESIAN_POINT ( 'NONE',  ( 190.2318383114841254, 301.1557861577188078, 3.177919994438449525 ) ) ;
#61390=CARTESIAN_POINT ( 'NONE',  ( 141.3928138467258009, 240.8932355074535678, -2.679491924311248496 ) ) ;
#61391=EDGE_CURVE ( 'NONE', #18565, #21768, #4060, .T. ) ;
#61392=CARTESIAN_POINT ( 'NONE',  ( 191.6444038793167977, 298.7091508252102017, 8.370770059625519011 ) ) ;
#61394=CARTESIAN_POINT ( 'NONE',  ( 191.2211340522693774, 299.4422756709672626, -8.405362570633277741 ) ) ;
#61395=B_SPLINE_CURVE_WITH_KNOTS ( 'NONE', 3,
 ( #30561, #36650, #37640, #99476 ),
 .UNSPECIFIED., .F., .F.,
 ( 4, 4 ),
 ( 0.01120786676255014318, 0.01708091092720957077 ),
 .UNSPECIFIED. ) ;
#61396=CARTESIAN_POINT ( 'NONE',  ( 162.3596268837808907, 257.1951048930611705, 15.63890487423926601 ) ) ;
#61400=CARTESIAN_POINT ( 'NONE',  ( 169.8554095453154105, 287.3059200333181025, 4.097349522332975447 ) ) ;
#61403=CARTESIAN_POINT ( 'NONE',  ( 149.6625482771057420, 271.4238577242598467, -11.76596961571646460 ) ) ;
#61404=CARTESIAN_POINT ( 'NONE',  ( 81.75096066047075283, 229.5530062829863027, -4.648177544792955347E-16 ) ) ;
#61405=CARTESIAN_POINT ( 'NONE',  ( -27.42236680055714260, 166.5217562850347406, 1.224646799147364892E-15 ) ) ;
#61411=CARTESIAN_POINT ( 'NONE',  ( 208.3194307158603067, 269.8271571267425770, -2.120200867047394855 ) ) ;
#61412=( BOUNDED_CURVE ( )  B_SPLINE_CURVE ( 2, ( #8368, #262, #755, #32658, #46859, #31143, #71183, #31639, #85931 ),
 .UNSPECIFIED., .F., .T. ) 
 B_SPLINE_CURVE_WITH_KNOTS ( ( 3, 2, 2, 2, 3 ),
 ( 0.7540322580645161255, 0.7553763440860215006, 0.7580645161290322509, 0.7607526881720430012, 0.7620967741935483764 ),
 .UNSPECIFIED. ) 
 CURVE ( )  GEOMETRIC_REPRESENTATION_ITEM ( )  RATIONAL_B_SPLINE_CURVE ( ( 0.9330127018922194093, 0.9330127018922194093, 1.000000000000000000, 0.8660254037844387076, 1.000000000000000000, 0.8660254037844387076, 1.000000000000000000, 0.9330127018922194093, 0.9330127018922194093 ) ) 
 REPRESENTATION_ITEM ( '' )  );
#61414=CARTESIAN_POINT ( 'NONE',  ( 45.32607884611513072, 203.6427522451419065, 10.00000000000009237 ) ) ;
#61415=CARTESIAN_POINT ( 'NONE',  ( 125.3701074643745699, 249.3149278399160949, 9.188101187500093303 ) ) ;
#61416=CARTESIAN_POINT ( 'NONE',  ( 180.6483990817532685, 294.3080752668889772, -3.362655399551144786 ) ) ;
#61419=CARTESIAN_POINT ( 'NONE',  ( 196.0034224882197975, 291.1591091234520263, 17.53794140922627776 ) ) ;
#61420=CARTESIAN_POINT ( 'NONE',  ( 175.4077757953151604, 253.5139745403514553, -3.897595921025101884 ) ) ;
#61421=CARTESIAN_POINT ( 'NONE',  ( 45.45211389745056607, 206.2369531367911293, -4.594050593750048428 ) ) ;
#61426=CARTESIAN_POINT ( 'NONE',  ( 180.9399124977257145, 267.5927373598447048, 15.00208439449252751 ) ) ;
#61428=CARTESIAN_POINT ( 'NONE',  ( 162.8384627734353387, 250.8402808221231624, -13.07578932517241732 ) ) ;
#61432=CARTESIAN_POINT ( 'NONE',  ( 182.2055061536417497, 262.5723910214719581, 12.91931843363846966 ) ) ;
#61433=CARTESIAN_POINT ( 'NONE',  ( 101.6177300921036419, 236.1427522451419065, -10.00000000000009415 ) ) ;
#61434=B_SPLINE_SURFACE_WITH_KNOTS ( 'NONE', 3, 1, ( 
 ( #56630, #80987 ),
 ( #88597, #11052 ),
 ( #58125, #10044 ),
 ( #25227, #19160 ),
 ( #2968, #1941 ),
 ( #26242, #40907 ),
 ( #12044, #42897 ),
 ( #3455, #79975 ),
 ( #95695, #50034 ),
 ( #11553, #80481 ),
 ( #10544, #81470 ),
 ( #32827, #89106 ),
 ( #63735, #41418 ),
 ( #64745, #72865 ),
 ( #17643, #96173 ),
 ( #33861, #41929 ),
 ( #87613, #34334 ),
 ( #94670, #26734 ),
 ( #42412, #57116 ),
 ( #88099, #18141 ),
 ( #56114, #3933 ),
 ( #18648, #65230 ),
 ( #34816, #49528 ),
 ( #2452, #73346 ),
 ( #79480, #65717 ),
 ( #87105, #48541 ),
 ( #71855, #33334 ),
 ( #96673, #27241 ),
 ( #19656, #50518 ),
 ( #64231, #95181 ),
 ( #49041, #51017 ),
 ( #75847, #83459 ),
 ( #28222, #52511 ),
 ( #44412, #98650 ) ),
 .UNSPECIFIED., .T., .F., .F.,
 ( 4, 2, 2, 2, 2, 2, 2, 2, 2, 2, 2, 2, 2, 2, 2, 2, 4 ),
 ( 2, 2 ),
 ( 0.000000000000000000, 0.06250000000000000000, 0.1250000000000000000, 0.1875000000000000000, 0.2500000000000000000, 0.3125000000000000000, 0.3750000000000000000, 0.4375000000000000000, 0.5000000000000000000, 0.5625000000000000000, 0.6250000000000000000, 0.6875000000000000000, 0.7500000000000000000, 0.8125000000000000000, 0.8750000000000000000, 0.9375000000000000000, 1.000000000000000000 ),
 ( 0.000000000000000000, 1.000000000000000000 ),
 .UNSPECIFIED. ) ;
#61435=CARTESIAN_POINT ( 'NONE',  ( 198.2505066714982149, 285.2670451491296149, 0.000000000000000000 ) ) ;
#61437=CARTESIAN_POINT ( 'NONE',  ( 202.7599932440484451, 279.4563852894229967, 15.58249343055423353 ) ) ;
#61438=CARTESIAN_POINT ( 'NONE',  ( 208.3586375946586315, 269.7592488206576604, -1.970210487958146128 ) ) ;
#61441=CARTESIAN_POINT ( 'NONE',  ( 28.02335264628875677, 196.1744531367911293, 4.594050593750047540 ) ) ;
#61443=CARTESIAN_POINT ( 'NONE',  ( 192.4771936439569515, 272.0680645981377666, 14.18742438910983594 ) ) ;
#61444=CARTESIAN_POINT ( 'NONE',  ( 40.06784160394645511, 182.3932355074535394, -2.679491924311248496 ) ) ;
#61446=CARTESIAN_POINT ( 'NONE',  ( 198.1897299879200602, 277.3109323272205415, -15.34172296478933717 ) ) ;
#61447=CARTESIAN_POINT ( 'NONE',  ( 66.99449581658849695, 218.6744531367911293, 4.594050593750047540 ) ) ;
#61448=ADVANCED_FACE ( 'NONE', ( #68840 ), #44949, .F. ) ;
#61449=CARTESIAN_POINT ( 'NONE',  ( 200.2316334480823912, 283.8356329158505105, 17.02791935830326508 ) ) ;
#61454=CARTESIAN_POINT ( 'NONE',  ( 164.7681158011125717, 268.8552380765891030, 16.67724236807602267 ) ) ;
#61455=CARTESIAN_POINT ( 'NONE',  ( 14.81672556217377235, 179.3615022471902591, -10.00000000000009592 ) ) ;
#61456=CARTESIAN_POINT ( 'NONE',  ( 164.1821508476733698, 246.2751683663292397, -7.347745041495428175 ) ) ;
#61457=CARTESIAN_POINT ( 'NONE',  ( 144.4230134433972239, 248.0643266524160140, 9.188101187500095079 ) ) ;
#61459=CARTESIAN_POINT ( 'NONE',  ( 167.6696528517744014, 262.3690162733964826, -17.00514220863813364 ) ) ;
#61460=EDGE_CURVE ( 'NONE', #86782, #74702, #93123, .T. ) ;
#61461=CARTESIAN_POINT ( 'NONE',  ( 185.2747196154622316, 260.3698368134728867, 6.698900342170079902 ) ) ;
#61464=CARTESIAN_POINT ( 'NONE',  ( 185.1984267626157248, 277.5364252950313357, -17.64468014200656398 ) ) ;
#61467=CARTESIAN_POINT ( 'NONE',  ( 150.6790040019602088, 269.6633047651677089, 15.38315204620803378 ) ) ;
#61473=CARTESIAN_POINT ( 'NONE',  ( 206.7778081894269064, 272.4973256686178615, 7.979133442510888408 ) ) ;
#61476=ADVANCED_FACE ( 'NONE', ( #17143 ), #86117, .T. ) ;
#61477=CARTESIAN_POINT ( 'NONE',  ( 148.8985332352210946, 273.2084804242117571, -9.391003212318970839 ) ) ;
#61479=CARTESIAN_POINT ( 'NONE',  ( 149.6987302396718178, 272.4200664568434718, 11.31912059095424183 ) ) ;
#61480=CARTESIAN_POINT ( 'NONE',  ( 208.0421103033489771, 270.3074901711881353, -2.473242163239977476 ) ) ;
#61481=CARTESIAN_POINT ( 'NONE',  ( 153.0927037754837556, 265.4826541232073964, -16.15085267704102634 ) ) ;
#61482=ORIENTED_EDGE ( 'NONE', *, *, #79693, .T. ) ;
#61483=CARTESIAN_POINT ( 'NONE',  ( 191.4544176431711264, 281.2354317515596449, 16.67543541242699945 ) ) ;
#61486=CARTESIAN_POINT ( 'NONE',  ( 149.5593209768671841, 271.6026526530012575, 11.55487339793564949 ) ) ;
#61487=CARTESIAN_POINT ( 'NONE',  ( 15.15952728095722613, 172.8927522451418213, 10.00000000000009948 ) ) ;
#61493=CARTESIAN_POINT ( 'NONE',  ( 149.5796913320911870, 271.5673701627850960, -12.80793412251569841 ) ) ;
#61496=CARTESIAN_POINT ( 'NONE',  ( 101.2839494695023603, 229.2833772461660544, -9.188101187500095079 ) ) ;
#61497=CARTESIAN_POINT ( 'NONE',  ( 155.6860346224306682, 260.9908733354596961, 18.34621944435518870 ) ) ;
#61498=B_SPLINE_CURVE_WITH_KNOTS ( 'NONE', 3,
 ( #6927, #47419, #85479, #46411 ),
 .UNSPECIFIED., .F., .F.,
 ( 4, 4 ),
 ( 0.003806595552051763101, 0.007765155676520470000 ),
 .UNSPECIFIED. ) ;
#61499=CARTESIAN_POINT ( 'NONE',  ( 151.0099717111976076, 269.0900518771037468, 15.84752309685681659 ) ) ;
#61500=CARTESIAN_POINT ( 'NONE',  ( 139.8671854259164320, 244.8927522451418497, 10.00000000000009948 ) ) ;
#61502=EDGE_CURVE ( 'NONE', #41184, #61039, #87062, .T. ) ;
#61503=ORIENTED_EDGE ( 'NONE', *, *, #27895, .T. ) ;
#61504=ORIENTED_EDGE ( 'NONE', *, *, #86975, .F. ) ;
#61507=CARTESIAN_POINT ( 'NONE',  ( 192.5672132233574700, 296.7161803602032819, 11.26440590052197521 ) ) ;
#61508=CIRCLE ( 'NONE', #17855, 17.82106496071138935 ) ;
#61509=ORIENTED_EDGE ( 'NONE', *, *, #56009, .T. ) ;
#61510=EDGE_CURVE ( 'NONE', #15709, #24115, #26231, .T. ) ;
#61511=CARTESIAN_POINT ( 'NONE',  ( 163.7038023771459052, 247.1036922210055025, -6.448491958542482472 ) ) ;
#61513=CARTESIAN_POINT ( 'NONE',  ( 171.0838469510729283, 283.5197208256832937, 12.13844873189909457 ) ) ;
#61514=CARTESIAN_POINT ( 'NONE',  ( 148.3625667886952044, 273.6754917110858401, -8.960758510948144462 ) ) ;
#61515=EDGE_CURVE ( 'NONE', #47543, #77760, #30299, .T. ) ;
#61520=CARTESIAN_POINT ( 'NONE',  ( 199.3479728691114587, 277.9353724323879078, -15.41277036647585597 ) ) ;
#61523=ORIENTED_EDGE ( 'NONE', *, *, #37929, .T. ) ;
#61525=APPLICATION_CONTEXT ( 'automotive_design' ) ;
#61526=CARTESIAN_POINT ( 'NONE',  ( 202.4017613376760494, 280.0768611521521620, 15.73960524502980540 ) ) ;
#61528=CARTESIAN_POINT ( 'NONE',  ( 188.1240574672448247, 260.7517132086819629, 2.838756651779489104 ) ) ;
#61531=CARTESIAN_POINT ( 'NONE',  ( 200.5438717407500917, 283.2948203288816558, 18.39667691545567152 ) ) ;
#61532=CARTESIAN_POINT ( 'NONE',  ( 157.9492502841812893, 281.0771850073649034, 1.816109525321617291 ) ) ;
#61534=CARTESIAN_POINT ( 'NONE',  ( 155.4220579613188704, 261.4480943245178537, -17.00714975260428474 ) ) ;
#61536=FACE_OUTER_BOUND ( 'NONE', #89121, .T. ) ;
#61537=CARTESIAN_POINT ( 'NONE',  ( 8.086986483384336566, 162.1427522451417644, 1.119607411625061291E-15 ) ) ;
#61538=CARTESIAN_POINT ( 'NONE',  ( 193.2604171883379536, 267.6068621284443907, -10.96396649826040282 ) ) ;
#61540=CARTESIAN_POINT ( 'NONE',  ( 204.2359371119229650, 276.8999755211443130, -15.33127121419060401 ) ) ;
#61541=CARTESIAN_POINT ( 'NONE',  ( 161.5226180746127227, 251.2552919257010728, -12.89472374756154949 ) ) ;
#61542=CARTESIAN_POINT ( 'NONE',  ( -6.860972828079417773, 166.8458772461660544, 9.188101187500095079 ) ) ;
#61544=CARTESIAN_POINT ( 'NONE',  ( 58.25224935450648189, 215.9860189848785694, -2.679491924311252493 ) ) ;
#61550=PLANE ( 'NONE',  #47861 ) ;
#61552=CARTESIAN_POINT ( 'NONE',  ( 149.9586195398654525, 276.8495302347727147, 3.185754299552747248 ) ) ;
#61553=CARTESIAN_POINT ( 'NONE',  ( 29.48529115882250551, 178.6423013555409796, -4.594050593750043987 ) ) ;
#61554=CARTESIAN_POINT ( 'NONE',  ( 124.8563387505838165, 233.7048013555409796, 4.594050593750051981 ) ) ;
#61556=CARTESIAN_POINT ( 'NONE',  ( -17.42236680055705023, 149.2012482093457777, 0.000000000000000000 ) ) ;
#61557=CARTESIAN_POINT ( 'NONE',  ( 33.07542782529571923, 183.2365022471901739, -10.00000000000009237 ) ) ;
#61558=CARTESIAN_POINT ( 'NONE',  ( 178.4974649003195850, 283.7799215797293755, -14.74701626068640259 ) ) ;
#61561=CARTESIAN_POINT ( 'NONE',  ( 155.6276701977099890, 261.0919634844306643, 17.49722577287685255 ) ) ;
#61562=CARTESIAN_POINT ( 'NONE',  ( 161.1150691641480535, 251.5875096731584506, -13.48836942566120101 ) ) ;
#61564=CARTESIAN_POINT ( 'NONE',  ( 193.1995342044276640, 264.0813980297376133, 7.606167026564889966 ) ) ;
#61565=CARTESIAN_POINT ( 'NONE',  ( 171.5385771854158179, 279.8808931372358302, 13.92051632058779198 ) ) ;
#61566=CARTESIAN_POINT ( 'NONE',  ( 204.0884846259506276, 275.1553707185394728, 13.46337290381501717 ) ) ;
#61568=CARTESIAN_POINT ( 'NONE',  ( 147.7870527676176948, 274.6723112360602386, 9.257357958194809555 ) ) ;
#61569=CARTESIAN_POINT ( 'NONE',  ( 180.9828039363494554, 267.0267840551962877, -14.76148221183092524 ) ) ;
#61570=ORIENTED_EDGE ( 'NONE', *, *, #61826, .T. ) ;
#61571=CARTESIAN_POINT ( 'NONE',  ( 152.5396176296194710, 266.8690347833386909, -15.56576981617802424 ) ) ;
#61572=CARTESIAN_POINT ( 'NONE',  ( 184.6479839499307332, 269.5423948272451753, 15.39131224564481037 ) ) ;
#61573=CARTESIAN_POINT ( 'NONE',  ( 90.37718171876834106, 232.1744531367911293, 4.594050593750047540 ) ) ;
#61578=DIRECTION ( 'NONE',  ( -0.8660254037844387076, -0.4999999999999998890, -0.000000000000000000 ) ) ;
#61579=CARTESIAN_POINT ( 'NONE',  ( 191.6023198849542837, 276.9562025558888081, 16.79891912045939151 ) ) ;
#61580=CARTESIAN_POINT ( 'NONE',  ( 149.5130609720542623, 271.6827773316956609, 13.04552708959771934 ) ) ;
#61581=DIRECTION ( 'NONE',  ( -0.8660254037844387076, -0.4999999999999998890, -0.000000000000000000 ) ) ;
#61583=CARTESIAN_POINT ( 'NONE',  ( 55.59208832369112230, 196.2365022471902307, 10.00000000000009948 ) ) ;
#61588=CARTESIAN_POINT ( 'NONE',  ( 177.9874092160698069, 279.9792724555832706, 15.65335057370039884 ) ) ;
#61589=CARTESIAN_POINT ( 'NONE',  ( 199.9859019575963259, 270.1052791603114542, 9.171208846631140332 ) ) ;
#61590=CARTESIAN_POINT ( 'NONE',  ( 149.3629284598386278, 271.9428144707212027, -12.99253781774931049 ) ) ;
#61592=ORIENTED_EDGE ( 'NONE', *, *, #41565, .T. ) ;
#61596=CARTESIAN_POINT ( 'NONE',  ( 180.4572463832561482, 261.7460625851787199, -13.63662180976220384 ) ) ;
#61597=CARTESIAN_POINT ( 'NONE',  ( 169.7161983584676932, 251.3797710867630713, -8.400916520806605448 ) ) ;
#61598=CARTESIAN_POINT ( 'NONE',  ( 152.6656396574222754, 266.2223508737794759, 17.04346597795114349 ) ) ;
#61604=CARTESIAN_POINT ( 'NONE',  ( 169.0079941869541074, 269.5332732215450733, -17.80121103236473346 ) ) ;
#61605=ORIENTED_EDGE ( 'NONE', *, *, #72309, .T. ) ;
#61607=CARTESIAN_POINT ( 'NONE',  ( 158.8194364388402562, 255.9479314064563766, 16.03906445419635673 ) ) ;
#61609=CARTESIAN_POINT ( 'NONE',  ( 192.8739241956344017, 296.5795591684099577, -13.56467825654580928 ) ) ;
#61610=CARTESIAN_POINT ( 'NONE',  ( 201.2139346379346705, 282.1342373466909521, -16.65315141107179286 ) ) ;
#61614=CARTESIAN_POINT ( 'NONE',  ( 148.6023484834014425, 275.2601776331305814, 7.517535991345212665 ) ) ;
#61615=ORIENTED_EDGE ( 'NONE', *, *, #44813, .F. ) ;
#61616=CARTESIAN_POINT ( 'NONE',  ( 176.3865323452404823, 258.8737835494043225, 13.24306684835586623 ) ) ;
#61618=VERTEX_POINT ( 'NONE', #58140 ) ;
#61619=CARTESIAN_POINT ( 'NONE',  ( 172.8702133838303041, 271.0664845223420230, 16.42754727834196160 ) ) ;
#61620=VERTEX_POINT ( 'NONE', #42913 ) ;
#61622=CARTESIAN_POINT ( 'NONE',  ( 172.6025460550783919, 256.6729997644848140, -11.64617786982520897 ) ) ;
#61624=CARTESIAN_POINT ( 'NONE',  ( 175.3932935011599170, 269.2958584618301643, -17.65833184418574930 ) ) ;
#61625=CARTESIAN_POINT ( 'NONE',  ( 201.2723982155681028, 274.9066758845833647, -14.03142259981584772 ) ) ;
#61626=CARTESIAN_POINT ( 'NONE',  ( 160.1795347027651815, 282.8633239002924711, 5.491715875156680582 ) ) ;
#61628=CARTESIAN_POINT ( 'NONE',  ( 184.5123196318015459, 277.1383014161853566, -17.82024832176989904 ) ) ;
#61631=CARTESIAN_POINT ( 'NONE',  ( 178.0470025766832123, 255.4632854186900772, 5.005086694065276731 ) ) ;
#61633=CARTESIAN_POINT ( 'NONE',  ( 114.9778026189612632, 243.3149278399160664, 9.188101187500093303 ) ) ;
#61635=CARTESIAN_POINT ( 'NONE',  ( 161.3088938790619409, 283.6794878094777914, 2.159307202287777727 ) ) ;
#61636=CARTESIAN_POINT ( 'NONE',  ( 188.0760642469317645, 273.6708693882125090, 17.00871842608619033 ) ) ;
#61638=EDGE_CURVE ( 'NONE', #64789, #82018, #48111, .T. ) ;
#61639=CARTESIAN_POINT ( 'NONE',  ( 164.1654149204426858, 248.3041558426086226, -9.671695341034215687 ) ) ;
#61640=ADVANCED_FACE ( 'NONE', ( #89120 ), #95709, .T. ) ;
#61642=EDGE_CURVE ( 'NONE', #7878, #74497, #15851, .T. ) ;
#61644=CARTESIAN_POINT ( 'NONE',  ( 157.3363371328520088, 258.1324655395517311, 18.24585617226787093 ) ) ;
#61649=CARTESIAN_POINT ( 'NONE',  ( 147.9745743502305118, 274.3475143274592938, 10.02752110366533778 ) ) ;
#61651=ORIENTED_EDGE ( 'NONE', *, *, #48180, .T. ) ;
#61652=CARTESIAN_POINT ( 'NONE',  ( 148.1974503712686158, 273.9614817352322120, -7.884397846570731616 ) ) ;
#61653=CARTESIAN_POINT ( 'NONE',  ( 39.26390101962405055, 200.1427522451419350, -10.00000000000009592 ) ) ;
#61655=CARTESIAN_POINT ( 'NONE',  ( 188.0293636999220723, 266.1540144583576648, -11.80271381409143672 ) ) ;
#61656=CARTESIAN_POINT ( 'NONE',  ( 159.9714013527444649, 278.6080261497965580, 10.43375755400861848 ) ) ;
#61657=CARTESIAN_POINT ( 'NONE',  ( 176.0575385324409865, 258.1988160713917182, -12.86591411535773233 ) ) ;
#61658=CARTESIAN_POINT ( 'NONE',  ( 157.7045215221510830, 262.9535044009366516, 17.16314129935500077 ) ) ;
#61660=CARTESIAN_POINT ( 'NONE',  ( 184.7099738404339178, 289.1045521149691808, -13.19732552672321368 ) ) ;
#61662=CARTESIAN_POINT ( 'NONE',  ( 158.1690553627090310, 281.8858333404083965, -5.006681078564091614 ) ) ;
#61664=CARTESIAN_POINT ( 'NONE',  ( 205.2564848266901834, 271.9733254596621350, -9.597888780111448526 ) ) ;
#61666=CARTESIAN_POINT ( 'NONE',  ( 163.6101490995871472, 247.6943118105651536, -7.655108696039592431 ) ) ;
#61668=CARTESIAN_POINT ( 'NONE',  ( 192.5677150043008794, 271.3893586466145962, -15.08671890483280009 ) ) ;
#61669=CARTESIAN_POINT ( 'NONE',  ( 188.3311882918543745, 299.0666206182007159, -3.691789600375173563 ) ) ;
#61674=CARTESIAN_POINT ( 'NONE',  ( 66.66973629016931113, 218.4869531367911293, 4.594050593750046652 ) ) ;
#61676=CARTESIAN_POINT ( 'NONE',  ( 147.3715240516018810, 275.3920280842035595, -3.728968767617475866 ) ) ;
#61677=CARTESIAN_POINT ( 'NONE',  ( 208.2912792141756029, 269.8759169579697641, -2.198672330625011995 ) ) ;
#61678=ADVANCED_FACE ( 'NONE', ( #87126 ), #79497, .T. ) ;
#61679=CARTESIAN_POINT ( 'NONE',  ( 154.8833801513861772, 262.3811116602312268, -17.49275566389638215 ) ) ;
#61680=CARTESIAN_POINT ( 'NONE',  ( 161.8839333999304415, 250.2557977526613229, -13.90128376743482441 ) ) ;
#61681=FACE_OUTER_BOUND ( 'NONE', #91803, .T. ) ;
#61685=CARTESIAN_POINT ( 'NONE',  ( 169.1862348568044752, 252.0532904165472701, -8.781961744297172245 ) ) ;
#61686=CARTESIAN_POINT ( 'NONE',  ( 205.4186965677407954, 274.8513760505354639, -12.35476167499131783 ) ) ;
#61687=CARTESIAN_POINT ( 'NONE',  ( 195.7617614321055157, 291.5776783508526364, 16.33009124109666033 ) ) ;
#61688=( BOUNDED_CURVE ( )  B_SPLINE_CURVE ( 2, ( #49539, #11065, #72876, #34345, #96186, #26745, #19173, #50046, #80999 ),
 .UNSPECIFIED., .F., .T. ) 
 B_SPLINE_CURVE_WITH_KNOTS ( ( 3, 2, 2, 2, 3 ),
 ( 0.7459677419354838745, 0.7473118279569892497, 0.7500000000000000000, 0.7526881720430107503, 0.7540322580645161255 ),
 .UNSPECIFIED. ) 
 CURVE ( )  GEOMETRIC_REPRESENTATION_ITEM ( )  RATIONAL_B_SPLINE_CURVE ( ( 0.9330127018922194093, 0.9330127018922194093, 1.000000000000000000, 0.8660254037844387076, 1.000000000000000000, 0.8660254037844387076, 1.000000000000000000, 0.9330127018922194093, 0.9330127018922194093 ) ) 
 REPRESENTATION_ITEM ( '' )  );
#61689=CARTESIAN_POINT ( 'NONE',  ( 24.36989474801440636, 191.0024278399160949, 9.188101187500095079 ) ) ;
#61690=CARTESIAN_POINT ( 'NONE',  ( 50.97302584657637681, 209.4244531367911577, -4.594050593750046652 ) ) ;
#61691=CARTESIAN_POINT ( 'NONE',  ( 163.9845428888737047, 247.2485266795014240, -6.654263628452329549 ) ) ;
#61693=ADVANCED_FACE ( 'NONE', ( #56645 ), #57634, .T. ) ;
#61695=CARTESIAN_POINT ( 'NONE',  ( -4.668846022976054222, 158.1115022471902023, -5.000000000000041744 ) ) ;
#61696=CARTESIAN_POINT ( 'NONE',  ( -22.42236680055709641, 157.8615022471902591, 0.000000000000000000 ) ) ;
#61697=CARTESIAN_POINT ( 'NONE',  ( 200.1825662459639261, 270.8510622867177631, -11.52056956463778548 ) ) ;
#61699=CARTESIAN_POINT ( 'NONE',  ( -5.101858724868275630, 157.8615022471902023, 5.000000000000051514 ) ) ;
#61700=CARTESIAN_POINT ( 'NONE',  ( 197.0226655822963551, 289.3937282992477549, -17.28982543158101493 ) ) ;
#61702=CARTESIAN_POINT ( 'NONE',  ( 54.73473692032376903, 214.6589784336661637, -6.496448406907676862E-16 ) ) ;
#61703=CARTESIAN_POINT ( 'NONE',  ( 158.6690659153649676, 256.5285302911307781, -16.39959907094835856 ) ) ;
#61704=CARTESIAN_POINT ( 'NONE',  ( 175.0401671226080680, 292.0372585584420904, 2.009743414037639120 ) ) ;
#61705=CARTESIAN_POINT ( 'NONE',  ( 159.8416255366773839, 253.7931787365127434, 16.77980437810719394 ) ) ;
#61706=CARTESIAN_POINT ( 'NONE',  ( 50.52223126882174142, 206.6427522451419065, 10.00000000000009415 ) ) ;
#61707=CARTESIAN_POINT ( 'NONE',  ( 153.4268044563982301, 264.9039747690200670, 17.87503003910495636 ) ) ;
#61709=B_SPLINE_CURVE_WITH_KNOTS ( 'NONE', 3,
 ( #30171, #84411, #90537, #14959, #21109, #45847, #13012, #76770, #43871, #7363, #100093, #13502, #51987, #30679 ),
 .UNSPECIFIED., .F., .F.,
 ( 4, 2, 2, 2, 2, 2, 4 ),
 ( 0.001101397475338417335, 0.001342408758887880284, 0.001583420042437343233, 0.001824431325986806181, 0.002065442609536269347, 0.002547465176635195245, 0.003029487743734121143 ),
 .UNSPECIFIED. ) ;
#61710=( BOUNDED_CURVE ( )  B_SPLINE_CURVE ( 2, ( #45073, #98808, #60750, #28376, #99298, #50673, #81626, #12199, #75001 ),
 .UNSPECIFIED., .F., .T. ) 
 B_SPLINE_CURVE_WITH_KNOTS ( ( 3, 2, 2, 2, 3 ),
 ( 0.7943548387096773800, 0.7956989247311827551, 0.7983870967741935054, 0.8010752688172042557, 0.8024193548387096309 ),
 .UNSPECIFIED. ) 
 CURVE ( )  GEOMETRIC_REPRESENTATION_ITEM ( )  RATIONAL_B_SPLINE_CURVE ( ( 0.9330127018922194093, 0.9330127018922194093, 1.000000000000000000, 0.8660254037844387076, 1.000000000000000000, 0.8660254037844387076, 1.000000000000000000, 0.9330127018922194093, 0.9330127018922194093 ) ) 
 REPRESENTATION_ITEM ( '' )  );
#61712=VECTOR ( 'NONE', #9155, 1000.000000000000000 ) ;
#61714=CARTESIAN_POINT ( 'NONE',  ( 111.8115707860309556, 225.3615022471902023, 5.000000000000051514 ) ) ;
#61715=CARTESIAN_POINT ( 'NONE',  ( 198.1847055346428590, 286.9842163890704683, 16.95145238430053070 ) ) ;
#61716=CARTESIAN_POINT ( 'NONE',  ( 164.9836323268835940, 244.8869617230113249, -2.696511969808454534 ) ) ;
#61719=DIRECTION ( 'NONE',  ( 0.4999999999999992784, -0.8660254037844390407, 0.000000000000000000 ) ) ;
#61720=ORIENTED_EDGE ( 'NONE', *, *, #8345, .T. ) ;
#61721=CARTESIAN_POINT ( 'NONE',  ( 160.0061168334508750, 253.5082714530983026, -16.02306982074888708 ) ) ;
#61722=CARTESIAN_POINT ( 'NONE',  ( 186.8219716465515603, 276.5816512141889802, -17.20317318536942963 ) ) ;
#61725=ORIENTED_EDGE ( 'NONE', *, *, #13960, .F. ) ;
#61727=CARTESIAN_POINT ( 'NONE',  ( 194.2389208611690492, 294.2153155915419802, -15.75132567904764791 ) ) ;
#61729=VERTEX_POINT ( 'NONE', #19178 ) ;
#61734=B_SPLINE_CURVE_WITH_KNOTS ( 'NONE', 3,
 ( #82480, #67212, #97647, #82959 ),
 .UNSPECIFIED., .F., .F.,
 ( 4, 4 ),
 ( 0.02668887203020185034, 0.03591784413385134406 ),
 .UNSPECIFIED. ) ;
#61735=VERTEX_POINT ( 'NONE', #42427 ) ;
#61743=CARTESIAN_POINT ( 'NONE',  ( 207.6050568035884680, 271.0644890383991310, -1.456818755242089702 ) ) ;
#61744=CARTESIAN_POINT ( 'NONE',  ( 204.2556901454867955, 276.8657622634082713, 13.61111001399713949 ) ) ;
#61745=CARTESIAN_POINT ( 'NONE',  ( 159.9628729326222754, 253.5831720864507588, 15.75051413866357386 ) ) ;
#61746=CARTESIAN_POINT ( 'NONE',  ( 164.3451451116536077, 265.7028218483132491, -17.76432900134729564 ) ) ;
#61747=CARTESIAN_POINT ( 'NONE',  ( 142.8531688511554307, 253.2833772461660544, -9.188101187500095079 ) ) ;
#61748=CARTESIAN_POINT ( 'NONE',  ( 177.2332613454938723, 269.3467744458365587, 16.08370027918090628 ) ) ;
#61749=CARTESIAN_POINT ( 'NONE',  ( 178.7347573768907125, 257.9333752825167494, 9.867161600535267141 ) ) ;
#61750=CARTESIAN_POINT ( 'NONE',  ( 73.40858323730823543, 219.3149278399160664, 9.188101187500093303 ) ) ;
#61751=ORIENTED_EDGE ( 'NONE', *, *, #21436, .F. ) ;
#61752=CARTESIAN_POINT ( 'NONE',  ( 151.2057546125658973, 268.7509459446807227, 15.78031848731319187 ) ) ;
#61756=CARTESIAN_POINT ( 'NONE',  ( 195.9908276381054009, 291.1809240437640369, -15.88407441854119995 ) ) ;
#61761=CARTESIAN_POINT ( 'NONE',  ( 197.6456421031980994, 287.3858497455466932, 17.15283754821559015 ) ) ;
#61763=B_SPLINE_SURFACE_WITH_KNOTS ( 'NONE', 3, 1, ( 
 ( #87423, #62006 ),
 ( #70626, #54923 ),
 ( #94468, #41214 ),
 ( #8335, #25021 ),
 ( #79782, #86390 ),
 ( #78748, #9336 ),
 ( #17431, #46830 ),
 ( #78247, #23510 ),
 ( #85901, #86896 ),
 ( #71154, #233 ),
 ( #17951, #92957 ),
 ( #48339, #32631 ),
 ( #725, #39696 ),
 ( #15924, #8827 ),
 ( #79285, #9858 ),
 ( #62505, #1236 ),
 ( #52675, #80280 ),
 ( #14198, #29399 ),
 ( #72667, #83636 ),
 ( #97453, #96979 ),
 ( #65037, #27548 ),
 ( #18955, #66526 ),
 ( #50818, #43207 ),
 ( #42707, #73156 ),
 ( #64539, #49832 ),
 ( #88399, #95984 ),
 ( #58415, #33650 ),
 ( #57419, #80790 ),
 ( #95498, #72154 ),
 ( #10846, #26048 ),
 ( #11366, #12341 ),
 ( #3261, #42219 ),
 ( #74150, #65526 ),
 ( #88905, #19467 ) ),
 .UNSPECIFIED., .T., .F., .F.,
 ( 4, 2, 2, 2, 2, 2, 2, 2, 2, 2, 2, 2, 2, 2, 2, 2, 4 ),
 ( 2, 2 ),
 ( 0.000000000000000000, 0.06250000000000000000, 0.1250000000000000000, 0.1875000000000000000, 0.2500000000000000000, 0.3125000000000000000, 0.3750000000000000000, 0.4375000000000000000, 0.5000000000000000000, 0.5625000000000000000, 0.6250000000000000000, 0.6875000000000000000, 0.7500000000000000000, 0.8125000000000000000, 0.8750000000000000000, 0.9375000000000000000, 1.000000000000000000 ),
 ( 0.000000000000000000, 1.000000000000000000 ),
 .UNSPECIFIED. ) ;
#61765=CARTESIAN_POINT ( 'NONE',  ( 155.2695601165254402, 261.7122283397445131, 16.98599069618989077 ) ) ;
#61767=CARTESIAN_POINT ( 'NONE',  ( 70.64795371486285092, 223.8464784336661637, 1.353441290958777327E-15 ) ) ;
#61769=ORIENTED_EDGE ( 'NONE', *, *, #84009, .T. ) ;
#61771=CARTESIAN_POINT ( 'NONE',  ( 161.3988253665112609, 251.0960295137030300, -12.85133671850337223 ) ) ;
#61774=B_SPLINE_CURVE_WITH_KNOTS ( 'NONE', 3,
 ( #46978, #77897, #39846, #1393 ),
 .UNSPECIFIED., .F., .F.,
 ( 4, 4 ),
 ( 0.004106122421884165000, 0.008436222502574928020 ),
 .UNSPECIFIED. ) ;
#61776=EDGE_CURVE ( 'NONE', #76998, #83448, #35144, .T. ) ;
#61777=CARTESIAN_POINT ( 'NONE',  ( 187.7317787694285869, 273.6764366694279147, -17.17214744287320372 ) ) ;
#61778=CARTESIAN_POINT ( 'NONE',  ( 181.4204268205617154, 259.5203828285251006, -11.17471347674236348 ) ) ;
#61783=CARTESIAN_POINT ( 'NONE',  ( 147.9810571718830658, 275.4328967230283070, -5.053263300117055934 ) ) ;
#61784=CARTESIAN_POINT ( 'NONE',  ( 200.9812045408918380, 282.5373376992193926, -16.61165062382494284 ) ) ;
#61788=CARTESIAN_POINT ( 'NONE',  ( 195.9804492347847997, 265.5343886315737905, 4.427495290768495018 ) ) ;
#61790=CARTESIAN_POINT ( 'NONE',  ( 2.672015980952107572, 183.8967562850347122, -4.648177544792955347E-16 ) ) ;
#61795=CARTESIAN_POINT ( 'NONE',  ( 167.4391039490435844, 267.1861514467046845, 17.82254523450562900 ) ) ;
#61796=CARTESIAN_POINT ( 'NONE',  ( 202.3139361598622372, 280.2289788223093865, 15.93832709035092421 ) ) ;
#61797=CARTESIAN_POINT ( 'NONE',  ( 161.2535912560966551, 263.0844709175967182, -17.80682751047658030 ) ) ;
#61798=CARTESIAN_POINT ( 'NONE',  ( 194.5051734451974426, 293.7541525883582381, 14.61790433731063921 ) ) ;
#61801=CARTESIAN_POINT ( 'NONE',  ( 28.21411888609903684, 175.5494855054051584, -2.679491924311248496 ) ) ;
#61802=CARTESIAN_POINT ( 'NONE',  ( 166.5910668850809486, 286.3200580136348208, -3.227223869863532713 ) ) ;
#61804=DIRECTION ( 'NONE',  ( 0.4999999999999998890, -0.8660254037844385966, 0.000000000000000000 ) ) ;
#61805=CARTESIAN_POINT ( 'NONE',  ( 152.3523849971420532, 248.7677522451417929, -5.000000000000041744 ) ) ;
#61806=CARTESIAN_POINT ( 'NONE',  ( 150.5287101026835330, 271.9236214347867531, -12.89083132144543775 ) ) ;
#61811=CARTESIAN_POINT ( 'NONE',  ( 23.96437920969670898, 175.4548013555409796, -4.594050593750042211 ) ) ;
#61817=CARTESIAN_POINT ( 'NONE',  ( 188.6570295601639771, 259.3016035056324426, -0.8096508949806298094 ) ) ;
#61818=EDGE_CURVE ( 'NONE', #33225, #37254, #12190, .T. ) ;
#61820=CARTESIAN_POINT ( 'NONE',  ( 64.25234236153544032, 221.2365022471903444, 2.944929066748280225E-16 ) ) ;
#61822=DIRECTION ( 'NONE',  ( -0.8660254037844387076, -0.4999999999999998890, -0.000000000000000000 ) ) ;
#61824=CARTESIAN_POINT ( 'NONE',  ( 31.35205101814392847, 201.1589784336661353, -6.496448406907675876E-16 ) ) ;
#61826=EDGE_CURVE ( 'NONE', #57520, #46269, #99318, .T. ) ;
#61828=CARTESIAN_POINT ( 'NONE',  ( 206.2026304802515142, 271.4126985892297057, -6.607972036968888574 ) ) ;
#61830=CARTESIAN_POINT ( 'NONE',  ( 206.9942764641839688, 270.1223916185117560, -3.431663675821580828 ) ) ;
#61831=FACE_OUTER_BOUND ( 'NONE', #44847, .T. ) ;
#61832=CARTESIAN_POINT ( 'NONE',  ( 194.1493756275458793, 294.3704124857528655, 13.94613522129020744 ) ) ;
#61834=CARTESIAN_POINT ( 'NONE',  ( 202.5562236059581664, 279.2319112406736963, -15.43681043966012290 ) ) ;
#61836=CARTESIAN_POINT ( 'NONE',  ( 200.1133476818314705, 272.1141633677412415, 12.87458617912082914 ) ) ;
#61838=CARTESIAN_POINT ( 'NONE',  ( 189.8314329296643450, 301.8493086226544619, -0.8085564604676659384 ) ) ;
#61840=CARTESIAN_POINT ( 'NONE',  ( 187.3962380822248406, 269.0893220905305157, -14.11458629364903672 ) ) ;
#61841=ORIENTED_EDGE ( 'NONE', *, *, #46025, .F. ) ;
#61844=CARTESIAN_POINT ( 'NONE',  ( 193.6564271169084464, 262.6014873983580742, -4.146719891036213745 ) ) ;
#61846=ORIENTED_EDGE ( 'NONE', *, *, #75091, .T. ) ;
#61847=CARTESIAN_POINT ( 'NONE',  ( 161.8882824960653579, 250.2482648971885340, -13.83574485983625557 ) ) ;
#61850=CARTESIAN_POINT ( 'NONE',  ( 181.1761209317502335, 257.6610458391679117, -7.556567974831167156 ) ) ;
#61851=ORIENTED_EDGE ( 'NONE', *, *, #38899, .F. ) ;
#61853=CYLINDRICAL_SURFACE ( 'NONE', #38938, 17.82106496071139645 ) ;
#61856=CARTESIAN_POINT ( 'NONE',  ( 201.2949053258274148, 281.9939920013367782, -18.04004790210578335 ) ) ;
#61861=CARTESIAN_POINT ( 'NONE',  ( 148.4049257185216106, 273.6021238924720365, 8.639190357831699529 ) ) ;
#61864=CARTESIAN_POINT ( 'NONE',  ( 161.9954662403825978, 266.8975016676487826, 16.59001395411891266 ) ) ;
#61867=CARTESIAN_POINT ( 'NONE',  ( 190.6094661480870798, 300.5017155583701083, 4.598210453186021951 ) ) ;
#61869=ORIENTED_EDGE ( 'NONE', *, *, #76233, .T. ) ;
#61871=CARTESIAN_POINT ( 'NONE',  ( 150.6533415055477008, 269.7077535128032082, 14.84621632544246062 ) ) ;
#61875=ORIENTED_EDGE ( 'NONE', *, *, #3648, .F. ) ;
#61876=FACE_OUTER_BOUND ( 'NONE', #13361, .T. ) ;
#61879=CARTESIAN_POINT ( 'NONE',  ( 190.0550686570564949, 301.4619601804237732, 4.203010638620038542 ) ) ;
#61880=CARTESIAN_POINT ( 'NONE',  ( 173.9176872785688204, 276.9430746053678263, -15.64548591645994335 ) ) ;
#61881=CARTESIAN_POINT ( 'NONE',  ( 146.5457113009716466, 276.8223777258335758, 0.3536082318825463644 ) ) ;
#61882=CARTESIAN_POINT ( 'NONE',  ( 147.0314375879888757, 275.9810751181479986, -5.168577011192616588 ) ) ;
#61884=CARTESIAN_POINT ( 'NONE',  ( 163.4732498979778086, 257.8043807661392179, 15.53864332294564043 ) ) ;
#61886=AXIS2_PLACEMENT_3D ( 'NONE', #80849, #73207, #41271 ) ;
#61889=CARTESIAN_POINT ( 'NONE',  ( 91.45997379709659469, 223.6115022471902307, 10.00000000000009592 ) ) ;
#61893=CARTESIAN_POINT ( 'NONE',  ( 103.8820256808556906, 230.7833772461660544, -9.188101187500095079 ) ) ;
#61895=CARTESIAN_POINT ( 'NONE',  ( 147.0721334091522294, 275.9105878882373304, 0.7242168585908188572 ) ) ;
#61899=CARTESIAN_POINT ( 'NONE',  ( 154.8545429534089237, 262.4310591522755089, -17.81746354318405778 ) ) ;
#61900=CARTESIAN_POINT ( 'NONE',  ( 181.7937950796055588, 283.7749071970079626, -15.03297549846545778 ) ) ;
#61901=CARTESIAN_POINT ( 'NONE',  ( 189.8106237464670585, 301.8853511852161091, -0.6577604834569344971 ) ) ;
#61902=CARTESIAN_POINT ( 'NONE',  ( 165.3728640525272340, 283.7448754721146429, -8.387219889811008855 ) ) ;
#61903=ORIENTED_EDGE ( 'NONE', *, *, #98217, .F. ) ;
#61904=CARTESIAN_POINT ( 'NONE',  ( 207.6523394534040392, 270.9825930866021508, -2.115019688068903392 ) ) ;
#61906=EDGE_CURVE ( 'NONE', #346, #65763, #10941, .T. ) ;
#61907=CARTESIAN_POINT ( 'NONE',  ( 53.62548896571606605, 191.7677522451418213, -5.000000000000041744 ) ) ;
#61908=CARTESIAN_POINT ( 'NONE',  ( 129.3758220526426044, 239.3768266524159856, -9.188101187500093303 ) ) ;
#61909=CARTESIAN_POINT ( 'NONE',  ( 150.6438662863770332, 269.7241650738195631, -14.92510732909997628 ) ) ;
#61911=CARTESIAN_POINT ( 'NONE',  ( 164.7396270603856294, 269.0037874151494179, 17.61975801440670608 ) ) ;
#61912=CARTESIAN_POINT ( 'NONE',  ( 196.1241105319816143, 290.9500712997905794, 15.97146679939154268 ) ) ;
#61913=CARTESIAN_POINT ( 'NONE',  ( 45.14796862286864609, 185.3262482093457493, 3.021315404115420679E-15 ) ) ;
#61914=CARTESIAN_POINT ( 'NONE',  ( 50.56751030825869009, 193.8768266524160140, 9.188101187500098632 ) ) ;
#61920=CARTESIAN_POINT ( 'NONE',  ( 147.5848197185516142, 275.0225891520124151, 4.420251097676741736 ) ) ;
#61922=CARTESIAN_POINT ( 'NONE',  ( 152.8642676789094423, 276.0723602830860273, -10.03519574156767469 ) ) ;
#61923=CARTESIAN_POINT ( 'NONE',  ( 178.5937152032327333, 260.7852093525231680, 13.58383975110821673 ) ) ;
#61924=CARTESIAN_POINT ( 'NONE',  ( 99.16399144804771026, 241.3927522451419634, 2.944929066748280225E-16 ) ) ;
#61926=ORIENTED_EDGE ( 'NONE', *, *, #69640, .T. ) ;
#61927=CARTESIAN_POINT ( 'NONE',  ( 189.8480911035503880, 301.8204558191226283, -0.8992086515915015399 ) ) ;
#61928=CARTESIAN_POINT ( 'NONE',  ( 163.4178923001155681, 247.5989030008181260, -10.38047187240561442 ) ) ;
#61929=CARTESIAN_POINT ( 'NONE',  ( 22.04262502322622908, 183.5333772461660544, 9.188101187500095079 ) ) ;
#61931=CARTESIAN_POINT ( 'NONE',  ( 194.8387898011405355, 273.2648853755486016, 14.40873911934531648 ) ) ;
#61932=CARTESIAN_POINT ( 'NONE',  ( 35.60133525300030755, 191.3615022471902591, -10.00000000000009592 ) ) ;
#61934=CARTESIAN_POINT ( 'NONE',  ( 174.9526703860257726, 286.4149860108961434, 10.48728481691800773 ) ) ;
#61935=CARTESIAN_POINT ( 'NONE',  ( 67.67116493723634107, 216.0024278399160664, -9.188101187500093303 ) ) ;
#61936=CARTESIAN_POINT ( 'NONE',  ( 161.1611771195837548, 251.5076483517112536, 14.17749514252127163 ) ) ;
#61940=VERTEX_POINT ( 'NONE', #23115 ) ;
#61941=CARTESIAN_POINT ( 'NONE',  ( 165.4470874010085026, 269.3013239833477996, 16.98587756655855330 ) ) ;
#61942=CARTESIAN_POINT ( 'NONE',  ( 30.40518283029366842, 188.3615022471902591, -10.00000000000009592 ) ) ;
#61943=CARTESIAN_POINT ( 'NONE',  ( 163.8398374448017591, 246.8680725722146008, -5.948785025486735378 ) ) ;
#61944=CARTESIAN_POINT ( 'NONE',  ( 1.691375130056927079, 159.5327760586659451, 1.948934522072303157E-15 ) ) ;
#61947=EDGE_CURVE ( 'NONE', #72615, #71188, #80951, .T. ) ;
#61948=CARTESIAN_POINT ( 'NONE',  ( 185.4642089758430927, 260.0334125403911685, 7.310543569370538286 ) ) ;
#61949=CARTESIAN_POINT ( 'NONE',  ( 205.7867067512454184, 274.2139637150027056, 10.62737868262404106 ) ) ;
#61952=ORIENTED_EDGE ( 'NONE', *, *, #72713, .F. ) ;
#61953=B_SPLINE_CURVE_WITH_KNOTS ( 'NONE', 3,
 ( #39970, #70905, #23787, #1514 ),
 .UNSPECIFIED., .F., .F.,
 ( 4, 4 ),
 ( 0.03743099264120831882, 0.04603662255807886017 ),
 .UNSPECIFIED. ) ;
#61954=CARTESIAN_POINT ( 'NONE',  ( 164.1303272795579176, 246.3649294193346009, 8.276858000922496572 ) ) ;
#61959=CARTESIAN_POINT ( 'NONE',  ( 160.0298054686767557, 253.4672415333249376, 14.79725849075877520 ) ) ;
#61962=CARTESIAN_POINT ( 'NONE',  ( 178.6603775665675187, 266.7231829388173878, 16.69313589097744455 ) ) ;
#61963=CARTESIAN_POINT ( 'NONE',  ( 207.8446715390582540, 270.6494641423232679, -2.429516028743652800 ) ) ;
#61964=CARTESIAN_POINT ( 'NONE',  ( 152.9251141908703175, 265.7729277985770864, -16.20110192949203309 ) ) ;
#61965=VERTEX_POINT ( 'NONE', #45906 ) ;
#61966=ORIENTED_EDGE ( 'NONE', *, *, #81441, .T. ) ;
#61967=CARTESIAN_POINT ( 'NONE',  ( 190.8154370666929367, 280.9968047295526503, 16.65367678528672002 ) ) ;
#61968=CARTESIAN_POINT ( 'NONE',  ( 151.3011447763744570, 269.1990464485573966, 14.21186556778774168 ) ) ;
#61969=VERTEX_POINT ( 'NONE', #54007 ) ;
#61972=EDGE_LOOP ( 'NONE', ( #5539, #51144 ) ) ;
#61973=CARTESIAN_POINT ( 'NONE',  ( 191.4082244002820516, 299.1182256826033949, -8.271837126846561361 ) ) ;
#61976=LINE ( 'NONE', #69598, #91796 ) ;
#61979=CARTESIAN_POINT ( 'NONE',  ( 161.1238074876215478, 251.5723744529297505, 13.42537408252843179 ) ) ;
#61980=CARTESIAN_POINT ( 'NONE',  ( 191.5451565139252068, 298.8810523045859213, 7.782291334092181323 ) ) ;
#61981=CARTESIAN_POINT ( 'NONE',  ( 170.6653991834546389, 280.1030447246535005, -15.19489322104400664 ) ) ;
#61986=CARTESIAN_POINT ( 'NONE',  ( 160.0205417486836836, 268.7952604174922158, -17.12082356920033277 ) ) ;
#61987=EDGE_LOOP ( 'NONE', ( #31558, #33670, #10129 ) ) ;
#61989=EDGE_LOOP ( 'NONE', ( #57654, #87421, #41599, #57019 ) ) ;
#61990=CARTESIAN_POINT ( 'NONE',  ( 207.6471633721571379, 270.9915583223058206, 2.196965492132801678 ) ) ;
#61991=( BOUNDED_CURVE ( )  B_SPLINE_CURVE ( 2, ( #48821, #89725, #96824, #82630, #66374, #27873, #20286, #58269, #13191 ),
 .UNSPECIFIED., .F., .T. ) 
 B_SPLINE_CURVE_WITH_KNOTS ( ( 3, 2, 2, 2, 3 ),
 ( 0.8104838709677418818, 0.8118279569892472569, 0.8145161290322581182, 0.8172043010752688685, 0.8185483870967742437 ),
 .UNSPECIFIED. ) 
 CURVE ( )  GEOMETRIC_REPRESENTATION_ITEM ( )  RATIONAL_B_SPLINE_CURVE ( ( 0.9330127018922194093, 0.9330127018922194093, 1.000000000000000000, 0.8660254037844387076, 1.000000000000000000, 0.8660254037844387076, 1.000000000000000000, 0.9330127018922194093, 0.9330127018922194093 ) ) 
 REPRESENTATION_ITEM ( '' )  );
#61993=CARTESIAN_POINT ( 'NONE',  ( 165.0763782876348955, 271.0110069803866963, 16.91995621439599162 ) ) ;
#61994=CARTESIAN_POINT ( 'NONE',  ( 167.6829735571818674, 281.1103996008106378, 11.56255526439067260 ) ) ;
#61995=CARTESIAN_POINT ( 'NONE',  ( 148.1632261683078013, 274.0207597936089883, -7.853210555358286271 ) ) ;
#61997=CARTESIAN_POINT ( 'NONE',  ( 197.6146187704118802, 288.3684353017289936, -18.03711460092097241 ) ) ;
#61998=ORIENTED_EDGE ( 'NONE', *, *, #56609, .T. ) ;
#61999=CARTESIAN_POINT ( 'NONE',  ( 202.1660481100201423, 271.6014475893761073, -11.28653549010346246 ) ) ;
#62001=EDGE_CURVE ( 'NONE', #8790, #81989, #61498, .T. ) ;
#62002=CARTESIAN_POINT ( 'NONE',  ( 198.5695182982529730, 276.9374223074942165, -15.29489990819768686 ) ) ;
#62003=CARTESIAN_POINT ( 'NONE',  ( 185.6299035038124430, 291.5639447024825586, -13.39789161462089773 ) ) ;
#62004=CARTESIAN_POINT ( 'NONE',  ( 206.8218526254527490, 270.5579068801799849, 5.033309423535771820 ) ) ;
#62005=ORIENTED_EDGE ( 'NONE', *, *, #67686, .F. ) ;
#62006=CARTESIAN_POINT ( 'NONE',  ( 146.6807985088175030, 276.5883998183917925, -3.564129467591749201 ) ) ;
#62007=CARTESIAN_POINT ( 'NONE',  ( 58.82164138842265544, 204.7677522451418781, 10.00000000000009592 ) ) ;
#62008=CARTESIAN_POINT ( 'NONE',  ( 159.2122473525774069, 254.8832937285494609, -16.22689353966294590 ) ) ;
#62012=CARTESIAN_POINT ( 'NONE',  ( 171.4761949442340665, 255.4795810469701109, 11.08406205635473185 ) ) ;
#62013=CARTESIAN_POINT ( 'NONE',  ( 157.4580857293093743, 281.9160373083212221, 1.421786535070352686 ) ) ;
#62014=ORIENTED_EDGE ( 'NONE', *, *, #86236, .T. ) ;
#62015=CARTESIAN_POINT ( 'NONE',  ( 194.1377662266459936, 294.3905205579567905, -15.67343962259168322 ) ) ;
#62018=ADVANCED_FACE ( 'NONE', ( #30738 ), #53523, .T. ) ;
#62019=CARTESIAN_POINT ( 'NONE',  ( -2.305318362029010082, 176.1427522451419350, -10.00000000000009415 ) ) ;
#62020=CARTESIAN_POINT ( 'NONE',  ( 85.20852645963621796, 213.8768266524159856, -9.188101187500093303 ) ) ;
#62021=CARTESIAN_POINT ( 'NONE',  ( 196.0579333247489160, 269.4436101228905613, -10.81265959875389626 ) ) ;
#62022=CARTESIAN_POINT ( 'NONE',  ( 174.6308490632290500, 282.2634308488150623, -14.29746604333752202 ) ) ;
#62023=CARTESIAN_POINT ( 'NONE',  ( 170.2443324258450730, 280.7353186831560379, -14.04127619006417582 ) ) ;
#62025=CARTESIAN_POINT ( 'NONE',  ( 2.394500126984267396, 178.3149278399160949, -9.188101187500095079 ) ) ;
#62028=CARTESIAN_POINT ( 'NONE',  ( 200.8432122835317841, 282.7763473000181307, 17.15137370990203891 ) ) ;
#62030=VERTEX_POINT ( 'NONE', #37816 ) ;
#62031=CARTESIAN_POINT ( 'NONE',  ( 188.7958840745704663, 260.8248006898061817, -6.220177282829866705 ) ) ;
#62034=CARTESIAN_POINT ( 'NONE',  ( 161.4250356354754672, 267.9004136800010656, 17.49898951125957680 ) ) ;
#62036=CARTESIAN_POINT ( 'NONE',  ( 19.17374232530777078, 188.0024278399160949, 9.188101187500095079 ) ) ;
#62037=CARTESIAN_POINT ( 'NONE',  ( 129.3758220526426044, 239.3768266524160140, -9.188101187500091527 ) ) ;
#62040=CARTESIAN_POINT ( 'NONE',  ( -22.42236680055709641, 157.8615022471902591, 0.000000000000000000 ) ) ;
#62041=VECTOR ( 'NONE', #75675, 1000.000000000000000 ) ;
#62042=CARTESIAN_POINT ( 'NONE',  ( 177.2802394469194383, 252.6157282624358231, 1.078711111416747359 ) ) ;
#62045=CARTESIAN_POINT ( 'NONE',  ( 155.6435836392643637, 261.0644005951349982, 17.58841156286628049 ) ) ;
#62046=CARTESIAN_POINT ( 'NONE',  ( 207.8575108622103755, 270.6272257822888037, -6.381720258959569847 ) ) ;
#62048=CARTESIAN_POINT ( 'NONE',  ( 194.9819925439454664, 292.9282776833073285, -15.33279721168237586 ) ) ;
#62049=EDGE_CURVE ( 'NONE', #9692, #18680, #1039, .T. ) ;
#62050=EDGE_CURVE ( 'NONE', #60494, #7831, #55381, .T. ) ;
#62051=CARTESIAN_POINT ( 'NONE',  ( 190.2071741674316456, 263.6913551221517196, 7.843308196823155498 ) ) ;
#62052=CARTESIAN_POINT ( 'NONE',  ( 169.0861754935146450, 278.6444814197644746, 14.06024944971096957 ) ) ;
#62053=CARTESIAN_POINT ( 'NONE',  ( 192.6564221164474020, 265.0321580081510433, 8.767841527359648168 ) ) ;
#62055=CARTESIAN_POINT ( 'NONE',  ( 190.6036479972031259, 300.5117928913073797, -0.6824572005520307405 ) ) ;
#62056=CARTESIAN_POINT ( 'NONE',  ( 180.8238051759404073, 266.9217313885388876, -14.75443455289115313 ) ) ;
#62057=ORIENTED_EDGE ( 'NONE', *, *, #11338, .F. ) ;
#62060=CARTESIAN_POINT ( 'NONE',  ( 207.5583741822599393, 271.1453457103705205, 3.140867606700001424 ) ) ;
#62061=CARTESIAN_POINT ( 'NONE',  ( 188.7764831123630529, 299.4247982080598263, -5.354475200873774376 ) ) ;
#62062=CARTESIAN_POINT ( 'NONE',  ( 110.7287787077026451, 243.9244531367911293, -4.594050593750046652 ) ) ;
#62064=CARTESIAN_POINT ( 'NONE',  ( 150.8359915840788688, 269.3913942967808453, 15.73449616766854575 ) ) ;
#62065=ADVANCED_FACE ( 'NONE', ( #40308 ), #25120, .T. ) ;
#62068=CARTESIAN_POINT ( 'NONE',  ( 195.6116440902121383, 278.4173475472090900, 16.65080808324301742 ) ) ;
#62069=CARTESIAN_POINT ( 'NONE',  ( 191.3034052106035858, 299.2997778447344785, -7.689850778203263459 ) ) ;
#62070=CARTESIAN_POINT ( 'NONE',  ( 150.6815632051821581, 269.6588720951601772, -14.68790257316217307 ) ) ;
#62071=CARTESIAN_POINT ( 'NONE',  ( 165.8206990081297931, 283.8978799598649516, 9.576760697357309837 ) ) ;
#62072=CARTESIAN_POINT ( 'NONE',  ( 80.61430232155159104, 228.8967562850347122, -4.648177544792955347E-16 ) ) ;
#62073=CARTESIAN_POINT ( 'NONE',  ( 204.1284829764352367, 276.6911759709722105, 13.49772714134504170 ) ) ;
#62076=CARTESIAN_POINT ( 'NONE',  ( 193.0390622633530029, 267.0550773046203972, 11.36550167083046503 ) ) ;
#62079=CARTESIAN_POINT ( 'NONE',  ( 200.0400595503645036, 270.0189624897442968, 9.074847133236374930 ) ) ;
#62080=CARTESIAN_POINT ( 'NONE',  ( 196.6800254274587019, 289.9871984561398222, -17.90749311895638129 ) ) ;
#62081=EDGE_CURVE ( 'NONE', #26754, #88465, #9973, .T. ) ;
#62084=CARTESIAN_POINT ( 'NONE',  ( 152.7893866619400001, 275.1786922041311527, 10.91924690663370612 ) ) ;
#62086=CARTESIAN_POINT ( 'NONE',  ( 182.3702127349715738, 264.1602241078386442, -12.99238495943751914 ) ) ;
#62088=CARTESIAN_POINT ( 'NONE',  ( 192.1396999271463812, 297.8512729055811974, 12.32430960859512403 ) ) ;
#62092=VERTEX_POINT ( 'NONE', #1841 ) ;
#62094=FACE_OUTER_BOUND ( 'NONE', #59514, .T. ) ;
#62095=VERTEX_POINT ( 'NONE', #63626 ) ;
#62097=CARTESIAN_POINT ( 'NONE',  ( 158.9057798085220838, 255.4141110857242154, 17.55677396874652629 ) ) ;
#62104=ORIENTED_EDGE ( 'NONE', *, *, #11432, .T. ) ;
#62105=CARTESIAN_POINT ( 'NONE',  ( 196.0580054393319642, 290.6771910296030796, 16.00258381118181461 ) ) ;
#62112=CARTESIAN_POINT ( 'NONE',  ( 165.8334311161731023, 274.4591478290780060, -15.12211806599400532 ) ) ;
#62113=CARTESIAN_POINT ( 'NONE',  ( 206.0316325540811704, 273.7897397804065918, -11.04223638802967322 ) ) ;
#62114=CARTESIAN_POINT ( 'NONE',  ( 190.6240973886985159, 300.4763735062533669, 2.216935469364557321 ) ) ;
#62115=CARTESIAN_POINT ( 'NONE',  ( 198.2399221193978462, 285.6735130211258138, -17.04706178669553296 ) ) ;
#62117=CARTESIAN_POINT ( 'NONE',  ( 167.7086961934988096, 249.0458231482594158, -5.172654644684703484 ) ) ;
#62119=CARTESIAN_POINT ( 'NONE',  ( 186.0598909074496419, 286.3830271726962451, -15.31043294068512672 ) ) ;
#62120=CARTESIAN_POINT ( 'NONE',  ( 126.3990332750161087, 231.5327760586659736, 1.948934522072303157E-15 ) ) ;
#62123=CARTESIAN_POINT ( 'NONE',  ( 177.4031824437115574, 288.8941654109167416, -9.335669202574084835 ) ) ;
#62124=ORIENTED_EDGE ( 'NONE', *, *, #39597, .F. ) ;
#62127=CARTESIAN_POINT ( 'NONE',  ( 177.6201654249851174, 253.7431718786475869, 1.360499885134917708 ) ) ;
#62130=CARTESIAN_POINT ( 'NONE',  ( 171.0924760015939512, 287.7303114454449542, -4.798180175186202767 ) ) ;
#62131=CARTESIAN_POINT ( 'NONE',  ( 146.6795228420702983, 276.5906093380114612, 3.172940435457009656 ) ) ;
#62133=CARTESIAN_POINT ( 'NONE',  ( 153.0927037754837556, 265.4826541232073964, -16.15085267704102634 ) ) ;
#62134=CARTESIAN_POINT ( 'NONE',  ( 177.2355366647990991, 288.8864627520729869, -9.231742449898762359 ) ) ;
#62136=CARTESIAN_POINT ( 'NONE',  ( 194.7489730912498658, 293.3318792145281009, 16.23511080478873225 ) ) ;
#62138=ORIENTED_EDGE ( 'NONE', *, *, #95871, .F. ) ;
#62139=CARTESIAN_POINT ( 'NONE',  ( 194.6356465353167948, 293.5281665672507643, -16.13180903283129197 ) ) ;
#62140=CARTESIAN_POINT ( 'NONE',  ( 165.8841617674041515, 247.6200161724019324, -6.929307956321339113 ) ) ;
#62141=ORIENTED_EDGE ( 'NONE', *, *, #67135, .F. ) ;
#62142=CARTESIAN_POINT ( 'NONE',  ( 191.6390250992932920, 267.7947042169313931, -12.26094334802855812 ) ) ;
#62143=EDGE_CURVE ( 'NONE', #42238, #97169, #85801, .T. ) ;
#62144=CARTESIAN_POINT ( 'NONE',  ( 156.8824101620476483, 276.5798998049355646, 10.22994899405466640 ) ) ;
#62145=CARTESIAN_POINT ( 'NONE',  ( 193.4656735081794068, 262.7486161809156897, 4.740984612795180908 ) ) ;
#62146=CARTESIAN_POINT ( 'NONE',  ( 149.7162292714551199, 271.3308795146458010, 12.12826134257344357 ) ) ;
#62147=CARTESIAN_POINT ( 'NONE',  ( 202.8499463704053198, 279.3005819042728604, 17.04674939340617001 ) ) ;
#62148=CARTESIAN_POINT ( 'NONE',  ( 153.3701107251964402, 270.1885625906204496, 14.06860214899441530 ) ) ;
#62149=CARTESIAN_POINT ( 'NONE',  ( 156.8098655126457572, 280.3055410020735962, 5.930865079079680413 ) ) ;
#62150=CARTESIAN_POINT ( 'NONE',  ( 199.9276962100341564, 267.5423408568639161, 6.196014648939567770 ) ) ;
#62151=ORIENTED_EDGE ( 'NONE', *, *, #98949, .T. ) ;
#62152=CARTESIAN_POINT ( 'NONE',  ( 146.8201187048455267, 276.3470901603510015, 4.112223577763169047 ) ) ;
#62154=CARTESIAN_POINT ( 'NONE',  ( 186.7460581780939322, 262.7394680154919229, -8.960597522048372454 ) ) ;
#62155=CARTESIAN_POINT ( 'NONE',  ( 168.8563211758018099, 286.0187424789903048, -9.056861680415359217 ) ) ;
#62156=CARTESIAN_POINT ( 'NONE',  ( 147.3907811248416238, 249.2365022471901739, -10.00000000000009237 ) ) ;
#62157=EDGE_CURVE ( 'NONE', #78498, #77729, #17050, .T. ) ;
#62158=CARTESIAN_POINT ( 'NONE',  ( 186.5739769617673289, 297.4340541020540059, -4.270514905203655509 ) ) ;
#62159=EDGE_CURVE ( 'NONE', #25883, #34337, #69100, .T. ) ;
#62160=CARTESIAN_POINT ( 'NONE',  ( 192.2431834237441706, 297.6720342317289578, 11.07782187406058938 ) ) ;
#62162=CARTESIAN_POINT ( 'NONE',  ( 194.4263876777154394, 293.8906135405502482, 15.23185943445137802 ) ) ;
#62163=CARTESIAN_POINT ( 'NONE',  ( 191.1334016331724399, 283.3379655378311099, -16.58600049649699670 ) ) ;
#62165=CARTESIAN_POINT ( 'NONE',  ( 73.67938972387338481, 213.3458772461660544, 9.188101187500095079 ) ) ;
#62166=DIRECTION ( 'NONE',  ( -0.8660254037844387076, -0.4999999999999998890, -0.000000000000000000 ) ) ;
#62167=CARTESIAN_POINT ( 'NONE',  ( 147.5540328368684300, 275.0759135952944234, -4.750028533202499403 ) ) ;
#62168=CARTESIAN_POINT ( 'NONE',  ( 55.08690683815017763, 202.6115022471902591, 10.00000000000009592 ) ) ;
#62170=FACE_OUTER_BOUND ( 'NONE', #38073, .T. ) ;
#62175=CARTESIAN_POINT ( 'NONE',  ( 161.8677343474444683, 250.2838553346012986, 14.13526557951369433 ) ) ;
#62177=CARTESIAN_POINT ( 'NONE',  ( 161.3523358740237938, 251.5903407549832593, 13.23360137856301932 ) ) ;
#62178=CARTESIAN_POINT ( 'NONE',  ( 157.6673516573649181, 257.5591315650518141, 16.79781451397666103 ) ) ;
#62182=CARTESIAN_POINT ( 'NONE',  ( 49.83688814775681664, 190.3923013555410080, 4.594050593750050204 ) ) ;
#62183=CARTESIAN_POINT ( 'NONE',  ( 56.60219097117523290, 212.6744531367911293, 4.594050593750047540 ) ) ;
#62187=EDGE_CURVE ( 'NONE', #91328, #19784, #66353, .T. ) ;
#62188=CARTESIAN_POINT ( 'NONE',  ( 163.6024448037938157, 257.9599251185455273, 15.55702952704531761 ) ) ;
#62189=CARTESIAN_POINT ( 'NONE',  ( 142.6906155400633622, 259.3149278399160380, -9.188101187500095079 ) ) ;
#62191=CARTESIAN_POINT ( 'NONE',  ( 196.7067773240564748, 268.6313083337223588, -10.65017239398339655 ) ) ;
#62193=CARTESIAN_POINT ( 'NONE',  ( 198.9225589249066957, 286.1030165008847916, -17.03502353404871883 ) ) ;
#62196=CARTESIAN_POINT ( 'NONE',  ( 55.84441874286383722, 212.2369531367911293, -4.594050593750048428 ) ) ;
#62200=CARTESIAN_POINT ( 'NONE',  ( 198.4264492142971221, 286.9623037257889564, 17.00126466006521397 ) ) ;
#62201=CARTESIAN_POINT ( 'NONE',  ( 56.72874666261028409, 196.8927522451418497, 10.00000000000009948 ) ) ;
#62202=CARTESIAN_POINT ( 'NONE',  ( 201.4399981830169111, 281.7426838008692584, 17.62180968337201392 ) ) ;
#62203=EDGE_CURVE ( 'NONE', #72620, #7391, #25264, .T. ) ;
#62205=CARTESIAN_POINT ( 'NONE',  ( 109.1413257910288479, 240.4865022471902876, 10.00000000000009237 ) ) ;
#62207=CARTESIAN_POINT ( 'NONE',  ( 207.1059763530604698, 271.9289217357780899, 6.370907250589925575 ) ) ;
#62212=CARTESIAN_POINT ( 'NONE',  ( 206.3018347371251195, 273.3217358710584790, -9.309724106897926177 ) ) ;
#62213=CARTESIAN_POINT ( 'NONE',  ( 188.4547781097711834, 277.6015940764860375, -16.57049336306976883 ) ) ;
#62214=CARTESIAN_POINT ( 'NONE',  ( 164.6063343576543048, 274.4739709976624908, 16.17759516952312637 ) ) ;
#62217=ORIENTED_EDGE ( 'NONE', *, *, #38710, .F. ) ;
#62219=CARTESIAN_POINT ( 'NONE',  ( 148.3253847707240141, 273.7398928553401447, -9.074433450356286457 ) ) ;
#62221=ORIENTED_EDGE ( 'NONE', *, *, #18327, .F. ) ;
#62228=CARTESIAN_POINT ( 'NONE',  ( -0.4807448425718762741, 158.9824982072973683, 3.021315404115420679E-15 ) ) ;
#62229=EDGE_LOOP ( 'NONE', ( #28351, #59794, #88142, #22387 ) ) ;
#62230=CARTESIAN_POINT ( 'NONE',  ( 171.3153268440470356, 284.6697624753109039, 10.75620792707900009 ) ) ;
#62234=CARTESIAN_POINT ( 'NONE',  ( 204.9768178125733016, 275.6167325052707611, 13.98665089523138505 ) ) ;
#62236=CARTESIAN_POINT ( 'NONE',  ( 204.9658583905037688, 275.6357147811169170, -12.57240504404813564 ) ) ;
#62237=CARTESIAN_POINT ( 'NONE',  ( 138.1979352100490530, 262.8464784336661637, 1.353441290958777525E-15 ) ) ;
#62238=CARTESIAN_POINT ( 'NONE',  ( 206.4634061315404665, 270.6220774564198450, 2.471500839510567094 ) ) ;
#62239=CARTESIAN_POINT ( 'NONE',  ( 182.5855175857635686, 259.4356802941314299, 9.332393434239792285 ) ) ;
#62240=CARTESIAN_POINT ( 'NONE',  ( 78.52397964811635234, 206.9548013555409796, -4.594050593750042211 ) ) ;
#62242=CARTESIAN_POINT ( 'NONE',  ( 150.6571681785161445, 269.7011255207979730, 15.24894850018880454 ) ) ;
#62246=CARTESIAN_POINT ( 'NONE',  ( 195.8873709255798587, 291.3601163262420641, -15.74573728859107646 ) ) ;
#62250=CARTESIAN_POINT ( 'NONE',  ( 73.70645301951556405, 223.3615022471903160, 5.000000000000046185 ) ) ;
#62251=CARTESIAN_POINT ( 'NONE',  ( 191.8456210280128005, 298.3606325003146367, -9.135603544929113085 ) ) ;
#62252=DIRECTION ( 'NONE',  ( -0.8660254037844387076, -0.4999999999999998890, -0.000000000000000000 ) ) ;
#62254=CARTESIAN_POINT ( 'NONE',  ( 207.8833583980453739, 270.5824565369721313, 1.564926904161892285 ) ) ;
#62255=CARTESIAN_POINT ( 'NONE',  ( 75.84410613756948294, 226.8464784336661353, 1.353441290958777327E-15 ) ) ;
#62256=ORIENTED_EDGE ( 'NONE', *, *, #51234, .F. ) ;
#62258=CARTESIAN_POINT ( 'NONE',  ( 161.2850924390880323, 251.2930207224935373, -13.14774649685070074 ) ) ;
#62264=CARTESIAN_POINT ( 'NONE',  ( 165.0087721269838710, 244.8434183119457543, 2.604344609212914108 ) ) ;
#62265=CARTESIAN_POINT ( 'NONE',  ( 161.5502493243027402, 284.0868935703256852, 0.5284661774659209499 ) ) ;
#62270=CARTESIAN_POINT ( 'NONE',  ( 154.7823760652066198, 279.7145020948755700, 5.599380836552000140 ) ) ;
#62271=CARTESIAN_POINT ( 'NONE',  ( 152.6873874250818517, 266.1846826352417565, -16.66598363829485763 ) ) ;
#62272=ADVANCED_FACE ( 'NONE', ( #3668 ), #3186, .T. ) ;
#62278=CYLINDRICAL_SURFACE ( 'NONE', #34827, 17.82106496071139645 ) ;
#62279=( BOUNDED_CURVE ( )  B_SPLINE_CURVE ( 2, ( #7901, #39261, #38270, #38776, #54979, #780, #39753, #86450, #70682 ),
 .UNSPECIFIED., .F., .T. ) 
 B_SPLINE_CURVE_WITH_KNOTS ( ( 3, 2, 2, 2, 3 ),
 ( 0.01209677419354838850, 0.01344086021505376365, 0.01612903225806451568, 0.01881720430107526945, 0.02016129032258064807 ),
 .UNSPECIFIED. ) 
 CURVE ( )  GEOMETRIC_REPRESENTATION_ITEM ( )  RATIONAL_B_SPLINE_CURVE ( ( 0.9330127018922194093, 0.9330127018922194093, 1.000000000000000000, 0.8660254037844387076, 1.000000000000000000, 0.8660254037844387076, 1.000000000000000000, 0.9330127018922191873, 0.9330127018922192983 ) ) 
 REPRESENTATION_ITEM ( '' )  );
#62280=CARTESIAN_POINT ( 'NONE',  ( 181.6597933908766436, 291.8373067516729407, 10.47321924421550321 ) ) ;
#62288=AXIS2_PLACEMENT_3D ( 'NONE', #82587, #91659, #36921 ) ;
#62289=FACE_OUTER_BOUND ( 'NONE', #43206, .T. ) ;
#62294=CARTESIAN_POINT ( 'NONE',  ( 172.0916398547322785, 275.0630559527974697, 16.92144769315549979 ) ) ;
#62295=CARTESIAN_POINT ( 'NONE',  ( 163.2303979562223333, 283.9008525415044346, -3.773057203759900169 ) ) ;
#62297=CARTESIAN_POINT ( 'NONE',  ( 192.0195900110790319, 262.3135081745301704, 2.967184076358189593 ) ) ;
#62299=CARTESIAN_POINT ( 'NONE',  ( 0.1211834420501121806, 177.0024278399160949, -9.188101187500093303 ) ) ;
#62300=CYLINDRICAL_SURFACE ( 'NONE', #93802, 10.00000000000010658 ) ;
#62302=CARTESIAN_POINT ( 'NONE',  ( 178.3300713922748457, 256.8661311210547638, 8.413408369093348327 ) ) ;
#62303=EDGE_CURVE ( 'NONE', #11947, #51377, #19732, .T. ) ;
#62305=CARTESIAN_POINT ( 'NONE',  ( 161.9296067209906198, 272.1511200004533180, 16.47594105373750750 ) ) ;
#62306=CARTESIAN_POINT ( 'NONE',  ( 20.95974617273066443, 195.1589784336661637, -6.496448406907676862E-16 ) ) ;
#62310=CARTESIAN_POINT ( 'NONE',  ( 191.8456210280128005, 298.3606325003146367, -9.135603544929113085 ) ) ;
#62314=CARTESIAN_POINT ( 'NONE',  ( 188.0081030067536858, 260.0748169616455243, -0.7643377115716368797 ) ) ;
#62316=B_SPLINE_CURVE_WITH_KNOTS ( 'NONE', 3,
 ( #62631, #9967, #25143, #23631 ),
 .UNSPECIFIED., .F., .F.,
 ( 4, 4 ),
 ( 0.01247596805550315810, 0.01873461069493020936 ),
 .UNSPECIFIED. ) ;
#62317=CARTESIAN_POINT ( 'NONE',  ( 62.88113547221008304, 217.1115022471903160, -5.000000000000047962 ) ) ;
#62320=CARTESIAN_POINT ( 'NONE',  ( 32.38097682878547090, 183.3768266524159856, 9.188101187500098632 ) ) ;
#62322=B_SPLINE_CURVE_WITH_KNOTS ( 'NONE', 3,
 ( #29129, #67108, #99527, #97547, #68108, #52904, #59996, #90965, #44303, #36700, #37207, #28610 ),
 .UNSPECIFIED., .F., .F.,
 ( 4, 2, 2, 2, 2, 4 ),
 ( 0.001941519080533212534, 0.002048514964777567709, 0.002155510849021922883, 0.002369502617510633666, 0.002797486154488115079, 0.003653453228443075736 ),
 .UNSPECIFIED. ) ;
#62324=CARTESIAN_POINT ( 'NONE',  ( 65.47921168356340615, 218.6115022471903160, -5.000000000000047962 ) ) ;
#62325=CARTESIAN_POINT ( 'NONE',  ( 151.4376533647338476, 268.3492855237141725, -15.16853828792834236 ) ) ;
#62329=B_SPLINE_CURVE_WITH_KNOTS ( 'NONE', 3,
 ( #59419, #30032, #60918, #37622 ),
 .UNSPECIFIED., .F., .F.,
 ( 4, 4 ),
 ( 0.01532915748665746730, 0.02410358160937203786 ),
 .UNSPECIFIED. ) ;
#62330=CARTESIAN_POINT ( 'NONE',  ( 202.7787896891747721, 278.0581983447742118, -15.29768258928314317 ) ) ;
#62334=CARTESIAN_POINT ( 'NONE',  ( 147.6300909839706321, 274.9441770201837585, 8.328755691084779755 ) ) ;
#62344=CARTESIAN_POINT ( 'NONE',  ( 150.6931560952953646, 269.6387926204777727, 14.65021044537114037 ) ) ;
#62345=CARTESIAN_POINT ( 'NONE',  ( 180.9708674785521794, 257.0886412231608347, -7.749587717661919228 ) ) ;
#62348=ORIENTED_EDGE ( 'NONE', *, *, #58561, .T. ) ;
#62349=CARTESIAN_POINT ( 'NONE',  ( 189.6768609436964539, 274.4077930505946483, -17.07046811116321550 ) ) ;
#62351=CARTESIAN_POINT ( 'NONE',  ( 153.4613150239306094, 264.8442007126561748, -16.86932470306368259 ) ) ;
#62356=CARTESIAN_POINT ( 'NONE',  ( 147.6618183892331331, 274.8892235422768522, 8.990680574201936892 ) ) ;
#62358=ORIENTED_EDGE ( 'NONE', *, *, #69634, .F. ) ;
#62360=CARTESIAN_POINT ( 'NONE',  ( 162.0988651326803165, 266.7229752693668274, 16.74775755896888896 ) ) ;
#62361=ORIENTED_EDGE ( 'NONE', *, *, #44670, .T. ) ;
#62363=CARTESIAN_POINT ( 'NONE',  ( 190.4249800432324662, 300.8212548652687133, 3.085047376053959400 ) ) ;
#62366=CARTESIAN_POINT ( 'NONE',  ( 179.6160012257981862, 295.0481727651569486, 1.085779272287555663 ) ) ;
#62368=CARTESIAN_POINT ( 'NONE',  ( 150.7576929667484080, 269.5270114801595582, 13.75028158740543205 ) ) ;
#62375=CARTESIAN_POINT ( 'NONE',  ( 172.3935366929414954, 290.1034599593647840, 4.993860462594684080 ) ) ;
#62376=CARTESIAN_POINT ( 'NONE',  ( 189.8136646974935786, 301.8800841035353528, -0.6430783927310335102 ) ) ;
#62377=VERTEX_POINT ( 'NONE', #36030 ) ;
#62378=CARTESIAN_POINT ( 'NONE',  ( 190.4163244163388242, 300.8362468508201459, 4.691083071570470331 ) ) ;
#62381=CARTESIAN_POINT ( 'NONE',  ( 146.8312060062178830, 276.3278863910550172, -4.807241325481028227 ) ) ;
#62382=CARTESIAN_POINT ( 'NONE',  ( 159.9495225368867466, 255.4964586287468080, 16.29484429292893566 ) ) ;
#62384=CARTESIAN_POINT ( 'NONE',  ( 164.3022921857394749, 246.0670774647090582, 1.862798784958315856 ) ) ;
#62388=CARTESIAN_POINT ( 'NONE',  ( 115.5733686319456126, 237.5333772461660544, 9.188101187500095079 ) ) ;
#62390=CARTESIAN_POINT ( 'NONE',  ( 146.6363376198206652, 276.6654083370839885, -0.5879280619134327202 ) ) ;
#62393=CARTESIAN_POINT ( 'NONE',  ( 155.6328838216860220, 261.0829332228125850, -17.51014940606912518 ) ) ;
#62396=CARTESIAN_POINT ( 'NONE',  ( 204.5730103890532519, 276.3161474792809145, 14.88139715235883109 ) ) ;
#62399=CARTESIAN_POINT ( 'NONE',  ( 165.4745112603759196, 283.5991399024592852, -8.288623825315429627 ) ) ;
#62401=CARTESIAN_POINT ( 'NONE',  ( 162.6341128535665064, 248.9564488241690299, -10.63508949045170660 ) ) ;
#62406=CARTESIAN_POINT ( 'NONE',  ( 186.3568650544643788, 297.0301385972502999, 4.669442245733694818 ) ) ;
#62407=CARTESIAN_POINT ( 'NONE',  ( 157.4177733328310467, 257.9914139036126812, 18.29188238796808363 ) ) ;
#62409=CARTESIAN_POINT ( 'NONE',  ( 56.62968813474974894, 197.3768266524160140, -9.188101187500091527 ) ) ;
#62415=CARTESIAN_POINT ( 'NONE',  ( 174.5460195235792185, 262.1449155284953463, 14.31061777505408550 ) ) ;
#62417=CARTESIAN_POINT ( 'NONE',  ( 154.9048824156581361, 262.3438686460345366, -17.40627786727128168 ) ) ;
#62418=CARTESIAN_POINT ( 'NONE',  ( 9.458193372709603253, 186.2677522451419065, -5.000000000000047962 ) ) ;
#62419=EDGE_CURVE ( 'NONE', #75738, #92597, #40988, .T. ) ;
#62420=CARTESIAN_POINT ( 'NONE',  ( 106.9582200821077578, 225.8927522451417929, -10.00000000000009059 ) ) ;
#62422=ORIENTED_EDGE ( 'NONE', *, *, #12183, .T. ) ;
#62423=CARTESIAN_POINT ( 'NONE',  ( 147.6857584380539095, 274.8477581613835810, 8.112022437684441201 ) ) ;
#62424=DIRECTION ( 'NONE',  ( 0.4999999999999992784, -0.8660254037844390407, 0.000000000000000000 ) ) ;
#62426=CARTESIAN_POINT ( 'NONE',  ( 26.88721494746919660, 177.1423013555409796, -4.594050593750043987 ) ) ;
#62428=CARTESIAN_POINT ( 'NONE',  ( 71.47468121884192271, 223.6199935810940929, 2.679491924311251605 ) ) ;
#62431=CARTESIAN_POINT ( 'NONE',  ( 70.10703493326258240, 211.2833772461660544, -9.188101187500095079 ) ) ;
#62432=CARTESIAN_POINT ( 'NONE',  ( 200.2631011806900005, 283.7811292041749311, 18.23377125296567058 ) ) ;
#62436=EDGE_LOOP ( 'NONE', ( #61869, #19279, #92938 ) ) ;
#62438=CARTESIAN_POINT ( 'NONE',  ( 25.13686162393831225, 191.9865022471903444, -10.00000000000009415 ) ) ;
#62439=CARTESIAN_POINT ( 'NONE',  ( 202.7865629936218284, 279.4103651332174536, 17.10878160033216133 ) ) ;
#62440=CARTESIAN_POINT ( 'NONE',  ( -2.449395605728673875, 160.2048013555409796, 4.594050593750051981 ) ) ;
#62442=CARTESIAN_POINT ( 'NONE',  ( 187.0083344850037008, 268.0836409071914090, -15.22627500120235133 ) ) ;
#62443=CARTESIAN_POINT ( 'NONE',  ( 185.2872327023346486, 260.3622127835997162, 6.490969198090009051 ) ) ;
#62444=CARTESIAN_POINT ( 'NONE',  ( 205.9642072045669465, 273.9065239114831911, 10.22128930895731536 ) ) ;
#62445=CARTESIAN_POINT ( 'NONE',  ( 187.1191678700340049, 259.2397217809819381, -2.406884300832496493 ) ) ;
#62451=CARTESIAN_POINT ( 'NONE',  ( 178.8256996136875046, 285.6663809771316096, 13.03525068864620629 ) ) ;
#62454=VERTEX_POINT ( 'NONE', #47123 ) ;
#62455=CARTESIAN_POINT ( 'NONE',  ( 206.6658056343182182, 272.6913197846437242, 8.075000410244337345 ) ) ;
#62457=CARTESIAN_POINT ( 'NONE',  ( 198.2505066714982149, 285.2670451491296149, 0.000000000000000000 ) ) ;
#62459=FACE_OUTER_BOUND ( 'NONE', #43204, .T. ) ;
#62460=VECTOR ( 'NONE', #65305, 1000.000000000000000 ) ;
#62462=CARTESIAN_POINT ( 'NONE',  ( 162.6341128535665064, 248.9564488241690299, -10.63508949045170660 ) ) ;
#62463=CARTESIAN_POINT ( 'NONE',  ( 152.7691010214056462, 266.0431505347400503, -16.40662330462167162 ) ) ;
#62467=CARTESIAN_POINT ( 'NONE',  ( 191.3455589609127117, 293.0590026861491424, 14.61618767810703368 ) ) ;
#62471=ORIENTED_EDGE ( 'NONE', *, *, #28439, .F. ) ;
#62472=DIRECTION ( 'NONE',  ( -0.8660254037844387076, -0.4999999999999998890, -0.000000000000000000 ) ) ;
#62473=DIRECTION ( 'NONE',  ( -0.8660254037844387076, -0.4999999999999998890, -0.000000000000000000 ) ) ;
#62474=B_SPLINE_CURVE_WITH_KNOTS ( 'NONE', 3,
 ( #50587, #66303, #80045, #64812 ),
 .UNSPECIFIED., .F., .F.,
 ( 4, 4 ),
 ( 0.01047594276644663036, 0.01576736478584307016 ),
 .UNSPECIFIED. ) ;
#62475=CARTESIAN_POINT ( 'NONE',  ( 149.6191398986701415, 271.4990432411842676, -11.66821883946526839 ) ) ;
#62479=CARTESIAN_POINT ( 'NONE',  ( 203.5973318405936823, 278.0060722970681582, 15.26090353908968211 ) ) ;
#62480=CARTESIAN_POINT ( 'NONE',  ( 182.1983635332545646, 295.7656116556308916, 4.955917269626422872 ) ) ;
#62481=CARTESIAN_POINT ( 'NONE',  ( 191.2645787786270262, 299.3670271975948367, 7.309947121636420242 ) ) ;
#62489=ORIENTED_EDGE ( 'NONE', *, *, #63745, .T. ) ;
#62490=CARTESIAN_POINT ( 'NONE',  ( 163.7183543885751078, 247.0784873978576854, -6.786164904910574336 ) ) ;
#62492=CARTESIAN_POINT ( 'NONE',  ( 167.0546803224166297, 282.1702852132879684, 12.27869116404093752 ) ) ;
#62493=CARTESIAN_POINT ( 'NONE',  ( 194.6943296385021824, 293.4265244509877562, -16.10917128197217352 ) ) ;
#62498=VECTOR ( 'NONE', #47586, 1000.000000000000000 ) ;
#62499=CARTESIAN_POINT ( 'NONE',  ( 199.1397118623803522, 277.8245601848594220, -15.39428571812815960 ) ) ;
#62502=CARTESIAN_POINT ( 'NONE',  ( 206.9717321439337070, 271.7310522289461119, 5.619150226236434342 ) ) ;
#62505=CARTESIAN_POINT ( 'NONE',  ( 191.1000974364045533, 299.6519172392214614, 6.286483878122098190 ) ) ;
#62506=DIRECTION ( 'NONE',  ( 0.4999999999999992784, -0.8660254037844390407, 0.000000000000000000 ) ) ;
#62507=CARTESIAN_POINT ( 'NONE',  ( 159.2536436069973718, 254.8115933126508992, -15.76697951715411250 ) ) ;
#62508=FACE_OUTER_BOUND ( 'NONE', #31846, .T. ) ;
#62510=AXIS2_PLACEMENT_3D ( 'NONE', #76264, #6836, #27672 ) ;
#62512=CARTESIAN_POINT ( 'NONE',  ( 161.4844649541891499, 250.9476973967054789, 12.93553496455142415 ) ) ;
#62513=EDGE_CURVE ( 'NONE', #33184, #93443, #43376, .T. ) ;
#62515=ORIENTED_EDGE ( 'NONE', *, *, #27586, .F. ) ;
#62516=CARTESIAN_POINT ( 'NONE',  ( 194.0381243828431650, 294.5631052939833125, -15.60241059258410345 ) ) ;
#62519=EDGE_CURVE ( 'NONE', #77581, #941, #99031, .T. ) ;
#62520=CARTESIAN_POINT ( 'NONE',  ( 21.07736754015083491, 189.6427522451419350, -10.00000000000009415 ) ) ;
#62521=CARTESIAN_POINT ( 'NONE',  ( 86.31820828217628616, 211.4548013555409796, -4.594050593750042211 ) ) ;
#62524=DIRECTION ( 'NONE',  ( -0.8660254037844387076, -0.4999999999999998890, -0.000000000000000000 ) ) ;
#62525=CARTESIAN_POINT ( 'NONE',  ( 167.0653908164138386, 277.9579550851513545, -13.96737994587077125 ) ) ;
#62527=CARTESIAN_POINT ( 'NONE',  ( 16.17015057563676450, 170.9548013555409796, -4.594050593750042211 ) ) ;
#62529=CARTESIAN_POINT ( 'NONE',  ( 200.5438717407500917, 283.2948203288816558, 18.39667691545567152 ) ) ;
#62530=VECTOR ( 'NONE', #84297, 1000.000000000000000 ) ;
#62531=VERTEX_POINT ( 'NONE', #95787 ) ;
#62532=AXIS2_PLACEMENT_3D ( 'NONE', #91471, #36234, #59521 ) ;
#62535=CARTESIAN_POINT ( 'NONE',  ( 199.5099933602457725, 266.9753653439566392, -2.851387091630914750 ) ) ;
#62538=CARTESIAN_POINT ( 'NONE',  ( 207.1572261440131797, 271.8401544939704877, -5.633070628900782140 ) ) ;
#62539=CARTESIAN_POINT ( 'NONE',  ( 154.2853090730916676, 265.4170011543745886, 17.16471700533586642 ) ) ;
#62541=CARTESIAN_POINT ( 'NONE',  ( 39.44458330234355969, 184.3923013555410080, 4.594050593750050204 ) ) ;
#62542=CARTESIAN_POINT ( 'NONE',  ( 199.4811141560337830, 277.5223964234930349, 15.18207637411607713 ) ) ;
#62544=CARTESIAN_POINT ( 'NONE',  ( 152.7370761390478719, 273.3427822079428324, -11.76210696558454494 ) ) ;
#62545=CARTESIAN_POINT ( 'NONE',  ( 182.5577216196124368, 260.8327824712812344, -10.71828994691334991 ) ) ;
#62546=CARTESIAN_POINT ( 'NONE',  ( -15.46727382606978374, 168.0024278399160664, -9.188101187500093303 ) ) ;
#62548=CARTESIAN_POINT ( 'NONE',  ( 155.4812142336614329, 261.3456326552338282, 18.45193178807985745 ) ) ;
#62549=CARTESIAN_POINT ( 'NONE',  ( 161.8839333999304415, 250.2557977526613229, -13.90128376743482441 ) ) ;
#62550=CARTESIAN_POINT ( 'NONE',  ( 186.2937303235093509, 283.1136418602877143, 16.27610940549458363 ) ) ;
#62551=CARTESIAN_POINT ( 'NONE',  ( 194.6356465353167948, 293.5281665672507643, -16.13180903283129197 ) ) ;
#62552=CARTESIAN_POINT ( 'NONE',  ( 188.2775767336528077, 300.0131076322000467, 1.527577962863595928 ) ) ;
#62553=CARTESIAN_POINT ( 'NONE',  ( 168.6822647293072919, 279.1257522418852659, 15.04337825401500872 ) ) ;
#62554=CARTESIAN_POINT ( 'NONE',  ( 192.9401904040553575, 264.5424255672033382, 8.944766451130574225 ) ) ;
#62555=CARTESIAN_POINT ( 'NONE',  ( 191.0862225170008628, 299.6759493045793192, -9.402218231374108726 ) ) ;
#62556=CARTESIAN_POINT ( 'NONE',  ( 189.8123550829396891, 301.8823524224806647, -0.5679054518196169354 ) ) ;
#62557=CARTESIAN_POINT ( 'NONE',  ( 152.8593402092683959, 275.2840601128194749, 10.96293945604634068 ) ) ;
#62558=ORIENTED_EDGE ( 'NONE', *, *, #20338, .T. ) ;
#62561=CARTESIAN_POINT ( 'NONE',  ( 117.8198823448352499, 229.6423013555409796, -4.594050593750043987 ) ) ;
#62563=CARTESIAN_POINT ( 'NONE',  ( 191.5694344253287511, 298.8390017285333897, 8.250976118904059575 ) ) ;
#62565=CARTESIAN_POINT ( 'NONE',  ( 196.0727848089514964, 291.0389700598140621, 17.56388901715066808 ) ) ;
#62566=CARTESIAN_POINT ( 'NONE',  ( 195.4573685308723725, 278.6848871218847989, 16.36961590483237927 ) ) ;
#62567=CARTESIAN_POINT ( 'NONE',  ( 150.9461593943442494, 269.2005780520424878, -15.05333791105169183 ) ) ;
#62568=CARTESIAN_POINT ( 'NONE',  ( 192.8878213245067741, 263.8246972048095245, -4.383899104128338386 ) ) ;
#62573=CARTESIAN_POINT ( 'NONE',  ( 192.4172326059820648, 297.3705722050773943, -12.52563289807247848 ) ) ;
#62575=ORIENTED_EDGE ( 'NONE', *, *, #67570, .F. ) ;
#62576=CARTESIAN_POINT ( 'NONE',  ( 192.2904205063093457, 267.0998989569302466, 11.00927096432294405 ) ) ;
#62577=CARTESIAN_POINT ( 'NONE',  ( 178.5783945668096635, 280.6919621351586898, 16.55962231343580982 ) ) ;
#62579=CARTESIAN_POINT ( 'NONE',  ( 198.5628662595931928, 269.3592121023095274, 9.255750010703465591 ) ) ;
#62581=B_SPLINE_CURVE_WITH_KNOTS ( 'NONE', 3,
 ( #68578, #38674, #54872, #7275 ),
 .UNSPECIFIED., .F., .F.,
 ( 4, 4 ),
 ( 0.000000000000000000, 0.0004986248048571736676 ),
 .UNSPECIFIED. ) ;
#62584=CARTESIAN_POINT ( 'NONE',  ( 179.9482942753538737, 262.6328355063881190, -12.71399655598229472 ) ) ;
#62585=EDGE_CURVE ( 'NONE', #27498, #32613, #48232, .T. ) ;
#62587=CARTESIAN_POINT ( 'NONE',  ( 149.9888573361949398, 250.7365022471902023, -10.00000000000009059 ) ) ;
#62589=( BOUNDED_CURVE ( )  B_SPLINE_CURVE ( 2, ( #70983, #69461, #32468, #9168, #8663, #54235, #55241, #85205, #93809 ),
 .UNSPECIFIED., .F., .T. ) 
 B_SPLINE_CURVE_WITH_KNOTS ( ( 3, 2, 2, 2, 3 ),
 ( 0.2056451612903225923, 0.2069892473118279674, 0.2096774193548387177, 0.2123655913978494680, 0.2137096774193548432 ),
 .UNSPECIFIED. ) 
 CURVE ( )  GEOMETRIC_REPRESENTATION_ITEM ( )  RATIONAL_B_SPLINE_CURVE ( ( 0.9330127018922194093, 0.9330127018922194093, 1.000000000000000000, 0.8660254037844387076, 1.000000000000000000, 0.8660254037844387076, 1.000000000000000000, 0.9330127018922194093, 0.9330127018922194093 ) ) 
 REPRESENTATION_ITEM ( '' )  );
#62592=AXIS2_PLACEMENT_3D ( 'NONE', #5891, #90545, #35291 ) ;
#62595=CARTESIAN_POINT ( 'NONE',  ( 167.6412282369280433, 249.8708500537493933, 6.876476337372752212 ) ) ;
#62596=EDGE_CURVE ( 'NONE', #74262, #44920, #76066, .T. ) ;
#62599=ORIENTED_EDGE ( 'NONE', *, *, #69580, .F. ) ;
#62601=CARTESIAN_POINT ( 'NONE',  ( 159.1291222501505445, 255.0272706293370106, 16.74886675395809021 ) ) ;
#62602=CARTESIAN_POINT ( 'NONE',  ( 192.5550983588679514, 297.1317817164552935, -12.35927356157043278 ) ) ;
#62606=CARTESIAN_POINT ( 'NONE',  ( 203.1705638993064156, 278.7452560544191442, -15.08126533799095093 ) ) ;
#62607=VERTEX_POINT ( 'NONE', #98749 ) ;
#62609=CARTESIAN_POINT ( 'NONE',  ( 175.1299035677911036, 258.4933098028565155, 12.91181667424501711 ) ) ;
#62610=ORIENTED_EDGE ( 'NONE', *, *, #62050, .T. ) ;
#62612=ORIENTED_EDGE ( 'NONE', *, *, #20214, .F. ) ;
#62613=CARTESIAN_POINT ( 'NONE',  ( 162.7505971618529088, 252.7026393492068905, 14.43551447597413961 ) ) ;
#62614=CARTESIAN_POINT ( 'NONE',  ( 203.5477091018662748, 278.0920214017542662, -16.09930363698006062 ) ) ;
#62617=CARTESIAN_POINT ( 'NONE',  ( 206.1670584421323724, 273.5551752616418639, -11.23038754588519694 ) ) ;
#62618=CARTESIAN_POINT ( 'NONE',  ( 147.9200371497832123, 274.4419755295365917, -6.891776270191406262 ) ) ;
#62619=FACE_OUTER_BOUND ( 'NONE', #9559, .T. ) ;
#62621=CARTESIAN_POINT ( 'NONE',  ( 190.1758200331204876, 279.2204749713225169, -17.78067544974210890 ) ) ;
#62622=CARTESIAN_POINT ( 'NONE',  ( 55.54027346828191725, 191.3262482093457777, 3.021315404115420679E-15 ) ) ;
#62623=CARTESIAN_POINT ( 'NONE',  ( 156.1956445759811345, 280.1375863634569328, 2.096082644243150384 ) ) ;
#62624=CARTESIAN_POINT ( 'NONE',  ( 118.6312605172356598, 248.4869531367911293, 4.594050593750046652 ) ) ;
#62625=CARTESIAN_POINT ( 'NONE',  ( 187.1031252671867833, 262.0538351896231575, -10.23227223353319992 ) ) ;
#62629=CARTESIAN_POINT ( 'NONE',  ( 203.6365213803127574, 276.2628368528385749, 13.36267271551829339 ) ) ;
#62631=CARTESIAN_POINT ( 'NONE',  ( 170.9811431790156462, 280.9458665424763240, 14.82329785628973440 ) ) ;
#62637=CARTESIAN_POINT ( 'NONE',  ( 173.5810627320022945, 281.9567074468304213, 15.04350262901273361 ) ) ;
#62639=VERTEX_POINT ( 'NONE', #19747 ) ;
#62640=CARTESIAN_POINT ( 'NONE',  ( 148.3025927079438304, 273.7793698660844939, -8.046026357031887954 ) ) ;
#62641=CARTESIAN_POINT ( 'NONE',  ( 12.62566161797914077, 166.5494855054052152, -2.679491924311248496 ) ) ;
#62642=VERTEX_POINT ( 'NONE', #67314 ) ;
#62643=EDGE_CURVE ( 'NONE', #54972, #49538, #33718, .T. ) ;
#62644=CARTESIAN_POINT ( 'NONE',  ( 188.0677593861371122, 266.1968029486987461, -11.81955941906698726 ) ) ;
#62645=EDGE_CURVE ( 'NONE', #3137, #9601, #7125, .T. ) ;
#62646=EDGE_CURVE ( 'NONE', #91958, #9648, #19198, .T. ) ;
#62647=CARTESIAN_POINT ( 'NONE',  ( 160.1665334620766430, 278.8148693431429592, 10.49729549887374525 ) ) ;
#62648=CARTESIAN_POINT ( 'NONE',  ( 152.5070194032087727, 266.4970892131865980, -16.37820007917167686 ) ) ;
#62649=FACE_OUTER_BOUND ( 'NONE', #51932, .T. ) ;
#62650=AXIS2_PLACEMENT_3D ( 'NONE', #22586, #36784, #59571 ) ;
#62652=CARTESIAN_POINT ( 'NONE',  ( 163.4583656713151356, 282.7452325144295742, -6.635438818464283628 ) ) ;
#62653=CARTESIAN_POINT ( 'NONE',  ( 160.6618029133832408, 282.0177171234115576, 6.619462234459586369 ) ) ;
#62654=CARTESIAN_POINT ( 'NONE',  ( 153.1627746953036535, 265.3612877299463548, -17.72069958822647351 ) ) ;
#62655=ORIENTED_EDGE ( 'NONE', *, *, #84547, .T. ) ;
#62657=CARTESIAN_POINT ( 'NONE',  ( 146.8881680668833951, 276.2292252078784145, 4.973452195244782104 ) ) ;
#62660=CARTESIAN_POINT ( 'NONE',  ( 191.0481485323713571, 274.9721303180398877, -15.73758095991607853 ) ) ;
#62662=CARTESIAN_POINT ( 'NONE',  ( 188.5479317267626698, 298.6910045167662133, -3.988169708390922885 ) ) ;
#62663=CARTESIAN_POINT ( 'NONE',  ( 204.1633547645365638, 275.3510256380408237, 13.36249479004741580 ) ) ;
#62668=CARTESIAN_POINT ( 'NONE',  ( -2.639098984630277922, 169.2833772461660828, -9.188101187500095079 ) ) ;
#62669=CARTESIAN_POINT ( 'NONE',  ( 96.71051312758956442, 217.4548013555409511, -4.594050593750042211 ) ) ;
#62671=CARTESIAN_POINT ( 'NONE',  ( 147.1034852426517148, 275.8562849197056153, -3.648177088342072327 ) ) ;
#62673=CARTESIAN_POINT ( 'NONE',  ( -27.42236680055714260, 166.5217562850347406, 1.224646799147364892E-15 ) ) ;
#62677=CARTESIAN_POINT ( 'NONE',  ( 160.8600223638921705, 264.2357221146763777, 17.82164827449318523 ) ) ;
#62680=CARTESIAN_POINT ( 'NONE',  ( 179.0414368791381321, 290.1589939638860187, 9.426711296681993701 ) ) ;
#62681=CARTESIAN_POINT ( 'NONE',  ( 165.9936732699065658, 249.2531922495258812, -9.278618579411492817 ) ) ;
#62682=CARTESIAN_POINT ( 'NONE',  ( 205.5916367843585135, 274.5518348086813489, -12.90939787341577372 ) ) ;
#62683=CARTESIAN_POINT ( 'NONE',  ( 196.3021893095863959, 290.6416298092292436, 17.45656988653421138 ) ) ;
#62684=DIRECTION ( 'NONE',  ( -0.8660254037844387076, -0.4999999999999998890, -0.000000000000000000 ) ) ;
#62685=CARTESIAN_POINT ( 'NONE',  ( 207.7666684749232786, 270.7845694125510931, -6.630926507062123498 ) ) ;
#62686=CARTESIAN_POINT ( 'NONE',  ( 34.27488675591641965, 202.8464784336661353, 1.353441290958777327E-15 ) ) ;
#62688=CARTESIAN_POINT ( 'NONE',  ( 62.31280629920263436, 206.7833772461660828, -9.188101187500095079 ) ) ;
#62692=CARTESIAN_POINT ( 'NONE',  ( -17.22621437785049636, 170.8615022471903160, 5.000000000000046185 ) ) ;
#62694=CARTESIAN_POINT ( 'NONE',  ( 14.08495376150009371, 190.4860189848785126, -2.679491924311252493 ) ) ;
#62695=EDGE_CURVE ( 'NONE', #84442, #62377, #37274, .T. ) ;
#62697=CARTESIAN_POINT ( 'NONE',  ( 198.5970767652345899, 286.6667681383942181, -17.17073100918929640 ) ) ;
#62698=CARTESIAN_POINT ( 'NONE',  ( 196.4501996009505831, 290.3852684645433442, -17.82325615854289680 ) ) ;
#62700=CARTESIAN_POINT ( 'NONE',  ( 68.75404378773188796, 204.3768266524160140, 9.188101187500096856 ) ) ;
#62703=CARTESIAN_POINT ( 'NONE',  ( 159.6610344727618269, 254.1059716346071866, 15.33388637456589620 ) ) ;
#62707=CARTESIAN_POINT ( 'NONE',  ( 117.0077232087375734, 228.3615022471901739, 5.000000000000051514 ) ) ;
#62708=CARTESIAN_POINT ( 'NONE',  ( 200.6129772034685175, 283.1751261563724142, 18.36811917402039640 ) ) ;
#62709=CARTESIAN_POINT ( 'NONE',  ( 207.3502731283117555, 271.5057873089173768, 6.280625384230454245 ) ) ;
#62713=CARTESIAN_POINT ( 'NONE',  ( 184.8664429911153206, 271.3566499112901624, 16.06020675104017670 ) ) ;
#62714=ORIENTED_EDGE ( 'NONE', *, *, #22537, .F. ) ;
#62715=CARTESIAN_POINT ( 'NONE',  ( 206.3454060440500086, 273.2462681537123785, -9.268083217908118954 ) ) ;
#62716=CARTESIAN_POINT ( 'NONE',  ( 187.6832578813660177, 277.1412041823390382, -16.69151914137464487 ) ) ;
#62720=CARTESIAN_POINT ( 'NONE',  ( 175.5613651706662210, 252.8860800517080918, -0.2536904810274192013 ) ) ;
#62721=ORIENTED_EDGE ( 'NONE', *, *, #52257, .T. ) ;
#62723=CARTESIAN_POINT ( 'NONE',  ( 148.2670916631250861, 273.8408594794321971, -7.980554973576580835 ) ) ;
#62724=CARTESIAN_POINT ( 'NONE',  ( 206.9413969004818057, 271.3616952779818234, -5.376728341096632668 ) ) ;
#62725=AXIS2_PLACEMENT_3D ( 'NONE', #88290, #57813, #18346 ) ;
#62726=ORIENTED_EDGE ( 'NONE', *, *, #96617, .F. ) ;
#62728=CARTESIAN_POINT ( 'NONE',  ( 202.5650245025327081, 277.7940810556053179, -15.59262966521933791 ) ) ;
#62734=CARTESIAN_POINT ( 'NONE',  ( -10.89340361622470610, 174.5177522451419350, 5.000000000000046185 ) ) ;
#62737=AXIS2_PLACEMENT_3D ( 'NONE', #42784, #51912, #4301 ) ;
#62741=CARTESIAN_POINT ( 'NONE',  ( 193.9401685343300699, 294.7327698005063326, 14.01047396938887069 ) ) ;
#62742=CARTESIAN_POINT ( 'NONE',  ( 185.1491161497484370, 292.9437783688060222, -11.97406807593424993 ) ) ;
#62743=CARTESIAN_POINT ( 'NONE',  ( 157.3029956111992362, 258.1902147490555421, -18.22269824972649843 ) ) ;
#62744=CARTESIAN_POINT ( 'NONE',  ( 141.5541307454787727, 252.5333772461660260, 9.188101187500095079 ) ) ;
#62745=CARTESIAN_POINT ( 'NONE',  ( 162.7006039569504594, 261.3497057169571463, 17.57720365097131676 ) ) ;
#62747=CARTESIAN_POINT ( 'NONE',  ( 179.7049408000989956, 258.9102790531361507, 9.610927518812550474 ) ) ;
#62748=CARTESIAN_POINT ( 'NONE',  ( 80.71549903385694336, 229.6589784336661637, -6.496448406907675876E-16 ) ) ;
#62750=CARTESIAN_POINT ( 'NONE',  ( 190.7779368023172708, 300.2099158256590385, 8.142228434510803581 ) ) ;
#62752=ORIENTED_EDGE ( 'NONE', *, *, #88375, .F. ) ;
#62753=CARTESIAN_POINT ( 'NONE',  ( 195.4107521409361539, 292.1856442770869080, -15.96705206423837353 ) ) ;
#62756=EDGE_CURVE ( 'NONE', #86705, #55644, #2277, .T. ) ;
#62758=CARTESIAN_POINT ( 'NONE',  ( 81.57285043722427531, 211.2365022471902023, 10.00000000000009948 ) ) ;
#62759=CARTESIAN_POINT ( 'NONE',  ( 191.6823192895500370, 298.6434794082964572, -8.424208857102787107 ) ) ;
#62762=CARTESIAN_POINT ( 'NONE',  ( 156.0507216674837707, 279.5060275253360373, 7.618106348741741307 ) ) ;
#62763=CARTESIAN_POINT ( 'NONE',  ( 78.84873917453550973, 207.1423013555409796, -4.594050593750043987 ) ) ;
#62768=CARTESIAN_POINT ( 'NONE',  ( 161.7519069501884132, 250.4844742715573886, -14.24248196453219073 ) ) ;
#62772=EDGE_CURVE ( 'NONE', #68451, #49174, #90636, .T. ) ;
#62773=CARTESIAN_POINT ( 'NONE',  ( 183.8966011539753254, 275.3119708187981018, 16.41707298570698725 ) ) ;
#62775=CARTESIAN_POINT ( 'NONE',  ( 161.6130071796497418, 284.2796802195229020, 0.5328386277561626416 ) ) ;
#62778=ORIENTED_EDGE ( 'NONE', *, *, #47417, .T. ) ;
#62782=CARTESIAN_POINT ( 'NONE',  ( 159.6962080797732710, 254.0450491601782232, -15.33973334987084947 ) ) ;
#62785=DIRECTION ( 'NONE',  ( 0.4999999999999992784, -0.8660254037844390407, 0.000000000000000000 ) ) ;
#62787=CARTESIAN_POINT ( 'NONE',  ( 111.2365322456207224, 223.4824982072973683, 3.021315404115420679E-15 ) ) ;
#62790=CARTESIAN_POINT ( 'NONE',  ( 189.7493380202622291, 294.8126471784881915, -12.68491631734921299 ) ) ;
#62791=CARTESIAN_POINT ( 'NONE',  ( 200.1103929410127762, 284.0456276340304953, 17.67835211026828901 ) ) ;
#62793=VECTOR ( 'NONE', #89061, 1000.000000000000000 ) ;
#62794=CARTESIAN_POINT ( 'NONE',  ( 169.4846735095618442, 250.9656555291483357, 6.963129758109078082 ) ) ;
#62796=CARTESIAN_POINT ( 'NONE',  ( 155.8025440274901428, 271.6998552528711457, 14.08447433373405921 ) ) ;
#62801=CARTESIAN_POINT ( 'NONE',  ( 207.6900289502458179, 270.9173129631602706, 7.178327969100043227 ) ) ;
#62802=CARTESIAN_POINT ( 'NONE',  ( 155.3017250444513024, 261.6565170503553190, 18.58368563027307374 ) ) ;
#62804=CARTESIAN_POINT ( 'NONE',  ( 199.1275226280280890, 281.8858470971437100, -16.59877271873514459 ) ) ;
#62806=CARTESIAN_POINT ( 'NONE',  ( 165.8896735243662306, 286.5189455822670652, -3.328331710570921143 ) ) ;
#62808=CARTESIAN_POINT ( 'NONE',  ( 163.8003088823192286, 260.8948240748503054, -17.39314492925268141 ) ) ;
#62809=CARTESIAN_POINT ( 'NONE',  ( 195.1808244021223686, 265.5951289396304560, -7.339755448317591302 ) ) ;
#62811=CARTESIAN_POINT ( 'NONE',  ( -8.782727014549898570, 174.9244531367911293, -4.594050593750046652 ) ) ;
#62812=CARTESIAN_POINT ( 'NONE',  ( 73.95673202641080479, 225.0530062829863311, -4.648177544792955347E-16 ) ) ;
#62814=AXIS2_PLACEMENT_3D ( 'NONE', #31109, #32111, #79276 ) ;
#62815=CARTESIAN_POINT ( 'NONE',  ( 178.1796287192598527, 256.8239042684534184, 8.391128143578042042 ) ) ;
#62816=DIRECTION ( 'NONE',  ( 0.8660254037844387076, 0.4999999999999998890, 0.000000000000000000 ) ) ;
#62817=CARTESIAN_POINT ( 'NONE',  ( 182.0442112598040580, 290.9601537038038259, 12.16457704577017829 ) ) ;
#62818=CARTESIAN_POINT ( 'NONE',  ( 23.53136650780448491, 175.2048013555409796, 4.594050593750051981 ) ) ;
#62819=CARTESIAN_POINT ( 'NONE',  ( 62.88113547221008304, 217.1115022471903160, -5.000000000000047962 ) ) ;
#62822=CARTESIAN_POINT ( 'NONE',  ( 146.7818291168261453, 276.4134096722012828, -0.7617065417431535534 ) ) ;
#62823=CARTESIAN_POINT ( 'NONE',  ( 135.3927208396967785, 255.6427522451419065, -10.00000000000009592 ) ) ;
#62824=B_SPLINE_SURFACE_WITH_KNOTS ( 'NONE', 3, 1, ( 
 ( #21112, #5396 ),
 ( #67179, #35788 ),
 ( #50482, #58091 ),
 ( #11519, #89073 ),
 ( #43378, #27203 ),
 ( #51484, #19122 ),
 ( #80953, #65682 ),
 ( #20603, #35288 ),
 ( #19624, #59057 ),
 ( #42864, #81436 ),
 ( #51990, #97139 ),
 ( #66684, #4390 ),
 ( #82452, #90541 ),
 ( #26697, #57582 ),
 ( #58575, #88556 ),
 ( #50978, #13015 ),
 ( #73308, #59566 ),
 ( #36280, #43874 ),
 ( #96638, #44374 ),
 ( #74817, #28185 ),
 ( #74322, #49996 ),
 ( #12006, #98103 ),
 ( #28682, #5887 ),
 ( #82929, #73798 ),
 ( #42375, #27707 ),
 ( #65193, #13505 ),
 ( #89548, #20109 ),
 ( #75306, #96139 ),
 ( #81931, #3899 ),
 ( #34780, #12507 ),
 ( #4905, #97618 ),
 ( #90028, #100098 ),
 ( #46871, #14489 ),
 ( #15969, #77795 ) ),
 .UNSPECIFIED., .T., .F., .F.,
 ( 4, 2, 2, 2, 2, 2, 2, 2, 2, 2, 2, 2, 2, 2, 2, 2, 4 ),
 ( 2, 2 ),
 ( 0.000000000000000000, 0.06250000000000000000, 0.1250000000000000000, 0.1875000000000000000, 0.2500000000000000000, 0.3125000000000000000, 0.3750000000000000000, 0.4375000000000000000, 0.5000000000000000000, 0.5625000000000000000, 0.6250000000000000000, 0.6875000000000000000, 0.7500000000000000000, 0.8125000000000000000, 0.8750000000000000000, 0.9375000000000000000, 1.000000000000000000 ),
 ( 0.000000000000000000, 1.000000000000000000 ),
 .UNSPECIFIED. ) ;
#62825=CARTESIAN_POINT ( 'NONE',  ( 186.6562845357111087, 296.1148510662804370, -8.718888755099150956 ) ) ;
#62826=CARTESIAN_POINT ( 'NONE',  ( 187.7495819260542476, 259.1541535816100463, -0.7945162718502817301 ) ) ;
#62827=CARTESIAN_POINT ( 'NONE',  ( 67.64427519302456915, 199.8615022471901739, 5.000000000000051514 ) ) ;
#62829=AXIS2_PLACEMENT_3D ( 'NONE', #84096, #14648, #68334 ) ;
#62830=CARTESIAN_POINT ( 'NONE',  ( 204.2047590417662093, 270.4847546024170697, 6.040547820020366387 ) ) ;
#62831=CARTESIAN_POINT ( 'NONE',  ( 39.55283647781661216, 184.4548013555409796, -4.594050593750042211 ) ) ;
#62835=CARTESIAN_POINT ( 'NONE',  ( 199.1216527653377000, 285.7581758537840528, -18.37739894744384728 ) ) ;
#62838=CARTESIAN_POINT ( 'NONE',  ( 194.1011995340913074, 294.4538559273262877, 13.93949783759920713 ) ) ;
#62840=CARTESIAN_POINT ( 'NONE',  ( 162.6725657724230700, 281.1335366253323400, -10.40723503984205500 ) ) ;
#62841=CARTESIAN_POINT ( 'NONE',  ( -17.42236680055705023, 149.2012482093457777, 0.000000000000000000 ) ) ;
#62843=CARTESIAN_POINT ( 'NONE',  ( 202.2576150004249200, 280.3265299319959354, 16.24828394350762295 ) ) ;
#62844=CARTESIAN_POINT ( 'NONE',  ( 196.7823306783968746, 289.8100005636337073, -17.85370042640856170 ) ) ;
#62845=CARTESIAN_POINT ( 'NONE',  ( 185.6575085028373451, 267.5770612294242596, -14.83682210475602581 ) ) ;
#62851=EDGE_CURVE ( 'NONE', #94448, #18147, #56316, .T. ) ;
#62852=ORIENTED_EDGE ( 'NONE', *, *, #61202, .T. ) ;
#62855=EDGE_CURVE ( 'NONE', #53789, #78498, #68566, .T. ) ;
#62856=CARTESIAN_POINT ( 'NONE',  ( 180.6644785651033658, 257.6587254813057370, -7.431609338059112169 ) ) ;
#62859=CARTESIAN_POINT ( 'NONE',  ( 189.7042809424692393, 274.2741113227406800, -15.67635319055484366 ) ) ;
#62862=CARTESIAN_POINT ( 'NONE',  ( 200.8665851640556070, 282.7358642834317948, -16.69422397739980823 ) ) ;
#62866=CARTESIAN_POINT ( 'NONE',  ( 185.2570508126727873, 282.0811717828997303, -17.42469797758589678 ) ) ;
#62867=CARTESIAN_POINT ( 'NONE',  ( 148.2267527339363369, 273.9107285543102535, 7.913369084260907016 ) ) ;
#62870=CARTESIAN_POINT ( 'NONE',  ( 184.0985169280008620, 289.0250432102490663, -13.04961936838414971 ) ) ;
#62871=ORIENTED_EDGE ( 'NONE', *, *, #41241, .F. ) ;
#62872=CARTESIAN_POINT ( 'NONE',  ( 195.8627871995700502, 291.4026965887302936, 17.41145040657729481 ) ) ;
#62874=CARTESIAN_POINT ( 'NONE',  ( 160.0114177933981523, 266.1051921132770417, 16.66372494280312111 ) ) ;
#62877=CYLINDRICAL_SURFACE ( 'NONE', #19673, 17.82106496071139645 ) ;
#62878=CARTESIAN_POINT ( 'NONE',  ( 153.6392919293977002, 266.5359356698173769, -16.75038546547492402 ) ) ;
#62879=CARTESIAN_POINT ( 'NONE',  ( 61.28457468009112574, 200.0643266524160140, 9.188101187500095079 ) ) ;
#62880=ORIENTED_EDGE ( 'NONE', *, *, #2424, .T. ) ;
#62883=FACE_OUTER_BOUND ( 'NONE', #55751, .T. ) ;
#62884=CARTESIAN_POINT ( 'NONE',  ( 175.7055711947306520, 272.7582102363617764, 17.70512484591946034 ) ) ;
#62887=( BOUNDED_CURVE ( )  B_SPLINE_CURVE ( 2, ( #67379, #26901, #91216, #30381, #52668, #67888, #68866, #84618, #83120 ),
 .UNSPECIFIED., .F., .F. ) 
 B_SPLINE_CURVE_WITH_KNOTS ( ( 3, 2, 2, 2, 3 ),
 ( 0.5604838709677418818, 0.5618279569892472569, 0.5645161290322581182, 0.5672043010752688685, 0.5685483870967742437 ),
 .UNSPECIFIED. ) 
 CURVE ( )  GEOMETRIC_REPRESENTATION_ITEM ( )  RATIONAL_B_SPLINE_CURVE ( ( 0.9330127018922194093, 0.9330127018922194093, 1.000000000000000000, 0.8660254037844387076, 1.000000000000000000, 0.8660254037844387076, 1.000000000000000000, 0.9330127018922194093, 0.9330127018922194093 ) ) 
 REPRESENTATION_ITEM ( '' )  );
#62889=CARTESIAN_POINT ( 'NONE',  ( 190.4456243223121987, 299.4994646951487880, 6.453196029206972995 ) ) ;
#62891=CARTESIAN_POINT ( 'NONE',  ( 172.6727388731993358, 285.6664956175675911, 12.05044444168489548 ) ) ;
#62893=CARTESIAN_POINT ( 'NONE',  ( 171.7219487607086990, 259.3602272249703447, -13.79533293788550985 ) ) ;
#62894=CARTESIAN_POINT ( 'NONE',  ( 140.8234218128096700, 242.1115022471902023, -5.000000000000041744 ) ) ;
#62895=CARTESIAN_POINT ( 'NONE',  ( 161.8807657183444064, 250.2612843381103573, -13.52770735624900311 ) ) ;
#62896=CARTESIAN_POINT ( 'NONE',  ( 192.5284579606305613, 297.1779242397361713, -13.15228012403107272 ) ) ;
#62898=EDGE_CURVE ( 'NONE', #97214, #55984, #69597, .T. ) ;
#62899=CARTESIAN_POINT ( 'NONE',  ( 190.0340467409721441, 301.4983712071542641, 4.077645795029533282 ) ) ;
#62900=CARTESIAN_POINT ( 'NONE',  ( 178.1116250315744196, 269.9460939148322041, 16.11468309730568294 ) ) ;
#62902=CARTESIAN_POINT ( 'NONE',  ( 206.3907062969896060, 273.1678058140250300, 11.56942460516550675 ) ) ;
#62905=CARTESIAN_POINT ( 'NONE',  ( 163.8398374448017591, 246.8680725722146008, -5.948785025486735378 ) ) ;
#62906=CARTESIAN_POINT ( 'NONE',  ( 116.3314879560220163, 225.7202760586659736, -5.415160957724236172E-17 ) ) ;
#62907=VERTEX_POINT ( 'NONE', #45268 ) ;
#62908=CARTESIAN_POINT ( 'NONE',  ( 146.6138605399200117, 276.7043397814778132, -0.5394499176159462950 ) ) ;
#62912=CARTESIAN_POINT ( 'NONE',  ( 202.8535267948003593, 279.2943804273081696, -15.36804658072946062 ) ) ;
#62913=CARTESIAN_POINT ( 'NONE',  ( 204.6780326111993986, 276.1342436545999703, 14.85609018352459287 ) ) ;
#62914=DIRECTION ( 'NONE',  ( 0.4999999999999998890, -0.8660254037844385966, 0.000000000000000000 ) ) ;
#62917=CARTESIAN_POINT ( 'NONE',  ( 207.7625791259561652, 270.7916523727319031, -1.015623356719550063 ) ) ;
#62919=CARTESIAN_POINT ( 'NONE',  ( 185.5294769923299327, 262.0336625405320206, 9.760107401958277862 ) ) ;
#62920=CARTESIAN_POINT ( 'NONE',  ( 165.0604371780248982, 244.7539318185670822, -1.421758703131883017 ) ) ;
#62921=CARTESIAN_POINT ( 'NONE',  ( 127.9681836757279001, 250.8149278399160949, 9.188101187500093303 ) ) ;
#62922=CARTESIAN_POINT ( 'NONE',  ( 198.5954523381739989, 286.6695817285962562, -18.45134152028667174 ) ) ;
#62923=CARTESIAN_POINT ( 'NONE',  ( 189.1621392246859443, 299.6514946570117104, 4.921827439568769336 ) ) ;
#62924=CARTESIAN_POINT ( 'NONE',  ( 196.4677418905696129, 290.3548843276421394, 17.08610552292358520 ) ) ;
#62926=CARTESIAN_POINT ( 'NONE',  ( 56.25097556847656932, 191.0327760586659451, 1.948934522072303157E-15 ) ) ;
#62928=VERTEX_POINT ( 'NONE', #44759 ) ;
#62932=CARTESIAN_POINT ( 'NONE',  ( 175.0809028706871118, 261.2525943152746208, 15.25527675994286092 ) ) ;
#62933=CARTESIAN_POINT ( 'NONE',  ( 151.2652836043610876, 278.4243225337131662, -1.677173973228833548 ) ) ;
#62935=CARTESIAN_POINT ( 'NONE',  ( 178.6782777294722848, 260.6412425082613709, 13.57969907341511551 ) ) ;
#62936=CARTESIAN_POINT ( 'NONE',  ( 122.4023397829302553, 228.1427522451417360, 1.119607411625061291E-15 ) ) ;
#62941=CARTESIAN_POINT ( 'NONE',  ( 147.8503508990560533, 274.5626756563852950, 7.845851077393495743 ) ) ;
#62944=CARTESIAN_POINT ( 'NONE',  ( 33.57176175898906934, 184.0643266524159856, -9.188101187500093303 ) ) ;
#62945=CIRCLE ( 'NONE', #79198, 17.82106496071138935 ) ;
#62950=CARTESIAN_POINT ( 'NONE',  ( 198.1618177255134015, 277.6368070017157947, -15.56499484391458843 ) ) ;
#62951=CARTESIAN_POINT ( 'NONE',  ( 69.21394623383595501, 200.7677522451417929, -5.000000000000041744 ) ) ;
#62953=CARTESIAN_POINT ( 'NONE',  ( 163.1794579292409253, 256.1406810980501518, -15.00038027609048363 ) ) ;
#62954=CARTESIAN_POINT ( 'NONE',  ( 205.4029933437358295, 274.8785748323546159, -13.50815392427034922 ) ) ;
#62955=CARTESIAN_POINT ( 'NONE',  ( 162.0223120223976423, 251.6753896847266958, -12.96689075600689911 ) ) ;
#62956=ORIENTED_EDGE ( 'NONE', *, *, #2424, .F. ) ;
#62957=B_SPLINE_CURVE_WITH_KNOTS ( 'NONE', 3,
 ( #87830, #16850, #78674, #33566, #12134, #63952, #4520, #25454, #47738, #41136, #93396, #72075, #42996, #73934, #86819, #79205, #35421, #23947, #9265, #16357, #39629, #1677, #70550, #40136, #1166, #32560, #63458, #24947, #55825, #9779, #51108, #28825, #67823, #14122, #75432, #98745, #91648, #67311, #45003, #5032, #58701, #97743, #13140, #53112, #12643, #43997, #27825, #37401, #6016, #74939, #59708, #66326 ),
 .UNSPECIFIED., .F., .F.,
 ( 4, 2, 2, 2, 2, 2, 2, 2, 2, 2, 2, 2, 2, 2, 2, 2, 2, 2, 2, 2, 2, 2, 2, 2, 2, 4 ),
 ( 9.655427817053376463E-05, 0.001108321745685109366, 0.001361263612563711704, 0.001614205479442313608, 0.001740676412881614777, 0.001867147346320915946, 0.001993618279760217115, 0.002120089213199518284, 0.002373031080078007431, 0.002625972946956497012, 0.003131856680713594569, 0.004143624148227681263, 0.005155391615741768824, 0.005661275349498765333, 0.005914217216377265322, 0.006040688149816550445, 0.006167159083255834701, 0.006230394549975405705, 0.006293630016694975841, 0.006420100950134061471, 0.006673042817012199771, 0.006925984683890338937, 0.007178926550768477237, 0.007431868417646616404, 0.007684810284524755571, 0.008190694018281138855 ),
 .UNSPECIFIED. ) ;
#62959=CARTESIAN_POINT ( 'NONE',  ( 22.61095419623372038, 183.8615022471902591, -10.00000000000009592 ) ) ;
#62960=CARTESIAN_POINT ( 'NONE',  ( 143.5566409438477820, 259.8149278399160949, 9.188101187500093303 ) ) ;
#62962=CARTESIAN_POINT ( 'NONE',  ( -9.188242552867592394, 159.3768266524160140, 9.188101187500098632 ) ) ;
#62964=CARTESIAN_POINT ( 'NONE',  ( 164.1063306464232596, 260.5560046979782669, -16.15882112840923668 ) ) ;
#62965=CARTESIAN_POINT ( 'NONE',  ( 169.3931091469603984, 263.1051856239939184, 15.88219003239466431 ) ) ;
#62966=CARTESIAN_POINT ( 'NONE',  ( 188.9967343574858489, 261.2041156289865285, 6.779708859182053793 ) ) ;
#62967=CARTESIAN_POINT ( 'NONE',  ( 164.2572333502590709, 246.1451216570909253, 2.155809084027023204 ) ) ;
#62969=CARTESIAN_POINT ( 'NONE',  ( 183.8752768387326171, 258.1900781452185356, -2.303537087110122616 ) ) ;
#62972=B_SPLINE_CURVE_WITH_KNOTS ( 'NONE', 3,
 ( #894, #62677, #31774, #78923 ),
 .UNSPECIFIED., .F., .F.,
 ( 4, 4 ),
 ( 0.002549164959714402164, 0.01048964830214099697 ),
 .UNSPECIFIED. ) ;
#62974=CARTESIAN_POINT ( 'NONE',  ( 178.4184685675666628, 285.5228835851044096, 12.97023324045351345 ) ) ;
#62975=CARTESIAN_POINT ( 'NONE',  ( 168.8231301974613530, 288.1409873211621857, 0.5233980140626269817 ) ) ;
#62978=CARTESIAN_POINT ( 'NONE',  ( 159.0854911330092420, 259.4224917152533294, 16.69341444665720076 ) ) ;
#62979=CARTESIAN_POINT ( 'NONE',  ( 159.5050723400634638, 254.3761059724978679, -15.34938048045353298 ) ) ;
#62980=CARTESIAN_POINT ( 'NONE',  ( 55.08690683815012790, 212.6115022471903444, -5.000000000000047962 ) ) ;
#62982=CARTESIAN_POINT ( 'NONE',  ( 192.1396999271463812, 297.8512729055811974, 12.32430960859512403 ) ) ;
#62983=DIRECTION ( 'NONE',  ( -0.8660254037844387076, -0.4999999999999998890, -0.000000000000000000 ) ) ;
#62984=CARTESIAN_POINT ( 'NONE',  ( 191.2827847134780654, 298.6246597018299553, 8.274781095337747416 ) ) ;
#62986=CARTESIAN_POINT ( 'NONE',  ( 208.3764315856425640, 269.7284287242038658, -1.833640725398759441 ) ) ;
#62987=CARTESIAN_POINT ( 'NONE',  ( 194.1011995340913074, 294.4538559273262877, 13.93949783759920713 ) ) ;
#62989=EDGE_CURVE ( 'NONE', #59756, #14425, #89597, .T. ) ;
#62990=ORIENTED_EDGE ( 'NONE', *, *, #52257, .F. ) ;
#62991=CARTESIAN_POINT ( 'NONE',  ( 131.6579862894242581, 253.4865022471902876, -10.00000000000009592 ) ) ;
#62993=VERTEX_POINT ( 'NONE', #78690 ) ;
#62996=B_SPLINE_CURVE_WITH_KNOTS ( 'NONE', 3,
 ( #404, #9001, #93133, #8018 ),
 .UNSPECIFIED., .F., .F.,
 ( 4, 4 ),
 ( 0.003861517607683099228, 0.009339119252991781930 ),
 .UNSPECIFIED. ) ;
#62997=VERTEX_POINT ( 'NONE', #94908 ) ;
#62998=CARTESIAN_POINT ( 'NONE',  ( 162.7752149807717785, 250.7913148208739074, -13.06579887205573165 ) ) ;
#63000=FACE_OUTER_BOUND ( 'NONE', #60137, .T. ) ;
#63003=CARTESIAN_POINT ( 'NONE',  ( 200.3134965941964651, 283.6938417875134064, 18.29802468362849766 ) ) ;
#63004=CARTESIAN_POINT ( 'NONE',  ( 151.0715479399129606, 268.9833987204304435, 14.24612252017116987 ) ) ;
#63005=CARTESIAN_POINT ( 'NONE',  ( 151.2990042328006552, 274.9136309945131416, -8.631800923121661029 ) ) ;
#63007=VERTEX_POINT ( 'NONE', #8773 ) ;
#63008=ORIENTED_EDGE ( 'NONE', *, *, #54624, .T. ) ;
#63011=ORIENTED_EDGE ( 'NONE', *, *, #33774, .F. ) ;
#63014=CARTESIAN_POINT ( 'NONE',  ( 208.2764314485352770, 269.9016340424377063, 2.433736665191914117 ) ) ;
#63018=CARTESIAN_POINT ( 'NONE',  ( 147.6054094044680198, 274.9869267698931594, -8.596541856229405809 ) ) ;
#63024=CARTESIAN_POINT ( 'NONE',  ( 198.7255116566313404, 276.6639372973349964, -15.44186690118796790 ) ) ;
#63025=CARTESIAN_POINT ( 'NONE',  ( 205.7829192689729325, 274.2205238267313234, 11.21202327925415254 ) ) ;
#63027=CARTESIAN_POINT ( 'NONE',  ( 198.1300353965528984, 287.4757075181870505, 18.48278456664528946 ) ) ;
#63030=CARTESIAN_POINT ( 'NONE',  ( 168.2217537332210782, 256.9393902984222109, -14.62648326016065425 ) ) ;
#63031=CARTESIAN_POINT ( 'NONE',  ( 206.2313482792274328, 273.4438219973828268, -9.403385562213845361 ) ) ;
#63032=CARTESIAN_POINT ( 'NONE',  ( 137.7719789713245291, 261.8967562850346553, -4.648177544792955347E-16 ) ) ;
#63033=B_SPLINE_CURVE_WITH_KNOTS ( 'NONE', 3,
 ( #27265, #97194, #26266, #11079, #58148, #97679, #11577, #95718, #58633, #81498 ),
 .UNSPECIFIED., .F., .F.,
 ( 4, 2, 2, 2, 4 ),
 ( 0.001426788465073381296, 0.001827427548930433184, 0.002228066632787485506, 0.002628705716644537393, 0.003029344800501589281 ),
 .UNSPECIFIED. ) ;
#63034=CARTESIAN_POINT ( 'NONE',  ( 161.8289209813647176, 250.3510820566641257, 13.28523796267037937 ) ) ;
#63035=CARTESIAN_POINT ( 'NONE',  ( 191.3965809556215731, 262.3234640945070737, -0.7488543785338046543 ) ) ;
#63036=VECTOR ( 'NONE', #53987, 1000.000000000000227 ) ;
#63038=DIRECTION ( 'NONE',  ( 0.4999999999999998890, -0.8660254037844385966, 0.000000000000000000 ) ) ;
#63039=CARTESIAN_POINT ( 'NONE',  ( 153.4232513496498598, 270.1086993216917449, 15.21047082690287588 ) ) ;
#63041=CARTESIAN_POINT ( 'NONE',  ( 15.95338390109293059, 180.0177522451418497, -10.00000000000009592 ) ) ;
#63042=CARTESIAN_POINT ( 'NONE',  ( 89.53865347855843027, 216.3768266524160140, 9.188101187500096856 ) ) ;
#63046=CARTESIAN_POINT ( 'NONE',  ( 167.7942470979873235, 278.7647128809718993, -13.37312110774118068 ) ) ;
#63047=EDGE_CURVE ( 'NONE', #81989, #38189, #49804, .T. ) ;
#63048=CARTESIAN_POINT ( 'NONE',  ( -1.935626891937928917, 175.8149278399160664, 9.188101187500093303 ) ) ;
#63051=CARTESIAN_POINT ( 'NONE',  ( 188.9177621428281952, 297.3148466342770462, 9.216719020081887592 ) ) ;
#63053=ORIENTED_EDGE ( 'NONE', *, *, #60741, .T. ) ;
#63055=CARTESIAN_POINT ( 'NONE',  ( 188.9943711983743242, 261.4777017766879794, -6.044221521033104061 ) ) ;
#63059=CARTESIAN_POINT ( 'NONE',  ( 207.1770866921659717, 271.8057550155037347, -5.569195235244989384 ) ) ;
#63060=CARTESIAN_POINT ( 'NONE',  ( 185.2008289883677321, 286.4076746189350615, 16.12297053898278421 ) ) ;
#63062=CARTESIAN_POINT ( 'NONE',  ( 34.68144358152915174, 181.6423013555409796, -4.594050593750043987 ) ) ;
#63063=CARTESIAN_POINT ( 'NONE',  ( 78.37938175722123901, 209.3927522451418213, -10.00000000000009059 ) ) ;
#63065=VERTEX_POINT ( 'NONE', #63472 ) ;
#63067=CARTESIAN_POINT ( 'NONE',  ( 182.0886690003881370, 260.7994180317198811, -10.55243971876994635 ) ) ;
#63068=CARTESIAN_POINT ( 'NONE',  ( 195.7578697689113199, 291.5844189092309193, 17.18796537138345215 ) ) ;
#63070=CARTESIAN_POINT ( 'NONE',  ( 207.2683629543511756, 271.6476598918739001, -6.694388351944108528 ) ) ;
#63071=CARTESIAN_POINT ( 'NONE',  ( 186.6830932896762931, 282.6891639578413447, 16.18349308428762257 ) ) ;
#63073=CARTESIAN_POINT ( 'NONE',  ( 189.7132495166375747, 263.2796367915959195, 7.902202450138100964 ) ) ;
#63074=CARTESIAN_POINT ( 'NONE',  ( 163.8990931530087494, 246.7654386749614162, 5.873176884778091633 ) ) ;
#63076=CARTESIAN_POINT ( 'NONE',  ( 146.7373254022577100, 276.4904923669593586, -0.7242168585908188572 ) ) ;
#63077=CARTESIAN_POINT ( 'NONE',  ( 189.9052851100924215, 301.7213928939034986, -1.077181946533001256 ) ) ;
#63079=CARTESIAN_POINT ( 'NONE',  ( 207.0624025450594843, 270.0043937851150417, -2.644299678167422840 ) ) ;
#63080=CARTESIAN_POINT ( 'NONE',  ( 207.5792673731680793, 271.1091576421853233, 2.359198794924813214 ) ) ;
#63081=CARTESIAN_POINT ( 'NONE',  ( 181.2378726859789140, 268.0551774814318833, 15.16452475098612140 ) ) ;
#63082=CARTESIAN_POINT ( 'NONE',  ( 107.5083335113205578, 239.0024278399160949, 9.188101187500095079 ) ) ;
#63085=CARTESIAN_POINT ( 'NONE',  ( 157.7529601300917363, 257.4108533407307959, 16.91445305439664892 ) ) ;
#63087=CARTESIAN_POINT ( 'NONE',  ( 152.8894687064977234, 278.3516875449029158, -6.243347624783317507 ) ) ;
#63089=CARTESIAN_POINT ( 'NONE',  ( 196.9098758191317700, 289.5890858996224324, -16.54412079817003800 ) ) ;
#63090=CARTESIAN_POINT ( 'NONE',  ( 161.3261849411383650, 273.2032229615781489, 15.91718547624222957 ) ) ;
#63091=CARTESIAN_POINT ( 'NONE',  ( 146.9129474150286683, 276.1863061179126930, -5.016087650759920358 ) ) ;
#63094=CARTESIAN_POINT ( 'NONE',  ( 189.5250749145859857, 265.8481487713520437, 10.75668547210380410 ) ) ;
#63096=CARTESIAN_POINT ( 'NONE',  ( 157.7498836780145268, 278.8187344995880039, 10.12965930615278509 ) ) ;
#63098=ADVANCED_FACE ( 'NONE', ( #63965 ), #59469, .F. ) ;
#63100=CARTESIAN_POINT ( 'NONE',  ( 182.3161647400480092, 256.3089014165817616, 4.988711622375854304 ) ) ;
#63101=EDGE_CURVE ( 'NONE', #28370, #62030, #42645, .T. ) ;
#63104=CARTESIAN_POINT ( 'NONE',  ( 148.1575212202267551, 275.3167594263540536, 5.922338269673835143 ) ) ;
#63106=CARTESIAN_POINT ( 'NONE',  ( 190.4441833906855379, 280.6464714971045282, 16.63408401792300495 ) ) ;
#63107=B_SPLINE_SURFACE_WITH_KNOTS ( 'NONE', 3, 1, ( 
 ( #70576, #63484 ),
 ( #62982, #78198 ),
 ( #31567, #8784 ),
 ( #54357, #1192 ),
 ( #41167, #93927 ),
 ( #47764, #32070 ),
 ( #23466, #78702 ),
 ( #94924, #25485 ),
 ( #40164, #15874 ),
 ( #46786, #56376 ),
 ( #24977, #79733 ),
 ( #55853, #86848 ),
 ( #17381, #10294 ),
 ( #72104, #31072 ),
 ( #77706, #8291 ),
 ( #39156, #81229 ),
 ( #81720, #74096 ),
 ( #4689, #35581 ),
 ( #50769, #57877 ),
 ( #3702, #26991 ),
 ( #43155, #51264 ),
 ( #66476, #26496 ),
 ( #33595, #97402 ),
 ( #27499, #64490 ),
 ( #58849, #34102 ),
 ( #41672, #12296 ),
 ( #20394, #73594 ),
 ( #95451, #19898 ),
 ( #96427, #26003 ),
 ( #88348, #10799 ),
 ( #50276, #82230 ),
 ( #11804, #57375 ),
 ( #27970, #3219 ),
 ( #88855, #73109 ) ),
 .UNSPECIFIED., .T., .F., .F.,
 ( 4, 2, 2, 2, 2, 2, 2, 2, 2, 2, 2, 2, 2, 2, 2, 2, 4 ),
 ( 2, 2 ),
 ( 0.000000000000000000, 0.06250000000000000000, 0.1250000000000000000, 0.1875000000000000000, 0.2500000000000000000, 0.3125000000000000000, 0.3750000000000000000, 0.4375000000000000000, 0.5000000000000000000, 0.5625000000000000000, 0.6250000000000000000, 0.6875000000000000000, 0.7500000000000000000, 0.8125000000000000000, 0.8750000000000000000, 0.9375000000000000000, 1.000000000000000000 ),
 ( 0.000000000000000000, 1.000000000000000000 ),
 .UNSPECIFIED. ) ;
#63108=EDGE_CURVE ( 'NONE', #35157, #64789, #30059, .T. ) ;
#63110=CARTESIAN_POINT ( 'NONE',  ( 177.2690896250785215, 274.8578734701023905, -17.19570748498711765 ) ) ;
#63111=ORIENTED_EDGE ( 'NONE', *, *, #4915, .F. ) ;
#63116=EDGE_LOOP ( 'NONE', ( #54335, #12797, #25353 ) ) ;
#63118=CARTESIAN_POINT ( 'NONE',  ( 166.6173964342836484, 252.1147280582555084, 12.30655765920312028 ) ) ;
#63124=ORIENTED_EDGE ( 'NONE', *, *, #97668, .F. ) ;
#63125=ORIENTED_EDGE ( 'NONE', *, *, #91497, .F. ) ;
#63126=CARTESIAN_POINT ( 'NONE',  ( 175.0450529704226028, 258.5646980256989309, 12.79576524686047634 ) ) ;
#63127=ORIENTED_EDGE ( 'NONE', *, *, #75286, .T. ) ;
#63132=ORIENTED_EDGE ( 'NONE', *, *, #62081, .F. ) ;
#63133=CARTESIAN_POINT ( 'NONE',  ( 205.9281787291064347, 273.9689270615001533, -10.62323193457751458 ) ) ;
#63134=CARTESIAN_POINT ( 'NONE',  ( 147.1831281302520154, 275.7183393919203809, -6.957138126403704881 ) ) ;
#63135=CARTESIAN_POINT ( 'NONE',  ( 196.2063030037021747, 284.5084424747770413, -17.41934349069538257 ) ) ;
#63137=CARTESIAN_POINT ( 'NONE',  ( 167.6597423760104846, 249.1366150583754404, -5.304815820813105987 ) ) ;
#63139=CARTESIAN_POINT ( 'NONE',  ( 154.6182242168042933, 279.6024264367558771, 2.136621738763494704 ) ) ;
#63140=CARTESIAN_POINT ( 'NONE',  ( 135.6816562978893330, 239.9548013555409796, -4.594050593750042211 ) ) ;
#63141=VERTEX_POINT ( 'NONE', #80725 ) ;
#63147=CARTESIAN_POINT ( 'NONE',  ( 200.1076438251647289, 273.8820182500477358, 13.66411480140315504 ) ) ;
#63148=CARTESIAN_POINT ( 'NONE',  ( 180.9880944519944990, 255.9245501647149297, 0.6744818687597132767 ) ) ;
#63150=CARTESIAN_POINT ( 'NONE',  ( 190.5133192800734605, 300.2599720837126824, 2.418563999166301492 ) ) ;
#63155=CARTESIAN_POINT ( 'NONE',  ( 178.5657226154280863, 254.2359737251016440, -5.272414496410398499 ) ) ;
#63158=CARTESIAN_POINT ( 'NONE',  ( 147.9311236323648870, 274.4227731784279172, -7.799459659034405412 ) ) ;
#63160=ORIENTED_EDGE ( 'NONE', *, *, #26638, .T. ) ;
#63163=CARTESIAN_POINT ( 'NONE',  ( 159.6062986900120393, 279.1035829519316849, 10.91088360456809880 ) ) ;
#63164=CARTESIAN_POINT ( 'NONE',  ( 152.2699040063036477, 266.9077851278831872, -16.94750107875206524 ) ) ;
#63168=CARTESIAN_POINT ( 'NONE',  ( 161.4752606922666018, 281.4891156921501079, -6.619806771727822614 ) ) ;
#63169=CARTESIAN_POINT ( 'NONE',  ( 151.4916375207045860, 274.9412589285112745, -8.761911672441238252 ) ) ;
#63170=CARTESIAN_POINT ( 'NONE',  ( 160.1291429304770872, 283.8063366971030064, -1.115091271670870077 ) ) ;
#63172=CARTESIAN_POINT ( 'NONE',  ( 146.8058449195592061, 276.3718130816831149, 4.181814292810413392 ) ) ;
#63174=CARTESIAN_POINT ( 'NONE',  ( 193.0787258475831720, 275.9904400578145669, -16.13630732494317499 ) ) ;
#63176=CARTESIAN_POINT ( 'NONE',  ( 184.6784730347474976, 297.3114112913945632, -4.489973865576921241 ) ) ;
#63177=CARTESIAN_POINT ( 'NONE',  ( 192.0712386031329686, 297.9698513971258649, 12.12276320360788873 ) ) ;
#63180=CARTESIAN_POINT ( 'NONE',  ( -8.565960340006073537, 165.8615022471902591, -10.00000000000009592 ) ) ;
#63182=CARTESIAN_POINT ( 'NONE',  ( -4.722712290662820500, 158.8923013555410080, 4.594050593750050204 ) ) ;
#63183=CARTESIAN_POINT ( 'NONE',  ( 85.53293889029040997, 226.3149278399160949, -9.188101187500095079 ) ) ;
#63186=CARTESIAN_POINT ( 'NONE',  ( 148.0908005895309714, 275.9119617183158084, 5.017397701950214284 ) ) ;
#63187=EDGE_CURVE ( 'NONE', #66923, #20951, #91343, .T. ) ;
#63194=CARTESIAN_POINT ( 'NONE',  ( 161.4331051045346612, 251.0366552657761190, 12.80125893768088652 ) ) ;
#63196=CARTESIAN_POINT ( 'NONE',  ( -0.9341114727035790821, 160.2677522451418213, -5.000000000000041744 ) ) ;
#63198=( BOUNDED_CURVE ( )  B_SPLINE_CURVE ( 2, ( #44409, #33456, #41540, #64352, #13050, #59094, #95316, #18268, #52509 ),
 .UNSPECIFIED., .F., .T. ) 
 B_SPLINE_CURVE_WITH_KNOTS ( ( 3, 2, 2, 2, 3 ),
 ( 0.6411290322580645018, 0.6424731182795698770, 0.6451612903225806273, 0.6478494623655913776, 0.6491935483870967527 ),
 .UNSPECIFIED. ) 
 CURVE ( )  GEOMETRIC_REPRESENTATION_ITEM ( )  RATIONAL_B_SPLINE_CURVE ( ( 0.9330127018922194093, 0.9330127018922194093, 1.000000000000000000, 0.8660254037844387076, 1.000000000000000000, 0.8660254037844387076, 1.000000000000000000, 0.9330127018922194093, 0.9330127018922194093 ) ) 
 REPRESENTATION_ITEM ( '' )  );
#63199=CARTESIAN_POINT ( 'NONE',  ( 195.8947060313465443, 291.3474115503753410, 16.07878593000791767 ) ) ;
#63200=CARTESIAN_POINT ( 'NONE',  ( -5.560871861494070423, 156.0494855054051868, -2.679491924311250717 ) ) ;
#63201=CARTESIAN_POINT ( 'NONE',  ( 161.7412967960748915, 250.5028515975580774, -14.36228887024421041 ) ) ;
#63202=CARTESIAN_POINT ( 'NONE',  ( 42.82723471405275717, 195.5333772461660544, 9.188101187500095079 ) ) ;
#63203=( BOUNDED_CURVE ( )  B_SPLINE_CURVE ( 2, ( #74476, #92191, #22744, #53623, #28334, #84579, #43535, #5054, #35934 ),
 .UNSPECIFIED., .F., .T. ) 
 B_SPLINE_CURVE_WITH_KNOTS ( ( 3, 2, 2, 2, 3 ),
 ( 0.4879032258064516236, 0.4892473118279569988, 0.4919354838709677491, 0.4946236559139784994, 0.4959677419354838745 ),
 .UNSPECIFIED. ) 
 CURVE ( )  GEOMETRIC_REPRESENTATION_ITEM ( )  RATIONAL_B_SPLINE_CURVE ( ( 0.9330127018922194093, 0.9330127018922194093, 1.000000000000000000, 0.8660254037844387076, 1.000000000000000000, 0.8660254037844387076, 1.000000000000000000, 0.9330127018922194093, 0.9330127018922194093 ) ) 
 REPRESENTATION_ITEM ( '' )  );
#63204=CARTESIAN_POINT ( 'NONE',  ( 68.02342162723002161, 200.8923013555409796, 4.594050593750050204 ) ) ;
#63205=CARTESIAN_POINT ( 'NONE',  ( 81.52103558181507026, 206.3262482093457777, 3.021315404115420679E-15 ) ) ;
#63210=CARTESIAN_POINT ( 'NONE',  ( 200.0411626275569574, 270.6720010161316736, -11.59284015024147152 ) ) ;
#63213=CARTESIAN_POINT ( 'NONE',  ( 196.3174919959537306, 290.6151247789487684, -17.61248417473235151 ) ) ;
#63215=CARTESIAN_POINT ( 'NONE',  ( 65.12704176573704729, 220.6589784336661637, -6.496448406907676862E-16 ) ) ;
#63216=CARTESIAN_POINT ( 'NONE',  ( 90.95479231155565003, 229.9865022471903160, 10.00000000000009415 ) ) ;
#63217=CARTESIAN_POINT ( 'NONE',  ( 203.0026270830780675, 279.0361311525880978, -16.61345826058821373 ) ) ;
#63218=CARTESIAN_POINT ( 'NONE',  ( 197.9952413503812352, 287.7091776547143809, 17.17611241386010690 ) ) ;
#63219=CARTESIAN_POINT ( 'NONE',  ( 189.4608361404499703, 260.4689339591389512, -5.099727369828423562 ) ) ;
#63220=CARTESIAN_POINT ( 'NONE',  ( 202.1048707099531612, 280.5910908036593128, 17.24634036681479898 ) ) ;
#63224=CARTESIAN_POINT ( 'NONE',  ( 116.2138665886018458, 231.2365022471901739, -10.00000000000009059 ) ) ;
#63226=CARTESIAN_POINT ( 'NONE',  ( 207.1601050488701503, 271.8351680844880889, 6.320235450527015075 ) ) ;
#63229=CARTESIAN_POINT ( 'NONE',  ( 185.3033850351416163, 271.6740437919646070, 15.89117118174857701 ) ) ;
#63230=VERTEX_POINT ( 'NONE', #59845 ) ;
#63231=CARTESIAN_POINT ( 'NONE',  ( 206.0930919633010774, 273.6832889610345774, -9.866500005465628220 ) ) ;
#63232=CARTESIAN_POINT ( 'NONE',  ( 147.4047294057049271, 275.3345147238139248, 0.000000000000000000 ) ) ;
#63233=CYLINDRICAL_SURFACE ( 'NONE', #72602, 10.00000000000010658 ) ;
#63236=CARTESIAN_POINT ( 'NONE',  ( 176.8706069101428113, 252.4357694602331037, -0.2696942673409187252 ) ) ;
#63237=VERTEX_POINT ( 'NONE', #76083 ) ;
#63239=B_SPLINE_CURVE_WITH_KNOTS ( 'NONE', 3,
 ( #77484, #29869, #22265, #7560 ),
 .UNSPECIFIED., .F., .F.,
 ( 4, 4 ),
 ( 0.02524676605399324425, 0.03021559084467593387 ),
 .UNSPECIFIED. ) ;
#63240=CARTESIAN_POINT ( 'NONE',  ( 167.7537490005853726, 248.2253239148561192, 3.510291536348892905 ) ) ;
#63243=VERTEX_POINT ( 'NONE', #13751 ) ;
#63248=ORIENTED_EDGE ( 'NONE', *, *, #4083, .T. ) ;
#63252=CARTESIAN_POINT ( 'NONE',  ( 174.6327531315653516, 286.2036907333609292, 10.50852000950855114 ) ) ;
#63256=CARTESIAN_POINT ( 'NONE',  ( 194.2199708651012600, 294.2481379475345875, 15.50834247347371253 ) ) ;
#63258=CARTESIAN_POINT ( 'NONE',  ( 204.7242223814549504, 276.0542406257275161, -13.93608974681376189 ) ) ;
#63262=CARTESIAN_POINT ( 'NONE',  ( 95.60083130504949622, 219.8768266524159856, -9.188101187500091527 ) ) ;
#63263=ORIENTED_EDGE ( 'NONE', *, *, #93065, .F. ) ;
#63264=CARTESIAN_POINT ( 'NONE',  ( 191.4484954869714954, 299.0484741143815199, 8.684991747358081327 ) ) ;
#63268=CARTESIAN_POINT ( 'NONE',  ( 156.8233863690425949, 259.0209223242507619, -17.03117928572234163 ) ) ;
#63275=CARTESIAN_POINT ( 'NONE',  ( 207.5987293781265919, 271.0754484607800237, 1.965225377555418484 ) ) ;
#63276=CARTESIAN_POINT ( 'NONE',  ( 82.58295308470839302, 227.6744531367911293, 4.594050593750047540 ) ) ;
#63277=ORIENTED_EDGE ( 'NONE', *, *, #8287, .F. ) ;
#63280=CARTESIAN_POINT ( 'NONE',  ( 161.3190080243304294, 251.2342772056852596, -13.92386533781515823 ) ) ;
#63283=EDGE_CURVE ( 'NONE', #33600, #48389, #99906, .T. ) ;
#63284=CARTESIAN_POINT ( 'NONE',  ( 161.8153693897043581, 283.8862103938810719, 0.5193901413821779833 ) ) ;
#63285=CARTESIAN_POINT ( 'NONE',  ( 188.6301707762981152, 265.0060877223691591, -12.46499516475016733 ) ) ;
#63287=VERTEX_POINT ( 'NONE', #90807 ) ;
#63290=CARTESIAN_POINT ( 'NONE',  ( 206.7893622945242385, 272.4773133715531230, -10.52881283832460291 ) ) ;
#63293=CARTESIAN_POINT ( 'NONE',  ( 174.8907460544039907, 283.7088854317884739, 13.39808451214262597 ) ) ;
#63296=EDGE_LOOP ( 'NONE', ( #9536, #34266, #32210, #66480, #13456, #31455 ) ) ;
#63298=CARTESIAN_POINT ( 'NONE',  ( 161.7101619467568980, 250.5567787384628389, 13.05644392949610655 ) ) ;
#63300=CARTESIAN_POINT ( 'NONE',  ( 187.8346858434329931, 266.3636700819703265, -12.51853185516833200 ) ) ;
#63304=CARTESIAN_POINT ( 'NONE',  ( 153.3235868295895443, 270.3046677488850378, 13.98602533532146808 ) ) ;
#63306=CARTESIAN_POINT ( 'NONE',  ( 162.8996025780091941, 248.4966071325470125, 11.23567065566008516 ) ) ;
#63308=CARTESIAN_POINT ( 'NONE',  ( 180.4959160764321950, 267.2319826678609047, -15.69780135396540288 ) ) ;
#63313=CARTESIAN_POINT ( 'NONE',  ( 169.5324435264030285, 273.3137144743971021, 15.97368087251608770 ) ) ;
#63314=CYLINDRICAL_SURFACE ( 'NONE', #96669, 17.82106496071139645 ) ;
#63316=CARTESIAN_POINT ( 'NONE',  ( 188.2302642645468325, 260.8303285139414243, 3.048995242728016031 ) ) ;
#63317=AXIS2_PLACEMENT_3D ( 'NONE', #71985, #70464, #1078 ) ;
#63318=CARTESIAN_POINT ( 'NONE',  ( 195.2504147615859722, 265.4741584869784674, -7.388824739121020890 ) ) ;
#63319=CARTESIAN_POINT ( 'NONE',  ( 1.528821818964843482, 165.5643266524160140, 9.188101187500095079 ) ) ;
#63321=EDGE_LOOP ( 'NONE', ( #6089, #637, #10315, #8103 ) ) ;
#63322=CARTESIAN_POINT ( 'NONE',  ( 178.6359886761176767, 256.9051424919618398, 8.482123690867066301 ) ) ;
#63323=DIRECTION ( 'NONE',  ( -0.4999999999999998890, 0.8660254037844387076, 0.000000000000000000 ) ) ;
#63324=CARTESIAN_POINT ( 'NONE',  ( 203.1492446519190196, 274.7365285824323564, -12.75106828035650430 ) ) ;
#63326=CARTESIAN_POINT ( 'NONE',  ( 30.27021345494340565, 176.0327760586659736, 1.948934522072302763E-15 ) ) ;
#63329=CARTESIAN_POINT ( 'NONE',  ( 120.4718248238752523, 250.3615022471903444, 5.000000000000046185 ) ) ;
#63330=CARTESIAN_POINT ( 'NONE',  ( 191.8453338867844877, 298.3611298435110371, -9.039024722281077118 ) ) ;
#63332=CARTESIAN_POINT ( 'NONE',  ( 98.24615118885414233, 215.9824982072973683, 3.021315404115420679E-15 ) ) ;
#63333=EDGE_CURVE ( 'NONE', #3950, #76357, #78037, .T. ) ;
#63334=EDGE_CURVE ( 'NONE', #26223, #14773, #79339, .T. ) ;
#63335=CARTESIAN_POINT ( 'NONE',  ( 186.8249449129527875, 295.8321347383906073, -7.822565083202927205 ) ) ;
#63338=CARTESIAN_POINT ( 'NONE',  ( 193.0683888610418251, 295.7999875024635799, -12.37974131660941168 ) ) ;
#63339=CARTESIAN_POINT ( 'NONE',  ( 59.77787777531585789, 211.9865022471903160, 10.00000000000009237 ) ) ;
#63341=CARTESIAN_POINT ( 'NONE',  ( 185.6249487197370627, 277.7860891304547408, -17.37263783417377283 ) ) ;
#63342=CARTESIAN_POINT ( 'NONE',  ( 204.0146600430397825, 270.3923057891465760, 6.034712041982294828 ) ) ;
#63343=CARTESIAN_POINT ( 'NONE',  ( 28.75397480679061246, 199.6589784336661637, -6.496448406907675876E-16 ) ) ;
#63344=CARTESIAN_POINT ( 'NONE',  ( 159.4230536986738400, 254.5181664265525683, 16.83068086755798376 ) ) ;
#63345=CARTESIAN_POINT ( 'NONE',  ( 203.3078925370309094, 270.2142520429687806, -6.437359224241015809 ) ) ;
#63350=CARTESIAN_POINT ( 'NONE',  ( 181.4954090331713417, 255.0423029034424189, 0.9094182891644410072 ) ) ;
#63351=CARTESIAN_POINT ( 'NONE',  ( -16.97593537095525917, 172.5530062829863027, 9.296355089585912665E-16 ) ) ;
#63352=CARTESIAN_POINT ( 'NONE',  ( 160.6748876787037261, 279.0008800672539451, -9.788185859664068289 ) ) ;
#63355=CARTESIAN_POINT ( 'NONE',  ( 163.4260108471723640, 247.5848412648317662, 10.45113099391573108 ) ) ;
#63356=CARTESIAN_POINT ( 'NONE',  ( 149.2923684163597784, 272.0650280510108701, -12.99082738998495756 ) ) ;
#63357=CARTESIAN_POINT ( 'NONE',  ( 188.8822098553512774, 269.9998124647885334, -14.09010591559789560 ) ) ;
#63360=EDGE_CURVE ( 'NONE', #95735, #22875, #35683, .T. ) ;
#63365=CARTESIAN_POINT ( 'NONE',  ( 27.80710661894035596, 186.8615022471902591, -10.00000000000009592 ) ) ;
#63366=CARTESIAN_POINT ( 'NONE',  ( 178.9192782167860400, 282.6651468670382883, 15.91033708812528857 ) ) ;
#63367=FACE_OUTER_BOUND ( 'NONE', #14419, .T. ) ;
#63368=CARTESIAN_POINT ( 'NONE',  ( 177.9916226237585022, 256.4884131028754268, -7.270326030790868366 ) ) ;
#63369=CARTESIAN_POINT ( 'NONE',  ( 190.1190668544949460, 301.3511120508678118, 4.410340539513557090 ) ) ;
#63372=CARTESIAN_POINT ( 'NONE',  ( 189.6356796452440960, 274.2048668380136291, -15.66483313100485297 ) ) ;
#63375=CARTESIAN_POINT ( 'NONE',  ( 201.0732166862245549, 282.3779679885897167, -18.18766936363638820 ) ) ;
#63379=CARTESIAN_POINT ( 'NONE',  ( 157.8043799545718286, 257.3217915922150496, -17.97575562758749257 ) ) ;
#63380=CARTESIAN_POINT ( 'NONE',  ( 95.57333414147498729, 235.1744531367911293, 4.594050593750047540 ) ) ;
#63381=CARTESIAN_POINT ( 'NONE',  ( 180.6932115607800711, 287.5180014335019791, -14.02160881230857825 ) ) ;
#63383=CARTESIAN_POINT ( 'NONE',  ( 164.4405316900629259, 245.8276396196081350, -6.144538123479245328 ) ) ;
#63384=ORIENTED_EDGE ( 'NONE', *, *, #4123, .T. ) ;
#63386=CARTESIAN_POINT ( 'NONE',  ( 157.2050054949160085, 258.7463102223470628, 16.83784704105675090 ) ) ;
#63387=CARTESIAN_POINT ( 'NONE',  ( 204.8570393888089711, 275.3272488847674708, -12.22745498495193139 ) ) ;
#63388=CARTESIAN_POINT ( 'NONE',  ( 52.08270766911643079, 207.0024278399160949, -9.188101187500093303 ) ) ;
#63389=ORIENTED_EDGE ( 'NONE', *, *, #63976, .T. ) ;
#63392=DIRECTION ( 'NONE',  ( 0.4999999999999998890, -0.8660254037844385966, 0.000000000000000000 ) ) ;
#63393=CARTESIAN_POINT ( 'NONE',  ( 176.2490144399759799, 273.0463910110868255, 16.82721827330342990 ) ) ;
#63394=AXIS2_PLACEMENT_3D ( 'NONE', #3078, #94282, #18257 ) ;
#63395=ORIENTED_EDGE ( 'NONE', *, *, #5945, .F. ) ;
#63398=CARTESIAN_POINT ( 'NONE',  ( 190.7403173041394950, 300.2750747078583800, -4.254144485856557800 ) ) ;
#63401=CARTESIAN_POINT ( 'NONE',  ( 171.6923735590184776, 259.4456783946538394, -13.83651731890436842 ) ) ;
#63403=CARTESIAN_POINT ( 'NONE',  ( 148.3005007218871754, 275.7829932922234093, 6.053100225771809839 ) ) ;
#63404=CARTESIAN_POINT ( 'NONE',  ( 193.1977289678065404, 296.0187128512746995, -12.37159405312863925 ) ) ;
#63405=CARTESIAN_POINT ( 'NONE',  ( 149.0359194785865498, 272.5092106407810206, 12.76357969772040590 ) ) ;
#63406=CARTESIAN_POINT ( 'NONE',  ( 177.4464577649037267, 269.5727937689871965, 16.09739030304116625 ) ) ;
#63411=CARTESIAN_POINT ( 'NONE',  ( 173.2798715285074991, 281.8114527337138497, 15.08241540710736750 ) ) ;
#63412=CARTESIAN_POINT ( 'NONE',  ( 103.3675627755349353, 239.6744531367911577, 4.594050593750047540 ) ) ;
#63413=ORIENTED_EDGE ( 'NONE', *, *, #4513, .F. ) ;
#63414=CARTESIAN_POINT ( 'NONE',  ( 191.7934382699952494, 298.4510156884799699, -8.680100145728863126 ) ) ;
#63416=EDGE_CURVE ( 'NONE', #54608, #29477, #61156, .T. ) ;
#63417=CARTESIAN_POINT ( 'NONE',  ( 155.5066938333533528, 261.3015006940112244, -18.40036130547566273 ) ) ;
#63418=B_SPLINE_CURVE_WITH_KNOTS ( 'NONE', 3,
 ( #11690, #5562, #72999, #50170 ),
 .UNSPECIFIED., .F., .F.,
 ( 4, 4 ),
 ( 0.03543422572240963880, 0.04418364752788525585 ),
 .UNSPECIFIED. ) ;
#63419=CARTESIAN_POINT ( 'NONE',  ( 192.3022390788198948, 296.3001551186897018, 12.15446248225496362 ) ) ;
#63424=CARTESIAN_POINT ( 'NONE',  ( 155.0578869440801668, 273.4002611782738654, -12.96254817455158026 ) ) ;
#63425=CARTESIAN_POINT ( 'NONE',  ( 182.1222588711129049, 260.5114411684929223, 9.510826267769539655 ) ) ;
#63426=CARTESIAN_POINT ( 'NONE',  ( 164.8329707752360491, 245.1479151852119855, -0.9471001479485156027 ) ) ;
#63427=CARTESIAN_POINT ( 'NONE',  ( 131.1886288721100300, 255.7369531367911293, -4.594050593750048428 ) ) ;
#63429=CARTESIAN_POINT ( 'NONE',  ( 150.7850480413316632, 269.4796311011364764, -14.43114374163211089 ) ) ;
#63431=CARTESIAN_POINT ( 'NONE',  ( 189.1715903421739711, 282.2647416125370796, -16.61583580824111905 ) ) ;
#63433=CARTESIAN_POINT ( 'NONE',  ( 42.50247518763358556, 195.3458772461660544, 9.188101187500095079 ) ) ;
#63434=AXIS2_PLACEMENT_3D ( 'NONE', #50645, #27366, #66848 ) ;
#63437=ADVANCED_FACE ( 'NONE', ( #22845 ), #13413, .F. ) ;
#63438=B_SPLINE_SURFACE_WITH_KNOTS ( 'NONE', 3, 1, ( 
 ( #6772, #91912 ),
 ( #29572, #14378 ),
 ( #5770, #37651 ),
 ( #92406, #76671 ),
 ( #54338, #99487 ),
 ( #99986, #15343 ),
 ( #30571, #85310 ),
 ( #38660, #52861 ),
 ( #46239, #44753 ),
 ( #45262, #13872 ),
 ( #91403, #61943 ),
 ( #37167, #77165 ),
 ( #36659, #83310 ),
 ( #29089, #76196 ),
 ( #44262, #6272 ),
 ( #68065, #7766 ),
 ( #22954, #31054 ),
 ( #98989, #53362 ),
 ( #60449, #21968 ),
 ( #68561, #7258 ),
 ( #67565, #83811 ),
 ( #92895, #30065 ),
 ( #59955, #60954 ),
 ( #38141, #84312 ),
 ( #69563, #61456 ),
 ( #23448, #22468 ),
 ( #14859, #53843 ),
 ( #84803, #45746 ),
 ( #170, #75195 ),
 ( #98499, #90927 ),
 ( #21477, #52364 ),
 ( #17881, #46763 ),
 ( #86322, #8767 ),
 ( #79214, #56852 ) ),
 .UNSPECIFIED., .T., .F., .F.,
 ( 4, 2, 2, 2, 2, 2, 2, 2, 2, 2, 2, 2, 2, 2, 2, 2, 4 ),
 ( 2, 2 ),
 ( 0.000000000000000000, 0.06250000000000000000, 0.1250000000000000000, 0.1875000000000000000, 0.2500000000000000000, 0.3125000000000000000, 0.3750000000000000000, 0.4375000000000000000, 0.5000000000000000000, 0.5625000000000000000, 0.6250000000000000000, 0.6875000000000000000, 0.7500000000000000000, 0.8125000000000000000, 0.8750000000000000000, 0.9375000000000000000, 1.000000000000000000 ),
 ( 0.000000000000000000, 1.000000000000000000 ),
 .UNSPECIFIED. ) ;
#63441=CARTESIAN_POINT ( 'NONE',  ( 171.2286470186971599, 260.0105123088750361, 14.87178018877357211 ) ) ;
#63443=CARTESIAN_POINT ( 'NONE',  ( 178.8762406774828833, 291.7387019793334275, -6.276231018507565373 ) ) ;
#63444=CARTESIAN_POINT ( 'NONE',  ( 155.5066938333533528, 261.3015006940112244, -18.40036130547566273 ) ) ;
#63445=CARTESIAN_POINT ( 'NONE',  ( 156.9489656246467177, 270.6608685179890585, -14.74928785623654548 ) ) ;
#63446=CARTESIAN_POINT ( 'NONE',  ( 113.3812418268422562, 246.2677522451419065, -5.000000000000047962 ) ) ;
#63448=ORIENTED_EDGE ( 'NONE', *, *, #22897, .F. ) ;
#63449=FACE_OUTER_BOUND ( 'NONE', #93058, .T. ) ;
#63450=CARTESIAN_POINT ( 'NONE',  ( -22.42236680055709641, 157.8615022471902591, 0.000000000000000000 ) ) ;
#63451=CARTESIAN_POINT ( 'NONE',  ( 30.10766014385131939, 182.0643266524160424, 9.188101187500095079 ) ) ;
#63453=CARTESIAN_POINT ( 'NONE',  ( 77.00817486789587463, 215.2677522451418497, 10.00000000000009592 ) ) ;
#63454=CARTESIAN_POINT ( 'NONE',  ( 190.1858949294064871, 301.2353624297489887, -5.249932979468886707 ) ) ;
#63456=CARTESIAN_POINT ( 'NONE',  ( 188.5781848808776431, 266.4637148640482565, 13.66955406155852515 ) ) ;
#63457=CARTESIAN_POINT ( 'NONE',  ( 49.80054343233469893, 212.8927522451419350, 2.944929066748280225E-16 ) ) ;
#63458=CARTESIAN_POINT ( 'NONE',  ( 172.0085750275486305, 287.0065044570835653, 7.467149297792258444 ) ) ;
#63459=CARTESIAN_POINT ( 'NONE',  ( 181.0892345485566750, 256.4416356510156447, 1.320446355720552134 ) ) ;
#63460=CARTESIAN_POINT ( 'NONE',  ( 1.826344505407192287, 171.8615022471902591, -10.00000000000009592 ) ) ;
#63463=ADVANCED_FACE ( 'NONE', ( #96282 ), #23161, .F. ) ;
#63464=CARTESIAN_POINT ( 'NONE',  ( 26.00288702772274618, 192.4865022471903160, 10.00000000000009237 ) ) ;
#63465=CARTESIAN_POINT ( 'NONE',  ( 199.1165320752825494, 285.7670451491295580, 0.000000000000000000 ) ) ;
#63467=CARTESIAN_POINT ( 'NONE',  ( 141.9056932439424372, 261.9244531367911577, -4.594050593750046652 ) ) ;
#63470=CARTESIAN_POINT ( 'NONE',  ( 170.3374160014410563, 263.6467931189878868, 15.82539456636149566 ) ) ;
#63472=CARTESIAN_POINT ( 'NONE',  ( 205.8099205723994203, 269.1131406545866298, -1.356034389334280776 ) ) ;
#63473=CARTESIAN_POINT ( 'NONE',  ( 183.2877288483369966, 257.5383218783772463, -1.784234248563232317 ) ) ;
#63474=EDGE_CURVE ( 'NONE', #79225, #20045, #94939, .T. ) ;
#63478=CARTESIAN_POINT ( 'NONE',  ( 178.5703031916296766, 285.5232265560228484, 13.02254804488858753 ) ) ;
#63479=CARTESIAN_POINT ( 'NONE',  ( 153.4041778544338399, 277.7584533569226437, -5.214878617845980280 ) ) ;
#63481=CARTESIAN_POINT ( 'NONE',  ( 160.4502686134403007, 252.7389780038842844, 16.14074205763531111 ) ) ;
#63482=EDGE_CURVE ( 'NONE', #17038, #1077, #12746, .T. ) ;
#63483=CARTESIAN_POINT ( 'NONE',  ( 160.0061168334508750, 253.5082714530983026, -16.02306982074888708 ) ) ;
#63484=CARTESIAN_POINT ( 'NONE',  ( 152.7153488183568300, 266.1362520814392951, 17.33540622643059237 ) ) ;
#63486=CARTESIAN_POINT ( 'NONE',  ( 191.0568446278853116, 298.2033705976817828, 9.492902989315558315 ) ) ;
#63487=CARTESIAN_POINT ( 'NONE',  ( 208.2124092825819162, 270.0125236866795149, -2.339659020816897694 ) ) ;
#63488=CARTESIAN_POINT ( 'NONE',  ( 155.3738696901333469, 261.5315588585399951, 17.02116401938635804 ) ) ;
#63489=ORIENTED_EDGE ( 'NONE', *, *, #23185, .T. ) ;
#63490=( BOUNDED_CURVE ( )  B_SPLINE_CURVE ( 2, ( #5811, #35215, #67105, #13914, #74744, #5324, #21039, #13434, #98536 ),
 .UNSPECIFIED., .F., .T. ) 
 B_SPLINE_CURVE_WITH_KNOTS ( ( 3, 2, 2, 2, 3 ),
 ( 0.4153225806451613100, 0.4166666666666666852, 0.4193548387096774355, 0.4220430107526881858, 0.4233870967741935609 ),
 .UNSPECIFIED. ) 
 CURVE ( )  GEOMETRIC_REPRESENTATION_ITEM ( )  RATIONAL_B_SPLINE_CURVE ( ( 0.9330127018922194093, 0.9330127018922194093, 1.000000000000000000, 0.8660254037844387076, 1.000000000000000000, 0.8660254037844387076, 1.000000000000000000, 0.9330127018922194093, 0.9330127018922194093 ) ) 
 REPRESENTATION_ITEM ( '' )  );
#63500=DIRECTION ( 'NONE',  ( -0.8660254037844359321, -0.5000000000000051070, -0.000000000000000000 ) ) ;
#63501=ORIENTED_EDGE ( 'NONE', *, *, #92550, .T. ) ;
#63502=CARTESIAN_POINT ( 'NONE',  ( 200.8432122835317841, 282.7763473000181307, 17.15137370990203891 ) ) ;
#63504=CARTESIAN_POINT ( 'NONE',  ( 151.3589047706063582, 268.4856820897672378, 14.56544807350869419 ) ) ;
#63508=CARTESIAN_POINT ( 'NONE',  ( 163.1484656051875106, 248.0655637253488806, 9.714247672444804138 ) ) ;
#63514=CARTESIAN_POINT ( 'NONE',  ( -22.42236680055709641, 157.8615022471902591, 0.000000000000000000 ) ) ;
#63520=CARTESIAN_POINT ( 'NONE',  ( 174.7053765443823465, 290.4798731644879695, 6.449017960443486963 ) ) ;
#63521=CARTESIAN_POINT ( 'NONE',  ( -27.42236680055714260, 166.5217562850347406, 1.224646799147364892E-15 ) ) ;
#63522=EDGE_LOOP ( 'NONE', ( #45294, #19710, #96945, #97308 ) ) ;
#63523=CARTESIAN_POINT ( 'NONE',  ( 187.1869727329149100, 258.4604987923206068, 2.244340846906317299 ) ) ;
#63525=CARTESIAN_POINT ( 'NONE',  ( 164.2572333502590709, 246.1451216570909253, 2.155809084027023204 ) ) ;
#63526=CARTESIAN_POINT ( 'NONE',  ( 159.4889735931715222, 254.4039898200529706, 16.88104032092801887 ) ) ;
#63527=ORIENTED_EDGE ( 'NONE', *, *, #8680, .F. ) ;
#63529=CARTESIAN_POINT ( 'NONE',  ( 157.0239713899953244, 269.7369771206523978, 16.31777668093047851 ) ) ;
#63530=CARTESIAN_POINT ( 'NONE',  ( 206.6298919378964740, 272.7535241315335384, -9.267551915974392429 ) ) ;
#63532=CARTESIAN_POINT ( 'NONE',  ( 200.1102648775588193, 284.0458494464393198, 17.54251420653697835 ) ) ;
#63534=VERTEX_POINT ( 'NONE', #82595 ) ;
#63535=CARTESIAN_POINT ( 'NONE',  ( 193.9864735853334707, 294.6525670995212067, -15.54227678654798694 ) ) ;
#63537=CARTESIAN_POINT ( 'NONE',  ( 54.63354020801842381, 213.8967562850347122, -4.648177544792955347E-16 ) ) ;
#63538=CARTESIAN_POINT ( 'NONE',  ( 16.81940930487741426, 170.5177522451417929, 5.000000000000051514 ) ) ;
#63539=CARTESIAN_POINT ( 'NONE',  ( 79.22710464504368133, 225.7369531367911293, -4.594050593750048428 ) ) ;
#63542=DIRECTION ( 'NONE',  ( -0.5000000000000006661, 0.8660254037844382635, -1.877843081442121204E-16 ) ) ;
#63544=CARTESIAN_POINT ( 'NONE',  ( 7.428446334363822956, 175.0958772461660544, -9.188101187500095079 ) ) ;
#63549=VERTEX_POINT ( 'NONE', #63232 ) ;
#63551=CARTESIAN_POINT ( 'NONE',  ( 187.9019955452718023, 260.0457317612239194, -6.306085470763082235 ) ) ;
#63552=EDGE_CURVE ( 'NONE', #83741, #73589, #81663, .T. ) ;
#63555=EDGE_CURVE ( 'NONE', #8043, #41536, #11666, .T. ) ;
#63557=CARTESIAN_POINT ( 'NONE',  ( 161.8807657183444064, 250.2612843381103573, -13.52770735624900311 ) ) ;
#63558=CARTESIAN_POINT ( 'NONE',  ( 185.7234768551323896, 286.5997348792201933, 15.91907032080574780 ) ) ;
#63560=CARTESIAN_POINT ( 'NONE',  ( 43.09804120061789945, 189.5643266524160140, 9.188101187500095079 ) ) ;
#63561=CARTESIAN_POINT ( 'NONE',  ( 86.02927282398381692, 207.1427522451417644, 1.119607411625061291E-15 ) ) ;
#63562=CARTESIAN_POINT ( 'NONE',  ( 198.1145155272607212, 276.7736982920383753, 15.18375391169536393 ) ) ;
#63565=CARTESIAN_POINT ( 'NONE',  ( 175.1244175801234348, 281.4242832285925147, -15.54073688850160018 ) ) ;
#63566=CIRCLE ( 'NONE', #19914, 17.82106496071138224 ) ;
#63567=CARTESIAN_POINT ( 'NONE',  ( -9.134289513013563067, 165.5333772461660828, 9.188101187500095079 ) ) ;
#63569=CARTESIAN_POINT ( 'NONE',  ( 151.2964716097791325, 268.5938194963972592, -15.66250187539618111 ) ) ;
#63570=CARTESIAN_POINT ( 'NONE',  ( 187.2161039051867704, 282.9898844212582958, 16.21219487239775958 ) ) ;
#63571=CARTESIAN_POINT ( 'NONE',  ( 194.8432095198904221, 293.1686569321988145, -14.74101036184996616 ) ) ;
#63573=CARTESIAN_POINT ( 'NONE',  ( 189.5675921607796965, 262.4732863060856971, 8.237194270739541579 ) ) ;
#63574=CARTESIAN_POINT ( 'NONE',  ( 204.2556901454867955, 276.8657622634082713, 13.61111001399713949 ) ) ;
#63575=CARTESIAN_POINT ( 'NONE',  ( 147.0721334091522294, 275.9105878882373304, 0.7242168585908188572 ) ) ;
#63576=CARTESIAN_POINT ( 'NONE',  ( 190.1730848958311810, 301.2575500587478814, 0.2415986433272204748 ) ) ;
#63577=ORIENTED_EDGE ( 'NONE', *, *, #85775, .T. ) ;
#63578=EDGE_CURVE ( 'NONE', #44048, #59643, #38177, .T. ) ;
#63579=CARTESIAN_POINT ( 'NONE',  ( 163.9354095869165633, 246.7025367662834014, -7.289870401565430313 ) ) ;
#63580=CARTESIAN_POINT ( 'NONE',  ( 181.1268834691935297, 268.2382088362665513, 15.85390869987196538 ) ) ;
#63581=CARTESIAN_POINT ( 'NONE',  ( 101.8248682511026573, 241.8464784336661353, 1.353441290958777327E-15 ) ) ;
#63584=DIRECTION ( 'NONE',  ( 0.4999999999999992784, -0.8660254037844390407, 0.000000000000000000 ) ) ;
#63586=CARTESIAN_POINT ( 'NONE',  ( 196.0395593785976018, 291.0965181932902510, 15.97855489120023087 ) ) ;
#63588=CARTESIAN_POINT ( 'NONE',  ( 151.4352206443128068, 277.3697824090307336, -6.572806124296932673 ) ) ;
#63590=CARTESIAN_POINT ( 'NONE',  ( 196.6288634187112052, 290.0758136547079289, -16.31544900032282186 ) ) ;
#63592=CARTESIAN_POINT ( 'NONE',  ( 203.8165033694633621, 276.7299672189732291, 13.95262359560297583 ) ) ;
#63594=ORIENTED_EDGE ( 'NONE', *, *, #62851, .F. ) ;
#63595=CARTESIAN_POINT ( 'NONE',  ( 189.3573010603350895, 265.1416018912782420, 12.05679781153855323 ) ) ;
#63597=CARTESIAN_POINT ( 'NONE',  ( 197.8518484210461281, 268.8967432528903032, 9.285919980081231984 ) ) ;
#63598=ADVANCED_FACE ( 'NONE', ( #32331 ), #33862, .T. ) ;
#63603=CARTESIAN_POINT ( 'NONE',  ( 153.3920560952016956, 264.9641606960921649, 16.50453917291963535 ) ) ;
#63607=CARTESIAN_POINT ( 'NONE',  ( 195.2456755912178323, 290.2219180048303429, -16.53585882530188655 ) ) ;
#63609=B_SPLINE_CURVE_WITH_KNOTS ( 'NONE', 3,
 ( #86569, #17101, #36789, #89558 ),
 .UNSPECIFIED., .F., .F.,
 ( 4, 4 ),
 ( 0.03111358529414371549, 0.04015756546154605061 ),
 .UNSPECIFIED. ) ;
#63610=CARTESIAN_POINT ( 'NONE',  ( 166.8963927329958494, 280.5591284459779331, 11.67036085821709612 ) ) ;
#63611=CARTESIAN_POINT ( 'NONE',  ( 148.0346525705264469, 274.2434557974783615, -9.381294579651672905 ) ) ;
#63612=CARTESIAN_POINT ( 'NONE',  ( 193.9979983253333842, 262.2552985615510579, -0.8131695963413709816 ) ) ;
#63613=ORIENTED_EDGE ( 'NONE', *, *, #54575, .T. ) ;
#63615=CYLINDRICAL_SURFACE ( 'NONE', #92901, 17.82106496071139645 ) ;
#63616=B_SPLINE_CURVE_WITH_KNOTS ( 'NONE', 3,
 ( #66399, #20312, #4097, #5596 ),
 .UNSPECIFIED., .F., .F.,
 ( 4, 4 ),
 ( 0.008060310584812914458, 0.01415263866924437036 ),
 .UNSPECIFIED. ) ;
#63617=CARTESIAN_POINT ( 'NONE',  ( 72.14936367153653407, 200.9155109091896065, 2.679491924311254714 ) ) ;
#63623=CARTESIAN_POINT ( 'NONE',  ( 203.0862352702880003, 278.8913175244117610, -15.09542727681365015 ) ) ;
#63626=CARTESIAN_POINT ( 'NONE',  ( 202.6051175132338926, 273.9538057854381350, -13.19822448684500849 ) ) ;
#63629=EDGE_CURVE ( 'NONE', #43398, #61969, #89070, .T. ) ;
#63631=CARTESIAN_POINT ( 'NONE',  ( 173.1389949595530311, 270.9080448422716927, 16.48212318985030578 ) ) ;
#63634=CARTESIAN_POINT ( 'NONE',  ( 184.8055014132766303, 281.5399926389359280, -16.29175395855951791 ) ) ;
#63635=CARTESIAN_POINT ( 'NONE',  ( 165.0748171242677245, 244.7290250210644729, -1.867635796467185028 ) ) ;
#63636=CARTESIAN_POINT ( 'NONE',  ( 190.4843783887033055, 300.7183739130279037, 3.438264421829949402 ) ) ;
#63637=DIRECTION ( 'NONE',  ( 0.8660254037844395958, 0.4999999999999985567, 0.000000000000000000 ) ) ;
#63639=CARTESIAN_POINT ( 'NONE',  ( 153.1961624462112752, 265.3034584490234806, -16.19494717845262954 ) ) ;
#63641=FACE_OUTER_BOUND ( 'NONE', #6963, .T. ) ;
#63642=CARTESIAN_POINT ( 'NONE',  ( 154.0986224399686648, 280.1916420498395155, 2.233781007141098396 ) ) ;
#63643=CARTESIAN_POINT ( 'NONE',  ( 126.9399520566163773, 244.0958772461660544, -9.188101187500095079 ) ) ;
#63649=CARTESIAN_POINT ( 'NONE',  ( 203.6418419907373902, 276.2461351259622688, 13.34765691815280952 ) ) ;
#63651=CARTESIAN_POINT ( 'NONE',  ( 171.5263804624986790, 288.0246480763028671, -4.629733576150550256 ) ) ;
#63652=CARTESIAN_POINT ( 'NONE',  ( 192.7575593570047090, 296.7811089811312399, 12.30688046782918121 ) ) ;
#63654=CARTESIAN_POINT ( 'NONE',  ( 194.8644079090977357, 267.3518508506872990, 11.26063562417210484 ) ) ;
#63655=CARTESIAN_POINT ( 'NONE',  ( 175.6817329609027354, 287.9557713606999982, -9.344572807206340315 ) ) ;
#63657=CARTESIAN_POINT ( 'NONE',  ( 177.1731152019401350, 256.0265825107734372, -7.293953335171803332 ) ) ;
#63658=ORIENTED_EDGE ( 'NONE', *, *, #67437, .T. ) ;
#63659=CARTESIAN_POINT ( 'NONE',  ( 147.6054094044680198, 274.9869267698931594, -8.596541856229405809 ) ) ;
#63660=CARTESIAN_POINT ( 'NONE',  ( 3.692648916086829658, 184.4860189848785410, -2.679491924311252493 ) ) ;
#63662=VERTEX_POINT ( 'NONE', #1942 ) ;
#63663=CARTESIAN_POINT ( 'NONE',  ( 168.1726423428391399, 255.4859975196775963, 14.21197738914692366 ) ) ;
#63665=CARTESIAN_POINT ( 'NONE',  ( 190.9492529716546017, 283.2944616250604213, -16.57272652201862329 ) ) ;
#63667=CARTESIAN_POINT ( 'NONE',  ( 149.6676065383367416, 271.4150965588098074, 11.80358707172367261 ) ) ;
#63668=CARTESIAN_POINT ( 'NONE',  ( 202.6070187115982719, 279.7213449518906145, 15.56322169823762280 ) ) ;
#63669=CARTESIAN_POINT ( 'NONE',  ( 164.6578333510718721, 283.8482461527818259, -6.790344748163971822 ) ) ;
#63670=CARTESIAN_POINT ( 'NONE',  ( 154.4470374439381146, 277.6591429590598068, -9.115886381272481742 ) ) ;
#63671=CARTESIAN_POINT ( 'NONE',  ( 153.0308080659177392, 265.5898606369461277, -17.74682723936668438 ) ) ;
#63673=CARTESIAN_POINT ( 'NONE',  ( 166.4230964287024506, 281.1278175241628787, -10.97197584377154200 ) ) ;
#63675=CARTESIAN_POINT ( 'NONE',  ( 187.4171132689631634, 261.5282790321019206, -9.397869408254909018 ) ) ;
#63676=DIRECTION ( 'NONE',  ( -0.8660254037844359321, -0.5000000000000051070, -0.000000000000000000 ) ) ;
#63677=FACE_OUTER_BOUND ( 'NONE', #59874, .T. ) ;
#63680=CARTESIAN_POINT ( 'NONE',  ( 204.2465476932143531, 275.5256217290955192, 13.24663835785611710 ) ) ;
#63683=CARTESIAN_POINT ( 'NONE',  ( 155.1376601545389917, 261.9406857754215707, 18.55063430030667959 ) ) ;
#63684=CARTESIAN_POINT ( 'NONE',  ( 167.2415451205598345, 247.5609011665888772, -4.849568200425117048 ) ) ;
#63686=CARTESIAN_POINT ( 'NONE',  ( 93.00275509369619442, 218.3768266524159856, -9.188101187500091527 ) ) ;
#63688=CARTESIAN_POINT ( 'NONE',  ( 146.9700173529739970, 276.0874580858064746, -5.099093031535578469 ) ) ;
#63689=CARTESIAN_POINT ( 'NONE',  ( 148.0447915602865976, 275.7505707160540283, 4.987173999238420308 ) ) ;
#63690=EDGE_CURVE ( 'NONE', #4764, #5671, #92604, .T. ) ;
#63691=CARTESIAN_POINT ( 'NONE',  ( 155.2193237801463113, 261.7992402267395846, -18.58295809893692407 ) ) ;
#63696=B_SPLINE_CURVE_WITH_KNOTS ( 'NONE', 3,
 ( #69005, #30015, #23402, #99438, #85262, #91863, #38094, #83258, #99935, #83764, #15295, #92360, #52807, #14325, #29527, #76151 ),
 .UNSPECIFIED., .F., .F.,
 ( 4, 2, 2, 2, 2, 2, 2, 4 ),
 ( 3.103167691559091397E-17, 0.0003787177898467000204, 0.0007574355796933690326, 0.001136153369540038099, 0.001514871159386707057, 0.001893588949233376015, 0.002272306739080045407, 0.003029742318773331715 ),
 .UNSPECIFIED. ) ;
#63698=CARTESIAN_POINT ( 'NONE',  ( 178.8990464802429017, 290.1033400482242541, 9.442229793486959011 ) ) ;
#63699=CARTESIAN_POINT ( 'NONE',  ( 169.2468562361510465, 252.1710243214491527, -8.924574812386079969 ) ) ;
#63700=CARTESIAN_POINT ( 'NONE',  ( 172.4419760422836134, 290.9306500000749907, -0.6531725299933459628 ) ) ;
#63702=CARTESIAN_POINT ( 'NONE',  ( -10.02737821244022776, 165.0177522451418781, -10.00000000000009592 ) ) ;
#63704=CARTESIAN_POINT ( 'NONE',  ( 42.55642822748761489, 201.5024278399160949, 9.188101187500095079 ) ) ;
#63707=CARTESIAN_POINT ( 'NONE',  ( 72.16419236301562989, 200.2202760586659736, -5.415160957724236172E-17 ) ) ;
#63708=CARTESIAN_POINT ( 'NONE',  ( 164.1344181360771870, 246.9811661530827962, -5.863116506140533701 ) ) ;
#63713=CARTESIAN_POINT ( 'NONE',  ( 11.71892835771565800, 189.1199935810941213, 2.679491924311251605 ) ) ;
#63716=CARTESIAN_POINT ( 'NONE',  ( 196.2379679265050925, 290.7528645076583871, -16.93678934971137906 ) ) ;
#63719=CARTESIAN_POINT ( 'NONE',  ( 72.21814540286966633, 206.3768266524159571, -9.188101187500093303 ) ) ;
#63721=CARTESIAN_POINT ( 'NONE',  ( 155.5066938333533528, 261.3015006940112244, -18.40036130547566273 ) ) ;
#63722=CARTESIAN_POINT ( 'NONE',  ( 172.9367659230471190, 289.5787789514328097, -1.054365525152276772 ) ) ;
#63724=CARTESIAN_POINT ( 'NONE',  ( 201.5239699368452193, 281.5972404568383354, 17.74311413406459792 ) ) ;
#63727=CARTESIAN_POINT ( 'NONE',  ( 123.1420698188773315, 235.2365022471902023, 10.00000000000009592 ) ) ;
#63729=CARTESIAN_POINT ( 'NONE',  ( 164.6649740431187183, 245.4388940607451843, -1.430729255012818557 ) ) ;
#63732=CARTESIAN_POINT ( 'NONE',  ( 149.0466799873937020, 273.2901661242311206, -9.699341834421078445 ) ) ;
#63733=CARTESIAN_POINT ( 'NONE',  ( 187.9132866086108891, 273.2693441326987340, 15.64203133854969963 ) ) ;
#63735=CARTESIAN_POINT ( 'NONE',  ( 202.2712651538608668, 280.3028871727136675, 16.13191389836473988 ) ) ;
#63739=CARTESIAN_POINT ( 'NONE',  ( 176.7648174719832639, 252.3281646357263241, -0.2701238880731380854 ) ) ;
#63741=ORIENTED_EDGE ( 'NONE', *, *, #80079, .T. ) ;
#63743=CARTESIAN_POINT ( 'NONE',  ( 170.6258808213388249, 250.4240718389760332, 3.381858602187873153 ) ) ;
#63744=CARTESIAN_POINT ( 'NONE',  ( 159.5606259118165724, 264.0648208006689401, -17.79391822139266566 ) ) ;
#63745=EDGE_CURVE ( 'NONE', #66781, #49648, #36934, .T. ) ;
#63753=ORIENTED_EDGE ( 'NONE', *, *, #63360, .T. ) ;
#63755=CARTESIAN_POINT ( 'NONE',  ( 186.3453228331337073, 298.4577095622237835, 1.059573036266669765 ) ) ;
#63757=CARTESIAN_POINT ( 'NONE',  ( 148.1974503712686158, 273.9614817352322120, -7.884397846570731616 ) ) ;
#63759=CARTESIAN_POINT ( 'NONE',  ( 155.4186054393023255, 261.4540742680644598, 17.05753227160644769 ) ) ;
#63760=CARTESIAN_POINT ( 'NONE',  ( 185.4122142602475378, 292.4855490106422735, -11.52758158381046449 ) ) ;
#63761=CARTESIAN_POINT ( 'NONE',  ( 157.4211152037729562, 257.9856256133486454, -16.71526195140576831 ) ) ;
#63762=CARTESIAN_POINT ( 'NONE',  ( 164.7117522571876123, 245.3578718172906292, 5.414774406097063064 ) ) ;
#63763=CARTESIAN_POINT ( 'NONE',  ( 206.6977975800406284, 270.2202961249453779, 3.296240252125988146 ) ) ;
#63765=CARTESIAN_POINT ( 'NONE',  ( 87.80660267098954819, 215.3768266524160140, -9.188101187500091527 ) ) ;
#63767=CARTESIAN_POINT ( 'NONE',  ( 191.5544531425776427, 298.8649500714207647, 8.366689293739112188 ) ) ;
#63768=CARTESIAN_POINT ( 'NONE',  ( 179.0110060009473045, 253.5811209532878934, 0.3050717900565249607 ) ) ;
#63770=CARTESIAN_POINT ( 'NONE',  ( 156.6814027994969933, 259.2668450805435896, -17.66460052862722918 ) ) ;
#63772=CARTESIAN_POINT ( 'NONE',  ( 187.0997774576600534, 269.0605681235749671, -15.68935166958139149 ) ) ;
#63775=CARTESIAN_POINT ( 'NONE',  ( 164.2083349707763489, 249.9453208731862048, 10.14950949454277485 ) ) ;
#63777=CARTESIAN_POINT ( 'NONE',  ( 98.14495447654879001, 215.2202760586659167, -5.415160957724236172E-17 ) ) ;
#63780=CARTESIAN_POINT ( 'NONE',  ( 161.2672255145357383, 251.3239671435932223, -13.23747325324243995 ) ) ;
#63784=CARTESIAN_POINT ( 'NONE',  ( 207.2384045602068454, 270.5804084916183001, -2.409301690515441408 ) ) ;
#63786=EDGE_LOOP ( 'NONE', ( #93201, #12206 ) ) ;
#63787=CARTESIAN_POINT ( 'NONE',  ( 190.8806404710506399, 295.7339764775937851, 11.26209325552490448 ) ) ;
#63788=CARTESIAN_POINT ( 'NONE',  ( 160.4728670955267944, 275.6021364759136532, 12.83076506165803465 ) ) ;
#63789=DIRECTION ( 'NONE',  ( 0.4999999999999998890, -0.8660254037844385966, 0.000000000000000000 ) ) ;
#63790=CARTESIAN_POINT ( 'NONE',  ( 147.9515918652886342, 275.3690718889737923, -4.989113661445183645 ) ) ;
#63792=( BOUNDED_CURVE ( )  B_SPLINE_CURVE ( 2, ( #46174, #77094, #23382, #7696, #39568, #38588, #47189, #54272, #78110 ),
 .UNSPECIFIED., .F., .T. ) 
 B_SPLINE_CURVE_WITH_KNOTS ( ( 3, 2, 2, 2, 3 ),
 ( 0.5282258064516128782, 0.5295698924731182533, 0.5322580645161290036, 0.5349462365591397539, 0.5362903225806451291 ),
 .UNSPECIFIED. ) 
 CURVE ( )  GEOMETRIC_REPRESENTATION_ITEM ( )  RATIONAL_B_SPLINE_CURVE ( ( 0.9330127018922194093, 0.9330127018922194093, 1.000000000000000000, 0.8660254037844387076, 1.000000000000000000, 0.8660254037844387076, 1.000000000000000000, 0.9330127018922194093, 0.9330127018922194093 ) ) 
 REPRESENTATION_ITEM ( '' )  );
#63794=CARTESIAN_POINT ( 'NONE',  ( -22.42236680055709641, 157.8615022471902591, 0.000000000000000000 ) ) ;
#63795=AXIS2_PLACEMENT_3D ( 'NONE', #20223, #3050, #49609 ) ;
#63797=ORIENTED_EDGE ( 'NONE', *, *, #42285, .F. ) ;
#63799=CARTESIAN_POINT ( 'NONE',  ( 203.6072550072871081, 277.2840265471566568, -14.24554571798122460 ) ) ;
#63800=CARTESIAN_POINT ( 'NONE',  ( 200.4403816905005158, 283.4740703539914648, 16.81798557643505987 ) ) ;
#63802=CARTESIAN_POINT ( 'NONE',  ( 188.2118626355560025, 265.7141890007951019, -13.18290805338666694 ) ) ;
#63804=CARTESIAN_POINT ( 'NONE',  ( 109.6465072765697641, 244.1115022471903160, -5.000000000000047962 ) ) ;
#63805=CYLINDRICAL_SURFACE ( 'NONE', #49474, 17.82106496071139645 ) ;
#63806=ADVANCED_FACE ( 'NONE', ( #52512 ), #28730, .T. ) ;
#63810=CARTESIAN_POINT ( 'NONE',  ( 207.0200405408487541, 272.0777669287182334, 6.494273599193515878 ) ) ;
#63811=CARTESIAN_POINT ( 'NONE',  ( 185.6955650132851758, 265.8818490688272504, 13.06349922320766410 ) ) ;
#63812=CARTESIAN_POINT ( 'NONE',  ( 199.3598424642473219, 281.4464541862251394, -16.65811581254586926 ) ) ;
#63814=DIRECTION ( 'NONE',  ( 0.4999999999999992784, -0.8660254037844390407, 0.000000000000000000 ) ) ;
#63815=CARTESIAN_POINT ( 'NONE',  ( 182.4040233711584449, 274.1968787646982264, 16.41695686085575190 ) ) ;
#63817=CARTESIAN_POINT ( 'NONE',  ( 191.4759666451473947, 261.1522761069668945, 3.097452836964068812 ) ) ;
#63818=CARTESIAN_POINT ( 'NONE',  ( 207.7320178805681508, 270.8445860024863237, -5.379955943374661764 ) ) ;
#63819=CARTESIAN_POINT ( 'NONE',  ( 1.258015332399702757, 171.5333772461660828, 9.188101187500095079 ) ) ;
#63822=CARTESIAN_POINT ( 'NONE',  ( 161.0189972650558445, 253.0741054593400179, -14.82454529635133333 ) ) ;
#63825=CARTESIAN_POINT ( 'NONE',  ( 25.45277359850996390, 179.3768266524159856, -9.188101187500093303 ) ) ;
#63826=CARTESIAN_POINT ( 'NONE',  ( 149.8083888948594335, 271.5779462620446338, 11.70101749353969645 ) ) ;
#63828=CARTESIAN_POINT ( 'NONE',  ( 179.1815112968807568, 292.0126970491061229, 6.085306834880822358 ) ) ;
#63829=CARTESIAN_POINT ( 'NONE',  ( 191.4852287632733123, 298.9848502134979071, -9.870565261052552941 ) ) ;
#63830=CARTESIAN_POINT ( 'NONE',  ( 196.5969449268226299, 290.1310981043597508, 16.37092889558107345 ) ) ;
#63835=CARTESIAN_POINT ( 'NONE',  ( 193.0625067496444558, 295.7221012308248760, -12.50071909232508460 ) ) ;
#63836=CARTESIAN_POINT ( 'NONE',  ( 81.06766895168330223, 227.6115022471903160, -5.000000000000047962 ) ) ;
#63838=CARTESIAN_POINT ( 'NONE',  ( 156.6812872898450735, 261.2670451491295012, 0.000000000000000000 ) ) ;
#63840=CARTESIAN_POINT ( 'NONE',  ( 52.54321753458319932, 191.9548013555410080, -4.594050593750042211 ) ) ;
#63843=CARTESIAN_POINT ( 'NONE',  ( 190.2510882691990730, 301.1224442529128851, -5.480893437181090455 ) ) ;
#63845=ORIENTED_EDGE ( 'NONE', *, *, #42069, .F. ) ;
#63847=CARTESIAN_POINT ( 'NONE',  ( -16.85990996717081813, 172.6199935810941213, 2.679491924311252049 ) ) ;
#63848=CARTESIAN_POINT ( 'NONE',  ( 193.2843052833196111, 295.8687582740735138, 14.08193878756009632 ) ) ;
#63849=CARTESIAN_POINT ( 'NONE',  ( 204.7200661083698776, 274.0614395018808978, 12.25436898028725530 ) ) ;
#63851=CARTESIAN_POINT ( 'NONE',  ( 162.8042930031641049, 248.6616881586264469, 11.14389129512055554 ) ) ;
#63852=CARTESIAN_POINT ( 'NONE',  ( 149.3629284598386278, 271.9428144707212027, -12.99253781774931049 ) ) ;
#63854=CARTESIAN_POINT ( 'NONE',  ( 188.8413990936387279, 270.2136967773887477, -14.28180970089109714 ) ) ;
#63864=CARTESIAN_POINT ( 'NONE',  ( 190.8187029736043883, 300.1393067457597681, 3.941064102378585954 ) ) ;
#63869=CARTESIAN_POINT ( 'NONE',  ( 187.7049306102153139, 273.0437162969578822, -15.74079531760049910 ) ) ;
#63870=FACE_OUTER_BOUND ( 'NONE', #96575, .T. ) ;
#63877=CARTESIAN_POINT ( 'NONE',  ( 204.6235849755581455, 276.2285497258825444, -13.59355699282649432 ) ) ;
#63879=CARTESIAN_POINT ( 'NONE',  ( 92.97525793012167128, 233.6744531367911293, 4.594050593750047540 ) ) ;
#63880=CARTESIAN_POINT ( 'NONE',  ( 180.3582177101254729, 287.0947775038071654, -13.76116533618757742 ) ) ;
#63881=VERTEX_POINT ( 'NONE', #36816 ) ;
#63882=CARTESIAN_POINT ( 'NONE',  ( 160.6949176047705805, 266.4836554915148099, 16.57512223367676185 ) ) ;
#63883=ORIENTED_EDGE ( 'NONE', *, *, #65844, .F. ) ;
#63887=CARTESIAN_POINT ( 'NONE',  ( 65.85835811776894388, 199.6423013555410080, -4.594050593750043987 ) ) ;
#63889=CARTESIAN_POINT ( 'NONE',  ( 191.5544531425776427, 298.8649500714207647, 8.366689293739112188 ) ) ;
#63890=CARTESIAN_POINT ( 'NONE',  ( 198.0355408163131585, 287.6393769322024241, 18.20720360189982756 ) ) ;
#63894=CARTESIAN_POINT ( 'NONE',  ( 177.8972298254044802, 288.9764328270704823, 11.11871301495054531 ) ) ;
#63897=CARTESIAN_POINT ( 'NONE',  ( 175.4772207271338686, 261.2202791896218628, -14.50271330228049926 ) ) ;
#63899=CARTESIAN_POINT ( 'NONE',  ( 161.2488013048736377, 251.3558788108169040, -13.10044423494716170 ) ) ;
#63900=CARTESIAN_POINT ( 'NONE',  ( 193.2053309019613891, 296.0055459150826778, -12.79465285318189061 ) ) ;
#63902=CARTESIAN_POINT ( 'NONE',  ( 180.9036116742409206, 271.3736204808990919, 16.91026336658080709 ) ) ;
#63908=CARTESIAN_POINT ( 'NONE',  ( 106.6423081075360813, 238.5024278399160949, -9.188101187500093303 ) ) ;
#63910=CARTESIAN_POINT ( 'NONE',  ( 191.7741832257749195, 298.4843664033717801, -8.615487418695501276 ) ) ;
#63912=CARTESIAN_POINT ( 'NONE',  ( 203.0498946958275326, 278.9542612457532869, -15.11479947333269003 ) ) ;
#63913=CARTESIAN_POINT ( 'NONE',  ( 164.2059258710715994, 246.2339888178522926, 7.329631442356459914 ) ) ;
#63915=CARTESIAN_POINT ( 'NONE',  ( 175.9918762399839238, 254.0358301690074825, 4.937466140392421821 ) ) ;
#63916=ORIENTED_EDGE ( 'NONE', *, *, #5956, .T. ) ;
#63918=CARTESIAN_POINT ( 'NONE',  ( 158.0762504856774342, 274.7363926669914349, -12.55549483934156640 ) ) ;
#63919=CARTESIAN_POINT ( 'NONE',  ( 185.4471331129824705, 262.0162576244363208, 9.741638050158547557 ) ) ;
#63920=CARTESIAN_POINT ( 'NONE',  ( 206.0061733044583434, 273.8338364942757153, -9.988470584493322590 ) ) ;
#63921=CARTESIAN_POINT ( 'NONE',  ( 139.9303331133829715, 251.5958772461660544, -9.188101187500095079 ) ) ;
#63922=CARTESIAN_POINT ( 'NONE',  ( 189.9884557574413293, 294.6014195808287468, -12.37837975822646186 ) ) ;
#63924=CARTESIAN_POINT ( 'NONE',  ( 185.8673354792971111, 296.7643724201381588, 4.550508980395866487 ) ) ;
#63927=CARTESIAN_POINT ( 'NONE',  ( 53.67935523340274528, 210.9869531367911009, 4.594050593750046652 ) ) ;
#63929=CARTESIAN_POINT ( 'NONE',  ( 157.7733463334721478, 257.3755434007023268, -16.94489513499352995 ) ) ;
#63932=CARTESIAN_POINT ( 'NONE',  ( 174.4487186589523731, 262.1766023258701352, 14.34670417327684255 ) ) ;
#63933=CARTESIAN_POINT ( 'NONE',  ( 191.2278159864466431, 297.4307022214792937, -10.96893880474589267 ) ) ;
#63934=CARTESIAN_POINT ( 'NONE',  ( 178.4999909733569154, 292.3696688670564185, -7.228411343512463283 ) ) ;
#63936=CARTESIAN_POINT ( 'NONE',  ( 203.3740894404336927, 278.3927394765486838, -15.19753795879846869 ) ) ;
#63937=CARTESIAN_POINT ( 'NONE',  ( 178.4492094125899087, 261.1672851353984584, 12.23577833629752831 ) ) ;
#63938=CARTESIAN_POINT ( 'NONE',  ( 123.3405339703633672, 232.0177522451417929, 5.000000000000051514 ) ) ;
#63939=B_SPLINE_SURFACE_WITH_KNOTS ( 'NONE', 3, 1, ( 
 ( #96009, #43236 ),
 ( #66552, #36138 ),
 ( #74178, #57445 ),
 ( #28046, #82308 ),
 ( #18985, #12879 ),
 ( #4250, #27069 ),
 ( #43737, #74682 ),
 ( #57952, #19496 ),
 ( #50350, #81305 ),
 ( #11876, #42731 ),
 ( #73669, #22440 ),
 ( #67540, #91888 ),
 ( #83279, #59930 ),
 ( #13847, #61920 ),
 ( #30544, #31031 ),
 ( #23422, #53816 ),
 ( #69032, #21450 ),
 ( #29547, #38114 ),
 ( #7741, #77660 ),
 ( #21940, #38627 ),
 ( #53334, #68536 ),
 ( #68042, #84288 ),
 ( #44724, #76172 ),
 ( #76645, #75657 ),
 ( #14834, #14347 ),
 ( #8248, #60421 ),
 ( #45722, #98964 ),
 ( #84779, #52338 ),
 ( #99459, #91377 ),
 ( #54313, #69537 ),
 ( #6749, #98470 ),
 ( #7230, #6242 ),
 ( #90900, #37137 ),
 ( #92869, #145 ) ),
 .UNSPECIFIED., .T., .F., .F.,
 ( 4, 2, 2, 2, 2, 2, 2, 2, 2, 2, 2, 2, 2, 2, 2, 2, 4 ),
 ( 2, 2 ),
 ( 0.000000000000000000, 0.06250000000000000000, 0.1250000000000000000, 0.1875000000000000000, 0.2500000000000000000, 0.3125000000000000000, 0.3750000000000000000, 0.4375000000000000000, 0.5000000000000000000, 0.5625000000000000000, 0.6250000000000000000, 0.6875000000000000000, 0.7500000000000000000, 0.8125000000000000000, 0.8750000000000000000, 0.9375000000000000000, 1.000000000000000000 ),
 ( 0.000000000000000000, 1.000000000000000000 ),
 .UNSPECIFIED. ) ;
#63942=CARTESIAN_POINT ( 'NONE',  ( 148.2980785574368952, 273.7871886041155562, 9.134436720559454770 ) ) ;
#63944=CARTESIAN_POINT ( 'NONE',  ( 30.18841615574984516, 197.4244531367911293, -4.594050593750046652 ) ) ;
#63948=CARTESIAN_POINT ( 'NONE',  ( 147.5848197185516142, 275.0225891520124151, 4.420251097676741736 ) ) ;
#63951=CARTESIAN_POINT ( 'NONE',  ( 58.82164138842261991, 214.7677522451419350, -5.000000000000047962 ) ) ;
#63952=CARTESIAN_POINT ( 'NONE',  ( 174.1683193666472960, 289.3678892813664447, 7.962606529223953622 ) ) ;
#63955=ORIENTED_EDGE ( 'NONE', *, *, #53150, .F. ) ;
#63956=CARTESIAN_POINT ( 'NONE',  ( 29.10614472461697133, 197.6115022471903160, -5.000000000000047962 ) ) ;
#63958=CARTESIAN_POINT ( 'NONE',  ( 202.2712651538608668, 280.3028871727136675, 16.13191389836473988 ) ) ;
#63959=CARTESIAN_POINT ( 'NONE',  ( -6.860972828079417773, 166.8458772461660544, 9.188101187500095079 ) ) ;
#63961=CARTESIAN_POINT ( 'NONE',  ( 164.3425516374517201, 252.4759456939266613, 13.51613706407178306 ) ) ;
#63962=CARTESIAN_POINT ( 'NONE',  ( 170.7811188501789559, 263.0771675258006894, 15.96733366579245583 ) ) ;
#63963=CARTESIAN_POINT ( 'NONE',  ( 192.7944000592152634, 296.7172990131160759, 11.44860011299869740 ) ) ;
#63965=FACE_OUTER_BOUND ( 'NONE', #41843, .T. ) ;
#63966=CARTESIAN_POINT ( 'NONE',  ( 183.3546644584063472, 257.9009421642305142, -2.296804517617567321 ) ) ;
#63972=CARTESIAN_POINT ( 'NONE',  ( 168.1557382078134424, 288.1736776346151601, 0.5343211543652907070 ) ) ;
#63976=EDGE_CURVE ( 'NONE', #48299, #93959, #510, .T. ) ;
#63979=EDGE_CURVE ( 'NONE', #64017, #45286, #88871, .T. ) ;
#63982=CARTESIAN_POINT ( 'NONE',  ( 207.6860335175200589, 270.9242332556395922, 6.913225035677485586 ) ) ;
#63986=CARTESIAN_POINT ( 'NONE',  ( 194.2321518193436987, 294.2270399159019121, 13.98132384850917020 ) ) ;
#63988=EDGE_LOOP ( 'NONE', ( #69454, #50038, #58272, #20769 ) ) ;
#63989=CARTESIAN_POINT ( 'NONE',  ( 158.0371712374162882, 277.6164995809708103, -9.872139935335178862 ) ) ;
#63993=CARTESIAN_POINT ( 'NONE',  ( 188.8073495538124575, 297.5103159715075662, 7.738326755456107264 ) ) ;
#63994=ORIENTED_EDGE ( 'NONE', *, *, #58563, .T. ) ;
#63995=ADVANCED_FACE ( 'NONE', ( #15002 ), #45890, .T. ) ;
#63999=CARTESIAN_POINT ( 'NONE',  ( 173.0837253472800796, 264.8280141993791972, 17.07053884509587860 ) ) ;
#64001=CARTESIAN_POINT ( 'NONE',  ( 200.7583183585857967, 282.9233878912788214, 16.96937806979494212 ) ) ;
#64002=CARTESIAN_POINT ( 'NONE',  ( 168.4098293865724827, 275.5469783040978200, -15.30805618485334385 ) ) ;
#64005=CARTESIAN_POINT ( 'NONE',  ( 150.8987980144153767, 274.7068622528165633, -8.647764889241976505 ) ) ;
#64007=CARTESIAN_POINT ( 'NONE',  ( 200.5039526449628795, 267.3497397166782434, 6.370409075474873006 ) ) ;
#64009=EDGE_CURVE ( 'NONE', #3513, #59744, #6620, .T. ) ;
#64013=CARTESIAN_POINT ( 'NONE',  ( 156.9907511051827385, 266.1419335827932287, -16.70578678711312293 ) ) ;
#64016=DIRECTION ( 'NONE',  ( -0.8660254037844387076, -0.4999999999999998890, -0.000000000000000000 ) ) ;
#64017=VERTEX_POINT ( 'NONE', #32207 ) ;
#64018=CARTESIAN_POINT ( 'NONE',  ( 168.0637158183493227, 272.4661608228503837, 15.99915743202654284 ) ) ;
#64019=CARTESIAN_POINT ( 'NONE',  ( 193.3392202435183549, 295.7736427729139450, 14.53615558183985534 ) ) ;
#64023=CARTESIAN_POINT ( 'NONE',  ( 175.0213034474378446, 290.8364490856844213, 6.509122669734152211 ) ) ;
#64025=VERTEX_POINT ( 'NONE', #94056 ) ;
#64028=CARTESIAN_POINT ( 'NONE',  ( 206.4768661561222984, 273.0185725604343361, 11.39716120335626925 ) ) ;
#64029=CARTESIAN_POINT ( 'NONE',  ( 206.4537138826727301, 273.0586734743599209, 11.45643784582899016 ) ) ;
#64030=CARTESIAN_POINT ( 'NONE',  ( 198.0792648159935538, 287.5636447432459022, 17.04758482866669667 ) ) ;
#64031=EDGE_LOOP ( 'NONE', ( #98829, #69609, #36950, #86948 ) ) ;
#64033=EDGE_CURVE ( 'NONE', #46582, #28117, #3058, .T. ) ;
#64034=CARTESIAN_POINT ( 'NONE',  ( 169.2275080599221440, 257.9151911612065078, -14.10194183318204963 ) ) ;
#64035=CARTESIAN_POINT ( 'NONE',  ( 206.2041691044954348, 273.4908977089264113, -9.455375957961031474 ) ) ;
#64036=DIRECTION ( 'NONE',  ( 0.4999999999999998890, -0.8660254037844385966, 0.000000000000000000 ) ) ;
#64038=CARTESIAN_POINT ( 'NONE',  ( 161.3644539559160478, 251.1555625431813894, 12.97746593258196413 ) ) ;
#64039=CARTESIAN_POINT ( 'NONE',  ( 171.3171204526115616, 271.4791138034659070, -17.75561031716327420 ) ) ;
#64044=CARTESIAN_POINT ( 'NONE',  ( -1.501377777706596639, 158.3932355074535678, -2.679491924311248496 ) ) ;
#64045=CARTESIAN_POINT ( 'NONE',  ( 15.08735849730845402, 189.5177522451419065, 5.000000000000046185 ) ) ;
#64046=CARTESIAN_POINT ( 'NONE',  ( 94.46399941469991290, 225.3458772461660544, 9.188101187500095079 ) ) ;
#64047=CARTESIAN_POINT ( 'NONE',  ( 196.3535209228541021, 269.2310135407589655, -12.05999164192846074 ) ) ;
#64049=CARTESIAN_POINT ( 'NONE',  ( 175.7882114856885210, 291.4026636951798537, -6.622811550496607857 ) ) ;
#64050=CARTESIAN_POINT ( 'NONE',  ( 207.8040920112677270, 270.7197499462034784, 3.100718407159808176 ) ) ;
#64051=CARTESIAN_POINT ( 'NONE',  ( 14.68175618682350780, 167.0327760586659451, 1.948934522072303157E-15 ) ) ;
#64056=ORIENTED_EDGE ( 'NONE', *, *, #62187, .T. ) ;
#64057=EDGE_CURVE ( 'NONE', #47928, #75148, #96018, .T. ) ;
#64058=CARTESIAN_POINT ( 'NONE',  ( 197.5569596757523811, 265.3403027263088916, -2.927114525079438589 ) ) ;
#64059=ADVANCED_FACE ( 'NONE', ( #51402 ), #88990, .T. ) ;
#64063=CARTESIAN_POINT ( 'NONE',  ( 193.0560632045236673, 263.9002708199371909, -4.325864479350134850 ) ) ;
#64064=CARTESIAN_POINT ( 'NONE',  ( 161.4816992964961742, 250.9524876563463067, -12.92750327687364198 ) ) ;
#64065=CARTESIAN_POINT ( 'NONE',  ( 184.2146915786734098, 285.2824563773917816, 15.08884348642498452 ) ) ;
#64067=CARTESIAN_POINT ( 'NONE',  ( 31.67681054456310719, 201.3464784336661637, 1.353441290958777525E-15 ) ) ;
#64068=CARTESIAN_POINT ( 'NONE',  ( 85.30758498749676733, 213.3927522451418213, 10.00000000000009592 ) ) ;
#64069=CARTESIAN_POINT ( 'NONE',  ( 199.5024589829807837, 277.4988332975255503, 15.16960785487432162 ) ) ;
#64072=CARTESIAN_POINT ( 'NONE',  ( 174.9671601572613326, 281.6994072225486434, -15.63500919100072473 ) ) ;
#64073=CARTESIAN_POINT ( 'NONE',  ( -7.320788502016136512, 157.3923013555410080, 4.594050593750050204 ) ) ;
#64075=FACE_OUTER_BOUND ( 'NONE', #96717, .T. ) ;
#64076=AXIS2_PLACEMENT_3D ( 'NONE', #59038, #19099, #90007 ) ;
#64078=CARTESIAN_POINT ( 'NONE',  ( 148.0826818691893152, 274.1602666119424043, -9.371267383421741926 ) ) ;
#64080=CARTESIAN_POINT ( 'NONE',  ( 204.2133777088835700, 276.9390495533970693, 13.75768580338462144 ) ) ;
#64081=CARTESIAN_POINT ( 'NONE',  ( 191.3413020738616410, 299.2341385521244774, -8.295023558158421295 ) ) ;
#64082=CARTESIAN_POINT ( 'NONE',  ( 164.2672861321391053, 246.1277097281173667, -2.417001679502223777 ) ) ;
#64083=EDGE_LOOP ( 'NONE', ( #25906, #63916, #9822, #82766 ) ) ;
#64084=( BOUNDED_CURVE ( )  B_SPLINE_CURVE ( 2, ( #59065, #36286, #28189, #67691, #51995, #21117, #99602, #60563, #97623 ),
 .UNSPECIFIED., .F., .T. ) 
 B_SPLINE_CURVE_WITH_KNOTS ( ( 3, 2, 2, 2, 3 ),
 ( 0.3750000000000000000, 0.3763440860215053752, 0.3790322580645161255, 0.3817204301075268758, 0.3830645161290322509 ),
 .UNSPECIFIED. ) 
 CURVE ( )  GEOMETRIC_REPRESENTATION_ITEM ( )  RATIONAL_B_SPLINE_CURVE ( ( 0.9330127018922194093, 0.9330127018922194093, 1.000000000000000000, 0.8660254037844387076, 1.000000000000000000, 0.8660254037844387076, 1.000000000000000000, 0.9330127018922194093, 0.9330127018922194093 ) ) 
 REPRESENTATION_ITEM ( '' )  );
#64085=CARTESIAN_POINT ( 'NONE',  ( 181.1902717559939617, 268.1300628243799338, 16.16177986835113600 ) ) ;
#64086=CARTESIAN_POINT ( 'NONE',  ( 116.7102005222951817, 232.0643266524159856, -9.188101187500093303 ) ) ;
#64089=CARTESIAN_POINT ( 'NONE',  ( 150.9690640482209574, 269.7773037333962520, 13.74186519101368020 ) ) ;
#64090=CARTESIAN_POINT ( 'NONE',  ( 195.9359860111818250, 291.2759125279654882, 17.49638312768267312 ) ) ;
#64092=CARTESIAN_POINT ( 'NONE',  ( 150.9724169730098424, 269.1550985917100434, -14.05609013274548857 ) ) ;
#64094=CARTESIAN_POINT ( 'NONE',  ( 190.0093170351423169, 261.0487610539813659, -4.602376092151496678 ) ) ;
#64095=CARTESIAN_POINT ( 'NONE',  ( 149.1429535397850827, 272.3238222086447990, -12.91457852089092384 ) ) ;
#64096=CARTESIAN_POINT ( 'NONE',  ( 190.0435459140688295, 300.0465545779896388, 4.679742701079471878 ) ) ;
#64097=CARTESIAN_POINT ( 'NONE',  ( 174.3263853019044802, 290.4440848627237983, -1.067528433193902115 ) ) ;
#64098=CARTESIAN_POINT ( 'NONE',  ( 194.5504213170283094, 270.8435279203088157, -14.24376176104693137 ) ) ;
#64099=ORIENTED_EDGE ( 'NONE', *, *, #61818, .T. ) ;
#64101=CARTESIAN_POINT ( 'NONE',  ( 175.6701573864172587, 278.5910633658755842, 15.45497855305149137 ) ) ;
#64102=CARTESIAN_POINT ( 'NONE',  ( 165.5507010442709657, 269.3226483685077710, -16.52342293238164217 ) ) ;
#64103=CARTESIAN_POINT ( 'NONE',  ( 200.2567476884168514, 272.3152526771139037, 12.76741103404060951 ) ) ;
#64104=CARTESIAN_POINT ( 'NONE',  ( 155.9844261609601688, 261.1831564919472157, 17.17349893481298650 ) ) ;
#64106=CARTESIAN_POINT ( 'NONE',  ( 148.2541920228352126, 274.5676210274151003, 6.886971996321211265 ) ) ;
#64107=ORIENTED_EDGE ( 'NONE', *, *, #5651, .T. ) ;
#64108=CARTESIAN_POINT ( 'NONE',  ( 164.9054020227948740, 260.6345827824168282, 17.20773913071212391 ) ) ;
#64110=CARTESIAN_POINT ( 'NONE',  ( 192.6861190271732767, 288.4908837155273886, -15.91154857267342315 ) ) ;
#64112=CARTESIAN_POINT ( 'NONE',  ( 167.8373819884664897, 280.7956131110225897, 12.19395811520589490 ) ) ;
#64113=CARTESIAN_POINT ( 'NONE',  ( 148.0637215040603394, 274.1931069276759558, -7.795633835291665648 ) ) ;
#64114=CARTESIAN_POINT ( 'NONE',  ( 165.5752708168755305, 245.8622137986321832, -1.085626278946311585 ) ) ;
#64115=ORIENTED_EDGE ( 'NONE', *, *, #28716, .F. ) ;
#64118=DIRECTION ( 'NONE',  ( 0.4999999999999998890, -0.8660254037844385966, 0.000000000000000000 ) ) ;
#64119=B_SPLINE_CURVE_WITH_KNOTS ( 'NONE', 3,
 ( #97337, #73525, #34512, #27905 ),
 .UNSPECIFIED., .F., .F.,
 ( 4, 4 ),
 ( 0.000000000000000000, 0.0009678251226235170916 ),
 .UNSPECIFIED. ) ;
#64123=CIRCLE ( 'NONE', #93291, 17.82106496071138935 ) ;
#64124=CARTESIAN_POINT ( 'NONE',  ( 24.59328401069779702, 196.5530062829863311, -4.648177544792955347E-16 ) ) ;
#64128=CARTESIAN_POINT ( 'NONE',  ( 175.4420607406781585, 259.0809407130348632, 12.51945158449231776 ) ) ;
#64131=EDGE_LOOP ( 'NONE', ( #74395, #42740, #71614, #47932 ) ) ;
#64137=CARTESIAN_POINT ( 'NONE',  ( 164.9590787296926067, 244.9294898008548387, -2.278052160087662870 ) ) ;
#64138=CARTESIAN_POINT ( 'NONE',  ( 147.2164090273763009, 275.6606951871798969, -7.081586236283015090 ) ) ;
#64139=CARTESIAN_POINT ( 'NONE',  ( 161.2311971278517433, 276.6540853535840370, -12.65640296859774239 ) ) ;
#64140=CARTESIAN_POINT ( 'NONE',  ( 193.1169444172380167, 296.1586357973259283, -13.13373377033755318 ) ) ;
#64141=CARTESIAN_POINT ( 'NONE',  ( 201.0844796915553161, 282.3584598911111812, -16.59562674965125950 ) ) ;
#64143=CARTESIAN_POINT ( 'NONE',  ( 183.4841190084916605, 284.4425740377230909, -16.26519031814292759 ) ) ;
#64144=CARTESIAN_POINT ( 'NONE',  ( 125.2893514524760548, 233.9548013555409796, -4.594050593750042211 ) ) ;
#64147=VERTEX_POINT ( 'NONE', #73230 ) ;
#64151=CARTESIAN_POINT ( 'NONE',  ( 200.7003661377988522, 274.4207182511248106, 13.44867137911134414 ) ) ;
#64152=CARTESIAN_POINT ( 'NONE',  ( 177.5731418194271498, 253.4711720865799975, 1.377694960479720176 ) ) ;
#64153=CARTESIAN_POINT ( 'NONE',  ( 171.3124147562957944, 287.8937356591647472, -4.632457808386030607 ) ) ;
#64155=CARTESIAN_POINT ( 'NONE',  ( 156.7733467512841798, 279.4475125893658856, 7.423369370622811658 ) ) ;
#64156=CARTESIAN_POINT ( 'NONE',  ( 152.6740002182599767, 266.2078699576288159, -17.16212636348624088 ) ) ;
#64157=CARTESIAN_POINT ( 'NONE',  ( 173.3566611292251594, 287.3586671341846568, -9.788589206785145436 ) ) ;
#64159=CARTESIAN_POINT ( 'NONE',  ( 171.5128195627625018, 280.0544377941017160, 13.82747465963291589 ) ) ;
#64160=CARTESIAN_POINT ( 'NONE',  ( 177.0796805162949568, 255.9639923578327512, -7.284429273897122137 ) ) ;
#64161=ORIENTED_EDGE ( 'NONE', *, *, #67390, .T. ) ;
#64162=DIRECTION ( 'NONE',  ( -0.8660254037844387076, -0.4999999999999998890, -0.000000000000000000 ) ) ;
#64163=EDGE_CURVE ( 'NONE', #43672, #85978, #83997, .T. ) ;
#64164=B_SPLINE_CURVE_WITH_KNOTS ( 'NONE', 3,
 ( #4022, #74447, #97738, #3546 ),
 .UNSPECIFIED., .F., .F.,
 ( 4, 4 ),
 ( 0.01475334623982018159, 0.02347991049736522506 ),
 .UNSPECIFIED. ) ;
#64167=CARTESIAN_POINT ( 'NONE',  ( 164.0279908745103796, 278.0166827825981954, 13.19491288999882350 ) ) ;
#64169=CARTESIAN_POINT ( 'NONE',  ( 203.2959387668414308, 268.8872303932580508, -2.890917808293821611 ) ) ;
#64170=CARTESIAN_POINT ( 'NONE',  ( 191.4144919117340180, 299.1073700343318365, -9.990130103278371365 ) ) ;
#64172=CARTESIAN_POINT ( 'NONE',  ( 162.6476498368881494, 248.9330020812748785, 10.75824100428386743 ) ) ;
#64173=CARTESIAN_POINT ( 'NONE',  ( 164.6230904413119447, 284.1771003334332590, -6.922202500276794623 ) ) ;
#64174=CARTESIAN_POINT ( 'NONE',  ( 154.7022681145324441, 277.6819014155639138, -9.051459774888167331 ) ) ;
#64175=CARTESIAN_POINT ( 'NONE',  ( 153.2283961777204695, 265.2476279883323400, -17.66880461074566000 ) ) ;
#64178=ADVANCED_FACE ( 'NONE', ( #29117 ), #58494, .T. ) ;
#64179=CARTESIAN_POINT ( 'NONE',  ( 193.4969218094394989, 276.1359876676401086, -16.38138015012474824 ) ) ;
#64182=CARTESIAN_POINT ( 'NONE',  ( 64.47116044126103418, 196.4824982072973683, 3.021315404115420679E-15 ) ) ;
#64184=CARTESIAN_POINT ( 'NONE',  ( 168.2008345946905479, 248.1884056956802453, -5.064766917302788052 ) ) ;
#64185=CARTESIAN_POINT ( 'NONE',  ( -7.673045192009834814, 172.5024278399160664, -9.188101187500093303 ) ) ;
#64186=CARTESIAN_POINT ( 'NONE',  ( 96.27750042569734035, 217.2048013555409796, 4.594050593750051981 ) ) ;
#64189=CARTESIAN_POINT ( 'NONE',  ( -12.80041588338334790, 174.9637435831424739, 2.679491924311258266 ) ) ;
#64192=CARTESIAN_POINT ( 'NONE',  ( 160.9048106541811762, 281.6641488084669618, 5.546786390428459335 ) ) ;
#64194=CARTESIAN_POINT ( 'NONE',  ( 162.7459776558209228, 248.7626933030860812, -9.895605163646791880 ) ) ;
#64195=CARTESIAN_POINT ( 'NONE',  ( 161.6965001858482083, 250.5804416024775492, 12.67320179257150414 ) ) ;
#64199=CARTESIAN_POINT ( 'NONE',  ( 147.7256246083515521, 244.5494855054051868, -2.679491924311248496 ) ) ;
#64200=CARTESIAN_POINT ( 'NONE',  ( 86.10144160763246646, 220.5177522451418497, -10.00000000000009592 ) ) ;
#64202=CARTESIAN_POINT ( 'NONE',  ( 40.22915850269944116, 194.0333772461660544, 9.188101187500095079 ) ) ;
#64205=CARTESIAN_POINT ( 'NONE',  ( 65.93911412966747321, 215.0024278399160949, 9.188101187500095079 ) ) ;
#64206=CARTESIAN_POINT ( 'NONE',  ( 161.8926315922002743, 250.2407320417157166, -13.77020595223768495 ) ) ;
#64207=CARTESIAN_POINT ( 'NONE',  ( 107.3857722915638249, 221.2592609112380160, 2.679491924311254714 ) ) ;
#64210=CARTESIAN_POINT ( 'NONE',  ( 162.8931802014337791, 249.0911889412991229, -10.32038157250286048 ) ) ;
#64213=CARTESIAN_POINT ( 'NONE',  ( 148.9285945872975390, 272.6951028054104427, -12.01265727652413240 ) ) ;
#64214=EDGE_LOOP ( 'NONE', ( #23965, #18933, #88131, #60249 ) ) ;
#64216=CARTESIAN_POINT ( 'NONE',  ( 75.92590343676303632, 205.4548013555409796, -4.594050593750042211 ) ) ;
#64219=CARTESIAN_POINT ( 'NONE',  ( -22.42236680055709641, 157.8615022471902591, 0.000000000000000000 ) ) ;
#64220=FACE_OUTER_BOUND ( 'NONE', #62229, .T. ) ;
#64225=CARTESIAN_POINT ( 'NONE',  ( 133.0291931787496935, 237.6115022471901739, -5.000000000000041744 ) ) ;
#64226=CARTESIAN_POINT ( 'NONE',  ( 200.8432122835317841, 282.7763473000181307, 17.15137370990203891 ) ) ;
#64231=CARTESIAN_POINT ( 'NONE',  ( 202.9972156839127990, 279.0455039708822937, 16.77197898838388213 ) ) ;
#64232=CARTESIAN_POINT ( 'NONE',  ( 176.1478293119272109, 282.8961218008153651, 15.39372813948029339 ) ) ;
#64235=CARTESIAN_POINT ( 'NONE',  ( 173.9559965888401507, 252.0681728601754799, -0.2505477230817378387 ) ) ;
#64237=EDGE_CURVE ( 'NONE', #7544, #79399, #29577, .T. ) ;
#64239=CARTESIAN_POINT ( 'NONE',  ( 194.3442947553755005, 294.0328026529847421, -15.97648891113594871 ) ) ;
#64240=B_SPLINE_CURVE_WITH_KNOTS ( 'NONE', 3,
 ( #11983, #2902, #42839, #82425 ),
 .UNSPECIFIED., .F., .F.,
 ( 4, 4 ),
 ( 0.01015053972906150397, 0.01849756262824885783 ),
 .UNSPECIFIED. ) ;
#64249=DIRECTION ( 'NONE',  ( -0.8660254037844387076, -0.4999999999999998890, -0.000000000000000000 ) ) ;
#64251=ORIENTED_EDGE ( 'NONE', *, *, #26253, .T. ) ;
#64254=CARTESIAN_POINT ( 'NONE',  ( 204.8523313866422484, 275.8323493198358847, 14.65426965484541100 ) ) ;
#64255=CARTESIAN_POINT ( 'NONE',  ( 148.4083960970861256, 273.5961130204771052, -8.574185186226726429 ) ) ;
#64257=CARTESIAN_POINT ( 'NONE',  ( 155.6126298223767890, 261.1180141786725244, 18.15400560664037855 ) ) ;
#64258=CARTESIAN_POINT ( 'NONE',  ( 185.3642616951140383, 292.5731700952273968, -11.69566502907712469 ) ) ;
#64259=LINE ( 'NONE', #89129, #58118 ) ;
#64260=CARTESIAN_POINT ( 'NONE',  ( 207.3688238152966790, 271.4736565765441583, -4.151733834809656187 ) ) ;
#64261=CARTESIAN_POINT ( 'NONE',  ( 206.4466068143230757, 270.6103183474565981, 2.450360801254404475 ) ) ;
#64263=CARTESIAN_POINT ( 'NONE',  ( 85.88519558028406209, 211.2048013555409796, 4.594050593750051981 ) ) ;
#64264=ORIENTED_EDGE ( 'NONE', *, *, #50491, .F. ) ;
#64268=ORIENTED_EDGE ( 'NONE', *, *, #56543, .T. ) ;
#64269=CARTESIAN_POINT ( 'NONE',  ( 167.7949682406799639, 266.8640267017669885, -17.72765487805554585 ) ) ;
#64276=B_SPLINE_SURFACE_WITH_KNOTS ( 'NONE', 3, 1, ( 
 ( #96907, #58830 ),
 ( #66456, #97381 ),
 ( #27948, #20370 ),
 ( #51241, #82208 ),
 ( #43644, #66941 ),
 ( #97871, #28443 ),
 ( #99855, #60324 ),
 ( #45137, #91779 ),
 ( #52728, #82706 ),
 ( #51764, #91280 ),
 ( #52242, #61328 ),
 ( #38019, #46117 ),
 ( #21357, #68434 ),
 ( #28960, #98373 ),
 ( #21846, #22344 ),
 ( #13273, #44626 ),
 ( #53723, #77033 ),
 ( #83690, #75069 ),
 ( #6654, #53240 ),
 ( #83186, #22838 ),
 ( #14743, #13746 ),
 ( #14251, #84195 ),
 ( #45624, #37041 ),
 ( #76553, #6147 ),
 ( #75560, #67951 ),
 ( #29447, #90304 ),
 ( #98869, #67443 ),
 ( #76078, #84682 ),
 ( #68930, #30440 ),
 ( #60817, #37528 ),
 ( #44135, #99363 ),
 ( #7132, #92289 ),
 ( #15222, #7639 ),
 ( #36538, #38531 ) ),
 .UNSPECIFIED., .T., .F., .F.,
 ( 4, 2, 2, 2, 2, 2, 2, 2, 2, 2, 2, 2, 2, 2, 2, 2, 4 ),
 ( 2, 2 ),
 ( 0.000000000000000000, 0.06250000000000000000, 0.1250000000000000000, 0.1875000000000000000, 0.2500000000000000000, 0.3125000000000000000, 0.3750000000000000000, 0.4375000000000000000, 0.5000000000000000000, 0.5625000000000000000, 0.6250000000000000000, 0.6875000000000000000, 0.7500000000000000000, 0.8125000000000000000, 0.8750000000000000000, 0.9375000000000000000, 1.000000000000000000 ),
 ( 0.000000000000000000, 1.000000000000000000 ),
 .UNSPECIFIED. ) ;
#64279=CARTESIAN_POINT ( 'NONE',  ( 162.4419666585835387, 249.2892557963607203, 10.75794555938079711 ) ) ;
#64280=CARTESIAN_POINT ( 'NONE',  ( 100.7430306879021202, 216.7202760586659736, -5.415160957724236172E-17 ) ) ;
#64283=ORIENTED_EDGE ( 'NONE', *, *, #56931, .T. ) ;
#64285=CARTESIAN_POINT ( 'NONE',  ( 200.8245636081238104, 282.8086477533188940, -18.30100074294778523 ) ) ;
#64287=FACE_OUTER_BOUND ( 'NONE', #16401, .T. ) ;
#64290=CARTESIAN_POINT ( 'NONE',  ( -12.62545442379354554, 163.5177522451418781, -10.00000000000009592 ) ) ;
#64295=CARTESIAN_POINT ( 'NONE',  ( 160.7563763136490991, 275.4827502265731027, 13.67813126869715745 ) ) ;
#64296=CARTESIAN_POINT ( 'NONE',  ( 206.5081929095101998, 272.9643130319303737, -9.215516226794479238 ) ) ;
#64300=CARTESIAN_POINT ( 'NONE',  ( 198.2505066714982149, 285.2670451491296149, 0.000000000000000000 ) ) ;
#64301=ORIENTED_EDGE ( 'NONE', *, *, #67909, .T. ) ;
#64302=CARTESIAN_POINT ( 'NONE',  ( 149.0237174825091415, 274.5263358477994871, 9.114370506038131481 ) ) ;
#64303=CARTESIAN_POINT ( 'NONE',  ( 200.5810378487751393, 283.2304467414622877, 18.38516374632547112 ) ) ;
#64307=CARTESIAN_POINT ( 'NONE',  ( 202.4027882010644248, 280.0750825725909863, -15.81779609180605739 ) ) ;
#64310=B_SPLINE_CURVE_WITH_KNOTS ( 'NONE', 3,
 ( #26197, #33813, #41377, #88056 ),
 .UNSPECIFIED., .F., .F.,
 ( 4, 4 ),
 ( 0.02623590123331938015, 0.03547298285468161727 ),
 .UNSPECIFIED. ) ;
#64312=CARTESIAN_POINT ( 'NONE',  ( 165.0532575723395041, 244.7663672603923715, -2.144843157699870773 ) ) ;
#64316=CARTESIAN_POINT ( 'NONE',  ( 169.6737827488630330, 273.3960839505391505, 15.97819652875916496 ) ) ;
#64318=CARTESIAN_POINT ( 'NONE',  ( 161.1037873772034743, 273.3404041746127291, -15.20289387583265928 ) ) ;
#64321=CARTESIAN_POINT ( 'NONE',  ( 3.585285057187872493, 179.0024278399160949, 9.188101187500095079 ) ) ;
#64324=CARTESIAN_POINT ( 'NONE',  ( 160.2808189788048026, 253.4324493631022222, -14.69790056671751977 ) ) ;
#64327=CARTESIAN_POINT ( 'NONE',  ( 27.69859311986958872, 195.9869531367911293, 4.594050593750046652 ) ) ;
#64329=CARTESIAN_POINT ( 'NONE',  ( -22.42236680055709641, 157.8615022471902591, 0.000000000000000000 ) ) ;
#64332=CARTESIAN_POINT ( 'NONE',  ( 178.5672342955430736, 291.6450058653585415, 6.041949026109024956 ) ) ;
#64333=CARTESIAN_POINT ( 'NONE',  ( 98.80083580102481733, 239.3967562850347122, -4.648177544792955347E-16 ) ) ;
#64334=CARTESIAN_POINT ( 'NONE',  ( 196.4226663688725978, 290.4329574213987257, 16.56158086743572611 ) ) ;
#64335=CARTESIAN_POINT ( 'NONE',  ( 178.9629750711524423, 278.2817214550511835, -16.74959616653973171 ) ) ;
#64337=CARTESIAN_POINT ( 'NONE',  ( 190.1149742248946382, 298.7024877295776264, -8.095583997651624841 ) ) ;
#64339=CARTESIAN_POINT ( 'NONE',  ( 82.29453827371133912, 204.9865022471901170, 1.119607411625061291E-15 ) ) ;
#64341=CARTESIAN_POINT ( 'NONE',  ( -17.42236680055705023, 149.2012482093457777, 0.000000000000000000 ) ) ;
#64342=CARTESIAN_POINT ( 'NONE',  ( 48.99766571601688270, 199.0958772461660544, -9.188101187500095079 ) ) ;
#64343=CARTESIAN_POINT ( 'NONE',  ( 159.3767386493506137, 254.5983864451355032, 15.47015898230477760 ) ) ;
#64346=CARTESIAN_POINT ( 'NONE',  ( 150.9584389135710865, 269.1793093008492406, -15.82751450793727699 ) ) ;
#64349=CARTESIAN_POINT ( 'NONE',  ( 169.0845258451994084, 285.4515155598613774, 7.530877004957813980 ) ) ;
#64350=LINE ( 'NONE', #68579, #32856 ) ;
#64352=CARTESIAN_POINT ( 'NONE',  ( 93.96783902534114929, 218.3927522451417929, -10.00000000000009237 ) ) ;
#64354=CARTESIAN_POINT ( 'NONE',  ( 202.8167949821795446, 279.3580017930215149, 15.61966256214195070 ) ) ;
#64355=CARTESIAN_POINT ( 'NONE',  ( 197.0184425104562820, 289.4010428742387262, -16.90752553128928426 ) ) ;
#64356=CARTESIAN_POINT ( 'NONE',  ( 204.5840280042472159, 276.2970644099866036, 14.65559382949596667 ) ) ;
#64360=CARTESIAN_POINT ( 'NONE',  ( 171.7156989675575289, 252.4012571563561949, 8.733959727973424236 ) ) ;
#64363=CARTESIAN_POINT ( 'NONE',  ( 178.8612031755637020, 282.6164454953549807, 15.88195292133873160 ) ) ;
#64365=CARTESIAN_POINT ( 'NONE',  ( 191.2056514706806070, 299.4690922889112699, 7.290007621276087590 ) ) ;
#64367=CARTESIAN_POINT ( 'NONE',  ( 170.0730192398974339, 270.7478067695028017, 17.76568905885011418 ) ) ;
#64368=ADVANCED_FACE ( 'NONE', ( #11460, #34234 ), #10950, .F. ) ;
#64370=ORIENTED_EDGE ( 'NONE', *, *, #72996, .T. ) ;
#64373=CARTESIAN_POINT ( 'NONE',  ( 151.3542526322075901, 269.2885850756041464, -14.28695254860580199 ) ) ;
#64374=CARTESIAN_POINT ( 'NONE',  ( 196.5475899070771675, 290.2165835061676944, -17.89382743182097002 ) ) ;
#64376=CARTESIAN_POINT ( 'NONE',  ( 152.7375212135632125, 266.0978483664162582, -16.47968945089317572 ) ) ;
#64382=EDGE_CURVE ( 'NONE', #70225, #8907, #74258, .T. ) ;
#64383=CARTESIAN_POINT ( 'NONE',  ( 119.3082767336485404, 233.5643266524159856, -9.188101187500093303 ) ) ;
#64384=CARTESIAN_POINT ( 'NONE',  ( 183.9133946104620918, 288.6285713628617486, -13.17071474273308951 ) ) ;
#64386=CARTESIAN_POINT ( 'NONE',  ( 201.4968513823492060, 281.2160229052847171, 16.24425496473199004 ) ) ;
#64387=VERTEX_POINT ( 'NONE', #72256 ) ;
#64389=CARTESIAN_POINT ( 'NONE',  ( 168.9579038699606315, 279.3139280689009070, 15.08363371378442608 ) ) ;
#64391=CARTESIAN_POINT ( 'NONE',  ( 67.34675250658217749, 203.5643266524159856, -9.188101187500093303 ) ) ;
#64394=CARTESIAN_POINT ( 'NONE',  ( 191.2645787786270262, 299.3670271975948367, 7.309947121636420242 ) ) ;
#64395=CARTESIAN_POINT ( 'NONE',  ( 198.5386315514599858, 286.7679982181109608, 17.03868888912368718 ) ) ;
#64396=CARTESIAN_POINT ( 'NONE',  ( 173.2942936627640620, 271.3368914396714331, 16.42383385673190332 ) ) ;
#64403=ORIENTED_EDGE ( 'NONE', *, *, #42003, .F. ) ;
#64404=CARTESIAN_POINT ( 'NONE',  ( 173.7340210619385914, 260.6390436719518675, -13.93636029417189093 ) ) ;
#64405=CARTESIAN_POINT ( 'NONE',  ( 174.2364561098118259, 277.1437767697490813, -15.63526590635042446 ) ) ;
#64406=CARTESIAN_POINT ( 'NONE',  ( 160.5819451565263023, 258.3323579126541745, -16.82900739823111991 ) ) ;
#64407=CARTESIAN_POINT ( 'NONE',  ( 207.0171084425618346, 270.8969818057616408, 2.452340968668444532 ) ) ;
#64408=CARTESIAN_POINT ( 'NONE',  ( 190.2389970918280540, 301.1433867864428748, 4.601241515604689525 ) ) ;
#64410=CARTESIAN_POINT ( 'NONE',  ( 180.7126655808842202, 271.3309753198433327, 16.61443135770589308 ) ) ;
#64411=CARTESIAN_POINT ( 'NONE',  ( 164.7762319088960794, 245.2461897844768828, 2.994040459560653122 ) ) ;
#64412=CARTESIAN_POINT ( 'NONE',  ( 164.1893796463498632, 253.9140536989919497, 14.56309422521135843 ) ) ;
#64413=FACE_OUTER_BOUND ( 'NONE', #24545, .T. ) ;
#64415=CARTESIAN_POINT ( 'NONE',  ( 137.1160976468485444, 237.7202760586660020, -5.415160957724236172E-17 ) ) ;
#64416=ORIENTED_EDGE ( 'NONE', *, *, #34279, .T. ) ;
#64420=CARTESIAN_POINT ( 'NONE',  ( 182.7913689746213777, 285.6300500007765777, -15.59955371092600807 ) ) ;
#64422=CARTESIAN_POINT ( 'NONE',  ( 175.2976070117660186, 253.4435804238109426, 4.989098000593277682 ) ) ;
#64427=CARTESIAN_POINT ( 'NONE',  ( 147.6346879868728479, 275.5076572718856482, 2.918840859857055658 ) ) ;
#64428=CARTESIAN_POINT ( 'NONE',  ( 181.9401144352162021, 260.5691112182036591, 10.07005861877500763 ) ) ;
#64430=CARTESIAN_POINT ( 'NONE',  ( 141.5001777056247931, 246.3768266524160140, 9.188101187500096856 ) ) ;
#64431=EDGE_CURVE ( 'NONE', #70505, #39044, #48975, .T. ) ;
#64433=FACE_OUTER_BOUND ( 'NONE', #21529, .T. ) ;
#64434=CARTESIAN_POINT ( 'NONE',  ( 177.6699396433555762, 293.4499100638861364, -3.987850357589190153 ) ) ;
#64435=CARTESIAN_POINT ( 'NONE',  ( 65.10058588945754821, 199.2048013555409796, 4.594050593750051981 ) ) ;
#64438=CARTESIAN_POINT ( 'NONE',  ( 205.4103625296683617, 274.8658110279089897, -13.38953657917851814 ) ) ;
#64439=CARTESIAN_POINT ( 'NONE',  ( 192.5260769942808281, 296.7927711323272888, 11.16196026814283471 ) ) ;
#64440=CARTESIAN_POINT ( 'NONE',  ( 171.1373347109045824, 259.7557668617522495, 15.18341589746758480 ) ) ;
#64441=CARTESIAN_POINT ( 'NONE',  ( 154.9517153487096550, 280.5398731376675414, -0.8905349252829396489 ) ) ;
#64442=CARTESIAN_POINT ( 'NONE',  ( 172.6345960983117322, 287.6965781455015190, -8.272603404180184583 ) ) ;
#64443=CARTESIAN_POINT ( 'NONE',  ( 155.0619429961492983, 262.0718317407570339, -17.08853361476647592 ) ) ;
#64444=CARTESIAN_POINT ( 'NONE',  ( 157.2429883677972100, 271.5286301573580658, -14.65303208119756562 ) ) ;
#64445=CARTESIAN_POINT ( 'NONE',  ( 112.1543725048142903, 248.8927522451419634, 2.944929066748280225E-16 ) ) ;
#64447=EDGE_LOOP ( 'NONE', ( #66368, #45832, #54424, #48760 ) ) ;
#64448=EDGE_CURVE ( 'NONE', #67853, #41536, #69409, .T. ) ;
#64449=CARTESIAN_POINT ( 'NONE',  ( 159.2951220875037848, 257.7226857971661502, -17.27556336337253740 ) ) ;
#64450=CARTESIAN_POINT ( 'NONE',  ( -4.533703103291246705, 174.3149278399161233, 9.188101187500093303 ) ) ;
#64451=CARTESIAN_POINT ( 'NONE',  ( 37.63108229134613225, 192.5333772461660544, 9.188101187500095079 ) ) ;
#64454=CARTESIAN_POINT ( 'NONE',  ( 180.9701587135972431, 266.4289169444708705, -14.70082405781458945 ) ) ;
#64455=CARTESIAN_POINT ( 'NONE',  ( 71.35865581505748878, 223.5530062829863027, -4.648177544792955347E-16 ) ) ;
#64456=CARTESIAN_POINT ( 'NONE',  ( 190.7908437487391780, 300.1875603386860689, -4.317984972589949955 ) ) ;
#64459=CARTESIAN_POINT ( 'NONE',  ( 61.41971759977600698, 196.2677522451418213, -5.000000000000041744 ) ) ;
#64461=CARTESIAN_POINT ( 'NONE',  ( 184.7298463175202698, 257.7777764843742148, 1.366536233435324821 ) ) ;
#64463=CARTESIAN_POINT ( 'NONE',  ( 171.3171204526115616, 271.4791138034659070, -17.75561031716327420 ) ) ;
#64464=CARTESIAN_POINT ( 'NONE',  ( 161.4023172760800833, 267.9375969907274566, 17.21476449095039030 ) ) ;
#64465=CARTESIAN_POINT ( 'NONE',  ( 43.32339510341152788, 202.4865022471903160, -10.00000000000009415 ) ) ;
#64466=B_SPLINE_CURVE_WITH_KNOTS ( 'NONE', 3,
 ( #94750, #96756, #26327, #81069, #72946, #33419, #17729, #3052, #87696, #56713, #64318, #4507, #3539, #25838, #42013, #57201, #65316, #25312, #49124, #19734, #80060, #72446, #33940, #27324, #96255, #26820, #64826, #95771, #57700, #88677, #50115, #11632, #58208, #50600, #12119, #42984, #35407, #59696, #74440, #28809, #22204, #75421, #97247, #74928, #67300, #27813, #5511, #83045 ),
 .UNSPECIFIED., .F., .F.,
 ( 4, 2, 2, 2, 2, 2, 2, 2, 2, 2, 2, 2, 2, 2, 2, 2, 2, 2, 2, 2, 2, 2, 2, 4 ),
 ( 0.002425426540219128169, 0.002845973489409292512, 0.003056246964004374900, 0.003161383701301915660, 0.003266520438599456854, 0.003371657175896998048, 0.003476793913194539242, 0.003687067387789621196, 0.004107614336979621174, 0.004948708235359621128, 0.005789802133739620216, 0.006630896032119620170, 0.007051442981309627087, 0.007471989930499632268, 0.007577126667797215095, 0.007629695036445971815, 0.007682263405094728534, 0.007734831773743485253, 0.007787400142392240238, 0.007892536879689727655, 0.008102810354284695551, 0.008313083828879661713, 0.008733630778069562811, 0.009154177727259465644 ),
 .UNSPECIFIED. ) ;
#64468=CARTESIAN_POINT ( 'NONE',  ( 202.6070187115982719, 279.7213449518906145, 15.56322169823762280 ) ) ;
#64470=CARTESIAN_POINT ( 'NONE',  ( 8.727484440040480962, 175.8458772461660828, 9.188101187500095079 ) ) ;
#64472=CARTESIAN_POINT ( 'NONE',  ( 163.9905008462251317, 247.0786441245412561, 6.065918779697442531 ) ) ;
#64473=CARTESIAN_POINT ( 'NONE',  ( 170.4606321698994407, 263.6007259650322680, 15.80273850856594997 ) ) ;
#64474=CARTESIAN_POINT ( 'NONE',  ( 152.9920137376499838, 265.6570543845515431, 16.15798175643282164 ) ) ;
#64476=CARTESIAN_POINT ( 'NONE',  ( 184.0255633751473852, 258.2697744397484598, -2.304790711699857830 ) ) ;
#64479=CARTESIAN_POINT ( 'NONE',  ( 196.2421909983451940, 290.7455499326673021, -17.31908925000307065 ) ) ;
#64481=VECTOR ( 'NONE', #89253, 1000.000000000000000 ) ;
#64483=CARTESIAN_POINT ( 'NONE',  ( 167.3422145247286039, 287.9343817845129934, 0.5404251914103093135 ) ) ;
#64485=CARTESIAN_POINT ( 'NONE',  ( 206.9809521314431606, 272.1454700397959527, 9.518650961382352449 ) ) ;
#64486=CARTESIAN_POINT ( 'NONE',  ( 152.9566069573676543, 278.2300974794858917, -4.664778606640360259 ) ) ;
#64487=CARTESIAN_POINT ( 'NONE',  ( 76.55480823776410659, 226.5530062829863027, -4.648177544792955347E-16 ) ) ;
#64488=CARTESIAN_POINT ( 'NONE',  ( 159.9788992190088948, 253.5554137441726255, -15.81862932303382330 ) ) ;
#64489=ORIENTED_EDGE ( 'NONE', *, *, #43447, .T. ) ;
#64490=CARTESIAN_POINT ( 'NONE',  ( 153.3616370783189211, 265.0168479788495688, 17.48287904751960653 ) ) ;
#64491=CARTESIAN_POINT ( 'NONE',  ( 164.7694554770609159, 245.2579269087094076, -3.003635650077957742 ) ) ;
#64497=ORIENTED_EDGE ( 'NONE', *, *, #20714, .F. ) ;
#64498=CARTESIAN_POINT ( 'NONE',  ( 129.9777503372646095, 257.3967562850347122, -4.648177544792955347E-16 ) ) ;
#64500=ORIENTED_EDGE ( 'NONE', *, *, #76532, .T. ) ;
#64502=CARTESIAN_POINT ( 'NONE',  ( 188.9968840092409437, 297.1838958854766588, 7.940645936764939350 ) ) ;
#64504=FACE_OUTER_BOUND ( 'NONE', #44518, .T. ) ;
#64511=CARTESIAN_POINT ( 'NONE',  ( 174.5422266480219662, 267.5925051635639420, 17.37569662752725463 ) ) ;
#64512=CARTESIAN_POINT ( 'NONE',  ( 206.4943150373521803, 272.9883502116088039, 11.34100825923693101 ) ) ;
#64513=CARTESIAN_POINT ( 'NONE',  ( 151.4015714417470519, 275.0754632453579802, -8.499728915061472989 ) ) ;
#64516=CARTESIAN_POINT ( 'NONE',  ( 171.4187126090420747, 256.0395575307684339, -11.60209380571112625 ) ) ;
#64517=CARTESIAN_POINT ( 'NONE',  ( 203.0535368433499457, 278.9479528611958585, 16.46202213522710167 ) ) ;
#64520=CARTESIAN_POINT ( 'NONE',  ( 156.7755893566837244, 266.6085710678392502, -16.22358508212092687 ) ) ;
#64521=EDGE_LOOP ( 'NONE', ( #71369, #9103, #28942, #81123, #64370 ) ) ;
#64522=CARTESIAN_POINT ( 'NONE',  ( 161.1235494854506953, 271.0628771894291731, 16.08318537909542556 ) ) ;
#64523=ORIENTED_EDGE ( 'NONE', *, *, #87504, .F. ) ;
#64524=CARTESIAN_POINT ( 'NONE',  ( 168.6046935506172417, 272.7627849129413562, 15.97842110015704264 ) ) ;
#64525=CARTESIAN_POINT ( 'NONE',  ( 193.7351983448268129, 295.0877885827630962, 13.32537352665005059 ) ) ;
#64526=CARTESIAN_POINT ( 'NONE',  ( 180.4994900830837992, 291.2687899966102236, -9.662810889139459292 ) ) ;
#64528=CARTESIAN_POINT ( 'NONE',  ( 193.7987916076703243, 294.5354169763049867, 13.61361374954321768 ) ) ;
#64529=CARTESIAN_POINT ( 'NONE',  ( 174.6180048270524594, 290.3475991095135100, 6.420941954033795973 ) ) ;
#64530=CARTESIAN_POINT ( 'NONE',  ( 197.6885739199660463, 288.2403412252199928, -17.06545875591766759 ) ) ;
#64532=CARTESIAN_POINT ( 'NONE',  ( 174.9358745049650565, 292.2217799751211942, 2.235529367806339263 ) ) ;
#64534=CARTESIAN_POINT ( 'NONE',  ( 206.1215120922853146, 273.6340638536760821, 10.12238414215620885 ) ) ;
#64535=CARTESIAN_POINT ( 'NONE',  ( 206.4943150373521803, 272.9883502116088039, 11.34100825923693101 ) ) ;
#64536=CARTESIAN_POINT ( 'NONE',  ( 198.2414483977475754, 287.2827345394944700, 16.94931984969033678 ) ) ;
#64539=CARTESIAN_POINT ( 'NONE',  ( 190.5800505906290141, 300.5526647984205511, 6.752949403983271814 ) ) ;
#64540=CARTESIAN_POINT ( 'NONE',  ( 171.5607332741838036, 259.4587583041368930, -13.88734664787412321 ) ) ;
#64543=CARTESIAN_POINT ( 'NONE',  ( 160.4869048512927918, 252.6755221785256822, -16.09843817406293809 ) ) ;
#64544=CARTESIAN_POINT ( 'NONE',  ( 190.8232856196690079, 262.0104826008901568, -0.7083013378410631944 ) ) ;
#64545=ORIENTED_EDGE ( 'NONE', *, *, #99485, .F. ) ;
#64546=B_SPLINE_CURVE_WITH_KNOTS ( 'NONE', 3,
 ( #24454, #47248, #63456, #31542 ),
 .UNSPECIFIED., .F., .F.,
 ( 4, 4 ),
 ( 0.01245835406871842466, 0.02099269020319429607 ),
 .UNSPECIFIED. ) ;
#64548=CARTESIAN_POINT ( 'NONE',  ( 60.28305926085685229, 195.6115022471902023, -5.000000000000041744 ) ) ;
#64551=CARTESIAN_POINT ( 'NONE',  ( 24.61363793893735874, 175.0177522451417929, 5.000000000000051514 ) ) ;
#64552=CARTESIAN_POINT ( 'NONE',  ( 106.6698052711106186, 223.2048013555410080, 4.594050593750051981 ) ) ;
#64556=CARTESIAN_POINT ( 'NONE',  ( 162.5082079047825800, 249.1745225923870919, 11.52567592363465465 ) ) ;
#64558=CARTESIAN_POINT ( 'NONE',  ( 11.67712314985746858, 186.7369531367911293, -4.594050593750048428 ) ) ;
#64560=CARTESIAN_POINT ( 'NONE',  ( 200.8551880497955437, 282.7556046643899776, 18.00894873733387058 ) ) ;
#64561=EDGE_LOOP ( 'NONE', ( #81725, #62138, #84223, #72812 ) ) ;
#64565=CARTESIAN_POINT ( 'NONE',  ( 147.6130911253305271, 276.0666186809932015, -0.7644645089462269727 ) ) ;
#64566=ADVANCED_FACE ( 'NONE', ( #76244 ), #75242, .T. ) ;
#64569=CARTESIAN_POINT ( 'NONE',  ( 192.9940517273955720, 263.8598628230966483, -4.307169378521571446 ) ) ;
#64573=CARTESIAN_POINT ( 'NONE',  ( 168.0837743945575369, 251.4641930119366293, 10.72931100272645644 ) ) ;
#64574=CARTESIAN_POINT ( 'NONE',  ( 47.67182463829572470, 189.1423013555410080, -4.594050593750043987 ) ) ;
#64575=CARTESIAN_POINT ( 'NONE',  ( 79.60625107924921906, 206.7677522451417929, -5.000000000000041744 ) ) ;
#64577=EDGE_CURVE ( 'NONE', #37080, #65018, #52539, .T. ) ;
#64579=B_SPLINE_CURVE_WITH_KNOTS ( 'NONE', 3,
 ( #214, #61986, #92939, #54382, #93451, #24005, #54903, #34125, #43185, #49319, #25517, #88885, #3242, #48829, #95963, #18430, #94953, #72131, #81255, #11343, #4202, #19925, #33623, #95477, #56900, #27022, #50303, #89370, #26526, #35099, #26030, #33113, #64520, #73619, #34607, #66010, #74126, #81747, #57905, #11830, #80772, #80258, #19446, #65019, #64013, #87884, #10824, #41703, #88380, #42199, #72646, #57400 ),
 .UNSPECIFIED., .F., .F.,
 ( 4, 2, 2, 2, 2, 2, 2, 2, 2, 2, 2, 2, 2, 2, 2, 2, 2, 2, 2, 2, 2, 2, 2, 2, 2, 4 ),
 ( 0.002899484069035259196, 0.003100245425264694290, 0.003301006781494129384, 0.003401387459608835873, 0.003501768137723542795, 0.003602148815838249283, 0.003702529493952955771, 0.003903290850182310201, 0.004104052206411664197, 0.004505574918870284586, 0.005308620343787543577, 0.006111665768704803436, 0.006914711193622062428, 0.007717756618539321420, 0.007818137296653968060, 0.007868327635711292248, 0.007918517974768614701, 0.007968708313825938888, 0.008018898652883261341, 0.008119279330997875022, 0.008320040687227098913, 0.008520802043456319336, 0.008721563399685543228, 0.008922324755914767119, 0.009123086112143989276, 0.009323847468373211433 ),
 .UNSPECIFIED. ) ;
#64580=CARTESIAN_POINT ( 'NONE',  ( -22.42236680055709641, 157.8615022471902591, 0.000000000000000000 ) ) ;
#64582=CARTESIAN_POINT ( 'NONE',  ( 4.126898030318161936, 167.0643266524160424, 9.188101187500095079 ) ) ;
#64584=CARTESIAN_POINT ( 'NONE',  ( 199.0363797504450929, 285.9058730480928716, -17.12190301149298222 ) ) ;
#64585=CARTESIAN_POINT ( 'NONE',  ( 186.5011568818524381, 282.7666149734188821, 16.16427038733343480 ) ) ;
#64586=CARTESIAN_POINT ( 'NONE',  ( 193.1444937042664094, 296.1109190324805240, -12.15243020627156767 ) ) ;
#64588=CARTESIAN_POINT ( 'NONE',  ( 163.9942050550062049, 246.6007000282974673, 5.791111691696777974 ) ) ;
#64589=CARTESIAN_POINT ( 'NONE',  ( 147.2229325088103735, 275.6493961858936927, -0.4918294119671829390 ) ) ;
#64590=CARTESIAN_POINT ( 'NONE',  ( 206.8968397926183229, 272.2911568841838061, 7.145103750817420440 ) ) ;
#64592=ORIENTED_EDGE ( 'NONE', *, *, #28146, .T. ) ;
#64593=CARTESIAN_POINT ( 'NONE',  ( -7.772103719870364635, 172.9865022471902876, 10.00000000000009237 ) ) ;
#64594=CARTESIAN_POINT ( 'NONE',  ( 181.2112225862389323, 268.1041159954503996, 15.22766750904507660 ) ) ;
#64595=CARTESIAN_POINT ( 'NONE',  ( 114.4365367415960293, 243.0024278399160949, -9.188101187500093303 ) ) ;
#64598=DIRECTION ( 'NONE',  ( 0.4999999999999998890, -0.8660254037844385966, 0.000000000000000000 ) ) ;
#64599=CARTESIAN_POINT ( 'NONE',  ( 196.1613785401733878, 290.8855212161054737, 15.98157687694135021 ) ) ;
#64600=CARTESIAN_POINT ( 'NONE',  ( 149.3118911495987788, 247.0312136851381126, 5.028230608967417581 ) ) ;
#64601=CARTESIAN_POINT ( 'NONE',  ( 150.4341052900205682, 270.0874817769553147, -15.18648472748443368 ) ) ;
#64602=ORIENTED_EDGE ( 'NONE', *, *, #49871, .F. ) ;
#64603=CARTESIAN_POINT ( 'NONE',  ( 189.7662698355838984, 261.5339742162131529, -4.454810789157368944 ) ) ;
#64604=CARTESIAN_POINT ( 'NONE',  ( 196.7823306783968746, 289.8100005636337073, -17.85370042640856170 ) ) ;
#64608=CARTESIAN_POINT ( 'NONE',  ( 189.1592966827000737, 265.6623959474144954, 10.76674785942434909 ) ) ;
#64609=CARTESIAN_POINT ( 'NONE',  ( 175.0739399029997116, 279.4198807484980307, 16.07690566252637510 ) ) ;
#64610=CARTESIAN_POINT ( 'NONE',  ( 168.0272649302995092, 271.2940026294745053, -16.46671956731438158 ) ) ;
#64613=CARTESIAN_POINT ( 'NONE',  ( 200.0499121993288441, 272.4670071845189909, 12.52220648084497512 ) ) ;
#64616=CARTESIAN_POINT ( 'NONE',  ( 148.1311260530199547, 274.4913500102855437, 6.529054274877645447 ) ) ;
#64618=EDGE_LOOP ( 'NONE', ( #32704, #95946, #40792, #42559 ) ) ;
#64619=CARTESIAN_POINT ( 'NONE',  ( 190.9966433480338139, 280.6469662536845817, 16.69273669211117550 ) ) ;
#64621=CARTESIAN_POINT ( 'NONE',  ( 194.5455058173357372, 289.6927750867642999, -16.22697001666201189 ) ) ;
#64622=ORIENTED_EDGE ( 'NONE', *, *, #232, .T. ) ;
#64623=CARTESIAN_POINT ( 'NONE',  ( 165.3079345244091769, 279.7873310763220047, 11.79426121657854765 ) ) ;
#64624=CARTESIAN_POINT ( 'NONE',  ( 194.8598199529639317, 293.1398868181796615, -15.91766051364927570 ) ) ;
#64631=CARTESIAN_POINT ( 'NONE',  ( -22.42236680055709641, 157.8615022471902591, 0.000000000000000000 ) ) ;
#64632=CARTESIAN_POINT ( 'NONE',  ( 190.8604783348975502, 300.0669496974951471, 7.597731640149610222 ) ) ;
#64636=CARTESIAN_POINT ( 'NONE',  ( 35.89232211637455094, 179.9824982072973683, 3.021315404115420679E-15 ) ) ;
#64637=EDGE_CURVE ( 'NONE', #94303, #73115, #64579, .T. ) ;
#64638=ORIENTED_EDGE ( 'NONE', *, *, #65791, .F. ) ;
#64641=CARTESIAN_POINT ( 'NONE',  ( 178.5336676047381843, 260.8667924985600166, 12.04724365429595068 ) ) ;
#64644=VERTEX_POINT ( 'NONE', #42688 ) ;
#64648=ORIENTED_EDGE ( 'NONE', *, *, #26842, .F. ) ;
#64650=CARTESIAN_POINT ( 'NONE',  ( 161.7900223312657033, 277.1148125758700189, -12.79293641940870785 ) ) ;
#64651=CARTESIAN_POINT ( 'NONE',  ( 192.4259603496955719, 297.3554553095298729, -12.40738485318142814 ) ) ;
#64652=CARTESIAN_POINT ( 'NONE',  ( 153.2583947049096764, 265.1956690150883560, -17.64103123457563882 ) ) ;
#64654=CARTESIAN_POINT ( 'NONE',  ( 157.8859435148417560, 280.9531261477192743, 2.096246200910757196 ) ) ;
#64655=CARTESIAN_POINT ( 'NONE',  ( 143.0428722300570143, 244.2048013555409511, 4.594050593750051981 ) ) ;
#64656=ORIENTED_EDGE ( 'NONE', *, *, #33240, .F. ) ;
#64663=CARTESIAN_POINT ( 'NONE',  ( 172.8210543149999978, 253.0650713199155177, -9.347212986753337560 ) ) ;
#64664=DIRECTION ( 'NONE',  ( 0.8660254037844395958, 0.4999999999999985567, 0.000000000000000000 ) ) ;
#64667=CARTESIAN_POINT ( 'NONE',  ( 154.0294858510416418, 277.2251019646651571, 7.160722724867846445 ) ) ;
#64668=CARTESIAN_POINT ( 'NONE',  ( 200.8147387322574957, 282.8256649374973790, -18.02438097732020239 ) ) ;
#64669=CARTESIAN_POINT ( 'NONE',  ( 177.1701925416140000, 289.0260261616784874, -9.098077640916422126 ) ) ;
#64670=CARTESIAN_POINT ( 'NONE',  ( 170.9473896922761185, 281.0006420345936817, 14.48361075345193605 ) ) ;
#64671=CARTESIAN_POINT ( 'NONE',  ( 153.4281311866982946, 266.9016768047333130, 16.59090889036721350 ) ) ;
#64672=CARTESIAN_POINT ( 'NONE',  ( 177.4410471705273835, 255.7678460362017177, -8.335468945180984690 ) ) ;
#64674=CARTESIAN_POINT ( 'NONE',  ( 147.8505793332463725, 274.5622799967613332, -9.317516487097901035 ) ) ;
#64678=CARTESIAN_POINT ( 'NONE',  ( 204.6061119446403040, 269.2277531849183561, -2.953647597350912424 ) ) ;
#64679=CARTESIAN_POINT ( 'NONE',  ( 191.8032754232698380, 298.4339772392067403, -9.388979487922194167 ) ) ;
#64681=CARTESIAN_POINT ( 'NONE',  ( 202.7041331321765938, 279.5531378413010657, 17.14708438049711248 ) ) ;
#64683=CARTESIAN_POINT ( 'NONE',  ( 151.4841312259729307, 274.9661650195698712, -8.701711564166631163 ) ) ;
#64684=CARTESIAN_POINT ( 'NONE',  ( 65.38900070045468738, 201.8927522451417929, -10.00000000000009237 ) ) ;
#64687=CARTESIAN_POINT ( 'NONE',  ( 193.3270472431910321, 276.0883453641457095, -16.25275238486911888 ) ) ;
#64689=CARTESIAN_POINT ( 'NONE',  ( 152.7314557461996571, 266.1083540640618708, 17.39314074348802208 ) ) ;
#64690=( BOUNDED_CURVE ( )  B_SPLINE_CURVE ( 2, ( #69942, #559, #1060, #78068, #39526, #31939, #95319, #40034, #25876 ),
 .UNSPECIFIED., .F., .T. ) 
 B_SPLINE_CURVE_WITH_KNOTS ( ( 3, 2, 2, 2, 3 ),
 ( 0.7298387096774193727, 0.7311827956989247479, 0.7338709677419354982, 0.7365591397849462485, 0.7379032258064516236 ),
 .UNSPECIFIED. ) 
 CURVE ( )  GEOMETRIC_REPRESENTATION_ITEM ( )  RATIONAL_B_SPLINE_CURVE ( ( 0.9330127018922194093, 0.9330127018922194093, 1.000000000000000000, 0.8660254037844387076, 1.000000000000000000, 0.8660254037844387076, 1.000000000000000000, 0.9330127018922194093, 0.9330127018922194093 ) ) 
 REPRESENTATION_ITEM ( '' )  );
#64693=CARTESIAN_POINT ( 'NONE',  ( 198.7045056313791633, 284.4806958840320021, 17.79791830837532274 ) ) ;
#64694=CARTESIAN_POINT ( 'NONE',  ( 87.80660267098954819, 215.3768266524160140, -9.188101187500091527 ) ) ;
#64697=ADVANCED_FACE ( 'NONE', ( #96960 ), #56407, .T. ) ;
#64699=CARTESIAN_POINT ( 'NONE',  ( -1.733428585275474942, 158.2592609112379876, 2.679491924311254714 ) ) ;
#64702=CARTESIAN_POINT ( 'NONE',  ( 160.8705110431349397, 281.6868185791299766, 5.475142679507278842 ) ) ;
#64704=CARTESIAN_POINT ( 'NONE',  ( 207.6163508138795635, 271.0449272387537576, -1.385071889578343152 ) ) ;
#64705=CARTESIAN_POINT ( 'NONE',  ( 207.7395400852921341, 270.8315571617199566, 6.369933974605918259 ) ) ;
#64706=EDGE_CURVE ( 'NONE', #19414, #91958, #74120, .T. ) ;
#64713=AXIS2_PLACEMENT_3D ( 'NONE', #42362, #50968, #90017 ) ;
#64714=CARTESIAN_POINT ( 'NONE',  ( 47.26526781268299260, 210.3464784336661637, 1.353441290958777327E-15 ) ) ;
#64716=CARTESIAN_POINT ( 'NONE',  ( 74.76226857436894591, 201.7202760586659167, -5.415160957724236172E-17 ) ) ;
#64717=CARTESIAN_POINT ( 'NONE',  ( 164.8489450237687493, 247.1202469751449939, -7.123750760659631531 ) ) ;
#64721=CARTESIAN_POINT ( 'NONE',  ( 14.20097916528452942, 190.5530062829863311, -4.648177544792955347E-16 ) ) ;
#64722=CARTESIAN_POINT ( 'NONE',  ( 176.3506576600417191, 270.0042805746620616, -16.66995943565067861 ) ) ;
#64726=CARTESIAN_POINT ( 'NONE',  ( -3.869528910404237632, 180.1199935810941781, 2.679491924311264039 ) ) ;
#64727=ORIENTED_EDGE ( 'NONE', *, *, #86807, .F. ) ;
#64729=CARTESIAN_POINT ( 'NONE',  ( 82.23173768200972233, 206.0327760586659451, 1.948934522072302763E-15 ) ) ;
#64736=CARTESIAN_POINT ( 'NONE',  ( 192.8985195491038098, 288.1185855829259594, 16.03958602435291780 ) ) ;
#64738=CARTESIAN_POINT ( 'NONE',  ( 120.4718248238752523, 250.3615022471903444, 5.000000000000046185 ) ) ;
#64743=CARTESIAN_POINT ( 'NONE',  ( 165.6937111782763452, 246.6359652278159160, -1.301814763765337224 ) ) ;
#64745=CARTESIAN_POINT ( 'NONE',  ( 202.3139361598622372, 280.2289788223093865, 15.93832709035092421 ) ) ;
#64746=CARTESIAN_POINT ( 'NONE',  ( 207.4413961551520913, 270.9595189787718255, -0.9988337982141689553 ) ) ;
#64750=EDGE_CURVE ( 'NONE', #83009, #46531, #26018, .T. ) ;
#64754=CARTESIAN_POINT ( 'NONE',  ( 170.5847424161334800, 250.4031697645958729, 3.399405397972957488 ) ) ;
#64755=CARTESIAN_POINT ( 'NONE',  ( 191.7451945007296956, 296.7399137238037952, -11.83242997637808713 ) ) ;
#64756=ORIENTED_EDGE ( 'NONE', *, *, #41666, .F. ) ;
#64757=EDGE_CURVE ( 'NONE', #50323, #34720, #59701, .T. ) ;
#64764=CARTESIAN_POINT ( 'NONE',  ( 183.4383719652804530, 295.9431572655629452, 1.012549917523295040 ) ) ;
#64766=CARTESIAN_POINT ( 'NONE',  ( 194.9455394410084921, 292.9914163096879065, -15.01116663483170655 ) ) ;
#64768=CARTESIAN_POINT ( 'NONE',  ( 193.8365934467825298, 294.9121671145370556, 14.14845633038902584 ) ) ;
#64769=CARTESIAN_POINT ( 'NONE',  ( 162.5148320529283126, 285.2034568178174254, 0.5437328601018158736 ) ) ;
#64770=CARTESIAN_POINT ( 'NONE',  ( 169.6258775464486632, 274.3344629316208056, -17.15914146219304115 ) ) ;
#64771=CARTESIAN_POINT ( 'NONE',  ( 164.3630144314164170, 245.9619034500468331, 5.823830253651713029 ) ) ;
#64773=CARTESIAN_POINT ( 'NONE',  ( 166.1457379652601105, 265.4834180535647761, 16.56432196572769300 ) ) ;
#64775=CARTESIAN_POINT ( 'NONE',  ( 88.99704050542813150, 228.3149278399160664, 9.188101187500093303 ) ) ;
#64779=CARTESIAN_POINT ( 'NONE',  ( 166.2783657372584116, 279.3061210340277398, -13.84400717950042470 ) ) ;
#64780=VERTEX_POINT ( 'NONE', #67492 ) ;
#64781=B_SPLINE_CURVE_WITH_KNOTS ( 'NONE', 3,
 ( #75291, #20588, #85277, #46209 ),
 .UNSPECIFIED., .F., .F.,
 ( 4, 4 ),
 ( 0.004610365127728928078, 0.009594302975941142869 ),
 .UNSPECIFIED. ) ;
#64782=ORIENTED_EDGE ( 'NONE', *, *, #39277, .F. ) ;
#64784=CARTESIAN_POINT ( 'NONE',  ( 146.8637854207107409, 276.2714571898724216, 0.7988785540157756770 ) ) ;
#64785=CARTESIAN_POINT ( 'NONE',  ( 155.8152618860606253, 260.7670451491295012, 0.000000000000000000 ) ) ;
#64786=CARTESIAN_POINT ( 'NONE',  ( 159.9770824720811220, 253.5585604421560788, -16.42166711341322483 ) ) ;
#64788=CARTESIAN_POINT ( 'NONE',  ( 90.37718171876834106, 232.1744531367911293, 4.594050593750047540 ) ) ;
#64789=VERTEX_POINT ( 'NONE', #97917 ) ;
#64792=CARTESIAN_POINT ( 'NONE',  ( 162.6396274730868186, 248.9468972229755082, -10.26162218571527518 ) ) ;
#64793=EDGE_LOOP ( 'NONE', ( #12832, #52288, #99751, #60874, #11058, #7822, #72126, #96066, #31819, #13543, #73034, #25278, #30620, #68213, #31591, #97550, #9281, #71627, #75883, #92918 ) ) ;
#64796=DIRECTION ( 'NONE',  ( -0.8660254037844387076, -0.4999999999999998890, -0.000000000000000000 ) ) ;
#64797=CARTESIAN_POINT ( 'NONE',  ( 134.2197177853555843, 257.4869531367911577, 4.594050593750046652 ) ) ;
#64799=CARTESIAN_POINT ( 'NONE',  ( -2.305318362028928370, 156.1427522451417644, 1.119607411625061291E-15 ) ) ;
#64801=VERTEX_POINT ( 'NONE', #83737 ) ;
#64802=CARTESIAN_POINT ( 'NONE',  ( 156.7423333928520890, 259.1613101971172455, 17.21575223094429319 ) ) ;
#64805=CARTESIAN_POINT ( 'NONE',  ( 149.7854447168632817, 277.1467554076948545, 4.663160563959508842 ) ) ;
#64806=DIRECTION ( 'NONE',  ( -0.8660254037844387076, -0.4999999999999998890, -0.000000000000000000 ) ) ;
#64809=CARTESIAN_POINT ( 'NONE',  ( 66.16250339235085676, 220.5530062829863027, -4.648177544792955347E-16 ) ) ;
#64810=CARTESIAN_POINT ( 'NONE',  ( 161.8289209813647176, 250.3510820566641257, 13.28523796267037937 ) ) ;
#64812=CARTESIAN_POINT ( 'NONE',  ( 195.2495212664957194, 275.1290853193528392, -16.26662379558266380 ) ) ;
#64815=CARTESIAN_POINT ( 'NONE',  ( 202.2123796483002138, 280.4048798601741623, -15.85247869902013740 ) ) ;
#64818=CARTESIAN_POINT ( 'NONE',  ( 180.4828997427432569, 266.7556949304461682, -14.76840115687851274 ) ) ;
#64819=CARTESIAN_POINT ( 'NONE',  ( 185.3509297750883889, 266.4368487342368326, 13.13595510978240277 ) ) ;
#64825=CARTESIAN_POINT ( 'NONE',  ( 181.5682298158554602, 273.5681932549885573, 17.67500197916986693 ) ) ;
#64826=CARTESIAN_POINT ( 'NONE',  ( 157.8797407370935559, 271.1684435876110228, -14.71067124673816018 ) ) ;
#64829=CARTESIAN_POINT ( 'NONE',  ( 13.11156449881669595, 184.5024278399160949, -9.188101187500093303 ) ) ;
#64832=B_SPLINE_CURVE_WITH_KNOTS ( 'NONE', 3,
 ( #86786, #95391, #40106, #31508, #47706, #24427, #70012, #78139, #85792, #628, #16819, #93359, #70518, #32010, #54815, #71545 ),
 .UNSPECIFIED., .F., .F.,
 ( 4, 2, 2, 2, 2, 2, 2, 4 ),
 ( 1.190910092370080074E-16, 0.0003787177898467455569, 0.0007574355796933719600, 0.001136153369539998634, 0.001514871159386624875, 0.001893588949233251332, 0.002272306739079878440, 0.003029742318773052424 ),
 .UNSPECIFIED. ) ;
#64834=CARTESIAN_POINT ( 'NONE',  ( 204.3165321041017251, 270.7059293579960126, 8.545054412317711012 ) ) ;
#64836=CARTESIAN_POINT ( 'NONE',  ( 27.26558041797736465, 195.7369531367911293, -4.594050593750048428 ) ) ;
#64837=CARTESIAN_POINT ( 'NONE',  ( 200.8769374536528858, 282.7179335918746688, 17.26928237494566787 ) ) ;
#64838=CARTESIAN_POINT ( 'NONE',  ( 190.1635032421960148, 301.2741459696644029, -5.047660290019184259 ) ) ;
#64840=CARTESIAN_POINT ( 'NONE',  ( 177.9038217119459091, 292.6972127826384735, 5.767030569036280419 ) ) ;
#64841=CARTESIAN_POINT ( 'NONE',  ( 178.6854534826287022, 293.3287072856790587, 2.638351066326640737 ) ) ;
#64842=CARTESIAN_POINT ( 'NONE',  ( 181.8955405286666860, 279.8176704957666630, -16.10530862137905928 ) ) ;
#64844=CARTESIAN_POINT ( 'NONE',  ( 166.7371348775683941, 257.8943008475421834, -15.20426139718983194 ) ) ;
#64845=LINE ( 'NONE', #32931, #85721 ) ;
#64848=CARTESIAN_POINT ( 'NONE',  ( 90.23310447506868570, 216.2365022471902023, -10.00000000000009059 ) ) ;
#64849=CARTESIAN_POINT ( 'NONE',  ( 18.28082717731156848, 171.3615022471901739, 5.000000000000051514 ) ) ;
#64850=EDGE_CURVE ( 'NONE', #47527, #48040, #33937, .T. ) ;
#64852=CARTESIAN_POINT ( 'NONE',  ( 46.56179571999062716, 203.8149278399160949, -9.188101187500095079 ) ) ;
#64853=CARTESIAN_POINT ( 'NONE',  ( 198.0858447170796524, 287.5522480202560018, 18.44384186289807559 ) ) ;
#64854=ORIENTED_EDGE ( 'NONE', *, *, #39768, .F. ) ;
#64859=CARTESIAN_POINT ( 'NONE',  ( 171.2389088083422166, 286.7460130492871713, 8.408771775780483182 ) ) ;
#64860=CARTESIAN_POINT ( 'NONE',  ( 164.2600772519394923, 246.1401958748887182, -2.110785484364219311 ) ) ;
#64861=LINE ( 'NONE', #3086, #68713 ) ;
#64864=CARTESIAN_POINT ( 'NONE',  ( 162.7561251957091031, 248.7451172484279027, 11.07313294959361194 ) ) ;
#64865=CARTESIAN_POINT ( 'NONE',  ( 148.9285945872975390, 272.6951028054104427, -12.01265727652413240 ) ) ;
#64866=CARTESIAN_POINT ( 'NONE',  ( 156.9652392049574132, 258.7752260052484985, 18.40175728539550448 ) ) ;
#64875=CARTESIAN_POINT ( 'NONE',  ( 190.9907605556751093, 299.8412942717858414, 8.799173206188184437 ) ) ;
#64877=FACE_OUTER_BOUND ( 'NONE', #28477, .T. ) ;
#64879=ORIENTED_EDGE ( 'NONE', *, *, #75707, .T. ) ;
#64880=CARTESIAN_POINT ( 'NONE',  ( 161.2488013048736377, 251.3558788108169040, -13.10044423494716170 ) ) ;
#64881=CARTESIAN_POINT ( 'NONE',  ( 150.9309360722972428, 269.7956109838555108, -13.68607459661258297 ) ) ;
#64882=CARTESIAN_POINT ( 'NONE',  ( 204.8523313866422484, 275.8323493198358847, 14.65426965484541100 ) ) ;
#64883=EDGE_LOOP ( 'NONE', ( #25787, #96049, #87373, #82352 ) ) ;
#64885=CARTESIAN_POINT ( 'NONE',  ( 159.7608930362198407, 253.9330115291272421, 15.38895778945778581 ) ) ;
#64888=CARTESIAN_POINT ( 'NONE',  ( 204.8878784573704195, 275.7707799872745795, -14.13380496213581594 ) ) ;
#64889=CARTESIAN_POINT ( 'NONE',  ( 120.4179585561885659, 231.1423013555409796, -4.594050593750043987 ) ) ;
#64891=CARTESIAN_POINT ( 'NONE',  ( 79.60625107924913380, 226.7677522451419350, -5.000000000000047962 ) ) ;
#64893=CARTESIAN_POINT ( 'NONE',  ( 207.8302079587528794, 270.6745157982714431, 3.572475529330238153 ) ) ;
#64894=VERTEX_POINT ( 'NONE', #39065 ) ;
#64896=CARTESIAN_POINT ( 'NONE',  ( 157.4627203480516755, 258.4629190429250798, 16.86169483958236626 ) ) ;
#64898=CARTESIAN_POINT ( 'NONE',  ( 61.77188751760235874, 194.2202760586659167, -5.415160957724236172E-17 ) ) ;
#64900=CARTESIAN_POINT ( 'NONE',  ( 151.2648146047323507, 268.6486510375538614, 15.71323890031163550 ) ) ;
#64901=CARTESIAN_POINT ( 'NONE',  ( 150.7471914551857708, 269.5452006317422047, 15.29409085476701691 ) ) ;
#64903=ORIENTED_EDGE ( 'NONE', *, *, #35547, .T. ) ;
#64906=CARTESIAN_POINT ( 'NONE',  ( 174.3506819931331506, 286.9267872025895940, 11.76311152586403885 ) ) ;
#64907=VERTEX_POINT ( 'NONE', #24394 ) ;
#64908=CARTESIAN_POINT ( 'NONE',  ( 174.0105655393888355, 260.7770664459772547, -13.96503775365264133 ) ) ;
#64911=CARTESIAN_POINT ( 'NONE',  ( 161.5757715694810770, 250.7895496999525449, -14.51803553215175135 ) ) ;
#64913=CARTESIAN_POINT ( 'NONE',  ( 190.6023073677431512, 300.5141149296460981, 3.174888932019753973 ) ) ;
#64915=CARTESIAN_POINT ( 'NONE',  ( 164.6869624841032191, 245.4008089637804346, 1.435659848726088317 ) ) ;
#64917=CARTESIAN_POINT ( 'NONE',  ( 153.8464967062441815, 264.7140010578719398, -16.51288510356084061 ) ) ;
#64918=CARTESIAN_POINT ( 'NONE',  ( 164.0854748117396582, 246.4426161724408928, -5.757837433625331514 ) ) ;
#64919=B_SPLINE_CURVE_WITH_KNOTS ( 'NONE', 3,
 ( #6129, #14236, #76059, #37513, #7621, #92277, #29926, #22824, #15207, #46102, #78542, #48638, #10131, #71940, #79063, #63322, #77544, #62302, #62815, #79572, #2544, #39496, #85166, #24329, #94263, #86682, #47615, #55693, #33427, #71442, #40999, #40000, #46612, #2030, #94757, #23814, #24818, #55205, #93259, #15711, #70422, #86186, #25320, #40508, #56207, #48120, #8134, #54706, #16723, #39007 ),
 .UNSPECIFIED., .F., .F.,
 ( 4, 2, 2, 2, 2, 2, 2, 2, 2, 2, 2, 2, 2, 2, 2, 2, 2, 2, 2, 2, 2, 2, 2, 2, 4 ),
 ( 0.001230839774562330572, 0.001705398597812425978, 0.002179957421062521383, 0.002417236832687631645, 0.002535876538500167043, 0.002654516244312702007, 0.002773155950125237405, 0.002891795655937772803, 0.003129075067562843600, 0.003603633890813042005, 0.004078192714063240409, 0.005027310360563775130, 0.005976428007064311584, 0.006450986830314656140, 0.006925545653565000695, 0.007044185359377666197, 0.007103505212284000683, 0.007162825065190333435, 0.007281464771003024958, 0.007400104476815714746, 0.007637383888441099528, 0.007874663300066486044, 0.008111942711691870825, 0.008349222123317257341, 0.008823780946568158742 ),
 .UNSPECIFIED. ) ;
#64920=CARTESIAN_POINT ( 'NONE',  ( 131.9199452241419124, 234.7202760586659736, -5.415160957724236172E-17 ) ) ;
#64921=EDGE_LOOP ( 'NONE', ( #81491, #25498, #6174, #58742 ) ) ;
#64924=CARTESIAN_POINT ( 'NONE',  ( 203.1044072055706806, 278.8598428092302584, -16.67109798570195878 ) ) ;
#64925=CARTESIAN_POINT ( 'NONE',  ( 204.9004517216375518, 275.7490024547470853, 14.55104398969427670 ) ) ;
#64926=CARTESIAN_POINT ( 'NONE',  ( -10.20233967203003544, 176.4637435831425023, 2.679491924311251605 ) ) ;
#64931=B_SPLINE_CURVE_WITH_KNOTS ( 'NONE', 3,
 ( #3244, #34127, #18432, #9319 ),
 .UNSPECIFIED., .F., .F.,
 ( 4, 4 ),
 ( 0.01260167760416553567, 0.01881583619385329004 ),
 .UNSPECIFIED. ) ;
#64932=CARTESIAN_POINT ( 'NONE',  ( 158.0556171945634674, 275.8819595179413682, -12.51247609328395782 ) ) ;
#64933=CARTESIAN_POINT ( 'NONE',  ( 147.7395812515338491, 275.4447818272566337, 3.760927250875937489 ) ) ;
#64934=CARTESIAN_POINT ( 'NONE',  ( 185.7731237309448034, 262.0522970092281980, 9.834746716364003660 ) ) ;
#64935=CARTESIAN_POINT ( 'NONE',  ( 157.8501323257721083, 280.8042112442767007, -7.123878780571343050 ) ) ;
#64936=CARTESIAN_POINT ( 'NONE',  ( 135.7624123097878623, 255.3149278399160949, 9.188101187500093303 ) ) ;
#64937=CARTESIAN_POINT ( 'NONE',  ( 23.90999230191038549, 184.6115022471902591, 10.00000000000009592 ) ) ;
#64939=CARTESIAN_POINT ( 'NONE',  ( 71.35211999908521818, 205.8768266524160140, 9.188101187500098632 ) ) ;
#64940=CARTESIAN_POINT ( 'NONE',  ( 174.5577213332984456, 251.6462513678240498, 3.602869039157936104 ) ) ;
#64943=CARTESIAN_POINT ( 'NONE',  ( 148.9694607950094394, 272.6243204573405592, 11.81236034532910573 ) ) ;
#64944=CARTESIAN_POINT ( 'NONE',  ( 155.4130510163440988, 279.6938839982619811, -1.521710589521471535 ) ) ;
#64945=CARTESIAN_POINT ( 'NONE',  ( 171.1527898587758045, 287.5703274966900835, -8.623511503197541117 ) ) ;
#64946=CARTESIAN_POINT ( 'NONE',  ( 155.2193237801463113, 261.7992402267395846, -18.58295809893692407 ) ) ;
#64947=EDGE_CURVE ( 'NONE', #30618, #76229, #13787, .T. ) ;
#64948=CARTESIAN_POINT ( 'NONE',  ( 194.6028008291465881, 289.1389010384484664, 16.14037336114297361 ) ) ;
#64949=CARTESIAN_POINT ( 'NONE',  ( 122.5466773502275544, 254.8927522451419634, 2.944929066748280225E-16 ) ) ;
#64952=ORIENTED_EDGE ( 'NONE', *, *, #87124, .T. ) ;
#64953=EDGE_CURVE ( 'NONE', #23257, #26637, #71513, .T. ) ;
#64955=CARTESIAN_POINT ( 'NONE',  ( 147.6220714307702622, 274.9580672937808572, 8.392894244419288441 ) ) ;
#64956=CARTESIAN_POINT ( 'NONE',  ( -4.614459115189767147, 158.9548013555409796, -4.594050593750042211 ) ) ;
#64957=CARTESIAN_POINT ( 'NONE',  ( 34.76219959342768107, 197.0024278399161233, 9.188101187500095079 ) ) ;
#64958=CARTESIAN_POINT ( 'NONE',  ( 175.6508819106952615, 256.4707162311754587, -10.98076396042754155 ) ) ;
#64961=CARTESIAN_POINT ( 'NONE',  ( 185.8492146212669240, 258.6745004276652935, -5.862532207920108540 ) ) ;
#64962=CARTESIAN_POINT ( 'NONE',  ( 192.4867222293441387, 292.6075778101206879, -14.23530027676960863 ) ) ;
#64963=CARTESIAN_POINT ( 'NONE',  ( 190.9441801652054096, 299.9219738747156043, -4.765040093794296716 ) ) ;
#64965=CARTESIAN_POINT ( 'NONE',  ( 167.5258143496386367, 256.6353381695413987, 13.78324095373011104 ) ) ;
#64966=CARTESIAN_POINT ( 'NONE',  ( 65.38900070045468738, 201.8927522451418213, -10.00000000000009059 ) ) ;
#64967=CARTESIAN_POINT ( 'NONE',  ( 163.0331642552320659, 256.4053458108576251, -15.77289028494504031 ) ) ;
#64968=CARTESIAN_POINT ( 'NONE',  ( 205.0716081116550527, 275.4525508911965517, -12.57761053684872188 ) ) ;
#64969=CARTESIAN_POINT ( 'NONE',  ( 162.1559275291031099, 252.0210818530713652, -13.25156758742917518 ) ) ;
#64970=( BOUNDED_CURVE ( )  B_SPLINE_CURVE ( 2, ( #83903, #52452, #68648, #36751, #23033, #29173, #14465, #30151, #38739 ),
 .UNSPECIFIED., .F., .T. ) 
 B_SPLINE_CURVE_WITH_KNOTS ( ( 3, 2, 2, 2, 3 ),
 ( 0.06854838709677418818, 0.06989247311827956333, 0.07258064516129032751, 0.07526881720430107781, 0.07661290322580645296 ),
 .UNSPECIFIED. ) 
 CURVE ( )  GEOMETRIC_REPRESENTATION_ITEM ( )  RATIONAL_B_SPLINE_CURVE ( ( 0.9330127018922194093, 0.9330127018922194093, 1.000000000000000000, 0.8660254037844387076, 1.000000000000000000, 0.8660254037844387076, 1.000000000000000000, 0.9330127018922194093, 0.9330127018922194093 ) ) 
 REPRESENTATION_ITEM ( '' )  );
#64971=CARTESIAN_POINT ( 'NONE',  ( 31.70422093597028734, 199.1115022471903160, -5.000000000000047962 ) ) ;
#64972=CARTESIAN_POINT ( 'NONE',  ( 169.9469112398214747, 250.9785751410766750, -8.718312767540300712 ) ) ;
#64974=CARTESIAN_POINT ( 'NONE',  ( 14.68175618682350780, 167.0327760586659451, 1.948934522072303157E-15 ) ) ;
#64976=CARTESIAN_POINT ( 'NONE',  ( 164.1042149987925427, 252.5458357570947783, 13.30367259394180479 ) ) ;
#64977=CARTESIAN_POINT ( 'NONE',  ( 192.1149248854976861, 297.8941845364767005, 12.26771790733441314 ) ) ;
#64979=CARTESIAN_POINT ( 'NONE',  ( 206.5280879940269756, 272.9298537347264642, 11.21709153681466731 ) ) ;
#64980=CARTESIAN_POINT ( 'NONE',  ( 164.9779129355220562, 244.8968679994381148, -1.771286574179712803 ) ) ;
#64981=FACE_OUTER_BOUND ( 'NONE', #57624, .T. ) ;
#64983=CARTESIAN_POINT ( 'NONE',  ( -17.42236680055705023, 149.2012482093457777, 0.000000000000000000 ) ) ;
#64985=CARTESIAN_POINT ( 'NONE',  ( 168.7862764537476608, 288.1668982680979525, 0.5246234862430114720 ) ) ;
#64987=CARTESIAN_POINT ( 'NONE',  ( 175.0387250457744983, 253.3993311541219953, -7.863511161993287146 ) ) ;
#64989=CARTESIAN_POINT ( 'NONE',  ( 112.2445834879231796, 225.6115022471901739, -5.000000000000041744 ) ) ;
#64990=CARTESIAN_POINT ( 'NONE',  ( 160.0081047537594543, 253.5048282741223602, -16.11956848123596941 ) ) ;
#64993=( BOUNDED_CURVE ( )  B_SPLINE_CURVE ( 2, ( #51784, #19893, #64989, #11312, #90322, #57872, #35575, #89341, #5179 ),
 .UNSPECIFIED., .F., .T. ) 
 B_SPLINE_CURVE_WITH_KNOTS ( ( 3, 2, 2, 2, 3 ),
 ( 0.7540322580645161255, 0.7553763440860215006, 0.7580645161290322509, 0.7607526881720430012, 0.7620967741935483764 ),
 .UNSPECIFIED. ) 
 CURVE ( )  GEOMETRIC_REPRESENTATION_ITEM ( )  RATIONAL_B_SPLINE_CURVE ( ( 0.9330127018922194093, 0.9330127018922194093, 1.000000000000000000, 0.8660254037844387076, 1.000000000000000000, 0.8660254037844387076, 1.000000000000000000, 0.9330127018922194093, 0.9330127018922194093 ) ) 
 REPRESENTATION_ITEM ( '' )  );
#64994=CYLINDRICAL_SURFACE ( 'NONE', #71636, 10.00000000000010658 ) ;
#64995=CARTESIAN_POINT ( 'NONE',  ( 165.0509870607838252, 244.7702999017660375, -2.356357909806504392 ) ) ;
#64999=ORIENTED_EDGE ( 'NONE', *, *, #38048, .T. ) ;
#65000=ORIENTED_EDGE ( 'NONE', *, *, #99831, .F. ) ;
#65003=VERTEX_POINT ( 'NONE', #99907 ) ;
#65005=CARTESIAN_POINT ( 'NONE',  ( 178.2293965766191661, 264.0593690949378356, 14.86337493992927605 ) ) ;
#65009=ADVANCED_FACE ( 'NONE', ( #69487 ), #46623, .F. ) ;
#65011=VERTEX_POINT ( 'NONE', #73501 ) ;
#65012=CARTESIAN_POINT ( 'NONE',  ( 200.6097954076514895, 283.1806371883870383, 16.82611162221071766 ) ) ;
#65013=CARTESIAN_POINT ( 'NONE',  ( 169.3073612053613317, 276.1872213954042081, -15.55595306670203293 ) ) ;
#65016=CARTESIAN_POINT ( 'NONE',  ( 170.6728735680048317, 255.5809563222128418, -11.58821030780939765 ) ) ;
#65017=CARTESIAN_POINT ( 'NONE',  ( 203.0337691736598629, 278.9821914694464340, 16.08167820133810011 ) ) ;
#65018=VERTEX_POINT ( 'NONE', #42568 ) ;
#65019=CARTESIAN_POINT ( 'NONE',  ( 156.9771955771814476, 266.1637941048814469, -16.64471738717700688 ) ) ;
#65023=CARTESIAN_POINT ( 'NONE',  ( 193.2916431108056088, 295.8560487840508699, 14.28858925737053909 ) ) ;
#65024=CARTESIAN_POINT ( 'NONE',  ( 177.8598173235638740, 289.1843520170486386, -9.332820079591703788 ) ) ;
#65027=CARTESIAN_POINT ( 'NONE',  ( 183.7975612849717777, 256.6346208101135176, -2.981236333899912161 ) ) ;
#65029=CARTESIAN_POINT ( 'NONE',  ( 191.2190380946134951, 260.9445496458436651, 3.106810577783889915 ) ) ;
#65031=CARTESIAN_POINT ( 'NONE',  ( 92.02724010209958294, 235.4860189848785410, -2.679491924311252493 ) ) ;
#65034=CARTESIAN_POINT ( 'NONE',  ( 159.7953104873542145, 253.8733987550956783, 15.41928249285404107 ) ) ;
#65037=CARTESIAN_POINT ( 'NONE',  ( 190.9260630086136530, 299.9533537104214247, 6.698530349890277513 ) ) ;
#65038=CARTESIAN_POINT ( 'NONE',  ( 171.5198295675851057, 259.4245737330473389, -13.88290939651866829 ) ) ;
#65039=CARTESIAN_POINT ( 'NONE',  ( 189.3423859142968695, 300.6963629005612120, 0.4146017780601669589 ) ) ;
#65041=CARTESIAN_POINT ( 'NONE',  ( 46.06580888206229929, 190.7365022471901739, -10.00000000000009237 ) ) ;
#65042=CARTESIAN_POINT ( 'NONE',  ( 148.6603736319484597, 273.1596751277295425, -9.224525803417190417 ) ) ;
#65044=CARTESIAN_POINT ( 'NONE',  ( 175.7882114856885210, 291.4026636951798537, -6.622811550496607857 ) ) ;
#65047=CARTESIAN_POINT ( 'NONE',  ( 164.9335952247126045, 244.9736285262353306, -1.661461410667423255 ) ) ;
#65048=CARTESIAN_POINT ( 'NONE',  ( 31.46967238556418422, 175.6427522451417644, 1.119607411625061291E-15 ) ) ;
#65049=CARTESIAN_POINT ( 'NONE',  ( 102.2582280487598609, 229.8458772461660544, 9.188101187500095079 ) ) ;
#65050=CARTESIAN_POINT ( 'NONE',  ( 166.8965953329662568, 259.4083194189263963, 16.50658842888446642 ) ) ;
#65051=CARTESIAN_POINT ( 'NONE',  ( 168.6156890688689884, 286.4116463664167895, -8.226575548882113509 ) ) ;
#65052=CARTESIAN_POINT ( 'NONE',  ( 162.6419541827858950, 248.9428672435623184, 10.30167521348375459 ) ) ;
#65053=CARTESIAN_POINT ( 'NONE',  ( 31.75860784375665702, 179.9548013555409796, -4.594050593750042211 ) ) ;
#65054=CARTESIAN_POINT ( 'NONE',  ( 172.0630936339023265, 254.4764114392720273, 11.54978638049990103 ) ) ;
#65055=ORIENTED_EDGE ( 'NONE', *, *, #3337, .T. ) ;
#65057=CARTESIAN_POINT ( 'NONE',  ( 185.1598287763772532, 259.9719152823935815, -5.764292841724723893 ) ) ;
#65060=CARTESIAN_POINT ( 'NONE',  ( 193.5605340833295998, 262.7645764782593005, -3.913255771308810971 ) ) ;
#65062=CARTESIAN_POINT ( 'NONE',  ( 182.7015270599942767, 284.3474866054488643, 14.96321108283051515 ) ) ;
#65064=CARTESIAN_POINT ( 'NONE',  ( 48.02338713675939630, 198.5333772461660828, 9.188101187500095079 ) ) ;
#65065=CARTESIAN_POINT ( 'NONE',  ( 91.22542524669046315, 210.1427522451417360, 1.119607411625061291E-15 ) ) ;
#65069=B_SPLINE_CURVE_WITH_KNOTS ( 'NONE', 3,
 ( #21542, #45320, #76255, #52425 ),
 .UNSPECIFIED., .F., .F.,
 ( 4, 4 ),
 ( 0.03623143502817663397, 0.04492301886968718544 ),
 .UNSPECIFIED. ) ;
#65070=CARTESIAN_POINT ( 'NONE',  ( 158.5653840560831043, 282.4927873443422754, -1.666044833076710585 ) ) ;
#65071=CARTESIAN_POINT ( 'NONE',  ( 5.155129649429669669, 173.7833772461660828, -9.188101187500095079 ) ) ;
#65073=CARTESIAN_POINT ( 'NONE',  ( 151.0426280674448378, 269.0334894088936153, -15.84467774422408581 ) ) ;
#65075=CARTESIAN_POINT ( 'NONE',  ( 147.1034852426517148, 275.8562849197056153, -3.648177088342072327 ) ) ;
#65077=CARTESIAN_POINT ( 'NONE',  ( 164.3853877993040840, 245.9231516401292197, 5.995325337583643943 ) ) ;
#65078=CARTESIAN_POINT ( 'NONE',  ( 67.62392126478502519, 221.3967562850346837, -4.648177544792955347E-16 ) ) ;
#65079=FACE_OUTER_BOUND ( 'NONE', #18776, .T. ) ;
#65081=CARTESIAN_POINT ( 'NONE',  ( -8.493791556357424000, 179.2365022471903160, 2.944929066748280225E-16 ) ) ;
#65083=CARTESIAN_POINT ( 'NONE',  ( 128.5637496887121927, 245.0333772461660544, 9.188101187500095079 ) ) ;
#65087=CARTESIAN_POINT ( 'NONE',  ( 157.8092552871339365, 257.3133472685137235, 17.04082256169242626 ) ) ;
#65088=CARTESIAN_POINT ( 'NONE',  ( 185.5460614991013983, 288.0617137868250666, 14.93142655311823397 ) ) ;
#65090=VERTEX_POINT ( 'NONE', #12708 ) ;
#65091=CARTESIAN_POINT ( 'NONE',  ( 191.5694459269389824, 298.8389818071599962, 7.944420692511652504 ) ) ;
#65092=CARTESIAN_POINT ( 'NONE',  ( 196.3507576896697344, 290.5575069072837664, -17.68249398312240928 ) ) ;
#65094=CARTESIAN_POINT ( 'NONE',  ( 174.5937358169846902, 290.6289298292567764, -1.069262448657138043 ) ) ;
#65098=VECTOR ( 'NONE', #72988, 1000.000000000000000 ) ;
#65100=CARTESIAN_POINT ( 'NONE',  ( 175.8408436088426186, 278.6720592842420956, 15.46214555605372531 ) ) ;
#65101=CARTESIAN_POINT ( 'NONE',  ( 166.8389619083949924, 270.5748136803991883, -16.31214114901503720 ) ) ;
#65103=B_SPLINE_SURFACE_WITH_KNOTS ( 'NONE', 3, 1, ( 
 ( #5323, #28604 ),
 ( #21038, #52899 ),
 ( #13912, #90961 ),
 ( #36199, #83851 ),
 ( #52402, #74743 ),
 ( #67104, #67605 ),
 ( #30106, #44299 ),
 ( #68599, #29612 ),
 ( #51920, #6311 ),
 ( #22504, #75727 ),
 ( #44791, #90468 ),
 ( #59487, #82860 ),
 ( #98534, #99522 ),
 ( #12942, #91442 ),
 ( #5810, #36696 ),
 ( #13432, #60988 ),
 ( #98029, #75228 ),
 ( #4833, #37202 ),
 ( #29125, #60484 ),
 ( #20529, #97542 ),
 ( #14416, #83346 ),
 ( #51409, #45299 ),
 ( #76232, #82371 ),
 ( #12431, #68104 ),
 ( #59991, #6807 ),
 ( #21518, #74247 ),
 ( #37689, #66613 ),
 ( #99025, #91955 ),
 ( #81855, #43300 ),
 ( #35714, #58983 ),
 ( #28109, #89952 ),
 ( #32087, #85872 ),
 ( #54372, #100022 ),
 ( #64882, #203 ) ),
 .UNSPECIFIED., .T., .F., .F.,
 ( 4, 2, 2, 2, 2, 2, 2, 2, 2, 2, 2, 2, 2, 2, 2, 2, 4 ),
 ( 2, 2 ),
 ( 0.000000000000000000, 0.06250000000000000000, 0.1250000000000000000, 0.1875000000000000000, 0.2500000000000000000, 0.3125000000000000000, 0.3750000000000000000, 0.4375000000000000000, 0.5000000000000000000, 0.5625000000000000000, 0.6250000000000000000, 0.6875000000000000000, 0.7500000000000000000, 0.8125000000000000000, 0.8750000000000000000, 0.9375000000000000000, 1.000000000000000000 ),
 ( 0.000000000000000000, 1.000000000000000000 ),
 .UNSPECIFIED. ) ;
#65106=CARTESIAN_POINT ( 'NONE',  ( 155.6661834545002989, 261.4322516281303592, 17.01228065901951325 ) ) ;
#65108=CARTESIAN_POINT ( 'NONE',  ( 153.4389798490260262, 264.8828863703868137, 16.68923469758090761 ) ) ;
#65110=DIRECTION ( 'NONE',  ( 0.5000000000000048850, -0.8660254037844358210, 0.000000000000000000 ) ) ;
#65112=CARTESIAN_POINT ( 'NONE',  ( 191.8248132796572918, 287.9113088684474064, -15.87179701694280176 ) ) ;
#65115=CARTESIAN_POINT ( 'NONE',  ( 148.0826818691893152, 274.1602666119424043, -9.371267383421741926 ) ) ;
#65116=CARTESIAN_POINT ( 'NONE',  ( 156.0874977470830345, 262.0026131717037856, -16.96117934707180552 ) ) ;
#65120=AXIS2_PLACEMENT_3D ( 'NONE', #56430, #71157, #64036 ) ;
#65121=EDGE_CURVE ( 'NONE', #734, #43672, #66890, .T. ) ;
#65122=ORIENTED_EDGE ( 'NONE', *, *, #28684, .F. ) ;
#65125=ORIENTED_EDGE ( 'NONE', *, *, #69452, .F. ) ;
#65126=ORIENTED_EDGE ( 'NONE', *, *, #34437, .T. ) ;
#65128=ORIENTED_EDGE ( 'NONE', *, *, #84190, .T. ) ;
#65129=CARTESIAN_POINT ( 'NONE',  ( 171.7383634674231416, 249.5738785302591509, -2.481706805167441576 ) ) ;
#65133=CARTESIAN_POINT ( 'NONE',  ( 155.3513572141771704, 261.5705516107003064, -17.00592413546589299 ) ) ;
#65135=CARTESIAN_POINT ( 'NONE',  ( 183.0440910913980872, 280.4743473074019562, -16.11601913062221669 ) ) ;
#65137=CARTESIAN_POINT ( 'NONE',  ( 151.3884156280674063, 268.8244654414531283, 14.32026866203507076 ) ) ;
#65138=CARTESIAN_POINT ( 'NONE',  ( 161.8067806907298518, 277.5376414676186982, -13.20325758529581961 ) ) ;
#65139=CARTESIAN_POINT ( 'NONE',  ( 147.2089949622447875, 275.6735367246781720, -3.633014386235353221 ) ) ;
#65140=CARTESIAN_POINT ( 'NONE',  ( 200.7134601498536028, 283.0010845879393742, -16.98649239173277792 ) ) ;
#65141=EDGE_CURVE ( 'NONE', #88888, #87622, #61710, .T. ) ;
#65143=CARTESIAN_POINT ( 'NONE',  ( 10.48659854325162222, 166.8615022471902023, 5.000000000000051514 ) ) ;
#65144=CARTESIAN_POINT ( 'NONE',  ( 138.2797325092426490, 241.4548013555409796, -4.594050593750042211 ) ) ;
#65145=CARTESIAN_POINT ( 'NONE',  ( 196.2953682204578456, 263.5854184417236752, 0.8810977108677261471 ) ) ;
#65148=CARTESIAN_POINT ( 'NONE',  ( 204.0395441575055031, 271.6647427339178762, 9.749783370949133499 ) ) ;
#65150=B_SPLINE_CURVE_WITH_KNOTS ( 'NONE', 3,
 ( #18845, #88793, #57814, #96368 ),
 .UNSPECIFIED., .F., .F.,
 ( 4, 4 ),
 ( 0.003259762943304704563, 0.01121638692189557036 ),
 .UNSPECIFIED. ) ;
#65153=CARTESIAN_POINT ( 'NONE',  ( 157.6339405821837829, 280.6012083038259561, -7.094479895829409521 ) ) ;
#65159=CARTESIAN_POINT ( 'NONE',  ( 194.2389208611690492, 294.2153155915419802, -15.75132567904764791 ) ) ;
#65161=ORIENTED_EDGE ( 'NONE', *, *, #82176, .F. ) ;
#65162=CARTESIAN_POINT ( 'NONE',  ( 163.2575071667584723, 277.3374444033298118, 12.94744084712231569 ) ) ;
#65163=CARTESIAN_POINT ( 'NONE',  ( 201.1240395725599228, 267.4342541147308339, -2.284400240072811172 ) ) ;
#65165=CARTESIAN_POINT ( 'NONE',  ( 149.0359194785865498, 272.5092106407810206, 12.76357969772040590 ) ) ;
#65166=CARTESIAN_POINT ( 'NONE',  ( 162.6220573360242270, 248.9773295930640131, 10.49878733418918486 ) ) ;
#65169=CARTESIAN_POINT ( 'NONE',  ( 151.3150518705357683, 275.2366200239924297, -9.722076783269896438 ) ) ;
#65171=CARTESIAN_POINT ( 'NONE',  ( 203.4543820542745891, 269.9310094597221337, 5.750300676160139624 ) ) ;
#65177=VECTOR ( 'NONE', #70458, 1000.000000000000000 ) ;
#65179=CARTESIAN_POINT ( 'NONE',  ( 192.8323852661406761, 296.6515067047851062, 11.86505947732313615 ) ) ;
#65181=CARTESIAN_POINT ( 'NONE',  ( -17.42236680055705023, 149.2012482093457777, 0.000000000000000000 ) ) ;
#65182=CARTESIAN_POINT ( 'NONE',  ( 202.6070187115982719, 279.7213449518906145, 15.56322169823762280 ) ) ;
#65183=CARTESIAN_POINT ( 'NONE',  ( 13.46382118881039602, 169.3923013555410080, 4.594050593750050204 ) ) ;
#65184=CARTESIAN_POINT ( 'NONE',  ( 106.6698052711106186, 223.2048013555410080, 4.594050593750051981 ) ) ;
#65185=CARTESIAN_POINT ( 'NONE',  ( 154.9528145190857344, 262.2608478075840708, -17.26679351315302213 ) ) ;
#65187=CARTESIAN_POINT ( 'NONE',  ( 183.9260584196478874, 294.3655144402644055, -7.753805750097078509 ) ) ;
#65192=CARTESIAN_POINT ( 'NONE',  ( 161.6289632141471486, 282.0538248220675541, 5.604263265739757749 ) ) ;
#65193=CARTESIAN_POINT ( 'NONE',  ( 194.2223991963907963, 294.2439319543634610, -14.97294938100067441 ) ) ;
#65195=CARTESIAN_POINT ( 'NONE',  ( 181.7974296340893261, 291.5457255195387916, 9.383524427102701182 ) ) ;
#65198=FACE_OUTER_BOUND ( 'NONE', #89743, .T. ) ;
#65199=CARTESIAN_POINT ( 'NONE',  ( 6.860117161356369841, 164.7677522451418213, -5.000000000000041744 ) ) ;
#65202=CARTESIAN_POINT ( 'NONE',  ( 81.63493525668631889, 229.4860189848785410, -2.679491924311252493 ) ) ;
#65204=CARTESIAN_POINT ( 'NONE',  ( 90.35072584248885619, 210.7202760586659736, -5.415160957724236172E-17 ) ) ;
#65205=CARTESIAN_POINT ( 'NONE',  ( 161.7412967960748915, 250.5028515975580774, -14.36228887024421041 ) ) ;
#65208=CARTESIAN_POINT ( 'NONE',  ( 197.5862184977020490, 286.6310308989096711, -17.64960021936426671 ) ) ;
#65209=CARTESIAN_POINT ( 'NONE',  ( 151.7785311547446270, 267.7588678722433428, 16.64796787849914850 ) ) ;
#65210=CARTESIAN_POINT ( 'NONE',  ( 173.2447795235415811, 268.2516447256268179, -16.29229155239807980 ) ) ;
#65216=CARTESIAN_POINT ( 'NONE',  ( 74.97842782955004282, 214.0958772461660544, -9.188101187500095079 ) ) ;
#65217=CARTESIAN_POINT ( 'NONE',  ( 169.3398175065472344, 288.7630245530638717, -1.132601341623118874 ) ) ;
#65219=CARTESIAN_POINT ( 'NONE',  ( 191.7460210811677541, 287.9459192371517133, -15.84374680109877609 ) ) ;
#65220=EDGE_LOOP ( 'NONE', ( #55342, #80363, #64264 ) ) ;
#65222=CARTESIAN_POINT ( 'NONE',  ( 190.3592232750935409, 286.7364522702076215, 16.27178271100322249 ) ) ;
#65224=CARTESIAN_POINT ( 'NONE',  ( 125.6679772465819127, 253.3615022471903444, 5.000000000000046185 ) ) ;
#65225=CARTESIAN_POINT ( 'NONE',  ( 157.1458804504438831, 258.4623461901232417, -17.08829597948888335 ) ) ;
#65227=ORIENTED_EDGE ( 'NONE', *, *, #28717, .T. ) ;
#65228=CARTESIAN_POINT ( 'NONE',  ( 165.5469766331900985, 246.9197538857407608, -1.831016119632084438 ) ) ;
#65229=ORIENTED_EDGE ( 'NONE', *, *, #28974, .F. ) ;
#65230=CARTESIAN_POINT ( 'NONE',  ( 163.2437751800324293, 247.9004826992694461, 9.806027032984305336 ) ) ;
#65231=CARTESIAN_POINT ( 'NONE',  ( 207.2447263765708954, 270.1464842563735829, -0.1082122603863571730 ) ) ;
#65234=ORIENTED_EDGE ( 'NONE', *, *, #12227, .F. ) ;
#65236=CARTESIAN_POINT ( 'NONE',  ( 167.4483379500863407, 247.4779818019835034, 3.613496412595774920 ) ) ;
#65237=CARTESIAN_POINT ( 'NONE',  ( 194.0917849768643748, 280.7715605316444680, -17.25264104449663449 ) ) ;
#65238=CARTESIAN_POINT ( 'NONE',  ( 201.3053657339852691, 274.7141922394133076, -14.27644254562359372 ) ) ;
#65242=LINE ( 'NONE', #71363, #57567 ) ;
#65243=AXIS2_PLACEMENT_3D ( 'NONE', #40373, #56066, #86552 ) ;
#65245=CARTESIAN_POINT ( 'NONE',  ( 162.8751945631634612, 272.8900720096677333, -16.40198242748087054 ) ) ;
#65247=ORIENTED_EDGE ( 'NONE', *, *, #95333, .T. ) ;
#65248=CARTESIAN_POINT ( 'NONE',  ( 186.1378587046176847, 298.7759093635723389, 1.082710523946170733 ) ) ;
#65249=CARTESIAN_POINT ( 'NONE',  ( 163.9704062730716032, 246.6419207277664327, 7.317582738093436845 ) ) ;
#65250=CARTESIAN_POINT ( 'NONE',  ( 148.2352135776142177, 273.8960739431854563, -9.245976304249309052 ) ) ;
#65256=CARTESIAN_POINT ( 'NONE',  ( 164.7586010964001844, 245.2767272474987408, 5.149004892315893755 ) ) ;
#65260=CARTESIAN_POINT ( 'NONE',  ( 103.7194723697636221, 236.8149278399160949, -9.188101187500095079 ) ) ;
#65264=CARTESIAN_POINT ( 'NONE',  ( 166.3892922564430705, 279.1128815750697640, -13.41989996223110282 ) ) ;
#65265=ORIENTED_EDGE ( 'NONE', *, *, #59265, .T. ) ;
#65268=ADVANCED_FACE ( 'NONE', ( #23261 ), #47566, .T. ) ;
#65269=CARTESIAN_POINT ( 'NONE',  ( 180.0871239489544848, 293.6764218470086689, -2.637204768131844013 ) ) ;
#65274=CARTESIAN_POINT ( 'NONE',  ( 98.68587325814904432, 227.7833772461660544, -9.188101187500095079 ) ) ;
#65276=( BOUNDED_CURVE ( )  B_SPLINE_CURVE ( 2, ( #550, #31431, #55713, #59, #48143, #9670, #62324, #79087, #92778 ),
 .UNSPECIFIED., .F., .T. ) 
 B_SPLINE_CURVE_WITH_KNOTS ( ( 3, 2, 2, 2, 3 ),
 ( 0.5120967741935483764, 0.5134408602150537515, 0.5161290322580645018, 0.5188172043010752521, 0.5201612903225806273 ),
 .UNSPECIFIED. ) 
 CURVE ( )  GEOMETRIC_REPRESENTATION_ITEM ( )  RATIONAL_B_SPLINE_CURVE ( ( 0.9330127018922194093, 0.9330127018922194093, 1.000000000000000000, 0.8660254037844387076, 1.000000000000000000, 0.8660254037844387076, 1.000000000000000000, 0.9330127018922194093, 0.9330127018922194093 ) ) 
 REPRESENTATION_ITEM ( '' )  );
#65278=CARTESIAN_POINT ( 'NONE',  ( 169.7005567072155259, 288.7155782076579271, 4.430715832634252394 ) ) ;
#65279=CARTESIAN_POINT ( 'NONE',  ( 207.6523394534040392, 270.9825930866021508, -2.115019688068903392 ) ) ;
#65280=VERTEX_POINT ( 'NONE', #979 ) ;
#65284=CARTESIAN_POINT ( 'NONE',  ( 139.9303331133829715, 251.5958772461660544, -9.188101187500095079 ) ) ;
#65286=CARTESIAN_POINT ( 'NONE',  ( -9.233521592304517966, 172.1427522451419065, 10.00000000000009237 ) ) ;
#65290=CARTESIAN_POINT ( 'NONE',  ( 157.1184542243154567, 258.5098498072379698, 16.84490127433854667 ) ) ;
#65291=CARTESIAN_POINT ( 'NONE',  ( 160.3188448450098065, 275.5225805274294544, 12.83265129500923685 ) ) ;
#65294=CARTESIAN_POINT ( 'NONE',  ( 188.9450937826650545, 269.5268139213692962, 14.88809917091533741 ) ) ;
#65295=CARTESIAN_POINT ( 'NONE',  ( 45.03194321908421927, 185.2592609112380160, 2.679491924311254714 ) ) ;
#65302=CARTESIAN_POINT ( 'NONE',  ( 160.0061168334508750, 253.5082714530983026, -16.02306982074888708 ) ) ;
#65304=CARTESIAN_POINT ( 'NONE',  ( 163.1096928939807924, 248.1327200311062882, -9.690381021358412283 ) ) ;
#65305=DIRECTION ( 'NONE',  ( -0.8660254037844387076, -0.4999999999999998890, -0.000000000000000000 ) ) ;
#65308=CARTESIAN_POINT ( 'NONE',  ( 177.7502759686835816, 264.9915612121205299, -15.08494360417384961 ) ) ;
#65309=CARTESIAN_POINT ( 'NONE',  ( 190.9474291326297930, 266.7645650087163745, -12.82661358031884546 ) ) ;
#65311=CARTESIAN_POINT ( 'NONE',  ( 182.4009855739953991, 264.2690820246323256, -14.57423425229302438 ) ) ;
#65313=B_SPLINE_CURVE_WITH_KNOTS ( 'NONE', 3,
 ( #5535, #91165, #22735, #36419 ),
 .UNSPECIFIED., .F., .F.,
 ( 4, 4 ),
 ( 0.007625806130884848696, 0.01343629536117592511 ),
 .UNSPECIFIED. ) ;
#65314=CARTESIAN_POINT ( 'NONE',  ( 99.70756906128829655, 216.8262482093457493, 3.021315404115420679E-15 ) ) ;
#65316=CARTESIAN_POINT ( 'NONE',  ( 160.7004439013812487, 272.9463992000354438, -14.94530573250521144 ) ) ;
#65318=CARTESIAN_POINT ( 'NONE',  ( 14.24839638916628459, 179.0333772461660544, 9.188101187500095079 ) ) ;
#65321=ORIENTED_EDGE ( 'NONE', *, *, #87184, .F. ) ;
#65324=CARTESIAN_POINT ( 'NONE',  ( 186.0400780920065529, 271.7087950812899066, 16.90619359840448510 ) ) ;
#65326=CARTESIAN_POINT ( 'NONE',  ( 39.55283647781661216, 184.4548013555409796, -4.594050593750042211 ) ) ;
#65328=CARTESIAN_POINT ( 'NONE',  ( 147.5634954182374372, 275.0595239235922236, 4.682022975662822439 ) ) ;
#65330=CARTESIAN_POINT ( 'NONE',  ( 180.5087874685112581, 292.9443678237462336, 6.144088910392417446 ) ) ;
#65331=CARTESIAN_POINT ( 'NONE',  ( 146.6138605399200117, 276.7043397814778132, -0.5394499176159462950 ) ) ;
#65338=CARTESIAN_POINT ( 'NONE',  ( 74.50030963965132003, 220.4865022471902876, -10.00000000000009415 ) ) ;
#65340=CARTESIAN_POINT ( 'NONE',  ( 162.2378898886269951, 268.0060074806465309, -16.71809273753259717 ) ) ;
#65341=CARTESIAN_POINT ( 'NONE',  ( 51.59574192737019160, 200.5958772461660544, -9.188101187500095079 ) ) ;
#65343=CARTESIAN_POINT ( 'NONE',  ( 179.0484917649878298, 259.9789987921100192, 12.89662402083353854 ) ) ;
#65344=CARTESIAN_POINT ( 'NONE',  ( 147.0670278774466908, 275.9194309285509235, 3.666898409139099257 ) ) ;
#65347=CARTESIAN_POINT ( 'NONE',  ( 170.8335652545856362, 286.3135742921572273, 7.469445898408281437 ) ) ;
#65348=CARTESIAN_POINT ( 'NONE',  ( 207.5338226493333025, 271.1878702128032614, 6.432541580693135863 ) ) ;
#65351=CARTESIAN_POINT ( 'NONE',  ( 186.8024928136323695, 263.1790814610873213, 11.56963523927125337 ) ) ;
#65359=ORIENTED_EDGE ( 'NONE', *, *, #82586, .T. ) ;
#65360=DIRECTION ( 'NONE',  ( 0.4999999999999998890, -0.8660254037844385966, 0.000000000000000000 ) ) ;
#65361=CARTESIAN_POINT ( 'NONE',  ( 151.2648146047323507, 268.6486510375538614, 15.71323890031163550 ) ) ;
#65362=CARTESIAN_POINT ( 'NONE',  ( 177.3160476213384982, 256.0269507273385443, -7.165014414593925629 ) ) ;
#65364=ORIENTED_EDGE ( 'NONE', *, *, #79642, .F. ) ;
#65366=CARTESIAN_POINT ( 'NONE',  ( 207.8575108622103755, 270.6272257822888037, -6.381720258959569847 ) ) ;
#65367=CARTESIAN_POINT ( 'NONE',  ( 151.3023505463322067, 269.2715888188440090, -14.21498388727478535 ) ) ;
#65368=CARTESIAN_POINT ( 'NONE',  ( 184.3388797322841981, 264.0495600577374375, -13.68812008961389282 ) ) ;
#65371=CARTESIAN_POINT ( 'NONE',  ( 159.4230536986738400, 254.5181664265525683, 16.83068086755798376 ) ) ;
#65372=CARTESIAN_POINT ( 'NONE',  ( 156.6812872898450735, 261.2670451491295012, 0.000000000000000000 ) ) ;
#65374=CARTESIAN_POINT ( 'NONE',  ( 204.6075833744878878, 276.2562653119390461, -13.34672481898815910 ) ) ;
#65375=CARTESIAN_POINT ( 'NONE',  ( 115.2218061334819623, 228.1423013555409796, -4.594050593750043987 ) ) ;
#65379=CARTESIAN_POINT ( 'NONE',  ( 163.8455942243524248, 246.8581015375447691, -7.178103170949780676 ) ) ;
#65380=ORIENTED_EDGE ( 'NONE', *, *, #28700, .F. ) ;
#65382=CARTESIAN_POINT ( 'NONE',  ( 159.4889735931715222, 254.4039898200529706, 16.88104032092801887 ) ) ;
#65384=CARTESIAN_POINT ( 'NONE',  ( 70.26924114858965709, 217.5024278399160664, -9.188101187500093303 ) ) ;
#65385=ADVANCED_FACE ( 'NONE', ( #95228 ), #85500, .T. ) ;
#65387=CARTESIAN_POINT ( 'NONE',  ( 151.0036289208911171, 269.1010379121764799, 14.24595189915657478 ) ) ;
#65388=CARTESIAN_POINT ( 'NONE',  ( 201.7511365947159163, 271.6656860447648114, 11.60973541740156101 ) ) ;
#65389=CARTESIAN_POINT ( 'NONE',  ( 175.6541281476291090, 278.4009151887023563, 16.88439838973073037 ) ) ;
#65390=EDGE_CURVE ( 'NONE', #19593, #78035, #69245, .T. ) ;
#65395=CARTESIAN_POINT ( 'NONE',  ( 155.5587153255869453, 261.2113968263770971, -18.30500480654006878 ) ) ;
#65397=CARTESIAN_POINT ( 'NONE',  ( 194.9643996604583833, 292.9587494513586989, 15.17976699960614440 ) ) ;
#65400=CARTESIAN_POINT ( 'NONE',  ( 70.10597207235390727, 222.8297689869269220, -2.679491924311252493 ) ) ;
#65402=CARTESIAN_POINT ( 'NONE',  ( 190.1519139143167081, 301.2942192743771557, 4.481136594690903863 ) ) ;
#65403=CARTESIAN_POINT ( 'NONE',  ( 177.1262862392189845, 269.6057104283654553, 17.56656865388298172 ) ) ;
#65404=CARTESIAN_POINT ( 'NONE',  ( 164.7462163020046262, 245.2981783406326599, 1.451255823150352064 ) ) ;
#65406=CARTESIAN_POINT ( 'NONE',  ( 167.3995633324949210, 256.4415895850399352, 13.70966202949693091 ) ) ;
#65407=CARTESIAN_POINT ( 'NONE',  ( 1.210598108517954463, 183.0530062829863596, 2.649461200531984646E-14 ) ) ;
#65408=CARTESIAN_POINT ( 'NONE',  ( 129.3218690127885964, 233.2202760586659736, -5.415160957724236172E-17 ) ) ;
#65414=CARTESIAN_POINT ( 'NONE',  ( 164.3853877993040840, 245.9231516401292197, 5.995325337583643943 ) ) ;
#65419=EDGE_CURVE ( 'NONE', #18680, #21764, #2874, .T. ) ;
#65420=CARTESIAN_POINT ( 'NONE',  ( 183.8037341582430884, 275.4624792557407318, 17.77592483611231700 ) ) ;
#65422=CARTESIAN_POINT ( 'NONE',  ( 164.2960764465929060, 246.0778434407177713, -1.520364048796653877 ) ) ;
#65423=CARTESIAN_POINT ( 'NONE',  ( 148.6720373546558847, 247.4548013555409796, -4.594050593750042211 ) ) ;
#65424=CARTESIAN_POINT ( 'NONE',  ( 20.80673460501611771, 189.4865022471903160, 10.00000000000009415 ) ) ;
#65425=ADVANCED_FACE ( 'NONE', ( #27774 ), #24000, .F. ) ;
#65427=CARTESIAN_POINT ( 'NONE',  ( 174.6584545799940145, 251.8359307791901927, 3.578998500653847614 ) ) ;
#65428=EDGE_CURVE ( 'NONE', #73620, #66637, #51465, .T. ) ;
#65430=CARTESIAN_POINT ( 'NONE',  ( 149.1903793729515257, 272.2416782560088677, 12.95958987445043675 ) ) ;
#65431=CARTESIAN_POINT ( 'NONE',  ( 155.2991919149069133, 279.6252298253222079, -1.573765988037651553 ) ) ;
#65432=CARTESIAN_POINT ( 'NONE',  ( 169.8115178593924099, 285.4166933214704045, -7.965421809193424352 ) ) ;
#65434=CARTESIAN_POINT ( 'NONE',  ( 157.4774070382625837, 270.9583249496453163, -14.71635891169374943 ) ) ;
#65435=CARTESIAN_POINT ( 'NONE',  ( 133.6606700321278822, 254.6427522451419065, 10.00000000000009237 ) ) ;
#65436=CARTESIAN_POINT ( 'NONE',  ( 173.1778226176500084, 284.7536295044762369, -13.02365280795374858 ) ) ;
#65438=CARTESIAN_POINT ( 'NONE',  ( 196.4390255720217908, 290.4046224503736653, 16.34739044515864848 ) ) ;
#65439=CARTESIAN_POINT ( 'NONE',  ( 148.2159754900428936, 273.9293952882992471, 9.267836332806297150 ) ) ;
#65440=CARTESIAN_POINT ( 'NONE',  ( 0.1486806056246424423, 161.7048013555410080, 4.594050593750051981 ) ) ;
#65441=CARTESIAN_POINT ( 'NONE',  ( 39.95835201613431309, 200.0024278399160949, 9.188101187500095079 ) ) ;
#65442=CARTESIAN_POINT ( 'NONE',  ( 178.8711053662235599, 258.8915962790593994, -11.54485168611661194 ) ) ;
#65445=DIRECTION ( 'NONE',  ( 0.9659258262890740854, -0.2588190451024993677, 8.659560562354725782E-17 ) ) ;
#65447=CARTESIAN_POINT ( 'NONE',  ( 190.1696443193688708, 301.2635093119881162, -4.804312979389741223 ) ) ;
#65449=CARTESIAN_POINT ( 'NONE',  ( 71.81202244518924260, 212.2677522451418497, 10.00000000000009592 ) ) ;
#65450=CARTESIAN_POINT ( 'NONE',  ( 69.64695893572810803, 221.0177522451419065, 5.000000000000046185 ) ) ;
#65453=CARTESIAN_POINT ( 'NONE',  ( 175.8939073520130592, 252.7054158260212375, 5.280091837693253964 ) ) ;
#65455=EDGE_CURVE ( 'NONE', #6076, #55290, #17368, .T. ) ;
#65456=CARTESIAN_POINT ( 'NONE',  ( 181.6779078793408075, 294.9161590443458749, 1.016312488909408618 ) ) ;
#65457=CARTESIAN_POINT ( 'NONE',  ( 52.05581792490468729, 190.8615022471902023, 5.000000000000051514 ) ) ;
#65458=CARTESIAN_POINT ( 'NONE',  ( 184.8842770087186125, 293.8891543674287732, 9.635832499575185395 ) ) ;
#65459=CARTESIAN_POINT ( 'NONE',  ( 163.1484656051875106, 248.0655637253488806, 9.714247672444804138 ) ) ;
#65460=CARTESIAN_POINT ( 'NONE',  ( 6.400214715252306341, 168.3768266524160140, 9.188101187500098632 ) ) ;
#65462=CARTESIAN_POINT ( 'NONE',  ( 163.8910887309009468, 247.2502849824839473, 6.562832656486317973 ) ) ;
#65463=EDGE_CURVE ( 'NONE', #12604, #25883, #40322, .T. ) ;
#65466=CARTESIAN_POINT ( 'NONE',  ( 156.2207618296380360, 261.2732867776778107, -17.42379591280306883 ) ) ;
#65467=VECTOR ( 'NONE', #23495, 1000.000000000000000 ) ;
#65468=CARTESIAN_POINT ( 'NONE',  ( 179.7401746537150871, 276.9590119395865031, 16.29634411216163414 ) ) ;
#65469=CARTESIAN_POINT ( 'NONE',  ( 149.0203866098534888, 272.5361143586139860, -12.73049804737905255 ) ) ;
#65470=CARTESIAN_POINT ( 'NONE',  ( 179.7646569558871192, 262.8383775195224530, -12.87982295168864866 ) ) ;
#65473=CARTESIAN_POINT ( 'NONE',  ( 165.6219050428149728, 285.3937648927450255, 0.4054896356418120629 ) ) ;
#65475=CARTESIAN_POINT ( 'NONE',  ( 159.1821849787265535, 259.3862596468384254, 16.68185694244520079 ) ) ;
#65478=CARTESIAN_POINT ( 'NONE',  ( 159.8597520197352537, 253.7617827468940277, -16.74905990210778839 ) ) ;
#65480=CARTESIAN_POINT ( 'NONE',  ( 152.4260784792123218, 267.7455040185449775, 15.55703180322229429 ) ) ;
#65481=CARTESIAN_POINT ( 'NONE',  ( 207.6007741873543750, 271.0719067473055475, 7.587922723682903658 ) ) ;
#65486=CARTESIAN_POINT ( 'NONE',  ( 159.1467459328969483, 279.6928109942932110, -9.939058806323174622 ) ) ;
#65487=FACE_OUTER_BOUND ( 'NONE', #1622, .T. ) ;
#65488=CARTESIAN_POINT ( 'NONE',  ( 152.7153488183568300, 266.1362520814392951, 17.33540622643059237 ) ) ;
#65495=CARTESIAN_POINT ( 'NONE',  ( 35.43895548624276159, 201.2677522451419350, -5.000000000000047962 ) ) ;
#65496=VECTOR ( 'NONE', #35817, 1000.000000000000000 ) ;
#65498=CARTESIAN_POINT ( 'NONE',  ( 200.7523954295751594, 282.9336467052548869, 18.23634913067694185 ) ) ;
#65499=CARTESIAN_POINT ( 'NONE',  ( 168.7291386885503641, 276.2063200971475112, -16.27615330769202728 ) ) ;
#65502=FACE_OUTER_BOUND ( 'NONE', #94704, .T. ) ;
#65505=ADVANCED_FACE ( 'NONE', ( #6955 ), #99195, .F. ) ;
#65509=DIRECTION ( 'NONE',  ( 0.4999999999999998890, -0.8660254037844385966, 0.000000000000000000 ) ) ;
#65511=CARTESIAN_POINT ( 'NONE',  ( 168.8236688076963787, 272.7617961321510620, 16.01230988885185624 ) ) ;
#65512=CARTESIAN_POINT ( 'NONE',  ( 147.5457841970795414, 275.0902006585022264, 5.820375447813823655 ) ) ;
#65513=CARTESIAN_POINT ( 'NONE',  ( 180.1740792144395016, 291.5944223663697699, -9.968613414868679357 ) ) ;
#65515=FACE_OUTER_BOUND ( 'NONE', #46927, .T. ) ;
#65517=CARTESIAN_POINT ( 'NONE',  ( 158.8485397013565148, 255.5132538595654808, -17.60067122166952913 ) ) ;
#65521=CARTESIAN_POINT ( 'NONE',  ( 164.3090168944849836, 246.0554299274959931, 2.641760039552302430 ) ) ;
#65522=CARTESIAN_POINT ( 'NONE',  ( 206.5479446040613141, 272.8954610772809133, 10.74757481123993230 ) ) ;
#65523=DIRECTION ( 'NONE',  ( -0.8660254037844387076, -0.4999999999999998890, -0.000000000000000000 ) ) ;
#65524=ORIENTED_EDGE ( 'NONE', *, *, #29297, .T. ) ;
#65526=CARTESIAN_POINT ( 'NONE',  ( 146.6728205609862528, 276.6022180293756492, -3.499970163110023513 ) ) ;
#65531=CARTESIAN_POINT ( 'NONE',  ( 198.8804936074056400, 286.1758757680331087, -18.57050748239813487 ) ) ;
#65532=CARTESIAN_POINT ( 'NONE',  ( 93.55286852290896604, 231.4865022471903444, 10.00000000000009415 ) ) ;
#65534=CARTESIAN_POINT ( 'NONE',  ( 167.6146168596400514, 252.8497314824998909, -12.44459218179994231 ) ) ;
#65536=CARTESIAN_POINT ( 'NONE',  ( 60.85245129477298320, 194.3932355074535678, -2.679491924311248496 ) ) ;
#65537=CARTESIAN_POINT ( 'NONE',  ( 164.4858674010174298, 245.7491158648375347, -2.958464974013825355 ) ) ;
#65538=CARTESIAN_POINT ( 'NONE',  ( 32.84087927488953085, 179.7677522451417929, -5.000000000000041744 ) ) ;
#65539=CARTESIAN_POINT ( 'NONE',  ( 103.0428032491157779, 239.4869531367911293, 4.594050593750046652 ) ) ;
#65540=VECTOR ( 'NONE', #96288, 1000.000000000000000 ) ;
#65541=CARTESIAN_POINT ( 'NONE',  ( 184.0050395437343980, 296.7880006952361214, -2.759016181532926382 ) ) ;
#65542=CARTESIAN_POINT ( 'NONE',  ( 164.1364888002910618, 280.6458552486410554, -11.61947351137251516 ) ) ;
#65545=CARTESIAN_POINT ( 'NONE',  ( 162.4198556707359842, 249.3275531507180460, 11.06129461055015106 ) ) ;
#65546=CARTESIAN_POINT ( 'NONE',  ( 20.25662117580333188, 176.3768266524159856, -9.188101187500091527 ) ) ;
#65547=CARTESIAN_POINT ( 'NONE',  ( 170.0754848107476960, 276.6018564280034866, -16.56579670670192073 ) ) ;
#65548=ORIENTED_EDGE ( 'NONE', *, *, #64953, .T. ) ;
#65550=CARTESIAN_POINT ( 'NONE',  ( 185.8492146212669240, 258.6745004276652935, -5.862532207920108540 ) ) ;
#65553=CARTESIAN_POINT ( 'NONE',  ( 193.3495834857956481, 263.1287464498848294, -3.752072735475438847 ) ) ;
#65555=( BOUNDED_CURVE ( )  B_SPLINE_CURVE ( 2, ( #48390, #86447, #72208, #48894, #8882, #95029, #79333, #55460, #9903 ),
 .UNSPECIFIED., .F., .T. ) 
 B_SPLINE_CURVE_WITH_KNOTS ( ( 3, 2, 2, 2, 3 ),
 ( 0.9475806451612903691, 0.9489247311827957443, 0.9516129032258064946, 0.9543010752688172449, 0.9556451612903226200 ),
 .UNSPECIFIED. ) 
 CURVE ( )  GEOMETRIC_REPRESENTATION_ITEM ( )  RATIONAL_B_SPLINE_CURVE ( ( 0.9330127018922194093, 0.9330127018922194093, 1.000000000000000000, 0.8660254037844387076, 1.000000000000000000, 0.8660254037844387076, 1.000000000000000000, 0.9330127018922194093, 0.9330127018922194093 ) ) 
 REPRESENTATION_ITEM ( '' )  );
#65556=CARTESIAN_POINT ( 'NONE',  ( 181.8556362198626175, 285.1488821084953429, 15.75693339034319251 ) ) ;
#65558=CARTESIAN_POINT ( 'NONE',  ( 43.96406660440233338, 190.0643266524159856, -9.188101187500093303 ) ) ;
#65559=CARTESIAN_POINT ( 'NONE',  ( 88.77168660263443201, 235.3927522451419634, 2.944929066748280225E-16 ) ) ;
#65562=B_SPLINE_CURVE_WITH_KNOTS ( 'NONE', 3,
 ( #33632, #349, #48836, #25525 ),
 .UNSPECIFIED., .F., .F.,
 ( 4, 4 ),
 ( 0.01050920366396543466, 0.01592988117231719167 ),
 .UNSPECIFIED. ) ;
#65563=CARTESIAN_POINT ( 'NONE',  ( 179.2174706742607952, 259.4863410742793235, -10.30736484160015465 ) ) ;
#65566=CARTESIAN_POINT ( 'NONE',  ( 2.394847222749281190, 166.0643266524160140, -9.188101187500093303 ) ) ;
#65569=CARTESIAN_POINT ( 'NONE',  ( 181.5558742819051474, 255.2544784655372894, -2.503599602330015994 ) ) ;
#65570=CARTESIAN_POINT ( 'NONE',  ( 193.1649355862271591, 296.0755126543221536, -12.21556774862162698 ) ) ;
#65572=CARTESIAN_POINT ( 'NONE',  ( 204.9608076533459950, 275.6444629144898499, 14.31488288944633069 ) ) ;
#65574=CARTESIAN_POINT ( 'NONE',  ( 147.6088797830324779, 274.9809158978982850, 8.531536684623960198 ) ) ;
#65576=CARTESIAN_POINT ( 'NONE',  ( 164.3602934812760452, 245.9666162739349318, -7.171958108566009571 ) ) ;
#65577=CARTESIAN_POINT ( 'NONE',  ( 8.321535033790526725, 165.6115022471902023, -5.000000000000041744 ) ) ;
#65579=CARTESIAN_POINT ( 'NONE',  ( 119.6326891643026471, 246.0024278399160949, -9.188101187500093303 ) ) ;
#65584=CARTESIAN_POINT ( 'NONE',  ( 187.7402798015425844, 292.1894069392869824, 13.83160755710144052 ) ) ;
#65587=CARTESIAN_POINT ( 'NONE',  ( 191.3375250863502970, 299.2406804863936145, 8.828791580707859410 ) ) ;
#65588=CARTESIAN_POINT ( 'NONE',  ( 163.7818144303927284, 246.9685713811793164, 8.963733003589158699 ) ) ;
#65589=CARTESIAN_POINT ( 'NONE',  ( 190.0601721553029222, 300.2863949309033842, 3.228815124723532382 ) ) ;
#65590=CARTESIAN_POINT ( 'NONE',  ( 173.5762231131973010, 289.9594224631762813, -1.068267067776312196 ) ) ;
#65594=CARTESIAN_POINT ( 'NONE',  ( 165.4786559991963202, 269.4527545339830681, -16.40171962000061967 ) ) ;
#65598=CARTESIAN_POINT ( 'NONE',  ( 30.67581576542834654, 198.5177522451419350, 5.000000000000046185 ) ) ;
#65600=CARTESIAN_POINT ( 'NONE',  ( 150.6217852516201106, 277.7502518432382885, -5.874856709598950559E-05 ) ) ;
#65601=CARTESIAN_POINT ( 'NONE',  ( 194.5273606940714330, 283.0013335026653181, 17.66207452344210438 ) ) ;
#65603=CARTESIAN_POINT ( 'NONE',  ( 186.1370921618058674, 283.3846817430978149, 17.26256540491417368 ) ) ;
#65605=CARTESIAN_POINT ( 'NONE',  ( 167.7082397602646324, 281.0209505053426824, 12.79449922633788894 ) ) ;
#65606=CARTESIAN_POINT ( 'NONE',  ( 194.4666154385731431, 293.8209370148700827, -14.56896502715340702 ) ) ;
#65611=CARTESIAN_POINT ( 'NONE',  ( 185.5891282490076435, 291.1072362729600513, 12.16301403431581818 ) ) ;
#65614=CARTESIAN_POINT ( 'NONE',  ( 93.48972083544241229, 224.7833772461660260, -9.188101187500095079 ) ) ;
#65617=CARTESIAN_POINT ( 'NONE',  ( 183.8303768749067899, 259.1719814329002816, -5.825300294667353995 ) ) ;
#65620=CARTESIAN_POINT ( 'NONE',  ( 105.1540004908901693, 221.5177522451418213, 5.000000000000051514 ) ) ;
#65622=CARTESIAN_POINT ( 'NONE',  ( 176.1640045926653499, 252.3529155287689321, -3.563159428949892682 ) ) ;
#65624=EDGE_CURVE ( 'NONE', #62997, #40327, #3384, .T. ) ;
#65626=CARTESIAN_POINT ( 'NONE',  ( 203.2187760522547819, 278.6617501559703101, -15.08675642319914978 ) ) ;
#65628=CARTESIAN_POINT ( 'NONE',  ( 206.8044235653369185, 272.4512264852788235, -7.311027623652901042 ) ) ;
#65629=CARTESIAN_POINT ( 'NONE',  ( 151.3601338604896682, 268.8932253746694983, 14.28446672321297939 ) ) ;
#65630=CARTESIAN_POINT ( 'NONE',  ( 158.6259107095311833, 274.9228465685866354, -12.63726120636060379 ) ) ;
#65631=EDGE_CURVE ( 'NONE', #61239, #11450, #28132, .T. ) ;
#65632=CARTESIAN_POINT ( 'NONE',  ( 200.6680263064462792, 283.0797783131037022, -17.21821073473145347 ) ) ;
#65636=CARTESIAN_POINT ( 'NONE',  ( 134.2197177853555843, 257.4869531367911577, 4.594050593750046652 ) ) ;
#65640=ORIENTED_EDGE ( 'NONE', *, *, #56188, .F. ) ;
#65642=CARTESIAN_POINT ( 'NONE',  ( 204.0134405048271447, 271.6787652324207443, 9.733109749488880524 ) ) ;
#65645=CARTESIAN_POINT ( 'NONE',  ( 170.7750159713022811, 288.2613212839527250, -5.614454501361259453 ) ) ;
#65646=CARTESIAN_POINT ( 'NONE',  ( 153.3013304660010760, 276.9256174101875558, 7.023167453551987904 ) ) ;
#65647=DIRECTION ( 'NONE',  ( 0.4999999999999992784, -0.8660254037844390407, 0.000000000000000000 ) ) ;
#65649=CARTESIAN_POINT ( 'NONE',  ( 192.6560709476634372, 292.3755120997685140, -14.35773016799012680 ) ) ;
#65651=CARTESIAN_POINT ( 'NONE',  ( 194.2605386096435893, 292.8896166215183143, 15.20382020497128472 ) ) ;
#65652=VERTEX_POINT ( 'NONE', #43710 ) ;
#65654=ORIENTED_EDGE ( 'NONE', *, *, #92042, .F. ) ;
#65656=CARTESIAN_POINT ( 'NONE',  ( 204.8652996567902278, 269.2354455564837963, -2.974687384846896876 ) ) ;
#65657=CARTESIAN_POINT ( 'NONE',  ( 163.9582657378243766, 246.6629487516456720, -7.496770747748987773 ) ) ;
#65659=CARTESIAN_POINT ( 'NONE',  ( 202.8499463704053198, 279.3005819042728604, 17.04674939340617001 ) ) ;
#65662=CARTESIAN_POINT ( 'NONE',  ( 166.1325645896313006, 247.4337816087006559, 6.210353822890861686 ) ) ;
#65663=ORIENTED_EDGE ( 'NONE', *, *, #12845, .T. ) ;
#65667=CARTESIAN_POINT ( 'NONE',  ( 190.2629546459234859, 273.4080951500121159, -16.67925241984795903 ) ) ;
#65670=CARTESIAN_POINT ( 'NONE',  ( 192.1640094933931096, 297.8091675017319062, 12.36911124822534447 ) ) ;
#65672=CARTESIAN_POINT ( 'NONE',  ( 41.64315915125185086, 206.3967562850347122, -4.648177544792955347E-16 ) ) ;
#65673=CARTESIAN_POINT ( 'NONE',  ( 16.06189740016370848, 170.8923013555409796, 4.594050593750050204 ) ) ;
#65674=CARTESIAN_POINT ( 'NONE',  ( 104.0981849360367875, 243.1589784336661921, -6.496448406907675876E-16 ) ) ;
#65675=CARTESIAN_POINT ( 'NONE',  ( 202.8151641853381477, 279.3608264160075692, -16.28741359973609448 ) ) ;
#65677=CARTESIAN_POINT ( 'NONE',  ( 180.9300408734833923, 255.0300470106541297, -2.486323749695340091 ) ) ;
#65679=EDGE_CURVE ( 'NONE', #51044, #33408, #55915, .T. ) ;
#65681=CARTESIAN_POINT ( 'NONE',  ( 164.0096516886412701, 284.3946043071177883, 5.908419196777021654 ) ) ;
#65682=CARTESIAN_POINT ( 'NONE',  ( 148.2352135776142177, 273.8960739431854563, -9.245976304249309052 ) ) ;
#65686=CARTESIAN_POINT ( 'NONE',  ( 140.5888732624033821, 258.6427522451418781, -10.00000000000009592 ) ) ;
#65688=CARTESIAN_POINT ( 'NONE',  ( 89.99855592466249732, 212.7677522451417929, -5.000000000000041744 ) ) ;
#65691=CARTESIAN_POINT ( 'NONE',  ( 78.44218234892278474, 228.3464784336661353, 1.353441290958777327E-15 ) ) ;
#65692=CARTESIAN_POINT ( 'NONE',  ( 161.0974665087481981, 251.6179983666593216, -13.69252715295363210 ) ) ;
#65695=CARTESIAN_POINT ( 'NONE',  ( 157.1837449796689725, 258.3967629017010381, 16.97243084443542216 ) ) ;
#65696=CARTESIAN_POINT ( 'NONE',  ( 199.8196579795990715, 284.5491953587354601, 17.07111731403734822 ) ) ;
#65697=CARTESIAN_POINT ( 'NONE',  ( 198.8157103782086210, 286.2880836124806478, -18.60729372713428020 ) ) ;
#65698=CARTESIAN_POINT ( 'NONE',  ( 173.1711317957924052, 268.1345242171204859, -16.28840157703276859 ) ) ;
#65702=VERTEX_POINT ( 'NONE', #85778 ) ;
#65705=DIRECTION ( 'NONE',  ( 0.5000000000000048850, -0.8660254037844358210, 0.000000000000000000 ) ) ;
#65709=CARTESIAN_POINT ( 'NONE',  ( 193.5969836369176562, 288.4623895989528251, 16.08576061698174797 ) ) ;
#65711=CARTESIAN_POINT ( 'NONE',  ( 131.8023238567217277, 240.2365022471901739, -10.00000000000009059 ) ) ;
#65712=CARTESIAN_POINT ( 'NONE',  ( 157.8811243250769110, 257.1888664433053009, -17.39256699147873064 ) ) ;
#65715=CARTESIAN_POINT ( 'NONE',  ( 169.5987612212706210, 248.4539404957666591, -1.946464333004839675 ) ) ;
#65717=CARTESIAN_POINT ( 'NONE',  ( 163.4004183463084416, 247.6291687766210146, 10.19167732382099345 ) ) ;
#65718=CARTESIAN_POINT ( 'NONE',  ( 173.2798715285074991, 281.8114527337138497, 15.08241540710736750 ) ) ;
#65723=CARTESIAN_POINT ( 'NONE',  ( 205.8720179146364160, 274.0662004455563761, 12.32128734042425933 ) ) ;
#65724=CARTESIAN_POINT ( 'NONE',  ( 142.3387059458346755, 262.1744531367911009, 4.594050593750047540 ) ) ;
#65726=CARTESIAN_POINT ( 'NONE',  ( 202.0271362839079643, 275.0056074051718724, -14.19488698628315326 ) ) ;
#65731=EDGE_CURVE ( 'NONE', #4325, #90496, #70924, .T. ) ;
#65732=CARTESIAN_POINT ( 'NONE',  ( 156.6812872898450735, 261.2670451491295012, 0.000000000000000000 ) ) ;
#65737=CARTESIAN_POINT ( 'NONE',  ( 184.8890758847559823, 296.9636581320273763, 1.025268066086537644 ) ) ;
#65738=CARTESIAN_POINT ( 'NONE',  ( 204.3371846825755824, 276.7246095846310823, 14.72513001683937262 ) ) ;
#65739=CARTESIAN_POINT ( 'NONE',  ( 147.9791529310278122, 274.3395839928920168, -7.789432462804474433 ) ) ;
#65742=CARTESIAN_POINT ( 'NONE',  ( 157.3834985187485529, 282.2511498796980050, -0.4876292292492137581 ) ) ;
#65744=EDGE_CURVE ( 'NONE', #46006, #1717, #25828, .T. ) ;
#65745=CARTESIAN_POINT ( 'NONE',  ( 208.1381420012782542, 270.1411583912371270, -4.612438132219912390 ) ) ;
#65749=CARTESIAN_POINT ( 'NONE',  ( 109.2678814824639204, 224.7048013555410080, 4.594050593750051981 ) ) ;
#65753=CARTESIAN_POINT ( 'NONE',  ( 163.0140611511896793, 276.5848272863240709, -14.06802711415683760 ) ) ;
#65754=ORIENTED_EDGE ( 'NONE', *, *, #8290, .T. ) ;
#65757=CARTESIAN_POINT ( 'NONE',  ( 177.0163663914809433, 292.4487994013190928, -2.715256582491245130 ) ) ;
#65758=CARTESIAN_POINT ( 'NONE',  ( 157.6335212189247557, 257.6177276032722716, 16.76495363836117036 ) ) ;
#65760=CARTESIAN_POINT ( 'NONE',  ( 208.2018443082727970, 270.0308227589636090, 1.727811837614598556 ) ) ;
#65761=CARTESIAN_POINT ( 'NONE',  ( 97.11602866590727956, 233.0024278399160664, 9.188101187500095079 ) ) ;
#65762=EDGE_LOOP ( 'NONE', ( #35927, #18654, #40189, #29981 ) ) ;
#65763=VERTEX_POINT ( 'NONE', #10720 ) ;
#65766=CARTESIAN_POINT ( 'NONE',  ( 194.2751985042537513, 266.1072248296521252, -7.746649050517742552 ) ) ;
#65769=CARTESIAN_POINT ( 'NONE',  ( 165.5604721375479755, 285.4306498218772390, 0.8607609473838128133 ) ) ;
#65770=CARTESIAN_POINT ( 'NONE',  ( 136.7913381204293728, 237.5327760586659736, 1.948934522072303157E-15 ) ) ;
#65773=FACE_OUTER_BOUND ( 'NONE', #36214, .T. ) ;
#65776=CARTESIAN_POINT ( 'NONE',  ( 205.0608432903593155, 275.4711961086152883, 13.55071766891341412 ) ) ;
#65780=CARTESIAN_POINT ( 'NONE',  ( 174.0424481033923314, 287.4814580433055653, 10.99910921803667208 ) ) ;
#65783=CARTESIAN_POINT ( 'NONE',  ( 197.1048653879311132, 280.7190563205994067, -16.61298024664429107 ) ) ;
#65784=CARTESIAN_POINT ( 'NONE',  ( 129.2042476453684117, 238.7365022471901739, -10.00000000000009237 ) ) ;
#65787=CARTESIAN_POINT ( 'NONE',  ( 206.7923762329701276, 272.4720930770340033, -9.496103119940368487 ) ) ;
#65789=CARTESIAN_POINT ( 'NONE',  ( 178.1281481821618797, 292.9991590599575488, -6.064681374715556572 ) ) ;
#65790=CARTESIAN_POINT ( 'NONE',  ( 163.2015365837845309, 247.9736420940113248, -10.76959291176343747 ) ) ;
#65791=EDGE_CURVE ( 'NONE', #47928, #39924, #32970, .T. ) ;
#65799=VECTOR ( 'NONE', #59149, 1000.000000000000000 ) ;
#65801=CARTESIAN_POINT ( 'NONE',  ( 14.51920287573142510, 173.0643266524160140, 9.188101187500095079 ) ) ;
#65802=CARTESIAN_POINT ( 'NONE',  ( -22.42236680055709641, 157.8615022471902591, 0.000000000000000000 ) ) ;
#65806=DIRECTION ( 'NONE',  ( 0.4999999999999992784, -0.8660254037844390407, 0.000000000000000000 ) ) ;
#65808=CARTESIAN_POINT ( 'NONE',  ( 44.74898890052324418, 187.4548013555409796, -4.594050593750042211 ) ) ;
#65809=CARTESIAN_POINT ( 'NONE',  ( 161.8811854682448939, 250.2605573099562264, 13.51112293479948789 ) ) ;
#65810=CARTESIAN_POINT ( 'NONE',  ( 190.7908437487391780, 300.1875603386860689, -4.317984972589949955 ) ) ;
#65812=CARTESIAN_POINT ( 'NONE',  ( 202.9528762288709061, 270.0503579255801014, -6.478656441495562746 ) ) ;
#65813=CARTESIAN_POINT ( 'NONE',  ( 191.6823192895500370, 298.6434794082964572, -8.424208857102787107 ) ) ;
#65816=CARTESIAN_POINT ( 'NONE',  ( 84.80240350195578003, 229.7677522451419350, -5.000000000000047962 ) ) ;
#65819=CARTESIAN_POINT ( 'NONE',  ( 192.5112645657038684, 295.4124808762264252, -13.34516070875820759 ) ) ;
#65820=CARTESIAN_POINT ( 'NONE',  ( 77.96441125478908418, 222.4865022471903160, 10.00000000000009237 ) ) ;
#65824=CARTESIAN_POINT ( 'NONE',  ( 43.80151329331025067, 196.0958772461660544, -9.188101187500095079 ) ) ;
#65826=CARTESIAN_POINT ( 'NONE',  ( 162.5761427237234784, 263.2594962941460608, 17.31260787709388538 ) ) ;
#65827=CARTESIAN_POINT ( 'NONE',  ( 198.7136873185829984, 286.4647927352960437, -18.57144721070432070 ) ) ;
#65830=CARTESIAN_POINT ( 'NONE',  ( 171.3312619405691066, 286.5464919449711374, 7.566358419436266303 ) ) ;
#65831=CARTESIAN_POINT ( 'NONE',  ( 164.2723164851102808, 246.1189969011916503, -1.993789335506892302 ) ) ;
#65834=CARTESIAN_POINT ( 'NONE',  ( 189.6437701857260549, 264.6299060724186347, 10.65328101858895771 ) ) ;
#65837=CARTESIAN_POINT ( 'NONE',  ( 171.2977123844769949, 255.8120995149402859, 11.88195947517418283 ) ) ;
#65838=ORIENTED_EDGE ( 'NONE', *, *, #89036, .T. ) ;
#65842=CARTESIAN_POINT ( 'NONE',  ( 174.7964402711189393, 255.1616715225093515, 8.226461705621156639 ) ) ;
#65844=EDGE_CURVE ( 'NONE', #18147, #34226, #11299, .T. ) ;
#65845=ORIENTED_EDGE ( 'NONE', *, *, #68247, .F. ) ;
#65846=CARTESIAN_POINT ( 'NONE',  ( 182.6345022024692355, 283.7833407587357897, 15.47623830145432855 ) ) ;
#65848=CARTESIAN_POINT ( 'NONE',  ( 169.1311965936330353, 247.8770103324328034, 7.134965090537657859E-13 ) ) ;
#65849=ORIENTED_EDGE ( 'NONE', *, *, #23090, .T. ) ;
#65852=VECTOR ( 'NONE', #28642, 1000.000000000000000 ) ;
#65853=( BOUNDED_CURVE ( )  B_SPLINE_CURVE ( 2, ( #9271, #41650, #87351, #71085, #24955, #93404, #32047, #17358, #93910 ),
 .UNSPECIFIED., .F., .T. ) 
 B_SPLINE_CURVE_WITH_KNOTS ( ( 3, 2, 2, 2, 3 ),
 ( 0.3024193548387096864, 0.3037634408602150615, 0.3064516129032258118, 0.3091397849462365621, 0.3104838709677419373 ),
 .UNSPECIFIED. ) 
 CURVE ( )  GEOMETRIC_REPRESENTATION_ITEM ( )  RATIONAL_B_SPLINE_CURVE ( ( 0.9330127018922194093, 0.9330127018922194093, 1.000000000000000000, 0.8660254037844387076, 1.000000000000000000, 0.8660254037844387076, 1.000000000000000000, 0.9330127018922194093, 0.9330127018922194093 ) ) 
 REPRESENTATION_ITEM ( '' )  );
#65854=CARTESIAN_POINT ( 'NONE',  ( 161.5083988044524119, 250.9062427520286178, -14.53522982831775856 ) ) ;
#65856=CARTESIAN_POINT ( 'NONE',  ( 149.0598351764325002, 272.4677874370131576, -11.59078276432863674 ) ) ;
#65859=CARTESIAN_POINT ( 'NONE',  ( 159.3169041484411537, 254.7020228407560580, 16.67170756419672628 ) ) ;
#65860=CARTESIAN_POINT ( 'NONE',  ( 180.9962514683335257, 255.6518059654043782, 5.281628127585873855 ) ) ;
#65863=CARTESIAN_POINT ( 'NONE',  ( 114.2743305262689404, 236.7833772461660544, -9.188101187500095079 ) ) ;
#65865=CARTESIAN_POINT ( 'NONE',  ( 190.3167824967908643, 299.0086585129598689, -8.112609889089975823 ) ) ;
#65866=CARTESIAN_POINT ( 'NONE',  ( 149.2923684163597784, 272.0650280510108701, -12.99082738998495756 ) ) ;
#65867=CARTESIAN_POINT ( 'NONE',  ( 35.89232211637455094, 179.9824982072973683, 3.021315404115420679E-15 ) ) ;
#65870=CARTESIAN_POINT ( 'NONE',  ( 201.3965252030675686, 280.5319479810296457, 16.51675258086747533 ) ) ;
#65874=CARTESIAN_POINT ( 'NONE',  ( 159.9307118030769175, 253.6388767968520881, 16.60600887889890487 ) ) ;
#65877=CARTESIAN_POINT ( 'NONE',  ( 69.15955932604958889, 219.9244531367911293, -4.594050593750046652 ) ) ;
#65880=CARTESIAN_POINT ( 'NONE',  ( 190.9501423151522772, 299.9116471280854626, 8.746938802470586083 ) ) ;
#65882=CARTESIAN_POINT ( 'NONE',  ( 172.2733305175966620, 277.0538235811624759, 16.56964073552936867 ) ) ;
#65883=ORIENTED_EDGE ( 'NONE', *, *, #52238, .F. ) ;
#65884=CARTESIAN_POINT ( 'NONE',  ( 179.5196496019146650, 266.1175816663657656, 16.29367087753972498 ) ) ;
#65886=CARTESIAN_POINT ( 'NONE',  ( 203.1705638993064156, 278.7452560544191442, -15.08126533799095093 ) ) ;
#65888=CARTESIAN_POINT ( 'NONE',  ( 194.7178830804197673, 293.3857286928936219, 15.96025387054093869 ) ) ;
#65890=CARTESIAN_POINT ( 'NONE',  ( 163.8562647933944731, 260.4330591941297826, -16.17453866336511581 ) ) ;
#65893=CARTESIAN_POINT ( 'NONE',  ( 206.4943150373521803, 272.9883502116088039, 11.34100825923693101 ) ) ;
#65894=CARTESIAN_POINT ( 'NONE',  ( 206.3106310032756596, 273.3065002911688453, 10.17860425536756175 ) ) ;
#65895=CARTESIAN_POINT ( 'NONE',  ( 134.1658515176688411, 238.2677522451417929, -5.000000000000041744 ) ) ;
#65896=CARTESIAN_POINT ( 'NONE',  ( 167.6280379227422941, 256.4154598753431742, 13.62701025628873097 ) ) ;
#65898=CARTESIAN_POINT ( 'NONE',  ( 208.3152833949211526, 269.8343404973242059, 2.763633873278860342 ) ) ;
#65899=CARTESIAN_POINT ( 'NONE',  ( 128.8345561752773278, 239.0643266524160140, 9.188101187500095079 ) ) ;
#65903=CARTESIAN_POINT ( 'NONE',  ( 168.6768854746088664, 281.1804913396564984, -13.82603935691987296 ) ) ;
#65904=CARTESIAN_POINT ( 'NONE',  ( 164.3330377059402849, 246.0138246616164110, 7.208046019122525294 ) ) ;
#65909=B_SPLINE_CURVE_WITH_KNOTS ( 'NONE', 3,
 ( #21448, #21937, #75167, #7228, #69026, #60919, #36135, #52829, #45233, #99457, #76642, #67538, #30033, #22926, #98467, #22438, #53331, #76169, #99956, #53813, #38112, #75655, #29061, #97963, #52334, #20975, #61426, #84777, #28538, #6240, #59420, #83783, #90400, #84286, #14830, #37134, #59928, #29545, #68040, #14345, #90898, #51856, #60418, #37623, #68534, #82797, #13363, #16829 ),
 .UNSPECIFIED., .F., .F.,
 ( 4, 2, 2, 2, 2, 2, 2, 2, 2, 2, 2, 2, 2, 2, 2, 2, 2, 2, 2, 2, 2, 2, 2, 4 ),
 ( 0.0001718391672230527530, 0.001192457371175957440, 0.001702766473152372839, 0.001830343748646495608, 0.001957921024140618811, 0.002085498299634741797, 0.002213075575128864783, 0.002468230126117043101, 0.002723384677105221852, 0.003233693779081678234, 0.004254311983034685975, 0.005274930186987694149, 0.005785239288964233798, 0.006040393839952425993, 0.006295548390940617321, 0.006359337028687664720, 0.006423125666434712118, 0.006550702941928721046, 0.006805857492916878547, 0.007316166594893006199, 0.007571321145881069158, 0.007826475696869132984, 0.008081630247857197677, 0.008336784798845260636 ),
 .UNSPECIFIED. ) ;
#65910=DIRECTION ( 'NONE',  ( -0.8660254037844387076, -0.4999999999999998890, -0.000000000000000000 ) ) ;
#65911=CARTESIAN_POINT ( 'NONE',  ( 164.9133935349224203, 245.0086188793504505, -2.355115420316610919 ) ) ;
#65913=CARTESIAN_POINT ( 'NONE',  ( 195.5576243985897236, 263.4396298511827013, 0.8694183353164576245 ) ) ;
#65914=CARTESIAN_POINT ( 'NONE',  ( 190.3791419447713906, 300.9006487807255326, -5.688668718458480988 ) ) ;
#65918=CARTESIAN_POINT ( 'NONE',  ( 170.7113395477583424, 250.4904927623917104, 3.433421072208380220 ) ) ;
#65921=CARTESIAN_POINT ( 'NONE',  ( 190.8153366230912411, 300.1451374358846920, 3.771947273125533684 ) ) ;
#65922=CARTESIAN_POINT ( 'NONE',  ( 188.4688990864094080, 295.3997683978527675, -11.43812978727723717 ) ) ;
#65923=CARTESIAN_POINT ( 'NONE',  ( 169.2909702781398664, 285.2592091808388659, -8.894609513033637782 ) ) ;
#65924=B_SPLINE_CURVE_WITH_KNOTS ( 'NONE', 3,
 ( #55903, #86897, #1237, #94977, #31117, #32120, #63030, #69626, #79286, #24527, #55406, #9859, #40718, #71663, #92958, #33132, #64034, #25541, #56428, #46307, #77232, #7839, #38720, #56920, #80281, #48850, #50325, #19469, #65038, #19944, #64540, #80792, #10348, #49833, #43208, #2761, #10847, #81277, #41724, #87909, #57926, #42708, #88906, #11367, #33651, #18956, #95985, #26049, #26548, #3750 ),
 .UNSPECIFIED., .F., .F.,
 ( 4, 2, 2, 2, 2, 2, 2, 2, 2, 2, 2, 2, 2, 2, 2, 2, 2, 2, 2, 2, 2, 2, 2, 2, 4 ),
 ( 0.0006375827441053666606, 0.001063963319884116175, 0.001277153607773526441, 0.001383748751718216069, 0.001490343895662905697, 0.001703534183552284954, 0.001916724471441664211, 0.002343105047220586656, 0.003195866198778431980, 0.004048627350336277304, 0.004901388501894122195, 0.005327769077673054181, 0.005540959365562520174, 0.005647554509507253170, 0.005700852081479585408, 0.005754149653451917645, 0.005807447225424249883, 0.005860744797396582120, 0.005967339941341270881, 0.006180530229230528708, 0.006606910805009000125, 0.006820101092898229328, 0.007033291380787459399, 0.007246481668676688602, 0.007459671956565918673 ),
 .UNSPECIFIED. ) ;
#65925=CARTESIAN_POINT ( 'NONE',  ( 155.3716771045260714, 261.5353565282119348, -18.54934131471355840 ) ) ;
#65926=CARTESIAN_POINT ( 'NONE',  ( 193.9750484533059591, 288.7567388352306352, 16.08761660616773170 ) ) ;
#65928=CARTESIAN_POINT ( 'NONE',  ( 141.5270674498366077, 242.5177522451417929, 5.000000000000051514 ) ) ;
#65932=CARTESIAN_POINT ( 'NONE',  ( 195.9920715006079490, 291.1787696107118677, 15.99608784761372071 ) ) ;
#65933=B_SPLINE_CURVE_WITH_KNOTS ( 'NONE', 3,
 ( #68039, #29544, #98960, #14829, #43734, #84285, #66548, #97477, #83782, #67036, #28043, #52333, #58919, #91372 ),
 .UNSPECIFIED., .F., .F.,
 ( 4, 2, 2, 2, 2, 2, 4 ),
 ( 0.001016148850039182410, 0.001267816211751153889, 0.001519483573463125368, 0.001771150935175097065, 0.002022818296887068327, 0.002526153020311010418, 0.003029487743734952075 ),
 .UNSPECIFIED. ) ;
#65934=CARTESIAN_POINT ( 'NONE',  ( 148.3519871123208986, 273.6938162480936398, 8.180046468253793890 ) ) ;
#65935=CARTESIAN_POINT ( 'NONE',  ( -7.131779314644562717, 172.8149278399161233, 9.188101187500093303 ) ) ;
#65936=B_SPLINE_CURVE_WITH_KNOTS ( 'NONE', 3,
 ( #93179, #23732, #46024, #54627 ),
 .UNSPECIFIED., .F., .F.,
 ( 4, 4 ),
 ( 0.04193484224020654905, 0.04887066958154938356 ),
 .UNSPECIFIED. ) ;
#65937=CARTESIAN_POINT ( 'NONE',  ( 36.87296296726972855, 204.3464784336661637, 1.353441290958777327E-15 ) ) ;
#65938=CARTESIAN_POINT ( 'NONE',  ( 179.0286630115520552, 258.6160276279643995, -11.58942154470568120 ) ) ;
#65940=DIRECTION ( 'NONE',  ( 0.4999999999999998890, -0.8660254037844385966, 0.000000000000000000 ) ) ;
#65942=CARTESIAN_POINT ( 'NONE',  ( 157.8696211474012330, 257.2087905314882619, -17.27527248276125604 ) ) ;
#65945=CARTESIAN_POINT ( 'NONE',  ( 149.7049461522049398, 276.2981810546235693, 3.707541583551217546 ) ) ;
#65946=CARTESIAN_POINT ( 'NONE',  ( 77.46154149802761424, 203.9824982072973967, 3.021315404115420679E-15 ) ) ;
#65949=CARTESIAN_POINT ( 'NONE',  ( 157.5487431480040925, 257.7645675294749594, -18.29554785922338311 ) ) ;
#65950=CARTESIAN_POINT ( 'NONE',  ( 198.0355408163131585, 287.6393769322024241, 18.20720360189982756 ) ) ;
#65952=CARTESIAN_POINT ( 'NONE',  ( 179.0941012263468224, 294.2742093295549921, 1.060795132963676446 ) ) ;
#65953=CARTESIAN_POINT ( 'NONE',  ( 38.12724268070488876, 199.4865022471903160, -10.00000000000009415 ) ) ;
#65954=CARTESIAN_POINT ( 'NONE',  ( 181.7815335863513155, 291.6605149460361304, 9.238327825430930673 ) ) ;
#65957=CARTESIAN_POINT ( 'NONE',  ( 6.129408228687162286, 174.3458772461660828, 9.188101187500095079 ) ) ;
#65958=CARTESIAN_POINT ( 'NONE',  ( 164.8661019620574564, 285.8049561880657734, 4.405979315412141162 ) ) ;
#65960=CARTESIAN_POINT ( 'NONE',  ( 192.8010417052266234, 296.7057953447782097, 12.10593424093686643 ) ) ;
#65963=CARTESIAN_POINT ( 'NONE',  ( 207.5686001603237116, 271.1276337968068333, 7.659944433763431704 ) ) ;
#65964=CARTESIAN_POINT ( 'NONE',  ( 154.8596847415876994, 262.4221533139083817, 17.65401077761399762 ) ) ;
#65965=CARTESIAN_POINT ( 'NONE',  ( 149.1004267900891307, 272.3974806997987343, -12.86882154300063341 ) ) ;
#65966=CARTESIAN_POINT ( 'NONE',  ( 177.9552638626009298, 260.7378092407702184, -13.94576028113082877 ) ) ;
#65969=CARTESIAN_POINT ( 'NONE',  ( 165.5860183037962088, 285.4175239968740243, 0.2436608606880265870 ) ) ;
#65971=CARTESIAN_POINT ( 'NONE',  ( 185.5826357821268289, 271.8226265777869912, -17.01680751177637063 ) ) ;
#65972=CARTESIAN_POINT ( 'NONE',  ( 152.6547697591180111, 278.7515079535921814, -4.825746761778547445 ) ) ;
#65973=EDGE_LOOP ( 'NONE', ( #24272, #70747, #66252, #52045 ) ) ;
#65976=CARTESIAN_POINT ( 'NONE',  ( 159.7692415128758228, 253.9185515433934768, -16.85856106119654285 ) ) ;
#65978=ORIENTED_EDGE ( 'NONE', *, *, #66888, .F. ) ;
#65979=CARTESIAN_POINT ( 'NONE',  ( 152.3689561497722025, 267.5166801192429489, 15.45798366088414433 ) ) ;
#65980=CARTESIAN_POINT ( 'NONE',  ( 206.9026071836525205, 272.2811674698855313, 7.240992997279449561 ) ) ;
#65984=VERTEX_POINT ( 'NONE', #33865 ) ;
#65986=CARTESIAN_POINT ( 'NONE',  ( 159.7094009514765673, 278.7085482198767181, -9.578478531124655859 ) ) ;
#65987=CARTESIAN_POINT ( 'NONE',  ( 204.2457645315488719, 276.8829539310449945, 14.53406579917280261 ) ) ;
#65988=CARTESIAN_POINT ( 'NONE',  ( 192.0332533962074706, 298.0356437054567778, 11.70630383928353346 ) ) ;
#65989=ORIENTED_EDGE ( 'NONE', *, *, #25121, .F. ) ;
#65991=CARTESIAN_POINT ( 'NONE',  ( 178.0177195456097934, 264.0150987585001303, 14.74376966487514728 ) ) ;
#65996=EDGE_CURVE ( 'NONE', #70505, #45420, #83793, .T. ) ;
#65998=CARTESIAN_POINT ( 'NONE',  ( 181.8559320684326224, 273.7276056269956257, 17.73031764801637067 ) ) ;
#65999=ORIENTED_EDGE ( 'NONE', *, *, #89791, .T. ) ;
#66000=CARTESIAN_POINT ( 'NONE',  ( 159.7174048142719300, 254.4296914360206188, -15.32135016668171268 ) ) ;
#66001=CARTESIAN_POINT ( 'NONE',  ( 166.2676906195303843, 273.7285489158338123, -15.68808713425968726 ) ) ;
#66005=ADVANCED_FACE ( 'NONE', ( #61103 ), #13056, .T. ) ;
#66006=CARTESIAN_POINT ( 'NONE',  ( 177.8451913026518696, 279.4803919955936635, -16.40387529202023487 ) ) ;
#66007=CARTESIAN_POINT ( 'NONE',  ( 169.2792358738191467, 261.7039271258366853, -15.92131019875227871 ) ) ;
#66010=CARTESIAN_POINT ( 'NONE',  ( 156.7768383517496886, 266.5326515087351140, -16.24880001600576662 ) ) ;
#66016=CARTESIAN_POINT ( 'NONE',  ( 193.3179319617974556, 295.8105151584606460, 14.44946628013603984 ) ) ;
#66017=CARTESIAN_POINT ( 'NONE',  ( 189.5844812082644921, 299.2301777039353397, -4.284560523659924236 ) ) ;
#66019=CARTESIAN_POINT ( 'NONE',  ( 152.6992418905140028, 266.1641500988167763, 17.27767170937316621 ) ) ;
#66021=CARTESIAN_POINT ( 'NONE',  ( 159.0721002551609615, 255.1260356218077447, -16.41935828481064163 ) ) ;
#66023=ORIENTED_EDGE ( 'NONE', *, *, #57162, .T. ) ;
#66026=CARTESIAN_POINT ( 'NONE',  ( 165.6020508749395219, 253.3981458705029013, 13.80445833791507404 ) ) ;
#66029=VERTEX_POINT ( 'NONE', #93551 ) ;
#66030=ORIENTED_EDGE ( 'NONE', *, *, #94579, .T. ) ;
#66032=CARTESIAN_POINT ( 'NONE',  ( 186.7717813178919641, 276.6902415280541732, 16.68087175089405250 ) ) ;
#66034=CARTESIAN_POINT ( 'NONE',  ( 163.7042615485562749, 247.9028158862528244, 8.306869792309049316 ) ) ;
#66036=CARTESIAN_POINT ( 'NONE',  ( 199.3060188183595471, 285.4388444827598050, -18.38090059002489696 ) ) ;
#66037=CARTESIAN_POINT ( 'NONE',  ( 190.1033615149403033, 301.3783144969264640, 0.1109884230970359376 ) ) ;
#66039=CARTESIAN_POINT ( 'NONE',  ( -22.42236680055709641, 157.8615022471902591, 0.000000000000000000 ) ) ;
#66040=CARTESIAN_POINT ( 'NONE',  ( 185.0338664617105735, 285.2265299937916438, -16.56857016979445874 ) ) ;
#66045=CARTESIAN_POINT ( 'NONE',  ( 35.43895548624280423, 191.2677522451418781, 10.00000000000009592 ) ) ;
#66046=CARTESIAN_POINT ( 'NONE',  ( 112.2989703957094605, 226.4548013555409796, -4.594050593750042211 ) ) ;
#66047=CARTESIAN_POINT ( 'NONE',  ( 181.0435294081004827, 294.2478791158599165, -2.647642130805165195 ) ) ;
#66048=CARTESIAN_POINT ( 'NONE',  ( 167.2900023830132170, 283.1360949131732809, -11.47530909209802275 ) ) ;
#66050=CARTESIAN_POINT ( 'NONE',  ( 208.3210024379012282, 269.8244348243121635, 2.045688540111487264 ) ) ;
#66051=CARTESIAN_POINT ( 'NONE',  ( 22.47598482088346117, 171.5327760586659451, 1.948934522072303157E-15 ) ) ;
#66052=DIRECTION ( 'NONE',  ( 0.4999999999999992784, -0.8660254037844390407, 0.000000000000000000 ) ) ;
#66053=ORIENTED_EDGE ( 'NONE', *, *, #40780, .F. ) ;
#66054=ORIENTED_EDGE ( 'NONE', *, *, #41807, .F. ) ;
#66056=CARTESIAN_POINT ( 'NONE',  ( 185.7739710534217181, 258.8015903883575675, -5.557864263316704800 ) ) ;
#66058=CARTESIAN_POINT ( 'NONE',  ( 193.6400864899449914, 264.2141502298499631, -4.346378420391690867 ) ) ;
#66060=CARTESIAN_POINT ( 'NONE',  ( 185.5250016208995874, 286.2042338949377722, 15.39722344320556680 ) ) ;
#66062=CARTESIAN_POINT ( 'NONE',  ( 46.88655524640979166, 204.0024278399160949, -9.188101187500093303 ) ) ;
#66063=CARTESIAN_POINT ( 'NONE',  ( 85.23541620384800410, 230.0177522451419350, 5.000000000000046185 ) ) ;
#66064=CIRCLE ( 'NONE', #22375, 17.82106496071138224 ) ;
#66067=ADVANCED_FACE ( 'NONE', ( #16014 ), #47894, .T. ) ;
#66068=CARTESIAN_POINT ( 'NONE',  ( -5.174027508517049512, 174.4865022471903160, 10.00000000000009415 ) ) ;
#66070=CARTESIAN_POINT ( 'NONE',  ( -1.340060878953613477, 170.0333772461660828, 9.188101187500095079 ) ) ;
#66073=CARTESIAN_POINT ( 'NONE',  ( 198.9590707264871412, 286.0397762054715827, -17.05306195936250191 ) ) ;
#66075=CARTESIAN_POINT ( 'NONE',  ( 146.8153075009282134, 276.3554234099810287, -4.113808735271278216 ) ) ;
#66080=CARTESIAN_POINT ( 'NONE',  ( 164.4858674010174298, 245.7491158648375347, -2.958464974013825355 ) ) ;
#66081=VERTEX_POINT ( 'NONE', #70712 ) ;
#66083=CARTESIAN_POINT ( 'NONE',  ( -4.668846022976141263, 178.1115022471903160, -5.000000000000047962 ) ) ;
#66085=CARTESIAN_POINT ( 'NONE',  ( 125.1810982770029881, 233.8923013555409796, 4.594050593750050204 ) ) ;
#66091=ORIENTED_EDGE ( 'NONE', *, *, #36457, .T. ) ;
#66092=CARTESIAN_POINT ( 'NONE',  ( 151.4361976351029000, 268.3518069213970421, 15.15218985681980612 ) ) ;
#66093=CARTESIAN_POINT ( 'NONE',  ( 207.6125545502318346, 271.0515025602701940, -0.9531936345505281905 ) ) ;
#66094=CARTESIAN_POINT ( 'NONE',  ( 190.6291740046558232, 300.0075276777452586, 3.996728472176227509 ) ) ;
#66097=ORIENTED_EDGE ( 'NONE', *, *, #36360, .F. ) ;
#66102=CARTESIAN_POINT ( 'NONE',  ( 198.9271290976750208, 272.1319763448123581, 12.23897718048457151 ) ) ;
#66103=DIRECTION ( 'NONE',  ( 0.8660254037844395958, 0.4999999999999985567, 0.000000000000000000 ) ) ;
#66105=CARTESIAN_POINT ( 'NONE',  ( 148.5064712399015718, 274.2256579647487342, -7.884393238739946241 ) ) ;
#66106=EDGE_CURVE ( 'NONE', #90058, #44657, #27079, .T. ) ;
#66111=CARTESIAN_POINT ( 'NONE',  ( 148.3874010092782498, 273.6324775792697892, -8.328854486678444857 ) ) ;
#66112=CARTESIAN_POINT ( 'NONE',  ( 159.5557817863224557, 264.0312905115982289, -17.30914965676515038 ) ) ;
#66117=CARTESIAN_POINT ( 'NONE',  ( 189.5650719070094112, 268.9827374331138685, -14.62586421207108955 ) ) ;
#66119=CARTESIAN_POINT ( 'NONE',  ( 83.63833477162943097, 231.3464784336661637, 1.353441290958777525E-15 ) ) ;
#66125=CARTESIAN_POINT ( 'NONE',  ( 198.2505066714982149, 285.2670451491296149, 0.000000000000000000 ) ) ;
#66128=B_SPLINE_CURVE_WITH_KNOTS ( 'NONE', 3,
 ( #80018, #85633, #31862, #62762 ),
 .UNSPECIFIED., .F., .F.,
 ( 4, 4 ),
 ( 0.009429426956353095107, 0.01478986007845733280 ),
 .UNSPECIFIED. ) ;
#66130=CARTESIAN_POINT ( 'NONE',  ( 171.5402001534711189, 272.6215992900089873, -17.66257148859359560 ) ) ;
#66131=CARTESIAN_POINT ( 'NONE',  ( 203.0862352702880003, 278.8913175244117610, -15.09542727681365015 ) ) ;
#66132=ORIENTED_EDGE ( 'NONE', *, *, #19988, .T. ) ;
#66133=CARTESIAN_POINT ( 'NONE',  ( 192.3926678149021825, 295.4131196713046847, -13.42882169270698256 ) ) ;
#66135=CARTESIAN_POINT ( 'NONE',  ( 151.4587940952941381, 268.7129208180788851, 14.41012130913438050 ) ) ;
#66138=CARTESIAN_POINT ( 'NONE',  ( 172.6505904036989136, 280.8448313155626579, -15.39888677054324440 ) ) ;
#66141=CARTESIAN_POINT ( 'NONE',  ( 141.2293712190596011, 252.3458772461660260, 9.188101187500095079 ) ) ;
#66142=DIRECTION ( 'NONE',  ( -0.8660254037844387076, -0.4999999999999998890, -0.000000000000000000 ) ) ;
#66144=B_SPLINE_CURVE_WITH_KNOTS ( 'NONE', 3,
 ( #47756, #85848, #17893, #8777, #9800, #56862 ),
 .UNSPECIFIED., .F., .F.,
 ( 4, 2, 4 ),
 ( 0.000000000000000000, 0.0004889391310944574218, 0.0009778782621889148437 ),
 .UNSPECIFIED. ) ;
#66149=CARTESIAN_POINT ( 'NONE',  ( 163.9835549846052913, 281.8964108386193743, 8.550639651353808546 ) ) ;
#66153=DIRECTION ( 'NONE',  ( -0.8660254037844387076, -0.4999999999999998890, -0.000000000000000000 ) ) ;
#66154=CARTESIAN_POINT ( 'NONE',  ( 170.5277015564773535, 288.6887139008781560, -5.574706778066785162 ) ) ;
#66155=CARTESIAN_POINT ( 'NONE',  ( 154.7406134505728232, 277.6489013670466193, 7.166873607358588139 ) ) ;
#66156=CARTESIAN_POINT ( 'NONE',  ( 165.4256356872135427, 246.8481156136332970, -1.873358472144460274 ) ) ;
#66157=CARTESIAN_POINT ( 'NONE',  ( 174.8559098654806689, 282.1809755462382441, 14.33990550510826090 ) ) ;
#66161=( BOUNDED_CURVE ( )  B_SPLINE_CURVE ( 2, ( #75273, #5366, #97586, #21560, #36743, #98582, #75771, #66166, #28158 ),
 .UNSPECIFIED., .F., .T. ) 
 B_SPLINE_CURVE_WITH_KNOTS ( ( 3, 2, 2, 2, 3 ),
 ( 0.1250000000000000000, 0.1263440860215053752, 0.1290322580645161255, 0.1317204301075268758, 0.1330645161290322509 ),
 .UNSPECIFIED. ) 
 CURVE ( )  GEOMETRIC_REPRESENTATION_ITEM ( )  RATIONAL_B_SPLINE_CURVE ( ( 0.9330127018922194093, 0.9330127018922194093, 1.000000000000000000, 0.8660254037844387076, 1.000000000000000000, 0.8660254037844387076, 1.000000000000000000, 0.9330127018922194093, 0.9330127018922194093 ) ) 
 REPRESENTATION_ITEM ( '' )  );
#66162=ORIENTED_EDGE ( 'NONE', *, *, #15644, .F. ) ;
#66163=CARTESIAN_POINT ( 'NONE',  ( 184.9083320494203235, 273.0902778310993426, -16.51607607619348528 ) ) ;
#66166=CARTESIAN_POINT ( 'NONE',  ( 2.555990577167667421, 183.8297689869268936, -2.679491924311252493 ) ) ;
#66167=CARTESIAN_POINT ( 'NONE',  ( 202.8161320915185968, 268.6936331435907732, -2.878963594486870115 ) ) ;
#66169=CARTESIAN_POINT ( 'NONE',  ( 190.0707697440390689, 301.4347651000360884, 4.271360729158901748 ) ) ;
#66176=B_SPLINE_SURFACE_WITH_KNOTS ( 'NONE', 3, 1, ( 
 ( #58104, #89086 ),
 ( #65697, #80966 ),
 ( #5901, #21127 ),
 ( #43393, #67198 ),
 ( #74832, #75323 ),
 ( #13030, #81943 ),
 ( #43892, #89560 ),
 ( #27221, #59581 ),
 ( #5412, #36792 ),
 ( #82947, #66698 ),
 ( #73324, #67704 ),
 ( #20121, #19635 ),
 ( #50495, #36295 ),
 ( #52004, #13520 ),
 ( #50993, #81449 ),
 ( #12521, #11531 ),
 ( #4405, #42391 ),
 ( #3913, #12021 ),
 ( #73811, #35301 ),
 ( #74336, #44883 ),
 ( #75823, #46891 ),
 ( #30194, #15992 ),
 ( #45868, #62070 ),
 ( #37782, #6410 ),
 ( #77815, #83438 ),
 ( #91532, #29212 ),
 ( #61080, #69187 ),
 ( #60080, #23573 ),
 ( #92051, #92532 ),
 ( #14004, #23079 ),
 ( #53971, #6892 ),
 ( #76793, #15474 ),
 ( #99616, #84437 ),
 ( #69687, #85443 ) ),
 .UNSPECIFIED., .T., .F., .F.,
 ( 4, 2, 2, 2, 2, 2, 2, 2, 2, 2, 2, 2, 2, 2, 2, 2, 4 ),
 ( 2, 2 ),
 ( 0.000000000000000000, 0.06250000000000000000, 0.1250000000000000000, 0.1875000000000000000, 0.2500000000000000000, 0.3125000000000000000, 0.3750000000000000000, 0.4375000000000000000, 0.5000000000000000000, 0.5625000000000000000, 0.6250000000000000000, 0.6875000000000000000, 0.7500000000000000000, 0.8125000000000000000, 0.8750000000000000000, 0.9375000000000000000, 1.000000000000000000 ),
 ( 0.000000000000000000, 1.000000000000000000 ),
 .UNSPECIFIED. ) ;
#66180=B_SPLINE_CURVE_WITH_KNOTS ( 'NONE', 3,
 ( #61844, #47644, #8659, #15745 ),
 .UNSPECIFIED., .F., .F.,
 ( 4, 4 ),
 ( 0.01054893006521931756, 0.01602403026634139499 ),
 .UNSPECIFIED. ) ;
#66182=CARTESIAN_POINT ( 'NONE',  ( 174.9101025265537999, 290.5686053034625047, 2.562613730387248712 ) ) ;
#66183=CARTESIAN_POINT ( 'NONE',  ( 192.8325075361489382, 296.6512949269187516, 11.74553025762331515 ) ) ;
#66186=CARTESIAN_POINT ( 'NONE',  ( 12.40843950188935629, 165.7202760586659736, -5.415160957724236172E-17 ) ) ;
#66187=CARTESIAN_POINT ( 'NONE',  ( 98.36111373172988692, 227.5958772461660260, -9.188101187500095079 ) ) ;
#66188=CARTESIAN_POINT ( 'NONE',  ( 203.5555343017997529, 278.0784677578903370, -15.71723084798551362 ) ) ;
#66189=CARTESIAN_POINT ( 'NONE',  ( 38.12724268070488876, 199.4865022471903160, -10.00000000000009592 ) ) ;
#66190=CARTESIAN_POINT ( 'NONE',  ( 186.7244937263979523, 295.9831862837335734, -7.509257591937855913 ) ) ;
#66192=CARTESIAN_POINT ( 'NONE',  ( 195.2221546850906009, 283.6286238037334897, 17.82163192674956420 ) ) ;
#66193=CARTESIAN_POINT ( 'NONE',  ( 150.8555837531579868, 276.0290483310748755, -8.437460036063264113 ) ) ;
#66194=FACE_OUTER_BOUND ( 'NONE', #61267, .T. ) ;
#66196=B_SPLINE_CURVE_WITH_KNOTS ( 'NONE', 3,
 ( #55123, #32834, #70335, #23723, #17651, #87115, #93681, #2460, #47532, #48033, #17135, #78460, #18150, #9044, #78975, #9562, #40425, #71358 ),
 .UNSPECIFIED., .F., .F.,
 ( 4, 2, 2, 2, 2, 2, 2, 2, 4 ),
 ( 0.000000000000000000, 0.0003132019396418706447, 0.0006264038792837412894, 0.0009396058189256119341, 0.001252807758567482579, 0.001566009698209353332, 0.001879211637851223868, 0.002192413577493094404, 0.002505615517134965158 ),
 .UNSPECIFIED. ) ;
#66199=CARTESIAN_POINT ( 'NONE',  ( 207.3589495855971450, 271.0586446502292119, 2.456771036675355457 ) ) ;
#66200=CARTESIAN_POINT ( 'NONE',  ( 138.7926119064592569, 262.4860189848785694, -2.679491924311252493 ) ) ;
#66203=EDGE_CURVE ( 'NONE', #73362, #60492, #23597, .T. ) ;
#66206=CARTESIAN_POINT ( 'NONE',  ( 72.19064823929512897, 221.6744531367911293, 4.594050593750047540 ) ) ;
#66207=CARTESIAN_POINT ( 'NONE',  ( 207.2707369601997982, 271.6435479931266173, -5.381413637561199614 ) ) ;
#66208=DIRECTION ( 'NONE',  ( 0.4999999999999992784, -0.8660254037844390407, 0.000000000000000000 ) ) ;
#66211=CARTESIAN_POINT ( 'NONE',  ( 196.0395593785976018, 291.0965181932902510, 15.97855489120023087 ) ) ;
#66217=CARTESIAN_POINT ( 'NONE',  ( 135.6272693901030379, 239.1115022471902023, -5.000000000000041744 ) ) ;
#66218=ORIENTED_EDGE ( 'NONE', *, *, #90808, .F. ) ;
#66220=VECTOR ( 'NONE', #67163, 1000.000000000000000 ) ;
#66223=CARTESIAN_POINT ( 'NONE',  ( 191.4139643784075702, 288.5963964191323612, -15.97086743186968150 ) ) ;
#66224=ORIENTED_EDGE ( 'NONE', *, *, #56597, .F. ) ;
#66226=CARTESIAN_POINT ( 'NONE',  ( 153.7445562035061073, 266.9407863685345319, 16.39162974861245559 ) ) ;
#66227=LINE ( 'NONE', #26727, #38740 ) ;
#66229=CARTESIAN_POINT ( 'NONE',  ( 137.7201641159153098, 256.9865022471903444, 10.00000000000009237 ) ) ;
#66232=ORIENTED_EDGE ( 'NONE', *, *, #53447, .F. ) ;
#66234=ORIENTED_EDGE ( 'NONE', *, *, #427, .T. ) ;
#66241=DIRECTION ( 'NONE',  ( -0.8660254037844387076, -0.4999999999999998890, -0.000000000000000000 ) ) ;
#66242=CARTESIAN_POINT ( 'NONE',  ( 194.1641048280396262, 280.7869678786154282, -17.47222775142457962 ) ) ;
#66244=CARTESIAN_POINT ( 'NONE',  ( 201.1060504099706350, 282.3210983108598384, -18.18000168485860257 ) ) ;
#66246=CYLINDRICAL_SURFACE ( 'NONE', #25168, 17.82106496071139645 ) ;
#66249=CARTESIAN_POINT ( 'NONE',  ( 166.9861783932322226, 275.8614021614311014, 14.86566658955477216 ) ) ;
#66250=CARTESIAN_POINT ( 'NONE',  ( 189.9696409261737529, 300.5309180763717904, 0.2178362128448007862 ) ) ;
#66252=ORIENTED_EDGE ( 'NONE', *, *, #81130, .F. ) ;
#66253=CARTESIAN_POINT ( 'NONE',  ( 182.6529124911135114, 296.5506374232393227, 0.2862361614567174861 ) ) ;
#66256=CARTESIAN_POINT ( 'NONE',  ( 194.2389208611690492, 294.2153155915419802, -15.75132567904764791 ) ) ;
#66259=CARTESIAN_POINT ( 'NONE',  ( 131.1347626044233152, 236.5177522451417929, 5.000000000000051514 ) ) ;
#66260=CARTESIAN_POINT ( 'NONE',  ( 205.1793861064249711, 275.2658739283173759, -14.08953480709093675 ) ) ;
#66261=CARTESIAN_POINT ( 'NONE',  ( 183.4954143574004206, 273.2329798171908237, -17.56828100048216257 ) ) ;
#66265=CARTESIAN_POINT ( 'NONE',  ( 94.46399941469991290, 225.3458772461660544, 9.188101187500095079 ) ) ;
#66266=VERTEX_POINT ( 'NONE', #100138 ) ;
#66268=CARTESIAN_POINT ( 'NONE',  ( 166.8004966849435959, 278.2115916653574459, -13.35053495303439952 ) ) ;
#66269=ADVANCED_FACE ( 'NONE', ( #62094 ), #40294, .T. ) ;
#66273=FACE_OUTER_BOUND ( 'NONE', #25904, .T. ) ;
#66274=CARTESIAN_POINT ( 'NONE',  ( 157.8092552871339365, 257.3133472685137235, 17.04082256169242626 ) ) ;
#66275=CARTESIAN_POINT ( 'NONE',  ( 206.4484807199597753, 273.0677375780628608, -9.220527398138528952 ) ) ;
#66276=CARTESIAN_POINT ( 'NONE',  ( 163.1394982460384995, 248.0810956470044175, 11.48951572717839298 ) ) ;
#66281=ORIENTED_EDGE ( 'NONE', *, *, #96234, .T. ) ;
#66282=ADVANCED_FACE ( 'NONE', ( #24610 ), #94444, .F. ) ;
#66284=CARTESIAN_POINT ( 'NONE',  ( 194.6771686668232917, 266.3497618079242670, -7.776454509335324339 ) ) ;
#66285=CARTESIAN_POINT ( 'NONE',  ( 153.3729367728608679, 265.3919680633787834, 16.19611827385041281 ) ) ;
#66287=CARTESIAN_POINT ( 'NONE',  ( 125.9924764494033980, 252.7369531367911293, -4.594050593750048428 ) ) ;
#66292=CARTESIAN_POINT ( 'NONE',  ( 204.2956748066270620, 276.7965067987898919, 13.85972809245231119 ) ) ;
#66296=CARTESIAN_POINT ( 'NONE',  ( 178.5955509887552353, 285.1658660899858546, 13.49892897318265561 ) ) ;
#66303=CARTESIAN_POINT ( 'NONE',  ( 191.9281725887558991, 273.9750938816710004, -16.55071879691933390 ) ) ;
#66304=CARTESIAN_POINT ( 'NONE',  ( -6.813555604197667037, 155.3262482093457777, -6.972266317189433020E-16 ) ) ;
#66305=CARTESIAN_POINT ( 'NONE',  ( 162.7007457333762090, 248.8410372908842021, -10.94671474643812914 ) ) ;
#66310=CARTESIAN_POINT ( 'NONE',  ( 175.8027662909930484, 284.8719843250962072, 14.11304877541382119 ) ) ;
#66314=FACE_OUTER_BOUND ( 'NONE', #42727, .T. ) ;
#66316=CARTESIAN_POINT ( 'NONE',  ( 5.696048431029936410, 186.3464784336661637, 1.353441290958777327E-15 ) ) ;
#66320=EDGE_CURVE ( 'NONE', #19447, #26502, #58267, .T. ) ;
#66324=CARTESIAN_POINT ( 'NONE',  ( 39.63359248971512727, 199.8149278399161233, 9.188101187500093303 ) ) ;
#66326=CARTESIAN_POINT ( 'NONE',  ( 170.5993847053230468, 287.8722104901659691, 7.679145147933459370 ) ) ;
#66327=CARTESIAN_POINT ( 'NONE',  ( 190.5541309856500050, 300.5975588711562523, -4.167177996129430184 ) ) ;
#66329=CARTESIAN_POINT ( 'NONE',  ( 170.8463542321686077, 287.4393069310528972, -8.645854640182026429 ) ) ;
#66330=CARTESIAN_POINT ( 'NONE',  ( 191.0862225170008628, 299.6759493045793192, -9.402218231374108726 ) ) ;
#66331=CARTESIAN_POINT ( 'NONE',  ( 180.0904441998713992, 279.0932581032296298, -17.39800262650857832 ) ) ;
#66334=CARTESIAN_POINT ( 'NONE',  ( 183.8210692855788864, 257.9504670327482927, 6.873620218444065344 ) ) ;
#66335=CARTESIAN_POINT ( 'NONE',  ( 94.56323149399085537, 218.7365022471902023, 10.00000000000009592 ) ) ;
#66337=CARTESIAN_POINT ( 'NONE',  ( 161.5955478064990416, 267.7463613786376868, -17.24529233156741981 ) ) ;
#66339=CARTESIAN_POINT ( 'NONE',  ( 66.64328041388984047, 197.0327760586659736, 1.948934522072303157E-15 ) ) ;
#66341=CARTESIAN_POINT ( 'NONE',  ( 162.5527276353931825, 263.2273425849169257, 17.54043303782436425 ) ) ;
#66342=CARTESIAN_POINT ( 'NONE',  ( 186.8003541658358984, 299.2222177555264011, -0.6103433986344138917 ) ) ;
#66344=ORIENTED_EDGE ( 'NONE', *, *, #30523, .T. ) ;
#66346=CARTESIAN_POINT ( 'NONE',  ( 164.3774690880109119, 245.9368672504194819, -2.805681983503304000 ) ) ;
#66349=CARTESIAN_POINT ( 'NONE',  ( 189.0372613391137975, 265.5483559667888471, 10.71995464741518767 ) ) ;
#66353=B_SPLINE_CURVE_WITH_KNOTS ( 'NONE', 3,
 ( #67114, #60002, #12442, #50420, #21048, #82870, #74752, #20044, #13443, #50915 ),
 .UNSPECIFIED., .F., .F.,
 ( 4, 2, 2, 2, 4 ),
 ( 1.148183921853115802E-16, 0.0004091266720098301062, 0.0008182533440195453953, 0.001227380016029260956, 0.001636506688038975432 ),
 .UNSPECIFIED. ) ;
#66360=CARTESIAN_POINT ( 'NONE',  ( 190.8623743139412454, 300.0636657654615647, 8.577953960666059530 ) ) ;
#66363=AXIS2_PLACEMENT_3D ( 'NONE', #59413, #5735, #44713 ) ;
#66364=ORIENTED_EDGE ( 'NONE', *, *, #93065, .T. ) ;
#66365=CARTESIAN_POINT ( 'NONE',  ( 207.1572261440131797, 271.8401544939704877, -5.633070628900782140 ) ) ;
#66367=CARTESIAN_POINT ( 'NONE',  ( 196.4783028304046013, 290.3365922432724346, -16.37291435488387492 ) ) ;
#66368=ORIENTED_EDGE ( 'NONE', *, *, #58382, .T. ) ;
#66370=CARTESIAN_POINT ( 'NONE',  ( 198.1300353965528984, 287.4757075181870505, 18.48278456664528946 ) ) ;
#66373=CARTESIAN_POINT ( 'NONE',  ( 117.3868696429430258, 229.3923013555409796, 4.594050593750050204 ) ) ;
#66374=CARTESIAN_POINT ( 'NONE',  ( 117.4407359106297406, 238.6115022471902307, 10.00000000000009592 ) ) ;
#66375=CARTESIAN_POINT ( 'NONE',  ( 206.3023480738090996, 271.3208467458289874, 7.632938913807082670 ) ) ;
#66376=CARTESIAN_POINT ( 'NONE',  ( 117.7780771369770463, 227.2592609112379876, 2.679491924311254714 ) ) ;
#66379=CARTESIAN_POINT ( 'NONE',  ( 164.4414259850711915, 245.8260906552167171, -6.983224448873608381 ) ) ;
#66380=ORIENTED_EDGE ( 'NONE', *, *, #44800, .T. ) ;
#66382=CARTESIAN_POINT ( 'NONE',  ( 198.6562788533279615, 286.5642271139020636, 17.47134757795404525 ) ) ;
#66384=CARTESIAN_POINT ( 'NONE',  ( 66.56148311469628709, 218.4244531367911293, -4.594050593750046652 ) ) ;
#66386=CYLINDRICAL_SURFACE ( 'NONE', #46551, 10.00000000000010658 ) ;
#66388=CARTESIAN_POINT ( 'NONE',  ( 198.0542955016221924, 287.6068928643675804, 18.26164672886581997 ) ) ;
#66389=CARTESIAN_POINT ( 'NONE',  ( -18.11259370987442452, 171.8967562850347690, 9.296355089585912665E-16 ) ) ;
#66391=CARTESIAN_POINT ( 'NONE',  ( 112.9278751967105450, 247.5530062829863311, -4.648177544792955347E-16 ) ) ;
#66392=DIRECTION ( 'NONE',  ( -0.8660254037844387076, -0.4999999999999998890, -0.000000000000000000 ) ) ;
#66393=ORIENTED_EDGE ( 'NONE', *, *, #53103, .F. ) ;
#66398=CARTESIAN_POINT ( 'NONE',  ( 206.4767272400630134, 270.6244814104205716, 2.441409265890493785 ) ) ;
#66399=CARTESIAN_POINT ( 'NONE',  ( 180.1168005803277481, 295.2192856762299016, -2.191971455912026467 ) ) ;
#66400=FACE_OUTER_BOUND ( 'NONE', #82188, .T. ) ;
#66401=CARTESIAN_POINT ( 'NONE',  ( 206.5479446040613141, 272.8954610772809133, 10.74757481123993230 ) ) ;
#66402=CARTESIAN_POINT ( 'NONE',  ( 153.2593913506692616, 267.1939427739956727, -16.45456985337825984 ) ) ;
#66405=CARTESIAN_POINT ( 'NONE',  ( 127.1025053677084742, 238.0643266524160424, -9.188101187500093303 ) ) ;
#66406=ORIENTED_EDGE ( 'NONE', *, *, #91951, .F. ) ;
#66408=B_SPLINE_CURVE_WITH_KNOTS ( 'NONE', 3,
 ( #60866, #46682, #93836, #62878 ),
 .UNSPECIFIED., .F., .F.,
 ( 4, 4 ),
 ( 0.002563918088655046078, 0.005315235947567602259 ),
 .UNSPECIFIED. ) ;
#66409=CARTESIAN_POINT ( 'NONE',  ( 184.0019883067494675, 259.5089881467251303, 6.346366111470802096 ) ) ;
#66410=CARTESIAN_POINT ( 'NONE',  ( 205.3095662483215733, 273.2405008374320801, -10.93512342935413884 ) ) ;
#66414=CARTESIAN_POINT ( 'NONE',  ( -22.42236680055709641, 157.8615022471902591, 0.000000000000000000 ) ) ;
#66417=CARTESIAN_POINT ( 'NONE',  ( 182.3798495899531247, 275.9165375621991529, -16.43942715639238017 ) ) ;
#66421=FACE_OUTER_BOUND ( 'NONE', #91542, .T. ) ;
#66423=CARTESIAN_POINT ( 'NONE',  ( 204.6075833744878878, 276.2562653119390461, -13.34672481898815910 ) ) ;
#66424=CARTESIAN_POINT ( 'NONE',  ( 170.8556692713231655, 250.1274861400973464, 4.270813221915627622 ) ) ;
#66428=CARTESIAN_POINT ( 'NONE',  ( 149.5593209768671841, 271.6026526530012575, 11.55487339793564949 ) ) ;
#66430=CARTESIAN_POINT ( 'NONE',  ( 172.1473514959812690, 287.0828204173988638, -8.113061055153803380 ) ) ;
#66431=CARTESIAN_POINT ( 'NONE',  ( 159.2303255284352304, 254.8519814094557603, 16.39103317446447150 ) ) ;
#66433=CARTESIAN_POINT ( 'NONE',  ( 188.7055302822745944, 298.7144859465759623, -6.936194914715221316 ) ) ;
#66434=ADVANCED_FACE ( 'NONE', ( #44785 ), #99020, .T. ) ;
#66435=CARTESIAN_POINT ( 'NONE',  ( 139.3620039403755015, 241.2677522451417929, -5.000000000000041744 ) ) ;
#66440=CARTESIAN_POINT ( 'NONE',  ( 151.3898985249405200, 268.4319993325432847, -14.65018536945715510 ) ) ;
#66441=CARTESIAN_POINT ( 'NONE',  ( -3.911334118262431936, 177.7369531367911293, -4.594050593750048428 ) ) ;
#66442=CARTESIAN_POINT ( 'NONE',  ( 62.15060008387555257, 200.5643266524159856, -9.188101187500093303 ) ) ;
#66443=CARTESIAN_POINT ( 'NONE',  ( 176.1391974210675357, 257.4512529022192666, -10.49415748218208932 ) ) ;
#66445=CARTESIAN_POINT ( 'NONE',  ( 204.6235849755581455, 276.2285497258825444, -13.59355699282649432 ) ) ;
#66449=CARTESIAN_POINT ( 'NONE',  ( 171.0430343787876382, 258.3364600833120903, 13.98411771018495386 ) ) ;
#66450=EDGE_CURVE ( 'NONE', #75103, #17277, #8302, .T. ) ;
#66451=CARTESIAN_POINT ( 'NONE',  ( 179.3339753375761347, 254.6678550771822529, -4.099179283769126769 ) ) ;
#66452=CARTESIAN_POINT ( 'NONE',  ( 150.3470217762446737, 270.2383148473169854, 15.04338213197856078 ) ) ;
#66453=( BOUNDED_CURVE ( )  B_SPLINE_CURVE ( 2, ( #14244, #45130, #99356, #75061, #22336, #53235, #14735, #45618, #9658 ),
 .UNSPECIFIED., .F., .T. ) 
 B_SPLINE_CURVE_WITH_KNOTS ( ( 3, 2, 2, 2, 3 ),
 ( 0.8750000000000000000, 0.8763440860215053752, 0.8790322580645161255, 0.8817204301075268758, 0.8830645161290322509 ),
 .UNSPECIFIED. ) 
 CURVE ( )  GEOMETRIC_REPRESENTATION_ITEM ( )  RATIONAL_B_SPLINE_CURVE ( ( 0.9330127018922194093, 0.9330127018922194093, 1.000000000000000000, 0.8660254037844387076, 1.000000000000000000, 0.8660254037844387076, 1.000000000000000000, 0.9330127018922194093, 0.9330127018922194093 ) ) 
 REPRESENTATION_ITEM ( '' )  );
#66454=CARTESIAN_POINT ( 'NONE',  ( 43.46773267070898328, 189.2365022471902023, -10.00000000000009059 ) ) ;
#66455=CARTESIAN_POINT ( 'NONE',  ( 184.3432414080211288, 293.3642184156927897, 9.509896531551312648 ) ) ;
#66456=CARTESIAN_POINT ( 'NONE',  ( 189.8123550829396891, 301.8823524224806647, -0.5679054518196169354 ) ) ;
#66457=CARTESIAN_POINT ( 'NONE',  ( -0.5279885150232012103, 164.3768266524160140, -9.188101187500091527 ) ) ;
#66461=CARTESIAN_POINT ( 'NONE',  ( 164.9171241593586217, 245.0021572482830550, 1.622680932994367220 ) ) ;
#66462=CARTESIAN_POINT ( 'NONE',  ( 164.3274319858398087, 246.0235340536434592, -1.770631424362269168 ) ) ;
#66463=FACE_OUTER_BOUND ( 'NONE', #12077, .T. ) ;
#66464=CARTESIAN_POINT ( 'NONE',  ( 153.3038478579095170, 266.0895745828713075, -16.28333902283113588 ) ) ;
#66465=CARTESIAN_POINT ( 'NONE',  ( 176.5163929983920355, 260.4762631834057061, -13.32580715195663146 ) ) ;
#66468=CARTESIAN_POINT ( 'NONE',  ( 165.6535135722015184, 285.4045712548459051, 0.4591178296265144287 ) ) ;
#66471=CARTESIAN_POINT ( 'NONE',  ( -27.42236680055714260, 166.5217562850347406, 1.224646799147364892E-15 ) ) ;
#66473=CARTESIAN_POINT ( 'NONE',  ( 156.8792359301817214, 276.4852139478325626, 11.15229350607063274 ) ) ;
#66476=CARTESIAN_POINT ( 'NONE',  ( 192.8325075361489382, 296.6512949269187516, 11.74553025762331515 ) ) ;
#66477=CARTESIAN_POINT ( 'NONE',  ( 72.76825883208245216, 219.4865022471902876, 10.00000000000009415 ) ) ;
#66479=CARTESIAN_POINT ( 'NONE',  ( 154.9067123643522734, 262.3406990819208886, -18.18534662427576265 ) ) ;
#66480=ORIENTED_EDGE ( 'NONE', *, *, #51836, .F. ) ;
#66481=VERTEX_POINT ( 'NONE', #39167 ) ;
#66482=CARTESIAN_POINT ( 'NONE',  ( 164.2858849336956268, 246.6305630168277503, -4.528670904437447575 ) ) ;
#66483=DIRECTION ( 'NONE',  ( -0.8660254037844387076, -0.4999999999999998890, -0.000000000000000000 ) ) ;
#66484=CARTESIAN_POINT ( 'NONE',  ( 192.4454213697443095, 297.3217478340386606, 12.58566886711101596 ) ) ;
#66491=CARTESIAN_POINT ( 'NONE',  ( 85.37179553587198200, 208.5494855054051584, -2.679491924311248496 ) ) ;
#66492=CARTESIAN_POINT ( 'NONE',  ( 149.7109319212262051, 271.3400547943878109, -12.38605961032017433 ) ) ;
#66496=CARTESIAN_POINT ( 'NONE',  ( 159.9381800915330416, 254.2419649056765820, -15.29477132317076915 ) ) ;
#66497=CARTESIAN_POINT ( 'NONE',  ( 206.5280879940269756, 272.9298537347264642, 11.21709153681466731 ) ) ;
#66500=CARTESIAN_POINT ( 'NONE',  ( 149.0323968763055689, 272.5153119669064949, 11.64231532207353403 ) ) ;
#66501=CARTESIAN_POINT ( 'NONE',  ( 171.8887382467565317, 263.4056550183183276, -15.47577216865978400 ) ) ;
#66503=ORIENTED_EDGE ( 'NONE', *, *, #20226, .F. ) ;
#66508=CARTESIAN_POINT ( 'NONE',  ( 156.6663764169331898, 266.5808990040749222, -16.21966367912098050 ) ) ;
#66512=CARTESIAN_POINT ( 'NONE',  ( 132.6918519524023736, 258.9637435831425023, 2.679491924311251605 ) ) ;
#66513=CARTESIAN_POINT ( 'NONE',  ( 157.2021838295288489, 258.7528274272191311, -16.83974058492033166 ) ) ;
#66515=CARTESIAN_POINT ( 'NONE',  ( 178.4260950018880294, 291.5365620954837027, 6.089707329432893168 ) ) ;
#66516=CARTESIAN_POINT ( 'NONE',  ( 158.5494479970505779, 256.0312958875455820, -16.13101935219385297 ) ) ;
#66519=CARTESIAN_POINT ( 'NONE',  ( 206.5508451493652444, 272.8904371854448527, 11.05407534521577695 ) ) ;
#66520=CARTESIAN_POINT ( 'NONE',  ( 205.8030308266901898, 274.1856895869457844, 10.55961490432110317 ) ) ;
#66522=ORIENTED_EDGE ( 'NONE', *, *, #57294, .T. ) ;
#66523=CARTESIAN_POINT ( 'NONE',  ( 192.6316891401646387, 296.9991225918579403, 12.51992576083217301 ) ) ;
#66526=CARTESIAN_POINT ( 'NONE',  ( 147.2752695334602322, 275.5587458000830452, -2.690728879113632566 ) ) ;
#66528=FACE_OUTER_BOUND ( 'NONE', #42317, .T. ) ;
#66531=EDGE_CURVE ( 'NONE', #74702, #1108, #318, .T. ) ;
#66532=CARTESIAN_POINT ( 'NONE',  ( 159.8699404666255930, 253.7441358392297843, -15.37844326134346673 ) ) ;
#66533=CARTESIAN_POINT ( 'NONE',  ( 190.6082082143898617, 300.5038943634461361, -0.5472910358126498176 ) ) ;
#66535=CARTESIAN_POINT ( 'NONE',  ( 163.3723087697842971, 247.6778559913402091, -10.08585062664141319 ) ) ;
#66536=CARTESIAN_POINT ( 'NONE',  ( 190.9103068040902258, 266.1559691903721045, 12.32197154148064655 ) ) ;
#66538=CARTESIAN_POINT ( 'NONE',  ( -22.42236680055709641, 157.8615022471902591, 0.000000000000000000 ) ) ;
#66539=CARTESIAN_POINT ( 'NONE',  ( 23.67544375150414737, 191.1427522451419634, -10.00000000000009415 ) ) ;
#66540=CARTESIAN_POINT ( 'NONE',  ( 101.5001087246834857, 241.6589784336661637, -6.496448406907676862E-16 ) ) ;
#66541=CARTESIAN_POINT ( 'NONE',  ( 181.2763874864546949, 294.3971386994905401, -2.647043256306043979 ) ) ;
#66542=CARTESIAN_POINT ( 'NONE',  ( 162.8931802014337791, 249.0911889412991229, -10.32038157250286048 ) ) ;
#66543=CARTESIAN_POINT ( 'NONE',  ( 157.0935036675524827, 258.5530654392286465, 17.32636058289560665 ) ) ;
#66545=CARTESIAN_POINT ( 'NONE',  ( 40.66251830035667325, 182.0327760586659451, 1.948934522072303157E-15 ) ) ;
#66548=CARTESIAN_POINT ( 'NONE',  ( 191.3401838285315080, 298.8338641635404542, 7.654257991345104095 ) ) ;
#66550=EDGE_CURVE ( 'NONE', #3978, #55003, #50768, .T. ) ;
#66551=CARTESIAN_POINT ( 'NONE',  ( 119.5854454918513170, 251.3967562850347122, -4.648177544792955347E-16 ) ) ;
#66552=CARTESIAN_POINT ( 'NONE',  ( 190.1752790837055045, 301.2537496138681945, -5.177773110520776711 ) ) ;
#66555=CARTESIAN_POINT ( 'NONE',  ( 68.53065452504849020, 198.8262482093457777, 3.021315404115420679E-15 ) ) ;
#66556=CARTESIAN_POINT ( 'NONE',  ( 102.9889369814290347, 230.2677522451418497, 10.00000000000009592 ) ) ;
#66558=CARTESIAN_POINT ( 'NONE',  ( 48.37494963522306080, 207.9244531367911293, -4.594050593750046652 ) ) ;
#66559=CARTESIAN_POINT ( 'NONE',  ( 90.43156862655462191, 233.0177522451419350, 5.000000000000046185 ) ) ;
#66560=VERTEX_POINT ( 'NONE', #86859 ) ;
#66561=CARTESIAN_POINT ( 'NONE',  ( 194.7965532219227498, 266.2737535417827530, -7.589310887033829722 ) ) ;
#66563=CARTESIAN_POINT ( 'NONE',  ( 178.8342571948529951, 258.9790443764770203, -10.10065873795960023 ) ) ;
#66564=CARTESIAN_POINT ( 'NONE',  ( 207.6050568035884680, 271.0644890383991310, -1.456818755242089702 ) ) ;
#66565=CARTESIAN_POINT ( 'NONE',  ( 10.51348828746337638, 183.0024278399160949, -9.188101187500093303 ) ) ;
#66566=EDGE_CURVE ( 'NONE', #33367, #8285, #99368, .T. ) ;
#66567=CARTESIAN_POINT ( 'NONE',  ( 199.2205425252482200, 285.5868937652708155, -18.05012564782189344 ) ) ;
#66570=CARTESIAN_POINT ( 'NONE',  ( 42.06911538997637479, 207.3464784336661353, 1.353441290958777327E-15 ) ) ;
#66571=CARTESIAN_POINT ( 'NONE',  ( 164.4698008747318738, 245.7769439046653019, -6.272955660526681854 ) ) ;
#66574=CARTESIAN_POINT ( 'NONE',  ( 207.6826438088389750, 270.9301044032979462, 7.252082088659585146 ) ) ;
#66575=B_SPLINE_CURVE_WITH_KNOTS ( 'NONE', 3,
 ( #19622, #50480, #3419, #73796, #18607, #66192, #97137, #2923, #66681, #57078 ),
 .UNSPECIFIED., .F., .F.,
 ( 4, 3, 3, 4 ),
 ( 5.849685106239000612E-15, 0.001498044977023057535, 0.004494154408229840761, 0.004642971226047358860 ),
 .UNSPECIFIED. ) ;
#66578=CARTESIAN_POINT ( 'NONE',  ( 4.496589500409242213, 166.7365022471902023, -10.00000000000009059 ) ) ;
#66580=CARTESIAN_POINT ( 'NONE',  ( 131.9199452241419124, 234.7202760586659736, -5.415160957724236172E-17 ) ) ;
#66582=B_SPLINE_CURVE_WITH_KNOTS ( 'NONE', 3,
 ( #5670, #77054, #7662, #69459 ),
 .UNSPECIFIED., .F., .F.,
 ( 4, 4 ),
 ( 0.002667466630201718782, 0.003029344800501278766 ),
 .UNSPECIFIED. ) ;
#66583=CARTESIAN_POINT ( 'NONE',  ( 165.0842110975921742, 244.7127541819816372, 1.670879517523061075 ) ) ;
#66587=CARTESIAN_POINT ( 'NONE',  ( 189.5521783559119342, 289.6378612515180748, 14.85317001376669843 ) ) ;
#66588=CARTESIAN_POINT ( 'NONE',  ( 150.3767742445782289, 270.1867820605125416, -15.10420222983148442 ) ) ;
#66590=CARTESIAN_POINT ( 'NONE',  ( 190.8094645593471341, 300.1553081486349015, 8.399847186519689757 ) ) ;
#66591=CARTESIAN_POINT ( 'NONE',  ( 164.1233341003454314, 246.3770419610369800, 7.970621798363497490 ) ) ;
#66592=CARTESIAN_POINT ( 'NONE',  ( 190.9904595088351584, 263.1162866600020038, -8.709768327411630651 ) ) ;
#66593=CARTESIAN_POINT ( 'NONE',  ( 169.5763875261042415, 266.0051543528422826, -17.23840913299506283 ) ) ;
#66595=ORIENTED_EDGE ( 'NONE', *, *, #6025, .F. ) ;
#66597=CARTESIAN_POINT ( 'NONE',  ( 171.2449227966682770, 284.2896847597517649, -11.26649335755497283 ) ) ;
#66599=CARTESIAN_POINT ( 'NONE',  ( 196.1582417222007848, 271.0076856177163904, 12.85313896011626333 ) ) ;
#66600=CARTESIAN_POINT ( 'NONE',  ( 182.1059484044376688, 295.6613757171786574, 4.943108598893879879 ) ) ;
#66603=CARTESIAN_POINT ( 'NONE',  ( 192.7251185966330240, 281.9663580653335089, 16.81651591906913978 ) ) ;
#66605=CARTESIAN_POINT ( 'NONE',  ( 94.76169564547690527, 215.5177522451417929, 5.000000000000051514 ) ) ;
#66606=ORIENTED_EDGE ( 'NONE', *, *, #62159, .F. ) ;
#66607=CARTESIAN_POINT ( 'NONE',  ( 169.5007657120409874, 248.2156828994837099, -1.963647642838588503 ) ) ;
#66608=DIRECTION ( 'NONE',  ( -0.8660254037844387076, -0.4999999999999998890, -0.000000000000000000 ) ) ;
#66609=CARTESIAN_POINT ( 'NONE',  ( 156.2535903939119635, 261.5009266245895674, -17.19818558915508433 ) ) ;
#66611=CARTESIAN_POINT ( 'NONE',  ( 147.2592533090473239, 275.5864867145116932, -0.3770461397900867762 ) ) ;
#66612=CARTESIAN_POINT ( 'NONE',  ( 205.0815341406070615, 273.1773411830968712, -9.768730833708779926 ) ) ;
#66613=CARTESIAN_POINT ( 'NONE',  ( 164.4990934228277411, 245.7262077230798809, 6.470820838822735510 ) ) ;
#66614=CARTESIAN_POINT ( 'NONE',  ( 189.5534384022301424, 269.0062095459838929, -14.92796778812864922 ) ) ;
#66616=CARTESIAN_POINT ( 'NONE',  ( 78.92949518643405327, 222.5024278399160949, 9.188101187500095079 ) ) ;
#66617=CARTESIAN_POINT ( 'NONE',  ( 155.5793834749241853, 261.1755985416265275, 17.09727664165891525 ) ) ;
#66619=CARTESIAN_POINT ( 'NONE',  ( 185.0654652685402368, 260.0011547607978741, -6.087314472554996136 ) ) ;
#66621=ORIENTED_EDGE ( 'NONE', *, *, #4795, .F. ) ;
#66623=B_SPLINE_CURVE_WITH_KNOTS ( 'NONE', 3,
 ( #86735, #48689, #25372, #2088 ),
 .UNSPECIFIED., .F., .F.,
 ( 4, 4 ),
 ( 0.005006823703232672271, 0.01302678491365392814 ),
 .UNSPECIFIED. ) ;
#66625=CARTESIAN_POINT ( 'NONE',  ( 192.7503840695331121, 293.9944895470539450, 14.24544604289089555 ) ) ;
#66627=CARTESIAN_POINT ( 'NONE',  ( 159.6023402823087451, 258.6676503891110883, 17.43025742997651761 ) ) ;
#66628=CARTESIAN_POINT ( 'NONE',  ( 155.1865148098964937, 261.8560670301561686, -16.99758927948949605 ) ) ;
#66629=ORIENTED_EDGE ( 'NONE', *, *, #67141, .F. ) ;
#66630=CARTESIAN_POINT ( 'NONE',  ( 207.0720832995076250, 271.9876262265548235, -6.798746899112098951 ) ) ;
#66633=CARTESIAN_POINT ( 'NONE',  ( 147.9500839974939197, 274.3899328626944225, -9.375093207164509224 ) ) ;
#66635=CARTESIAN_POINT ( 'NONE',  ( 157.5377142495414944, 281.7650987280287609, 2.959616700945237433 ) ) ;
#66636=CARTESIAN_POINT ( 'NONE',  ( 168.0409292894617295, 267.0411674002936024, -16.96956704154970907 ) ) ;
#66637=VERTEX_POINT ( 'NONE', #34112 ) ;
#66641=CARTESIAN_POINT ( 'NONE',  ( 167.4774516927647880, 284.1243695549201789, 9.174491941972370057 ) ) ;
#66642=CARTESIAN_POINT ( 'NONE',  ( 203.9281103364544379, 271.7020019549630661, 9.691553030514192812 ) ) ;
#66644=CARTESIAN_POINT ( 'NONE',  ( 3.694774645000036273, 161.3932355074535678, -2.679491924311248496 ) ) ;
#66647=CARTESIAN_POINT ( 'NONE',  ( 161.1791855798394408, 281.3418815567459319, -6.591164736166998495 ) ) ;
#66649=FACE_OUTER_BOUND ( 'NONE', #56762, .T. ) ;
#66650=LINE ( 'NONE', #60520, #85207 ) ;
#66652=CARTESIAN_POINT ( 'NONE',  ( 169.1311965936330353, 247.8770103324328034, 7.134965090537657859E-13 ) ) ;
#66653=CARTESIAN_POINT ( 'NONE',  ( 195.1498658919753098, 292.2566161375916636, 15.21824497126251785 ) ) ;
#66655=CARTESIAN_POINT ( 'NONE',  ( 181.5711328935895494, 270.9591510390133635, -15.96266144669950293 ) ) ;
#66658=CARTESIAN_POINT ( 'NONE',  ( 174.8981841478993147, 281.3293342729474489, -14.17585464771519810 ) ) ;
#66661=CARTESIAN_POINT ( 'NONE',  ( 160.8938801005855908, 272.8507423001361190, 15.74055753482374698 ) ) ;
#66662=CARTESIAN_POINT ( 'NONE',  ( 161.3681471114688293, 281.5053870741572837, -7.339062344004410043 ) ) ;
#66670=CARTESIAN_POINT ( 'NONE',  ( 175.6092358407374547, 290.9609716272898368, 2.612219778893893007 ) ) ;
#66671=CARTESIAN_POINT ( 'NONE',  ( 192.5049767439991513, 297.2185948999652965, 12.57567268027295881 ) ) ;
#66675=CARTESIAN_POINT ( 'NONE',  ( 4.207654042216683266, 182.4244531367911293, -4.594050593750046652 ) ) ;
#66676=CARTESIAN_POINT ( 'NONE',  ( 107.7251869580316281, 226.8768266524160140, 9.188101187500098632 ) ) ;
#66677=CARTESIAN_POINT ( 'NONE',  ( 186.6437685709837524, 295.7868322423274208, -7.682377513881603726 ) ) ;
#66680=AXIS2_PLACEMENT_3D ( 'NONE', #19796, #97794, #28364 ) ;
#66681=CARTESIAN_POINT ( 'NONE',  ( 194.3794555884949773, 282.9248721468028975, 17.82082507299162089 ) ) ;
#66682=CARTESIAN_POINT ( 'NONE',  ( 193.9966098916996771, 294.6350105018939871, 13.97117019253516013 ) ) ;
#66684=CARTESIAN_POINT ( 'NONE',  ( 194.9819925439454664, 292.9282776833073285, -15.33279721168237586 ) ) ;
#66685=ADVANCED_FACE ( 'NONE', ( #29976 ), #1083, .T. ) ;
#66687=CARTESIAN_POINT ( 'NONE',  ( 186.7826593668773398, 299.1805613592297846, -0.6094521799418902708 ) ) ;
#66688=CARTESIAN_POINT ( 'NONE',  ( 165.2952469160895816, 253.4663260364826556, -13.06521362961797550 ) ) ;
#66690=CARTESIAN_POINT ( 'NONE',  ( 174.5980114852178815, 264.9326092916348330, -15.54993198801018472 ) ) ;
#66691=CARTESIAN_POINT ( 'NONE',  ( 91.83912023130210400, 214.6423013555409796, -4.594050593750043987 ) ) ;
#66693=CARTESIAN_POINT ( 'NONE',  ( 163.2261234402530476, 258.2666102061564857, 16.06505531561552758 ) ) ;
#66694=CARTESIAN_POINT ( 'NONE',  ( 195.8248271798537417, 291.4684452715354155, 17.35175160929494709 ) ) ;
#66695=CARTESIAN_POINT ( 'NONE',  ( 200.2341212244148210, 283.8313239608446565, 18.44154502101277870 ) ) ;
#66696=CARTESIAN_POINT ( 'NONE',  ( 197.0938247690820049, 289.2704769723097797, 17.22904708886757774 ) ) ;
#66697=B_SPLINE_CURVE_WITH_KNOTS ( 'NONE', 3,
 ( #63079, #53790, #29036, #90876 ),
 .UNSPECIFIED., .F., .F.,
 ( 4, 4 ),
 ( 0.000000000000000000, 0.002280643322503841074 ),
 .UNSPECIFIED. ) ;
#66698=CARTESIAN_POINT ( 'NONE',  ( 151.4188942279983223, 268.3817773016460251, -14.77302265413830895 ) ) ;
#66701=CARTESIAN_POINT ( 'NONE',  ( 193.1444937042664094, 296.1109190324805240, -12.15243020627156767 ) ) ;
#66703=ORIENTED_EDGE ( 'NONE', *, *, #59917, .T. ) ;
#66706=CARTESIAN_POINT ( 'NONE',  ( 146.9700173529739970, 276.0874580858064746, -5.099093031535578469 ) ) ;
#66707=CARTESIAN_POINT ( 'NONE',  ( 191.2921030740457411, 288.8084469331090531, -16.29029516365350005 ) ) ;
#66711=CARTESIAN_POINT ( 'NONE',  ( 157.7255603307123408, 268.5163524934444013, 16.86592485641857309 ) ) ;
#66712=EDGE_CURVE ( 'NONE', #26873, #12604, #7481, .T. ) ;
#66714=CARTESIAN_POINT ( 'NONE',  ( 181.2305971022323661, 265.9781236237157032, -15.82518789413146010 ) ) ;
#66715=CARTESIAN_POINT ( 'NONE',  ( 129.0599100780709421, 251.9865022471903444, -10.00000000000009415 ) ) ;
#66716=CARTESIAN_POINT ( 'NONE',  ( 204.6475128369918082, 276.1871054541632020, -13.72068618491070779 ) ) ;
#66719=CARTESIAN_POINT ( 'NONE',  ( 165.5467306339926097, 246.9162971582917407, -1.814430410556957529 ) ) ;
#66721=DIRECTION ( 'NONE',  ( -0.8660254037844387076, -0.4999999999999998890, -0.000000000000000000 ) ) ;
#66722=CARTESIAN_POINT ( 'NONE',  ( -22.42236680055709641, 157.8615022471902591, 0.000000000000000000 ) ) ;
#66727=CARTESIAN_POINT ( 'NONE',  ( 189.4721059029944570, 290.0100815663928984, 14.44573074396852519 ) ) ;
#66728=FACE_OUTER_BOUND ( 'NONE', #60099, .T. ) ;
#66730=CARTESIAN_POINT ( 'NONE',  ( 192.9443876183610769, 296.4575129401721370, -13.55710008152484569 ) ) ;
#66731=CARTESIAN_POINT ( 'NONE',  ( 203.3087286698060723, 275.5229930796335793, -14.04662039663043061 ) ) ;
#66734=CARTESIAN_POINT ( 'NONE',  ( 164.1076778612453495, 275.3502986316374859, 15.09133881111785058 ) ) ;
#66735=CARTESIAN_POINT ( 'NONE',  ( 73.61078154397070250, 201.7592609112380160, 2.679491924311254714 ) ) ;
#66744=CARTESIAN_POINT ( 'NONE',  ( 184.6894110187365641, 293.7322318964822330, -10.88359728165448814 ) ) ;
#66745=CARTESIAN_POINT ( 'NONE',  ( 147.6088797830324779, 274.9809158978982850, 8.531536684623960198 ) ) ;
#66747=CARTESIAN_POINT ( 'NONE',  ( 169.7305867463648497, 267.4144629999083804, 17.02687474860264771 ) ) ;
#66749=CARTESIAN_POINT ( 'NONE',  ( 96.79126913948807953, 232.8149278399160949, 9.188101187500093303 ) ) ;
#66750=ORIENTED_EDGE ( 'NONE', *, *, #13656, .T. ) ;
#66751=CARTESIAN_POINT ( 'NONE',  ( 148.1250100625814241, 274.5153593849270237, -6.488543390179210668 ) ) ;
#66752=B_SPLINE_CURVE_WITH_KNOTS ( 'NONE', 3,
 ( #81644, #12214, #89270, #35986 ),
 .UNSPECIFIED., .F., .F.,
 ( 4, 4 ),
 ( 0.004401395493315057861, 0.009384348131726182735 ),
 .UNSPECIFIED. ) ;
#66753=CARTESIAN_POINT ( 'NONE',  ( 165.6972188542663389, 277.5909501293253925, -13.41042508424620294 ) ) ;
#66756=AXIS2_PLACEMENT_3D ( 'NONE', #85326, #92911, #69075 ) ;
#66760=AXIS2_PLACEMENT_3D ( 'NONE', #14877, #30089, #22489 ) ;
#66763=CARTESIAN_POINT ( 'NONE',  ( 196.1613785401733878, 290.8855212161054737, 15.98157687694135021 ) ) ;
#66764=FACE_OUTER_BOUND ( 'NONE', #53029, .T. ) ;
#66767=ORIENTED_EDGE ( 'NONE', *, *, #16299, .T. ) ;
#66772=VERTEX_POINT ( 'NONE', #34473 ) ;
#66773=EDGE_CURVE ( 'NONE', #25119, #65280, #4683, .T. ) ;
#66776=CARTESIAN_POINT ( 'NONE',  ( 102.9889369814290632, 220.2677522451417929, -5.000000000000041744 ) ) ;
#66778=CARTESIAN_POINT ( 'NONE',  ( 135.2486435959970947, 239.7048013555409796, 4.594050593750051981 ) ) ;
#66781=VERTEX_POINT ( 'NONE', #52153 ) ;
#66782=CARTESIAN_POINT ( 'NONE',  ( 157.3880781592554285, 258.0428474529849723, 18.15852591502753555 ) ) ;
#66785=CARTESIAN_POINT ( 'NONE',  ( 172.6858628785228120, 251.2885248701833234, -0.2562763602120753936 ) ) ;
#66786=CARTESIAN_POINT ( 'NONE',  ( 178.4306755334441448, 285.4540973033057298, 14.29586447726307874 ) ) ;
#66788=CARTESIAN_POINT ( 'NONE',  ( 198.9504127373876941, 281.7903563508199909, -16.59127471182994640 ) ) ;
#66792=CARTESIAN_POINT ( 'NONE',  ( 206.7812045875167257, 272.0977345600681474, 6.637818014026708902 ) ) ;
#66793=CARTESIAN_POINT ( 'NONE',  ( 65.88516108981343677, 208.8458772461660544, 9.188101187500095079 ) ) ;
#66794=CARTESIAN_POINT ( 'NONE',  ( 206.4484807199597753, 273.0677375780628608, -9.220527398138528952 ) ) ;
#66796=CARTESIAN_POINT ( 'NONE',  ( 163.4055107321044318, 247.6203485056908846, -10.24153090796238530 ) ) ;
#66804=CARTESIAN_POINT ( 'NONE',  ( 18.30771692152332975, 187.5024278399160949, -9.188101187500093303 ) ) ;
#66808=CARTESIAN_POINT ( 'NONE',  ( 202.4560076411394220, 279.0611292670678267, 15.58065739802832717 ) ) ;
#66811=CARTESIAN_POINT ( 'NONE',  ( 44.82974491242176640, 202.8149278399161233, 9.188101187500093303 ) ) ;
#66812=B_SPLINE_CURVE_WITH_KNOTS ( 'NONE', 3,
 ( #16555, #47449, #63155, #94102 ),
 .UNSPECIFIED., .F., .F.,
 ( 4, 4 ),
 ( 0.02705554120967477993, 0.03627623533732127897 ),
 .UNSPECIFIED. ) ;
#66814=CARTESIAN_POINT ( 'NONE',  ( 200.7523954295751594, 282.9336467052548869, 18.23634913067694185 ) ) ;
#66816=CARTESIAN_POINT ( 'NONE',  ( 190.2287563641723978, 301.1611242470490311, -4.521471513871881953 ) ) ;
#66818=CARTESIAN_POINT ( 'NONE',  ( 175.8346136117470166, 290.9171170946435723, -7.656592247309970567 ) ) ;
#66819=CARTESIAN_POINT ( 'NONE',  ( 178.5384570540184370, 293.1491523154654715, 2.625233457618431299 ) ) ;
#66820=CARTESIAN_POINT ( 'NONE',  ( 177.2719741535860578, 275.4483640892808012, 16.48456767178202043 ) ) ;
#66821=CARTESIAN_POINT ( 'NONE',  ( -22.42236680055709641, 157.8615022471902591, 0.000000000000000000 ) ) ;
#66823=CARTESIAN_POINT ( 'NONE',  ( 167.1132731660547961, 257.9384026749979171, -15.49077391459553432 ) ) ;
#66825=CARTESIAN_POINT ( 'NONE',  ( 188.0737869051473012, 299.5124861214166572, -3.734995909225475863 ) ) ;
#66826=CARTESIAN_POINT ( 'NONE',  ( 95.35708811412658292, 225.8615022471902591, -10.00000000000009592 ) ) ;
#66828=CARTESIAN_POINT ( 'NONE',  ( 165.0276504369421104, 270.2126989760424749, -16.40444607549173384 ) ) ;
#66830=CARTESIAN_POINT ( 'NONE',  ( 62.50250967810423930, 197.7048013555409796, 4.594050593750051981 ) ) ;
#66831=ORIENTED_EDGE ( 'NONE', *, *, #91254, .T. ) ;
#66832=CARTESIAN_POINT ( 'NONE',  ( 164.2588978958649193, 264.2780746704087846, 16.72791175256383411 ) ) ;
#66833=CARTESIAN_POINT ( 'NONE',  ( 190.1635032421960148, 301.2741459696644029, -5.047660290019184259 ) ) ;
#66835=EDGE_LOOP ( 'NONE', ( #27066, #6840, #88602, #89371 ) ) ;
#66837=DIRECTION ( 'NONE',  ( -0.8660254037844387076, -0.4999999999999998890, -0.000000000000000000 ) ) ;
#66841=CARTESIAN_POINT ( 'NONE',  ( 185.7886707784097950, 263.2411039711001877, 11.08596199193305232 ) ) ;
#66843=CARTESIAN_POINT ( 'NONE',  ( 204.6244483240926400, 276.2270543623566255, 13.10813453876796864 ) ) ;
#66844=ORIENTED_EDGE ( 'NONE', *, *, #79545, .T. ) ;
#66848=DIRECTION ( 'NONE',  ( -0.4999999999999987788, 0.8660254037844392627, 0.000000000000000000 ) ) ;
#66852=CARTESIAN_POINT ( 'NONE',  ( 206.5081929095101998, 272.9643130319303737, -9.215516226794479238 ) ) ;
#66854=ORIENTED_EDGE ( 'NONE', *, *, #41114, .F. ) ;
#66855=CARTESIAN_POINT ( 'NONE',  ( 161.8153478334749877, 250.3745914384277285, -14.21120979595050215 ) ) ;
#66856=CARTESIAN_POINT ( 'NONE',  ( 113.8346084569740242, 224.9824982072973967, 3.021315404115420679E-15 ) ) ;
#66860=CARTESIAN_POINT ( 'NONE',  ( 159.5284711081640125, 254.3355781173132755, 15.34104435652608522 ) ) ;
#66862=CARTESIAN_POINT ( 'NONE',  ( 161.0638154310756818, 262.9933345025709173, -17.40812897737963283 ) ) ;
#66863=CARTESIAN_POINT ( 'NONE',  ( 124.6666353716822186, 242.7833772461660544, -9.188101187500095079 ) ) ;
#66864=CARTESIAN_POINT ( 'NONE',  ( 150.6655900823359389, 269.6865383554857090, 15.31288044136207205 ) ) ;
#66865=DIRECTION ( 'NONE',  ( -0.8660254037844387076, -0.4999999999999998890, -0.000000000000000000 ) ) ;
#66866=VERTEX_POINT ( 'NONE', #20283 ) ;
#66867=CARTESIAN_POINT ( 'NONE',  ( 148.6500818154487433, 275.1775010768142238, 7.719411301773694944 ) ) ;
#66870=CARTESIAN_POINT ( 'NONE',  ( 159.7608930362198407, 253.9330115291272421, 15.38895778945778581 ) ) ;
#66871=CARTESIAN_POINT ( 'NONE',  ( 204.7308350088324289, 274.2642561119486686, -12.27241466464917963 ) ) ;
#66872=CARTESIAN_POINT ( 'NONE',  ( 82.06918437091763963, 212.0643266524160140, 9.188101187500095079 ) ) ;
#66873=ORIENTED_EDGE ( 'NONE', *, *, #44800, .F. ) ;
#66876=CARTESIAN_POINT ( 'NONE',  ( 151.0480362197490933, 269.0241222143274626, 14.53796507407317762 ) ) ;
#66877=ADVANCED_FACE ( 'NONE', ( #28360 ), #82626, .T. ) ;
#66878=CARTESIAN_POINT ( 'NONE',  ( 175.8464236115564461, 278.0655253321181704, 16.02019172894276267 ) ) ;
#66882=CARTESIAN_POINT ( 'NONE',  ( 121.1754704609022752, 230.7677522451417929, -5.000000000000041744 ) ) ;
#66883=CARTESIAN_POINT ( 'NONE',  ( 153.4613150239306094, 264.8442007126561748, -16.86932470306368259 ) ) ;
#66884=CARTESIAN_POINT ( 'NONE',  ( 203.5555343017997529, 278.0784677578903370, -15.71723084798551362 ) ) ;
#66886=CARTESIAN_POINT ( 'NONE',  ( 206.8806555995618055, 270.0414039046062271, 3.363062889176088976 ) ) ;
#66888=EDGE_CURVE ( 'NONE', #61729, #62607, #82555, .T. ) ;
#66889=CARTESIAN_POINT ( 'NONE',  ( 165.3552783545318050, 246.2432519206945472, 4.078954813822171843 ) ) ;
#66890=B_SPLINE_CURVE_WITH_KNOTS ( 'NONE', 3,
 ( #97808, #82645, #19806, #68373 ),
 .UNSPECIFIED., .F., .F.,
 ( 4, 4 ),
 ( 0.01738225534458222657, 0.02631611770651103369 ),
 .UNSPECIFIED. ) ;
#66891=CARTESIAN_POINT ( 'NONE',  ( 168.3557124657904467, 273.6222795104500278, 17.14480014634877136 ) ) ;
#66892=CARTESIAN_POINT ( 'NONE',  ( 185.9427433571077586, 257.7868782628476083, -2.501399907045548598 ) ) ;
#66893=CARTESIAN_POINT ( 'NONE',  ( 194.8870616291461886, 279.6787320282184055, 16.91106461190539179 ) ) ;
#66894=ORIENTED_EDGE ( 'NONE', *, *, #12408, .T. ) ;
#66895=CARTESIAN_POINT ( 'NONE',  ( 207.5230514910949182, 271.2065264061283756, 2.678931747975364708 ) ) ;
#66896=CARTESIAN_POINT ( 'NONE',  ( 141.2833242589136375, 258.5024278399160380, 9.188101187500095079 ) ) ;
#66902=LINE ( 'NONE', #44086, #41779 ) ;
#66907=VECTOR ( 'NONE', #90445, 1000.000000000000000 ) ;
#66908=CARTESIAN_POINT ( 'NONE',  ( 167.8403594995746175, 248.8093847173732058, -6.497506089718841693 ) ) ;
#66909=CARTESIAN_POINT ( 'NONE',  ( 164.2904957002474191, 246.0875095769322911, -1.594749884056509748 ) ) ;
#66910=CARTESIAN_POINT ( 'NONE',  ( 180.4572463832561482, 261.7460625851787199, -13.63662180976220384 ) ) ;
#66912=CARTESIAN_POINT ( 'NONE',  ( 183.3251615928574267, 281.0033614153954886, 17.25538570714889985 ) ) ;
#66913=CARTESIAN_POINT ( 'NONE',  ( 157.4893260420801653, 257.8674809757739013, -18.30842125257398223 ) ) ;
#66914=CARTESIAN_POINT ( 'NONE',  ( 196.5331985480450783, 270.3460110500564610, 11.78449596397654808 ) ) ;
#66916=CARTESIAN_POINT ( 'NONE',  ( 190.0896302098338424, 301.4020978150248311, 3.433521196325825642 ) ) ;
#66917=CARTESIAN_POINT ( 'NONE',  ( 204.7847318215661119, 274.1906186268559509, 12.16298107665122252 ) ) ;
#66921=CARTESIAN_POINT ( 'NONE',  ( 137.9907970510501514, 237.1427522451417360, 1.119607411625061291E-15 ) ) ;
#66922=CARTESIAN_POINT ( 'NONE',  ( 175.4968960841862895, 286.3374744733690136, -12.09459527608030172 ) ) ;
#66923=VERTEX_POINT ( 'NONE', #35959 ) ;
#66924=CARTESIAN_POINT ( 'NONE',  ( 157.7233946900069839, 257.4620621851055375, 16.86796251324260254 ) ) ;
#66925=CARTESIAN_POINT ( 'NONE',  ( 198.6894790592683080, 286.5067226703918095, -17.06774375037124614 ) ) ;
#66926=CARTESIAN_POINT ( 'NONE',  ( 16.79251956066557128, 174.3768266524160140, 9.188101187500096856 ) ) ;
#66928=CARTESIAN_POINT ( 'NONE',  ( 179.8888715531147682, 274.4711782159853328, -17.82026667163308531 ) ) ;
#66931=CARTESIAN_POINT ( 'NONE',  ( 157.3198323354746435, 258.1610526871778006, -16.77630483474704093 ) ) ;
#66933=CARTESIAN_POINT ( 'NONE',  ( 150.0923052775327449, 276.4933692631097983, 3.710611330911921524 ) ) ;
#66934=CARTESIAN_POINT ( 'NONE',  ( 167.4210765078939005, 256.7953526967608013, 14.03692215505185459 ) ) ;
#66935=CARTESIAN_POINT ( 'NONE',  ( 67.04888272437477781, 219.5177522451419065, 5.000000000000046185 ) ) ;
#66937=CARTESIAN_POINT ( 'NONE',  ( 197.9812996484125449, 287.7333253908681741, 17.50297787674340455 ) ) ;
#66939=CARTESIAN_POINT ( 'NONE',  ( 50.32376711733572705, 209.8615022471902876, 5.000000000000046185 ) ) ;
#66940=CARTESIAN_POINT ( 'NONE',  ( 181.8982906980151313, 291.6576164288949258, 9.318166351261279345 ) ) ;
#66941=CARTESIAN_POINT ( 'NONE',  ( 147.7157269441172218, 274.7958511862549926, 8.036290321896261801 ) ) ;
#66942=CARTESIAN_POINT ( 'NONE',  ( 17.82075117977708700, 181.0958772461660544, -9.188101187500095079 ) ) ;
#66947=CARTESIAN_POINT ( 'NONE',  ( 201.4636277339562298, 280.4837806593683354, -16.45470140429584660 ) ) ;
#66948=B_SPLINE_CURVE_WITH_KNOTS ( 'NONE', 3,
 ( #38955, #40453, #1485, #54143 ),
 .UNSPECIFIED., .F., .F.,
 ( 4, 4 ),
 ( 0.03503658997592057345, 0.04381483082515637284 ),
 .UNSPECIFIED. ) ;
#66949=CARTESIAN_POINT ( 'NONE',  ( 164.8251969117060298, 245.1613799118173063, -1.508678420156898348 ) ) ;
#66951=CARTESIAN_POINT ( 'NONE',  ( 153.2585711273538891, 265.9210912079520881, -16.19689858454334441 ) ) ;
#66952=CARTESIAN_POINT ( 'NONE',  ( 177.1159597426109258, 261.0416103176956426, -13.08779172971381044 ) ) ;
#66955=CARTESIAN_POINT ( 'NONE',  ( -14.37785915960194494, 174.0530062829863027, 6.972266317189433612E-15 ) ) ;
#66958=CARTESIAN_POINT ( 'NONE',  ( 154.9910882912764123, 262.1945556895526579, 18.38052604520346023 ) ) ;
#66960=CARTESIAN_POINT ( 'NONE',  ( 182.0334299555740074, 289.9311837412762998, 12.98645721431532785 ) ) ;
#66961=CARTESIAN_POINT ( 'NONE',  ( 156.8667541408265436, 276.4807214582178858, 10.34413747573048958 ) ) ;
#66962=CARTESIAN_POINT ( 'NONE',  ( 206.7680519836501958, 272.5142239127119979, -10.57935479673322021 ) ) ;
#66964=CARTESIAN_POINT ( 'NONE',  ( 196.6309300382015124, 289.4139301465927474, -16.57619966563450120 ) ) ;
#66965=CARTESIAN_POINT ( 'NONE',  ( 78.97477422587097351, 209.7365022471902307, 10.00000000000009948 ) ) ;
#66967=CARTESIAN_POINT ( 'NONE',  ( 202.8549823380854491, 279.2918593523859272, -16.39745931995414807 ) ) ;
#66971=B_SPLINE_CURVE_WITH_KNOTS ( 'NONE', 3,
 ( #55687, #86675, #54697, #17207 ),
 .UNSPECIFIED., .F., .F.,
 ( 4, 4 ),
 ( 0.008571673128587826290, 0.01494991930079212113 ),
 .UNSPECIFIED. ) ;
#66972=CARTESIAN_POINT ( 'NONE',  ( 164.6331389003996435, 246.4978176680588717, -4.355654215571391319 ) ) ;
#66973=CARTESIAN_POINT ( 'NONE',  ( 204.8762144138505903, 275.7909827032724479, 14.60855957933206817 ) ) ;
#66974=CARTESIAN_POINT ( 'NONE',  ( 153.1973045377566507, 265.3014802884401320, 17.70608187426261892 ) ) ;
#66976=CARTESIAN_POINT ( 'NONE',  ( 190.7851751463332164, 300.1973786460605425, 8.237717828100052486 ) ) ;
#66978=CARTESIAN_POINT ( 'NONE',  ( 174.5259399585505093, 262.2319009501799201, 15.75388500574217687 ) ) ;
#66979=ORIENTED_EDGE ( 'NONE', *, *, #15635, .F. ) ;
#66984=CARTESIAN_POINT ( 'NONE',  ( 165.0308887387863876, 244.8051112166122891, 1.948365933089477808 ) ) ;
#66985=CARTESIAN_POINT ( 'NONE',  ( 151.0104406072433960, 275.7624194085408362, -8.268042829941808947 ) ) ;
#66986=B_SPLINE_SURFACE_WITH_KNOTS ( 'NONE', 3, 1, ( 
 ( #43272, #27608 ),
 ( #72730, #73210 ),
 ( #66590, #82834 ),
 ( #27105, #57990 ),
 ( #97513, #58955 ),
 ( #13403, #20003 ),
 ( #3320, #59459 ),
 ( #98000, #74219 ),
 ( #88460, #82346 ),
 ( #34201, #80852 ),
 ( #36174, #4808 ),
 ( #26602, #50882 ),
 ( #73701, #89927 ),
 ( #81830, #11424 ),
 ( #4284, #20505 ),
 ( #49894, #88971 ),
 ( #5294, #28580 ),
 ( #42276, #51378 ),
 ( #57477, #35183 ),
 ( #65091, #66092 ),
 ( #12406, #67077 ),
 ( #89447, #58474 ),
 ( #90440, #3805 ),
 ( #12914, #43773 ),
 ( #21012, #34685 ),
 ( #65587, #96535 ),
 ( #50386, #19526 ),
 ( #85320, #5781 ),
 ( #54348, #92416 ),
 ( #7269, #75696 ),
 ( #76682, #52378 ),
 ( #22479, #61467 ),
 ( #13882, #69070 ),
 ( #46250, #99997 ) ),
 .UNSPECIFIED., .T., .F., .F.,
 ( 4, 2, 2, 2, 2, 2, 2, 2, 2, 2, 2, 2, 2, 2, 2, 2, 4 ),
 ( 2, 2 ),
 ( 0.000000000000000000, 0.06250000000000000000, 0.1250000000000000000, 0.1875000000000000000, 0.2500000000000000000, 0.3125000000000000000, 0.3750000000000000000, 0.4375000000000000000, 0.5000000000000000000, 0.5625000000000000000, 0.6250000000000000000, 0.6875000000000000000, 0.7500000000000000000, 0.8125000000000000000, 0.8750000000000000000, 0.9375000000000000000, 1.000000000000000000 ),
 ( 0.000000000000000000, 1.000000000000000000 ),
 .UNSPECIFIED. ) ;
#66988=CARTESIAN_POINT ( 'NONE',  ( 176.4997652591337669, 278.4766424938736122, -15.78386933605245623 ) ) ;
#66989=CARTESIAN_POINT ( 'NONE',  ( 169.8069776206597226, 261.6727971985682757, -16.70353856883196286 ) ) ;
#66991=CARTESIAN_POINT ( 'NONE',  ( 83.21237853290490705, 230.3967562850347122, -4.648177544792955347E-16 ) ) ;
#66992=CARTESIAN_POINT ( 'NONE',  ( 147.4824818982269790, 275.1998434563504929, -4.972419998968698351 ) ) ;
#66994=CARTESIAN_POINT ( 'NONE',  ( 157.1844736846585135, 269.4583905584224794, 15.72531959550208924 ) ) ;
#66995=ORIENTED_EDGE ( 'NONE', *, *, #59084, .F. ) ;
#66997=CARTESIAN_POINT ( 'NONE',  ( 37.58366506746438773, 204.0530062829863027, 1.101618078115930403E-13 ) ) ;
#66998=CARTESIAN_POINT ( 'NONE',  ( 188.6191100762007693, 298.5688725033372179, -4.585965395504582709 ) ) ;
#67000=CARTESIAN_POINT ( 'NONE',  ( 153.2712411579340426, 265.1734183057532732, 16.26687330118495467 ) ) ;
#67002=CARTESIAN_POINT ( 'NONE',  ( 178.5194744259596291, 291.5691938275101052, 6.150709895237527647 ) ) ;
#67004=CARTESIAN_POINT ( 'NONE',  ( 191.8000917695741805, 298.4394914891611847, -9.452573400474340914 ) ) ;
#67007=B_SPLINE_CURVE_WITH_KNOTS ( 'NONE', 3,
 ( #81266, #82270, #56910, #65029 ),
 .UNSPECIFIED., .F., .F.,
 ( 4, 4 ),
 ( 0.008211037360764261370, 0.01440753375246466364 ),
 .UNSPECIFIED. ) ;
#67009=CARTESIAN_POINT ( 'NONE',  ( 149.0164813726494799, 272.5428784278667536, -11.67305721329070423 ) ) ;
#67011=CARTESIAN_POINT ( 'NONE',  ( 198.3150362131025588, 287.1552767044814800, 18.53472937702030521 ) ) ;
#67012=ORIENTED_EDGE ( 'NONE', *, *, #15697, .T. ) ;
#67013=CARTESIAN_POINT ( 'NONE',  ( 167.7405389411880208, 287.2496306518623328, 3.554903326435361333 ) ) ;
#67015=EDGE_LOOP ( 'NONE', ( #9989, #661, #7977, #79098, #38295 ) ) ;
#67019=CARTESIAN_POINT ( 'NONE',  ( 160.3496834799760506, 252.9131965655305692, -14.64892343956422671 ) ) ;
#67020=CARTESIAN_POINT ( 'NONE',  ( 91.00660716696484087, 234.8967562850347122, -4.648177544792955347E-16 ) ) ;
#67021=EDGE_LOOP ( 'NONE', ( #81359, #97121, #3817, #54629 ) ) ;
#67022=CARTESIAN_POINT ( 'NONE',  ( 170.5601965100331654, 255.5687049720617949, -11.63993357083384872 ) ) ;
#67024=CARTESIAN_POINT ( 'NONE',  ( 153.2583947049096764, 265.1956690150883560, -17.64103123457563882 ) ) ;
#67025=CARTESIAN_POINT ( 'NONE',  ( 206.8968397926183229, 272.2911568841838061, 7.145103750817420440 ) ) ;
#67026=CARTESIAN_POINT ( 'NONE',  ( 31.61400995286156501, 182.3927522451417929, -10.00000000000009059 ) ) ;
#67027=CARTESIAN_POINT ( 'NONE',  ( 115.6001716039901055, 246.7369531367911009, -4.594050593750048428 ) ) ;
#67028=CARTESIAN_POINT ( 'NONE',  ( 180.8832283595195349, 294.1460411169432518, -2.655356583051106778 ) ) ;
#67029=CARTESIAN_POINT ( 'NONE',  ( 167.5733982946378546, 281.7299476539893135, -10.91913693171769495 ) ) ;
#67030=CARTESIAN_POINT ( 'NONE',  ( 157.2744851780909414, 258.2395962677452985, 18.17792129701959070 ) ) ;
#67031=CARTESIAN_POINT ( 'NONE',  ( -27.42236680055714260, 166.5217562850347406, 1.224646799147364892E-15 ) ) ;
#67033=CARTESIAN_POINT ( 'NONE',  ( 32.11017034222032862, 189.3458772461660544, 9.188101187500095079 ) ) ;
#67036=CARTESIAN_POINT ( 'NONE',  ( 190.9765749051877037, 299.0466983684623870, 7.380296417802154174 ) ) ;
#67044=CARTESIAN_POINT ( 'NONE',  ( 66.85041857288881317, 202.7365022471902023, -10.00000000000009237 ) ) ;
#67045=CARTESIAN_POINT ( 'NONE',  ( 182.2775398009696630, 262.7337698959310615, 12.80426946192887527 ) ) ;
#67046=CARTESIAN_POINT ( 'NONE',  ( 97.35977185683022128, 217.0177522451417929, 5.000000000000051514 ) ) ;
#67051=CARTESIAN_POINT ( 'NONE',  ( 202.3894997978090373, 280.0980987621804275, 16.95659012541789323 ) ) ;
#67052=CARTESIAN_POINT ( 'NONE',  ( 207.6067494229581314, 271.0615573356529353, -1.924113146155245868 ) ) ;
#67054=CARTESIAN_POINT ( 'NONE',  ( 9.836819166815537585, 185.6744531367911293, 4.594050593750047540 ) ) ;
#67060=FACE_OUTER_BOUND ( 'NONE', #58047, .T. ) ;
#67064=ORIENTED_EDGE ( 'NONE', *, *, #15275, .F. ) ;
#67065=CARTESIAN_POINT ( 'NONE',  ( 9.692741923115793412, 189.7365022471903444, 2.944929066748280225E-16 ) ) ;
#67066=CARTESIAN_POINT ( 'NONE',  ( 198.4198837630707715, 268.9924007542394406, -10.80133867637042222 ) ) ;
#67067=CARTESIAN_POINT ( 'NONE',  ( 136.0064158243085046, 240.1423013555409796, -4.594050593750043987 ) ) ;
#67072=CARTESIAN_POINT ( 'NONE',  ( 198.3089799798562467, 282.2162661195332021, -17.61972112454792949 ) ) ;
#67073=CARTESIAN_POINT ( 'NONE',  ( 157.8740713127050981, 257.2010826190796706, 17.31862062017425075 ) ) ;
#67074=CARTESIAN_POINT ( 'NONE',  ( 189.4308808934198680, 289.8491723414206831, 15.72891001903047048 ) ) ;
#67077=CARTESIAN_POINT ( 'NONE',  ( 151.4281781455628675, 268.3656970847310390, 15.24742929158552585 ) ) ;
#67078=CARTESIAN_POINT ( 'NONE',  ( 164.0386046892491549, 246.5237976059514153, 8.684266124902681128 ) ) ;
#67079=CARTESIAN_POINT ( 'NONE',  ( 171.6154833087297789, 255.2606305366970503, 12.53362356821959978 ) ) ;
#67080=CARTESIAN_POINT ( 'NONE',  ( 193.8726876411220701, 270.8218780147767575, -13.81544579610791956 ) ) ;
#67083=CARTESIAN_POINT ( 'NONE',  ( 171.1535303886575434, 284.5931741264590755, -11.54123640101257919 ) ) ;
#67086=EDGE_CURVE ( 'NONE', #39924, #20199, #80024, .T. ) ;
#67088=CARTESIAN_POINT ( 'NONE',  ( -22.42236680055709641, 157.8615022471902591, 0.000000000000000000 ) ) ;
#67089=CARTESIAN_POINT ( 'NONE',  ( 182.9953215290649950, 295.2195952053492647, 4.704045894889287815 ) ) ;
#67090=CARTESIAN_POINT ( 'NONE',  ( 162.9111474110223412, 248.4766108952035211, -9.702990628959184960 ) ) ;
#67091=CARTESIAN_POINT ( 'NONE',  ( 147.8158148994058365, 275.7822056701940028, 0.001258906972079423207 ) ) ;
#67093=ORIENTED_EDGE ( 'NONE', *, *, #35761, .T. ) ;
#67096=FACE_OUTER_BOUND ( 'NONE', #76700, .T. ) ;
#67097=ORIENTED_EDGE ( 'NONE', *, *, #2974, .F. ) ;
#67100=CARTESIAN_POINT ( 'NONE',  ( 156.3480092461931861, 261.3368746170128816, -17.50703484634064111 ) ) ;
#67101=ORIENTED_EDGE ( 'NONE', *, *, #25376, .T. ) ;
#67102=CARTESIAN_POINT ( 'NONE',  ( -17.42236680055705023, 149.2012482093457777, 0.000000000000000000 ) ) ;
#67103=CARTESIAN_POINT ( 'NONE',  ( 185.3708565686441716, 291.1367641197661555, 12.05567508508808672 ) ) ;
#67104=CARTESIAN_POINT ( 'NONE',  ( 204.5730103890532519, 276.3161474792809145, 14.88139715235883109 ) ) ;
#67105=CARTESIAN_POINT ( 'NONE',  ( 57.68498304950353628, 194.1115022471902023, -5.000000000000041744 ) ) ;
#67107=CARTESIAN_POINT ( 'NONE',  ( 79.55186417146283873, 225.9244531367911293, -4.594050593750046652 ) ) ;
#67108=CARTESIAN_POINT ( 'NONE',  ( 198.6931026323153162, 282.8313882593000130, 17.63783808752309668 ) ) ;
#67109=CARTESIAN_POINT ( 'NONE',  ( 181.3220768623721710, 271.3444700680324218, -16.03098847413529526 ) ) ;
#67110=CYLINDRICAL_SURFACE ( 'NONE', #91454, 17.82106496071139645 ) ;
#67112=ADVANCED_FACE ( 'NONE', ( #2753 ), #53888, .F. ) ;
#67114=CARTESIAN_POINT ( 'NONE',  ( 207.1181895030469491, 269.9077679394811753, 1.745611964362854929 ) ) ;
#67120=CARTESIAN_POINT ( 'NONE',  ( 203.3041373168503299, 278.5139001086923827, -16.61929732091214973 ) ) ;
#67121=ORIENTED_EDGE ( 'NONE', *, *, #54311, .F. ) ;
#67123=CARTESIAN_POINT ( 'NONE',  ( 182.7847760313759409, 280.0284915794045446, -17.53211380394024843 ) ) ;
#67124=CARTESIAN_POINT ( 'NONE',  ( 178.1281481821618797, 292.9991590599575488, -6.064681374715556572 ) ) ;
#67126=EDGE_CURVE ( 'NONE', #63881, #58975, #46221, .T. ) ;
#67130=CARTESIAN_POINT ( 'NONE',  ( 164.7913975190338078, 265.1675190917550822, -16.61937175513660492 ) ) ;
#67131=VERTEX_POINT ( 'NONE', #23274 ) ;
#67135=EDGE_CURVE ( 'NONE', #92664, #28922, #34062, .T. ) ;
#67136=CARTESIAN_POINT ( 'NONE',  ( 167.4788697440488932, 284.1975178938891418, 9.214407018017913842 ) ) ;
#67137=CARTESIAN_POINT ( 'NONE',  ( 199.8955426817768455, 270.2827091269795119, 9.689898955748889264 ) ) ;
#67139=EDGE_CURVE ( 'NONE', #62095, #40534, #57004, .T. ) ;
#67140=CARTESIAN_POINT ( 'NONE',  ( 202.3139361598622372, 280.2289788223093865, 15.93832709035092421 ) ) ;
#67141=EDGE_CURVE ( 'NONE', #27033, #61969, #75154, .T. ) ;
#67142=CARTESIAN_POINT ( 'NONE',  ( 206.8106726053982811, 272.4404028303941914, -10.47827087991598560 ) ) ;
#67143=CARTESIAN_POINT ( 'NONE',  ( 149.2575837200583067, 276.2297180982410509, -5.451514945794049716 ) ) ;
#67144=CARTESIAN_POINT ( 'NONE',  ( 165.0940603251445680, 246.6293290676431127, -1.873067877571933826 ) ) ;
#67145=CARTESIAN_POINT ( 'NONE',  ( 185.8626946602280441, 259.3471889805154547, 7.308832903665572367 ) ) ;
#67149=CARTESIAN_POINT ( 'NONE',  ( 181.8041777747191645, 271.4364937356251062, -15.98274022405578343 ) ) ;
#67152=CARTESIAN_POINT ( 'NONE',  ( 193.2165179683147471, 294.2034512776308475, -14.44099136285982254 ) ) ;
#67156=CARTESIAN_POINT ( 'NONE',  ( 164.3560589188577410, 274.2738242027600677, 14.76370921553832360 ) ) ;
#67157=CARTESIAN_POINT ( 'NONE',  ( -3.992090130160959482, 162.3768266524160140, 9.188101187500098632 ) ) ;
#67163=DIRECTION ( 'NONE',  ( -0.8660254037844387076, -0.4999999999999998890, -0.000000000000000000 ) ) ;
#67164=CARTESIAN_POINT ( 'NONE',  ( 190.0738558021110691, 273.7331793950331758, -15.69528651041143519 ) ) ;
#67169=CARTESIAN_POINT ( 'NONE',  ( 166.7187202459675746, 278.5591580196478958, -14.78021074750266273 ) ) ;
#67170=CARTESIAN_POINT ( 'NONE',  ( 5.669592554750444435, 164.8923013555410080, 4.594050593750050204 ) ) ;
#67171=CARTESIAN_POINT ( 'NONE',  ( 109.2678814824639204, 224.7048013555410080, 4.594050593750051981 ) ) ;
#67172=CARTESIAN_POINT ( 'NONE',  ( 40.06571587503326271, 205.4860189848785694, -2.679491924311252493 ) ) ;
#67173=CARTESIAN_POINT ( 'NONE',  ( 186.6662094383440262, 296.0905088883881149, -7.390743538549633840 ) ) ;
#67175=CARTESIAN_POINT ( 'NONE',  ( 176.6301829438279185, 282.3654047892467815, -14.24849079710228139 ) ) ;
#67177=CARTESIAN_POINT ( 'NONE',  ( 193.7999837595647250, 294.9755769528473479, 15.24609078262870199 ) ) ;
#67178=CARTESIAN_POINT ( 'NONE',  ( 184.1472144282555519, 274.8408247889214522, 16.39501531948747015 ) ) ;
#67179=CARTESIAN_POINT ( 'NONE',  ( 194.3708539535661259, 293.9868007723104029, -16.01585187499628304 ) ) ;
#67182=CARTESIAN_POINT ( 'NONE',  ( 187.1286666404986363, 298.8789080593439280, -0.5945842851373613902 ) ) ;
#67183=CARTESIAN_POINT ( 'NONE',  ( 47.29267820409018697, 208.1115022471903160, -5.000000000000047962 ) ) ;
#67184=CARTESIAN_POINT ( 'NONE',  ( 184.2717516226944952, 268.6604825781803356, -15.25338787826597198 ) ) ;
#67188=CARTESIAN_POINT ( 'NONE',  ( 84.74801659416949917, 228.9244531367911293, -4.594050593750046652 ) ) ;
#67190=CARTESIAN_POINT ( 'NONE',  ( 156.6812872898450735, 261.2670451491295012, 0.000000000000000000 ) ) ;
#67192=CARTESIAN_POINT ( 'NONE',  ( 159.0119062629668747, 259.2772906885834345, -17.27827472792992580 ) ) ;
#67193=CARTESIAN_POINT ( 'NONE',  ( 196.1573359623355088, 290.8925231663144473, 17.55680092534192482 ) ) ;
#67194=CARTESIAN_POINT ( 'NONE',  ( 200.2925563156679800, 283.7301114138494427, 18.37231090996849048 ) ) ;
#67195=B_SPLINE_CURVE_WITH_KNOTS ( 'NONE', 3,
 ( #49458, #89044, #11492, #10984, #73769, #19590, #73275, #34264, #81900, #88527, #35255, #81404, #41348, #11974, #19087, #66163, #97108, #12477, #43344, #56557, #87544, #33790, #52939, #14928, #76268, #4876, #51450, #44340, #67149, #60032, #37242, #74293, #90509, #82419, #68140, #35757, #68636, #98071, #75768, #66655, #6356, #30140, #12984, #60526, #36243, #14455, #36739, #99068, #29161, #99557, #61024, #75269 ),
 .UNSPECIFIED., .F., .F.,
 ( 4, 2, 2, 2, 2, 2, 2, 2, 2, 2, 2, 2, 2, 2, 2, 2, 2, 2, 2, 2, 2, 2, 2, 2, 2, 4 ),
 ( 0.0001034768661984681600, 0.001103434164929440256, 0.001353423489612237988, 0.001603412814295035720, 0.001728407476636464402, 0.001853402138977892650, 0.001978396801319321115, 0.002103391463660749579, 0.002353380788343550998, 0.002603370113026352850, 0.003103348762392025510, 0.004103306061123445855, 0.005103263359854866635, 0.005603242009220577025, 0.005853231333903432219, 0.005978225996244816882, 0.006103220658586201545, 0.006165717989756862652, 0.006228215320927522891, 0.006353209983268867656, 0.006603199307951555450, 0.006853188632634243244, 0.007103177957316931905, 0.007353167281999618832, 0.007603156606682307493, 0.008103135256047678744 ),
 .UNSPECIFIED. ) ;
#67196=CARTESIAN_POINT ( 'NONE',  ( 149.6188047043597180, 271.4996238147605823, 11.68007032781935628 ) ) ;
#67197=B_SPLINE_CURVE_WITH_KNOTS ( 'NONE', 3,
 ( #41292, #17509, #78831, #32706 ),
 .UNSPECIFIED., .F., .F.,
 ( 4, 4 ),
 ( 0.009381926372693255231, 0.01459774425476862911 ),
 .UNSPECIFIED. ) ;
#67198=CARTESIAN_POINT ( 'NONE',  ( 151.2567985338353935, 268.6625352796243646, -15.71756535662528798 ) ) ;
#67201=CARTESIAN_POINT ( 'NONE',  ( 146.7944005049231180, 276.3916353892955726, -4.243051111306586520 ) ) ;
#67203=ORIENTED_EDGE ( 'NONE', *, *, #92811, .T. ) ;
#67207=CARTESIAN_POINT ( 'NONE',  ( 191.7076580884861414, 287.9117833154688242, -15.84525881108999101 ) ) ;
#67208=EDGE_CURVE ( 'NONE', #53616, #74626, #87434, .T. ) ;
#67211=CARTESIAN_POINT ( 'NONE',  ( 198.5558597050348908, 286.7381581807989051, 17.16554469393394200 ) ) ;
#67212=CARTESIAN_POINT ( 'NONE',  ( 181.0931619117654634, 256.6297595461512060, 7.400322454308797759 ) ) ;
#67215=CARTESIAN_POINT ( 'NONE',  ( 134.2560625007776025, 254.9865022471903444, -10.00000000000009415 ) ) ;
#67219=CARTESIAN_POINT ( 'NONE',  ( 196.9612820325353368, 264.9694946870639569, -4.623214399652447959 ) ) ;
#67225=CARTESIAN_POINT ( 'NONE',  ( 158.6379490615327938, 255.8780075473385125, 17.62002732432160812 ) ) ;
#67226=CARTESIAN_POINT ( 'NONE',  ( 148.0493212738620628, 256.2833772461660828, -9.188101187500095079 ) ) ;
#67227=CARTESIAN_POINT ( 'NONE',  ( 153.6741866004717849, 264.4754963265993979, -18.11073193088522260 ) ) ;
#67228=CARTESIAN_POINT ( 'NONE',  ( 152.9607371460978129, 265.7112270302071124, -16.17698032818104537 ) ) ;
#67232=CARTESIAN_POINT ( 'NONE',  ( 164.6704117653912078, 274.4925094543679052, 14.73674799813685965 ) ) ;
#67233=CARTESIAN_POINT ( 'NONE',  ( 64.97403019802248991, 214.9865022471903160, 10.00000000000009415 ) ) ;
#67234=AXIS2_PLACEMENT_3D ( 'NONE', #46182, #52794, #7704 ) ;
#67236=VERTEX_POINT ( 'NONE', #41468 ) ;
#67238=ADVANCED_FACE ( 'NONE', ( #18198 ), #34385, .T. ) ;
#67239=CARTESIAN_POINT ( 'NONE',  ( 164.3010377730689981, 246.0692501711882869, 7.247566249275159578 ) ) ;
#67240=CARTESIAN_POINT ( 'NONE',  ( 162.2660344477049819, 272.4068407072390983, -16.13375623211421583 ) ) ;
#67241=CARTESIAN_POINT ( 'NONE',  ( 195.6664450926536460, 278.3245960621525796, 17.18455885460583232 ) ) ;
#67242=CARTESIAN_POINT ( 'NONE',  ( 194.0672051292551430, 294.5127359636757660, 15.53337744471869364 ) ) ;
#67244=CARTESIAN_POINT ( 'NONE',  ( 147.6220714307702622, 274.9580672937808572, 8.392894244419288441 ) ) ;
#67245=CARTESIAN_POINT ( 'NONE',  ( 167.2717594564306296, 286.8017429457753451, -4.937469463271268566 ) ) ;
#67247=CARTESIAN_POINT ( 'NONE',  ( 178.1826077084033102, 255.5164715494353516, 4.895996780289697092 ) ) ;
#67249=CARTESIAN_POINT ( 'NONE',  ( 101.1213961584103060, 235.3149278399160949, -9.188101187500095079 ) ) ;
#67251=CARTESIAN_POINT ( 'NONE',  ( 173.0837253472800796, 264.8280141993791972, 17.07053884509587860 ) ) ;
#67252=CARTESIAN_POINT ( 'NONE',  ( 165.3763302323083053, 271.0598910717424701, 16.49088855851117685 ) ) ;
#67253=CARTESIAN_POINT ( 'NONE',  ( 190.3288472781666201, 274.6029090957763401, 15.82415357830627833 ) ) ;
#67259=CARTESIAN_POINT ( 'NONE',  ( 180.7412255709484157, 294.1235929814394012, -2.454474088018941735 ) ) ;
#67260=CARTESIAN_POINT ( 'NONE',  ( 196.3720681610792553, 290.5205960880691691, 16.18360420724715354 ) ) ;
#67261=CARTESIAN_POINT ( 'NONE',  ( 190.2925905131754973, 300.4452873534128230, -0.07860713051909268279 ) ) ;
#67263=ORIENTED_EDGE ( 'NONE', *, *, #23403, .F. ) ;
#67266=CARTESIAN_POINT ( 'NONE',  ( 207.7837159184916231, 270.7550423741513441, -2.369602332675663448 ) ) ;
#67269=CARTESIAN_POINT ( 'NONE',  ( 153.2595589010950334, 265.6112048380699093, 16.12693562537618419 ) ) ;
#67271=CARTESIAN_POINT ( 'NONE',  ( 184.3063639896893164, 288.6967878748712337, -13.31555908468126503 ) ) ;
#67275=CARTESIAN_POINT ( 'NONE',  ( 58.48430016207534976, 216.1199935810940929, 2.679491924311251605 ) ) ;
#67276=B_SPLINE_CURVE_WITH_KNOTS ( 'NONE', 3,
 ( #83526, #44975, #29300, #91614 ),
 .UNSPECIFIED., .F., .F.,
 ( 4, 4 ),
 ( 0.04432367838347623518, 0.04887066958154932111 ),
 .UNSPECIFIED. ) ;
#67277=CARTESIAN_POINT ( 'NONE',  ( 62.44812277031795134, 196.8615022471901739, 5.000000000000051514 ) ) ;
#67279=CARTESIAN_POINT ( 'NONE',  ( 192.9108229344522840, 270.9309780692502159, 14.84737179462503676 ) ) ;
#67280=CARTESIAN_POINT ( 'NONE',  ( 116.0695290213043620, 244.4865022471902876, -10.00000000000009592 ) ) ;
#67282=CARTESIAN_POINT ( 'NONE',  ( 195.5549742635668622, 279.7421760486213884, -16.96403059063067431 ) ) ;
#67286=CARTESIAN_POINT ( 'NONE',  ( 69.24135662524314228, 198.5327760586659451, 1.948934522072303157E-15 ) ) ;
#67287=CARTESIAN_POINT ( 'NONE',  ( 206.5081929095101998, 272.9643130319303737, -9.215516226794479238 ) ) ;
#67289=CARTESIAN_POINT ( 'NONE',  ( 208.0006710756887287, 270.3792650189220126, -0.8737665032493013850 ) ) ;
#67290=ADVANCED_FACE ( 'NONE', ( #13587 ), #44461, .T. ) ;
#67293=CARTESIAN_POINT ( 'NONE',  ( 207.8792014703394671, 270.5896565469619759, -5.780233892547864905 ) ) ;
#67296=CARTESIAN_POINT ( 'NONE',  ( 185.8891070060977881, 265.5474094253055455, 13.37913739288876158 ) ) ;
#67300=CARTESIAN_POINT ( 'NONE',  ( 157.7666006523658666, 270.6297847174233766, -15.52481408403261298 ) ) ;
#67303=CARTESIAN_POINT ( 'NONE',  ( 27.99689677000926125, 174.7202760586659736, -5.415160957724236172E-17 ) ) ;
#67304=CARTESIAN_POINT ( 'NONE',  ( 157.8360072705708603, 257.2670114739976839, 17.12122855844125269 ) ) ;
#67306=EDGE_CURVE ( 'NONE', #23235, #73362, #78735, .T. ) ;
#67307=CARTESIAN_POINT ( 'NONE',  ( 194.3177355571849318, 294.0788045336591381, -15.93712594727561616 ) ) ;
#67309=CARTESIAN_POINT ( 'NONE',  ( 43.28705038798948124, 204.9869531367911293, 4.594050593750046652 ) ) ;
#67311=CARTESIAN_POINT ( 'NONE',  ( 171.3082047287566922, 286.6656704798778037, 7.347939393563489574 ) ) ;
#67314=CARTESIAN_POINT ( 'NONE',  ( 172.8951663193395234, 288.9549776225803157, 8.104654168245465584 ) ) ;
#67315=CARTESIAN_POINT ( 'NONE',  ( 175.7518161566136996, 291.0577149723374077, 2.541557124732606976 ) ) ;
#67316=CARTESIAN_POINT ( 'NONE',  ( 180.0693756861613508, 276.3240737636226072, 16.71396866487755517 ) ) ;
#67319=CARTESIAN_POINT ( 'NONE',  ( 191.9987047080313687, 267.0019276258636864, 10.95647444719745067 ) ) ;
#67325=CARTESIAN_POINT ( 'NONE',  ( 103.1513167481865310, 230.3615022471902591, -10.00000000000009592 ) ) ;
#67326=( BOUNDED_CURVE ( )  B_SPLINE_CURVE ( 2, ( #91517, #97141, #50484, #4392, #27710, #43381, #13508, #97621, #29200 ),
 .UNSPECIFIED., .F., .T. ) 
 B_SPLINE_CURVE_WITH_KNOTS ( ( 3, 2, 2, 2, 3 ),
 ( 0.5927419354838709964, 0.5940860215053763715, 0.5967741935483871218, 0.5994623655913978721, 0.6008064516129032473 ),
 .UNSPECIFIED. ) 
 CURVE ( )  GEOMETRIC_REPRESENTATION_ITEM ( )  RATIONAL_B_SPLINE_CURVE ( ( 0.9330127018922194093, 0.9330127018922194093, 1.000000000000000000, 0.8660254037844387076, 1.000000000000000000, 0.8660254037844387076, 1.000000000000000000, 0.9330127018922194093, 0.9330127018922194093 ) ) 
 REPRESENTATION_ITEM ( '' )  );
#67327=CARTESIAN_POINT ( 'NONE',  ( 200.1782072557437857, 283.9281697954355650, 18.05177561285849208 ) ) ;
#67328=CARTESIAN_POINT ( 'NONE',  ( 164.3266432466909635, 269.1343096826732335, -16.34300100545284806 ) ) ;
#67330=CARTESIAN_POINT ( 'NONE',  ( 65.53359859134977228, 199.4548013555410080, -4.594050593750042211 ) ) ;
#67332=CARTESIAN_POINT ( 'NONE',  ( 163.7906117146278007, 264.0004031999091580, 16.81624561942971141 ) ) ;
#67333=CARTESIAN_POINT ( 'NONE',  ( 190.1607982559816890, 301.2788311432216233, -4.972636536415983244 ) ) ;
#67334=CYLINDRICAL_SURFACE ( 'NONE', #88839, 10.00000000000010658 ) ;
#67335=VERTEX_POINT ( 'NONE', #55055 ) ;
#67336=DIRECTION ( 'NONE',  ( 0.4999999999999998890, -0.8660254037844385966, 0.000000000000000000 ) ) ;
#67338=FACE_OUTER_BOUND ( 'NONE', #29758, .T. ) ;
#67339=CARTESIAN_POINT ( 'NONE',  ( 189.1123083253427524, 265.5175477926164262, 10.65947824442831582 ) ) ;
#67340=CARTESIAN_POINT ( 'NONE',  ( 149.2223635749290622, 272.1862799931444670, -12.97307652490353647 ) ) ;
#67341=CARTESIAN_POINT ( 'NONE',  ( 157.4493702961534609, 257.9366863577731124, 17.30941950273115637 ) ) ;
#67342=ORIENTED_EDGE ( 'NONE', *, *, #91626, .T. ) ;
#67346=CARTESIAN_POINT ( 'NONE',  ( 15.68275096595825246, 169.8615022471901739, 5.000000000000051514 ) ) ;
#67347=ORIENTED_EDGE ( 'NONE', *, *, #16992, .F. ) ;
#67349=CARTESIAN_POINT ( 'NONE',  ( 206.1615484827472358, 273.5647187912443314, -9.556459874778100883 ) ) ;
#67350=ORIENTED_EDGE ( 'NONE', *, *, #16849, .F. ) ;
#67352=CARTESIAN_POINT ( 'NONE',  ( 159.9700686533283545, 282.3153680940349091, -3.195712497083830428 ) ) ;
#67353=CARTESIAN_POINT ( 'NONE',  ( 167.6278246310154714, 282.5728663012718584, -12.21306354836790220 ) ) ;
#67354=B_SPLINE_CURVE_WITH_KNOTS ( 'NONE', 3,
 ( #99994, #94776, #52868, #14385, #61464, #84811, #92413, #22962, #1560, #63341, #24834, #55708, #86698, #17231, #83144, #97836, #98831, #13713, #75523, #51728, #12742, #44588, #6107, #89762, #46458, #15556, #77389, #75033, #66417, #21318, #43090, #29413, #60282, #20835, #74543, #98330, #13236, #37003, #28405, #91240, #67913, #82671, #43606, #44090, #36002, #23164, #5611, #36503, #4623, #52196, #59285, #54055 ),
 .UNSPECIFIED., .F., .F.,
 ( 4, 2, 2, 2, 2, 2, 2, 2, 2, 2, 2, 2, 2, 2, 2, 2, 2, 2, 2, 2, 2, 2, 2, 2, 2, 4 ),
 ( 0.0001917148712815067418, 0.0006789549353198572144, 0.001166194999358207470, 0.001409815031377382706, 0.001531625047387005778, 0.001653435063396629066, 0.001775245079406251921, 0.001897055095415875210, 0.002140675127435058903, 0.002627915191473567669, 0.003115155255512077302, 0.004089635383589248357, 0.005064115511666418545, 0.005551355575704968945, 0.005794975607724279706, 0.005916785623733899525, 0.006038595639743519344, 0.006099500647748285452, 0.006160405655753053294, 0.006282215671762459742, 0.006525835703781275240, 0.006769455735800090738, 0.007013075767818906237, 0.007256695799837721735, 0.007500315831856535498, 0.007987555895894149147 ),
 .UNSPECIFIED. ) ;
#67355=CARTESIAN_POINT ( 'NONE',  ( 196.4242782546697015, 290.4301655533025155, -16.42402868779123537 ) ) ;
#67359=CARTESIAN_POINT ( 'NONE',  ( 164.1983466568012204, 264.8415231586690766, -16.64664350988114805 ) ) ;
#67360=CARTESIAN_POINT ( 'NONE',  ( 125.9656734773588767, 243.5333772461660544, 9.188101187500095079 ) ) ;
#67361=CARTESIAN_POINT ( 'NONE',  ( 190.8860811105559208, 300.0226043892405414, 8.636347304323541252 ) ) ;
#67362=EDGE_LOOP ( 'NONE', ( #85073, #45889, #93399, #21372, #81829 ) ) ;
#67363=CARTESIAN_POINT ( 'NONE',  ( 171.6951446231546754, 264.4514783956147994, 15.84364160967604107 ) ) ;
#67365=CARTESIAN_POINT ( 'NONE',  ( 205.7627300303947209, 272.2554926137148072, 9.584172220806708609 ) ) ;
#67366=AXIS2_PLACEMENT_3D ( 'NONE', #5082, #11208, #43048 ) ;
#67373=CARTESIAN_POINT ( 'NONE',  ( 167.7752291157694060, 263.0549901451653909, 17.37553087914205108 ) ) ;
#67374=CARTESIAN_POINT ( 'NONE',  ( 79.47110815956433783, 210.5643266524160424, 9.188101187500095079 ) ) ;
#67377=CARTESIAN_POINT ( 'NONE',  ( 194.2321518193436987, 294.2270399159019121, 13.98132384850917020 ) ) ;
#67379=CARTESIAN_POINT ( 'NONE',  ( 81.52103558181507026, 206.3262482093457493, 3.021315404115420679E-15 ) ) ;
#67382=CARTESIAN_POINT ( 'NONE',  ( 201.2139346379346705, 282.1342373466909521, -16.65315141107179286 ) ) ;
#67385=CARTESIAN_POINT ( 'NONE',  ( 164.9101359252495627, 286.5608941336866451, 1.040025780022917790 ) ) ;
#67388=CARTESIAN_POINT ( 'NONE',  ( 163.1711007600727896, 271.8830279655337563, 16.80804004369181470 ) ) ;
#67390=EDGE_CURVE ( 'NONE', #17277, #3978, #92822, .T. ) ;
#67392=CARTESIAN_POINT ( 'NONE',  ( 171.5015609157691756, 284.1786740197875361, -12.77546238284419644 ) ) ;
#67395=CARTESIAN_POINT ( 'NONE',  ( 163.9910908123517288, 246.6060940548019289, -7.333295033952830444 ) ) ;
#67396=CARTESIAN_POINT ( 'NONE',  ( 131.9464011004214115, 256.1744531367911009, 4.594050593750047540 ) ) ;
#67399=CARTESIAN_POINT ( 'NONE',  ( 182.2526911774749863, 258.0866462446188621, 6.496747210627928482 ) ) ;
#67400=CARTESIAN_POINT ( 'NONE',  ( 155.9752437318130092, 261.9691388090409987, -16.96517095716611223 ) ) ;
#67407=CARTESIAN_POINT ( 'NONE',  ( 167.7367314525692450, 248.9893787533955845, -6.380446527117325850 ) ) ;
#67409=CARTESIAN_POINT ( 'NONE',  ( 202.6348823940195416, 267.5801589924517430, 0.8677112048283521784 ) ) ;
#67410=CARTESIAN_POINT ( 'NONE',  ( 198.4463628819689518, 266.2085727128749681, 0.7937034711031139000 ) ) ;
#67415=CARTESIAN_POINT ( 'NONE',  ( 148.9232972370683399, 272.7042780851529642, 12.27045554427055940 ) ) ;
#67418=CARTESIAN_POINT ( 'NONE',  ( 198.4706398937704819, 286.8857632237200619, 17.04020736381253798 ) ) ;
#67419=CARTESIAN_POINT ( 'NONE',  ( 207.1656244175204904, 271.8256082575600772, 5.677357035859670553 ) ) ;
#67420=CARTESIAN_POINT ( 'NONE',  ( 138.8568224548345142, 257.6427522451418781, 10.00000000000009237 ) ) ;
#67421=CARTESIAN_POINT ( 'NONE',  ( 175.6294869978224824, 285.1187962335359884, -12.03725621959783965 ) ) ;
#67424=CARTESIAN_POINT ( 'NONE',  ( 198.5954523381739989, 286.6695817285962562, -18.45134152028667174 ) ) ;
#67425=CARTESIAN_POINT ( 'NONE',  ( 8.375921941576814689, 166.4548013555410080, -4.594050593750042211 ) ) ;
#67427=CARTESIAN_POINT ( 'NONE',  ( 176.5041649521335785, 257.7439588032058850, -10.43691933783435033 ) ) ;
#67430=CARTESIAN_POINT ( 'NONE',  ( 173.3022401097396994, 272.4925259712034062, -16.36549126867647885 ) ) ;
#67433=CARTESIAN_POINT ( 'NONE',  ( 159.9924463476198753, 283.3850188831759169, -3.371971149216307140 ) ) ;
#67434=CARTESIAN_POINT ( 'NONE',  ( 199.2940578277500947, 270.9390390980777852, -11.07481327316625475 ) ) ;
#67436=CARTESIAN_POINT ( 'NONE',  ( 198.3452313965520375, 287.1029771126029573, 18.55943827821351988 ) ) ;
#67437=EDGE_CURVE ( 'NONE', #22269, #8176, #92045, .T. ) ;
#67440=CARTESIAN_POINT ( 'NONE',  ( 179.6472821955170502, 294.1049463973150750, 1.034999459313757031 ) ) ;
#67441=CARTESIAN_POINT ( 'NONE',  ( 58.98402115518014455, 204.8615022471902307, -10.00000000000009592 ) ) ;
#67443=CARTESIAN_POINT ( 'NONE',  ( 147.7870527676176948, 274.6723112360602386, 9.257357958194809555 ) ) ;
#67444=EDGE_CURVE ( 'NONE', #41212, #32812, #7293, .T. ) ;
#67445=CARTESIAN_POINT ( 'NONE',  ( 19.87790860953014160, 170.0327760586659736, 1.948934522072303157E-15 ) ) ;
#67446=CARTESIAN_POINT ( 'NONE',  ( 164.3611296587836534, 285.2410164061814726, 4.345597304788310744 ) ) ;
#67450=CARTESIAN_POINT ( 'NONE',  ( 202.0843741143341674, 280.2366252626259211, -15.81775788646446301 ) ) ;
#67451=CARTESIAN_POINT ( 'NONE',  ( 206.9878665138179770, 272.1334939782196329, 6.566295309274049252 ) ) ;
#67452=CARTESIAN_POINT ( 'NONE',  ( 188.3628283273592956, 268.0339897934310329, 13.46669696773310498 ) ) ;
#67454=CARTESIAN_POINT ( 'NONE',  ( 179.7688937921471677, 262.9204303630262984, -13.99243624848556244 ) ) ;
#67460=CARTESIAN_POINT ( 'NONE',  ( 193.9844289374573520, 294.6561085335266625, 15.49818881749970245 ) ) ;
#67471=CARTESIAN_POINT ( 'NONE',  ( 202.9547455376043672, 279.1190644220934018, -15.19669173352461478 ) ) ;
#67474=CARTESIAN_POINT ( 'NONE',  ( 201.5801617693437890, 279.7599021095377907, 16.47958900488177036 ) ) ;
#67475=CARTESIAN_POINT ( 'NONE',  ( 204.9608076533459950, 275.6444629144898499, 14.31488288944633069 ) ) ;
#67476=CARTESIAN_POINT ( 'NONE',  ( 153.4477557824949940, 264.8676860077344486, 17.16010094972647693 ) ) ;
#67478=CARTESIAN_POINT ( 'NONE',  ( 150.6571681785161445, 269.7011255207979730, 15.24894850018880454 ) ) ;
#67482=CARTESIAN_POINT ( 'NONE',  ( 147.6220714307702622, 274.9580672937808572, 8.392894244419288441 ) ) ;
#67484=ORIENTED_EDGE ( 'NONE', *, *, #50380, .F. ) ;
#67485=CARTESIAN_POINT ( 'NONE',  ( 164.3754245770190039, 245.9404084473339083, 1.667926061651832992 ) ) ;
#67487=ORIENTED_EDGE ( 'NONE', *, *, #11338, .T. ) ;
#67488=CARTESIAN_POINT ( 'NONE',  ( 177.7398568146338107, 279.4700101068085019, -16.54123403330698849 ) ) ;
#67489=CARTESIAN_POINT ( 'NONE',  ( 172.2915296418940443, 263.9746128868251276, -15.63729134622028205 ) ) ;
#67491=CARTESIAN_POINT ( 'NONE',  ( 158.6626729816061925, 274.8399133342844607, -13.49366594499505645 ) ) ;
#67492=CARTESIAN_POINT ( 'NONE',  ( 60.96635096964421763, 217.5530062829863027, -4.648177544792955347E-16 ) ) ;
#67500=CARTESIAN_POINT ( 'NONE',  ( 148.9498507103374152, 272.6582861203333437, 11.90061892622094852 ) ) ;
#67501=CARTESIAN_POINT ( 'NONE',  ( 157.0701535447001334, 259.2118014948599694, -17.01617165317321323 ) ) ;
#67502=CARTESIAN_POINT ( 'NONE',  ( 147.2048811707249456, 275.6806620206021421, -0.5293868638167661400 ) ) ;
#67503=CARTESIAN_POINT ( 'NONE',  ( 191.2111338740054975, 299.4595964878050154, -9.718193530796334301 ) ) ;
#67508=CARTESIAN_POINT ( 'NONE',  ( 149.3545991938273971, 273.9572411826421217, -10.14243178476390028 ) ) ;
#67511=CARTESIAN_POINT ( 'NONE',  ( 171.5371663410915630, 288.9842175639024617, 4.255310109042821587 ) ) ;
#67515=CARTESIAN_POINT ( 'NONE',  ( 149.0323978447938202, 272.5153102894354333, -11.84998907946122060 ) ) ;
#67516=CARTESIAN_POINT ( 'NONE',  ( 198.2505066714982149, 285.2670451491296149, 0.000000000000000000 ) ) ;
#67517=CARTESIAN_POINT ( 'NONE',  ( 202.4560076411394220, 279.0611292670678267, 15.58065739802832717 ) ) ;
#67519=CARTESIAN_POINT ( 'NONE',  ( 39.49844957003023893, 203.6115022471903160, -5.000000000000047962 ) ) ;
#67522=CARTESIAN_POINT ( 'NONE',  ( 170.4914208022274522, 255.7692698374902136, -12.13427622590457844 ) ) ;
#67524=CARTESIAN_POINT ( 'NONE',  ( 205.7350094608039228, 273.2218331975091132, 10.02726759709120330 ) ) ;
#67525=CARTESIAN_POINT ( 'NONE',  ( 155.3085688348458007, 262.3516442638374997, 17.09768579440982705 ) ) ;
#67526=ADVANCED_FACE ( 'NONE', ( #45460 ), #61165, .F. ) ;
#67527=CARTESIAN_POINT ( 'NONE',  ( 38.47004439948830168, 203.0177522451419350, 5.000000000000046185 ) ) ;
#67528=CARTESIAN_POINT ( 'NONE',  ( 114.1117772151768577, 242.8149278399161233, -9.188101187500095079 ) ) ;
#67529=CARTESIAN_POINT ( 'NONE',  ( 151.0388915836658725, 269.0399611886400635, -14.24896787280406585 ) ) ;
#67530=CARTESIAN_POINT ( 'NONE',  ( 166.1193465202780715, 270.2353025340392492, 17.56265815376753636 ) ) ;
#67532=CARTESIAN_POINT ( 'NONE',  ( 172.3284624602130748, 251.0446003553498713, -4.012660189023237400 ) ) ;
#67533=CARTESIAN_POINT ( 'NONE',  ( 32.89474554257621719, 198.9869531367911293, 4.594050593750046652 ) ) ;
#67534=CARTESIAN_POINT ( 'NONE',  ( 147.6853019674385337, 275.3811002756974062, -3.519384196793790220 ) ) ;
#67537=DIRECTION ( 'NONE',  ( -0.8660254037844387076, -0.4999999999999998890, -0.000000000000000000 ) ) ;
#67538=CARTESIAN_POINT ( 'NONE',  ( 177.8945296157199039, 265.5031784322380304, 15.66114811942481033 ) ) ;
#67540=CARTESIAN_POINT ( 'NONE',  ( 190.8545714895799392, 300.0771806536980648, -5.516553996882049837 ) ) ;
#67541=CARTESIAN_POINT ( 'NONE',  ( 150.2076754159204484, 245.9824982072973683, 3.021315404115420679E-15 ) ) ;
#67542=CARTESIAN_POINT ( 'NONE',  ( 168.8244094625508751, 257.0541383169796745, -14.93690306707719628 ) ) ;
#67543=CARTESIAN_POINT ( 'NONE',  ( 178.2996191249796425, 286.8120259801574434, -12.18722290671415465 ) ) ;
#67545=AXIS2_PLACEMENT_3D ( 'NONE', #45025, #75968, #5050 ) ;
#67546=CARTESIAN_POINT ( 'NONE',  ( 96.49374645304573050, 226.5177522451418781, -10.00000000000009592 ) ) ;
#67547=B_SPLINE_CURVE_WITH_KNOTS ( 'NONE', 3,
 ( #33197, #64098, #95044, #44278, #76210, #51384, #97517, #29587, #13407, #98004, #67080, #28089, #14873, #13886, #58959, #98513, #67581, #21492, #36178, #21981, #74223, #29104, #52875, #6786, #83826, #52382, #59969, #82838, #53375, #75208, #44768, #28584, #89931, #82350, #5785, #37666, #12918, #20509, #60463, #36673, #59463, #68576 ),
 .UNSPECIFIED., .F., .F.,
 ( 4, 2, 2, 2, 2, 2, 2, 2, 2, 2, 2, 2, 2, 2, 2, 2, 2, 2, 2, 2, 4 ),
 ( 0.002284396617591029702, 0.002715654238588044358, 0.002931283049086530652, 0.003146911859585016947, 0.003254726264834252071, 0.003362540670083487629, 0.003578169480582080175, 0.004009427101579153378, 0.004871942343573404735, 0.005734457585567655225, 0.006596972827561904847, 0.007028230448559109021, 0.007459488069556312329, 0.007567302474805549621, 0.007621209677430168701, 0.007675116880054787781, 0.007782931285304025074, 0.007890745690553263234, 0.008322003311550044136, 0.008753260932546826772, 0.009184518553543607675 ),
 .UNSPECIFIED. ) ;
#67550=CARTESIAN_POINT ( 'NONE',  ( 155.4406061314905969, 279.7141320257344432, -1.823194431127334258 ) ) ;
#67552=CARTESIAN_POINT ( 'NONE',  ( 11.92112666437810908, 171.5643266524160140, 9.188101187500095079 ) ) ;
#67554=CARTESIAN_POINT ( 'NONE',  ( 194.0768453189403431, 272.9027882872081818, 14.29780024873114819 ) ) ;
#67558=CARTESIAN_POINT ( 'NONE',  ( 43.61180991440864574, 205.1744531367911293, 4.594050593750047540 ) ) ;
#67559=CARTESIAN_POINT ( 'NONE',  ( 163.8111161534324935, 246.9178193081252743, -7.110480325054721717 ) ) ;
#67562=CARTESIAN_POINT ( 'NONE',  ( 164.9971748156432056, 244.8635054444190757, -1.825016704039769788 ) ) ;
#67564=CARTESIAN_POINT ( 'NONE',  ( 23.90999230191042102, 174.6115022471901739, -5.000000000000041744 ) ) ;
#67565=CARTESIAN_POINT ( 'NONE',  ( 207.5792673731680793, 271.1091576421853233, 2.359198794924813214 ) ) ;
#67567=CARTESIAN_POINT ( 'NONE',  ( 133.4890956248536895, 254.0024278399161233, 9.188101187500095079 ) ) ;
#67569=CARTESIAN_POINT ( 'NONE',  ( 165.0777597283848195, 244.7239282812269039, 1.811418920707685842 ) ) ;
#67570=EDGE_CURVE ( 'NONE', #14773, #50052, #9848, .T. ) ;
#67573=CARTESIAN_POINT ( 'NONE',  ( 157.8849654228661166, 257.1822134667773980, 17.43614750057631468 ) ) ;
#67574=CARTESIAN_POINT ( 'NONE',  ( 187.9901615146041536, 289.1405255857209795, 14.44262214775099373 ) ) ;
#67576=ORIENTED_EDGE ( 'NONE', *, *, #91951, .T. ) ;
#67578=CARTESIAN_POINT ( 'NONE',  ( 208.3482402183368833, 269.7772576047121902, -1.475194656411285443 ) ) ;
#67579=CARTESIAN_POINT ( 'NONE',  ( 189.3775153017087973, 300.6355170167246911, -1.634152055493470757 ) ) ;
#67580=CARTESIAN_POINT ( 'NONE',  ( 169.5420174322075013, 266.0148534173676467, -17.05181222767901872 ) ) ;
#67581=CARTESIAN_POINT ( 'NONE',  ( 194.7603117279403477, 271.6192734837231910, -13.48552198304586547 ) ) ;
#67585=CARTESIAN_POINT ( 'NONE',  ( 169.5727729373952002, 284.0798650663272156, -11.84966624384599676 ) ) ;
#67590=CARTESIAN_POINT ( 'NONE',  ( 181.8958890403558541, 295.0801465899038476, 4.827918899673129260 ) ) ;
#67592=CARTESIAN_POINT ( 'NONE',  ( 201.2535035105529744, 282.0657020489176716, -18.08976065250591958 ) ) ;
#67593=CIRCLE ( 'NONE', #12593, 14.82106496071134671 ) ;
#67597=ORIENTED_EDGE ( 'NONE', *, *, #30639, .F. ) ;
#67601=VERTEX_POINT ( 'NONE', #21089 ) ;
#67602=CARTESIAN_POINT ( 'NONE',  ( 165.5298684834693574, 269.3554679133272884, -17.63324793928101997 ) ) ;
#67605=CARTESIAN_POINT ( 'NONE',  ( 163.9704062730716032, 246.6419207277664327, 7.317582738093436845 ) ) ;
#67608=CARTESIAN_POINT ( 'NONE',  ( 93.32751462011536603, 218.5643266524159856, -9.188101187500093303 ) ) ;
#67609=CARTESIAN_POINT ( 'NONE',  ( 155.5009445773975187, 261.3114586974326130, 17.03375350714145142 ) ) ;
#67610=CARTESIAN_POINT ( 'NONE',  ( 181.1363957779798284, 271.6931546333026972, -17.04292735804997605 ) ) ;
#67614=ORIENTED_EDGE ( 'NONE', *, *, #25360, .T. ) ;
#67615=B_SPLINE_CURVE_WITH_KNOTS ( 'NONE', 3,
 ( #3385, #34257, #65153, #96100, #95106, #87537, #18069, #26659, #11486, #80915, #57541, #88520, #49957, #98064, #44829, #60517, #60026, #91473, #59019, #6349, #4870, #12469, #13946, #83886, #12977, #5848, #68134, #66647, #90990, #67639, #37236, #35750, #75762, #22035, #83380, #74776, #43838, #14448, #28641, #99062, #89989, #43338, #36236, #29644, #21551, #82412, #52433, #5355, #52933, #74286 ),
 .UNSPECIFIED., .F., .F.,
 ( 4, 2, 2, 2, 2, 2, 2, 2, 2, 2, 2, 2, 2, 2, 2, 2, 2, 2, 2, 2, 2, 2, 2, 2, 4 ),
 ( 0.0005071336019138968695, 0.0009528387457653599620, 0.001175691317691181063, 0.001287117603654161328, 0.001398543889617141593, 0.001509970175580121858, 0.001621396461543102123, 0.001844249033469137896, 0.002289954177321128562, 0.003181364465025150225, 0.004072774752729171888, 0.004964185040433193551, 0.005409890184285204816, 0.005632742756211172284, 0.005744169042174153417, 0.005799882185155722479, 0.005855595328137289807, 0.005911308471118858002, 0.005967021614100427064, 0.006078447900063561719, 0.006301300471989755569, 0.006747005615842055666, 0.007192710759694355763, 0.007415563331620505377, 0.007638415903546654992 ),
 .UNSPECIFIED. ) ;
#67622=CARTESIAN_POINT ( 'NONE',  ( 190.6556843249743167, 294.0696558316880100, -13.68617225801477666 ) ) ;
#67626=CARTESIAN_POINT ( 'NONE',  ( 164.7820965459765148, 264.9732998066323262, -16.63464453842744462 ) ) ;
#67629=B_SPLINE_CURVE_WITH_KNOTS ( 'NONE', 3,
 ( #51992, #68669, #13017, #29199, #37767, #90031, #99594, #92034, #91030, #28186, #60067, #12509, #43380, #97620, #5890, #74324, #35790, #90544, #20605, #75809, #51486, #99103, #6394, #59060, #82455, #43877, #5399, #21594, #36283, #98106, #28688, #37279, #68176, #29687, #60559, #91516, #22083, #53957, #38767, #92514, #100102, #86440, #31164, #31657, #70162, #62053, #3184, #93004, #62554, #93517 ),
 .UNSPECIFIED., .F., .F.,
 ( 4, 2, 2, 2, 2, 2, 2, 2, 2, 2, 2, 2, 2, 2, 2, 2, 2, 2, 2, 2, 2, 2, 2, 2, 4 ),
 ( 0.0004205494687147382340, 0.0008747062255947330497, 0.001101784604034729970, 0.001328862982474727106, 0.001442402171694725458, 0.001555941360914724243, 0.001669480550134722595, 0.001783019739354720946, 0.002010098117794719384, 0.002237176496234717822, 0.003145490009994790070, 0.004053803523754863185, 0.004962117037514935866, 0.005416273794394934477, 0.005643352172834971078, 0.005756891362054951215, 0.005813660956664978147, 0.005870430551275005078, 0.005927200145885032009, 0.005983969740495058941, 0.006097508929715112803, 0.006324587308155201447, 0.006778744065035404755, 0.007232900821915607195, 0.007687057578795810503 ),
 .UNSPECIFIED. ) ;
#67631=ORIENTED_EDGE ( 'NONE', *, *, #68937, .F. ) ;
#67633=CARTESIAN_POINT ( 'NONE',  ( 165.4602035580446397, 282.3930620430364229, 8.860554159259999452 ) ) ;
#67634=CARTESIAN_POINT ( 'NONE',  ( 168.4809247738020019, 252.9187805847961670, 12.05003015331094041 ) ) ;
#67636=CARTESIAN_POINT ( 'NONE',  ( 162.8037981520209314, 248.6625452659484381, 9.809699077002424161 ) ) ;
#67638=CARTESIAN_POINT ( 'NONE',  ( 188.1792557714354928, 260.7783204226367388, 2.818005635731814618 ) ) ;
#67639=CARTESIAN_POINT ( 'NONE',  ( 161.2587810186207662, 281.3878282502170123, -6.584893775719714348 ) ) ;
#67641=( BOUNDED_CURVE ( )  B_SPLINE_CURVE ( 2, ( #9005, #16601, #39877, #87078, #47499, #8023, #71326, #31298, #94147 ),
 .UNSPECIFIED., .F., .T. ) 
 B_SPLINE_CURVE_WITH_KNOTS ( ( 3, 2, 2, 2, 3 ),
 ( 0.4637096774193548154, 0.4650537634408601906, 0.4677419354838709409, 0.4704301075268817467, 0.4717741935483871218 ),
 .UNSPECIFIED. ) 
 CURVE ( )  GEOMETRIC_REPRESENTATION_ITEM ( )  RATIONAL_B_SPLINE_CURVE ( ( 0.9330127018922194093, 0.9330127018922194093, 1.000000000000000000, 0.8660254037844387076, 1.000000000000000000, 0.8660254037844387076, 1.000000000000000000, 0.9330127018922194093, 0.9330127018922194093 ) ) 
 REPRESENTATION_ITEM ( '' )  );
#67643=FACE_OUTER_BOUND ( 'NONE', #84358, .T. ) ;
#67645=ORIENTED_EDGE ( 'NONE', *, *, #89260, .F. ) ;
#67646=CARTESIAN_POINT ( 'NONE',  ( 95.28491933047783391, 232.4865022471902876, -10.00000000000009592 ) ) ;
#67652=CARTESIAN_POINT ( 'NONE',  ( -7.501470784735642106, 173.1427522451419350, -10.00000000000009415 ) ) ;
#67653=CARTESIAN_POINT ( 'NONE',  ( 192.7865293790353860, 266.9527545350466653, -11.24613748226589927 ) ) ;
#67654=CARTESIAN_POINT ( 'NONE',  ( 171.3024615537961495, 279.7431976243712484, -14.91927184813412843 ) ) ;
#67655=CARTESIAN_POINT ( 'NONE',  ( 163.3482521698857113, 247.7195232446219677, -7.972463205267773745 ) ) ;
#67658=CARTESIAN_POINT ( 'NONE',  ( 161.0985561068035850, 273.0316086281096659, 15.84788186387147135 ) ) ;
#67659=CARTESIAN_POINT ( 'NONE',  ( -7.619092152155812592, 178.6589784336661637, -6.496448406907675876E-16 ) ) ;
#67660=CARTESIAN_POINT ( 'NONE',  ( 108.2753003872444424, 239.9865022471903444, -10.00000000000009592 ) ) ;
#67661=CARTESIAN_POINT ( 'NONE',  ( 22.44857442947622417, 183.7677522451418497, 10.00000000000009592 ) ) ;
#67664=ORIENTED_EDGE ( 'NONE', *, *, #34312, .F. ) ;
#67668=CARTESIAN_POINT ( 'NONE',  ( 175.5066696105806443, 290.9053867346144102, 2.574525986029098323 ) ) ;
#67673=CARTESIAN_POINT ( 'NONE',  ( 149.6148422561466305, 277.4437614652936190, 3.137689077364430368 ) ) ;
#67674=CARTESIAN_POINT ( 'NONE',  ( 12.43489537816885537, 187.1744531367911293, 4.594050593750047540 ) ) ;
#67675=CARTESIAN_POINT ( 'NONE',  ( 123.8009570636627785, 230.0327760586659736, 1.948934522072303157E-15 ) ) ;
#67676=CARTESIAN_POINT ( 'NONE',  ( 48.88270317314112390, 187.4824982072973967, 3.021315404115420679E-15 ) ) ;
#67677=CARTESIAN_POINT ( 'NONE',  ( 183.7975612849717777, 256.6346208101135176, -2.981236333899912161 ) ) ;
#67682=CARTESIAN_POINT ( 'NONE',  ( 154.8679462054080318, 262.4078440388265676, 17.98338675682672871 ) ) ;
#67683=CARTESIAN_POINT ( 'NONE',  ( 184.4117451362204179, 274.3934482926966894, 16.89443952929603654 ) ) ;
#67685=EDGE_CURVE ( 'NONE', #99270, #81649, #95650, .T. ) ;
#67686=EDGE_CURVE ( 'NONE', #15116, #42801, #85957, .T. ) ;
#67688=CARTESIAN_POINT ( 'NONE',  ( 187.9021647126450318, 299.0900879367926564, -0.5875642311020390363 ) ) ;
#67690=CARTESIAN_POINT ( 'NONE',  ( 164.9483336881469882, 253.3134267730691249, -13.01688559776908427 ) ) ;
#67691=CARTESIAN_POINT ( 'NONE',  ( 45.32607884611513072, 203.6427522451419065, 10.00000000000009415 ) ) ;
#67695=CARTESIAN_POINT ( 'NONE',  ( 92.54224522822943300, 233.4244531367911009, -4.594050593750046652 ) ) ;
#67697=CARTESIAN_POINT ( 'NONE',  ( 150.6533415055477008, 269.7077535128032082, 14.84621632544246062 ) ) ;
#67700=CARTESIAN_POINT ( 'NONE',  ( 195.9920715006079490, 291.1787696107118677, 15.99608784761372071 ) ) ;
#67701=CARTESIAN_POINT ( 'NONE',  ( 151.9591939046548532, 267.4459508103639109, 16.94431124488332685 ) ) ;
#67702=B_SPLINE_CURVE_WITH_KNOTS ( 'NONE', 3,
 ( #82160, #66410, #73040, #51193, #81652, #89278, #41603, #27426, #74027, #43084 ),
 .UNSPECIFIED., .F., .F.,
 ( 4, 2, 2, 2, 4 ),
 ( 1.223810221527376531E-16, 0.0004261671925493324634, 0.0008523343850985425204, 0.001278501577647752577, 0.001704668770196962526 ),
 .UNSPECIFIED. ) ;
#67703=CARTESIAN_POINT ( 'NONE',  ( 202.4098895269932257, 271.6205993907875040, -9.777904950607410939 ) ) ;
#67704=CARTESIAN_POINT ( 'NONE',  ( 151.3898985249405200, 268.4319993325432847, -14.65018536945715510 ) ) ;
#67705=CARTESIAN_POINT ( 'NONE',  ( 173.3835669379080002, 267.7164584622601069, -16.42089471915695142 ) ) ;
#67707=CARTESIAN_POINT ( 'NONE',  ( 192.7705129102570822, 296.7586727687594816, -13.39629674907774692 ) ) ;
#67708=CARTESIAN_POINT ( 'NONE',  ( 7.197458387703633775, 163.4155109091896065, 2.679491924311254714 ) ) ;
#67709=ORIENTED_EDGE ( 'NONE', *, *, #16914, .T. ) ;
#67711=CARTESIAN_POINT ( 'NONE',  ( -22.42236680055709641, 157.8615022471902591, 0.000000000000000000 ) ) ;
#67712=CARTESIAN_POINT ( 'NONE',  ( 192.5143468344189728, 297.2023654272867361, -12.06830393602581530 ) ) ;
#67714=EDGE_CURVE ( 'NONE', #90614, #12230, #6698, .T. ) ;
#67718=CARTESIAN_POINT ( 'NONE',  ( 198.3150362131025588, 287.1552767044814800, 18.53472937702030521 ) ) ;
#67719=CARTESIAN_POINT ( 'NONE',  ( 157.5665571574053274, 268.7536433892211676, 15.66352472898817005 ) ) ;
#67721=CARTESIAN_POINT ( 'NONE',  ( 143.4214980241629291, 253.6115022471902591, 10.00000000000009592 ) ) ;
#67723=CARTESIAN_POINT ( 'NONE',  ( 191.1741556875616936, 299.0312637876858730, -7.234752218208361896 ) ) ;
#67724=AXIS2_PLACEMENT_3D ( 'NONE', #42736, #89896, #73673 ) ;
#67726=CARTESIAN_POINT ( 'NONE',  ( 196.3812503439841350, 265.2916093225964005, -4.467972469483993514 ) ) ;
#67729=CARTESIAN_POINT ( 'NONE',  ( 181.5366145304931251, 290.8356853596638416, -11.02968432880147276 ) ) ;
#67730=ORIENTED_EDGE ( 'NONE', *, *, #70803, .F. ) ;
#67732=CARTESIAN_POINT ( 'NONE',  ( 50.22809564179084418, 188.2592609112380160, 2.679491924311254714 ) ) ;
#67733=CARTESIAN_POINT ( 'NONE',  ( 205.5135663444060583, 274.6870567772484151, 11.64894633698279591 ) ) ;
#67734=CARTESIAN_POINT ( 'NONE',  ( 190.6351135318297167, 278.8567387100862902, -16.51791015838286469 ) ) ;
#67736=CARTESIAN_POINT ( 'NONE',  ( 201.3505934466285510, 281.8975373467312693, -16.83770227898004279 ) ) ;
#67741=CARTESIAN_POINT ( 'NONE',  ( 164.3917948186382034, 274.8648391023518798, 14.67700265856982789 ) ) ;
#67746=CARTESIAN_POINT ( 'NONE',  ( 182.7510761219226367, 296.3781783941799972, 0.2738238006057779894 ) ) ;
#67748=CARTESIAN_POINT ( 'NONE',  ( 174.3158243945931929, 257.3296975315241184, -11.92724987409102866 ) ) ;
#67749=CARTESIAN_POINT ( 'NONE',  ( 165.8580863246405102, 274.0275451967436879, -15.18278219619561220 ) ) ;
#67750=CARTESIAN_POINT ( 'NONE',  ( 165.0604371780248982, 244.7539318185670822, -1.421758703131883017 ) ) ;
#67752=CARTESIAN_POINT ( 'NONE',  ( 156.5291010833105645, 261.3563040595462894, -17.73323587247505984 ) ) ;
#67754=CARTESIAN_POINT ( 'NONE',  ( 170.4100357732785938, 288.8733093880243814, -4.275907419887600369 ) ) ;
#67756=CARTESIAN_POINT ( 'NONE',  ( 178.0778109109441516, 255.4644557467126162, 4.928885342270551639 ) ) ;
#67757=CARTESIAN_POINT ( 'NONE',  ( 106.6962611473900893, 244.6589784336661069, -6.496448406907675876E-16 ) ) ;
#67758=EDGE_LOOP ( 'NONE', ( #24999, #51927, #13049, #43025 ) ) ;
#67761=CARTESIAN_POINT ( 'NONE',  ( 191.5084189041053833, 275.1726936830797285, 16.11283378800830590 ) ) ;
#67762=ORIENTED_EDGE ( 'NONE', *, *, #37707, .T. ) ;
#67764=EDGE_CURVE ( 'NONE', #69911, #25397, #24351, .T. ) ;
#67765=EDGE_LOOP ( 'NONE', ( #97253, #56678, #99745, #12290, #44151, #32859, #99532, #54663, #50793, #72753, #53134, #20540, #13197, #78727, #23446, #30990, #54411, #91203, #92072, #38110 ) ) ;
#67768=CARTESIAN_POINT ( 'NONE',  ( 195.7617614321055157, 291.5776783508526364, 16.33009124109666033 ) ) ;
#67775=ADVANCED_FACE ( 'NONE', ( #50706 ), #88284, .T. ) ;
#67776=CARTESIAN_POINT ( 'NONE',  ( 192.0661820761754655, 264.6237416276316026, -7.838450156236553390 ) ) ;
#67779=CARTESIAN_POINT ( 'NONE',  ( 184.3186041294927122, 288.8517029907596907, -13.19130426104491605 ) ) ;
#67780=CARTESIAN_POINT ( 'NONE',  ( 156.9053997192012559, 280.1665077765802039, 5.870242185082841679 ) ) ;
#67782=EDGE_LOOP ( 'NONE', ( #81275, #42824, #91310, #27662, #69226, #41783, #12218, #90615, #74522, #93920, #50522, #49564, #90896, #39255, #46071, #81258, #59458, #25319, #81247, #7313, #4949, #94204, #7300, #75125, #1465, #85973, #45794, #97310, #17772, #49031, #50412, #56402, #69875, #100035, #88184, #15386, #9673, #60104, #89369, #11584, #42313, #33008, #77724, #38923, #64592, #46134, #12950, #11552, #12440, #89963, #92667, #50764, #33621, #66132, #40911, #98919, #93956, #61503, #21269, #42527, #55312, #42689, #99314, #97560, #26135, #77953, #61570, #78228, #30368, #46665, #43451, #94714, #10379, #21685, #45408, #52284, #77519, #38916, #19323, #42180, #52689, #10541, #21397, #52161, #49791, #93295, #83594, #26553, #77071, #67101, #30082, #38729, #49208, #24589, #23637, #63489, #72274, #11315, #43461, #26277, #255, #22979, #11183, #60631, #74688, #84017, #74609, #4476, #60868, #21387, #73393, #64251, #88613, #87346, #89391, #85921, #44430, #78613, #49444, #71002, #70201, #54319, #50408, #42665, #1518, #67342 ) ) ;
#67783=CARTESIAN_POINT ( 'NONE',  ( 204.6487448717501252, 276.1849715073653897, 14.68262965895386607 ) ) ;
#67786=CARTESIAN_POINT ( 'NONE',  ( 173.2829648012871644, 251.6371116567045476, -0.4726387605917980461 ) ) ;
#67787=CARTESIAN_POINT ( 'NONE',  ( 191.7054276324227260, 271.4226667163613911, -14.33086474662383836 ) ) ;
#67790=EDGE_CURVE ( 'NONE', #62928, #2866, #62945, .T. ) ;
#67792=CARTESIAN_POINT ( 'NONE',  ( 146.7232198725432113, 245.5177522451417644, 5.000000000000051514 ) ) ;
#67793=CARTESIAN_POINT ( 'NONE',  ( 191.1548165151656349, 283.2771438751705091, -16.59944851309598235 ) ) ;
#67796=CARTESIAN_POINT ( 'NONE',  ( 77.06204113558260360, 224.4869531367911293, 4.594050593750046652 ) ) ;
#67797=CARTESIAN_POINT ( 'NONE',  ( 159.9470087484377814, 253.6106496594791508, -16.54933891566789939 ) ) ;
#67803=CARTESIAN_POINT ( 'NONE',  ( 161.6755750489535046, 250.6166850027345276, -13.01404233079112061 ) ) ;
#67811=AXIS2_PLACEMENT_3D ( 'NONE', #18533, #39782, #10426 ) ;
#67812=ADVANCED_FACE ( 'NONE', ( #41330 ), #58401, .T. ) ;
#67813=CARTESIAN_POINT ( 'NONE',  ( 20.22912401222880519, 191.6744531367911293, 4.594050593750047540 ) ) ;
#67815=CARTESIAN_POINT ( 'NONE',  ( 196.3021893095863959, 290.6416298092292436, 17.45656988653421138 ) ) ;
#67820=CARTESIAN_POINT ( 'NONE',  ( 47.34706511187656020, 188.9548013555409796, -4.594050593750042211 ) ) ;
#67823=CARTESIAN_POINT ( 'NONE',  ( 171.4669319504922385, 286.6849807880217895, 7.449759704774402636 ) ) ;
#67826=CARTESIAN_POINT ( 'NONE',  ( 205.1793861064249711, 275.2658739283173759, -14.08953480709093675 ) ) ;
#67827=CARTESIAN_POINT ( 'NONE',  ( 199.9617906637654414, 268.0814914357001157, -6.510969352826504242 ) ) ;
#67830=CARTESIAN_POINT ( 'NONE',  ( 179.0370437084304456, 276.4408010370251532, 16.31123546408546687 ) ) ;
#67831=DIRECTION ( 'NONE',  ( -0.8660254037844387076, -0.4999999999999998890, -0.000000000000000000 ) ) ;
#67833=CARTESIAN_POINT ( 'NONE',  ( 163.3268748246386508, 256.0845449802187090, -14.91924337074942208 ) ) ;
#67836=CARTESIAN_POINT ( 'NONE',  ( 97.95516432547988472, 227.3615022471902591, -10.00000000000009592 ) ) ;
#67837=CARTESIAN_POINT ( 'NONE',  ( 200.7583183585857967, 282.9233878912788214, 16.96937806979494212 ) ) ;
#67838=CARTESIAN_POINT ( 'NONE',  ( 162.6022651249607804, 268.1935412368399625, -16.60785439006982855 ) ) ;
#67839=ORIENTED_EDGE ( 'NONE', *, *, #7635, .F. ) ;
#67840=CARTESIAN_POINT ( 'NONE',  ( 61.82584055745639517, 200.3768266524159856, -9.188101187500091527 ) ) ;
#67843=CARTESIAN_POINT ( 'NONE',  ( 190.1693911629507738, 301.2639477917662703, -5.112716700269980485 ) ) ;
#67845=CARTESIAN_POINT ( 'NONE',  ( 190.7405042774493324, 298.2747508605859821, 9.591131971744578877 ) ) ;
#67846=ORIENTED_EDGE ( 'NONE', *, *, #99405, .F. ) ;
#67852=CARTESIAN_POINT ( 'NONE',  ( 116.4326846683273544, 226.4824982072973683, 3.021315404115420679E-15 ) ) ;
#67853=VERTEX_POINT ( 'NONE', #87430 ) ;
#67857=CARTESIAN_POINT ( 'NONE',  ( 155.3943609330853519, 266.5197459419810571, 17.05013864555025549 ) ) ;
#67858=ORIENTED_EDGE ( 'NONE', *, *, #61460, .T. ) ;
#67863=CARTESIAN_POINT ( 'NONE',  ( 161.0109787555256275, 282.6433080515603251, -3.149774697262186507 ) ) ;
#67865=CARTESIAN_POINT ( 'NONE',  ( 162.9383752892161397, 248.4294508267893491, -11.25953730674605957 ) ) ;
#67866=CARTESIAN_POINT ( 'NONE',  ( 164.0741338217690668, 246.4622593432776796, 7.359073626423302983 ) ) ;
#67867=CARTESIAN_POINT ( 'NONE',  ( 198.3523905153085423, 287.0905771551796306, 18.52598547438866206 ) ) ;
#67869=CYLINDRICAL_SURFACE ( 'NONE', #90575, 10.00000000000010658 ) ;
#67871=CARTESIAN_POINT ( 'NONE',  ( 123.7191597644692393, 251.4244531367911293, -4.594050593750046652 ) ) ;
#67873=CARTESIAN_POINT ( 'NONE',  ( 80.01237403692960015, 210.8768266524159856, -9.188101187500091527 ) ) ;
#67875=CARTESIAN_POINT ( 'NONE',  ( 170.1952319857192037, 264.1055084534233401, 17.01733452839312832 ) ) ;
#67879=CARTESIAN_POINT ( 'NONE',  ( 200.6938931563371398, 281.7467196835406753, 16.93566535195513723 ) ) ;
#67882=CARTESIAN_POINT ( 'NONE',  ( 84.80240350195582266, 219.7677522451418497, 10.00000000000009592 ) ) ;
#67883=CARTESIAN_POINT ( 'NONE',  ( 206.8073682671177664, 270.4461261121818438, -4.970999383176901709 ) ) ;
#67884=CARTESIAN_POINT ( 'NONE',  ( -2.233149578380279721, 169.5177522451418781, -10.00000000000009592 ) ) ;
#67885=CARTESIAN_POINT ( 'NONE',  ( 147.2180753513904961, 275.6578090293250511, 0.4909717733184589261 ) ) ;
#67887=CARTESIAN_POINT ( 'NONE',  ( 193.9204722154232741, 294.7668848255750049, 15.43855698596013859 ) ) ;
#67888=CARTESIAN_POINT ( 'NONE',  ( 74.50030963965132003, 220.4865022471902876, -10.00000000000009592 ) ) ;
#67893=CARTESIAN_POINT ( 'NONE',  ( 161.5489325017909437, 250.8360363288196311, -12.69404255266198867 ) ) ;
#67895=CARTESIAN_POINT ( 'NONE',  ( 163.9712236968778711, 260.5412544304000448, -16.17885422200931345 ) ) ;
#67896=CARTESIAN_POINT ( 'NONE',  ( 164.3420876084788347, 246.7786081070618991, 5.291571273027417810 ) ) ;
#67899=CARTESIAN_POINT ( 'NONE',  ( 196.4808189786114951, 290.3322341467384717, -17.84817245450773271 ) ) ;
#67900=CARTESIAN_POINT ( 'NONE',  ( 195.0720061818549880, 279.3691163892412987, 16.41141732502160622 ) ) ;
#67901=CARTESIAN_POINT ( 'NONE',  ( 156.1797501576022569, 269.6359076562748101, -16.17116838778184018 ) ) ;
#67902=CARTESIAN_POINT ( 'NONE',  ( 133.0017827873424494, 259.8464784336661637, 1.353441290958777327E-15 ) ) ;
#67903=ORIENTED_EDGE ( 'NONE', *, *, #84494, .F. ) ;
#67906=CARTESIAN_POINT ( 'NONE',  ( 183.5953950971229744, 289.9057545191589043, -13.74357891376704544 ) ) ;
#67909=EDGE_CURVE ( 'NONE', #35604, #54122, #54458, .T. ) ;
#67911=ORIENTED_EDGE ( 'NONE', *, *, #12126, .T. ) ;
#67913=CARTESIAN_POINT ( 'NONE',  ( 182.2364423096436497, 275.3866057150171969, -16.52884722923822380 ) ) ;
#67916=CARTESIAN_POINT ( 'NONE',  ( 201.6192218642991349, 267.5720127751881705, 0.8431288817150176529 ) ) ;
#67917=CARTESIAN_POINT ( 'NONE',  ( 197.0461256858581294, 265.3860351196537408, 0.8220420341949939980 ) ) ;
#67918=CARTESIAN_POINT ( 'NONE',  ( 147.5498377207569263, 275.0831797495432056, 4.097967709737811326 ) ) ;
#67919=CARTESIAN_POINT ( 'NONE',  ( 186.6116014577160058, 282.5156129276005004, 16.21094600413495357 ) ) ;
#67920=CARTESIAN_POINT ( 'NONE',  ( 157.6921299354026189, 257.5162143285667753, -18.18720974599499840 ) ) ;
#67921=CARTESIAN_POINT ( 'NONE',  ( 196.7445171685907894, 269.9811659379847129, 11.91596940811355765 ) ) ;
#67924=CARTESIAN_POINT ( 'NONE',  ( 205.2615535051069742, 274.5664020556757237, 11.36949175128528111 ) ) ;
#67926=CARTESIAN_POINT ( 'NONE',  ( 198.3449891235413531, 287.1033967417670283, 16.95540786497457120 ) ) ;
#67928=( BOUNDED_CURVE ( )  B_SPLINE_CURVE ( 2, ( #42019, #57210, #34905, #35909, #96765, #89192, #58214, #81560, #59184 ),
 .UNSPECIFIED., .F., .T. ) 
 B_SPLINE_CURVE_WITH_KNOTS ( ( 3, 2, 2, 2, 3 ),
 ( 0.2862903225806451846, 0.2876344086021505597, 0.2903225806451613100, 0.2930107526881720603, 0.2943548387096774355 ),
 .UNSPECIFIED. ) 
 CURVE ( )  GEOMETRIC_REPRESENTATION_ITEM ( )  RATIONAL_B_SPLINE_CURVE ( ( 0.9330127018922194093, 0.9330127018922194093, 1.000000000000000000, 0.8660254037844387076, 1.000000000000000000, 0.8660254037844387076, 1.000000000000000000, 0.9330127018922194093, 0.9330127018922194093 ) ) 
 REPRESENTATION_ITEM ( '' )  );
#67929=EDGE_CURVE ( 'NONE', #46611, #72868, #1404, .T. ) ;
#67930=CARTESIAN_POINT ( 'NONE',  ( 151.9193722952498717, 248.5177522451417644, 5.000000000000051514 ) ) ;
#67931=CARTESIAN_POINT ( 'NONE',  ( 175.4039180538638050, 286.4985578832265105, -12.71199677751706503 ) ) ;
#67932=EDGE_LOOP ( 'NONE', ( #98899, #74379, #81095, #41350 ) ) ;
#67936=CARTESIAN_POINT ( 'NONE',  ( 150.7133245577828689, 269.6038598187387834, -14.58664962216439598 ) ) ;
#67937=CARTESIAN_POINT ( 'NONE',  ( 10.54098545103790840, 167.7048013555410080, 4.594050593750051981 ) ) ;
#67938=CARTESIAN_POINT ( 'NONE',  ( 181.6434012404215821, 276.3923190036793471, -17.32158067431182147 ) ) ;
#67941=CARTESIAN_POINT ( 'NONE',  ( 157.6500260163024620, 257.5891404556457474, -18.23450497588216379 ) ) ;
#67943=CARTESIAN_POINT ( 'NONE',  ( 158.2916163944991865, 282.4761429051572463, -3.043442648455108479 ) ) ;
#67945=CARTESIAN_POINT ( 'NONE',  ( 198.2505066714982149, 285.2670451491296149, 0.000000000000000000 ) ) ;
#67946=CARTESIAN_POINT ( 'NONE',  ( 198.1915864813676933, 287.3690979120270867, 17.02875488965938189 ) ) ;
#67948=CARTESIAN_POINT ( 'NONE',  ( 183.0954089547747685, 295.7244723176602292, 1.069539124438823929 ) ) ;
#67949=CARTESIAN_POINT ( 'NONE',  ( 56.45811372747549228, 216.7365022471903444, 2.944929066748280225E-16 ) ) ;
#67951=CARTESIAN_POINT ( 'NONE',  ( 147.9748066657072627, 274.3471119452502762, 9.387104374042873900 ) ) ;
#67952=CARTESIAN_POINT ( 'NONE',  ( 9.079046938504149011, 185.2369531367911293, -4.594050593750048428 ) ) ;
#67956=CYLINDRICAL_SURFACE ( 'NONE', #1422, 17.82106496071139645 ) ;
#67957=CARTESIAN_POINT ( 'NONE',  ( 185.4027513566571201, 266.5856925186359945, 13.20686768916569243 ) ) ;
#67958=CARTESIAN_POINT ( 'NONE',  ( 171.6154833087297789, 255.2606305366970503, 12.53362356821959978 ) ) ;
#67959=CARTESIAN_POINT ( 'NONE',  ( 163.8257527437161514, 281.4247057528291975, 8.856190409526824681 ) ) ;
#67963=CARTESIAN_POINT ( 'NONE',  ( 190.4750160083620472, 300.7345900314585947, -1.159659205620361400 ) ) ;
#67965=CARTESIAN_POINT ( 'NONE',  ( 196.0051728737935832, 265.8263463907475170, 8.406970388261065352 ) ) ;
#67966=EDGE_LOOP ( 'NONE', ( #647, #55900, #72289, #5075 ) ) ;
#67967=CARTESIAN_POINT ( 'NONE',  ( 185.4084872802253585, 290.9630408421091943, 12.18521566798547795 ) ) ;
#67973=CARTESIAN_POINT ( 'NONE',  ( 202.8151641853381477, 279.3608264160075692, -16.28741359973609448 ) ) ;
#67977=CARTESIAN_POINT ( 'NONE',  ( 186.4055657536957540, 271.9883927876483654, -16.52192294486705038 ) ) ;
#67978=CARTESIAN_POINT ( 'NONE',  ( 149.8622666665893632, 273.0779353264732663, 11.47145096717591528 ) ) ;
#67980=CARTESIAN_POINT ( 'NONE',  ( 150.6533415055477008, 269.7077535128032082, 14.84621632544246062 ) ) ;
#67984=EDGE_CURVE ( 'NONE', #85768, #84087, #13427, .T. ) ;
#67986=CARTESIAN_POINT ( 'NONE',  ( 147.6300909839706321, 274.9441770201837585, 8.328755691084779755 ) ) ;
#67988=CARTESIAN_POINT ( 'NONE',  ( 205.9240884482826175, 273.9760116357041966, 10.27504561427317142 ) ) ;
#67991=CARTESIAN_POINT ( 'NONE',  ( 190.0707697440390689, 301.4347651000360884, 4.271360729158901748 ) ) ;
#67992=CARTESIAN_POINT ( 'NONE',  ( 172.3986314675530309, 263.7922717222033384, -16.89442142407995107 ) ) ;
#67995=CARTESIAN_POINT ( 'NONE',  ( 149.0237174825091415, 274.5263358477994871, 9.114370506038131481 ) ) ;
#67998=ORIENTED_EDGE ( 'NONE', *, *, #56357, .F. ) ;
#68002=CARTESIAN_POINT ( 'NONE',  ( 190.9335643195044838, 299.9403610588350944, -4.692880224846124548 ) ) ;
#68004=CARTESIAN_POINT ( 'NONE',  ( 190.7516742497373059, 300.2554039010641418, 4.342609251298632067 ) ) ;
#68005=CARTESIAN_POINT ( 'NONE',  ( 152.9262073036446168, 265.7710344717137900, 16.19159804214501008 ) ) ;
#68006=CARTESIAN_POINT ( 'NONE',  ( 191.1100977347303456, 299.6345962144299619, 9.508964441650325838 ) ) ;
#68007=CARTESIAN_POINT ( 'NONE',  ( 191.8453338867844877, 298.3611298435110371, -9.039024722281077118 ) ) ;
#68008=CARTESIAN_POINT ( 'NONE',  ( -18.76211276271274997, 171.5217562850347406, 1.224646799147364892E-15 ) ) ;
#68014=ORIENTED_EDGE ( 'NONE', *, *, #30515, .T. ) ;
#68015=CARTESIAN_POINT ( 'NONE',  ( 149.7327968382200538, 271.3021836472514678, -12.62649163920564988 ) ) ;
#68016=DIRECTION ( 'NONE',  ( 0.5000000000000048850, -0.8660254037844358210, 0.000000000000000000 ) ) ;
#68017=CARTESIAN_POINT ( 'NONE',  ( 149.1235161367207240, 273.2503626557173106, 9.887280554828780765 ) ) ;
#68020=CARTESIAN_POINT ( 'NONE',  ( 183.1940556755976104, 284.5769249909878909, -14.99598816525897504 ) ) ;
#68024=VERTEX_POINT ( 'NONE', #28030 ) ;
#68025=CARTESIAN_POINT ( 'NONE',  ( 170.4442219353800283, 255.4737032154624217, -11.62118961212506996 ) ) ;
#68027=ADVANCED_FACE ( 'NONE', ( #60905 ), #84272, .T. ) ;
#68030=CARTESIAN_POINT ( 'NONE',  ( 44.60439100962815218, 189.8927522451418213, -10.00000000000009059 ) ) ;
#68031=CARTESIAN_POINT ( 'NONE',  ( 113.4351080945290278, 245.4869531367911009, 4.594050593750046652 ) ) ;
#68032=CARTESIAN_POINT ( 'NONE',  ( 145.0115229932138163, 242.9824982072973683, 3.021315404115420679E-15 ) ) ;
#68034=CARTESIAN_POINT ( 'NONE',  ( 157.1135969804030310, 258.5182628004787944, 17.19660297500358226 ) ) ;
#68035=CARTESIAN_POINT ( 'NONE',  ( 175.7684342158191555, 253.0281421584272721, -4.824161474433333652 ) ) ;
#68036=CARTESIAN_POINT ( 'NONE',  ( 23.55782238408397689, 196.6589784336661637, -6.496448406907675876E-16 ) ) ;
#68039=CARTESIAN_POINT ( 'NONE',  ( 191.2827847134780654, 298.6246597018299553, 8.274781095337747416 ) ) ;
#68040=CARTESIAN_POINT ( 'NONE',  ( 181.7309266518924744, 267.1772924037041435, 15.05018902152789906 ) ) ;
#68042=CARTESIAN_POINT ( 'NONE',  ( 190.7908437487391780, 300.1875603386860689, -4.317984972589949955 ) ) ;
#68044=CARTESIAN_POINT ( 'NONE',  ( 196.9080397933726942, 269.7016881256661804, 12.39056067425276630 ) ) ;
#68045=CARTESIAN_POINT ( 'NONE',  ( 176.8277677751233625, 285.8241435940994393, -12.06137026359123432 ) ) ;
#68046=CARTESIAN_POINT ( 'NONE',  ( 182.2730873982721391, 262.7650441757560884, 12.77154113705879901 ) ) ;
#68047=CARTESIAN_POINT ( 'NONE',  ( 112.1543725048143614, 228.8927522451418213, -10.00000000000009059 ) ) ;
#68048=ORIENTED_EDGE ( 'NONE', *, *, #81869, .F. ) ;
#68049=CARTESIAN_POINT ( 'NONE',  ( 198.3800612005289281, 267.8743580568481093, -8.018411648243336742 ) ) ;
#68050=CARTESIAN_POINT ( 'NONE',  ( 162.6264071486809542, 248.9697954965390920, 10.36322805486644683 ) ) ;
#68051=CARTESIAN_POINT ( 'NONE',  ( 207.6875671281972870, 270.9215769640275653, -2.211577121115235300 ) ) ;
#68052=CARTESIAN_POINT ( 'NONE',  ( 9.052243966459650792, 176.0333772461660828, 9.188101187500095079 ) ) ;
#68057=CARTESIAN_POINT ( 'NONE',  ( 198.2470831392502646, 277.3477145600038511, -15.34583922742456430 ) ) ;
#68058=CARTESIAN_POINT ( 'NONE',  ( 62.15060008387555257, 200.5643266524159856, -9.188101187500093303 ) ) ;
#68059=CARTESIAN_POINT ( 'NONE',  ( 208.3117541397001844, 269.8404533466799080, 2.895672523916592578 ) ) ;
#68064=CARTESIAN_POINT ( 'NONE',  ( 22.53878541258507795, 170.4865022471901455, 1.119607411625061291E-15 ) ) ;
#68065=CARTESIAN_POINT ( 'NONE',  ( 207.5215400641004351, 271.2091442744748520, 2.886080616848571534 ) ) ;
#68066=CARTESIAN_POINT ( 'NONE',  ( 141.2025682470151366, 243.1423013555409796, -4.594050593750043987 ) ) ;
#68070=CARTESIAN_POINT ( 'NONE',  ( 73.97708595465037718, 203.5177522451417929, 5.000000000000051514 ) ) ;
#68073=B_SPLINE_CURVE_WITH_KNOTS ( 'NONE', 3,
 ( #38451, #21766, #15147, #67365 ),
 .UNSPECIFIED., .F., .F.,
 ( 4, 4 ),
 ( 0.04698075955296258932, 0.04887120950165263489 ),
 .UNSPECIFIED. ) ;
#68075=ORIENTED_EDGE ( 'NONE', *, *, #67139, .T. ) ;
#68077=CARTESIAN_POINT ( 'NONE',  ( 208.3927134385237991, 269.7002277277721873, -0.7867555975313439420 ) ) ;
#68078=ADVANCED_FACE ( 'NONE', ( #33394 ), #7814, .F. ) ;
#68079=CARTESIAN_POINT ( 'NONE',  ( 151.9329737526506960, 268.5275331363711757, -15.02064953801001757 ) ) ;
#68084=CARTESIAN_POINT ( 'NONE',  ( 169.8816400817638623, 284.2167566447287754, -11.81736336128774134 ) ) ;
#68087=CARTESIAN_POINT ( 'NONE',  ( 148.7541592998676947, 273.6883713208891322, -8.831557984469299072 ) ) ;
#68090=CARTESIAN_POINT ( 'NONE',  ( 143.4214980241629291, 253.6115022471902591, 10.00000000000009592 ) ) ;
#68092=CARTESIAN_POINT ( 'NONE',  ( 200.7134601498536028, 283.0010845879393742, -16.98649239173277792 ) ) ;
#68093=DIRECTION ( 'NONE',  ( -0.8660254037844387076, -0.4999999999999998890, -0.000000000000000000 ) ) ;
#68096=ORIENTED_EDGE ( 'NONE', *, *, #93944, .F. ) ;
#68097=CARTESIAN_POINT ( 'NONE',  ( 149.0802055316563326, 272.4325049467973940, 12.84384348890831085 ) ) ;
#68102=CARTESIAN_POINT ( 'NONE',  ( 191.8453338867844877, 298.3611298435110371, -9.039024722281077118 ) ) ;
#68104=CARTESIAN_POINT ( 'NONE',  ( 164.3853877993040840, 245.9231516401292197, 5.995325337583643943 ) ) ;
#68106=EDGE_LOOP ( 'NONE', ( #49225, #9632, #67350, #28384 ) ) ;
#68107=CARTESIAN_POINT ( 'NONE',  ( 92.54224522822943300, 233.4244531367911009, -4.594050593750046652 ) ) ;
#68108=CARTESIAN_POINT ( 'NONE',  ( 198.6807893054935619, 282.8457944317249826, 17.49506086463898313 ) ) ;
#68109=CARTESIAN_POINT ( 'NONE',  ( 178.1262429318011016, 269.1995414919144309, -16.42947538547102226 ) ) ;
#68115=ORIENTED_EDGE ( 'NONE', *, *, #68646, .T. ) ;
#68119=CARTESIAN_POINT ( 'NONE',  ( 208.1757572214753793, 270.0760069187178374, 2.172546422564154867 ) ) ;
#68123=CARTESIAN_POINT ( 'NONE',  ( 165.0818462652269432, 264.4362006198225572, -17.63156621922489720 ) ) ;
#68128=CARTESIAN_POINT ( 'NONE',  ( 167.6010540021560189, 247.4270797612363708, 3.638657435017179864 ) ) ;
#68129=CARTESIAN_POINT ( 'NONE',  ( 188.7930588916510999, 290.9633865388665299, 14.97457979531618832 ) ) ;
#68130=CARTESIAN_POINT ( 'NONE',  ( 200.1482866522123629, 269.8493581831766619, 10.43834433840694587 ) ) ;
#68132=CARTESIAN_POINT ( 'NONE',  ( 203.0398866899141126, 278.9715956204779559, 16.57839218037009132 ) ) ;
#68133=CARTESIAN_POINT ( 'NONE',  ( 187.9395208661097740, 260.6475812410266713, 2.852896766392861494 ) ) ;
#68134=CARTESIAN_POINT ( 'NONE',  ( 161.0824001485583494, 281.2882558135126487, -6.595532366314904138 ) ) ;
#68136=CARTESIAN_POINT ( 'NONE',  ( 192.7720849525608742, 292.1153051028871346, -15.41102863861109107 ) ) ;
#68137=CARTESIAN_POINT ( 'NONE',  ( 170.2269576865593308, 254.8920245254076633, 11.28111190939480046 ) ) ;
#68138=CARTESIAN_POINT ( 'NONE',  ( 194.7198309261459030, 262.9852205752617351, -0.8009190715571888886 ) ) ;
#68140=CARTESIAN_POINT ( 'NONE',  ( 181.4944501622172197, 271.2267610228687431, -15.97090179654585640 ) ) ;
#68142=CARTESIAN_POINT ( 'NONE',  ( 156.0507216674837707, 279.5060275253360373, 7.618106348741741307 ) ) ;
#68144=CARTESIAN_POINT ( 'NONE',  ( 13.28313890609096504, 165.1427522451417929, 1.119607411625061291E-15 ) ) ;
#68147=CARTESIAN_POINT ( 'NONE',  ( 163.4971673378707067, 247.4615946076538648, -7.522761844253225583 ) ) ;
#68149=CARTESIAN_POINT ( 'NONE',  ( 164.7521540125055992, 274.2224693477860455, 15.96929761590263475 ) ) ;
#68150=CARTESIAN_POINT ( 'NONE',  ( -8.674473839076844328, 174.9869531367911293, 4.594050593750046652 ) ) ;
#68152=CARTESIAN_POINT ( 'NONE',  ( 189.1219514243199455, 296.9589831032453162, 8.554710403106881245 ) ) ;
#68153=VERTEX_POINT ( 'NONE', #3027 ) ;
#68157=CARTESIAN_POINT ( 'NONE',  ( 174.3227904276429001, 290.2577864514880162, 2.565156313979267910 ) ) ;
#68158=DIRECTION ( 'NONE',  ( -0.8660254037844387076, -0.4999999999999998890, -0.000000000000000000 ) ) ;
#68160=CARTESIAN_POINT ( 'NONE',  ( 202.3483817376306035, 280.1693173315183003, -17.41571691969629043 ) ) ;
#68163=CARTESIAN_POINT ( 'NONE',  ( 24.28913873611587348, 175.6423013555409796, -4.594050593750043987 ) ) ;
#68164=CARTESIAN_POINT ( 'NONE',  ( 123.0428377395863890, 241.8458772461660544, 9.188101187500095079 ) ) ;
#68167=CARTESIAN_POINT ( 'NONE',  ( 206.6995622243289858, 271.9034532870905991, -6.768494619944537050 ) ) ;
#68171=CARTESIAN_POINT ( 'NONE',  ( 193.9401685343300699, 294.7327698005063326, 14.01047396938887069 ) ) ;
#68172=CARTESIAN_POINT ( 'NONE',  ( 207.8575108622103755, 270.6272257822888037, -6.381720258959569847 ) ) ;
#68173=CARTESIAN_POINT ( 'NONE',  ( 189.8411839564327863, 284.6317981244556563, 16.72185364084435832 ) ) ;
#68175=CARTESIAN_POINT ( 'NONE',  ( 165.0248146787475321, 249.8254979808875760, -10.64519944682263031 ) ) ;
#68176=CARTESIAN_POINT ( 'NONE',  ( 192.6536174980028875, 265.2563178382590650, 7.796075781698757368 ) ) ;
#68177=CARTESIAN_POINT ( 'NONE',  ( 197.0106579294310620, 265.8628023436195917, -7.468568667325064858 ) ) ;
#68178=CARTESIAN_POINT ( 'NONE',  ( 162.2926170091170945, 251.8178718525326190, -12.93660524614211482 ) ) ;
#68180=CARTESIAN_POINT ( 'NONE',  ( 98.17141035282828909, 236.6744531367911293, 4.594050593750047540 ) ) ;
#68182=CARTESIAN_POINT ( 'NONE',  ( 150.8167050463783312, 269.4247995599803289, 14.38040671671637938 ) ) ;
#68183=DIRECTION ( 'NONE',  ( 0.4999999999999998890, -0.8660254037844385966, 0.000000000000000000 ) ) ;
#68185=CARTESIAN_POINT ( 'NONE',  ( 152.2681919351047952, 266.9107505221858219, 15.47691051422547837 ) ) ;
#68186=CARTESIAN_POINT ( 'NONE',  ( 157.5373507488561131, 281.8578703925237505, -3.864990440558811358 ) ) ;
#68188=CARTESIAN_POINT ( 'NONE',  ( 204.1541407990405332, 272.6956988606675623, 11.22829397770025395 ) ) ;
#68189=ADVANCED_FACE ( 'NONE', ( #57178 ), #57678, .T. ) ;
#68191=CARTESIAN_POINT ( 'NONE',  ( 192.9523350703175311, 296.4437475495926719, -13.35611922184540923 ) ) ;
#68192=CARTESIAN_POINT ( 'NONE',  ( 201.0277610203388008, 266.5939165858319484, 3.083042990266529060 ) ) ;
#68195=CARTESIAN_POINT ( 'NONE',  ( 178.7021693527624677, 264.3200711924779398, 15.74069764637753366 ) ) ;
#68196=CARTESIAN_POINT ( 'NONE',  ( 192.9523350703175311, 296.4437475495926719, -13.35611922184540923 ) ) ;
#68198=VERTEX_POINT ( 'NONE', #27300 ) ;
#68199=B_SPLINE_SURFACE_WITH_KNOTS ( 'NONE', 3, 1, ( 
 ( #10675, #87246 ),
 ( #49176, #2080 ),
 ( #93811, #17779 ),
 ( #39537, #93299 ),
 ( #16760, #24371 ),
 ( #48680, #62344 ),
 ( #79613, #85733 ),
 ( #9170, #569 ),
 ( #70460, #78079 ),
 ( #41044, #33471 ),
 ( #8667, #31452 ),
 ( #64365, #56759 ),
 ( #31952, #55243 ),
 ( #47649, #40045 ),
 ( #70985, #32470 ),
 ( #74490, #72991 ),
 ( #3583, #34463 ),
 ( #73974, #43550 ),
 ( #81115, #13179 ),
 ( #11682, #96811 ),
 ( #89712, #27860 ),
 ( #4558, #72497 ),
 ( #18778, #3100 ),
 ( #49656, #65361 ),
 ( #19295, #58737 ),
 ( #81602, #51665 ),
 ( #59227, #42544 ),
 ( #33989, #4059 ),
 ( #50162, #97780 ),
 ( #64875, #20273 ),
 ( #80612, #27369 ),
 ( #51147, #96300 ),
 ( #66360, #58252 ),
 ( #26870, #97293 ) ),
 .UNSPECIFIED., .T., .F., .F.,
 ( 4, 2, 2, 2, 2, 2, 2, 2, 2, 2, 2, 2, 2, 2, 2, 2, 4 ),
 ( 2, 2 ),
 ( 0.000000000000000000, 0.06250000000000000000, 0.1250000000000000000, 0.1875000000000000000, 0.2500000000000000000, 0.3125000000000000000, 0.3750000000000000000, 0.4375000000000000000, 0.5000000000000000000, 0.5625000000000000000, 0.6250000000000000000, 0.6875000000000000000, 0.7500000000000000000, 0.8125000000000000000, 0.8750000000000000000, 0.9375000000000000000, 1.000000000000000000 ),
 ( 0.000000000000000000, 1.000000000000000000 ),
 .UNSPECIFIED. ) ;
#68204=CARTESIAN_POINT ( 'NONE',  ( 169.7329090781420291, 252.3771132214117188, -8.760384215664782204 ) ) ;
#68206=CARTESIAN_POINT ( 'NONE',  ( 142.9884853222707477, 243.3615022471901739, 5.000000000000051514 ) ) ;
#68212=CARTESIAN_POINT ( 'NONE',  ( 185.0613556293041597, 292.4148342362145740, -10.69734790306066152 ) ) ;
#68213=ORIENTED_EDGE ( 'NONE', *, *, #70795, .F. ) ;
#68215=CARTESIAN_POINT ( 'NONE',  ( 159.0816921219542905, 255.7002322326580952, 16.02278834591242784 ) ) ;
#68217=CARTESIAN_POINT ( 'NONE',  ( 153.6331558325334754, 264.5465637013422224, -16.53762606136138658 ) ) ;
#68218=CARTESIAN_POINT ( 'NONE',  ( 200.9061540366740246, 282.6673289856585143, -18.13083321883407351 ) ) ;
#68222=DIRECTION ( 'NONE',  ( -0.4999999999999987788, 0.8660254037844392627, 0.000000000000000000 ) ) ;
#68223=( BOUNDED_CURVE ( )  B_SPLINE_CURVE ( 2, ( #23695, #38902, #16116, #69806, #416, #54590, #47014, #33837, #11534 ),
 .UNSPECIFIED., .F., .T. ) 
 B_SPLINE_CURVE_WITH_KNOTS ( ( 3, 2, 2, 2, 3 ),
 ( 0.8991935483870967527, 0.9005376344086021279, 0.9032258064516128782, 0.9059139784946236285, 0.9072580645161290036 ),
 .UNSPECIFIED. ) 
 CURVE ( )  GEOMETRIC_REPRESENTATION_ITEM ( )  RATIONAL_B_SPLINE_CURVE ( ( 0.9330127018922194093, 0.9330127018922194093, 1.000000000000000000, 0.8660254037844387076, 1.000000000000000000, 0.8660254037844387076, 1.000000000000000000, 0.9330127018922194093, 0.9330127018922194093 ) ) 
 REPRESENTATION_ITEM ( '' )  );
#68227=ORIENTED_EDGE ( 'NONE', *, *, #23716, .F. ) ;
#68229=CARTESIAN_POINT ( 'NONE',  ( 176.5791842843404140, 272.9161298461250453, 17.82309232038752000 ) ) ;
#68231=LINE ( 'NONE', #59116, #71436 ) ;
#68232=CARTESIAN_POINT ( 'NONE',  ( 165.8263255788853030, 274.0082066433705563, -15.18430102088745137 ) ) ;
#68233=B_SPLINE_CURVE_WITH_KNOTS ( 'NONE', 3,
 ( #66910, #28928, #99327, #44093 ),
 .UNSPECIFIED., .F., .F.,
 ( 4, 4 ),
 ( 0.01280637797058834827, 0.01912828568769148890 ),
 .UNSPECIFIED. ) ;
#68234=FACE_OUTER_BOUND ( 'NONE', #7536, .T. ) ;
#68238=CARTESIAN_POINT ( 'NONE',  ( 168.2820353728258738, 287.7095463320123940, -5.019694092131335772 ) ) ;
#68240=CARTESIAN_POINT ( 'NONE',  ( 184.6191043844399644, 285.4259123777357559, -15.07684468139096445 ) ) ;
#68241=CARTESIAN_POINT ( 'NONE',  ( 107.4543804714665072, 232.8458772461660544, 9.188101187500095079 ) ) ;
#68245=CARTESIAN_POINT ( 'NONE',  ( 191.3077102587145646, 274.7514833773715850, 16.90660339326615969 ) ) ;
#68246=ORIENTED_EDGE ( 'NONE', *, *, #91995, .F. ) ;
#68247=EDGE_CURVE ( 'NONE', #29382, #86525, #46035, .T. ) ;
#68248=CARTESIAN_POINT ( 'NONE',  ( 162.8822533913248094, 248.9136777285836217, -9.954654975717463827 ) ) ;
#68249=EDGE_CURVE ( 'NONE', #50641, #93452, #59306, .T. ) ;
#68251=CARTESIAN_POINT ( 'NONE',  ( 147.3103884059524376, 275.4979181286220182, 2.739230376052490090 ) ) ;
#68258=ORIENTED_EDGE ( 'NONE', *, *, #56357, .T. ) ;
#68259=CARTESIAN_POINT ( 'NONE',  ( 165.0538309624641613, 244.7653741195639157, 2.311334310144196547 ) ) ;
#68260=EDGE_CURVE ( 'NONE', #72102, #58450, #8567, .T. ) ;
#68261=B_SPLINE_CURVE_WITH_KNOTS ( 'NONE', 3,
 ( #10875, #64573, #11394, #51347, #42247, #4774, #35657, #34171, #12883, #73183, #96013, #95529, #3775, #72184, #26074, #49365, #88429, #76648, #45239, #22443, #30547, #28545, #44728, #21454, #43741, #75174, #82802, #36142, #60425, #14351, #45725, #29551, #59427, #84782, #91382, #51863, #90405, #21943 ),
 .UNSPECIFIED., .F., .F.,
 ( 4, 2, 2, 2, 2, 2, 2, 2, 2, 2, 2, 2, 2, 2, 2, 2, 2, 2, 4 ),
 ( 0.003224435166570254439, 0.003418643166137364138, 0.003612851165704473403, 0.003709955165488081161, 0.003807059165271688920, 0.004001267164838904003, 0.004389683163973335037, 0.004778099163107765203, 0.005554931161376563953, 0.006331763159645363570, 0.007885427156183113725, 0.007982531155966712810, 0.008079635155750313630, 0.008128187155642150469, 0.008176739155533987308, 0.008273843155317693945, 0.008662259154452636722, 0.009050675153587579500, 0.009439091152722522277 ),
 .UNSPECIFIED. ) ;
#68262=B_SPLINE_CURVE_WITH_KNOTS ( 'NONE', 3,
 ( #92087, #7421, #22635, #71629 ),
 .UNSPECIFIED., .F., .F.,
 ( 4, 4 ),
 ( 0.0007376998311747307935, 0.008666068401041223529 ),
 .UNSPECIFIED. ) ;
#68264=CARTESIAN_POINT ( 'NONE',  ( 196.3956310503436953, 264.1850728776087180, 4.154333235580330630 ) ) ;
#68268=CARTESIAN_POINT ( 'NONE',  ( 157.4827499296481506, 280.1768083929792965, 5.769207439127447046 ) ) ;
#68269=CARTESIAN_POINT ( 'NONE',  ( 155.9200296242932495, 280.3860598674420430, -5.539708607631867565 ) ) ;
#68275=CARTESIAN_POINT ( 'NONE',  ( 173.1431250042722922, 251.5821726865244443, -0.2645228944078902855 ) ) ;
#68276=CARTESIAN_POINT ( 'NONE',  ( 192.8054871723947201, 271.6419448112512214, -14.92314579000926145 ) ) ;
#68279=CARTESIAN_POINT ( 'NONE',  ( 200.3293654959697392, 273.7156512906800572, 13.98704503334941229 ) ) ;
#68280=CARTESIAN_POINT ( 'NONE',  ( 194.3562588153086779, 294.0120802933159325, 14.11474987148825200 ) ) ;
#68281=CARTESIAN_POINT ( 'NONE',  ( 190.1774295428112396, 299.2500249094251217, 7.542682482482700124 ) ) ;
#68284=CARTESIAN_POINT ( 'NONE',  ( 76.62902843369037953, 224.2369531367911293, -4.594050593750048428 ) ) ;
#68285=CARTESIAN_POINT ( 'NONE',  ( 159.6288139302610887, 254.1617792512662675, -15.32287760493869477 ) ) ;
#68286=CARTESIAN_POINT ( 'NONE',  ( 197.4237242065244402, 287.4445287091903083, 17.29625570825889369 ) ) ;
#68288=CARTESIAN_POINT ( 'NONE',  ( 197.3452912936916732, 287.9947459898783109, -17.00996526260133734 ) ) ;
#68289=CARTESIAN_POINT ( 'NONE',  ( 207.2167723318516153, 271.7370174712370954, -6.606038862010207957 ) ) ;
#68291=CARTESIAN_POINT ( 'NONE',  ( 101.6177300921036419, 236.1427522451419065, -10.00000000000009592 ) ) ;
#68293=CARTESIAN_POINT ( 'NONE',  ( 186.9240681684178469, 258.1497295257914857, -0.2642925951357694148 ) ) ;
#68298=CARTESIAN_POINT ( 'NONE',  ( 34.24843087963692767, 181.3923013555409796, 4.594050593750050204 ) ) ;
#68299=CARTESIAN_POINT ( 'NONE',  ( 52.08270766911643079, 207.0024278399160664, -9.188101187500093303 ) ) ;
#68300=CARTESIAN_POINT ( 'NONE',  ( 157.3025066944120454, 258.1910615777721887, 18.21299529665260053 ) ) ;
#68304=CARTESIAN_POINT ( 'NONE',  ( 45.10055139898691579, 196.8458772461660544, 9.188101187500095079 ) ) ;
#68305=EDGE_CURVE ( 'NONE', #42521, #10970, #2888, .T. ) ;
#68307=CARTESIAN_POINT ( 'NONE',  ( -3.078821053925192786, 157.4824982072974251, -4.415768667553308270E-15 ) ) ;
#68308=CARTESIAN_POINT ( 'NONE',  ( 149.6191398986701415, 271.4990432411842676, -11.66821883946526839 ) ) ;
#68312=CARTESIAN_POINT ( 'NONE',  ( 194.9471474500919896, 290.9886311562445371, 16.55118206508679890 ) ) ;
#68313=CARTESIAN_POINT ( 'NONE',  ( 180.1034954954120053, 276.2679041092388275, 16.95561710916604170 ) ) ;
#68318=CARTESIAN_POINT ( 'NONE',  ( 92.83118068642190224, 237.7365022471903728, 2.944929066748280225E-16 ) ) ;
#68319=CARTESIAN_POINT ( 'NONE',  ( 161.5504728662519369, 250.8333683393111926, 12.94300825113363373 ) ) ;
#68320=CARTESIAN_POINT ( 'NONE',  ( 164.8610104253742463, 270.4993528865625194, -17.13915278852090296 ) ) ;
#68321=ORIENTED_EDGE ( 'NONE', *, *, #70925, .F. ) ;
#68322=CARTESIAN_POINT ( 'NONE',  ( 55.22204975783502334, 208.8149278399160664, 9.188101187500093303 ) ) ;
#68324=CARTESIAN_POINT ( 'NONE',  ( 166.5534370075956190, 264.7307956230007449, 16.99907680286884215 ) ) ;
#68325=CARTESIAN_POINT ( 'NONE',  ( 147.4963928429778264, 275.1757489932608109, 4.929816573182678852 ) ) ;
#68327=CARTESIAN_POINT ( 'NONE',  ( 175.1183745746886871, 267.9007702990796247, 17.47926410801357022 ) ) ;
#68332=CARTESIAN_POINT ( 'NONE',  ( 147.6884207308302450, 274.8431469350302336, -8.096293592099874203 ) ) ;
#68334=DIRECTION ( 'NONE',  ( 0.4999999999999998890, -0.8660254037844385966, 0.000000000000000000 ) ) ;
#68335=CARTESIAN_POINT ( 'NONE',  ( 157.1184542243154567, 258.5098498072379698, 16.84490127433854667 ) ) ;
#68336=CIRCLE ( 'NONE', #91023, 5.000000000000116351 ) ;
#68337=EDGE_LOOP ( 'NONE', ( #44187, #14788, #19514, #28521 ) ) ;
#68343=CARTESIAN_POINT ( 'NONE',  ( 205.2564848266901834, 271.9733254596621350, -9.597888780111448526 ) ) ;
#68344=EDGE_CURVE ( 'NONE', #82418, #59756, #21095, .T. ) ;
#68345=CARTESIAN_POINT ( 'NONE',  ( 160.0061168334508750, 253.5082714530983026, -16.02306982074888708 ) ) ;
#68351=CARTESIAN_POINT ( 'NONE',  ( 163.4055107321044318, 247.6203485056908846, -10.24153090796238530 ) ) ;
#68352=CARTESIAN_POINT ( 'NONE',  ( 164.3961040135806968, 245.9045906125373904, 7.095190383188031191 ) ) ;
#68354=CARTESIAN_POINT ( 'NONE',  ( 162.3559333012107118, 263.7644763565641597, -16.88032918853872744 ) ) ;
#68355=CARTESIAN_POINT ( 'NONE',  ( 136.6287848093373043, 243.5643266524160140, 9.188101187500095079 ) ) ;
#68358=CARTESIAN_POINT ( 'NONE',  ( 179.3127290521982218, 257.7669455533229552, 10.17447558847459632 ) ) ;
#68359=CARTESIAN_POINT ( 'NONE',  ( 74.97842782955004282, 214.0958772461660544, -9.188101187500095079 ) ) ;
#68363=DIRECTION ( 'NONE',  ( -0.8660254037844387076, -0.4999999999999998890, -0.000000000000000000 ) ) ;
#68364=ORIENTED_EDGE ( 'NONE', *, *, #20019, .T. ) ;
#68367=ORIENTED_EDGE ( 'NONE', *, *, #69849, .F. ) ;
#68369=CARTESIAN_POINT ( 'NONE',  ( 157.6304115535352537, 270.8650229002738001, -16.00510772102553858 ) ) ;
#68372=FACE_OUTER_BOUND ( 'NONE', #38755, .T. ) ;
#68373=CARTESIAN_POINT ( 'NONE',  ( 171.3751619920873281, 280.2398791927632828, 15.33202389549764888 ) ) ;
#68374=CARTESIAN_POINT ( 'NONE',  ( 193.8365934467825298, 294.9121671145370556, 14.14845633038902584 ) ) ;
#68376=B_SPLINE_CURVE_WITH_KNOTS ( 'NONE', 3,
 ( #12069, #89611, #74389, #81019 ),
 .UNSPECIFIED., .F., .F.,
 ( 4, 4 ),
 ( 0.03433908428602378687, 0.04316694911830618042 ),
 .UNSPECIFIED. ) ;
#68379=CARTESIAN_POINT ( 'NONE',  ( 201.1115987356403991, 282.3114883289032377, -17.53098215541816529 ) ) ;
#68380=ORIENTED_EDGE ( 'NONE', *, *, #37140, .F. ) ;
#68381=CARTESIAN_POINT ( 'NONE',  ( 163.7663664781766215, 260.9532688520450279, -16.55063263794407646 ) ) ;
#68384=CARTESIAN_POINT ( 'NONE',  ( 165.0297293518065658, 244.8071193337670195, 2.517333243890161665 ) ) ;
#68386=CARTESIAN_POINT ( 'NONE',  ( 194.9394717063963753, 279.5944888486219497, 16.67925351014588031 ) ) ;
#68387=CARTESIAN_POINT ( 'NONE',  ( 117.8941025407614802, 227.3262482093457777, 3.021315404115420679E-15 ) ) ;
#68388=CARTESIAN_POINT ( 'NONE',  ( 145.2890388471816721, 248.5643266524159856, -9.188101187500093303 ) ) ;
#68397=CARTESIAN_POINT ( 'NONE',  ( 196.7437068507956042, 265.9214190645141116, 4.435905237238339183 ) ) ;
#68398=CARTESIAN_POINT ( 'NONE',  ( 148.3688939817520236, 276.4429351530926624, -3.884194220488612626 ) ) ;
#68401=CARTESIAN_POINT ( 'NONE',  ( 198.5251006538473746, 266.1771426250413128, 0.5392996383993550191 ) ) ;
#68404=CARTESIAN_POINT ( 'NONE',  ( 186.7936673567182311, 282.2315393728885624, 16.42543875383614349 ) ) ;
#68406=CARTESIAN_POINT ( 'NONE',  ( 164.3706594650489023, 245.9486618633701482, -1.665857659249071698 ) ) ;
#68407=CARTESIAN_POINT ( 'NONE',  ( 177.3702169793795633, 264.4761424787041051, -15.61276723233572916 ) ) ;
#68412=CARTESIAN_POINT ( 'NONE',  ( 148.9719199701866899, 272.6200610409887872, 12.59512981512031438 ) ) ;
#68414=CARTESIAN_POINT ( 'NONE',  ( 32.15758756610207314, 177.8262482093457777, 3.021315404115420679E-15 ) ) ;
#68415=CARTESIAN_POINT ( 'NONE',  ( 159.4889735931715222, 254.4039898200529706, 16.88104032092801887 ) ) ;
#68416=CARTESIAN_POINT ( 'NONE',  ( 176.5750811079351763, 290.0661888821730372, -9.631901365267058424 ) ) ;
#68417=CARTESIAN_POINT ( 'NONE',  ( 138.1351346183474220, 263.8927522451419918, 2.944929066748280225E-16 ) ) ;
#68419=ORIENTED_EDGE ( 'NONE', *, *, #22528, .T. ) ;
#68422=CARTESIAN_POINT ( 'NONE',  ( 150.9003228897357189, 269.2799692068659283, -14.30003212299500781 ) ) ;
#68423=CARTESIAN_POINT ( 'NONE',  ( 0.6624493194153854292, 177.3149278399161233, 9.188101187500093303 ) ) ;
#68426=CARTESIAN_POINT ( 'NONE',  ( 170.1980103241066899, 270.7537944251233739, -16.96031082736039508 ) ) ;
#68428=CARTESIAN_POINT ( 'NONE',  ( 150.1511997935914735, 276.5102290984758611, 3.993493173212648184 ) ) ;
#68429=B_SPLINE_SURFACE_WITH_KNOTS ( 'NONE', 3, 1, ( 
 ( #65950, #3195 ),
 ( #28956, #5158 ),
 ( #29937, #66452 ),
 ( #36535, #98368 ),
 ( #37037, #44622 ),
 ( #83182, #43639 ),
 ( #66937, #19873 ),
 ( #81695, #91276 ),
 ( #97867, #82702 ),
 ( #67946, #75556 ),
 ( #13742, #74578 ),
 ( #90799, #28438 ),
 ( #58827, #29443 ),
 ( #59834, #52237 ),
 ( #21353, #98866 ),
 ( #83686, #6141 ),
 ( #60319, #35550 ),
 ( #59320, #21842 ),
 ( #36037, #90300 ),
 ( #89788, #20869 ),
 ( #60814, #76072 ),
 ( #52725, #14247 ),
 ( #51760, #45132 ),
 ( #20364, #12269 ),
 ( #6651, #13268 ),
 ( #44131, #75065 ),
 ( #43127, #5642 ),
 ( #67436, #37525 ),
 ( #68431, #74070 ),
 ( #99359, #50740 ),
 ( #4659, #97378 ),
 ( #27944, #51236 ),
 ( #82203, #12774 ),
 ( #40016, #1044 ) ),
 .UNSPECIFIED., .T., .F., .F.,
 ( 4, 2, 2, 2, 2, 2, 2, 2, 2, 2, 2, 2, 2, 2, 2, 2, 4 ),
 ( 2, 2 ),
 ( 0.000000000000000000, 0.06250000000000000000, 0.1250000000000000000, 0.1875000000000000000, 0.2500000000000000000, 0.3125000000000000000, 0.3750000000000000000, 0.4375000000000000000, 0.5000000000000000000, 0.5625000000000000000, 0.6250000000000000000, 0.6875000000000000000, 0.7500000000000000000, 0.8125000000000000000, 0.8750000000000000000, 0.9375000000000000000, 1.000000000000000000 ),
 ( 0.000000000000000000, 1.000000000000000000 ),
 .UNSPECIFIED. ) ;
#68430=CARTESIAN_POINT ( 'NONE',  ( 179.3296690506923596, 255.1525901867891548, -3.997749341247230248 ) ) ;
#68431=CARTESIAN_POINT ( 'NONE',  ( 198.2860450010354043, 287.2054909567549430, 18.54284983329501557 ) ) ;
#68432=CARTESIAN_POINT ( 'NONE',  ( 62.88113547221017541, 197.1115022471902023, -5.000000000000041744 ) ) ;
#68434=CARTESIAN_POINT ( 'NONE',  ( 148.3519871123208986, 273.6938162480936398, 8.180046468253793890 ) ) ;
#68435=CARTESIAN_POINT ( 'NONE',  ( 24.58674819472551931, 178.8768266524160140, 9.188101187500098632 ) ) ;
#68437=B_SPLINE_CURVE_WITH_KNOTS ( 'NONE', 3,
 ( #86309, #47734, #24942, #16844, #78668, #71071, #94389, #40636, #35038, #96391, #35545, #19385, #11767, #97374, #82199, #87826, #18365, #26465, #43634, #12261, #51230, #4143, #49260, #96896, #3188, #12769, #80196, #11280, #50244, #4652, #81198, #27466, #74573, #64962, #27940, #19866, #26955, #36032, #88315, #18869 ),
 .UNSPECIFIED., .F., .F.,
 ( 4, 2, 2, 2, 2, 2, 2, 2, 2, 2, 2, 2, 2, 2, 2, 2, 2, 2, 2, 4 ),
 ( 0.003212077463089395204, 0.003408847110664717413, 0.003605616758240039622, 0.003704001582027700509, 0.003802386405815361397, 0.003999156053390615952, 0.004392695348541125061, 0.004786234643691634170, 0.005573313233992653257, 0.006360391824293673210, 0.007934549004895784241, 0.008032933828683409133, 0.008131318652471034025, 0.008155914858417923768, 0.008180511064364815246, 0.008229703476258487180, 0.008328088300045874415, 0.008721627595195399069, 0.009115166890344923722, 0.009508706185494448376 ),
 .UNSPECIFIED. ) ;
#68438=CARTESIAN_POINT ( 'NONE',  ( 192.1640094933931096, 297.8091675017319062, 12.36911124822534447 ) ) ;
#68441=EDGE_CURVE ( 'NONE', #70911, #50641, #87334, .T. ) ;
#68442=CARTESIAN_POINT ( 'NONE',  ( 164.3774690880109119, 245.9368672504194819, -2.805681983503304000 ) ) ;
#68443=CARTESIAN_POINT ( 'NONE',  ( 185.3632523845489288, 266.5794829961192818, 13.21810060833462863 ) ) ;
#68444=CARTESIAN_POINT ( 'NONE',  ( 174.8023382843919080, 257.6605964823669979, 13.01024177398429060 ) ) ;
#68445=CARTESIAN_POINT ( 'NONE',  ( 162.7215588690989989, 280.8608052963692217, 8.891366490498469943 ) ) ;
#68448=CARTESIAN_POINT ( 'NONE',  ( 147.6430623265936219, 274.9217099957185155, 8.258152514891218487 ) ) ;
#68450=CARTESIAN_POINT ( 'NONE',  ( 193.8365934467825298, 294.9121671145370556, 14.14845633038902584 ) ) ;
#68451=VERTEX_POINT ( 'NONE', #91010 ) ;
#68452=CARTESIAN_POINT ( 'NONE',  ( 185.1474448761376834, 290.8322720534641803, 12.15833316867892044 ) ) ;
#68455=CARTESIAN_POINT ( 'NONE',  ( 156.0554652282150983, 271.1402087238444665, 15.46858972464315229 ) ) ;
#68457=VERTEX_POINT ( 'NONE', #59545 ) ;
#68459=CARTESIAN_POINT ( 'NONE',  ( 75.87151652897671283, 214.6115022471902591, 10.00000000000009592 ) ) ;
#68462=CARTESIAN_POINT ( 'NONE',  ( 203.3740894404336927, 278.3927394765486838, -15.19753795879846869 ) ) ;
#68465=CARTESIAN_POINT ( 'NONE',  ( 202.3903227094629926, 279.6965068557100267, 15.56271535450856192 ) ) ;
#68468=CARTESIAN_POINT ( 'NONE',  ( 191.2729698983822288, 299.3524933518466469, 8.871011392605806734 ) ) ;
#68471=CARTESIAN_POINT ( 'NONE',  ( 53.62548896571606605, 191.7677522451418213, -5.000000000000041744 ) ) ;
#68474=ORIENTED_EDGE ( 'NONE', *, *, #99560, .F. ) ;
#68475=CARTESIAN_POINT ( 'NONE',  ( 205.7668501412109663, 274.2483563724483133, 11.09689540819876896 ) ) ;
#68476=CARTESIAN_POINT ( 'NONE',  ( 148.7305541605275607, 275.0381188865328568, -8.045727261058747359 ) ) ;
#68478=CARTESIAN_POINT ( 'NONE',  ( 149.6896757981861583, 271.3768714794653647, 12.49809796062302603 ) ) ;
#68484=CARTESIAN_POINT ( 'NONE',  ( 93.62503730655774348, 214.8615022471902023, 5.000000000000051514 ) ) ;
#68493=VECTOR ( 'NONE', #41911, 1000.000000000000000 ) ;
#68494=CARTESIAN_POINT ( 'NONE',  ( 146.9709166616330549, 276.0859004375172390, 3.755270622130282732 ) ) ;
#68496=CARTESIAN_POINT ( 'NONE',  ( 190.8153366230912411, 300.1451374358846920, 3.771947273125533684 ) ) ;
#68497=CARTESIAN_POINT ( 'NONE',  ( 153.3920560952016956, 264.9641606960921649, 16.50453917291963535 ) ) ;
#68498=CARTESIAN_POINT ( 'NONE',  ( 147.2812597312705805, 275.5483704731282728, -0.2636021916935415432 ) ) ;
#68499=CARTESIAN_POINT ( 'NONE',  ( 146.7818291168261453, 276.4134096722012828, -0.7617065417431535534 ) ) ;
#68502=CARTESIAN_POINT ( 'NONE',  ( 190.0896302098338424, 301.4020978150248311, 3.433521196325825642 ) ) ;
#68504=CARTESIAN_POINT ( 'NONE',  ( 196.9431415128477170, 289.5314680279574304, -16.61413060656005669 ) ) ;
#68507=CARTESIAN_POINT ( 'NONE',  ( 168.2066918328904706, 286.4521719584415678, 3.767673903196911755 ) ) ;
#68509=CARTESIAN_POINT ( 'NONE',  ( 105.4518702730974979, 225.5643266524160140, 9.188101187500095079 ) ) ;
#68510=ORIENTED_EDGE ( 'NONE', *, *, #76717, .F. ) ;
#68511=CARTESIAN_POINT ( 'NONE',  ( -22.42236680055709641, 157.8615022471902591, 0.000000000000000000 ) ) ;
#68517=CARTESIAN_POINT ( 'NONE',  ( 187.7282692072121222, 287.3763760864540586, 16.35809696136310976 ) ) ;
#68518=CARTESIAN_POINT ( 'NONE',  ( 166.2797251853322109, 284.7563794900764265, -8.621111623322635253 ) ) ;
#68520=CARTESIAN_POINT ( 'NONE',  ( 208.1303168694798273, 270.1547119170880364, -0.9257663487928086132 ) ) ;
#68521=( BOUNDED_CURVE ( )  B_SPLINE_CURVE ( 2, ( #90199, #97290, #74973, #5554, #88722, #19292, #67346, #89228, #58733 ),
 .UNSPECIFIED., .F., .T. ) 
 B_SPLINE_CURVE_WITH_KNOTS ( ( 3, 2, 2, 2, 3 ),
 ( 0.1491935483870967805, 0.1505376344086021556, 0.1532258064516129059, 0.1559139784946236562, 0.1572580645161290314 ),
 .UNSPECIFIED. ) 
 CURVE ( )  GEOMETRIC_REPRESENTATION_ITEM ( )  RATIONAL_B_SPLINE_CURVE ( ( 0.9330127018922194093, 0.9330127018922194093, 1.000000000000000000, 0.8660254037844387076, 1.000000000000000000, 0.8660254037844387076, 1.000000000000000000, 0.9330127018922194093, 0.9330127018922194093 ) ) 
 REPRESENTATION_ITEM ( '' )  );
#68522=CARTESIAN_POINT ( 'NONE',  ( 159.2394649670193303, 254.8361514374751664, -16.43133403737800791 ) ) ;
#68524=CARTESIAN_POINT ( 'NONE',  ( 43.73836560584370403, 189.3927522451417929, 10.00000000000009592 ) ) ;
#68525=CARTESIAN_POINT ( 'NONE',  ( 111.5137010038235417, 241.3149278399160949, -9.188101187500095079 ) ) ;
#68526=CARTESIAN_POINT ( 'NONE',  ( 180.7361392967986831, 294.1568954366646267, -3.145899629403025699 ) ) ;
#68527=FACE_OUTER_BOUND ( 'NONE', #35609, .T. ) ;
#68528=CARTESIAN_POINT ( 'NONE',  ( 195.9359860111818250, 291.2759125279654882, 17.49638312768267312 ) ) ;
#68529=CARTESIAN_POINT ( 'NONE',  ( 175.5064957684375884, 253.4785342928385603, -4.458035672056321452 ) ) ;
#68530=CARTESIAN_POINT ( 'NONE',  ( 39.11982377592438809, 184.2048013555409796, 4.594050593750051981 ) ) ;
#68533=CARTESIAN_POINT ( 'NONE',  ( 4.262040950003013862, 173.2677522451418781, 10.00000000000009592 ) ) ;
#68534=CARTESIAN_POINT ( 'NONE',  ( 181.9013721714349856, 266.8816343884801086, 15.77960664470944430 ) ) ;
#68535=DIRECTION ( 'NONE',  ( -0.8660254037844387076, -0.4999999999999998890, -0.000000000000000000 ) ) ;
#68536=CARTESIAN_POINT ( 'NONE',  ( 147.3984236761635884, 275.3454365677582700, 5.108566646342994844 ) ) ;
#68540=CARTESIAN_POINT ( 'NONE',  ( 97.79278455872236009, 237.2677522451419065, -5.000000000000047962 ) ) ;
#68543=CARTESIAN_POINT ( 'NONE',  ( 207.4218731373931632, 271.3817724553659332, -5.249531240730909154 ) ) ;
#68544=CARTESIAN_POINT ( 'NONE',  ( 158.6837034624547016, 282.0065499102733497, -1.619886856338979886 ) ) ;
#68545=CARTESIAN_POINT ( 'NONE',  ( 207.7837159184916231, 270.7550423741513441, -2.369602332675663448 ) ) ;
#68547=CARTESIAN_POINT ( 'NONE',  ( 9.323050453024791295, 170.0643266524160140, 9.188101187500095079 ) ) ;
#68549=CARTESIAN_POINT ( 'NONE',  ( 196.1346637562676278, 273.7134257057076070, 14.83932934806210113 ) ) ;
#68552=CARTESIAN_POINT ( 'NONE',  ( 194.7866383867829256, 274.9940630606773198, -16.01128562500261054 ) ) ;
#68553=CARTESIAN_POINT ( 'NONE',  ( 62.47501251452968773, 213.0024278399160949, -9.188101187500093303 ) ) ;
#68554=CARTESIAN_POINT ( 'NONE',  ( 163.8398374448017591, 246.8680725722146008, -5.948785025486735378 ) ) ;
#68558=VERTEX_POINT ( 'NONE', #91495 ) ;
#68560=CARTESIAN_POINT ( 'NONE',  ( 7.816353548249534100, 181.9865022471903160, 10.00000000000009237 ) ) ;
#68561=CARTESIAN_POINT ( 'NONE',  ( 207.5570596878370679, 271.1476224814971374, 2.444960520848353358 ) ) ;
#68563=CARTESIAN_POINT ( 'NONE',  ( 138.6852480475602931, 257.0024278399161517, 9.188101187500095079 ) ) ;
#68566=LINE ( 'NONE', #45751, #40010 ) ;
#68572=CARTESIAN_POINT ( 'NONE',  ( 62.79092448910137847, 200.3927522451417929, -10.00000000000009237 ) ) ;
#68573=CARTESIAN_POINT ( 'NONE',  ( 208.3055888496142813, 269.8511319423524242, -0.4960542269038109575 ) ) ;
#68575=CARTESIAN_POINT ( 'NONE',  ( 156.6930436047642843, 280.2728101775987284, -5.381237359922138808 ) ) ;
#68576=CARTESIAN_POINT ( 'NONE',  ( 197.4075646047015482, 273.1427705089788560, -14.69744958829762815 ) ) ;
#68578=CARTESIAN_POINT ( 'NONE',  ( 165.5752708168755305, 245.8622137986321832, -1.085626278946311585 ) ) ;
#68579=CARTESIAN_POINT ( 'NONE',  ( -27.42236680055714260, 166.5217562850347406, 1.224646799147364892E-15 ) ) ;
#68581=EDGE_CURVE ( 'NONE', #93085, #57035, #60385, .T. ) ;
#68583=CARTESIAN_POINT ( 'NONE',  ( 26.50806851326369440, 186.1115022471902591, 10.00000000000009592 ) ) ;
#68584=CARTESIAN_POINT ( 'NONE',  ( 40.20209520705726192, 184.0177522451417929, 5.000000000000051514 ) ) ;
#68586=CARTESIAN_POINT ( 'NONE',  ( 163.1096928939807924, 248.1327200311062882, -9.690381021358412283 ) ) ;
#68587=CARTESIAN_POINT ( 'NONE',  ( 153.0308080659177392, 265.5898606369461277, -17.74682723936668438 ) ) ;
#68589=CARTESIAN_POINT ( 'NONE',  ( 190.8462995483115776, 280.9575646962753126, 16.64796827995540696 ) ) ;
#68593=CARTESIAN_POINT ( 'NONE',  ( 149.2561433752359505, 272.1277716627430436, 12.99353668144589946 ) ) ;
#68596=ORIENTED_EDGE ( 'NONE', *, *, #60522, .T. ) ;
#68597=CARTESIAN_POINT ( 'NONE',  ( 191.2111338740054975, 299.4595964878050154, -9.718193530796334301 ) ) ;
#68599=CARTESIAN_POINT ( 'NONE',  ( 204.3951397407346064, 276.6242284793436852, 14.79595971842109137 ) ) ;
#68601=ORIENTED_EDGE ( 'NONE', *, *, #2021, .T. ) ;
#68602=CARTESIAN_POINT ( 'NONE',  ( 97.38683515247240052, 227.0333772461660544, 9.188101187500095079 ) ) ;
#68603=CARTESIAN_POINT ( 'NONE',  ( 155.0006381209259132, 262.1780148993956345, 17.98662963467628728 ) ) ;
#68605=CARTESIAN_POINT ( 'NONE',  ( 181.3429656143923694, 271.2897672401974205, -16.00655333216852938 ) ) ;
#68610=CARTESIAN_POINT ( 'NONE',  ( 159.0836013084991123, 281.9351143348985715, -6.237652159340437485 ) ) ;
#68614=ORIENTED_EDGE ( 'NONE', *, *, #70380, .T. ) ;
#68617=CARTESIAN_POINT ( 'NONE',  ( 167.7068093616764486, 281.0861989796462694, 11.58686271003535850 ) ) ;
#68623=CARTESIAN_POINT ( 'NONE',  ( 201.2356561511845143, 278.8713745403558164, -15.71208516001683364 ) ) ;
#68628=CARTESIAN_POINT ( 'NONE',  ( 202.9685995779611858, 279.0950685203052899, 16.84977534244423580 ) ) ;
#68629=CARTESIAN_POINT ( 'NONE',  ( 186.1008340985782752, 259.4276452379801299, 2.884016300632598284 ) ) ;
#68632=AXIS2_PLACEMENT_3D ( 'NONE', #69664, #54960, #85939 ) ;
#68633=CARTESIAN_POINT ( 'NONE',  ( 161.2799361541916028, 251.3019516699124836, 14.40628917569557110 ) ) ;
#68634=CARTESIAN_POINT ( 'NONE',  ( 194.7648128082431072, 263.0520082674682953, -0.7993879730480621948 ) ) ;
#68636=CARTESIAN_POINT ( 'NONE',  ( 181.4811969836216861, 271.1666789078223019, -15.96325902370808159 ) ) ;
#68639=CARTESIAN_POINT ( 'NONE',  ( 9.458193372709686741, 166.2677522451418213, -5.000000000000041744 ) ) ;
#68642=CARTESIAN_POINT ( 'NONE',  ( 175.0267821627883507, 281.5489919625649122, -14.11785333599694425 ) ) ;
#68643=CARTESIAN_POINT ( 'NONE',  ( 204.2021211322627892, 276.9585465160237732, -15.48642194502425440 ) ) ;
#68644=B_SPLINE_CURVE_WITH_KNOTS ( 'NONE', 3,
 ( #45887, #99134, #70195, #15493, #38297, #804, #22118, #61098, #22619, #100132, #92069, #30719, #45407, #16008, #76338, #6911, #68705, #84948, #92552, #99633, #69207, #23098, #53989, #38799, #54484, #69705, #85463, #63106, #56996, #47889, #57495, #55486, #33209, #10927, #18027, #32202, #88476, #96058, #64619, #33729, #86472, #94052, #25620, #16999, #47401, #86978, #10420, #55981 ),
 .UNSPECIFIED., .F., .F.,
 ( 4, 2, 2, 2, 2, 2, 2, 2, 2, 2, 2, 2, 2, 2, 2, 2, 2, 2, 2, 2, 2, 2, 2, 4 ),
 ( 0.001976462477795229607, 0.002421830707482981737, 0.002644514822326855634, 0.002867198937170729964, 0.002978540994592638290, 0.003089883052014547483, 0.003201225109436455808, 0.003312567166858364567, 0.003535251281702188157, 0.003757935396546011747, 0.004648671855921450088, 0.005539408315296888430, 0.006430144774672326771, 0.006875513004360045075, 0.007320881234047764245, 0.007432223291469675606, 0.007487894320180630420, 0.007543565348891586100, 0.007654907406313499196, 0.007766249463735411425, 0.008211617693423052533, 0.008656985923110694509, 0.008879670037954518966, 0.009102354152798343423 ),
 .UNSPECIFIED. ) ;
#68646=EDGE_CURVE ( 'NONE', #53225, #76651, #91843, .T. ) ;
#68647=CARTESIAN_POINT ( 'NONE',  ( -7.997804718428996651, 172.3149278399160949, -9.188101187500095079 ) ) ;
#68648=CARTESIAN_POINT ( 'NONE',  ( -5.697251193518073187, 177.5177522451419350, 5.000000000000046185 ) ) ;
#68649=CARTESIAN_POINT ( 'NONE',  ( 163.8066603109232346, 248.5069834890703078, 9.830012707353159129 ) ) ;
#68650=VERTEX_POINT ( 'NONE', #77256 ) ;
#68653=CARTESIAN_POINT ( 'NONE',  ( -22.42236680055709641, 157.8615022471902591, 0.000000000000000000 ) ) ;
#68654=CARTESIAN_POINT ( 'NONE',  ( 163.8835510476618254, 277.4261113242017132, -14.47671527678674330 ) ) ;
#68655=CARTESIAN_POINT ( 'NONE',  ( 197.9278932102866122, 265.8241103735087449, -6.306740378884746256 ) ) ;
#68656=CARTESIAN_POINT ( 'NONE',  ( 162.6049147221665123, 249.0070214712401935, -10.34353492225723059 ) ) ;
#68657=CARTESIAN_POINT ( 'NONE',  ( 151.9458057874326755, 277.5688626660769387, 3.700970285374547419 ) ) ;
#68658=CARTESIAN_POINT ( 'NONE',  ( 10.89220085373657199, 189.3464784336661353, 1.353441290958777525E-15 ) ) ;
#68659=CARTESIAN_POINT ( 'NONE',  ( 113.9495709998497688, 236.5958772461660544, -9.188101187500095079 ) ) ;
#68660=CARTESIAN_POINT ( 'NONE',  ( 179.1166397756549316, 291.9316799655679233, -6.147037684395432855 ) ) ;
#68661=CARTESIAN_POINT ( 'NONE',  ( 121.6288370910339722, 229.4824982072973398, 3.021315404115420679E-15 ) ) ;
#68664=CYLINDRICAL_SURFACE ( 'NONE', #68632, 10.00000000000010658 ) ;
#68666=CARTESIAN_POINT ( 'NONE',  ( 161.7767236248226084, 250.4414905302161287, -13.15904643207033153 ) ) ;
#68668=CARTESIAN_POINT ( 'NONE',  ( 165.0391502558331069, 249.6778246878102436, -10.74756611015070717 ) ) ;
#68669=CARTESIAN_POINT ( 'NONE',  ( 196.1190320836150249, 265.9249367091900353, 8.391681110388155673 ) ) ;
#68670=B_SPLINE_CURVE_WITH_KNOTS ( 'NONE', 3,
 ( #56389, #93939, #9300, #40176 ),
 .UNSPECIFIED., .F., .F.,
 ( 4, 4 ),
 ( 0.001557053815687444972, 0.008487571838833373600 ),
 .UNSPECIFIED. ) ;
#68672=CARTESIAN_POINT ( 'NONE',  ( 206.9985020284622408, 270.1150727264914053, 3.388313042214953441 ) ) ;
#68674=ORIENTED_EDGE ( 'NONE', *, *, #29594, .F. ) ;
#68677=CARTESIAN_POINT ( 'NONE',  ( 92.97525793012167128, 233.6744531367911293, 4.594050593750047540 ) ) ;
#68679=CARTESIAN_POINT ( 'NONE',  ( 190.9061255863007318, 299.9878863388391892, 7.497146773253707153 ) ) ;
#68681=CARTESIAN_POINT ( 'NONE',  ( 140.6610420460521311, 252.0177522451418213, -10.00000000000009592 ) ) ;
#68682=CARTESIAN_POINT ( 'NONE',  ( 192.3574160861219298, 277.4804554469715185, 16.46682601177359473 ) ) ;
#68683=CARTESIAN_POINT ( 'NONE',  ( 196.3322077676189394, 290.5896363147520560, 17.46901783180497603 ) ) ;
#68684=CARTESIAN_POINT ( 'NONE',  ( 156.1857201963304362, 277.6936791020598889, 10.39727624116721749 ) ) ;
#68687=CARTESIAN_POINT ( 'NONE',  ( -22.42236680055709641, 157.8615022471902591, 0.000000000000000000 ) ) ;
#68688=VERTEX_POINT ( 'NONE', #7864 ) ;
#68690=CARTESIAN_POINT ( 'NONE',  ( 178.7251872717625929, 280.4929491208731065, 15.86704982540033981 ) ) ;
#68691=CARTESIAN_POINT ( 'NONE',  ( 147.5540328368684300, 275.0759135952944234, -4.750028533202499403 ) ) ;
#68692=CARTESIAN_POINT ( 'NONE',  ( 149.2765980486851731, 272.0923431290771646, -11.40617906909507973 ) ) ;
#68696=CARTESIAN_POINT ( 'NONE',  ( 152.7731995575106509, 275.0936207477257085, 10.86798791317738200 ) ) ;
#68697=CARTESIAN_POINT ( 'NONE',  ( 198.6742831389107096, 286.5330427765190393, 17.60232614297041565 ) ) ;
#68699=CARTESIAN_POINT ( 'NONE',  ( 180.4665312189673330, 261.7265043435623966, -13.29892058382729481 ) ) ;
#68701=CARTESIAN_POINT ( 'NONE',  ( 169.3882425167235795, 252.1626239731313888, -8.756318688425812624 ) ) ;
#68703=CARTESIAN_POINT ( 'NONE',  ( 147.3186123411928747, 255.8615022471902307, -10.00000000000009592 ) ) ;
#68704=VERTEX_POINT ( 'NONE', #70137 ) ;
#68705=CARTESIAN_POINT ( 'NONE',  ( 187.4090223870812792, 278.8944490661542659, 17.04039641662812343 ) ) ;
#68706=B_SPLINE_SURFACE_WITH_KNOTS ( 'NONE', 3, 1, ( 
 ( #78288, #85943 ),
 ( #17474, #9896 ),
 ( #55945, #7887 ),
 ( #16469, #39738 ),
 ( #86942, #64078 ),
 ( #62551, #31159 ),
 ( #94015, #46352 ),
 ( #56471, #32168 ),
 ( #40257, #48384 ),
 ( #71197, #95022 ),
 ( #32672, #1790 ),
 ( #62048, #15970 ),
 ( #47365, #46872 ),
 ( #93514, #93001 ),
 ( #79328, #40754 ),
 ( #47854, #77796 ),
 ( #63571, #94514 ),
 ( #71703, #24071 ),
 ( #1284, #54964 ),
 ( #8872, #24567 ),
 ( #55450, #86437 ),
 ( #70669, #16963 ),
 ( #78791, #70157 ),
 ( #2297, #25068 ),
 ( #33177, #25585 ),
 ( #23554, #38763 ),
 ( #9379, #15454 ),
 ( #54446, #77276 ),
 ( #69668, #274 ),
 ( #8381, #39247 ),
 ( #767, #31654 ),
 ( #44497, #98741 ),
 ( #67307, #21713 ),
 ( #13625, #54087 ) ),
 .UNSPECIFIED., .T., .F., .F.,
 ( 4, 2, 2, 2, 2, 2, 2, 2, 2, 2, 2, 2, 2, 2, 2, 2, 4 ),
 ( 2, 2 ),
 ( 0.000000000000000000, 0.06250000000000000000, 0.1250000000000000000, 0.1875000000000000000, 0.2500000000000000000, 0.3125000000000000000, 0.3750000000000000000, 0.4375000000000000000, 0.5000000000000000000, 0.5625000000000000000, 0.6250000000000000000, 0.6875000000000000000, 0.7500000000000000000, 0.8125000000000000000, 0.8750000000000000000, 0.9375000000000000000, 1.000000000000000000 ),
 ( 0.000000000000000000, 1.000000000000000000 ),
 .UNSPECIFIED. ) ;
#68709=ORIENTED_EDGE ( 'NONE', *, *, #2322, .F. ) ;
#68710=CARTESIAN_POINT ( 'NONE',  ( 167.2398491818434536, 249.6619807853312238, 6.963124153055272991 ) ) ;
#68712=CARTESIAN_POINT ( 'NONE',  ( 184.9360691488573423, 292.3413084151380303, -10.69521170824177503 ) ) ;
#68713=VECTOR ( 'NONE', #48149, 1000.000000000000000 ) ;
#68717=CARTESIAN_POINT ( 'NONE',  ( 190.8509455208771044, 278.0625209715795449, -16.97381849757700678 ) ) ;
#68718=CARTESIAN_POINT ( 'NONE',  ( 192.7905631387375820, 296.7239447543280448, -13.53553090723447205 ) ) ;
#68719=CARTESIAN_POINT ( 'NONE',  ( 153.3506059258413643, 265.0359544954067132, -16.39100908615009899 ) ) ;
#68722=B_SPLINE_CURVE_WITH_KNOTS ( 'NONE', 3,
 ( #44714, #60412, #7730, #69019, #21443, #99949, #84280, #14338, #45227, #13838, #30028, #67532, #82792, #51851, #91368, #91879, #53324, #76164, #52329, #83270, #21931, #84771, #20969, #46206, #38106, #75647, #138, #6741, #15307, #14825, #61420, #6233, #45714, #13358, #52821, #37618, #30533, #83777, #38618, #68529, #22432, #99452, #37128, #75160, #68035, #69527, #76637, #92372, #98956, #22920 ),
 .UNSPECIFIED., .F., .F.,
 ( 4, 2, 2, 2, 2, 2, 2, 2, 2, 2, 2, 2, 2, 2, 2, 2, 2, 2, 2, 2, 2, 2, 2, 2, 4 ),
 ( 0.0006152650805149372047, 0.001045760051675842604, 0.001261007537256295195, 0.001368631280046588711, 0.001476255022836882227, 0.001691502508417469476, 0.001906749993998056725, 0.002337244965159098950, 0.003198234907481184268, 0.004059224849803269586, 0.004920214792125354904, 0.005350709763286351159, 0.005565957248866859261, 0.005673580991657032647, 0.005727392863052129315, 0.005781204734447225983, 0.005835016605842323519, 0.005888828477237420186, 0.005996452220027617859, 0.006211699705608018408, 0.006642194676768819507, 0.006857442162349277302, 0.007072689647929735098, 0.007287937133510192893, 0.007503184619090650688 ),
 .UNSPECIFIED. ) ;
#68723=B_SPLINE_CURVE_WITH_KNOTS ( 'NONE', 3,
 ( #52888, #6300, #45772, #77714 ),
 .UNSPECIFIED., .F., .F.,
 ( 4, 4 ),
 ( 0.04263745385576789282, 0.04887120950165272509 ),
 .UNSPECIFIED. ) ;
#68725=VERTEX_POINT ( 'NONE', #55428 ) ;
#68726=CARTESIAN_POINT ( 'NONE',  ( 162.7395313153677989, 249.4784413565320165, 10.93946270999009052 ) ) ;
#68729=CARTESIAN_POINT ( 'NONE',  ( 198.1322097300599125, 286.5433749449028937, 17.04145067767304056 ) ) ;
#68730=CARTESIAN_POINT ( 'NONE',  ( 164.0781508658037637, 275.4055464209769752, 15.63836535835214114 ) ) ;
#68731=CARTESIAN_POINT ( 'NONE',  ( 183.3634088509504352, 284.6525016221286251, -16.42631288611494256 ) ) ;
#68733=FACE_OUTER_BOUND ( 'NONE', #11220, .T. ) ;
#68734=CARTESIAN_POINT ( 'NONE',  ( 197.4191597201339619, 273.2215227944986395, -13.36937406163023390 ) ) ;
#68737=CARTESIAN_POINT ( 'NONE',  ( 188.2892141557378807, 278.5232933803065976, -17.80357329707993941 ) ) ;
#68738=CARTESIAN_POINT ( 'NONE',  ( 165.8190036485819689, 266.0137150170749010, 17.53662559932599407 ) ) ;
#68739=CARTESIAN_POINT ( 'NONE',  ( 186.8225631894460150, 287.0909073165248628, -15.81189067252249458 ) ) ;
#68740=CARTESIAN_POINT ( 'NONE',  ( 115.2486091055264410, 237.3458772461660544, 9.188101187500095079 ) ) ;
#68742=CARTESIAN_POINT ( 'NONE',  ( 148.0508535842240008, 274.6303860046891145, -6.128032407862696651 ) ) ;
#68743=CARTESIAN_POINT ( 'NONE',  ( 160.0166746459236435, 283.6086068001695253, 2.232576205374148248 ) ) ;
#68744=CARTESIAN_POINT ( 'NONE',  ( 188.0633326902639624, 273.6994922365734055, 15.81873844000643992 ) ) ;
#68747=CARTESIAN_POINT ( 'NONE',  ( 163.5466103691548483, 248.4877639346904630, -9.576932048953096910 ) ) ;
#68749=CARTESIAN_POINT ( 'NONE',  ( 146.8833996772869170, 276.2374843009295660, 2.657187058495397824 ) ) ;
#68756=ORIENTED_EDGE ( 'NONE', *, *, #81856, .T. ) ;
#68757=CARTESIAN_POINT ( 'NONE',  ( 191.5633020375963156, 267.7816122967149113, -12.23337175531920451 ) ) ;
#68759=CARTESIAN_POINT ( 'NONE',  ( 192.9427994460758953, 263.5453600104565339, 4.477423407611991202 ) ) ;
#68760=CARTESIAN_POINT ( 'NONE',  ( -3.078821053925192786, 157.4824982072974251, -4.415768667553307481E-15 ) ) ;
#68763=CARTESIAN_POINT ( 'NONE',  ( 184.2872616852876604, 288.7374155515942107, -13.26387661018510222 ) ) ;
#68764=CARTESIAN_POINT ( 'NONE',  ( 160.6042429136753640, 281.4700839698870141, 5.616606705738245608 ) ) ;
#68765=CARTESIAN_POINT ( 'NONE',  ( 201.1755594471486859, 282.2007051268825535, -18.15567516623250910 ) ) ;
#68767=CARTESIAN_POINT ( 'NONE',  ( 60.91453611423501258, 212.6427522451419350, 10.00000000000009415 ) ) ;
#68769=CARTESIAN_POINT ( 'NONE',  ( 190.6570727744300200, 264.2611290600885354, -9.484224560939372495 ) ) ;
#68770=CARTESIAN_POINT ( 'NONE',  ( 173.6418964612505533, 251.0299360267638349, -1.052939569641322626 ) ) ;
#68774=EDGE_CURVE ( 'NONE', #61620, #63141, #74778, .T. ) ;
#68776=CARTESIAN_POINT ( 'NONE',  ( 59.39103342233883609, 193.5494855054051868, -2.679491924311248496 ) ) ;
#68777=CARTESIAN_POINT ( 'NONE',  ( 191.1788773557503305, 283.4033951996527776, -16.58345142176195708 ) ) ;
#68779=CARTESIAN_POINT ( 'NONE',  ( 87.42789010471635436, 209.0327760586659451, 1.948934522072303157E-15 ) ) ;
#68780=CARTESIAN_POINT ( 'NONE',  ( 206.3018347371251195, 273.3217358710584790, -9.309724106897926177 ) ) ;
#68781=CARTESIAN_POINT ( 'NONE',  ( 193.1169444172380167, 296.1586357973259283, -13.13373377033755318 ) ) ;
#68783=ADVANCED_FACE ( 'NONE', ( #8131 ), #62300, .T. ) ;
#68784=AXIS2_PLACEMENT_3D ( 'NONE', #15354, #91924, #23457 ) ;
#68785=CARTESIAN_POINT ( 'NONE',  ( 207.5785076975260779, 271.1104734389944042, -6.824813054587777650 ) ) ;
#68790=CARTESIAN_POINT ( 'NONE',  ( 204.8951067671525266, 275.7582601874789816, -12.50192486328161046 ) ) ;
#68791=CARTESIAN_POINT ( 'NONE',  ( 157.7529601300917363, 257.4108533407307959, 16.91445305439664892 ) ) ;
#68793=( BOUNDED_SURFACE ( )  B_SPLINE_SURFACE ( 1, 2, ( 
 ( #64290, #80029, #11607, #33910, #17696, #3511, #73400, #58177, #40960, #10096, #11114, #49094, #50574, #42466, #57673, #71905, #96227, #72920, #3986, #89162, #10597, #64799, #75274, #72418, #5859, #27295, #3022, #19708, #81524, #65286, #26791, #95744, #57172, #36744, #88152, #88651, #44343, #67652, #98583, #29166, #87164, #48599, #33388, #95239, #84385, #92480, #91482, #38733, #53920, #52443, #83390, #99071, #69636, #92970, #245, #29652, #44838, #14931, #6845, #61028, #37730, #62019, #6360, #22549, #13957, #91999, #85391, #75772, #22046, #61537, #83895, #60529, #15422, #99561, #7850, #52944, #37245, #14458, #69135, #8348, #45340, #76271, #68639, #53434, #38221, #45822, #76744, #30143, #7337, #100065, #30653, #23027, #84883, #68144, #46319, #77245, #31126, #23525, #54415, #15937, #46841, #77764, #39218, #21562, #70125, #738, #60034, #90999, #41226, #86908, #2263, #16439, #78760, #47821, #55417, #24037, #63538, #56934, #47334, #93986, #33145, #86402, #70638, #87433, #71167, #79794, #1252, #8839, #24536, #40727, #80289, #32133, #63041, #16934, #94480, #9870, #25035, #55914, #9347, #40223, #1763, #17445, #32643, #48351, #78259, #79301, #71673, #94990, #64045, #25552, #87919, #56440, #64551, #17967, #93482, #10861, #48862, #10360, #39710, #72167, #2772, #33661, #95512, #26058, #18462, #49350, #41735, #72679, #31622, #62520, #54936, #85912, #12356, #35637, #3273, #74666, #58427, #65048, #42718, #80804, #96486, #66539, #50337, #34156, #19954, #89879, #5243, #57432, #26558, #27562, #65538, #67026, #97466, #74163, #88411, #43222, #96991, #28033, #36123, #42230, #81288, #90389, #27056, #20963, #82294, #34640, #12864, #58909, #89403, #50831, #57937, #73655, #51846, #4234, #88920, #19480, #81780, #20453, #11862, #35134, #97953, #44217, #66045, #4755, #51327, #43724, #28526, #59409, #95998, #18969, #73169, #82787, #13351, #49845, #3759, #11380, #30022, #21926, #76159, #52815, #77118, #21437, #37612, #22427, #7217, #60907, #90888, #68524, #133, #37122, #91872, #68030, #36618, #83772, #7723, #75642, #67527, #6228, #38614, #99943, #52323, #14333, #45221, #6736, #15814, #99446, #53318, #84275, #69519, #69012, #30526, #91362, #38101, #83265, #29534, #46201, #44709, #45708, #75153, #14820, #13831, #61414, #54300, #23410, #76632, #92367, #61907, #22915, #92856, #53801, #98951, #98456, #84766, #85268, #15302, #31016, #5730, #29050, #59919, #60407, #40135, #87341, #57345, #18874, #80708, #87829, #72073, #86313, #71075, #71575, #41643, #72586, #86818, #11284, #16848, #63457, #32559, #55337, #18369, #40640, #17873, #10770, #64459, #1676, #47737, #94394, #3192, #33565, #95419, #78673, #48770, #34075, #24946, #55824, #42144, #32039, #17350, #48257, #79204, #9264, #79703, #9778, #73076, #2172, #26469, #95910, #33053, #64966, #88319, #49757, #63951, #94891, #10265, #49264, #25453, #56342, #41135, #2674, #62951, #25975, #56845, #24455, #80201, #93901, #58340, #19870, #50248, #28436, #50737, #34552, #81202, #97865, #5155, #88824, #12772, #58825, #59318, #5640, #42634, #81692, #90797, #12265, #21350, #44128, #35042, #75063, #51758, #36035, #66935, #43124, #74067, #52235, #4655, #36533, #98366, #59832, #83179, #13740, #44620, #3674, #65450, #26960, #57843, #19389, #11771, #73563, #64575, #63063, #24557, #40245, #49367, #3293, #80311, #71186, #55437, #25572, #17462, #71690, #48372, #72701, #47841, #33164, #86426, #2286, #96015, #78781, #32661, #72187, #94501, #63561, #26076, #40745, #18481, #25058, #55934, #86932, #10378, #18991, #79320, #64068, #95012, #56461, #41248, #87452, #17985, #2797, #33678, #95531, #56952, #87938, #10878, #41755, #34173, #65065, #26576, #57452, #88431, #49862, #80827, #11396, #1271, #32156, #21455, #4776, #74687, #19502, #51864, #97487, #12884, #27076, #89420, #58449, #66063, #19974, #35659, #81801, #82803, #13372, #5263, #51349, #36143, #42249, #44238, #28051, #3777, #12377, #50356, #35156, #67046, #50851, #73185, #58926, #28546, #75175, #96507, #65559, #66559, #4256, #5749, #89897, #97970, #20474, #57957, #82313, #67546, #97013, #43742, #27582, #34659, #43243, #36640, #42739, #88943, #73675, #98477, #59429, #81311, #74185, #90406, #20982, #83286, #29069, #59935, #90905, #52343, #11882, #69542, #30041, #77139, #21945, #68540, #85287, #83790, #84784, #54830, #60929, #91383, #7746, #93381, #62420, #76649, #61433, #645, #61924, #31529, #53340, #6753, #75664, #45727, #23933, #91893, #39117, #92874, #6247, #149, #7236, #52841, #69036, #70031, #13852, #44729, #31036, #53822, #68047, #14352, #84292, #23428, #54317, #99464, #37145, #98969, #45240, #76176, #29553, #15833, #22444, #99965, #46737, #46217, #37630, #60426, #14839, #77666, #15321, #38632, #38118, #30549, #8252, #92387, #22934, #95894, #85814, #9249, #40124, #1663, #1154, #40626, #62936, #26454, #8744, #80186, #49248, #63446, #64445, #10752, #3174, #24445, #55323, #63938, #2658, #79189, #70536, #86803, #24935, #16343, #16836, #86302, #78156, #55810, #32028, #47725, #71062, #93889, #10252, #32547, #47238, #78660, #41628, #17338, #48244, #87325, #9765, #71562, #41122, #2159, #33550, #33039, #94876, #25439, #56330, #34059, #17858, #48758, #79690, #72056, #95404, #25960, #56832, #87817, #18355, #72570, #64949, #39614, #50721, #73061, #74051, #4639, #20346, #97361, #57827, #82686, #96378, #90283, #11753, #18857, #36519, #19853, #89773, #34537, #66921, #12250, #27927, #42129, #4131, #73548, #81186, #35024, #81675, #96884, #97851, #28422, #51218, #66435, #82186, #57329, #59301, #43107, #49739, #27451, #65435, #50232, #12758, #65928, #88302, #35532, #43621, #20853, #11266, #80692, #58810, #19372, #51744, #74562, #5139, #3656, #36020, #13253, #44111, #75050, #26942, #58325, #5625, #42617, #67420, #98350, #88806, #89300, #22821, #53223, #84174, #52710, #99343, #77539, #68417, #14232, #83669, #76537, #53704, #60302, #6635, #33, #69909, #45119, #14723, #61311, #91261, #7618, #84659, #21333, #52217, #67930, #38507, #61805, #69421, #98852 ),
 ( #45605, #76054, #29923, #8130, #60796, #37510, #91757, #7115, #15203, #21824, #22321, #30919, #28940, #37999, #68913, #92273, #99837, #92754, #46099, #83163, #13728, #29428, #23308, #54196, #85163, #30422, #44605, #77013, #15707, #46609, #39004, #59816, #75539, #90783, #6125, #37021, #25842, #85684, #62811, #2027, #24325, #39492, #56203, #39997, #48635, #70419, #78033, #93767, #9646, #49127, #1028, #31906, #55200, #32424, #79060, #63319, #94259, #16718, #86184, #47612, #24813, #78539, #55690, #16221, #17210, #48117, #63819, #40505, #9127, #56717, #70936, #33423, #1541, #62299, #80063, #86679, #32912, #8625, #10127, #71438, #94754, #47114, #25317, #87201, #17733, #79569, #40993, #71936, #2541, #64321, #95280, #87699, #18232, #524, #10632, #41508, #93256, #31412, #23811, #54701, #35410, #19252, #3055, #89188, #58691, #43502, #26329, #95775, #96759, #34418, #35904, #66316, #42988, #57204, #81555, #65801, #97251, #27815, #51613, #20727, #34901, #19737, #59179, #20227, #90153, #11637, #65318, #33943, #4018, #82567, #50118, #97732, #51097, #64829, #89664, #27327, #80567, #58210, #28300, #13130, #72448, #82064, #12123, #88182, #11146, #42496, #12631, #74443, #26823, #18730, #49614, #3542, #72949, #42015, #5023, #81071, #50602, #66804, #4509, #96257, #57703, #88679, #73430, #73925, #6999, #67303, #29807, #15089, #44493, #6008, #85037, #43988, #67813, #29317, #60182, #59699, #60679, #52102, #74930, #98230, #38389, #69300, #52593, #53592, #100224, #61689, #83048, #13621, #53102, #61192, #37394, #28812, #75941, #83550, #5514, #36902, #14113, #36397, #6517, #90666, #68298, #84058, #45492, #68794, #37884, #99721, #30307, #92161, #84548, #45978, #76894, #92642, #40878, #77918, #32300, #8509, #77418, #93641, #17606, #16104, #8021, #47004, #79451, #40383, #93135, #55088, #86075, #24208, #56598, #16599, #9003, #70811, #10015, #9521, #71322, #31785, #78933, #23684, #70295, #87074, #85559, #86563, #15585, #62686, #54577, #906, #64202, #406, #39378, #47496, #38893, #1914, #78421, #1418, #94641, #47991, #39875, #31296, #63202, #25196, #17094, #32799, #69796, #94143, #48515, #24698, #55580, #25719, #46486, #63704, #56080, #71825, #62182, #2423, #33301, #95151, #10510, #83303, #52355, #66570, #67558, #13864, #6263, #26211, #57088, #97982, #5761, #82328, #72332, #89908, #97496, #87585, #18619, #88069, #79946, #28063, #2935, #50863, #74199, #33824, #13382, #12389, #18110, #64714, #36155, #20995, #74697, #95663, #12897, #44743, #81813, #5276, #43254, #49012, #58937, #90918, #4788, #35668, #20488, #75677, #44252, #51359, #28560, #59440, #90422, #29565, #51876, #82814, #75187, #37159, #36651, #98490, #29082, #59947, #21467, #68058, #98981, #30054, #31048, #1165, #76661, #37642, #23441, #39628, #8756, #22946, #7757, #47249, #8265, #78169, #99979, #53354, #21960, #92399, #70549, #38131, #85826, #39129, #52853, #15845, #53835, #68553, #15336, #16356, #60439, #91395, #46754, #160, #14368, #99478, #30563, #70043, #656, #69049, #83803, #31543, #45254, #77681, #84795, #60946, #46231, #76189, #6764, #91904, #62431, #61935, #22459, #84304, #61447, #93394, #23945, #14852, #45739, #7249, #77155, #38651, #69555, #54845, #92887, #54330, #85302, #93721, #49484, #76973, #69377, #39953, #62763, #24282, #84619, #47075, #32377, #61767, #23264, #71397, #61266, #85115, #15667, #77496, #7576, #16179, #38463, #1987, #15161, #55651, #24772, #38964, #70891, #86636, #79012, #30880, #92714, #39451, #78497, #54658, #46057, #62255, #69870, #92235, #54154, #46561, #53664, #482, #8089, #31371, #93210, #23764, #86145, #85634, #22786, #77993, #8586, #55158, #70372, #982, #31864, #17171, #16676, #47569, #9083, #1494, #63276, #94217, #48071, #9600, #40461, #96716, #57660, #10088, #72405, #3011, #41462, #73881, #33903, #26287, #88141, #27283, #26779, #88640, #49086, #96216, #40951, #87658, #3976, #2494, #3499, #32872, #80019, #33377, #19205, #63777, #94711, #95734, #80522, #19697, #81032, #50562, #64788, #25796, #25273, #57160, #56159, #64280, #17686, #18687, #10588, #49570, #11098, #34857, #56672, #41971, #87154, #72909, #58165, #48587, #18189, #34376, #65274, #50074, #11595, #42454, #73388, #65761, #89147, #13815, #60892, #120, #44697, #37110, #21911, #14319, #99431, #45206, #76145, #6719, #37598, #68509, #22414, #76618, #46187, #31004, #61893, #20950, #82773, #5718, #93345, #17826, #31496, #25407, #47202, #54285, #72027, #55289, #24905, #69999, #2125, #47694, #63412, #77632, #39584, #8714, #16309, #70504, #86269, #31997, #33007, #63908, #55781, #1635, #86772, #92844, #94846, #78629, #85255, #62906, #614, #85780, #17308, #1119, #23395, #9215, #79158, #56299, #46706, #15801, #16807, #54803, #87295, #48213, #94351, #8216, #32519, #40090, #9739, #48727, #62388, #93858, #79660, #78126, #10223, #71533, #23901, #41091, #40595, #71033, #2629, #24413, #33519, #39086, #3629, #49706, #88273, #11726, #58297, #95864, #42102, #35503, #5111, #18822, #88776, #96855, #26422, #43079, #89274, #56803, #87788, #3147, #74023, #97332, #4611, #34032, #49224, #19345, #11239, #65408, #73036, #66405, #10722, #26916, #18328, #96351, #89753, #80157, #57302, #65899, #80661, #64920, #19823, #34507, #12220, #57796, #41598, #50207, #73521, #12731, #81159, #42588, #4104, #34997, #27422, #50693, #81648, #27901, #58781, #20319, #51188, #82156, #43595, #72542, #74532, #64415, #95378, #25930, #75020, #84148, #13223, #22293, #98321, #97825, #37970, #44578, #52680, #82660, #99313, #36993, #21796, #90251, #90757, #59787, #67396, #21308, #75511, #52185, #29892, #60765, #83641, #60273, #14202, #35991, #91728, #67902, #28395, #83134, #44080, #28913, #45093, #13704, #59273, #98822, #37477, #53193, #20824, #51718, #29403, #6097, #14694, #76027, #6604, #5602, #91229, #68388, #45577, #76505, #36493, #7086, #68878, #66896, #43920, #4954, #57627, #35833, #20155, #50525, #81479, #50043, #96681, #74859, #65724, #11561, #80996, #73845, #51023, #88605, #3941, #97662, #67226 ) ),
 .UNSPECIFIED., .F., .F., .T. ) 
 B_SPLINE_SURFACE_WITH_KNOTS ( ( 2, 2 ),
 ( 3, 2, 2, 2, 2, 2, 2, 2, 2, 2, 2, 2, 2, 2, 2, 2, 2, 2, 2, 2, 2, 2, 2, 2, 2, 2, 2, 2, 2, 2, 2, 2, 2, 2, 2, 2, 2, 2, 2, 2, 2, 2, 2, 2, 2, 2, 2, 2, 2, 2, 2, 2, 2, 2, 2, 2, 2, 2, 2, 2, 2, 2, 2, 2, 2, 2, 2, 2, 2, 2, 2, 2, 2, 2, 2, 2, 2, 2, 2, 2, 2, 2, 2, 2, 2, 2, 2, 2, 2, 2, 2, 2, 2, 2, 2, 2, 2, 2, 2, 2, 2, 2, 2, 2, 2, 2, 2, 2, 2, 2, 2, 2, 2, 2, 2, 2, 2, 2, 2, 2, 2, 2, 2, 2, 2, 2, 2, 2, 2, 2, 2, 2, 2, 2, 2, 2, 2, 2, 2, 2, 2, 2, 2, 2, 2, 2, 2, 2, 2, 2, 2, 2, 2, 2, 2, 2, 2, 2, 2, 2, 2, 2, 2, 2, 2, 2, 2, 2, 2, 2, 2, 2, 2, 2, 2, 2, 2, 2, 2, 2, 2, 2, 2, 2, 2, 2, 2, 2, 2, 2, 2, 2, 2, 2, 2, 2, 2, 2, 2, 2, 2, 2, 2, 2, 2, 2, 2, 2, 2, 2, 2, 2, 2, 2, 2, 2, 2, 2, 2, 2, 2, 2, 2, 2, 2, 2, 2, 2, 2, 2, 2, 2, 2, 2, 2, 2, 2, 2, 2, 2, 2, 2, 2, 2, 2, 2, 2, 2, 2, 2, 2, 2, 2, 2, 2, 2, 2, 2, 2, 2, 2, 2, 2, 2, 2, 2, 2, 2, 2, 2, 2, 2, 2, 2, 2, 2, 2, 2, 2, 2, 2, 2, 2, 2, 2, 2, 2, 2, 2, 2, 2, 2, 2, 2, 2, 2, 2, 2, 2, 2, 2, 2, 2, 2, 2, 2, 2, 2, 2, 2, 2, 2, 2, 2, 2, 2, 2, 2, 2, 2, 2, 2, 2, 2, 2, 2, 2, 2, 2, 2, 2, 2, 2, 2, 2, 2, 2, 2, 2, 2, 2, 2, 2, 2, 2, 2, 2, 2, 2, 2, 2, 2, 2, 2, 2, 2, 2, 2, 2, 2, 2, 2, 2, 2, 2, 2, 2, 2, 2, 2, 2, 2, 3 ),
 ( 0.000000000000000000, 1.000000000000000000 ),
 ( 0.000000000000000000, 0.002688172043010752903, 0.005376344086021505805, 0.008064516129032257841, 0.01075268817204301161, 0.01344086021505376365, 0.01612903225806451568, 0.01881720430107526945, 0.02150537634408602322, 0.02419354838709677352, 0.02688172043010752729, 0.02956989247311828106, 0.03225806451612903136, 0.03494623655913978166, 0.03763440860215053890, 0.04032258064516128920, 0.04301075268817204644, 0.04569892473118279674, 0.04838709677419354704, 0.05107526881720430428, 0.05376344086021505458, 0.05645161290322580488, 0.05913978494623656212, 0.06182795698924731242, 0.06451612903225806273, 0.06720430107526881303, 0.06989247311827956333, 0.07258064516129032751, 0.07526881720430107781, 0.07795698924731182811, 0.08064516129032257841, 0.08333333333333332871, 0.08602150537634409289, 0.08870967741935484319, 0.09139784946236559349, 0.09408602150537634379, 0.09677419354838709409, 0.09946236559139784439, 0.1021505376344086086, 0.1048387096774193589, 0.1075268817204301092, 0.1102150537634408595, 0.1129032258064516098, 0.1155913978494623601, 0.1182795698924731242, 0.1209677419354838745, 0.1236559139784946248, 0.1263440860215053752, 0.1290322580645161255, 0.1317204301075268758, 0.1344086021505376261, 0.1370967741935483764, 0.1397849462365591267, 0.1424731182795699047, 0.1451612903225806550, 0.1478494623655914053, 0.1505376344086021556, 0.1532258064516129059, 0.1559139784946236562, 0.1586021505376344065, 0.1612903225806451568, 0.1639784946236559071, 0.1666666666666666574, 0.1693548387096774077, 0.1720430107526881858, 0.1747311827956989361, 0.1774193548387096864, 0.1801075268817204367, 0.1827956989247311870, 0.1854838709677419373, 0.1881720430107526876, 0.1908602150537634379, 0.1935483870967741882, 0.1962365591397849385, 0.1989247311827956888, 0.2016129032258064391, 0.2043010752688172171, 0.2069892473118279674, 0.2096774193548387177, 0.2123655913978494680, 0.2150537634408602183, 0.2177419354838709686, 0.2204301075268817189, 0.2231182795698924692, 0.2258064516129032195, 0.2284946236559139698, 0.2311827956989247201, 0.2338709677419354704, 0.2365591397849462485, 0.2392473118279569988, 0.2419354838709677491, 0.2446236559139784994, 0.2473118279569892497, 0.2500000000000000000, 0.2526881720430107503, 0.2553763440860215006, 0.2580645161290322509, 0.2607526881720430012, 0.2634408602150537515, 0.2661290322580645018, 0.2688172043010752521, 0.2715053763440860024, 0.2741935483870967527, 0.2768817204301075030, 0.2795698924731182533, 0.2822580645161290591, 0.2849462365591398094, 0.2876344086021505597, 0.2903225806451613100, 0.2930107526881720603, 0.2956989247311828106, 0.2983870967741935609, 0.3010752688172043112, 0.3037634408602150615, 0.3064516129032258118, 0.3091397849462365621, 0.3118279569892473124, 0.3145161290322580627, 0.3172043010752688130, 0.3198924731182795633, 0.3225806451612903136, 0.3252688172043010639, 0.3279569892473118142, 0.3306451612903225645, 0.3333333333333333148, 0.3360215053763440651, 0.3387096774193548154, 0.3413978494623655657, 0.3440860215053763715, 0.3467741935483871218, 0.3494623655913978721, 0.3521505376344086224, 0.3548387096774193727, 0.3575268817204301230, 0.3602150537634408733, 0.3629032258064516236, 0.3655913978494623739, 0.3682795698924731242, 0.3709677419354838745, 0.3736559139784946248, 0.3763440860215053752, 0.3790322580645161255, 0.3817204301075268758, 0.3844086021505376261, 0.3870967741935483764, 0.3897849462365591267, 0.3924731182795698770, 0.3951612903225806273, 0.3978494623655913776, 0.4005376344086021279, 0.4032258064516128782, 0.4059139784946236285, 0.4086021505376344343, 0.4112903225806451846, 0.4139784946236559349, 0.4166666666666666852, 0.4193548387096774355, 0.4220430107526881858, 0.4247311827956989361, 0.4274193548387096864, 0.4301075268817204367, 0.4327956989247311870, 0.4354838709677419373, 0.4381720430107526876, 0.4408602150537634379, 0.4435483870967741882, 0.4462365591397849385, 0.4489247311827956888, 0.4516129032258064391, 0.4543010752688171894, 0.4569892473118279397, 0.4596774193548386900, 0.4623655913978494403, 0.4650537634408601906, 0.4677419354838709409, 0.4704301075268817467, 0.4731182795698924970, 0.4758064516129032473, 0.4784946236559139976, 0.4811827956989247479, 0.4838709677419354982, 0.4865591397849462485, 0.4892473118279569988, 0.4919354838709677491, 0.4946236559139784994, 0.4973118279569892497, 0.5000000000000000000, 0.5026881720430107503, 0.5053763440860215006, 0.5080645161290322509, 0.5107526881720430012, 0.5134408602150537515, 0.5161290322580645018, 0.5188172043010752521, 0.5215053763440860024, 0.5241935483870967527, 0.5268817204301075030, 0.5295698924731182533, 0.5322580645161290036, 0.5349462365591397539, 0.5376344086021505042, 0.5403225806451612545, 0.5430107526881720048, 0.5456989247311827551, 0.5483870967741935054, 0.5510752688172042557, 0.5537634408602150060, 0.5564516129032257563, 0.5591397849462365066, 0.5618279569892472569, 0.5645161290322581182, 0.5672043010752688685, 0.5698924731182796188, 0.5725806451612903691, 0.5752688172043011194, 0.5779569892473118697, 0.5806451612903226200, 0.5833333333333333703, 0.5860215053763441206, 0.5887096774193548709, 0.5913978494623656212, 0.5940860215053763715, 0.5967741935483871218, 0.5994623655913978721, 0.6021505376344086224, 0.6048387096774193727, 0.6075268817204301230, 0.6102150537634408733, 0.6129032258064516236, 0.6155913978494623739, 0.6182795698924731242, 0.6209677419354838745, 0.6236559139784946248, 0.6263440860215053752, 0.6290322580645161255, 0.6317204301075268758, 0.6344086021505376261, 0.6370967741935483764, 0.6397849462365591267, 0.6424731182795698770, 0.6451612903225806273, 0.6478494623655913776, 0.6505376344086021279, 0.6532258064516128782, 0.6559139784946236285, 0.6586021505376343788, 0.6612903225806451291, 0.6639784946236558794, 0.6666666666666666297, 0.6693548387096773800, 0.6720430107526881303, 0.6747311827956988806, 0.6774193548387096309, 0.6801075268817203812, 0.6827956989247311315, 0.6854838709677418818, 0.6881720430107527431, 0.6908602150537634934, 0.6935483870967742437, 0.6962365591397849940, 0.6989247311827957443, 0.7016129032258064946, 0.7043010752688172449, 0.7069892473118279952, 0.7096774193548387455, 0.7123655913978494958, 0.7150537634408602461, 0.7177419354838709964, 0.7204301075268817467, 0.7231182795698924970, 0.7258064516129032473, 0.7284946236559139976, 0.7311827956989247479, 0.7338709677419354982, 0.7365591397849462485, 0.7392473118279569988, 0.7419354838709677491, 0.7446236559139784994, 0.7473118279569892497, 0.7500000000000000000, 0.7526881720430107503, 0.7553763440860215006, 0.7580645161290322509, 0.7607526881720430012, 0.7634408602150537515, 0.7661290322580645018, 0.7688172043010752521, 0.7715053763440860024, 0.7741935483870967527, 0.7768817204301075030, 0.7795698924731182533, 0.7822580645161290036, 0.7849462365591397539, 0.7876344086021505042, 0.7903225806451612545, 0.7930107526881720048, 0.7956989247311827551, 0.7983870967741935054, 0.8010752688172042557, 0.8037634408602150060, 0.8064516129032257563, 0.8091397849462365066, 0.8118279569892472569, 0.8145161290322581182, 0.8172043010752688685, 0.8198924731182796188, 0.8225806451612903691, 0.8252688172043011194, 0.8279569892473118697, 0.8306451612903226200, 0.8333333333333333703, 0.8360215053763441206, 0.8387096774193548709, 0.8413978494623656212, 0.8440860215053763715, 0.8467741935483871218, 0.8494623655913978721, 0.8521505376344086224, 0.8548387096774193727, 0.8575268817204301230, 0.8602150537634408733, 0.8629032258064516236, 0.8655913978494623739, 0.8682795698924731242, 0.8709677419354838745, 0.8736559139784946248, 0.8763440860215053752, 0.8790322580645161255, 0.8817204301075268758, 0.8844086021505376261, 0.8870967741935483764, 0.8897849462365591267, 0.8924731182795698770, 0.8951612903225806273, 0.8978494623655913776, 0.9005376344086021279, 0.9032258064516128782, 0.9059139784946236285, 0.9086021505376343788, 0.9112903225806451291, 0.9139784946236558794, 0.9166666666666666297, 0.9193548387096773800, 0.9220430107526881303, 0.9247311827956988806, 0.9274193548387096309, 0.9301075268817203812, 0.9327956989247311315, 0.9354838709677418818, 0.9381720430107527431, 0.9408602150537634934, 0.9435483870967742437, 0.9462365591397849940, 0.9489247311827957443, 0.9516129032258064946, 0.9543010752688172449, 0.9569892473118279952, 0.9596774193548387455, 0.9623655913978494958, 0.9650537634408602461, 0.9677419354838709964, 0.9704301075268817467, 0.9731182795698924970, 0.9758064516129032473, 0.9784946236559139976, 0.9811827956989247479, 0.9838709677419354982, 0.9865591397849462485, 0.9892473118279569988, 0.9919354838709677491, 0.9946236559139784994, 0.9973118279569892497, 1.000000000000000000 ),
 .UNSPECIFIED. ) 
 GEOMETRIC_REPRESENTATION_ITEM ( )  RATIONAL_B_SPLINE_SURFACE ( (
 ( 1.000000000000000000, 0.8660254037844387076, 1.000000000000000000, 0.8660254037844387076, 1.000000000000000000, 0.8660254037844387076, 1.000000000000000000, 0.8660254037844387076, 1.000000000000000000, 0.8660254037844387076, 1.000000000000000000, 0.8660254037844387076, 1.000000000000000000, 0.8660254037844387076, 1.000000000000000000, 0.8660254037844387076, 1.000000000000000000, 0.8660254037844387076, 1.000000000000000000, 0.8660254037844387076, 1.000000000000000000, 0.8660254037844387076, 1.000000000000000000, 0.8660254037844387076, 1.000000000000000000, 0.8660254037844387076, 1.000000000000000000, 0.8660254037844387076, 1.000000000000000000, 0.8660254037844387076, 1.000000000000000000, 0.8660254037844387076, 1.000000000000000000, 0.8660254037844387076, 1.000000000000000000, 0.8660254037844387076, 1.000000000000000000, 0.8660254037844387076, 1.000000000000000000, 0.8660254037844387076, 1.000000000000000000, 0.8660254037844387076, 1.000000000000000000, 0.8660254037844387076, 1.000000000000000000, 0.8660254037844387076, 1.000000000000000000, 0.8660254037844387076, 1.000000000000000000, 0.8660254037844387076, 1.000000000000000000, 0.8660254037844387076, 1.000000000000000000, 0.8660254037844387076, 1.000000000000000000, 0.8660254037844387076, 1.000000000000000000, 0.8660254037844387076, 1.000000000000000000, 0.8660254037844387076, 1.000000000000000000, 0.8660254037844387076, 1.000000000000000000, 0.8660254037844387076, 1.000000000000000000, 0.8660254037844387076, 1.000000000000000000, 0.8660254037844387076, 1.000000000000000000, 0.8660254037844387076, 1.000000000000000000, 0.8660254037844387076, 1.000000000000000000, 0.8660254037844387076, 1.000000000000000000, 0.8660254037844387076, 1.000000000000000000, 0.8660254037844387076, 1.000000000000000000, 0.8660254037844387076, 1.000000000000000000, 0.8660254037844387076, 1.000000000000000000, 0.8660254037844387076, 1.000000000000000000, 0.8660254037844387076, 1.000000000000000000, 0.8660254037844387076, 1.000000000000000000, 0.8660254037844387076, 1.000000000000000000, 0.8660254037844387076, 1.000000000000000000, 0.8660254037844387076, 1.000000000000000000, 0.8660254037844387076, 1.000000000000000000, 0.8660254037844387076, 1.000000000000000000, 0.8660254037844387076, 1.000000000000000000, 0.8660254037844387076, 1.000000000000000000, 0.8660254037844387076, 1.000000000000000000, 0.8660254037844387076, 1.000000000000000000, 0.8660254037844387076, 1.000000000000000000, 0.8660254037844387076, 1.000000000000000000, 0.8660254037844387076, 1.000000000000000000, 0.8660254037844387076, 1.000000000000000000, 0.8660254037844387076, 1.000000000000000000, 0.8660254037844387076, 1.000000000000000000, 0.8660254037844387076, 1.000000000000000000, 0.8660254037844387076, 1.000000000000000000, 0.8660254037844387076, 1.000000000000000000, 0.8660254037844387076, 1.000000000000000000, 0.8660254037844387076, 1.000000000000000000, 0.8660254037844387076, 1.000000000000000000, 0.8660254037844387076, 1.000000000000000000, 0.8660254037844387076, 1.000000000000000000, 0.8660254037844387076, 1.000000000000000000, 0.8660254037844387076, 1.000000000000000000, 0.8660254037844387076, 1.000000000000000000, 0.8660254037844387076, 1.000000000000000000, 0.8660254037844387076, 1.000000000000000000, 0.8660254037844387076, 1.000000000000000000, 0.8660254037844387076, 1.000000000000000000, 0.8660254037844387076, 1.000000000000000000, 0.8660254037844387076, 1.000000000000000000, 0.8660254037844387076, 1.000000000000000000, 0.8660254037844387076, 1.000000000000000000, 0.8660254037844387076, 1.000000000000000000, 0.8660254037844387076, 1.000000000000000000, 0.8660254037844387076, 1.000000000000000000, 0.8660254037844387076, 1.000000000000000000, 0.8660254037844387076, 1.000000000000000000, 0.8660254037844387076, 1.000000000000000000, 0.8660254037844387076, 1.000000000000000000, 0.8660254037844387076, 1.000000000000000000, 0.8660254037844387076, 1.000000000000000000, 0.8660254037844387076, 1.000000000000000000, 0.8660254037844387076, 1.000000000000000000, 0.8660254037844387076, 1.000000000000000000, 0.8660254037844387076, 1.000000000000000000, 0.8660254037844387076, 1.000000000000000000, 0.8660254037844387076, 1.000000000000000000, 0.8660254037844387076, 1.000000000000000000, 0.8660254037844387076, 1.000000000000000000, 0.8660254037844387076, 1.000000000000000000, 0.8660254037844387076, 1.000000000000000000, 0.8660254037844387076, 1.000000000000000000, 0.8660254037844387076, 1.000000000000000000, 0.8660254037844387076, 1.000000000000000000, 0.8660254037844387076, 1.000000000000000000, 0.8660254037844387076, 1.000000000000000000, 0.8660254037844387076, 1.000000000000000000, 0.8660254037844387076, 1.000000000000000000, 0.8660254037844387076, 1.000000000000000000, 0.8660254037844387076, 1.000000000000000000, 0.8660254037844387076, 1.000000000000000000, 0.8660254037844387076, 1.000000000000000000, 0.8660254037844387076, 1.000000000000000000, 0.8660254037844387076, 1.000000000000000000, 0.8660254037844387076, 1.000000000000000000, 0.8660254037844387076, 1.000000000000000000, 0.8660254037844387076, 1.000000000000000000, 0.8660254037844387076, 1.000000000000000000, 0.8660254037844387076, 1.000000000000000000, 0.8660254037844387076, 1.000000000000000000, 0.8660254037844387076, 1.000000000000000000, 0.8660254037844387076, 1.000000000000000000, 0.8660254037844387076, 1.000000000000000000, 0.8660254037844387076, 1.000000000000000000, 0.8660254037844387076, 1.000000000000000000, 0.8660254037844387076, 1.000000000000000000, 0.8660254037844387076, 1.000000000000000000, 0.8660254037844387076, 1.000000000000000000, 0.8660254037844387076, 1.000000000000000000, 0.8660254037844387076, 1.000000000000000000, 0.8660254037844387076, 1.000000000000000000, 0.8660254037844387076, 1.000000000000000000, 0.8660254037844387076, 1.000000000000000000, 0.8660254037844387076, 1.000000000000000000, 0.8660254037844387076, 1.000000000000000000, 0.8660254037844387076, 1.000000000000000000, 0.8660254037844387076, 1.000000000000000000, 0.8660254037844387076, 1.000000000000000000, 0.8660254037844387076, 1.000000000000000000, 0.8660254037844387076, 1.000000000000000000, 0.8660254037844387076, 1.000000000000000000, 0.8660254037844387076, 1.000000000000000000, 0.8660254037844387076, 1.000000000000000000, 0.8660254037844387076, 1.000000000000000000, 0.8660254037844387076, 1.000000000000000000, 0.8660254037844387076, 1.000000000000000000, 0.8660254037844387076, 1.000000000000000000, 0.8660254037844387076, 1.000000000000000000, 0.8660254037844387076, 1.000000000000000000, 0.8660254037844387076, 1.000000000000000000, 0.8660254037844387076, 1.000000000000000000, 0.8660254037844387076, 1.000000000000000000, 0.8660254037844387076, 1.000000000000000000, 0.8660254037844387076, 1.000000000000000000, 0.8660254037844387076, 1.000000000000000000, 0.8660254037844387076, 1.000000000000000000, 0.8660254037844387076, 1.000000000000000000, 0.8660254037844387076, 1.000000000000000000, 0.8660254037844387076, 1.000000000000000000, 0.8660254037844387076, 1.000000000000000000, 0.8660254037844387076, 1.000000000000000000, 0.8660254037844387076, 1.000000000000000000, 0.8660254037844387076, 1.000000000000000000, 0.8660254037844387076, 1.000000000000000000, 0.8660254037844387076, 1.000000000000000000, 0.8660254037844387076, 1.000000000000000000, 0.8660254037844387076, 1.000000000000000000, 0.8660254037844387076, 1.000000000000000000, 0.8660254037844387076, 1.000000000000000000, 0.8660254037844387076, 1.000000000000000000, 0.8660254037844387076, 1.000000000000000000, 0.8660254037844387076, 1.000000000000000000, 0.8660254037844387076, 1.000000000000000000, 0.8660254037844387076, 1.000000000000000000, 0.8660254037844387076, 1.000000000000000000, 0.8660254037844387076, 1.000000000000000000, 0.8660254037844387076, 1.000000000000000000, 0.8660254037844387076, 1.000000000000000000, 0.8660254037844387076, 1.000000000000000000, 0.8660254037844387076, 1.000000000000000000, 0.8660254037844387076, 1.000000000000000000, 0.8660254037844387076, 1.000000000000000000, 0.8660254037844387076, 1.000000000000000000, 0.8660254037844387076, 1.000000000000000000, 0.8660254037844387076, 1.000000000000000000, 0.8660254037844387076, 1.000000000000000000, 0.8660254037844387076, 1.000000000000000000, 0.8660254037844387076, 1.000000000000000000, 0.8660254037844387076, 1.000000000000000000, 0.8660254037844387076, 1.000000000000000000, 0.8660254037844387076, 1.000000000000000000, 0.8660254037844387076, 1.000000000000000000, 0.8660254037844387076, 1.000000000000000000, 0.8660254037844387076, 1.000000000000000000, 0.8660254037844387076, 1.000000000000000000, 0.8660254037844387076, 1.000000000000000000, 0.8660254037844387076, 1.000000000000000000, 0.8660254037844387076, 1.000000000000000000, 0.8660254037844387076, 1.000000000000000000, 0.8660254037844387076, 1.000000000000000000, 0.8660254037844387076, 1.000000000000000000, 0.8660254037844387076, 1.000000000000000000, 0.8660254037844387076, 1.000000000000000000, 0.8660254037844387076, 1.000000000000000000, 0.8660254037844387076, 1.000000000000000000, 0.8660254037844387076, 1.000000000000000000, 0.8660254037844387076, 1.000000000000000000, 0.8660254037844387076, 1.000000000000000000, 0.8660254037844387076, 1.000000000000000000, 0.8660254037844387076, 1.000000000000000000, 0.8660254037844387076, 1.000000000000000000, 0.8660254037844387076, 1.000000000000000000, 0.8660254037844387076, 1.000000000000000000, 0.8660254037844387076, 1.000000000000000000, 0.8660254037844387076, 1.000000000000000000, 0.8660254037844387076, 1.000000000000000000, 0.8660254037844387076, 1.000000000000000000, 0.8660254037844387076, 1.000000000000000000, 0.8660254037844387076, 1.000000000000000000, 0.8660254037844387076, 1.000000000000000000, 0.8660254037844387076, 1.000000000000000000, 0.8660254037844387076, 1.000000000000000000, 0.8660254037844387076, 1.000000000000000000, 0.8660254037844387076, 1.000000000000000000, 0.8660254037844387076, 1.000000000000000000, 0.8660254037844387076, 1.000000000000000000, 0.8660254037844387076, 1.000000000000000000, 0.8660254037844387076, 1.000000000000000000, 0.8660254037844387076, 1.000000000000000000, 0.8660254037844387076, 1.000000000000000000, 0.8660254037844387076, 1.000000000000000000, 0.8660254037844387076, 1.000000000000000000, 0.8660254037844387076, 1.000000000000000000, 0.8660254037844387076, 1.000000000000000000, 0.8660254037844387076, 1.000000000000000000, 0.8660254037844387076, 1.000000000000000000, 0.8660254037844387076, 1.000000000000000000, 0.8660254037844387076, 1.000000000000000000, 0.8660254037844387076, 1.000000000000000000, 0.8660254037844387076, 1.000000000000000000, 0.8660254037844387076, 1.000000000000000000, 0.8660254037844387076, 1.000000000000000000, 0.8660254037844387076, 1.000000000000000000, 0.8660254037844387076, 1.000000000000000000, 0.8660254037844387076, 1.000000000000000000, 0.8660254037844387076, 1.000000000000000000, 0.8660254037844387076, 1.000000000000000000, 0.8660254037844387076, 1.000000000000000000, 0.8660254037844387076, 1.000000000000000000, 0.8660254037844387076, 1.000000000000000000, 0.8660254037844387076, 1.000000000000000000, 0.8660254037844387076, 1.000000000000000000, 0.8660254037844387076, 1.000000000000000000, 0.8660254037844387076, 1.000000000000000000, 0.8660254037844387076, 1.000000000000000000, 0.8660254037844387076, 1.000000000000000000, 0.8660254037844387076, 1.000000000000000000, 0.8660254037844387076, 1.000000000000000000, 0.8660254037844387076, 1.000000000000000000, 0.8660254037844387076, 1.000000000000000000, 0.8660254037844387076, 1.000000000000000000, 0.8660254037844387076, 1.000000000000000000, 0.8660254037844387076, 1.000000000000000000, 0.8660254037844387076, 1.000000000000000000, 0.8660254037844387076, 1.000000000000000000, 0.8660254037844387076, 1.000000000000000000, 0.8660254037844387076, 1.000000000000000000, 0.8660254037844387076, 1.000000000000000000, 0.8660254037844387076, 1.000000000000000000, 0.8660254037844387076, 1.000000000000000000, 0.8660254037844387076, 1.000000000000000000, 0.8660254037844387076, 1.000000000000000000, 0.8660254037844387076, 1.000000000000000000, 0.8660254037844387076, 1.000000000000000000, 0.8660254037844387076, 1.000000000000000000, 0.8660254037844387076, 1.000000000000000000, 0.8660254037844387076, 1.000000000000000000, 0.8660254037844387076, 1.000000000000000000, 0.8660254037844387076, 1.000000000000000000, 0.8660254037844387076, 1.000000000000000000, 0.8660254037844387076, 1.000000000000000000, 0.8660254037844387076, 1.000000000000000000, 0.8660254037844387076, 1.000000000000000000, 0.8660254037844387076, 1.000000000000000000, 0.8660254037844387076, 1.000000000000000000, 0.8660254037844387076, 1.000000000000000000, 0.8660254037844387076, 1.000000000000000000, 0.8660254037844387076, 1.000000000000000000, 0.8660254037844387076, 1.000000000000000000, 0.8660254037844387076, 1.000000000000000000, 0.8660254037844387076, 1.000000000000000000, 0.8660254037844387076, 1.000000000000000000, 0.8660254037844387076, 1.000000000000000000, 0.8660254037844387076, 1.000000000000000000, 0.8660254037844387076, 1.000000000000000000, 0.8660254037844387076, 1.000000000000000000, 0.8660254037844387076, 1.000000000000000000, 0.8660254037844387076, 1.000000000000000000, 0.8660254037844387076, 1.000000000000000000, 0.8660254037844387076, 1.000000000000000000, 0.8660254037844387076, 1.000000000000000000, 0.8660254037844387076, 1.000000000000000000, 0.8660254037844387076, 1.000000000000000000, 0.8660254037844387076, 1.000000000000000000, 0.8660254037844387076, 1.000000000000000000, 0.8660254037844387076, 1.000000000000000000, 0.8660254037844387076, 1.000000000000000000, 0.8660254037844387076, 1.000000000000000000, 0.8660254037844387076, 1.000000000000000000, 0.8660254037844387076, 1.000000000000000000, 0.8660254037844387076, 1.000000000000000000, 0.8660254037844387076, 1.000000000000000000, 0.8660254037844387076, 1.000000000000000000, 0.8660254037844387076, 1.000000000000000000, 0.8660254037844387076, 1.000000000000000000, 0.8660254037844387076, 1.000000000000000000, 0.8660254037844387076, 1.000000000000000000, 0.8660254037844387076, 1.000000000000000000, 0.8660254037844387076, 1.000000000000000000, 0.8660254037844387076, 1.000000000000000000, 0.8660254037844387076, 1.000000000000000000, 0.8660254037844387076, 1.000000000000000000, 0.8660254037844387076, 1.000000000000000000, 0.8660254037844387076, 1.000000000000000000, 0.8660254037844387076, 1.000000000000000000, 0.8660254037844387076, 1.000000000000000000, 0.8660254037844387076, 1.000000000000000000, 0.8660254037844387076, 1.000000000000000000, 0.8660254037844387076, 1.000000000000000000, 0.8660254037844387076, 1.000000000000000000, 0.8660254037844387076, 1.000000000000000000, 0.8660254037844387076, 1.000000000000000000, 0.8660254037844387076, 1.000000000000000000, 0.8660254037844387076, 1.000000000000000000, 0.8660254037844387076, 1.000000000000000000, 0.8660254037844387076, 1.000000000000000000, 0.8660254037844387076, 1.000000000000000000, 0.8660254037844387076, 1.000000000000000000, 0.8660254037844387076, 1.000000000000000000, 0.8660254037844387076, 1.000000000000000000, 0.8660254037844387076, 1.000000000000000000, 0.8660254037844387076, 1.000000000000000000, 0.8660254037844387076, 1.000000000000000000, 0.8660254037844387076, 1.000000000000000000, 0.8660254037844387076, 1.000000000000000000, 0.8660254037844387076, 1.000000000000000000, 0.8660254037844387076, 1.000000000000000000, 0.8660254037844387076, 1.000000000000000000, 0.8660254037844387076, 1.000000000000000000, 0.8660254037844387076, 1.000000000000000000, 0.8660254037844387076, 1.000000000000000000, 0.8660254037844387076, 1.000000000000000000, 0.8660254037844387076, 1.000000000000000000, 0.8660254037844387076, 1.000000000000000000, 0.8660254037844387076, 1.000000000000000000, 0.8660254037844387076, 1.000000000000000000, 0.8660254037844387076, 1.000000000000000000, 0.8660254037844387076, 1.000000000000000000, 0.8660254037844387076, 1.000000000000000000, 0.8660254037844387076, 1.000000000000000000, 0.8660254037844387076, 1.000000000000000000, 0.8660254037844387076, 1.000000000000000000, 0.8660254037844387076, 1.000000000000000000, 0.8660254037844387076, 1.000000000000000000, 0.8660254037844387076, 1.000000000000000000, 0.8660254037844387076, 1.000000000000000000, 0.8660254037844387076, 1.000000000000000000, 0.8660254037844387076, 1.000000000000000000, 0.8660254037844387076, 1.000000000000000000, 0.8660254037844387076, 1.000000000000000000, 0.8660254037844387076, 1.000000000000000000, 0.8660254037844387076, 1.000000000000000000, 0.8660254037844387076, 1.000000000000000000, 0.8660254037844387076, 1.000000000000000000, 0.8660254037844387076, 1.000000000000000000, 0.8660254037844387076, 1.000000000000000000),
 ( 1.000000000000000000, 0.8660254037844387076, 1.000000000000000000, 0.8660254037844387076, 1.000000000000000000, 0.8660254037844387076, 1.000000000000000000, 0.8660254037844387076, 1.000000000000000000, 0.8660254037844387076, 1.000000000000000000, 0.8660254037844387076, 1.000000000000000000, 0.8660254037844387076, 1.000000000000000000, 0.8660254037844387076, 1.000000000000000000, 0.8660254037844387076, 1.000000000000000000, 0.8660254037844387076, 1.000000000000000000, 0.8660254037844387076, 1.000000000000000000, 0.8660254037844387076, 1.000000000000000000, 0.8660254037844387076, 1.000000000000000000, 0.8660254037844387076, 1.000000000000000000, 0.8660254037844387076, 1.000000000000000000, 0.8660254037844387076, 1.000000000000000000, 0.8660254037844387076, 1.000000000000000000, 0.8660254037844387076, 1.000000000000000000, 0.8660254037844387076, 1.000000000000000000, 0.8660254037844387076, 1.000000000000000000, 0.8660254037844387076, 1.000000000000000000, 0.8660254037844387076, 1.000000000000000000, 0.8660254037844387076, 1.000000000000000000, 0.8660254037844387076, 1.000000000000000000, 0.8660254037844387076, 1.000000000000000000, 0.8660254037844387076, 1.000000000000000000, 0.8660254037844387076, 1.000000000000000000, 0.8660254037844387076, 1.000000000000000000, 0.8660254037844387076, 1.000000000000000000, 0.8660254037844387076, 1.000000000000000000, 0.8660254037844387076, 1.000000000000000000, 0.8660254037844387076, 1.000000000000000000, 0.8660254037844387076, 1.000000000000000000, 0.8660254037844387076, 1.000000000000000000, 0.8660254037844387076, 1.000000000000000000, 0.8660254037844387076, 1.000000000000000000, 0.8660254037844387076, 1.000000000000000000, 0.8660254037844387076, 1.000000000000000000, 0.8660254037844387076, 1.000000000000000000, 0.8660254037844387076, 1.000000000000000000, 0.8660254037844387076, 1.000000000000000000, 0.8660254037844387076, 1.000000000000000000, 0.8660254037844387076, 1.000000000000000000, 0.8660254037844387076, 1.000000000000000000, 0.8660254037844387076, 1.000000000000000000, 0.8660254037844387076, 1.000000000000000000, 0.8660254037844387076, 1.000000000000000000, 0.8660254037844387076, 1.000000000000000000, 0.8660254037844387076, 1.000000000000000000, 0.8660254037844387076, 1.000000000000000000, 0.8660254037844387076, 1.000000000000000000, 0.8660254037844387076, 1.000000000000000000, 0.8660254037844387076, 1.000000000000000000, 0.8660254037844387076, 1.000000000000000000, 0.8660254037844387076, 1.000000000000000000, 0.8660254037844387076, 1.000000000000000000, 0.8660254037844387076, 1.000000000000000000, 0.8660254037844387076, 1.000000000000000000, 0.8660254037844387076, 1.000000000000000000, 0.8660254037844387076, 1.000000000000000000, 0.8660254037844387076, 1.000000000000000000, 0.8660254037844387076, 1.000000000000000000, 0.8660254037844387076, 1.000000000000000000, 0.8660254037844387076, 1.000000000000000000, 0.8660254037844387076, 1.000000000000000000, 0.8660254037844387076, 1.000000000000000000, 0.8660254037844387076, 1.000000000000000000, 0.8660254037844387076, 1.000000000000000000, 0.8660254037844387076, 1.000000000000000000, 0.8660254037844387076, 1.000000000000000000, 0.8660254037844387076, 1.000000000000000000, 0.8660254037844387076, 1.000000000000000000, 0.8660254037844387076, 1.000000000000000000, 0.8660254037844387076, 1.000000000000000000, 0.8660254037844387076, 1.000000000000000000, 0.8660254037844387076, 1.000000000000000000, 0.8660254037844387076, 1.000000000000000000, 0.8660254037844387076, 1.000000000000000000, 0.8660254037844387076, 1.000000000000000000, 0.8660254037844387076, 1.000000000000000000, 0.8660254037844387076, 1.000000000000000000, 0.8660254037844387076, 1.000000000000000000, 0.8660254037844387076, 1.000000000000000000, 0.8660254037844387076, 1.000000000000000000, 0.8660254037844387076, 1.000000000000000000, 0.8660254037844387076, 1.000000000000000000, 0.8660254037844387076, 1.000000000000000000, 0.8660254037844387076, 1.000000000000000000, 0.8660254037844387076, 1.000000000000000000, 0.8660254037844387076, 1.000000000000000000, 0.8660254037844387076, 1.000000000000000000, 0.8660254037844387076, 1.000000000000000000, 0.8660254037844387076, 1.000000000000000000, 0.8660254037844387076, 1.000000000000000000, 0.8660254037844387076, 1.000000000000000000, 0.8660254037844387076, 1.000000000000000000, 0.8660254037844387076, 1.000000000000000000, 0.8660254037844387076, 1.000000000000000000, 0.8660254037844387076, 1.000000000000000000, 0.8660254037844387076, 1.000000000000000000, 0.8660254037844387076, 1.000000000000000000, 0.8660254037844387076, 1.000000000000000000, 0.8660254037844387076, 1.000000000000000000, 0.8660254037844387076, 1.000000000000000000, 0.8660254037844387076, 1.000000000000000000, 0.8660254037844387076, 1.000000000000000000, 0.8660254037844387076, 1.000000000000000000, 0.8660254037844387076, 1.000000000000000000, 0.8660254037844387076, 1.000000000000000000, 0.8660254037844387076, 1.000000000000000000, 0.8660254037844387076, 1.000000000000000000, 0.8660254037844387076, 1.000000000000000000, 0.8660254037844387076, 1.000000000000000000, 0.8660254037844387076, 1.000000000000000000, 0.8660254037844387076, 1.000000000000000000, 0.8660254037844387076, 1.000000000000000000, 0.8660254037844387076, 1.000000000000000000, 0.8660254037844387076, 1.000000000000000000, 0.8660254037844387076, 1.000000000000000000, 0.8660254037844387076, 1.000000000000000000, 0.8660254037844387076, 1.000000000000000000, 0.8660254037844387076, 1.000000000000000000, 0.8660254037844387076, 1.000000000000000000, 0.8660254037844387076, 1.000000000000000000, 0.8660254037844387076, 1.000000000000000000, 0.8660254037844387076, 1.000000000000000000, 0.8660254037844387076, 1.000000000000000000, 0.8660254037844387076, 1.000000000000000000, 0.8660254037844387076, 1.000000000000000000, 0.8660254037844387076, 1.000000000000000000, 0.8660254037844387076, 1.000000000000000000, 0.8660254037844387076, 1.000000000000000000, 0.8660254037844387076, 1.000000000000000000, 0.8660254037844387076, 1.000000000000000000, 0.8660254037844387076, 1.000000000000000000, 0.8660254037844387076, 1.000000000000000000, 0.8660254037844387076, 1.000000000000000000, 0.8660254037844387076, 1.000000000000000000, 0.8660254037844387076, 1.000000000000000000, 0.8660254037844387076, 1.000000000000000000, 0.8660254037844387076, 1.000000000000000000, 0.8660254037844387076, 1.000000000000000000, 0.8660254037844387076, 1.000000000000000000, 0.8660254037844387076, 1.000000000000000000, 0.8660254037844387076, 1.000000000000000000, 0.8660254037844387076, 1.000000000000000000, 0.8660254037844387076, 1.000000000000000000, 0.8660254037844387076, 1.000000000000000000, 0.8660254037844387076, 1.000000000000000000, 0.8660254037844387076, 1.000000000000000000, 0.8660254037844387076, 1.000000000000000000, 0.8660254037844387076, 1.000000000000000000, 0.8660254037844387076, 1.000000000000000000, 0.8660254037844387076, 1.000000000000000000, 0.8660254037844387076, 1.000000000000000000, 0.8660254037844387076, 1.000000000000000000, 0.8660254037844387076, 1.000000000000000000, 0.8660254037844387076, 1.000000000000000000, 0.8660254037844387076, 1.000000000000000000, 0.8660254037844387076, 1.000000000000000000, 0.8660254037844387076, 1.000000000000000000, 0.8660254037844387076, 1.000000000000000000, 0.8660254037844387076, 1.000000000000000000, 0.8660254037844387076, 1.000000000000000000, 0.8660254037844387076, 1.000000000000000000, 0.8660254037844387076, 1.000000000000000000, 0.8660254037844387076, 1.000000000000000000, 0.8660254037844387076, 1.000000000000000000, 0.8660254037844387076, 1.000000000000000000, 0.8660254037844387076, 1.000000000000000000, 0.8660254037844387076, 1.000000000000000000, 0.8660254037844387076, 1.000000000000000000, 0.8660254037844387076, 1.000000000000000000, 0.8660254037844387076, 1.000000000000000000, 0.8660254037844387076, 1.000000000000000000, 0.8660254037844387076, 1.000000000000000000, 0.8660254037844387076, 1.000000000000000000, 0.8660254037844387076, 1.000000000000000000, 0.8660254037844387076, 1.000000000000000000, 0.8660254037844387076, 1.000000000000000000, 0.8660254037844387076, 1.000000000000000000, 0.8660254037844387076, 1.000000000000000000, 0.8660254037844387076, 1.000000000000000000, 0.8660254037844387076, 1.000000000000000000, 0.8660254037844387076, 1.000000000000000000, 0.8660254037844387076, 1.000000000000000000, 0.8660254037844387076, 1.000000000000000000, 0.8660254037844387076, 1.000000000000000000, 0.8660254037844387076, 1.000000000000000000, 0.8660254037844387076, 1.000000000000000000, 0.8660254037844387076, 1.000000000000000000, 0.8660254037844387076, 1.000000000000000000, 0.8660254037844387076, 1.000000000000000000, 0.8660254037844387076, 1.000000000000000000, 0.8660254037844387076, 1.000000000000000000, 0.8660254037844387076, 1.000000000000000000, 0.8660254037844387076, 1.000000000000000000, 0.8660254037844387076, 1.000000000000000000, 0.8660254037844387076, 1.000000000000000000, 0.8660254037844387076, 1.000000000000000000, 0.8660254037844387076, 1.000000000000000000, 0.8660254037844387076, 1.000000000000000000, 0.8660254037844387076, 1.000000000000000000, 0.8660254037844387076, 1.000000000000000000, 0.8660254037844387076, 1.000000000000000000, 0.8660254037844387076, 1.000000000000000000, 0.8660254037844387076, 1.000000000000000000, 0.8660254037844387076, 1.000000000000000000, 0.8660254037844387076, 1.000000000000000000, 0.8660254037844387076, 1.000000000000000000, 0.8660254037844387076, 1.000000000000000000, 0.8660254037844387076, 1.000000000000000000, 0.8660254037844387076, 1.000000000000000000, 0.8660254037844387076, 1.000000000000000000, 0.8660254037844387076, 1.000000000000000000, 0.8660254037844387076, 1.000000000000000000, 0.8660254037844387076, 1.000000000000000000, 0.8660254037844387076, 1.000000000000000000, 0.8660254037844387076, 1.000000000000000000, 0.8660254037844387076, 1.000000000000000000, 0.8660254037844387076, 1.000000000000000000, 0.8660254037844387076, 1.000000000000000000, 0.8660254037844387076, 1.000000000000000000, 0.8660254037844387076, 1.000000000000000000, 0.8660254037844387076, 1.000000000000000000, 0.8660254037844387076, 1.000000000000000000, 0.8660254037844387076, 1.000000000000000000, 0.8660254037844387076, 1.000000000000000000, 0.8660254037844387076, 1.000000000000000000, 0.8660254037844387076, 1.000000000000000000, 0.8660254037844387076, 1.000000000000000000, 0.8660254037844387076, 1.000000000000000000, 0.8660254037844387076, 1.000000000000000000, 0.8660254037844387076, 1.000000000000000000, 0.8660254037844387076, 1.000000000000000000, 0.8660254037844387076, 1.000000000000000000, 0.8660254037844387076, 1.000000000000000000, 0.8660254037844387076, 1.000000000000000000, 0.8660254037844387076, 1.000000000000000000, 0.8660254037844387076, 1.000000000000000000, 0.8660254037844387076, 1.000000000000000000, 0.8660254037844387076, 1.000000000000000000, 0.8660254037844387076, 1.000000000000000000, 0.8660254037844387076, 1.000000000000000000, 0.8660254037844387076, 1.000000000000000000, 0.8660254037844387076, 1.000000000000000000, 0.8660254037844387076, 1.000000000000000000, 0.8660254037844387076, 1.000000000000000000, 0.8660254037844387076, 1.000000000000000000, 0.8660254037844387076, 1.000000000000000000, 0.8660254037844387076, 1.000000000000000000, 0.8660254037844387076, 1.000000000000000000, 0.8660254037844387076, 1.000000000000000000, 0.8660254037844387076, 1.000000000000000000, 0.8660254037844387076, 1.000000000000000000, 0.8660254037844387076, 1.000000000000000000, 0.8660254037844387076, 1.000000000000000000, 0.8660254037844387076, 1.000000000000000000, 0.8660254037844387076, 1.000000000000000000, 0.8660254037844387076, 1.000000000000000000, 0.8660254037844387076, 1.000000000000000000, 0.8660254037844387076, 1.000000000000000000, 0.8660254037844387076, 1.000000000000000000, 0.8660254037844387076, 1.000000000000000000, 0.8660254037844387076, 1.000000000000000000, 0.8660254037844387076, 1.000000000000000000, 0.8660254037844387076, 1.000000000000000000, 0.8660254037844387076, 1.000000000000000000, 0.8660254037844387076, 1.000000000000000000, 0.8660254037844387076, 1.000000000000000000, 0.8660254037844387076, 1.000000000000000000, 0.8660254037844387076, 1.000000000000000000, 0.8660254037844387076, 1.000000000000000000, 0.8660254037844387076, 1.000000000000000000, 0.8660254037844387076, 1.000000000000000000, 0.8660254037844387076, 1.000000000000000000, 0.8660254037844387076, 1.000000000000000000, 0.8660254037844387076, 1.000000000000000000, 0.8660254037844387076, 1.000000000000000000, 0.8660254037844387076, 1.000000000000000000, 0.8660254037844387076, 1.000000000000000000, 0.8660254037844387076, 1.000000000000000000, 0.8660254037844387076, 1.000000000000000000, 0.8660254037844387076, 1.000000000000000000, 0.8660254037844387076, 1.000000000000000000, 0.8660254037844387076, 1.000000000000000000, 0.8660254037844387076, 1.000000000000000000, 0.8660254037844387076, 1.000000000000000000, 0.8660254037844387076, 1.000000000000000000, 0.8660254037844387076, 1.000000000000000000, 0.8660254037844387076, 1.000000000000000000, 0.8660254037844387076, 1.000000000000000000, 0.8660254037844387076, 1.000000000000000000, 0.8660254037844387076, 1.000000000000000000, 0.8660254037844387076, 1.000000000000000000, 0.8660254037844387076, 1.000000000000000000, 0.8660254037844387076, 1.000000000000000000, 0.8660254037844387076, 1.000000000000000000, 0.8660254037844387076, 1.000000000000000000, 0.8660254037844387076, 1.000000000000000000, 0.8660254037844387076, 1.000000000000000000, 0.8660254037844387076, 1.000000000000000000, 0.8660254037844387076, 1.000000000000000000, 0.8660254037844387076, 1.000000000000000000, 0.8660254037844387076, 1.000000000000000000, 0.8660254037844387076, 1.000000000000000000, 0.8660254037844387076, 1.000000000000000000, 0.8660254037844387076, 1.000000000000000000, 0.8660254037844387076, 1.000000000000000000, 0.8660254037844387076, 1.000000000000000000, 0.8660254037844387076, 1.000000000000000000, 0.8660254037844387076, 1.000000000000000000, 0.8660254037844387076, 1.000000000000000000, 0.8660254037844387076, 1.000000000000000000, 0.8660254037844387076, 1.000000000000000000, 0.8660254037844387076, 1.000000000000000000, 0.8660254037844387076, 1.000000000000000000, 0.8660254037844387076, 1.000000000000000000, 0.8660254037844387076, 1.000000000000000000, 0.8660254037844387076, 1.000000000000000000, 0.8660254037844387076, 1.000000000000000000, 0.8660254037844387076, 1.000000000000000000, 0.8660254037844387076, 1.000000000000000000, 0.8660254037844387076, 1.000000000000000000, 0.8660254037844387076, 1.000000000000000000, 0.8660254037844387076, 1.000000000000000000, 0.8660254037844387076, 1.000000000000000000, 0.8660254037844387076, 1.000000000000000000, 0.8660254037844387076, 1.000000000000000000, 0.8660254037844387076, 1.000000000000000000, 0.8660254037844387076, 1.000000000000000000, 0.8660254037844387076, 1.000000000000000000, 0.8660254037844387076, 1.000000000000000000, 0.8660254037844387076, 1.000000000000000000, 0.8660254037844387076, 1.000000000000000000, 0.8660254037844387076, 1.000000000000000000, 0.8660254037844387076, 1.000000000000000000, 0.8660254037844387076, 1.000000000000000000, 0.8660254037844387076, 1.000000000000000000, 0.8660254037844387076, 1.000000000000000000, 0.8660254037844387076, 1.000000000000000000, 0.8660254037844387076, 1.000000000000000000, 0.8660254037844387076, 1.000000000000000000, 0.8660254037844387076, 1.000000000000000000, 0.8660254037844387076, 1.000000000000000000, 0.8660254037844387076, 1.000000000000000000, 0.8660254037844387076, 1.000000000000000000, 0.8660254037844387076, 1.000000000000000000, 0.8660254037844387076, 1.000000000000000000, 0.8660254037844387076, 1.000000000000000000, 0.8660254037844387076, 1.000000000000000000, 0.8660254037844387076, 1.000000000000000000, 0.8660254037844387076, 1.000000000000000000, 0.8660254037844387076, 1.000000000000000000, 0.8660254037844387076, 1.000000000000000000, 0.8660254037844387076, 1.000000000000000000, 0.8660254037844387076, 1.000000000000000000, 0.8660254037844387076, 1.000000000000000000, 0.8660254037844387076, 1.000000000000000000, 0.8660254037844387076, 1.000000000000000000, 0.8660254037844387076, 1.000000000000000000, 0.8660254037844387076, 1.000000000000000000, 0.8660254037844387076, 1.000000000000000000, 0.8660254037844387076, 1.000000000000000000, 0.8660254037844387076, 1.000000000000000000, 0.8660254037844387076, 1.000000000000000000, 0.8660254037844387076, 1.000000000000000000, 0.8660254037844387076, 1.000000000000000000, 0.8660254037844387076, 1.000000000000000000, 0.8660254037844387076, 1.000000000000000000, 0.8660254037844387076, 1.000000000000000000, 0.8660254037844387076, 1.000000000000000000) ) ) 
 REPRESENTATION_ITEM ( '' )  SURFACE ( )  );
#68794=CARTESIAN_POINT ( 'NONE',  ( 33.57176175898906934, 184.0643266524159856, -9.188101187500093303 ) ) ;
#68795=CARTESIAN_POINT ( 'NONE',  ( 58.06412948370898164, 195.1423013555410080, -4.594050593750043987 ) ) ;
#68796=CARTESIAN_POINT ( 'NONE',  ( 196.0355168007595523, 291.1035201434990540, 17.55377893960077884 ) ) ;
#68799=CARTESIAN_POINT ( 'NONE',  ( -12.96825614257699755, 169.9865022471903160, 10.00000000000009237 ) ) ;
#68800=CARTESIAN_POINT ( 'NONE',  ( 51.75794814269726629, 206.8149278399160949, -9.188101187500095079 ) ) ;
#68801=AXIS2_PLACEMENT_3D ( 'NONE', #86904, #46316, #63038 ) ;
#68808=CARTESIAN_POINT ( 'NONE',  ( 159.7897726928491409, 253.8829904965402875, 16.83923858130328810 ) ) ;
#68809=CARTESIAN_POINT ( 'NONE',  ( 182.1727452308717830, 281.0742822384698911, -16.91150201624746785 ) ) ;
#68810=CARTESIAN_POINT ( 'NONE',  ( 149.6690105117817780, 275.3633762259814830, 7.431319680574127062 ) ) ;
#68812=( BOUNDED_CURVE ( )  B_SPLINE_CURVE ( 2, ( #67852, #98773, #60219, #70713, #48420, #26125, #33217, #47406, #3346 ),
 .UNSPECIFIED., .F., .T. ) 
 B_SPLINE_CURVE_WITH_KNOTS ( ( 3, 2, 2, 2, 3 ),
 ( 0.7701612903225806273, 0.7715053763440860024, 0.7741935483870967527, 0.7768817204301075030, 0.7782258064516128782 ),
 .UNSPECIFIED. ) 
 CURVE ( )  GEOMETRIC_REPRESENTATION_ITEM ( )  RATIONAL_B_SPLINE_CURVE ( ( 0.9330127018922194093, 0.9330127018922194093, 1.000000000000000000, 0.8660254037844387076, 1.000000000000000000, 0.8660254037844387076, 1.000000000000000000, 0.9330127018922194093, 0.9330127018922194093 ) ) 
 REPRESENTATION_ITEM ( '' )  );
#68815=CARTESIAN_POINT ( 'NONE',  ( 108.4196379545418125, 246.7365022471903444, 2.944929066748280225E-16 ) ) ;
#68816=CARTESIAN_POINT ( 'NONE',  ( 161.4025183475459073, 251.0896330829197041, 14.50747140106038735 ) ) ;
#68817=CARTESIAN_POINT ( 'NONE',  ( 193.8984187372643362, 285.0395281006325376, -16.96575577898347476 ) ) ;
#68820=VERTEX_POINT ( 'NONE', #85685 ) ;
#68821=CARTESIAN_POINT ( 'NONE',  ( 166.2218486525947583, 265.2797842516039282, 16.55497466531813089 ) ) ;
#68822=CARTESIAN_POINT ( 'NONE',  ( 194.2153129458476144, 293.5678207000269708, 14.48779561573898711 ) ) ;
#68824=EDGE_CURVE ( 'NONE', #74259, #76328, #88287, .T. ) ;
#68825=EDGE_LOOP ( 'NONE', ( #48687, #60116, #55624, #61926 ) ) ;
#68826=CARTESIAN_POINT ( 'NONE',  ( -22.42236680055709641, 157.8615022471902591, 0.000000000000000000 ) ) ;
#68828=CARTESIAN_POINT ( 'NONE',  ( 194.5252985417586729, 293.7192948986070178, -14.54632727629426370 ) ) ;
#68829=B_SPLINE_CURVE_WITH_KNOTS ( 'NONE', 3,
 ( #1370, #38846, #71278, #69751 ),
 .UNSPECIFIED., .F., .F.,
 ( 4, 4 ),
 ( 0.04862297438902305619, 0.04887066958154939050 ),
 .UNSPECIFIED. ) ;
#68831=FACE_OUTER_BOUND ( 'NONE', #34861, .T. ) ;
#68832=ORIENTED_EDGE ( 'NONE', *, *, #44670, .F. ) ;
#68836=CARTESIAN_POINT ( 'NONE',  ( 174.9422875208658184, 255.1437964849715456, 8.101495581286821235 ) ) ;
#68837=CYLINDRICAL_SURFACE ( 'NONE', #69917, 10.00000000000010658 ) ;
#68838=ORIENTED_EDGE ( 'NONE', *, *, #88176, .F. ) ;
#68839=CARTESIAN_POINT ( 'NONE',  ( 129.9777503372646095, 257.3967562850347122, -4.648177544792955347E-16 ) ) ;
#68840=FACE_OUTER_BOUND ( 'NONE', #89710, .T. ) ;
#68843=CARTESIAN_POINT ( 'NONE',  ( 174.5193691037453050, 286.1475687296140791, 10.49811431468850031 ) ) ;
#68846=CARTESIAN_POINT ( 'NONE',  ( 163.4178923001155681, 247.5989030008181260, -10.38047187240561442 ) ) ;
#68847=CARTESIAN_POINT ( 'NONE',  ( 204.9004517216375518, 275.7490024547470853, 14.55104398969427670 ) ) ;
#68848=CARTESIAN_POINT ( 'NONE',  ( 188.5315668109907961, 295.4050326786905316, -11.41571884897073552 ) ) ;
#68849=CARTESIAN_POINT ( 'NONE',  ( 161.2535912560966551, 263.0844709175967182, -17.80682751047658030 ) ) ;
#68850=CARTESIAN_POINT ( 'NONE',  ( 135.0589402170954827, 248.7833772461660544, -9.188101187500095079 ) ) ;
#68851=CARTESIAN_POINT ( 'NONE',  ( 176.5127557399464422, 269.0168359773951465, 16.11272065097649886 ) ) ;
#68852=CARTESIAN_POINT ( 'NONE',  ( 182.3555406741589877, 259.8314379914179426, 9.148843779236386808 ) ) ;
#68853=CARTESIAN_POINT ( 'NONE',  ( 79.63366147065640632, 204.5327760586659451, 1.948934522072303157E-15 ) ) ;
#68856=CARTESIAN_POINT ( 'NONE',  ( 184.8387315980094172, 297.9360420897670565, 2.319442688491891502 ) ) ;
#68857=ORIENTED_EDGE ( 'NONE', *, *, #17705, .F. ) ;
#68858=CARTESIAN_POINT ( 'NONE',  ( 161.5515493166768977, 252.8315038724842623, 14.92355679770252053 ) ) ;
#68859=VERTEX_POINT ( 'NONE', #54197 ) ;
#68862=CARTESIAN_POINT ( 'NONE',  ( 197.7352955435041792, 287.2275847242548821, 17.01394929260971978 ) ) ;
#68863=CARTESIAN_POINT ( 'NONE',  ( 146.8859094598974480, 276.2331372299326517, -0.7994986043261681496 ) ) ;
#68865=CARTESIAN_POINT ( 'NONE',  ( 154.8679462054080318, 262.4078440388265676, 17.98338675682672871 ) ) ;
#68866=CARTESIAN_POINT ( 'NONE',  ( 73.27344031762333998, 223.1115022471903160, -5.000000000000047962 ) ) ;
#68874=EDGE_CURVE ( 'NONE', #11051, #50774, #38688, .T. ) ;
#68876=CARTESIAN_POINT ( 'NONE',  ( 199.0034510736379048, 281.0923298783035875, 17.31675442061273529 ) ) ;
#68877=CARTESIAN_POINT ( 'NONE',  ( 193.9796946036068164, 292.6643086402947915, -15.64068455845557537 ) ) ;
#68878=CARTESIAN_POINT ( 'NONE',  ( 139.7406297344813311, 260.6744531367911009, 4.594050593750047540 ) ) ;
#68880=CARTESIAN_POINT ( 'NONE',  ( 0.5273063997305784678, 161.1115022471902023, -5.000000000000041744 ) ) ;
#68884=CARTESIAN_POINT ( 'NONE',  ( 201.4214977800931763, 281.7747274386935601, -17.04225209925078133 ) ) ;
#68890=CARTESIAN_POINT ( 'NONE',  ( 195.7435253745577484, 265.4158775244591197, 4.456225065319535439 ) ) ;
#68891=CARTESIAN_POINT ( 'NONE',  ( 77.44118756978804186, 225.5177522451419350, 5.000000000000046185 ) ) ;
#68896=CARTESIAN_POINT ( 'NONE',  ( 198.4613897724399862, 266.2157086906648260, 0.7828083158938100583 ) ) ;
#68899=CARTESIAN_POINT ( 'NONE',  ( 186.1523227505650482, 282.3592835991098582, 16.17628847161935468 ) ) ;
#68902=CARTESIAN_POINT ( 'NONE',  ( 207.6477529416552557, 270.9905371579805546, 7.447146952410988341 ) ) ;
#68903=CARTESIAN_POINT ( 'NONE',  ( 194.0672051292551430, 294.5127359636757660, 15.53337744471869364 ) ) ;
#68904=B_SPLINE_CURVE_WITH_KNOTS ( 'NONE', 3,
 ( #74397, #21182, #50069, #36353 ),
 .UNSPECIFIED., .F., .F.,
 ( 4, 4 ),
 ( 0.002991196628981945740, 0.01094109227149283985 ),
 .UNSPECIFIED. ) ;
#68908=CARTESIAN_POINT ( 'NONE',  ( 27.64472685218290238, 176.7677522451417929, -5.000000000000041744 ) ) ;
#68909=CARTESIAN_POINT ( 'NONE',  ( 166.1902696474969332, 285.7546370014056265, -3.171513238404533030 ) ) ;
#68912=CARTESIAN_POINT ( 'NONE',  ( 198.0792648159935538, 287.5636447432459022, 17.04758482866669667 ) ) ;
#68913=CARTESIAN_POINT ( 'NONE',  ( -13.97887943725652882, 171.9244531367911293, -4.594050593750046652 ) ) ;
#68915=ORIENTED_EDGE ( 'NONE', *, *, #77789, .F. ) ;
#68919=CARTESIAN_POINT ( 'NONE',  ( 5.858601742122021783, 180.3149278399161233, 9.188101187500093303 ) ) ;
#68922=CARTESIAN_POINT ( 'NONE',  ( 205.1793861064249711, 275.2658739283173759, -14.08953480709093675 ) ) ;
#68925=CARTESIAN_POINT ( 'NONE',  ( 179.1363749232007194, 255.1691260420666936, -3.970956364734916200 ) ) ;
#68926=CARTESIAN_POINT ( 'NONE',  ( 188.0010984285647453, 259.1527977912059555, -0.8004646550165761543 ) ) ;
#68928=CARTESIAN_POINT ( 'NONE',  ( 60.78824074639776143, 199.2365022471902307, 10.00000000000009592 ) ) ;
#68930=CARTESIAN_POINT ( 'NONE',  ( 189.9457600613112902, 301.6512882219586800, 0.04117870562599101891 ) ) ;
#68931=CARTESIAN_POINT ( 'NONE',  ( 14.70821206310299978, 188.4869531367911293, 4.594050593750046652 ) ) ;
#68935=CARTESIAN_POINT ( 'NONE',  ( 205.0859877718122561, 268.9368413191317586, -3.038556538008958974 ) ) ;
#68937=EDGE_CURVE ( 'NONE', #37468, #70599, #18731, .T. ) ;
#68938=CARTESIAN_POINT ( 'NONE',  ( 188.5872477108457019, 268.1141654234737643, 13.52445048591414434 ) ) ;
#68939=CARTESIAN_POINT ( 'NONE',  ( 163.2204695044033826, 281.0533932320078065, -10.15560040158997346 ) ) ;
#68940=CARTESIAN_POINT ( 'NONE',  ( 160.4256035324680454, 280.6369556960792124, 9.497879217036381050 ) ) ;
#68942=CARTESIAN_POINT ( 'NONE',  ( 148.1672759425158290, 274.0137453789218398, 7.847779094015780110 ) ) ;
#68945=CARTESIAN_POINT ( 'NONE',  ( 155.5660013421004919, 261.1987770755905558, 17.28709111629370199 ) ) ;
#68948=AXIS2_PLACEMENT_3D ( 'NONE', #35862, #50070, #73384 ) ;
#68949=CARTESIAN_POINT ( 'NONE',  ( 176.0893140685097364, 259.6469405521993394, 13.94800846836438879 ) ) ;
#68951=CARTESIAN_POINT ( 'NONE',  ( 148.7588072053147243, 273.7711778218048835, -8.803803025135483296 ) ) ;
#68954=ORIENTED_EDGE ( 'NONE', *, *, #57306, .T. ) ;
#68960=VERTEX_POINT ( 'NONE', #40995 ) ;
#68965=CARTESIAN_POINT ( 'NONE',  ( 191.5694459269389824, 298.8389818071599962, 7.944420692511652504 ) ) ;
#68970=CARTESIAN_POINT ( 'NONE',  ( 148.3930300673291640, 273.6227277647267897, 8.375036249079425232 ) ) ;
#68971=CARTESIAN_POINT ( 'NONE',  ( 149.4965729687386045, 271.7113353911534546, -11.48413836595348059 ) ) ;
#68972=ORIENTED_EDGE ( 'NONE', *, *, #91303, .F. ) ;
#68974=CARTESIAN_POINT ( 'NONE',  ( 195.8449251089225811, 291.4336346372613775, 16.14492769602857081 ) ) ;
#68989=CARTESIAN_POINT ( 'NONE',  ( 190.4281805785508084, 300.8157113754859893, -1.233909217199055774 ) ) ;
#68990=CARTESIAN_POINT ( 'NONE',  ( 190.2935937139882299, 301.0488226629397559, 4.649863831023156813 ) ) ;
#68991=CARTESIAN_POINT ( 'NONE',  ( 171.4241271215416020, 275.6058901121958229, -15.93988569491697938 ) ) ;
#68992=CARTESIAN_POINT ( 'NONE',  ( 146.9495969992948403, 276.1228271758872665, 0.7992850717744988120 ) ) ;
#68993=CARTESIAN_POINT ( 'NONE',  ( 146.8637854207107409, 276.2714571898724216, 0.7988785540157756770 ) ) ;
#68994=FACE_OUTER_BOUND ( 'NONE', #89507, .T. ) ;
#68998=CARTESIAN_POINT ( 'NONE',  ( 167.9052210226905970, 286.9632124721071591, 3.486985599330678198 ) ) ;
#69000=VERTEX_POINT ( 'NONE', #57704 ) ;
#69003=CARTESIAN_POINT ( 'NONE',  ( 173.2337249902883798, 270.7486416191997023, 17.82094672905207133 ) ) ;
#69005=CARTESIAN_POINT ( 'NONE',  ( 190.7685386727469279, 298.2261938635710976, -9.678376712886644029 ) ) ;
#69007=CARTESIAN_POINT ( 'NONE',  ( 168.6977591771627090, 286.2750216774235241, -7.847692359145494123 ) ) ;
#69009=CARTESIAN_POINT ( 'NONE',  ( 163.3409975114459485, 247.7320886816312111, -10.96358124877083640 ) ) ;
#69010=CARTESIAN_POINT ( 'NONE',  ( 206.3018347371251195, 273.3217358710584790, -9.309724106897926177 ) ) ;
#69012=CARTESIAN_POINT ( 'NONE',  ( 42.72800263476181470, 202.1427522451419350, 10.00000000000009237 ) ) ;
#69014=CARTESIAN_POINT ( 'NONE',  ( 124.8563387505838165, 233.7048013555409796, 4.594050593750051981 ) ) ;
#69016=CARTESIAN_POINT ( 'NONE',  ( 151.4428545556028780, 268.3402767968688067, -15.03309903163500749 ) ) ;
#69018=CARTESIAN_POINT ( 'NONE',  ( 196.4390255720217908, 290.4046224503736653, 16.34739044515864848 ) ) ;
#69019=CARTESIAN_POINT ( 'NONE',  ( 172.4760895491598092, 250.5888413570013711, -4.125262657830087498 ) ) ;
#69020=CARTESIAN_POINT ( 'NONE',  ( 42.23166870106845039, 201.3149278399160664, 9.188101187500093303 ) ) ;
#69022=CARTESIAN_POINT ( 'NONE',  ( 147.6309342515288847, 275.3284714954338028, -3.240618580837187235 ) ) ;
#69024=ORIENTED_EDGE ( 'NONE', *, *, #72281, .F. ) ;
#69026=CARTESIAN_POINT ( 'NONE',  ( 178.3097688579141220, 265.5568989673392366, 16.02486382646369023 ) ) ;
#69028=B_SPLINE_SURFACE_WITH_KNOTS ( 'NONE', 3, 1, ( 
 ( #55771, #54277 ),
 ( #47194, #8705 ),
 ( #85246, #15791 ),
 ( #85771, #62895 ),
 ( #78115, #46697 ),
 ( #1111, #24404 ),
 ( #71525, #55280 ),
 ( #78620, #9207 ),
 ( #71025, #86259 ),
 ( #94342, #16798 ),
 ( #40080, #10215 ),
 ( #24896, #86764 ),
 ( #17298, #63899 ),
 ( #79148, #94837 ),
 ( #48718, #40584 ),
 ( #25400, #56288 ),
 ( #69990, #39077 ),
 ( #87286, #17817 ),
 ( #79649, #72018 ),
 ( #57787, #82150 ),
 ( #81640, #72531 ),
 ( #95369, #11717 ),
 ( #43071, #27412 ),
 ( #88264, #58774 ),
 ( #49216, #50198 ),
 ( #88764, #18316 ),
 ( #27894, #64911 ),
 ( #19816, #58290 ),
 ( #4600, #3140 ),
 ( #34023, #95855 ),
 ( #4095, #74014 ),
 ( #43589, #73026 ),
 ( #42579, #56794 ),
 ( #2622, #35493 ) ),
 .UNSPECIFIED., .T., .F., .F.,
 ( 4, 2, 2, 2, 2, 2, 2, 2, 2, 2, 2, 2, 2, 2, 2, 2, 4 ),
 ( 2, 2 ),
 ( 0.000000000000000000, 0.06250000000000000000, 0.1250000000000000000, 0.1875000000000000000, 0.2500000000000000000, 0.3125000000000000000, 0.3750000000000000000, 0.4375000000000000000, 0.5000000000000000000, 0.5625000000000000000, 0.6250000000000000000, 0.6875000000000000000, 0.7500000000000000000, 0.8125000000000000000, 0.8750000000000000000, 0.9375000000000000000, 1.000000000000000000 ),
 ( 0.000000000000000000, 1.000000000000000000 ),
 .UNSPECIFIED. ) ;
#69032=CARTESIAN_POINT ( 'NONE',  ( 190.9559560067148425, 299.9015775189195665, -4.895152914295826108 ) ) ;
#69033=CARTESIAN_POINT ( 'NONE',  ( 151.9868571940785955, 278.2923008623533860, -1.631775907428277828 ) ) ;
#69035=CARTESIAN_POINT ( 'NONE',  ( 182.0568989607672563, 262.3880894348699258, 13.01387681392468032 ) ) ;
#69036=CARTESIAN_POINT ( 'NONE',  ( 105.0818317072414061, 238.1427522451419065, 10.00000000000009237 ) ) ;
#69037=CARTESIAN_POINT ( 'NONE',  ( 194.4068849611547876, 293.4209623680436039, -14.51840781236480815 ) ) ;
#69038=ORIENTED_EDGE ( 'NONE', *, *, #21458, .F. ) ;
#69039=CARTESIAN_POINT ( 'NONE',  ( 163.2442700311756596, 247.8996255919473697, 11.14021925110252020 ) ) ;
#69041=AXIS2_PLACEMENT_3D ( 'NONE', #68653, #22562, #15435 ) ;
#69042=CARTESIAN_POINT ( 'NONE',  ( 27.23877744593285755, 186.5333772461660544, 9.188101187500095079 ) ) ;
#69045=CARTESIAN_POINT ( 'NONE',  ( 195.0933036672505807, 273.3794171182236141, 14.45588861630873723 ) ) ;
#69048=CARTESIAN_POINT ( 'NONE',  ( 194.7402207200854605, 275.0729057474629258, -15.80694078002163927 ) ) ;
#69049=CARTESIAN_POINT ( 'NONE',  ( 65.07308872588301085, 214.5024278399160949, -9.188101187500093303 ) ) ;
#69050=CARTESIAN_POINT ( 'NONE',  ( 200.6129772034685175, 283.1751261563724142, 18.36811917402039640 ) ) ;
#69051=CARTESIAN_POINT ( 'NONE',  ( 55.79055247517715799, 193.0177522451417929, 5.000000000000051514 ) ) ;
#69053=ORIENTED_EDGE ( 'NONE', *, *, #27885, .T. ) ;
#69054=B_SPLINE_CURVE_WITH_KNOTS ( 'NONE', 3,
 ( #76126, #8197, #6197, #77087 ),
 .UNSPECIFIED., .F., .F.,
 ( 4, 4 ),
 ( 0.03237264616844526960, 0.04133669968024545477 ),
 .UNSPECIFIED. ) ;
#69057=CARTESIAN_POINT ( 'NONE',  ( 4.496589500409156948, 186.7365022471903444, 2.944929066748280225E-16 ) ) ;
#69059=CARTESIAN_POINT ( 'NONE',  ( 136.7095408212358052, 258.9244531367911577, -4.594050593750046652 ) ) ;
#69062=CARTESIAN_POINT ( 'NONE',  ( 174.6066048939933921, 262.0940252294753918, 15.79829227059981278 ) ) ;
#69066=DIRECTION ( 'NONE',  ( 0.8660254037844395958, 0.4999999999999985567, 0.000000000000000000 ) ) ;
#69067=EDGE_CURVE ( 'NONE', #3105, #4844, #75958, .T. ) ;
#69070=CARTESIAN_POINT ( 'NONE',  ( 150.6655900823359389, 269.6865383554857090, 15.31288044136207205 ) ) ;
#69071=CARTESIAN_POINT ( 'NONE',  ( 150.2076754159204484, 245.9824982072973683, 3.021315404115420679E-15 ) ) ;
#69072=CARTESIAN_POINT ( 'NONE',  ( 156.6715577256040035, 280.1715312555409128, -5.356107003133066868 ) ) ;
#69074=EDGE_LOOP ( 'NONE', ( #67762, #4867, #29071, #81802 ) ) ;
#69075=DIRECTION ( 'NONE',  ( 0.4999999999999998890, -0.8660254037844385966, 0.000000000000000000 ) ) ;
#69078=CARTESIAN_POINT ( 'NONE',  ( 157.6500260163024620, 257.5891404556457474, -18.23450497588216379 ) ) ;
#69080=ADVANCED_FACE ( 'NONE', ( #84423 ), #4019, .T. ) ;
#69081=CARTESIAN_POINT ( 'NONE',  ( 200.4906113350036776, 281.3870700576555919, -17.24871243658977704 ) ) ;
#69083=CARTESIAN_POINT ( 'NONE',  ( 188.6301707762981152, 265.0060877223691591, -12.46499516475016733 ) ) ;
#69084=CARTESIAN_POINT ( 'NONE',  ( 163.4139553296302267, 247.6057220337265505, -10.31482883765270842 ) ) ;
#69085=CARTESIAN_POINT ( 'NONE',  ( 152.7295469705997277, 266.1116601603806657, -17.40211458100010589 ) ) ;
#69086=CARTESIAN_POINT ( 'NONE',  ( 190.5057874690362212, 281.5141710404896571, 17.75392602039427459 ) ) ;
#69089=CARTESIAN_POINT ( 'NONE',  ( 190.7516742497373059, 300.2554039010641418, 4.342609251298632067 ) ) ;
#69090=CARTESIAN_POINT ( 'NONE',  ( 7.293129863248505984, 185.0177522451419065, 5.000000000000046185 ) ) ;
#69093=CARTESIAN_POINT ( 'NONE',  ( 162.8068419036826526, 250.8157941814552885, -13.07079287990798022 ) ) ;
#69095=CARTESIAN_POINT ( 'NONE',  ( 196.9319848161575806, 289.5507919934690335, -17.64330560362266453 ) ) ;
#69098=CARTESIAN_POINT ( 'NONE',  ( 110.0256537107753161, 225.1423013555409796, -4.594050593750043987 ) ) ;
#69099=CARTESIAN_POINT ( 'NONE',  ( 155.5050174552892486, 261.3044042659909110, 18.56563012484838282 ) ) ;
#69100=CIRCLE ( 'NONE', #14150, 17.82106496071138935 ) ;
#69101=CARTESIAN_POINT ( 'NONE',  ( 181.1059962512928507, 271.7445022709790123, -16.71226964961464390 ) ) ;
#69105=ORIENTED_EDGE ( 'NONE', *, *, #70380, .F. ) ;
#69106=VERTEX_POINT ( 'NONE', #20228 ) ;
#69111=CARTESIAN_POINT ( 'NONE',  ( 164.4698008747318738, 245.7769439046653019, -6.272955660526681854 ) ) ;
#69115=CARTESIAN_POINT ( 'NONE',  ( 170.6086979342741756, 283.5704196183729664, 12.42145073055875848 ) ) ;
#69116=EDGE_CURVE ( 'NONE', #19784, #49074, #51984, .T. ) ;
#69117=CARTESIAN_POINT ( 'NONE',  ( 147.6512387128590262, 274.9075480792844246, -8.209968531507987777 ) ) ;
#69119=CARTESIAN_POINT ( 'NONE',  ( 156.9694903541507074, 266.1758412851487492, -17.34135443527054576 ) ) ;
#69121=CARTESIAN_POINT ( 'NONE',  ( 198.3488621476923299, 277.3687303151504011, -15.33574521144890035 ) ) ;
#69126=CARTESIAN_POINT ( 'NONE',  ( 202.8787628851569593, 279.2506702366259788, 17.01435431865322556 ) ) ;
#69127=CARTESIAN_POINT ( 'NONE',  ( 185.6854299893530253, 258.0255741828406713, 3.062601813168996046 ) ) ;
#69129=CARTESIAN_POINT ( 'NONE',  ( 157.4371224504884594, 277.4660405788308140, -11.46929413857212410 ) ) ;
#69130=CARTESIAN_POINT ( 'NONE',  ( 200.6129772034685175, 283.1751261563724142, 18.36811917402039640 ) ) ;
#69131=CARTESIAN_POINT ( 'NONE',  ( 194.2393705908959305, 262.4612896885397504, -0.8107168165472325994 ) ) ;
#69132=CARTESIAN_POINT ( 'NONE',  ( 155.0127500294823051, 262.1570364583997161, -18.06877476110779668 ) ) ;
#69133=CIRCLE ( 'NONE', #83718, 17.82106496071138935 ) ;
#69135=CARTESIAN_POINT ( 'NONE',  ( 4.262040950003013862, 173.2677522451418781, 10.00000000000009592 ) ) ;
#69140=CARTESIAN_POINT ( 'NONE',  ( 168.7096392155106344, 280.2107777274362093, -14.47775774749160682 ) ) ;
#69143=CARTESIAN_POINT ( 'NONE',  ( -3.504777292649704279, 156.5327760586659451, 1.948934522072303157E-15 ) ) ;
#69145=CARTESIAN_POINT ( 'NONE',  ( 162.9933781180035339, 248.8079414735530008, 9.823679460557467991 ) ) ;
#69149=EDGE_CURVE ( 'NONE', #69588, #69000, #23559, .T. ) ;
#69151=DIRECTION ( 'NONE',  ( 0.4999999999999998890, -0.8660254037844385966, 0.000000000000000000 ) ) ;
#69152=ADVANCED_FACE ( 'NONE', ( #40758 ), #92767, .F. ) ;
#69153=CARTESIAN_POINT ( 'NONE',  ( 163.1000353707921704, 248.1494473519441044, -11.58334223833903920 ) ) ;
#69155=CARTESIAN_POINT ( 'NONE',  ( 150.1690433348657905, 276.5427391807701838, 3.674474410530066404 ) ) ;
#69156=CARTESIAN_POINT ( 'NONE',  ( 15.70964071017000663, 186.0024278399160949, -9.188101187500093303 ) ) ;
#69157=CARTESIAN_POINT ( 'NONE',  ( 118.6048046409561465, 227.0327760586659451, 1.948934522072303157E-15 ) ) ;
#69158=CARTESIAN_POINT ( 'NONE',  ( 182.0485676003057165, 294.3143584204422609, -6.380374882051434327 ) ) ;
#69159=CARTESIAN_POINT ( 'NONE',  ( 196.0359695149273591, 275.1637149607768151, 15.92387405639232867 ) ) ;
#69160=CARTESIAN_POINT ( 'NONE',  ( 151.0611737675045561, 272.2621515592074388, -11.66944463701014811 ) ) ;
#69165=CARTESIAN_POINT ( 'NONE',  ( 155.5204415533959548, 261.2776889444089647, 17.19127227448963424 ) ) ;
#69166=CARTESIAN_POINT ( 'NONE',  ( 207.1770866921659717, 271.8057550155037347, -5.569195235244989384 ) ) ;
#69168=CARTESIAN_POINT ( 'NONE',  ( 192.8228917618455398, 264.7295502452923870, 7.362112655479600143 ) ) ;
#69169=CARTESIAN_POINT ( 'NONE',  ( 164.8677655218696430, 249.8687689424382654, -10.55778266665861409 ) ) ;
#69170=CARTESIAN_POINT ( 'NONE',  ( 175.3859657801009178, 256.5741425621262124, -10.80191140654976500 ) ) ;
#69171=CARTESIAN_POINT ( 'NONE',  ( 146.9456733906991417, 276.1296230653242105, -0.7988785540157754550 ) ) ;
#69173=CARTESIAN_POINT ( 'NONE',  ( 181.2803014450269359, 265.8887025142350922, -15.50142388446617048 ) ) ;
#69176=AXIS2_PLACEMENT_3D ( 'NONE', #37384, #54072, #69291 ) ;
#69179=CARTESIAN_POINT ( 'NONE',  ( 96.60225995211651195, 217.3923013555410080, 4.594050593750050204 ) ) ;
#69181=CARTESIAN_POINT ( 'NONE',  ( 191.2729698983822288, 299.3524933518466469, 8.871011392605806734 ) ) ;
#69185=CARTESIAN_POINT ( 'NONE',  ( 191.7225392387177862, 276.9339074532402947, 17.14307201408091430 ) ) ;
#69186=DIRECTION ( 'NONE',  ( -0.8660254037844359321, -0.5000000000000051070, -0.000000000000000000 ) ) ;
#69187=CARTESIAN_POINT ( 'NONE',  ( 150.6916211261701619, 269.6414512649903941, -15.44346024757110847 ) ) ;
#69192=ORIENTED_EDGE ( 'NONE', *, *, #66773, .F. ) ;
#69195=CARTESIAN_POINT ( 'NONE',  ( 161.9632099598195509, 257.6781890077914454, 16.87053306877513847 ) ) ;
#69196=CARTESIAN_POINT ( 'NONE',  ( 196.7524321640172218, 268.0187694790326987, 9.426055234587533249 ) ) ;
#69197=CARTESIAN_POINT ( 'NONE',  ( 196.5114383562724072, 290.2791998289336561, -17.87308875047256862 ) ) ;
#69199=ORIENTED_EDGE ( 'NONE', *, *, #97284, .F. ) ;
#69202=CARTESIAN_POINT ( 'NONE',  ( 183.5350908500885510, 264.5469634027678580, -13.30375932693375773 ) ) ;
#69203=CARTESIAN_POINT ( 'NONE',  ( 169.5019237854968424, 251.7534625206462806, -8.423672671575513249 ) ) ;
#69206=ORIENTED_EDGE ( 'NONE', *, *, #55649, .T. ) ;
#69207=CARTESIAN_POINT ( 'NONE',  ( 188.1462912568056538, 279.3216201851784035, 16.80002852650974177 ) ) ;
#69209=ORIENTED_EDGE ( 'NONE', *, *, #7852, .F. ) ;
#69210=CARTESIAN_POINT ( 'NONE',  ( 167.6205390402564603, 249.8818047244939180, 6.913440952512820203 ) ) ;
#69211=CARTESIAN_POINT ( 'NONE',  ( 185.1680939005084383, 292.9008939279111132, -10.44728957843394568 ) ) ;
#69216=CARTESIAN_POINT ( 'NONE',  ( 192.7871527781657335, 296.7298516721106694, -12.00364781672877434 ) ) ;
#69217=CARTESIAN_POINT ( 'NONE',  ( 185.9800042062175862, 295.3878514961374435, 9.780988852953662160 ) ) ;
#69218=ADVANCED_FACE ( 'NONE', ( #65079 ), #77386, .F. ) ;
#69219=DIRECTION ( 'NONE',  ( -0.8660254037844387076, -0.4999999999999998890, -0.000000000000000000 ) ) ;
#69220=CARTESIAN_POINT ( 'NONE',  ( 110.3297989853572005, 246.0530062829863311, -4.648177544792955347E-16 ) ) ;
#69225=DIRECTION ( 'NONE',  ( 0.4999999999999998890, -0.8660254037844385966, 0.000000000000000000 ) ) ;
#69226=ORIENTED_EDGE ( 'NONE', *, *, #14087, .T. ) ;
#69229=CARTESIAN_POINT ( 'NONE',  ( 170.7208318451582443, 255.3949681855457925, -11.45774138149006660 ) ) ;
#69230=CARTESIAN_POINT ( 'NONE',  ( 185.3903474297596290, 282.1509521980658519, -17.39533353848089448 ) ) ;
#69238=CARTESIAN_POINT ( 'NONE',  ( 178.0352283463558081, 255.4622352572455384, 5.186437070723915355 ) ) ;
#69239=CARTESIAN_POINT ( 'NONE',  ( 110.4040191812834735, 243.7369531367911009, -4.594050593750048428 ) ) ;
#69240=CARTESIAN_POINT ( 'NONE',  ( 186.6446422895439525, 262.8178198450582386, -9.153827383837436216 ) ) ;
#69242=CARTESIAN_POINT ( 'NONE',  ( 188.8854333635352134, 273.8291574995095630, 15.67551265882508815 ) ) ;
#69245=CIRCLE ( 'NONE', #93583, 17.82106496071138935 ) ;
#69249=CARTESIAN_POINT ( 'NONE',  ( 192.8406302823137821, 296.6372259178641002, 11.87010547645091663 ) ) ;
#69251=CARTESIAN_POINT ( 'NONE',  ( 201.4066285247549786, 281.8004817444100354, -17.79749223817309201 ) ) ;
#69252=LINE ( 'NONE', #44453, #80401 ) ;
#69256=ORIENTED_EDGE ( 'NONE', *, *, #18130, .T. ) ;
#69259=ORIENTED_EDGE ( 'NONE', *, *, #86564, .F. ) ;
#69260=CARTESIAN_POINT ( 'NONE',  ( 189.4404814790326839, 266.9389309148366465, -11.88803597182145033 ) ) ;
#69262=CARTESIAN_POINT ( 'NONE',  ( 151.9683803660127808, 267.4300393925500998, -16.94882632825642332 ) ) ;
#69263=CARTESIAN_POINT ( 'NONE',  ( -4.759057006084864483, 161.3927522451417929, -10.00000000000009237 ) ) ;
#69265=CARTESIAN_POINT ( 'NONE',  ( 198.1641410069890696, 286.1601526949679055, 17.43024458236784824 ) ) ;
#69266=CARTESIAN_POINT ( 'NONE',  ( 156.8251583690820894, 280.2372100051578627, 5.906658021487110943 ) ) ;
#69267=CARTESIAN_POINT ( 'NONE',  ( 153.0444155045374544, 265.5662918618958201, -16.15173036748435109 ) ) ;
#69268=ORIENTED_EDGE ( 'NONE', *, *, #83228, .F. ) ;
#69269=CARTESIAN_POINT ( 'NONE',  ( 190.9380839614473473, 299.9325328093580652, -5.232187664503159752 ) ) ;
#69273=CARTESIAN_POINT ( 'NONE',  ( 148.6176504468695896, 246.6115022471902023, -5.000000000000041744 ) ) ;
#69274=CARTESIAN_POINT ( 'NONE',  ( 192.0969986600162827, 271.0201763999182845, -15.22553433325905736 ) ) ;
#69275=EDGE_CURVE ( 'NONE', #19179, #96323, #10901, .T. ) ;
#69276=CARTESIAN_POINT ( 'NONE',  ( 187.9556972102613486, 298.1788374127830252, -4.259537494478616182 ) ) ;
#69280=CARTESIAN_POINT ( 'NONE',  ( 191.2600711594267011, 283.4582610259524813, -16.58647876252101838 ) ) ;
#69284=CARTESIAN_POINT ( 'NONE',  ( 69.26781250152264136, 219.9869531367911293, 4.594050593750046652 ) ) ;
#69286=CARTESIAN_POINT ( 'NONE',  ( 147.2658550951450422, 275.5750520855697800, -5.215660180131691526 ) ) ;
#69289=CARTESIAN_POINT ( 'NONE',  ( 203.1044072055706806, 278.8598428092302584, -16.67109798570195878 ) ) ;
#69290=CARTESIAN_POINT ( 'NONE',  ( 161.8150574665248200, 250.3750943687383881, -13.25074899737357903 ) ) ;
#69291=DIRECTION ( 'NONE',  ( 0.4999999999999998890, -0.8660254037844385966, 0.000000000000000000 ) ) ;
#69293=DIRECTION ( 'NONE',  ( 0.4999999999999998890, -0.8660254037844385966, 0.000000000000000000 ) ) ;
#69296=CARTESIAN_POINT ( 'NONE',  ( 165.9646868419130215, 249.3316235501012272, -9.227677147359839793 ) ) ;
#69297=CARTESIAN_POINT ( 'NONE',  ( 204.8103939599436387, 275.9049870736169510, -13.21557707437574081 ) ) ;
#69298=CARTESIAN_POINT ( 'NONE',  ( 157.8849654228661166, 257.1822134667773980, 17.43614750057631468 ) ) ;
#69300=CARTESIAN_POINT ( 'NONE',  ( 23.50386934422995822, 190.5024278399160949, -9.188101187500093303 ) ) ;
#69301=B_SPLINE_CURVE_WITH_KNOTS ( 'NONE', 3,
 ( #74820, #35791, #21115, #29688 ),
 .UNSPECIFIED., .F., .F.,
 ( 4, 4 ),
 ( 0.01230808397153141873, 0.01852871432776161467 ),
 .UNSPECIFIED. ) ;
#69303=CARTESIAN_POINT ( 'NONE',  ( 51.40603854846860798, 209.6744531367911293, 4.594050593750047540 ) ) ;
#69304=CARTESIAN_POINT ( 'NONE',  ( 195.6914848190668863, 279.7035040353765680, -17.46620344769279853 ) ) ;
#69308=CARTESIAN_POINT ( 'NONE',  ( -7.266922234329370234, 156.6115022471902023, -5.000000000000041744 ) ) ;
#69309=DIRECTION ( 'NONE',  ( 0.4999999999999992784, -0.8660254037844390407, 0.000000000000000000 ) ) ;
#69311=CARTESIAN_POINT ( 'NONE',  ( 196.3531314006455091, 269.5910805997556849, -10.80433586473562713 ) ) ;
#69313=CARTESIAN_POINT ( 'NONE',  ( 198.5201458116119397, 286.8000164587433005, -18.30276554821096013 ) ) ;
#69316=CARTESIAN_POINT ( 'NONE',  ( 66.64328041388984047, 197.0327760586659736, 1.948934522072302763E-15 ) ) ;
#69320=CARTESIAN_POINT ( 'NONE',  ( 160.0105735053945182, 253.5005522708592594, 16.10371386499367929 ) ) ;
#69322=CARTESIAN_POINT ( 'NONE',  ( 149.1930131096921457, 275.4191784524399509, 7.566393461087619343 ) ) ;
#69323=CARTESIAN_POINT ( 'NONE',  ( 156.1857201963304362, 277.6936791020598889, 10.39727624116721749 ) ) ;
#69325=CARTESIAN_POINT ( 'NONE',  ( 112.6775961898153184, 245.8615022471903160, 5.000000000000046185 ) ) ;
#69326=CARTESIAN_POINT ( 'NONE',  ( 200.2316334480823912, 283.8356329158505105, 17.02791935830326508 ) ) ;
#69327=CARTESIAN_POINT ( 'NONE',  ( 207.0200405408487541, 272.0777669287182334, 6.494273599193515878 ) ) ;
#69328=EDGE_LOOP ( 'NONE', ( #41166, #74149, #44328, #61257, #15249, #21912, #40557, #41314, #78885, #11197, #46414, #43927, #73664, #76755, #40077, #14655, #17531, #5188, #78344, #8611, #10457 ) ) ;
#69332=CARTESIAN_POINT ( 'NONE',  ( 206.8106726053982811, 272.4404028303941914, -10.47827087991598560 ) ) ;
#69333=CARTESIAN_POINT ( 'NONE',  ( 186.9505214435809251, 276.6852383206837658, -16.96231179040420400 ) ) ;
#69336=ORIENTED_EDGE ( 'NONE', *, *, #87410, .T. ) ;
#69338=CARTESIAN_POINT ( 'NONE',  ( 147.9500839974939197, 274.3899328626944225, -9.375093207164509224 ) ) ;
#69340=EDGE_CURVE ( 'NONE', #81649, #31700, #40997, .T. ) ;
#69341=AXIS2_PLACEMENT_3D ( 'NONE', #27332, #73438, #65806 ) ;
#69342=ORIENTED_EDGE ( 'NONE', *, *, #97668, .T. ) ;
#69349=CARTESIAN_POINT ( 'NONE',  ( 161.9146335138334507, 283.9927115759381877, 5.150495195206919341 ) ) ;
#69350=ORIENTED_EDGE ( 'NONE', *, *, #68581, .F. ) ;
#69351=CARTESIAN_POINT ( 'NONE',  ( 171.0410219469655999, 285.1196576716371851, 11.19351320761253099 ) ) ;
#69352=CARTESIAN_POINT ( 'NONE',  ( 163.2409074158086639, 283.7204879113825768, -3.084300225432008435 ) ) ;
#69354=CARTESIAN_POINT ( 'NONE',  ( 208.3682389855799499, 269.7426187237583690, -1.431169231381201890 ) ) ;
#69355=CARTESIAN_POINT ( 'NONE',  ( 204.4781092559247782, 276.4805210635553863, 13.30606382016679490 ) ) ;
#69356=CARTESIAN_POINT ( 'NONE',  ( 159.6419305724666344, 254.1390605605417079, 16.92015248457581933 ) ) ;
#69357=CARTESIAN_POINT ( 'NONE',  ( 205.3704330671644414, 274.9349708856848338, -13.01557521325596944 ) ) ;
#69359=CARTESIAN_POINT ( 'NONE',  ( 140.0928864244750685, 245.5643266524160424, -9.188101187500093303 ) ) ;
#69360=CARTESIAN_POINT ( 'NONE',  ( 176.8005402467339024, 269.1829579716712715, 16.10165660169349877 ) ) ;
#69361=CARTESIAN_POINT ( 'NONE',  ( 178.7083948068321888, 257.8228082974438848, 9.925691156843040375 ) ) ;
#69362=CARTESIAN_POINT ( 'NONE',  ( 73.67938972387338481, 213.3458772461660544, 9.188101187500095079 ) ) ;
#69364=CARTESIAN_POINT ( 'NONE',  ( 150.8167050463783312, 269.4247995599803289, 14.38040671671637938 ) ) ;
#69367=CARTESIAN_POINT ( 'NONE',  ( 156.8626719559046876, 258.9528776918004382, -16.97501551230912042 ) ) ;
#69370=CARTESIAN_POINT ( 'NONE',  ( 186.6673878995319455, 276.5074556901925007, 17.73048906045012529 ) ) ;
#69372=CARTESIAN_POINT ( 'NONE',  ( 197.8876559304677585, 286.9678159391793884, 16.93603806477735318 ) ) ;
#69375=CARTESIAN_POINT ( 'NONE',  ( 155.5770330754656072, 261.1796695529068302, 18.26969263326161297 ) ) ;
#69377=CARTESIAN_POINT ( 'NONE',  ( 78.41572647264329987, 206.8923013555409796, 4.594050593750050204 ) ) ;
#69381=CARTESIAN_POINT ( 'NONE',  ( 201.0887433138568667, 282.3510750806604506, -17.79223670182895845 ) ) ;
#69383=VERTEX_POINT ( 'NONE', #10773 ) ;
#69385=CARTESIAN_POINT ( 'NONE',  ( 183.6431167994092561, 275.7377679000179569, 17.10282768236007556 ) ) ;
#69387=CARTESIAN_POINT ( 'NONE',  ( 205.8610808625997208, 274.0851439753691920, 10.38803237360972531 ) ) ;
#69388=CARTESIAN_POINT ( 'NONE',  ( 165.5245226950644053, 285.3287233769559066, 0.5282479373057951122 ) ) ;
#69389=CARTESIAN_POINT ( 'NONE',  ( 179.4037581149374034, 257.9870511612666064, -10.76565914641300736 ) ) ;
#69390=CARTESIAN_POINT ( 'NONE',  ( 154.7243163084728792, 268.4101332538514839, -16.32114699749692477 ) ) ;
#69391=AXIS2_PLACEMENT_3D ( 'NONE', #88916, #41732, #40217 ) ;
#69393=CARTESIAN_POINT ( 'NONE',  ( 188.7422858333208069, 294.9179404709084906, 11.58253606622573706 ) ) ;
#69394=CARTESIAN_POINT ( 'NONE',  ( 156.9440562780969231, 274.4750137900673508, 13.77464823823377316 ) ) ;
#69396=CARTESIAN_POINT ( 'NONE',  ( 200.7134601498536028, 283.0010845879393742, -16.98649239173277792 ) ) ;
#69400=CARTESIAN_POINT ( 'NONE',  ( 195.7220586188342111, 265.4108606537332662, 4.484546202810920867 ) ) ;
#69402=( BOUNDED_CURVE ( )  B_SPLINE_CURVE ( 2, ( #32297, #63200, #23189, #47987, #63702, #9520, #40380, #1912, #94638 ),
 .UNSPECIFIED., .F., .T. ) 
 B_SPLINE_CURVE_WITH_KNOTS ( ( 3, 2, 2, 2, 3 ),
 ( 0.01209677419354838850, 0.01344086021505376365, 0.01612903225806451568, 0.01881720430107526945, 0.02016129032258064807 ),
 .UNSPECIFIED. ) 
 CURVE ( )  GEOMETRIC_REPRESENTATION_ITEM ( )  RATIONAL_B_SPLINE_CURVE ( ( 0.9330127018922194093, 0.9330127018922194093, 1.000000000000000000, 0.8660254037844387076, 1.000000000000000000, 0.8660254037844387076, 1.000000000000000000, 0.9330127018922191873, 0.9330127018922192983 ) ) 
 REPRESENTATION_ITEM ( '' )  );
#69403=CARTESIAN_POINT ( 'NONE',  ( 181.5502188866845756, 292.0258448067215795, 10.54796749914566334 ) ) ;
#69404=CARTESIAN_POINT ( 'NONE',  ( 20.85854946042532276, 194.3967562850347122, -4.648177544792955347E-16 ) ) ;
#69407=CARTESIAN_POINT ( 'NONE',  ( 154.4723046951263825, 270.8738626539015968, 14.00925342371585636 ) ) ;
#69409=B_SPLINE_CURVE_WITH_KNOTS ( 'NONE', 3,
 ( #58514, #89486, #20046, #50917, #35726, #81867, #66625, #2861, #95593, #18546, #49427, #51422 ),
 .UNSPECIFIED., .F., .F.,
 ( 4, 2, 2, 2, 2, 4 ),
 ( 0.001587444564573364542, 0.001666700333226233842, 0.001745956101879103358, 0.001904467639184939535, 0.002221490713796634223, 0.002855536863020023165 ),
 .UNSPECIFIED. ) ;
#69411=CARTESIAN_POINT ( 'NONE',  ( 147.3984236761635884, 275.3454365677582700, 5.108566646342994844 ) ) ;
#69412=CARTESIAN_POINT ( 'NONE',  ( 162.6626107288841467, 248.9070890562113902, 10.12509462564867313 ) ) ;
#69413=CARTESIAN_POINT ( 'NONE',  ( 207.4285356523023154, 271.3702326410368642, 7.833982582429932506 ) ) ;
#69414=CARTESIAN_POINT ( 'NONE',  ( 194.2764122224708103, 294.1503786489221284, 15.46903869661980835 ) ) ;
#69417=CARTESIAN_POINT ( 'NONE',  ( 170.8843335314017509, 274.4719442773359219, 17.28596511953734449 ) ) ;
#69418=CARTESIAN_POINT ( 'NONE',  ( 163.2786353882781327, 283.8196446749163329, -3.634902129664387527 ) ) ;
#69420=CYLINDRICAL_SURFACE ( 'NONE', #78636, 17.82106496071139645 ) ;
#69421=CARTESIAN_POINT ( 'NONE',  ( 151.1255156751140873, 251.3927522451417929, -10.00000000000009059 ) ) ;
#69427=CARTESIAN_POINT ( 'NONE',  ( 23.17910981781079371, 190.3149278399160949, -9.188101187500095079 ) ) ;
#69428=CARTESIAN_POINT ( 'NONE',  ( 176.1700939719127064, 265.6259258544362751, -16.05018850396762176 ) ) ;
#69431=CARTESIAN_POINT ( 'NONE',  ( 72.26538907532096800, 200.9824982072973967, 3.021315404115420679E-15 ) ) ;
#69435=CARTESIAN_POINT ( 'NONE',  ( 71.90223342829800401, 218.9865022471902876, -10.00000000000009415 ) ) ;
#69438=CARTESIAN_POINT ( 'NONE',  ( 29.24128764430186322, 193.8149278399160664, 9.188101187500093303 ) ) ;
#69442=CARTESIAN_POINT ( 'NONE',  ( 198.9832789858017463, 285.9978462703757600, -18.55676541969546278 ) ) ;
#69443=CARTESIAN_POINT ( 'NONE',  ( 164.9779129355220562, 244.8968679994381148, -1.771286574179712803 ) ) ;
#69444=CARTESIAN_POINT ( 'NONE',  ( 155.2695601165254402, 261.7122283397445131, 16.98599069618989077 ) ) ;
#69445=CARTESIAN_POINT ( 'NONE',  ( 185.2204453182458508, 266.7228424648479859, 14.18578268008576337 ) ) ;
#69446=CARTESIAN_POINT ( 'NONE',  ( 161.3305864230751183, 279.4054883986951836, -9.803368587617336871 ) ) ;
#69447=CARTESIAN_POINT ( 'NONE',  ( 179.7260286473791666, 262.9842352772275262, -13.04977194216664849 ) ) ;
#69448=PRODUCT_CONTEXT ( 'NONE', #56961, 'mechanical' ) ;
#69452=EDGE_CURVE ( 'NONE', #86705, #43553, #89318, .T. ) ;
#69454=ORIENTED_EDGE ( 'NONE', *, *, #63101, .F. ) ;
#69458=CARTESIAN_POINT ( 'NONE',  ( 4.831432983919195401, 162.0494855054052152, -2.679491924311248496 ) ) ;
#69459=CARTESIAN_POINT ( 'NONE',  ( 155.7716105177659927, 262.8426515368366267, -17.72795275872529430 ) ) ;
#69461=CARTESIAN_POINT ( 'NONE',  ( 25.61604267474572083, 174.0494855054051584, -2.679491924311248496 ) ) ;
#69464=CARTESIAN_POINT ( 'NONE',  ( 181.2267447560696496, 257.4888273829192258, -7.641912445402520682 ) ) ;
#69467=CARTESIAN_POINT ( 'NONE',  ( 201.5074933251657399, 279.6257787853921286, 16.58790246189369100 ) ) ;
#69470=CARTESIAN_POINT ( 'NONE',  ( 190.9501423151522772, 299.9116471280854626, 8.746938802470586083 ) ) ;
#69474=ORIENTED_EDGE ( 'NONE', *, *, #8345, .F. ) ;
#69476=CARTESIAN_POINT ( 'NONE',  ( 190.5726849661229210, 300.5654224342945326, -0.2192718484028965964 ) ) ;
#69477=B_SPLINE_CURVE_WITH_KNOTS ( 'NONE', 3,
 ( #99794, #75005, #98812, #60261, #5095, #35976, #91217, #21780, #90475, #96574, #21044, #82378, #34718, #12948, #97549, #27642, #58507, #27139, #73732, #51925, #42798, #88490, #65617, #3833, #26630, #58990, #11941, #89480, #43809, #35721, #42309, #19052, #11453, #74749, #4841, #66619, #57514, #20039, #5329, #58024, #89006, #49926, #50912, #50416, #4318, #81374, #36207, #80884 ),
 .UNSPECIFIED., .F., .F.,
 ( 4, 2, 2, 2, 2, 2, 2, 2, 2, 2, 2, 2, 2, 2, 2, 2, 2, 2, 2, 2, 2, 2, 2, 4 ),
 ( 0.0001524510006530677771, 0.001166763548647211995, 0.001673919822644244016, 0.001800708891143506683, 0.001927497959642768917, 0.002054287028142031367, 0.002181076096641293600, 0.002434654233639839318, 0.002688232370638384168, 0.003195388644635474302, 0.004209701192629701841, 0.005224013740623929813, 0.005731170014621009105, 0.005984748151619504949, 0.006238326288618002528, 0.006301720822867608492, 0.006365115357117216190, 0.006491904425616409902, 0.006745482562614796458, 0.007252638836611600796, 0.007506216973610002965, 0.007759795110608406002, 0.008013373247606809038, 0.008266951384605210340 ),
 .UNSPECIFIED. ) ;
#69487=FACE_OUTER_BOUND ( 'NONE', #65973, .T. ) ;
#69495=CARTESIAN_POINT ( 'NONE',  ( 147.9748066657072627, 274.3471119452502762, 9.387104374042873900 ) ) ;
#69496=CARTESIAN_POINT ( 'NONE',  ( 190.7862358025146534, 300.1955415356651429, 3.573119809004446257 ) ) ;
#69497=CARTESIAN_POINT ( 'NONE',  ( 173.4808968322828946, 276.6942208921578867, -15.66287433468919943 ) ) ;
#69498=CARTESIAN_POINT ( 'NONE',  ( 191.7001674747973539, 298.6125654446252611, 8.448318027796386076 ) ) ;
#69499=CARTESIAN_POINT ( 'NONE',  ( 147.4563929227680603, 275.2450308873625886, -3.847749617713808412 ) ) ;
#69500=CARTESIAN_POINT ( 'NONE',  ( 190.0445576990143195, 301.4801656937889902, 4.140328216824785912 ) ) ;
#69507=CARTESIAN_POINT ( 'NONE',  ( 190.0410346281152272, 301.4862678315846551, -4.168183356896171254 ) ) ;
#69512=CARTESIAN_POINT ( 'NONE',  ( 180.1202963787140732, 282.9450741466765749, -15.29024642337825135 ) ) ;
#69513=DIRECTION ( 'NONE',  ( -0.8660254037844387076, -0.4999999999999998890, -0.000000000000000000 ) ) ;
#69515=EDGE_LOOP ( 'NONE', ( #65125, #98389, #27143, #93449 ) ) ;
#69516=CARTESIAN_POINT ( 'NONE',  ( 208.3699316049496133, 269.7396870210121733, -1.898463622294385811 ) ) ;
#69519=CARTESIAN_POINT ( 'NONE',  ( 41.06812061084161769, 204.5177522451419350, 5.000000000000046185 ) ) ;
#69520=CARTESIAN_POINT ( 'NONE',  ( 131.5951856977227123, 234.5327760586659451, 1.948934522072302763E-15 ) ) ;
#69521=CARTESIAN_POINT ( 'NONE',  ( 151.2646864780760723, 268.6488729594320830, -14.38346604407754548 ) ) ;
#69526=CARTESIAN_POINT ( 'NONE',  ( 196.1573359623355088, 290.8925231663144473, 17.55680092534192482 ) ) ;
#69527=CARTESIAN_POINT ( 'NONE',  ( 175.8386858396426646, 252.9025594026277304, -4.841821914686508244 ) ) ;
#69528=CARTESIAN_POINT ( 'NONE',  ( 54.70828104404427705, 193.2048013555409796, 4.594050593750051981 ) ) ;
#69537=CARTESIAN_POINT ( 'NONE',  ( 146.7845206192450007, 276.4087478532630939, 4.443586170796542945 ) ) ;
#69541=CARTESIAN_POINT ( 'NONE',  ( 178.2687518921240724, 261.3481827365934578, 12.71463598045219001 ) ) ;
#69542=CARTESIAN_POINT ( 'NONE',  ( 105.5870131927823792, 221.7677522451417929, -5.000000000000041744 ) ) ;
#69546=CARTESIAN_POINT ( 'NONE',  ( 202.8167949821795446, 279.3580017930215149, 15.61966256214195070 ) ) ;
#69549=CARTESIAN_POINT ( 'NONE',  ( 28.70002176693659379, 193.5024278399160949, -9.188101187500093303 ) ) ;
#69551=CARTESIAN_POINT ( 'NONE',  ( 195.9868235513005459, 273.6972693378553458, 14.73968791429838632 ) ) ;
#69554=CARTESIAN_POINT ( 'NONE',  ( 196.4846840357795088, 276.3116666789414353, -15.35900642488486945 ) ) ;
#69555=CARTESIAN_POINT ( 'NONE',  ( 72.70511114461589841, 212.7833772461660544, -9.188101187500095079 ) ) ;
#69556=CARTESIAN_POINT ( 'NONE',  ( 208.2175703429120688, 270.0035844679667889, 2.257951022351344150 ) ) ;
#69560=ORIENTED_EDGE ( 'NONE', *, *, #89108, .T. ) ;
#69561=B_SPLINE_CURVE_WITH_KNOTS ( 'NONE', 3,
 ( #18249, #49628, #57716, #11161 ),
 .UNSPECIFIED., .F., .F.,
 ( 4, 4 ),
 ( 0.03553003851185922851, 0.04427159934830902227 ),
 .UNSPECIFIED. ) ;
#69562=CARTESIAN_POINT ( 'NONE',  ( 18.71383987920370728, 191.6115022471903160, -5.000000000000047962 ) ) ;
#69563=CARTESIAN_POINT ( 'NONE',  ( 207.8725590214046406, 270.6011616060040410, 1.988011721677743093 ) ) ;
#69564=CARTESIAN_POINT ( 'NONE',  ( -7.131779314644562717, 172.8149278399161233, 9.188101187500093303 ) ) ;
#69566=CARTESIAN_POINT ( 'NONE',  ( 167.7808644153182911, 262.5190237135477673, -16.72764794300355717 ) ) ;
#69567=CARTESIAN_POINT ( 'NONE',  ( 189.2906976920214106, 261.6579632016146206, 6.676593444642060504 ) ) ;
#69568=CARTESIAN_POINT ( 'NONE',  ( 164.5813345449211624, 245.5837619211427523, 1.447064457712487373 ) ) ;
#69571=VERTEX_POINT ( 'NONE', #4149 ) ;
#69573=CARTESIAN_POINT ( 'NONE',  ( 145.8571944687587632, 255.0177522451418497, -10.00000000000009592 ) ) ;
#69577=CARTESIAN_POINT ( 'NONE',  ( 160.2542454754482151, 253.0785000383454815, 16.23321635550783881 ) ) ;
#69578=EDGE_CURVE ( 'NONE', #61965, #88529, #6035, .T. ) ;
#69579=CARTESIAN_POINT ( 'NONE',  ( 205.0520875136525376, 275.4863615587311756, -14.16385635411862509 ) ) ;
#69580=EDGE_CURVE ( 'NONE', #31573, #90058, #83414, .T. ) ;
#69582=CARTESIAN_POINT ( 'NONE',  ( 162.9383752892161397, 248.4294508267893491, -11.25953730674605957 ) ) ;
#69583=CARTESIAN_POINT ( 'NONE',  ( 153.2283961777204695, 265.2476279883323400, -17.66880461074566000 ) ) ;
#69586=CARTESIAN_POINT ( 'NONE',  ( 190.4730208157468212, 281.5709126222003533, 17.49935528176693111 ) ) ;
#69588=VERTEX_POINT ( 'NONE', #11774 ) ;
#69589=CARTESIAN_POINT ( 'NONE',  ( 149.1856130393175306, 272.2499337880290682, 11.44243872309708188 ) ) ;
#69590=CARTESIAN_POINT ( 'NONE',  ( 17.58976323311689782, 169.4155109091896065, 2.679491924311254714 ) ) ;
#69595=CARTESIAN_POINT ( 'NONE',  ( 146.5095091551180815, 276.8850816817948726, 0.1418322875769769398 ) ) ;
#69597=B_SPLINE_CURVE_WITH_KNOTS ( 'NONE', 3,
 ( #90932, #14383, #91918, #67072, #5289, #7263, #22474, #92411, #21482, #22960 ),
 .UNSPECIFIED., .F., .F.,
 ( 4, 3, 3, 4 ),
 ( 0.0009664718924630083313, 0.001498044977021742614, 0.004494154408225740742, 0.006233382939111537652 ),
 .UNSPECIFIED. ) ;
#69598=CARTESIAN_POINT ( 'NONE',  ( -27.42236680055714260, 166.5217562850347406, 1.224646799147364892E-15 ) ) ;
#69600=VERTEX_POINT ( 'NONE', #56849 ) ;
#69601=CARTESIAN_POINT ( 'NONE',  ( 203.5810809579637635, 278.0342196514508259, 16.28980717760872210 ) ) ;
#69602=CARTESIAN_POINT ( 'NONE',  ( 129.9259354818553902, 252.4865022471903160, 10.00000000000009415 ) ) ;
#69603=CARTESIAN_POINT ( 'NONE',  ( 150.6571681785161445, 269.7011255207979730, 15.24894850018880454 ) ) ;
#69605=ORIENTED_EDGE ( 'NONE', *, *, #83416, .T. ) ;
#69606=ADVANCED_FACE ( 'NONE', ( #35045 ), #68429, .F. ) ;
#69609=ORIENTED_EDGE ( 'NONE', *, *, #5103, .F. ) ;
#69611=ORIENTED_EDGE ( 'NONE', *, *, #48308, .F. ) ;
#69614=CARTESIAN_POINT ( 'NONE',  ( 163.7012083107868534, 247.1081852757374975, -6.544933039329257518 ) ) ;
#69616=CARTESIAN_POINT ( 'NONE',  ( 169.6649390567766886, 283.2330872627844656, 12.60183415381040106 ) ) ;
#69617=CARTESIAN_POINT ( 'NONE',  ( 194.8432095198904221, 293.1686569321988145, -14.74101036184996616 ) ) ;
#69619=CARTESIAN_POINT ( 'NONE',  ( 204.5265640781558432, 272.6391941324284289, -10.93223615312516195 ) ) ;
#69621=CARTESIAN_POINT ( 'NONE',  ( 163.6149864627186616, 282.5311289453194377, 8.575549053882928874 ) ) ;
#69623=CARTESIAN_POINT ( 'NONE',  ( 174.9671601572613326, 281.6994072225486434, -15.63500919100072473 ) ) ;
#69624=VERTEX_POINT ( 'NONE', #539 ) ;
#69626=CARTESIAN_POINT ( 'NONE',  ( 168.2119325052577778, 256.9784041376886421, -14.56702028336546384 ) ) ;
#69627=CARTESIAN_POINT ( 'NONE',  ( 159.6962080797732710, 254.0450491601782232, -15.33973334987084947 ) ) ;
#69630=CARTESIAN_POINT ( 'NONE',  ( 200.1444820856229967, 283.9865835035790269, 17.93386694781497326 ) ) ;
#69631=CARTESIAN_POINT ( 'NONE',  ( 158.6754561591581876, 281.3999859383739590, 2.074094494838789160 ) ) ;
#69632=EDGE_LOOP ( 'NONE', ( #30772, #35088, #58768 ) ) ;
#69633=CARTESIAN_POINT ( 'NONE',  ( 193.8226831119175984, 294.9362605212737662, -14.99963475610002739 ) ) ;
#69634=EDGE_CURVE ( 'NONE', #19800, #68024, #30068, .T. ) ;
#69636=CARTESIAN_POINT ( 'NONE',  ( -5.697251193518073187, 177.5177522451419350, 5.000000000000046185 ) ) ;
#69638=CARTESIAN_POINT ( 'NONE',  ( 87.45434598099585344, 230.4869531367911293, 4.594050593750046652 ) ) ;
#69639=CARTESIAN_POINT ( 'NONE',  ( 195.4769110598194573, 269.1066215422195000, -10.80299383076835618 ) ) ;
#69640=EDGE_CURVE ( 'NONE', #30521, #74797, #33681, .T. ) ;
#69642=CARTESIAN_POINT ( 'NONE',  ( 203.7394615857265023, 277.7598963572313551, -15.86198225853130417 ) ) ;
#69644=CARTESIAN_POINT ( 'NONE',  ( 15.73713787374454043, 170.7048013555409796, 4.594050593750051981 ) ) ;
#69646=CARTESIAN_POINT ( 'NONE',  ( 200.7583183585857967, 282.9233878912788214, 16.96937806979494212 ) ) ;
#69652=CARTESIAN_POINT ( 'NONE',  ( 162.4577219308423821, 249.2619668643215221, -10.67964597906097346 ) ) ;
#69655=CARTESIAN_POINT ( 'NONE',  ( 20.22912401222880519, 191.6744531367911293, 4.594050593750047540 ) ) ;
#69656=CARTESIAN_POINT ( 'NONE',  ( 131.5951856977227123, 234.5327760586659451, 1.948934522072303157E-15 ) ) ;
#69657=CARTESIAN_POINT ( 'NONE',  ( 183.1121120950856209, 257.7704774469726203, -2.388561198499064897 ) ) ;
#69658=ORIENTED_EDGE ( 'NONE', *, *, #84547, .F. ) ;
#69659=CARTESIAN_POINT ( 'NONE',  ( 153.4758031774517235, 274.2325035235903101, -12.14170705152958796 ) ) ;
#69660=B_SPLINE_CURVE_WITH_KNOTS ( 'NONE', 3,
 ( #77524, #9107, #39981, #71419, #1523, #93236, #87179, #85665, #94736, #47096, #54178, #40974, #24309, #94242, #39474, #2009, #56185, #17714, #8115, #1010, #62794, #48615, #79554, #10109, #85146, #27309, #89175, #49596, #96746, #41488, #88166, #4498, #3037, #4002, #74428, #80551, #10612, #58195, #12619, #82044, #96244, #35394, #87681, #56700, #57688, #95760, #97236, #19722, #34888, #18216 ),
 .UNSPECIFIED., .F., .F.,
 ( 4, 2, 2, 2, 2, 2, 2, 2, 2, 2, 2, 2, 2, 2, 2, 2, 2, 2, 2, 2, 2, 2, 2, 2, 4 ),
 ( 0.002713875006044959379, 0.003119435521400706294, 0.003220825650239643456, 0.003322215779078580618, 0.003423605907917517781, 0.003524996036756454943, 0.003727776294434217812, 0.003930556552111981114, 0.004336117067467507719, 0.005147238098178560928, 0.005958359128889613270, 0.006769480159600665611, 0.007580601190311718821, 0.007681991319150647743, 0.007732686383570167715, 0.007783381447989689422, 0.007834076512409211129, 0.007884771576828731102, 0.007986161705667788394, 0.008188941963345904712, 0.008391722221024021031, 0.008594502478702137349, 0.008797282736380253668, 0.009000062994058369986, 0.009202843251736486305 ),
 .UNSPECIFIED. ) ;
#69661=CARTESIAN_POINT ( 'NONE',  ( 175.2129986207789329, 281.2675690177629804, -15.37069089762922225 ) ) ;
#69664=CARTESIAN_POINT ( 'NONE',  ( -22.42236680055709641, 157.8615022471902591, 0.000000000000000000 ) ) ;
#69666=CARTESIAN_POINT ( 'NONE',  ( 207.5785076975260779, 271.1104734389944042, -6.824813054587777650 ) ) ;
#69668=CARTESIAN_POINT ( 'NONE',  ( 194.1852025340051284, 294.3083584634874796, -15.46421316575964688 ) ) ;
#69670=CARTESIAN_POINT ( 'NONE',  ( 167.7619341864813975, 278.3484540127419109, 14.70418198314342462 ) ) ;
#69673=CARTESIAN_POINT ( 'NONE',  ( 190.6071113721798156, 300.5057941498820924, -0.4754021072632813594 ) ) ;
#69677=AXIS2_PLACEMENT_3D ( 'NONE', #48808, #16885, #32594 ) ;
#69678=CARTESIAN_POINT ( 'NONE',  ( 163.7595992360150490, 247.0070492265414828, -6.976205010573520049 ) ) ;
#69679=CARTESIAN_POINT ( 'NONE',  ( 184.8703512676141827, 269.6233871522278491, 15.48342133112897123 ) ) ;
#69680=CARTESIAN_POINT ( 'NONE',  ( 107.7791399978856930, 233.0333772461660828, 9.188101187500095079 ) ) ;
#69682=CARTESIAN_POINT ( 'NONE',  ( 191.4484954869714954, 299.0484741143815199, 8.684991747358081327 ) ) ;
#69685=CARTESIAN_POINT ( 'NONE',  ( 195.3919583724417635, 278.7998134803532935, 16.31606295574663434 ) ) ;
#69686=DIRECTION ( 'NONE',  ( -0.8660254037844387076, -0.4999999999999998890, -0.000000000000000000 ) ) ;
#69687=CARTESIAN_POINT ( 'NONE',  ( 198.7829547491859330, 286.3448180261817129, -18.59838968157616179 ) ) ;
#69688=CARTESIAN_POINT ( 'NONE',  ( 139.4522149234842061, 257.9865022471903444, -10.00000000000009592 ) ) ;
#69693=CARTESIAN_POINT ( 'NONE',  ( 193.0262541023288918, 267.0219039627663165, 11.38476112752691982 ) ) ;
#69697=CARTESIAN_POINT ( 'NONE',  ( 196.8363552541316324, 289.7164272536036265, -17.80258609350122967 ) ) ;
#69703=CARTESIAN_POINT ( 'NONE',  ( 192.4202172926039793, 297.3654025762033370, 10.98569444949570872 ) ) ;
#69705=CARTESIAN_POINT ( 'NONE',  ( 190.0593414272333064, 280.4258356288787013, 16.63430549608987263 ) ) ;
#69707=ORIENTED_EDGE ( 'NONE', *, *, #16550, .T. ) ;
#69708=CARTESIAN_POINT ( 'NONE',  ( 166.6597750968865057, 249.2737811707126241, 6.985541172388376019 ) ) ;
#69709=CARTESIAN_POINT ( 'NONE',  ( 166.6845710576681654, 267.6039330892615453, -17.82176506903607915 ) ) ;
#69711=EDGE_CURVE ( 'NONE', #31470, #22323, #64845, .T. ) ;
#69713=CARTESIAN_POINT ( 'NONE',  ( 206.1870820878973518, 273.5204932898241168, 12.10889776728465961 ) ) ;
#69714=CARTESIAN_POINT ( 'NONE',  ( 153.3174834103889168, 265.0933243750448582, -17.43849572736497322 ) ) ;
#69722=CARTESIAN_POINT ( 'NONE',  ( 162.6827909417944227, 249.2597063335634004, 10.48648004974573311 ) ) ;
#69727=CARTESIAN_POINT ( 'NONE',  ( 170.6801095655508220, 269.8234966757721622, 16.62812258642549068 ) ) ;
#69730=CARTESIAN_POINT ( 'NONE',  ( 163.2919429874875448, 247.8170536094679903, 9.876785378511263147 ) ) ;
#69733=CARTESIAN_POINT ( 'NONE',  ( 192.6679047218190135, 296.9363953644068488, -13.34486378385621386 ) ) ;
#69734=CARTESIAN_POINT ( 'NONE',  ( 167.7899786429152584, 249.3113210190526559, -5.466766185341908724 ) ) ;
#69736=CARTESIAN_POINT ( 'NONE',  ( 183.4965467059954278, 284.4269586455677086, -15.20610756331047142 ) ) ;
#69737=CARTESIAN_POINT ( 'NONE',  ( 110.3232631693849726, 228.3768266524160140, 9.188101187500098632 ) ) ;
#69740=FACE_OUTER_BOUND ( 'NONE', #70896, .T. ) ;
#69741=ORIENTED_EDGE ( 'NONE', *, *, #91300, .T. ) ;
#69745=CARTESIAN_POINT ( 'NONE',  ( 171.1034016855470554, 287.7520123759660464, -4.697436788832531462 ) ) ;
#69746=CARTESIAN_POINT ( 'NONE',  ( 157.6286460899086137, 257.6261715744221306, 18.25526781158026779 ) ) ;
#69748=CARTESIAN_POINT ( 'NONE',  ( 153.4361244163197000, 264.8878321249116539, -17.23169627811277493 ) ) ;
#69749=CARTESIAN_POINT ( 'NONE',  ( 177.2134584772402093, 288.8126101685933236, -9.294799257062784648 ) ) ;
#69751=CARTESIAN_POINT ( 'NONE',  ( 153.4281311866982946, 266.9016768047333130, 16.59090889036721350 ) ) ;
#69755=CARTESIAN_POINT ( 'NONE',  ( 200.4592083165572092, 283.0503611105633013, -16.74591048218803735 ) ) ;
#69760=EDGE_CURVE ( 'NONE', #69588, #47527, #23536, .T. ) ;
#69761=CARTESIAN_POINT ( 'NONE',  ( 158.7649833156394550, 277.6848923185260105, 10.28015389956229342 ) ) ;
#69762=CARTESIAN_POINT ( 'NONE',  ( 193.0608394500619056, 263.6465134353720714, 4.469366988433737475 ) ) ;
#69763=CARTESIAN_POINT ( 'NONE',  ( 164.8705138155180521, 286.2009910768602481, -3.373684704351256780 ) ) ;
#69764=CARTESIAN_POINT ( 'NONE',  ( 165.8382246003566820, 285.1844245935532740, 7.589631688483079230 ) ) ;
#69765=CARTESIAN_POINT ( 'NONE',  ( 163.7170172071680554, 282.9345500121884811, -6.650731061596685478 ) ) ;
#69766=CARTESIAN_POINT ( 'NONE',  ( 160.8333331388420504, 281.5850016983533806, 5.638315465617829148 ) ) ;
#69767=CARTESIAN_POINT ( 'NONE',  ( 152.7375212135632125, 266.0978483664162582, -16.47968945089317572 ) ) ;
#69769=CARTESIAN_POINT ( 'NONE',  ( 146.9376205018946848, 276.1435710778808925, 5.066564108429441937 ) ) ;
#69771=CARTESIAN_POINT ( 'NONE',  ( 187.0789047048238558, 262.1108460767160295, -8.681453026525897343 ) ) ;
#69774=CARTESIAN_POINT ( 'NONE',  ( 24.59328401069779702, 196.5530062829863311, -4.648177544792955347E-16 ) ) ;
#69775=CARTESIAN_POINT ( 'NONE',  ( 188.5791505740767491, 298.5695105480600660, -4.259152367848529686 ) ) ;
#69777=CARTESIAN_POINT ( 'NONE',  ( 155.3017250444513024, 261.6565170503553190, 18.58368563027307374 ) ) ;
#69778=CARTESIAN_POINT ( 'NONE',  ( 191.1544238276611054, 283.3818065463574953, -16.58314240119747751 ) ) ;
#69780=CARTESIAN_POINT ( 'NONE',  ( 81.12205585946965414, 208.4548013555409796, -4.594050593750042211 ) ) ;
#69783=CARTESIAN_POINT ( 'NONE',  ( 60.73642589098854216, 194.3262482093457777, 3.021315404115420679E-15 ) ) ;
#69784=CARTESIAN_POINT ( 'NONE',  ( 203.3041373168503299, 278.5139001086923827, -16.61929732091214973 ) ) ;
#69785=DIRECTION ( 'NONE',  ( -0.8660254037844387076, -0.4999999999999998890, -0.000000000000000000 ) ) ;
#69791=CARTESIAN_POINT ( 'NONE',  ( 168.3799552507776696, 251.5246230850010534, -8.803241810830677139 ) ) ;
#69792=CARTESIAN_POINT ( 'NONE',  ( 164.0559412503519070, 246.4937698012927285, -5.533805667793892269 ) ) ;
#69793=CARTESIAN_POINT ( 'NONE',  ( 196.2048238403250764, 290.8102717488927169, 17.53926796892840656 ) ) ;
#69796=CARTESIAN_POINT ( 'NONE',  ( 47.67182463829572470, 189.1423013555410080, -4.594050593750043987 ) ) ;
#69798=CARTESIAN_POINT ( 'NONE',  ( 57.27886009182306282, 210.0024278399160949, -9.188101187500093303 ) ) ;
#69799=CARTESIAN_POINT ( 'NONE',  ( 163.9339498312803585, 247.2367830492466112, -6.562094630368194181 ) ) ;
#69801=CARTESIAN_POINT ( 'NONE',  ( 164.8422622293784627, 258.6706822939664789, 15.55324439361764277 ) ) ;
#69802=CARTESIAN_POINT ( 'NONE',  ( 141.5809337175232940, 261.7369531367911009, -4.594050593750048428 ) ) ;
#69804=CARTESIAN_POINT ( 'NONE',  ( 196.3172732138167191, 269.3125600491860041, -10.61832308323725549 ) ) ;
#69806=CARTESIAN_POINT ( 'NONE',  ( 135.5370584069941913, 242.3927522451417360, -10.00000000000009237 ) ) ;
#69809=CARTESIAN_POINT ( 'NONE',  ( 61.04057116557046925, 215.2369531367911009, -4.594050593750048428 ) ) ;
#69811=CARTESIAN_POINT ( 'NONE',  ( 154.8545429534089237, 262.4310591522755089, -17.81746354318405778 ) ) ;
#69812=CARTESIAN_POINT ( 'NONE',  ( 197.8977219949227049, 287.8780861330898801, 17.48564646125164046 ) ) ;
#69813=CARTESIAN_POINT ( 'NONE',  ( 59.15898261476995401, 193.4155109091896065, 2.679491924311254714 ) ) ;
#69814=CARTESIAN_POINT ( 'NONE',  ( 153.1683959517632729, 276.7515984265086786, 7.179112260468418327 ) ) ;
#69818=CARTESIAN_POINT ( 'NONE',  ( 103.2234855318351947, 243.7365022471903444, 2.944929066748280225E-16 ) ) ;
#69820=CARTESIAN_POINT ( 'NONE',  ( 206.9059968923335475, 272.2752963222270068, 6.902135944297345560 ) ) ;
#69825=CARTESIAN_POINT ( 'NONE',  ( 206.4484807199597753, 273.0677375780628608, -9.220527398138528952 ) ) ;
#69826=CARTESIAN_POINT ( 'NONE',  ( 188.1954655760533797, 277.4481781369921123, -16.60034468329214263 ) ) ;
#69827=DIRECTION ( 'NONE',  ( -0.8660254037844387076, -0.4999999999999998890, -0.000000000000000000 ) ) ;
#69832=CARTESIAN_POINT ( 'NONE',  ( 194.9757425430702824, 292.9391030023704161, -15.21392314336593365 ) ) ;
#69841=CARTESIAN_POINT ( 'NONE',  ( 159.7692415128758228, 253.9185515433934768, -16.85856106119654285 ) ) ;
#69844=CARTESIAN_POINT ( 'NONE',  ( 174.2237003172097332, 285.9827261121123456, 10.49758392901496329 ) ) ;
#69848=CARTESIAN_POINT ( 'NONE',  ( 164.4294002498235159, 245.8469198396639399, 6.098783631055905374 ) ) ;
#69849=EDGE_CURVE ( 'NONE', #6423, #55638, #57890, .T. ) ;
#69851=CARTESIAN_POINT ( 'NONE',  ( 204.9184781223158609, 275.7177798128946620, -12.59106622113254126 ) ) ;
#69852=CARTESIAN_POINT ( 'NONE',  ( 141.2025682470151366, 243.1423013555409796, -4.594050593750043987 ) ) ;
#69853=CARTESIAN_POINT ( 'NONE',  ( 206.5477884165873377, 270.4809506326999440, 3.067131091788421582 ) ) ;
#69854=CARTESIAN_POINT ( 'NONE',  ( 181.6318543639017662, 260.2046728290346209, 9.493342775386514276 ) ) ;
#69855=CARTESIAN_POINT ( 'NONE',  ( 68.21243081460160340, 216.3149278399160664, 9.188101187500093303 ) ) ;
#69857=CARTESIAN_POINT ( 'NONE',  ( 190.9907605556751093, 299.8412942717858414, 8.799173206188184437 ) ) ;
#69858=CARTESIAN_POINT ( 'NONE',  ( 199.5820190223589066, 281.0610403850588455, -17.29246150691365358 ) ) ;
#69861=CARTESIAN_POINT ( 'NONE',  ( 157.2289892027454528, 258.3183976085836662, -18.38247659754729924 ) ) ;
#69862=ORIENTED_EDGE ( 'NONE', *, *, #14654, .T. ) ;
#69865=CARTESIAN_POINT ( 'NONE',  ( 191.8232488616404225, 298.3993822291468518, -9.342381338555176384 ) ) ;
#69868=CARTESIAN_POINT ( 'NONE',  ( 56.67693180720107193, 191.9824982072973967, 3.021315404115420679E-15 ) ) ;
#69870=CARTESIAN_POINT ( 'NONE',  ( 77.38680066200176100, 224.6744531367911293, 4.594050593750047540 ) ) ;
#69871=VERTEX_POINT ( 'NONE', #47727 ) ;
#69874=CARTESIAN_POINT ( 'NONE',  ( 200.3340733048875393, 283.6582018791440873, -17.27431918982609460 ) ) ;
#69875=ORIENTED_EDGE ( 'NONE', *, *, #31857, .T. ) ;
#69878=CARTESIAN_POINT ( 'NONE',  ( 164.3754245770190039, 245.9404084473339083, 1.667926061651832992 ) ) ;
#69879=CARTESIAN_POINT ( 'NONE',  ( 162.2653288181836047, 284.9971543465875925, 0.5418273949422370839 ) ) ;
#69880=DIRECTION ( 'NONE',  ( -0.8660254037844382635, -0.5000000000000006661, 0.000000000000000000 ) ) ;
#69881=CARTESIAN_POINT ( 'NONE',  ( 160.2559598273567190, 260.1138223702041614, 16.66839514798089184 ) ) ;
#69884=CARTESIAN_POINT ( 'NONE',  ( 188.8294196202719206, 294.9100790419620921, 11.53803975672503235 ) ) ;
#69885=CARTESIAN_POINT ( 'NONE',  ( 185.3082215061529325, 260.2536058253289752, 6.219936519710626222 ) ) ;
#69887=CARTESIAN_POINT ( 'NONE',  ( 152.6692142062575499, 266.2161595735824449, -16.77985299603479419 ) ) ;
#69890=ORIENTED_EDGE ( 'NONE', *, *, #16924, .T. ) ;
#69891=FACE_OUTER_BOUND ( 'NONE', #59952, .T. ) ;
#69894=CARTESIAN_POINT ( 'NONE',  ( 187.2381800466000925, 265.7314477490792797, -11.83692723186113938 ) ) ;
#69895=CARTESIAN_POINT ( 'NONE',  ( 198.5136947552106221, 266.2255384214813603, 1.040791414451307295 ) ) ;
#69896=CARTESIAN_POINT ( 'NONE',  ( 152.8435137206748777, 271.1131880070238935, 14.11897916978259993 ) ) ;
#69897=ORIENTED_EDGE ( 'NONE', *, *, #72885, .F. ) ;
#69902=CARTESIAN_POINT ( 'NONE',  ( 155.6559071247401960, 261.0430556921643870, 17.79853447468815375 ) ) ;
#69904=CARTESIAN_POINT ( 'NONE',  ( 176.1208302163809662, 285.3140190418353086, -12.11730431473343295 ) ) ;
#69906=CARTESIAN_POINT ( 'NONE',  ( 188.0775634319173832, 267.1413101313072502, 14.31780989748781252 ) ) ;
#69908=CARTESIAN_POINT ( 'NONE',  ( 190.6996816925783946, 262.0116268005010056, 2.896814088563383294 ) ) ;
#69909=CARTESIAN_POINT ( 'NONE',  ( 148.5274394637607998, 249.8927522451418213, -10.00000000000009059 ) ) ;
#69911=VERTEX_POINT ( 'NONE', #39616 ) ;
#69912=FACE_OUTER_BOUND ( 'NONE', #9094, .T. ) ;
#69916=CARTESIAN_POINT ( 'NONE',  ( 20.41882739113040302, 182.5958772461660544, -9.188101187500095079 ) ) ;
#69917=AXIS2_PLACEMENT_3D ( 'NONE', #30349, #61235, #92199 ) ;
#69918=CARTESIAN_POINT ( 'NONE',  ( 181.9536094017156813, 275.8212133861905500, -16.44258783804268376 ) ) ;
#69921=CARTESIAN_POINT ( 'NONE',  ( 173.4026771546767804, 273.2456497557084845, -17.70700034978624515 ) ) ;
#69923=CARTESIAN_POINT ( 'NONE',  ( 186.8262740501982080, 295.8231315473516929, -8.285001673899497376 ) ) ;
#69925=CARTESIAN_POINT ( 'NONE',  ( 183.0976892694797868, 295.7619773535599279, 1.283268163629483816 ) ) ;
#69926=CARTESIAN_POINT ( 'NONE',  ( 62.88113547221012567, 207.1115022471902307, 10.00000000000009592 ) ) ;
#69928=CARTESIAN_POINT ( 'NONE',  ( 205.1661410800912506, 270.9228951919408814, 6.078262840308254589 ) ) ;
#69929=CARTESIAN_POINT ( 'NONE',  ( 28.37526224051743284, 193.3149278399160949, -9.188101187500095079 ) ) ;
#69932=CARTESIAN_POINT ( 'NONE',  ( 151.0013883899287066, 269.1049186256390726, -14.25461351222133466 ) ) ;
#69934=CARTESIAN_POINT ( 'NONE',  ( 193.9966098916996771, 294.6350105018939871, 13.97117019253516013 ) ) ;
#69936=CARTESIAN_POINT ( 'NONE',  ( 88.42888488385111145, 211.8615022471902023, 5.000000000000051514 ) ) ;
#69937=CARTESIAN_POINT ( 'NONE',  ( 159.9066067912097537, 278.3881009423306523, -10.16859343533022120 ) ) ;
#69942=CARTESIAN_POINT ( 'NONE',  ( 99.93749413994396491, 240.0530062829862743, -4.648177544792955347E-16 ) ) ;
#69944=ORIENTED_EDGE ( 'NONE', *, *, #7592, .F. ) ;
#69949=ORIENTED_EDGE ( 'NONE', *, *, #93373, .T. ) ;
#69950=CARTESIAN_POINT ( 'NONE',  ( 172.4831635826484444, 290.8796410925290843, -1.652085212636280609 ) ) ;
#69952=EDGE_CURVE ( 'NONE', #37573, #33225, #28814, .T. ) ;
#69956=EDGE_LOOP ( 'NONE', ( #21189, #30471, #10060, #27374 ) ) ;
#69958=CARTESIAN_POINT ( 'NONE',  ( 186.3691305807677168, 272.1350040206665426, -16.09258582117654868 ) ) ;
#69961=CARTESIAN_POINT ( 'NONE',  ( 151.2057546125658973, 268.7509459446807227, 15.78031848731319187 ) ) ;
#69965=B_SPLINE_CURVE_WITH_KNOTS ( 'NONE', 3,
 ( #74248, #58984, #13433, #59488 ),
 .UNSPECIFIED., .F., .F.,
 ( 4, 4 ),
 ( 0.01596741559801433119, 0.02157542978236621015 ),
 .UNSPECIFIED. ) ;
#69966=CARTESIAN_POINT ( 'NONE',  ( 148.4016473149517594, 273.6078022540229426, 8.470066617688926769 ) ) ;
#69967=EDGE_CURVE ( 'NONE', #30385, #61372, #9450, .T. ) ;
#69968=ORIENTED_EDGE ( 'NONE', *, *, #75861, .F. ) ;
#69971=VERTEX_POINT ( 'NONE', #92388 ) ;
#69973=CARTESIAN_POINT ( 'NONE',  ( 149.6676065383367416, 271.4150965588098074, 11.80358707172367261 ) ) ;
#69977=CARTESIAN_POINT ( 'NONE',  ( 159.9612433783809990, 254.2824735748564535, 15.35173791718965752 ) ) ;
#69978=CARTESIAN_POINT ( 'NONE',  ( 197.9723018751917039, 287.7489099912414758, 17.92592712455262571 ) ) ;
#69982=( BOUNDED_CURVE ( )  B_SPLINE_CURVE ( 2, ( #47591, #1519, #17191, #2519, #10609, #33401, #95757, #48092, #9623 ),
 .UNSPECIFIED., .F., .T. ) 
 B_SPLINE_CURVE_WITH_KNOTS ( ( 3, 2, 2, 2, 3 ),
 ( 0.1008064516129032334, 0.1021505376344086086, 0.1048387096774193589, 0.1075268817204301092, 0.1088709677419354843 ),
 .UNSPECIFIED. ) 
 CURVE ( )  GEOMETRIC_REPRESENTATION_ITEM ( )  RATIONAL_B_SPLINE_CURVE ( ( 0.9330127018922192983, 0.9330127018922196314, 1.000000000000000000, 0.8660254037844387076, 1.000000000000000000, 0.8660254037844387076, 1.000000000000000000, 0.9330127018922194093, 0.9330127018922194093 ) ) 
 REPRESENTATION_ITEM ( '' )  );
#69985=CARTESIAN_POINT ( 'NONE',  ( 147.0538900202505488, 275.9421863647172017, 5.192507380313251986 ) ) ;
#69986=CARTESIAN_POINT ( 'NONE',  ( 148.3707431749605234, 273.6613297946520902, 8.912574527564540716 ) ) ;
#69988=CARTESIAN_POINT ( 'NONE',  ( 149.7119746935222793, 271.3382486597900538, 12.05352563709836922 ) ) ;
#69989=CARTESIAN_POINT ( 'NONE',  ( 157.4655681218829670, 259.9086309006383431, -17.75190047967350893 ) ) ;
#69990=CARTESIAN_POINT ( 'NONE',  ( 207.1572261440131797, 271.8401544939704877, -5.633070628900782140 ) ) ;
#69991=CARTESIAN_POINT ( 'NONE',  ( 146.7943851877206214, 276.3916619194686746, -4.608908220452185844 ) ) ;
#69992=CARTESIAN_POINT ( 'NONE',  ( 160.0211798425829670, 255.5694664316391425, 16.22702261962307091 ) ) ;
#69999=CARTESIAN_POINT ( 'NONE',  ( 104.0442318961827652, 237.0024278399160949, -9.188101187500093303 ) ) ;
#70001=CARTESIAN_POINT ( 'NONE',  ( 147.2784190576484491, 275.5532906641692534, 0.2793038414862047958 ) ) ;
#70005=CARTESIAN_POINT ( 'NONE',  ( 155.2922060645262263, 261.6730044072216401, -16.98884022075611355 ) ) ;
#70006=CARTESIAN_POINT ( 'NONE',  ( 192.6212972830795707, 296.5656100641699595, 11.48306352210076220 ) ) ;
#70008=CARTESIAN_POINT ( 'NONE',  ( 169.0232498750005163, 285.7081439545306694, -7.538763084472316578 ) ) ;
#70010=CARTESIAN_POINT ( 'NONE',  ( 162.6757594134126350, 248.8843148665554281, -10.86406770146305867 ) ) ;
#70012=CARTESIAN_POINT ( 'NONE',  ( 206.3999048951260136, 272.5212040135120333, 8.078790923728028872 ) ) ;
#70013=CARTESIAN_POINT ( 'NONE',  ( 129.7002344832967538, 251.8149278399160949, -9.188101187500095079 ) ) ;
#70016=CARTESIAN_POINT ( 'NONE',  ( 186.1442180010177481, 296.8921586699537443, 4.664459278073469051 ) ) ;
#70017=CARTESIAN_POINT ( 'NONE',  ( 196.0395593785976018, 291.0965181932902510, 15.97855489120023087 ) ) ;
#70019=CARTESIAN_POINT ( 'NONE',  ( 58.84905177982988533, 192.5327760586659451, 1.948934522072303157E-15 ) ) ;
#70022=EDGE_LOOP ( 'NONE', ( #23097, #92236, #80536, #80632 ) ) ;
#70026=CARTESIAN_POINT ( 'NONE',  ( 172.4040405218840419, 260.9152829665344484, 14.52276536162257159 ) ) ;
#70031=CARTESIAN_POINT ( 'NONE',  ( 108.1850894041356810, 233.2677522451418497, 10.00000000000009592 ) ) ;
#70035=CARTESIAN_POINT ( 'NONE',  ( 162.8037981520209314, 248.6625452659484381, 9.809699077002424161 ) ) ;
#70037=CARTESIAN_POINT ( 'NONE',  ( 26.45420224557697608, 176.8923013555409796, 4.594050593750050204 ) ) ;
#70042=CARTESIAN_POINT ( 'NONE',  ( 174.0424481033923314, 287.4814580433055653, 10.99910921803667208 ) ) ;
#70043=CARTESIAN_POINT ( 'NONE',  ( 69.94482871793547929, 205.0643266524159856, -9.188101187500093303 ) ) ;
#70044=CARTESIAN_POINT ( 'NONE',  ( 161.2313178023453588, 251.3861611254901618, 13.12937145726518473 ) ) ;
#70046=CARTESIAN_POINT ( 'NONE',  ( 56.67693180720107193, 191.9824982072973967, 3.021315404115420679E-15 ) ) ;
#70049=CARTESIAN_POINT ( 'NONE',  ( 29.53915742650918830, 197.8615022471903160, 5.000000000000046185 ) ) ;
#70050=CARTESIAN_POINT ( 'NONE',  ( 116.9873692804980010, 249.8967562850347122, -4.648177544792955347E-16 ) ) ;
#70051=CARTESIAN_POINT ( 'NONE',  ( -13.87062626178347813, 171.9869531367911293, 4.594050593750046652 ) ) ;
#70055=CARTESIAN_POINT ( 'NONE',  ( 189.2272359299283266, 261.5041717493482452, 6.718889169067000289 ) ) ;
#70056=CARTESIAN_POINT ( 'NONE',  ( 164.2801755739368446, 246.1053845600426087, 2.518777461081745717 ) ) ;
#70057=CARTESIAN_POINT ( 'NONE',  ( 183.2104879449952364, 257.6787062734009623, -1.976312334137507287 ) ) ;
#70060=CARTESIAN_POINT ( 'NONE',  ( 135.1739027599712131, 260.3967562850347122, -4.648177544792955347E-16 ) ) ;
#70061=CARTESIAN_POINT ( 'NONE',  ( 181.6036457256498693, 287.6251638105166535, 13.44163109634966524 ) ) ;
#70062=CARTESIAN_POINT ( 'NONE',  ( 196.4935506854234575, 289.8709393705694879, 16.33153036150777737 ) ) ;
#70064=VERTEX_POINT ( 'NONE', #45728 ) ;
#70065=CARTESIAN_POINT ( 'NONE',  ( 159.9379022179727485, 253.6264226329247435, 14.98846149617483192 ) ) ;
#70066=CARTESIAN_POINT ( 'NONE',  ( 204.6075833744878878, 276.2562653119390461, -13.34672481898815910 ) ) ;
#70068=AXIS2_PLACEMENT_3D ( 'NONE', #83689, #84194, #53239 ) ;
#70071=CARTESIAN_POINT ( 'NONE',  ( 164.9586510554008782, 244.9302305544571823, -1.717556444319656039 ) ) ;
#70073=CARTESIAN_POINT ( 'NONE',  ( 207.7837159184916231, 270.7550423741513441, -2.369602332675663448 ) ) ;
#70074=CARTESIAN_POINT ( 'NONE',  ( 201.4520623681621316, 281.7217880192456505, -17.56577389517433119 ) ) ;
#70076=ORIENTED_EDGE ( 'NONE', *, *, #96740, .F. ) ;
#70077=CARTESIAN_POINT ( 'NONE',  ( 191.1055097870458042, 281.0373243973215267, 16.65489552781466287 ) ) ;
#70078=CARTESIAN_POINT ( 'NONE',  ( 164.2934308416063232, 248.6433794851443793, 10.01835112954314155 ) ) ;
#70088=B_SPLINE_CURVE_WITH_KNOTS ( 'NONE', 3,
 ( #19231, #50586, #20209, #27803, #51081, #82043, #66792, #12108, #12618, #42968, #89174, #28796, #59675, #36381, #96745, #4497 ),
 .UNSPECIFIED., .F., .F.,
 ( 4, 2, 2, 2, 2, 2, 2, 4 ),
 ( 0.0006989770276497502596, 0.0009902908671597099310, 0.001281604706669669603, 0.001572918546179629274, 0.001864232385689588945, 0.002155546225199548617, 0.002446860064709508072, 0.003029487743729583106 ),
 .UNSPECIFIED. ) ;
#70089=CARTESIAN_POINT ( 'NONE',  ( 149.6230451358742926, 271.4922791719315001, -12.72565967355361671 ) ) ;
#70092=CARTESIAN_POINT ( 'NONE',  ( 155.3513056799751553, 261.5706408705564741, 18.59020393050806064 ) ) ;
#70093=CARTESIAN_POINT ( 'NONE',  ( 150.0879970963906374, 274.3151389057389906, -8.688618402280457786 ) ) ;
#70094=B_SPLINE_SURFACE_WITH_KNOTS ( 'NONE', 3, 1, ( 
 ( #72489, #41035 ),
 ( #64356, #95320 ),
 ( #25877, #3091 ),
 ( #33982, #64866 ),
 ( #18769, #70200 ),
 ( #59218, #5060 ),
 ( #90193, #811 ),
 ( #75460, #53140 ),
 ( #74482, #31690 ),
 ( #6553, #28340 ),
 ( #51138, #75979 ),
 ( #8418, #89704 ),
 ( #98267, #35941 ),
 ( #20768, #22239 ),
 ( #66843, #97770 ),
 ( #28855, #99260 ),
 ( #83585, #39290 ),
 ( #60714, #12673 ),
 ( #52629, #68335 ),
 ( #51656, #82605 ),
 ( #84097, #13171 ),
 ( #82101, #29845 ),
 ( #37426, #44025 ),
 ( #20264, #67341 ),
 ( #74968, #43541 ),
 ( #5549, #91678 ),
 ( #36434, #14148 ),
 ( #45035, #21744 ),
 ( #59734, #90702 ),
 ( #14649, #46914 ),
 ( #13657, #77836 ),
 ( #21257, #52136 ),
 ( #29355, #83086 ),
 ( #44528, #91183 ) ),
 .UNSPECIFIED., .T., .F., .F.,
 ( 4, 2, 2, 2, 2, 2, 2, 2, 2, 2, 2, 2, 2, 2, 2, 2, 4 ),
 ( 2, 2 ),
 ( 0.000000000000000000, 0.06250000000000000000, 0.1250000000000000000, 0.1875000000000000000, 0.2500000000000000000, 0.3125000000000000000, 0.3750000000000000000, 0.4375000000000000000, 0.5000000000000000000, 0.5625000000000000000, 0.6250000000000000000, 0.6875000000000000000, 0.7500000000000000000, 0.8125000000000000000, 0.8750000000000000000, 0.9375000000000000000, 1.000000000000000000 ),
 ( 0.000000000000000000, 1.000000000000000000 ),
 .UNSPECIFIED. ) ;
#70096=ORIENTED_EDGE ( 'NONE', *, *, #43547, .T. ) ;
#70097=ORIENTED_EDGE ( 'NONE', *, *, #24989, .F. ) ;
#70102=CARTESIAN_POINT ( 'NONE',  ( 208.0692320075777957, 270.2605140014760536, 2.043861372130216569 ) ) ;
#70104=CARTESIAN_POINT ( 'NONE',  ( 165.0778591066108163, 270.9504257995093326, 16.70825090401362090 ) ) ;
#70105=CARTESIAN_POINT ( 'NONE',  ( 167.5814449122423753, 281.2627869255007340, 11.46311708006829200 ) ) ;
#70106=CARTESIAN_POINT ( 'NONE',  ( 194.3442947553755005, 294.0328026529847421, -15.97648891113594871 ) ) ;
#70107=CARTESIAN_POINT ( 'NONE',  ( 175.0270463369839149, 289.9902377644656895, 6.217893157806833493 ) ) ;
#70111=CARTESIAN_POINT ( 'NONE',  ( 198.7717544147009789, 276.5896982162381050, -15.52327009455605022 ) ) ;
#70113=CARTESIAN_POINT ( 'NONE',  ( 159.6978881494930249, 254.0421391940632532, 15.34888828951022610 ) ) ;
#70116=CARTESIAN_POINT ( 'NONE',  ( 206.5081929095101998, 272.9643130319303737, -9.215516226794479238 ) ) ;
#70119=CARTESIAN_POINT ( 'NONE',  ( 178.0302064638906074, 292.4640037680099454, 7.106335582765731296 ) ) ;
#70121=EDGE_LOOP ( 'NONE', ( #24893, #846, #68115, #76585 ) ) ;
#70122=CARTESIAN_POINT ( 'NONE',  ( 155.2374724870715568, 261.7678057442532804, -17.06470218616315648 ) ) ;
#70123=DIRECTION ( 'NONE',  ( -0.8660254037844387076, -0.4999999999999998890, -0.000000000000000000 ) ) ;
#70124=CARTESIAN_POINT ( 'NONE',  ( 162.5887743522035294, 284.9919049736276975, -2.844505511527740005 ) ) ;
#70125=CARTESIAN_POINT ( 'NONE',  ( 14.22133309352410002, 169.0177522451418213, 5.000000000000051514 ) ) ;
#70126=CARTESIAN_POINT ( 'NONE',  ( 81.82518085639701155, 227.2369531367911293, -4.594050593750048428 ) ) ;
#70129=CARTESIAN_POINT ( 'NONE',  ( 169.3174896907622156, 279.7497339657720090, -13.49786840205827509 ) ) ;
#70130=CARTESIAN_POINT ( 'NONE',  ( 7.094665711762558225, 168.2365022471902023, -10.00000000000009237 ) ) ;
#70131=CARTESIAN_POINT ( 'NONE',  ( 10.18872876104421366, 182.8149278399160949, -9.188101187500095079 ) ) ;
#70134=CARTESIAN_POINT ( 'NONE',  ( 200.2690241097007799, 283.7708703901988656, 16.96680019208369927 ) ) ;
#70136=ORIENTED_EDGE ( 'NONE', *, *, #67929, .F. ) ;
#70137=CARTESIAN_POINT ( 'NONE',  ( 164.9043417134678577, 286.5925546497160212, 0.04530247668140159611 ) ) ;
#70138=CARTESIAN_POINT ( 'NONE',  ( 189.0937190564843604, 261.2781646461646687, -6.128236982588672888 ) ) ;
#70139=EDGE_CURVE ( 'NONE', #58975, #39044, #60183, .T. ) ;
#70141=CARTESIAN_POINT ( 'NONE',  ( 202.4709886568992943, 279.9569559179853400, -17.37304959755336853 ) ) ;
#70142=CARTESIAN_POINT ( 'NONE',  ( 85.69442934047377491, 231.8297689869269220, -2.679491924311252493 ) ) ;
#70144=CARTESIAN_POINT ( 'NONE',  ( 36.84650709099022947, 182.8923013555409796, 4.594050593750050204 ) ) ;
#70146=CARTESIAN_POINT ( 'NONE',  ( 196.0366049223029563, 275.3890784149895694, 15.51794149486366159 ) ) ;
#70148=B_SPLINE_CURVE_WITH_KNOTS ( 'NONE', 3,
 ( #52721, #60809, #77551, #37521, #21836, #23320, #91769, #83174, #84185, #14734, #22830, #7126, #91271, #85176, #83681, #15720, #68426, #59828, #53233, #46621, #45617, #76546, #77024, #53715, #38009, #8140, #75551, #99848, #84673, #15215, #67430, #47622, #24826, #17746, #71450, #78047, #54713, #47124, #48646, #40515, #2040, #8636, #79581, #71949, #10142, #39503, #1040, #69921 ),
 .UNSPECIFIED., .F., .F.,
 ( 4, 2, 2, 2, 2, 2, 2, 2, 2, 2, 2, 2, 2, 2, 2, 2, 2, 2, 2, 2, 2, 2, 2, 4 ),
 ( 0.0001670487744419399021, 0.0006556382875749478499, 0.001144227800707955933, 0.001388522557274385165, 0.001632817313840814397, 0.001754964692124029229, 0.001877112070407243845, 0.001999259448690458244, 0.002121406826973672860, 0.002365701583540164975, 0.002609996340106656657, 0.003098585853239643490, 0.004075764879505538660, 0.005052943905771435130, 0.005541533418904341299, 0.005785828175470836450, 0.006030122932037331601, 0.006091196621178905299, 0.006152270310320478129, 0.006274417688603629861, 0.006518712445170039144, 0.007007301958302823881, 0.007495891471435606884, 0.007984480984568392489 ),
 .UNSPECIFIED. ) ;
#70152=CARTESIAN_POINT ( 'NONE',  ( 182.4282706175910391, 260.3850099854238920, -10.97823297164843126 ) ) ;
#70155=CARTESIAN_POINT ( 'NONE',  ( 161.8153478334749877, 250.3745914384277285, -14.21120979595050215 ) ) ;
#70156=DIRECTION ( 'NONE',  ( 0.4999999999999998890, -0.8660254037844385966, 0.000000000000000000 ) ) ;
#70157=CARTESIAN_POINT ( 'NONE',  ( 147.7785919239399846, 274.6869658471848652, -7.924750738206837397 ) ) ;
#70160=CARTESIAN_POINT ( 'NONE',  ( 192.4516364921933018, 265.1256046145381902, 7.763685239252594350 ) ) ;
#70161=CARTESIAN_POINT ( 'NONE',  ( 163.6414931044696175, 249.4718858119513527, -10.35415494711363849 ) ) ;
#70162=CARTESIAN_POINT ( 'NONE',  ( 192.5623620705172527, 265.1981932100166546, 8.541982082413346333 ) ) ;
#70163=CARTESIAN_POINT ( 'NONE',  ( 191.3041230083617563, 299.2985345825480863, -9.819045872446528378 ) ) ;
#70164=CARTESIAN_POINT ( 'NONE',  ( 148.2159754900428936, 273.9293952882992471, 9.267836332806297150 ) ) ;
#70165=CARTESIAN_POINT ( 'NONE',  ( 181.2668321688125843, 265.9111225571392083, -15.67575644871175022 ) ) ;
#70166=EDGE_CURVE ( 'NONE', #20148, #41802, #48201, .T. ) ;
#70169=CARTESIAN_POINT ( 'NONE',  ( 163.7323023463233937, 247.0543288263758086, -6.244751637846886361 ) ) ;
#70170=CARTESIAN_POINT ( 'NONE',  ( 182.3665809609293547, 271.4228521140648809, 17.36529365643261968 ) ) ;
#70171=CARTESIAN_POINT ( 'NONE',  ( 113.7334117446687145, 224.2202760586659736, -5.415160957724236172E-17 ) ) ;
#70173=CARTESIAN_POINT ( 'NONE',  ( 151.0099717111976076, 269.0900518771037468, 15.84752309685681659 ) ) ;
#70174=DIRECTION ( 'NONE',  ( -0.8660254037844387076, -0.4999999999999998890, -0.000000000000000000 ) ) ;
#70175=CARTESIAN_POINT ( 'NONE',  ( 196.0355168007595523, 291.1035201434990540, 17.55377893960077884 ) ) ;
#70176=CARTESIAN_POINT ( 'NONE',  ( 195.1258871920489071, 279.1051608108670621, 16.30780866269864049 ) ) ;
#70177=CARTESIAN_POINT ( 'NONE',  ( 204.6375318825442946, 272.9465897887138226, -9.753471222488339976 ) ) ;
#70178=CARTESIAN_POINT ( 'NONE',  ( 161.5977722445767313, 278.0340992893568455, 13.12270833059843156 ) ) ;
#70180=CARTESIAN_POINT ( 'NONE',  ( 107.6799079185947221, 239.6427522451419350, 10.00000000000009415 ) ) ;
#70185=CARTESIAN_POINT ( 'NONE',  ( 178.7992128730961952, 280.7823504994489667, 16.46972532697894565 ) ) ;
#70186=CARTESIAN_POINT ( 'NONE',  ( 200.1132727327846226, 269.8987286879626026, 8.973240105661503208 ) ) ;
#70187=ADVANCED_FACE ( 'NONE', ( #34091 ), #22337, .F. ) ;
#70188=ORIENTED_EDGE ( 'NONE', *, *, #59842, .T. ) ;
#70189=DIRECTION ( 'NONE',  ( -0.8660254037844387076, -0.4999999999999998890, -0.000000000000000000 ) ) ;
#70190=CARTESIAN_POINT ( 'NONE',  ( 183.6876657337322172, 264.4717431763341438, -13.48096450996037632 ) ) ;
#70192=CARTESIAN_POINT ( 'NONE',  ( 141.2564345147017946, 262.3615022471902876, 5.000000000000046185 ) ) ;
#70193=ADVANCED_FACE ( 'NONE', ( #13753 ), #67956, .T. ) ;
#70194=ORIENTED_EDGE ( 'NONE', *, *, #81348, .T. ) ;
#70195=CARTESIAN_POINT ( 'NONE',  ( 187.7551830709135174, 279.0899711224498105, 17.74026388000889654 ) ) ;
#70197=ORIENTED_EDGE ( 'NONE', *, *, #96350, .F. ) ;
#70198=CARTESIAN_POINT ( 'NONE',  ( 167.6110149314430942, 249.8830905776618181, 6.925631721972418831 ) ) ;
#70200=CARTESIAN_POINT ( 'NONE',  ( 156.9196333786560160, 258.8542176135235877, 18.37000459710097644 ) ) ;
#70201=ORIENTED_EDGE ( 'NONE', *, *, #23089, .T. ) ;
#70204=CARTESIAN_POINT ( 'NONE',  ( 159.2101406416221892, 256.7198602926216608, 16.95745424613295071 ) ) ;
#70206=CARTESIAN_POINT ( 'NONE',  ( 192.5090254847960693, 297.2115822751985093, -12.59048664097589487 ) ) ;
#70215=EDGE_LOOP ( 'NONE', ( #6819, #80896, #14517, #64301 ) ) ;
#70216=ADVANCED_FACE ( 'NONE', ( #61831 ), #60330, .T. ) ;
#70218=CARTESIAN_POINT ( 'NONE',  ( 175.6456982650794885, 258.5815163761128019, 13.11329590940762202 ) ) ;
#70222=EDGE_LOOP ( 'NONE', ( #21946, #96474, #2639, #23862 ) ) ;
#70225=VERTEX_POINT ( 'NONE', #32940 ) ;
#70227=CARTESIAN_POINT ( 'NONE',  ( 206.6347703933553532, 272.7450743988160866, -10.98802705318387574 ) ) ;
#70228=CARTESIAN_POINT ( 'NONE',  ( 190.7101769558895512, 300.3272793223849249, 2.683020982371553398 ) ) ;
#70229=CARTESIAN_POINT ( 'NONE',  ( 148.9266665119372703, 272.6984423298952152, 12.06339424062075061 ) ) ;
#70232=CARTESIAN_POINT ( 'NONE',  ( 44.35726076638960080, 207.9637435831424455, 2.679491924311251605 ) ) ;
#70233=CIRCLE ( 'NONE', #21657, 10.00000000000007816 ) ;
#70234=CARTESIAN_POINT ( 'NONE',  ( 186.8168172874784716, 287.0359679780673332, -15.71538299017341522 ) ) ;
#70235=CARTESIAN_POINT ( 'NONE',  ( 123.0428377395863890, 241.8458772461660544, 9.188101187500095079 ) ) ;
#70238=CARTESIAN_POINT ( 'NONE',  ( 177.1851276373975566, 289.0245988117038110, -10.43460913673951218 ) ) ;
#70241=ORIENTED_EDGE ( 'NONE', *, *, #54380, .T. ) ;
#70242=CARTESIAN_POINT ( 'NONE',  ( 200.0814620334770098, 273.7332971121043101, 13.81105051205792122 ) ) ;
#70243=CARTESIAN_POINT ( 'NONE',  ( 177.6597045081098827, 253.3888418680545556, 1.386942453458301250 ) ) ;
#70245=CARTESIAN_POINT ( 'NONE',  ( 146.9460647107688658, 276.1289452790811652, 2.604800266209711168 ) ) ;
#70248=CARTESIAN_POINT ( 'NONE',  ( 174.4665098196985298, 288.5002641398569949, -10.08633113632384237 ) ) ;
#70251=ORIENTED_EDGE ( 'NONE', *, *, #7239, .F. ) ;
#70252=CARTESIAN_POINT ( 'NONE',  ( 148.1829914015846157, 273.9865254053503349, -9.304102644963160529 ) ) ;
#70253=CARTESIAN_POINT ( 'NONE',  ( 12.50963621419470329, 166.4824982072973967, 3.021315404115420679E-15 ) ) ;
#70254=ORIENTED_EDGE ( 'NONE', *, *, #97232, .F. ) ;
#70256=CARTESIAN_POINT ( 'NONE',  ( 160.2824175349068412, 279.0229062109438587, 10.59256730584001716 ) ) ;
#70257=CARTESIAN_POINT ( 'NONE',  ( 180.4572463832561482, 261.7460625851787199, -13.63662180976220384 ) ) ;
#70258=CARTESIAN_POINT ( 'NONE',  ( 190.0226014859668453, 301.5181949703289774, 3.835066345245774500 ) ) ;
#70259=CARTESIAN_POINT ( 'NONE',  ( 13.42747647338834760, 171.8927522451418213, -10.00000000000009237 ) ) ;
#70260=CARTESIAN_POINT ( 'NONE',  ( 153.3273301907053394, 270.2101081292901767, 14.04008172480431327 ) ) ;
#70261=CARTESIAN_POINT ( 'NONE',  ( 160.8788117166195661, 281.5922145059649893, 5.693820771016479654 ) ) ;
#70262=CARTESIAN_POINT ( 'NONE',  ( -17.42236680055705023, 149.2012482093457777, 0.000000000000000000 ) ) ;
#70264=CARTESIAN_POINT ( 'NONE',  ( 190.9335643195044838, 299.9403610588350944, -4.692880224846124548 ) ) ;
#70267=CARTESIAN_POINT ( 'NONE',  ( 193.5643139362479701, 276.1245741781895617, -16.51112113933535497 ) ) ;
#70268=CARTESIAN_POINT ( 'NONE',  ( 31.61400995286156501, 182.3927522451417644, -10.00000000000009237 ) ) ;
#70269=CARTESIAN_POINT ( 'NONE',  ( 184.5863935663384154, 297.1395876791133333, -4.463175273155427725 ) ) ;
#70270=CARTESIAN_POINT ( 'NONE',  ( 192.4202172926039793, 297.3654025762033370, 10.98569444949570872 ) ) ;
#70271=CARTESIAN_POINT ( 'NONE',  ( 58.82164138842269097, 194.7677522451418213, -5.000000000000041744 ) ) ;
#70274=CARTESIAN_POINT ( 'NONE',  ( -1.691623377417284635, 160.6423013555410080, -4.594050593750043987 ) ) ;
#70275=CARTESIAN_POINT ( 'NONE',  ( 95.22211873877630239, 213.5327760586659451, 1.948934522072303157E-15 ) ) ;
#70276=CARTESIAN_POINT ( 'NONE',  ( 203.3041373168503299, 278.5139001086923827, -16.61929732091214973 ) ) ;
#70277=CARTESIAN_POINT ( 'NONE',  ( 193.0065576635309412, 296.3498312632291913, -11.90044991639595295 ) ) ;
#70283=CARTESIAN_POINT ( 'NONE',  ( 47.99632384111720995, 188.5177522451417929, 5.000000000000051514 ) ) ;
#70286=CARTESIAN_POINT ( 'NONE',  ( 207.7086642703471568, 270.8850356419295053, 6.393550561233467100 ) ) ;
#70288=CARTESIAN_POINT ( 'NONE',  ( 168.1679099710297578, 251.3796770727044247, -8.814879634955225640 ) ) ;
#70289=CARTESIAN_POINT ( 'NONE',  ( 164.1514344399216725, 246.3283707451809903, -4.343706172463206450 ) ) ;
#70291=CARTESIAN_POINT ( 'NONE',  ( 196.4982648257524147, 290.3020170531091821, 16.69353242256149628 ) ) ;
#70295=CARTESIAN_POINT ( 'NONE',  ( 42.47567221558909267, 186.1423013555410080, -4.594050593750043987 ) ) ;
#70296=CARTESIAN_POINT ( 'NONE',  ( 79.95842099707557793, 204.7202760586659167, -5.415160957724236172E-17 ) ) ;
#70297=CARTESIAN_POINT ( 'NONE',  ( 177.9714937548455680, 255.7189482022137383, 8.882064279750110813 ) ) ;
#70301=CARTESIAN_POINT ( 'NONE',  ( 140.4712518949831974, 264.1589784336661637, -6.496448406907675876E-16 ) ) ;
#70303=CARTESIAN_POINT ( 'NONE',  ( -22.42236680055709641, 157.8615022471902591, 0.000000000000000000 ) ) ;
#70304=CARTESIAN_POINT ( 'NONE',  ( 22.44857442947627035, 173.7677522451417929, -5.000000000000041744 ) ) ;
#70306=CARTESIAN_POINT ( 'NONE',  ( 150.9584389135710865, 269.1793093008492406, -15.82751450793727699 ) ) ;
#70309=CARTESIAN_POINT ( 'NONE',  ( 58.44249495421716745, 213.7369531367911293, -4.594050593750048428 ) ) ;
#70311=CARTESIAN_POINT ( 'NONE',  ( 155.3250150347760723, 261.6161776038049425, -18.57420904020362684 ) ) ;
#70312=CARTESIAN_POINT ( 'NONE',  ( 198.1230806404959139, 287.4877535090322453, 17.00698319228197164 ) ) ;
#70314=CARTESIAN_POINT ( 'NONE',  ( 153.3535503493361887, 265.0308546043145270, 16.96417449729259630 ) ) ;
#70317=CARTESIAN_POINT ( 'NONE',  ( 107.0484310652164481, 242.6115022471903160, -5.000000000000047962 ) ) ;
#70319=CARTESIAN_POINT ( 'NONE',  ( 207.2383675728608239, 271.6996134166075763, 7.873592648726489784 ) ) ;
#70322=CARTESIAN_POINT ( 'NONE',  ( 184.9087269013485013, 271.1903322944930892, 16.55683110539250436 ) ) ;
#70324=CARTESIAN_POINT ( 'NONE',  ( 206.1615484827472358, 273.5647187912443314, -9.556459874778100883 ) ) ;
#70325=CARTESIAN_POINT ( 'NONE',  ( 190.2191487900553852, 279.1426948662232803, -16.69313596982519243 ) ) ;
#70326=CARTESIAN_POINT ( 'NONE',  ( -22.42236680055709641, 157.8615022471902591, 0.000000000000000000 ) ) ;
#70328=CARTESIAN_POINT ( 'NONE',  ( 173.6323106214142626, 251.0528461505140285, 0.5214956749697322591 ) ) ;
#70330=ORIENTED_EDGE ( 'NONE', *, *, #97235, .F. ) ;
#70333=CARTESIAN_POINT ( 'NONE',  ( 147.8819534105757043, 274.5079385007862811, -9.338341377131436971 ) ) ;
#70334=B_SPLINE_CURVE_WITH_KNOTS ( 'NONE', 3,
 ( #67508, #98439, #81270, #27541 ),
 .UNSPECIFIED., .F., .F.,
 ( 4, 4 ),
 ( 0.000000000000000000, 0.002378078545638787674 ),
 .UNSPECIFIED. ) ;
#70335=CARTESIAN_POINT ( 'NONE',  ( 148.5942620090405342, 274.9790495171396856, 7.678286107965337948 ) ) ;
#70344=CARTESIAN_POINT ( 'NONE',  ( 170.8805640699686990, 257.7213711969266114, 14.63406020945912367 ) ) ;
#70346=CARTESIAN_POINT ( 'NONE',  ( 171.5339044271115370, 285.5759136860501144, 11.31677738237828557 ) ) ;
#70349=CARTESIAN_POINT ( 'NONE',  ( 208.0421103033489771, 270.3074901711881353, -2.473242163239977476 ) ) ;
#70350=CARTESIAN_POINT ( 'NONE',  ( 193.7275870247597425, 295.1009717758319084, 14.48058678254265885 ) ) ;
#70351=CARTESIAN_POINT ( 'NONE',  ( 158.3585752585947262, 263.3710999200782226, 17.79390465796247156 ) ) ;
#70352=CARTESIAN_POINT ( 'NONE',  ( 204.8385597977314490, 275.8562024115307167, -12.64672659107585240 ) ) ;
#70353=CARTESIAN_POINT ( 'NONE',  ( 145.2890388471816721, 248.5643266524160424, -9.188101187500093303 ) ) ;
#70354=CARTESIAN_POINT ( 'NONE',  ( 206.4643841499645305, 270.6241384910937882, 2.661278798003872570 ) ) ;
#70355=CARTESIAN_POINT ( 'NONE',  ( 178.7344501488548758, 257.7588143725840837, 9.974505692861084682 ) ) ;
#70356=CARTESIAN_POINT ( 'NONE',  ( 96.27750042569734035, 217.2048013555409796, 4.594050593750051981 ) ) ;
#70357=ORIENTED_EDGE ( 'NONE', *, *, #51075, .T. ) ;
#70358=CARTESIAN_POINT ( 'NONE',  ( 191.4922467593309250, 298.9726946877590876, 7.604184559945784017 ) ) ;
#70359=B_SPLINE_CURVE_WITH_KNOTS ( 'NONE', 3,
 ( #82713, #75076, #5657, #52735, #29457, #99371, #6660, #13281, #45147, #52250, #7140, #60331, #83698, #14258, #83192, #76559, #7647, #30448, #61338, #38027, #68938, #67452, #92296, #37050, #15230, #59847, #76086, #53730, #98380, #22847, #13754, #90311, #20883, #53248, #67957, #68443, #37537, #91288, #44634, #91786, #90810, #21364, #46126, #75567, #77040, #29950, #69445, #59331, #45631, #6156, #21854, #51772 ),
 .UNSPECIFIED., .F., .F.,
 ( 4, 2, 2, 2, 2, 2, 2, 2, 2, 2, 2, 2, 2, 2, 2, 2, 2, 2, 2, 2, 2, 2, 2, 2, 2, 4 ),
 ( 0.0001254446608424856873, 0.0006176921519154450479, 0.001109939642988404382, 0.001356063388524914081, 0.001602187134061423997, 0.001725249006829678846, 0.001848310879597933913, 0.001971372752366188329, 0.002094434625134443395, 0.002340558370670906690, 0.002586682116207370419, 0.003078929607280350787, 0.004063424589426311954, 0.005047919571572273556, 0.005540167062645214892, 0.005786290808181685993, 0.006032414553718157095, 0.006093945490102312817, 0.006155476426486468540, 0.006278538299254766974, 0.006524662044791365578, 0.006770785790327965049, 0.007016909535864564521, 0.007263033281401164859, 0.007509157026937763463, 0.008001404518010932915 ),
 .UNSPECIFIED. ) ;
#70360=CARTESIAN_POINT ( 'NONE',  ( 193.0512205562391159, 275.6825563886401369, -16.88465587640301280 ) ) ;
#70363=CARTESIAN_POINT ( 'NONE',  ( 157.0384757953324595, 258.6483765097458445, -16.84863706481609569 ) ) ;
#70365=B_SPLINE_CURVE_WITH_KNOTS ( 'NONE', 3,
 ( #36247, #67152, #98073, #99070, #28650, #6358, #52442, #83389, #37244, #29651, #89047, #19594, #81407, #42836, #4363, #35259 ),
 .UNSPECIFIED., .F., .F.,
 ( 4, 2, 2, 2, 2, 2, 2, 4 ),
 ( 3.688072698881470622E-17, 0.0004627479835026719417, 0.0006941219752539907551, 0.0009254959670053095142, 0.001156869958756628165, 0.001388243950507947033, 0.001619617942259265683, 0.001850991934010584551 ),
 .UNSPECIFIED. ) ;
#70368=CARTESIAN_POINT ( 'NONE',  ( 191.2211340522693774, 299.4422756709672626, -8.405362570633277741 ) ) ;
#70371=FACE_OUTER_BOUND ( 'NONE', #19543, .T. ) ;
#70372=CARTESIAN_POINT ( 'NONE',  ( 88.80803131805656392, 212.8923013555409796, 4.594050593750050204 ) ) ;
#70375=EDGE_LOOP ( 'NONE', ( #69741, #11800, #31038, #84854, #57730 ) ) ;
#70377=B_SPLINE_SURFACE_WITH_KNOTS ( 'NONE', 3, 1, ( 
 ( #53613, #84570 ),
 ( #15108, #98250 ),
 ( #13154, #68816 ),
 ( #83070, #46001 ),
 ( #74951, #21730 ),
 ( #92661, #83572 ),
 ( #14133, #52614 ),
 ( #67327, #98757 ),
 ( #76919, #7518 ),
 ( #45019, #28840 ),
 ( #82589, #7021 ),
 ( #13641, #38411 ),
 ( #99244, #37413 ),
 ( #69326, #29340 ),
 ( #91662, #29829 ),
 ( #22225, #75962 ),
 ( #53126, #100247 ),
 ( #59720, #68319 ),
 ( #84082, #30829 ),
 ( #21243, #44514 ),
 ( #14633, #45514 ),
 ( #75445, #36923 ),
 ( #67837, #37906 ),
 ( #64226, #40902 ),
 ( #932, #10039 ),
 ( #71344, #25222 ),
 ( #1444, #16622 ),
 ( #430, #55601 ),
 ( #31808, #46507 ),
 ( #78446, #38914 ),
 ( #23214, #9027 ),
 ( #15609, #77445 ),
 ( #32821, #77942 ),
 ( #62708, #32324 ) ),
 .UNSPECIFIED., .T., .F., .F.,
 ( 4, 2, 2, 2, 2, 2, 2, 2, 2, 2, 2, 2, 2, 2, 2, 2, 4 ),
 ( 2, 2 ),
 ( 0.000000000000000000, 0.06250000000000000000, 0.1250000000000000000, 0.1875000000000000000, 0.2500000000000000000, 0.3125000000000000000, 0.3750000000000000000, 0.4375000000000000000, 0.5000000000000000000, 0.5625000000000000000, 0.6250000000000000000, 0.6875000000000000000, 0.7500000000000000000, 0.8125000000000000000, 0.8750000000000000000, 0.9375000000000000000, 1.000000000000000000 ),
 ( 0.000000000000000000, 1.000000000000000000 ),
 .UNSPECIFIED. ) ;
#70378=CARTESIAN_POINT ( 'NONE',  ( 208.3682389855799499, 269.7426187237583690, -1.431169231381201890 ) ) ;
#70380=EDGE_CURVE ( 'NONE', #26607, #13801, #49944, .T. ) ;
#70383=CARTESIAN_POINT ( 'NONE',  ( 184.1072502077840909, 275.2075811318409819, 16.36983495193582172 ) ) ;
#70384=CARTESIAN_POINT ( 'NONE',  ( 162.3887597439333774, 285.1017702274234580, 0.5428779426774286154 ) ) ;
#70385=CARTESIAN_POINT ( 'NONE',  ( 98.91686120480925126, 239.4637435831424739, 2.679491924311251605 ) ) ;
#70389=CARTESIAN_POINT ( 'NONE',  ( 185.9605642706161746, 259.1549715882831606, 6.130847983954422986 ) ) ;
#70391=CARTESIAN_POINT ( 'NONE',  ( 201.0356089830534643, 282.4431064412383989, -18.18835788025466371 ) ) ;
#70393=CARTESIAN_POINT ( 'NONE',  ( 149.3118911495987788, 247.0312136851381126, 5.028230608967417581 ) ) ;
#70396=CARTESIAN_POINT ( 'NONE',  ( 161.4396252346964218, 251.0253620690641299, 14.51972485405798885 ) ) ;
#70398=CARTESIAN_POINT ( 'NONE',  ( 187.5257214801813461, 265.9040347152727009, -11.83413594510077260 ) ) ;
#70399=CARTESIAN_POINT ( 'NONE',  ( -22.42236680055709641, 157.8615022471902591, 0.000000000000000000 ) ) ;
#70400=CARTESIAN_POINT ( 'NONE',  ( 153.5335373734693576, 270.3435883613224178, 14.01947500330756391 ) ) ;
#70403=DIRECTION ( 'NONE',  ( 0.4999999999999998890, -0.8660254037844385966, 0.000000000000000000 ) ) ;
#70404=B_SPLINE_CURVE_WITH_KNOTS ( 'NONE', 3,
 ( #40564, #48695, #23868, #40060 ),
 .UNSPECIFIED., .F., .F.,
 ( 4, 4 ),
 ( 0.008181640604905312045, 0.01326458609140142818 ),
 .UNSPECIFIED. ) ;
#70405=CARTESIAN_POINT ( 'NONE',  ( 202.4943568615953779, 279.9164810001701085, 17.09064351659286984 ) ) ;
#70406=AXIS2_PLACEMENT_3D ( 'NONE', #29110, #90453, #59976 ) ;
#70408=CARTESIAN_POINT ( 'NONE',  ( 177.4749804298298272, 264.4991266834069279, -15.68007347713953514 ) ) ;
#70410=CARTESIAN_POINT ( 'NONE',  ( 199.1402566354874750, 281.8950033040109133, -16.59982190247651346 ) ) ;
#70413=CARTESIAN_POINT ( 'NONE',  ( 168.4187099521293760, 273.5093150913818363, 16.15648551869223937 ) ) ;
#70414=CARTESIAN_POINT ( 'NONE',  ( 163.3291633122615849, 283.7466658353214939, -3.311912926934972301 ) ) ;
#70416=CARTESIAN_POINT ( 'NONE',  ( 191.3487518683689359, 261.0470579585651194, 3.102467918029140126 ) ) ;
#70419=CARTESIAN_POINT ( 'NONE',  ( 2.016134656476094023, 159.7202760586659736, -5.415160957724236172E-17 ) ) ;
#70422=CARTESIAN_POINT ( 'NONE',  ( 174.8562727840514412, 255.3278782549236894, 8.725767214627929036 ) ) ;
#70426=CARTESIAN_POINT ( 'NONE',  ( 16.52171307410043255, 180.3458772461660544, 9.188101187500095079 ) ) ;
#70430=CARTESIAN_POINT ( 'NONE',  ( 100.4810717531844659, 235.4865022471902876, -10.00000000000009592 ) ) ;
#70432=CARTESIAN_POINT ( 'NONE',  ( 186.7314779716672888, 295.9876638862722871, -8.607072244006850781 ) ) ;
#70433=CARTESIAN_POINT ( 'NONE',  ( 189.8800752008499160, 261.4572743640761701, -0.7539990698043521622 ) ) ;
#70435=CARTESIAN_POINT ( 'NONE',  ( 67.57210640937580592, 216.4865022471902876, 10.00000000000009237 ) ) ;
#70437=EDGE_CURVE ( 'NONE', #63662, #21425, #89696, .T. ) ;
#70438=CARTESIAN_POINT ( 'NONE',  ( 167.6502826215564994, 287.3877002845107995, 4.891367078714356609 ) ) ;
#70439=CARTESIAN_POINT ( 'NONE',  ( 37.57712925149210292, 186.3768266524160140, 9.188101187500098632 ) ) ;
#70442=CARTESIAN_POINT ( 'NONE',  ( 203.0352482185525389, 270.0697959434764925, -6.424953051763736767 ) ) ;
#70447=CARTESIAN_POINT ( 'NONE',  ( 160.2764658979060926, 278.7662822791168651, -9.787372777049167638 ) ) ;
#70448=CARTESIAN_POINT ( 'NONE',  ( 205.7570824856458103, 269.1293880245460173, -1.352896656403272946 ) ) ;
#70450=CARTESIAN_POINT ( 'NONE',  ( 202.3425522658138505, 280.1794142728863903, 15.86053073629060961 ) ) ;
#70451=CARTESIAN_POINT ( 'NONE',  ( 196.6800254274587019, 289.9871984561398222, -17.90749311895638129 ) ) ;
#70452=CARTESIAN_POINT ( 'NONE',  ( 175.1308103651610963, 256.9497360334458449, 11.89887680739436071 ) ) ;
#70455=CYLINDRICAL_SURFACE ( 'NONE', #10646, 10.00000000000010658 ) ;
#70458=DIRECTION ( 'NONE',  ( -0.8660254037844387076, -0.4999999999999998890, -0.000000000000000000 ) ) ;
#70460=CARTESIAN_POINT ( 'NONE',  ( 190.9061255863007318, 299.9878863388391892, 7.497146773253707153 ) ) ;
#70461=CARTESIAN_POINT ( 'NONE',  ( 155.5066938333533528, 261.3015006940112244, -18.40036130547566273 ) ) ;
#70463=VERTEX_POINT ( 'NONE', #26357 ) ;
#70464=DIRECTION ( 'NONE',  ( -0.8660254037844387076, -0.4999999999999998890, -0.000000000000000000 ) ) ;
#70467=CARTESIAN_POINT ( 'NONE',  ( 201.3053499423511425, 281.9759013948520874, -16.75960365258566398 ) ) ;
#70469=CARTESIAN_POINT ( 'NONE',  ( 203.5726949774746117, 269.0034548673361883, -6.096665150295551783 ) ) ;
#70471=CARTESIAN_POINT ( 'NONE',  ( 189.8147415777049218, 301.8782188922952514, -0.5019643756309712934 ) ) ;
#70472=CARTESIAN_POINT ( 'NONE',  ( 196.2878005184348353, 290.6665519265632724, -16.69183432842427806 ) ) ;
#70476=ORIENTED_EDGE ( 'NONE', *, *, #96210, .F. ) ;
#70477=CARTESIAN_POINT ( 'NONE',  ( 178.8595466249924755, 265.0989930076032124, -16.03772641351113748 ) ) ;
#70478=CARTESIAN_POINT ( 'NONE',  ( 161.6952081746299825, 267.0400630579588892, 16.50188533208787334 ) ) ;
#70483=CARTESIAN_POINT ( 'NONE',  ( 58.14488549560751807, 210.5024278399160949, 9.188101187500095079 ) ) ;
#70488=CARTESIAN_POINT ( 'NONE',  ( 172.5948319566698501, 271.8727042802207734, 17.20912629143206374 ) ) ;
#70491=CARTESIAN_POINT ( 'NONE',  ( 165.0735250206753619, 246.7312630101393722, 5.989302113854410692 ) ) ;
#70492=CARTESIAN_POINT ( 'NONE',  ( 147.6121581866023007, 274.9752375363476631, 8.700660424766859080 ) ) ;
#70493=ORIENTED_EDGE ( 'NONE', *, *, #2303, .T. ) ;
#70494=CARTESIAN_POINT ( 'NONE',  ( 175.3681337606042803, 261.2921292801445929, -14.32318010708709544 ) ) ;
#70497=CARTESIAN_POINT ( 'NONE',  ( 146.8868584395697781, 276.2314935489248455, -3.891417269505058396 ) ) ;
#70500=CARTESIAN_POINT ( 'NONE',  ( 164.2801755739368446, 246.1053845600426087, 2.518777461081745717 ) ) ;
#70504=CARTESIAN_POINT ( 'NONE',  ( 113.7334117446687145, 224.2202760586659736, -5.415160957724236172E-17 ) ) ;
#70505=VERTEX_POINT ( 'NONE', #18759 ) ;
#70506=AXIS2_PLACEMENT_3D ( 'NONE', #95123, #47465, #23653 ) ;
#70507=CARTESIAN_POINT ( 'NONE',  ( 190.1981067718782015, 301.2142108981337287, -4.661316250821958995 ) ) ;
#70510=CARTESIAN_POINT ( 'NONE',  ( 154.9048824156581361, 262.3438686460345366, -17.40627786727128168 ) ) ;
#70512=CARTESIAN_POINT ( 'NONE',  ( 164.2413944571582078, 246.1725554246774834, 7.304616466633322425 ) ) ;
#70515=EDGE_LOOP ( 'NONE', ( #4935, #22301, #72789, #31702, #12811, #88354, #34625, #99502, #75257, #71423, #30462, #83907, #59654, #34142, #53753, #14320, #89031, #54922, #3106, #828, #86666 ) ) ;
#70517=CARTESIAN_POINT ( 'NONE',  ( 185.9527541470076812, 261.9448596265605715, 9.964853131083170723 ) ) ;
#70518=CARTESIAN_POINT ( 'NONE',  ( 206.1020338308353530, 272.8276230067459096, 9.011824622212118996 ) ) ;
#70519=CARTESIAN_POINT ( 'NONE',  ( 130.4855038751826726, 236.9548013555409796, -4.594050593750042211 ) ) ;
#70520=CARTESIAN_POINT ( 'NONE',  ( 150.7691137448031213, 269.5072301123068428, -15.63821625702598084 ) ) ;
#70521=CARTESIAN_POINT ( 'NONE',  ( 185.8363103352124881, 296.8156583057766511, 4.440193935637427813 ) ) ;
#70522=CARTESIAN_POINT ( 'NONE',  ( 157.7233946900069839, 257.4620621851055375, 16.86796251324260254 ) ) ;
#70524=CARTESIAN_POINT ( 'NONE',  ( 55.14129374593650113, 193.4548013555410080, -4.594050593750042211 ) ) ;
#70531=CARTESIAN_POINT ( 'NONE',  ( 173.9473224539459579, 261.8997203040686941, 14.37357808391092284 ) ) ;
#70533=CARTESIAN_POINT ( 'NONE',  ( 202.7973612924478743, 279.3916619310153919, -15.54732529288344089 ) ) ;
#70535=CARTESIAN_POINT ( 'NONE',  ( 153.8789445373735418, 269.2372782055974767, -15.31005183354254129 ) ) ;
#70536=CARTESIAN_POINT ( 'NONE',  ( 122.5466773502276254, 234.8927522451417360, -10.00000000000009059 ) ) ;
#70540=CARTESIAN_POINT ( 'NONE',  ( 202.2712651538608668, 280.3028871727136675, 16.13191389836473988 ) ) ;
#70541=CARTESIAN_POINT ( 'NONE',  ( 176.6558404752379090, 252.2237374370411942, -0.2705739152901737166 ) ) ;
#70542=AXIS2_PLACEMENT_3D ( 'NONE', #5990, #58190, #5495 ) ;
#70543=CARTESIAN_POINT ( 'NONE',  ( 29.83685365728618066, 188.0333772461660544, 9.188101187500095079 ) ) ;
#70549=CARTESIAN_POINT ( 'NONE',  ( 63.61184440487929947, 207.5333772461660544, 9.188101187500095079 ) ) ;
#70550=CARTESIAN_POINT ( 'NONE',  ( 173.3964598228361353, 287.9493122502211691, 7.531884089513041225 ) ) ;
#70551=CARTESIAN_POINT ( 'NONE',  ( 163.0344181721474968, 256.4022621988681863, -15.46606454548692788 ) ) ;
#70552=CARTESIAN_POINT ( 'NONE',  ( 157.0978663001774862, 258.5455091378672137, -17.31223197570816552 ) ) ;
#70554=ORIENTED_EDGE ( 'NONE', *, *, #47342, .T. ) ;
#70556=CARTESIAN_POINT ( 'NONE',  ( 24.34300500380255983, 194.8615022471903160, 5.000000000000046185 ) ) ;
#70557=CARTESIAN_POINT ( 'NONE',  ( 186.1263547150109900, 286.8862237501084564, -16.18252752151998308 ) ) ;
#70558=CARTESIAN_POINT ( 'NONE',  ( 202.3894997978090373, 280.0980987621804275, 16.95659012541789323 ) ) ;
#70559=CARTESIAN_POINT ( 'NONE',  ( -2.016382903836450691, 160.4548013555409796, -4.594050593750042211 ) ) ;
#70561=CARTESIAN_POINT ( 'NONE',  ( 167.3620191591094510, 262.1387632814340236, -17.17666365667549755 ) ) ;
#70562=CARTESIAN_POINT ( 'NONE',  ( 170.9167832255728285, 262.8446361638572739, 16.75413523746211908 ) ) ;
#70563=CARTESIAN_POINT ( 'NONE',  ( 189.2895335294923029, 261.7382647175048760, 6.647372333888422524 ) ) ;
#70564=DIRECTION ( 'NONE',  ( -0.8660254037844359321, -0.5000000000000051070, -0.000000000000000000 ) ) ;
#70568=CARTESIAN_POINT ( 'NONE',  ( 57.45043449909725553, 210.6427522451419634, -10.00000000000009592 ) ) ;
#70569=CARTESIAN_POINT ( 'NONE',  ( 178.2990217061593228, 285.7009041265487213, 12.88278519312938286 ) ) ;
#70570=CARTESIAN_POINT ( 'NONE',  ( 167.7231831693838728, 286.7520842802292691, 0.5032469995052184508 ) ) ;
#70572=CARTESIAN_POINT ( 'NONE',  ( 159.0402943516375274, 259.3997371224696735, 16.69638147318008947 ) ) ;
#70574=CARTESIAN_POINT ( 'NONE',  ( 206.6298919378964740, 272.7535241315335384, -9.267551915974392429 ) ) ;
#70575=CARTESIAN_POINT ( 'NONE',  ( 58.98402115518014455, 204.8615022471902307, -10.00000000000009592 ) ) ;
#70576=CARTESIAN_POINT ( 'NONE',  ( 192.1640094933931096, 297.8091675017319062, 12.36911124822534447 ) ) ;
#70577=CARTESIAN_POINT ( 'NONE',  ( 80.49827691776714289, 228.8297689869269220, -2.679491924311252493 ) ) ;
#70578=AXIS2_PLACEMENT_3D ( 'NONE', #95891, #26452, #4129 ) ;
#70579=CARTESIAN_POINT ( 'NONE',  ( 190.7405042774493324, 298.2747508605859821, 9.591131971744578877 ) ) ;
#70581=CARTESIAN_POINT ( 'NONE',  ( 193.7114073116034945, 295.1289958610702797, 14.86160832869823345 ) ) ;
#70583=( BOUNDED_CURVE ( )  B_SPLINE_CURVE ( 2, ( #83528, #68776, #70271, #7996, #99698, #22693, #99201, #14092, #54553 ),
 .UNSPECIFIED., .F., .T. ) 
 B_SPLINE_CURVE_WITH_KNOTS ( ( 3, 2, 2, 2, 3 ),
 ( 0.4153225806451613100, 0.4166666666666666852, 0.4193548387096774355, 0.4220430107526881858, 0.4233870967741935609 ),
 .UNSPECIFIED. ) 
 CURVE ( )  GEOMETRIC_REPRESENTATION_ITEM ( )  RATIONAL_B_SPLINE_CURVE ( ( 0.9330127018922194093, 0.9330127018922194093, 1.000000000000000000, 0.8660254037844387076, 1.000000000000000000, 0.8660254037844387076, 1.000000000000000000, 0.9330127018922194093, 0.9330127018922194093 ) ) 
 REPRESENTATION_ITEM ( '' )  );
#70585=CARTESIAN_POINT ( 'NONE',  ( 156.6183249201009176, 277.0683422884322340, -10.04461592201575648 ) ) ;
#70589=CARTESIAN_POINT ( 'NONE',  ( 188.4805308512120234, 298.0761574053781828, 7.892637567094712203 ) ) ;
#70591=CARTESIAN_POINT ( 'NONE',  ( 151.3542526322075901, 269.2885850756041464, -14.28695254860580199 ) ) ;
#70594=B_SPLINE_CURVE_WITH_KNOTS ( 'NONE', 3,
 ( #73613, #25507, #89362, #65499, #3236, #48820, #79753, #27519, #87393, #96953, #41186, #2728, #18422, #73129, #34120, #49803, #19440, #56892, #65013, #57395, #87876, #10317, #43176, #64002, #81249, #12314, #50295, #72123, #96447, #3722, #58388, #80764, #35094, #17922, #19918, #34600, #42194, #27014, #11335, #2224, #41693, #33105, #80250, #94943, #4194, #57898, #95957, #66001, #50789, #49312, #10817, #26518, #88370, #18928, #56398, #42681 ),
 .UNSPECIFIED., .F., .F.,
 ( 4, 2, 2, 2, 2, 2, 2, 2, 2, 2, 2, 2, 2, 2, 2, 2, 2, 2, 2, 2, 2, 2, 2, 2, 2, 2, 2, 4 ),
 ( 0.0009471700189065799689, 0.001428333720301369712, 0.001909497421696159779, 0.002150079272393554813, 0.002390661123090949414, 0.002510952048439690082, 0.002631242973788430750, 0.002751533899137171418, 0.002871824824485912087, 0.003112406675183393423, 0.003352988525880874759, 0.003834152227275901183, 0.004796479630065955332, 0.005758807032856009915, 0.006239970734251036773, 0.006480552584948509436, 0.006721134435645980364, 0.006781279898320428760, 0.006841425360994876290, 0.006901570823669324686, 0.006961716286343772216, 0.007082007211692641253, 0.007202298137041510291, 0.007442879987739348113, 0.007683461838437184201, 0.007924043689135020288, 0.008164625539832857243, 0.008645789241228626562 ),
 .UNSPECIFIED. ) ;
#70595=CARTESIAN_POINT ( 'NONE',  ( 149.4908848037268001, 271.7211875819559737, -12.92288068979413573 ) ) ;
#70597=ADVANCED_FACE ( 'NONE', ( #14641 ), #44521, .T. ) ;
#70599=VERTEX_POINT ( 'NONE', #38419 ) ;
#70600=CARTESIAN_POINT ( 'NONE',  ( 155.7792811089228735, 260.8293656832279908, 18.01238576999985952 ) ) ;
#70601=CARTESIAN_POINT ( 'NONE',  ( 191.0816511748900268, 299.6838671013740623, 7.311127128005925790 ) ) ;
#70608=CARTESIAN_POINT ( 'NONE',  ( 159.4238121903318017, 269.8920955656249134, 15.66160391340022606 ) ) ;
#70610=CARTESIAN_POINT ( 'NONE',  ( 208.2939409893161553, 269.8713066281881083, 2.523744790997269227 ) ) ;
#70612=CARTESIAN_POINT ( 'NONE',  ( 168.2234495781609667, 281.3103526383414419, 11.64684307458802870 ) ) ;
#70613=ADVANCED_FACE ( 'NONE', ( #36931 ), #67334, .T. ) ;
#70614=CARTESIAN_POINT ( 'NONE',  ( 194.4666154385731431, 293.8209370148700827, -14.56896502715340702 ) ) ;
#70615=LINE ( 'NONE', #33635, #25662 ) ;
#70618=CARTESIAN_POINT ( 'NONE',  ( 158.6532760188547400, 266.7985734874461627, -17.41301857359564309 ) ) ;
#70621=CARTESIAN_POINT ( 'NONE',  ( 198.4152875795883801, 277.4255225366634932, -15.34652983819002792 ) ) ;
#70623=CARTESIAN_POINT ( 'NONE',  ( 159.4230536986738400, 254.5181664265525683, 16.83068086755798376 ) ) ;
#70625=AXIS2_PLACEMENT_3D ( 'NONE', #72919, #58176, #57672 ) ;
#70626=CARTESIAN_POINT ( 'NONE',  ( 190.4035152335380019, 300.8584330062341792, 5.540201033361155325 ) ) ;
#70628=CARTESIAN_POINT ( 'NONE',  ( 159.3237119419271437, 254.6902313965507858, -15.56765445935501191 ) ) ;
#70632=CARTESIAN_POINT ( 'NONE',  ( 161.6256441450323678, 250.7031678651938762, 14.48526717260977037 ) ) ;
#70633=CARTESIAN_POINT ( 'NONE',  ( 114.4096469973842858, 226.8615022471902023, 5.000000000000051514 ) ) ;
#70635=FACE_OUTER_BOUND ( 'NONE', #11973, .T. ) ;
#70637=CARTESIAN_POINT ( 'NONE',  ( 182.5291792280718823, 296.7636338796572204, 0.3805386115670883473 ) ) ;
#70638=CARTESIAN_POINT ( 'NONE',  ( 9.458193372709603253, 186.2677522451419065, -5.000000000000047962 ) ) ;
#70639=CARTESIAN_POINT ( 'NONE',  ( 87.80660267098954819, 215.3768266524160424, -9.188101187500093303 ) ) ;
#70642=CARTESIAN_POINT ( 'NONE',  ( 167.0433667443437287, 277.9948742561587665, -14.29907309580385188 ) ) ;
#70643=CARTESIAN_POINT ( 'NONE',  ( 18.33521408509785644, 172.2048013555409796, 4.594050593750051981 ) ) ;
#70645=CARTESIAN_POINT ( 'NONE',  ( 161.7101619467568980, 250.5567787384628389, 13.05644392949610655 ) ) ;
#70647=CIRCLE ( 'NONE', #80468, 17.82106496071138224 ) ;
#70648=ORIENTED_EDGE ( 'NONE', *, *, #42069, .T. ) ;
#70650=CARTESIAN_POINT ( 'NONE',  ( 189.0990418739154961, 261.3597260687160428, -6.102409993698818980 ) ) ;
#70655=CARTESIAN_POINT ( 'NONE',  ( 161.8150574665248200, 250.3750943687383881, -13.25074899737357903 ) ) ;
#70656=CARTESIAN_POINT ( 'NONE',  ( 87.49069069641790009, 227.9865022471902876, -10.00000000000009592 ) ) ;
#70657=CARTESIAN_POINT ( 'NONE',  ( 180.6066648745947134, 283.7006809008031496, -16.18202752516933174 ) ) ;
#70658=CARTESIAN_POINT ( 'NONE',  ( 41.36599039304902448, 188.5643266524159571, -9.188101187500093303 ) ) ;
#70659=CARTESIAN_POINT ( 'NONE',  ( 197.4319809672400652, 276.3590923837395508, 15.22116115860616503 ) ) ;
#70661=CARTESIAN_POINT ( 'NONE',  ( 34.30229714732369217, 180.6115022471902023, -5.000000000000041744 ) ) ;
#70663=CARTESIAN_POINT ( 'NONE',  ( 175.2487935740293779, 281.5086999169899968, -14.18879801599889490 ) ) ;
#70665=CARTESIAN_POINT ( 'NONE',  ( 195.9359860111818250, 291.2759125279654882, 17.49638312768267312 ) ) ;
#70667=CARTESIAN_POINT ( 'NONE',  ( 65.98439316910436503, 202.2365022471902307, 10.00000000000009948 ) ) ;
#70668=CARTESIAN_POINT ( 'NONE',  ( 186.5665755256727039, 282.6830977147599810, 16.17162702254794482 ) ) ;
#70669=CARTESIAN_POINT ( 'NONE',  ( 194.5252985417586729, 293.7192948986070178, -14.54632727629426370 ) ) ;
#70671=CARTESIAN_POINT ( 'NONE',  ( 204.2129321040862919, 276.9398213635460024, 14.41515352680879758 ) ) ;
#70672=CARTESIAN_POINT ( 'NONE',  ( 188.4708381935227521, 298.8780472021338710, 6.289082596400687564 ) ) ;
#70674=CARTESIAN_POINT ( 'NONE',  ( 147.6220714307702622, 274.9580672937808572, 8.392894244419288441 ) ) ;
#70675=CARTESIAN_POINT ( 'NONE',  ( 180.8071464327592253, 266.9085124479379942, -14.75290084666368351 ) ) ;
#70677=CARTESIAN_POINT ( 'NONE',  ( 153.2593913506692616, 267.1939427739956727, -16.45456985337825984 ) ) ;
#70678=CARTESIAN_POINT ( 'NONE',  ( 207.5290616128274337, 271.1961165699281651, 2.604679844609484984 ) ) ;
#70680=CARTESIAN_POINT ( 'NONE',  ( 103.8820256808556906, 230.7833772461660544, -9.188101187500095079 ) ) ;
#70682=CARTESIAN_POINT ( 'NONE',  ( -15.51451749852110495, 173.3967562850347406, 6.972266317189433612E-15 ) ) ;
#70683=DIRECTION ( 'NONE',  ( 0.4999999999999998890, -0.8660254037844385966, 0.000000000000000000 ) ) ;
#70684=CARTESIAN_POINT ( 'NONE',  ( 175.3074307085254020, 254.5436327766159650, 9.407465564047683415 ) ) ;
#70685=CARTESIAN_POINT ( 'NONE',  ( 195.6664450926536460, 278.3245960621525796, 17.18455885460583232 ) ) ;
#70690=CARTESIAN_POINT ( 'NONE',  ( 116.4326846683273544, 226.4824982072973683, 3.021315404115420679E-15 ) ) ;
#70691=CARTESIAN_POINT ( 'NONE',  ( 110.0998739067015606, 222.8262482093458061, 3.021315404115420679E-15 ) ) ;
#70694=CARTESIAN_POINT ( 'NONE',  ( 189.8711135266105146, 266.0314335071855112, 10.76611041489257836 ) ) ;
#70697=CARTESIAN_POINT ( 'NONE',  ( 196.5244701160910665, 267.6823335762956049, 9.543964429419004247 ) ) ;
#70699=B_SPLINE_SURFACE_WITH_KNOTS ( 'NONE', 3, 1, ( 
 ( #1767, #32647 ),
 ( #86912, #9351 ),
 ( #25042, #48356 ),
 ( #9874, #79305 ),
 ( #40731, #33150 ),
 ( #87924, #2777 ),
 ( #64050, #56939 ),
 ( #72171, #94994 ),
 ( #56444, #10364 ),
 ( #33665, #64556 ),
 ( #95516, #26062 ),
 ( #77768, #19486 ),
 ( #10865, #65545 ),
 ( #12870, #27061 ),
 ( #89884, #18975 ),
 ( #50342, #88415 ),
 ( #96491, #36129 ),
 ( #42723, #57437 ),
 ( #19959, #97472 ),
 ( #57943, #65052 ),
 ( #18466, #49849 ),
 ( #81294, #11867 ),
 ( #72684, #51332 ),
 ( #88926, #96002 ),
 ( #73661, #34160 ),
 ( #66050, #80294 ),
 ( #20458, #82300 ),
 ( #43729, #49354 ),
 ( #97957, #4239 ),
 ( #26562, #50836 ),
 ( #28038, #4761 ),
 ( #59414, #35139 ),
 ( #80810, #35643 ),
 ( #74672, #5249 ) ),
 .UNSPECIFIED., .T., .F., .F.,
 ( 4, 2, 2, 2, 2, 2, 2, 2, 2, 2, 2, 2, 2, 2, 2, 2, 4 ),
 ( 2, 2 ),
 ( 0.000000000000000000, 0.06250000000000000000, 0.1250000000000000000, 0.1875000000000000000, 0.2500000000000000000, 0.3125000000000000000, 0.3750000000000000000, 0.4375000000000000000, 0.5000000000000000000, 0.5625000000000000000, 0.6250000000000000000, 0.6875000000000000000, 0.7500000000000000000, 0.8125000000000000000, 0.8750000000000000000, 0.9375000000000000000, 1.000000000000000000 ),
 ( 0.000000000000000000, 1.000000000000000000 ),
 .UNSPECIFIED. ) ;
#70701=B_SPLINE_CURVE_WITH_KNOTS ( 'NONE', 3,
 ( #99874, #90821, #68949, #92790 ),
 .UNSPECIFIED., .F., .F.,
 ( 4, 4 ),
 ( 0.01073252529666175389, 0.01912580236392939434 ),
 .UNSPECIFIED. ) ;
#70704=CARTESIAN_POINT ( 'NONE',  ( 152.4425959802508999, 245.4865022471901739, 1.119607411625061291E-15 ) ) ;
#70706=ORIENTED_EDGE ( 'NONE', *, *, #2322, .T. ) ;
#70711=CARTESIAN_POINT ( 'NONE',  ( 167.4640110857230582, 280.8630760984805192, 11.65775015378388169 ) ) ;
#70712=CARTESIAN_POINT ( 'NONE',  ( 166.0506673010352472, 274.1027903476490337, -16.62009509085023851 ) ) ;
#70713=CARTESIAN_POINT ( 'NONE',  ( 114.7524487161677058, 230.3927522451417929, -10.00000000000009237 ) ) ;
#70717=CARTESIAN_POINT ( 'NONE',  ( 204.1953342137782954, 276.9703018036655067, 13.84727111424505885 ) ) ;
#70718=CARTESIAN_POINT ( 'NONE',  ( 199.9502294570856407, 265.6703872523112295, 6.360370400932541246E-13 ) ) ;
#70721=CYLINDRICAL_SURFACE ( 'NONE', #4901, 10.00000000000010658 ) ;
#70723=CARTESIAN_POINT ( 'NONE',  ( 35.00594278435062989, 181.0177522451417929, 5.000000000000051514 ) ) ;
#70725=EDGE_CURVE ( 'NONE', #80478, #41871, #9446, .T. ) ;
#70727=CARTESIAN_POINT ( 'NONE',  ( 163.3548548005089174, 249.5016276120636860, 11.44428125521734962 ) ) ;
#70733=VERTEX_POINT ( 'NONE', #67845 ) ;
#70734=CARTESIAN_POINT ( 'NONE',  ( 183.7658459069459695, 280.9060072218711639, -16.15935528051975467 ) ) ;
#70735=CARTESIAN_POINT ( 'NONE',  ( 206.2880451275741223, 273.3456201754175368, -11.28869033117385534 ) ) ;
#70736=CARTESIAN_POINT ( 'NONE',  ( 190.1806134411257290, 301.2445102357908127, 1.963143373670005243 ) ) ;
#70739=CARTESIAN_POINT ( 'NONE',  ( 169.4595697446889631, 250.2531843026321496, -5.478044125683344312 ) ) ;
#70742=CARTESIAN_POINT ( 'NONE',  ( 157.7939826016823304, 280.9050555316971440, 2.087917227061603320 ) ) ;
#70743=CARTESIAN_POINT ( 'NONE',  ( 133.0835800865360170, 238.4548013555409796, -4.594050593750042211 ) ) ;
#70745=CARTESIAN_POINT ( 'NONE',  ( 185.1104244301751578, 261.7904637200641673, -9.069498223535303438 ) ) ;
#70747=ORIENTED_EDGE ( 'NONE', *, *, #48508, .F. ) ;
#70749=ORIENTED_EDGE ( 'NONE', *, *, #88057, .T. ) ;
#70750=CARTESIAN_POINT ( 'NONE',  ( 202.8857220437332955, 275.8096136465296695, 13.30856319272651511 ) ) ;
#70751=CARTESIAN_POINT ( 'NONE',  ( 180.7946767411322355, 256.2352744486502161, 1.150915517461931659 ) ) ;
#70752=CARTESIAN_POINT ( 'NONE',  ( 174.2171726394180666, 290.5684288936432154, -4.877197793559998829 ) ) ;
#70753=CARTESIAN_POINT ( 'NONE',  ( 147.4643594168521474, 275.2312325148511718, 3.404945201207095540 ) ) ;
#70755=CARTESIAN_POINT ( 'NONE',  ( 164.2897805489690768, 249.8104079013010335, 11.36607573508163505 ) ) ;
#70758=CARTESIAN_POINT ( 'NONE',  ( 174.9303175201940803, 282.4108518568261843, 14.59670604635778979 ) ) ;
#70759=CARTESIAN_POINT ( 'NONE',  ( 177.7342311040593756, 255.2532439957012684, -8.367404576774948310 ) ) ;
#70761=CARTESIAN_POINT ( 'NONE',  ( 148.1004780136491377, 274.1294427855589788, -7.811560775291159331 ) ) ;
#70765=CARTESIAN_POINT ( 'NONE',  ( 190.6453411250757313, 284.1316474202013183, -17.46766191648467625 ) ) ;
#70766=CARTESIAN_POINT ( 'NONE',  ( 191.9852310057781040, 298.1188209255817014, -9.473644331849939704 ) ) ;
#70767=CARTESIAN_POINT ( 'NONE',  ( 149.6036070299368532, 271.5259469590175740, 11.63513718912356865 ) ) ;
#70769=CARTESIAN_POINT ( 'NONE',  ( 204.6288132990387965, 273.0563504000126045, -9.947042290372426265 ) ) ;
#70770=CARTESIAN_POINT ( 'NONE',  ( 164.7092427929301550, 283.9547367519082854, -6.819220165404522582 ) ) ;
#70771=CARTESIAN_POINT ( 'NONE',  ( 151.4859849967579919, 274.9594807944311015, -8.716721077935043027 ) ) ;
#70772=DIRECTION ( 'NONE',  ( 0.4999999999999998890, -0.8660254037844385966, 0.000000000000000000 ) ) ;
#70775=CARTESIAN_POINT ( 'NONE',  ( 147.5177358149801421, 275.1387818813681179, 4.867883209065928085 ) ) ;
#70776=EDGE_CURVE ( 'NONE', #86172, #32812, #86830, .T. ) ;
#70778=CARTESIAN_POINT ( 'NONE',  ( 193.5405458432471164, 276.0738629501939272, -16.60598989773238188 ) ) ;
#70779=CARTESIAN_POINT ( 'NONE',  ( 149.0710170770012724, 245.3262482093457777, 3.021315404115420679E-15 ) ) ;
#70781=CARTESIAN_POINT ( 'NONE',  ( 188.5029508706952015, 298.7682505406680775, -3.886380934741553883 ) ) ;
#70782=B_SPLINE_CURVE_WITH_KNOTS ( 'NONE', 3,
 ( #83234, #97434, #82264, #82759, #83742, #14305, #97922, #91837, #28004, #5214, #43697, #66508, #98924, #51817, #59891, #45191, #75613, #12836, #58882, #51292, #76130, #35610, #89850, #36095, #6705, #28498 ),
 .UNSPECIFIED., .F., .F.,
 ( 4, 2, 2, 2, 2, 2, 2, 2, 2, 2, 2, 2, 4 ),
 ( 0.0004635842473323659716, 0.001626875584096156924, 0.002790166920859947931, 0.003371812589241843759, 0.003517224006337276842, 0.003662635423432709925, 0.003735341131980426683, 0.003808046840528143441, 0.003953458257623576957, 0.004244281091814402357, 0.004535103926005227756, 0.004825926760196054023, 0.005116749594386879423 ),
 .UNSPECIFIED. ) ;
#70785=EDGE_CURVE ( 'NONE', #6903, #37817, #36427, .T. ) ;
#70787=CARTESIAN_POINT ( 'NONE',  ( -5.895715345004023611, 160.7365022471902023, -10.00000000000009237 ) ) ;
#70789=CARTESIAN_POINT ( 'NONE',  ( -11.73236572436687730, 164.0333772461660544, 9.188101187500095079 ) ) ;
#70790=CARTESIAN_POINT ( 'NONE',  ( 92.21748570181026139, 233.2369531367911009, -4.594050593750048428 ) ) ;
#70792=CARTESIAN_POINT ( 'NONE',  ( 192.4743214706506365, 297.2716913909250707, -12.17804856100553046 ) ) ;
#70793=CARTESIAN_POINT ( 'NONE',  ( 182.2991478702006134, 275.2734891516705034, -17.80812521087705846 ) ) ;
#70794=CARTESIAN_POINT ( 'NONE',  ( 155.1601726304954809, 261.9016930232608615, -18.56587418422714464 ) ) ;
#70795=EDGE_CURVE ( 'NONE', #14672, #67236, #94174, .T. ) ;
#70796=B_SPLINE_CURVE_WITH_KNOTS ( 'NONE', 3,
 ( #61237, #37433, #84103, #68343 ),
 .UNSPECIFIED., .F., .F.,
 ( 4, 4 ),
 ( 0.03983647665132224180, 0.04828245132308466026 ),
 .UNSPECIFIED. ) ;
#70803=EDGE_CURVE ( 'NONE', #23380, #50052, #11977, .T. ) ;
#70804=CARTESIAN_POINT ( 'NONE',  ( 161.3538429669452512, 251.1739413151977089, 12.93463751804771533 ) ) ;
#70806=CARTESIAN_POINT ( 'NONE',  ( 165.9674733710236296, 249.3024098291379289, -9.244165487746641929 ) ) ;
#70807=CARTESIAN_POINT ( 'NONE',  ( 164.7631898711947827, 245.2687792564100562, -5.064413554850759169 ) ) ;
#70808=CARTESIAN_POINT ( 'NONE',  ( 195.7291850945597957, 291.6341022226063160, 17.08310330964873813 ) ) ;
#70811=CARTESIAN_POINT ( 'NONE',  ( 31.67681054456310008, 201.3464784336661353, 1.353441290958777327E-15 ) ) ;
#70813=CARTESIAN_POINT ( 'NONE',  ( 68.53719034102077501, 216.5024278399160664, 9.188101187500095079 ) ) ;
#70819=CARTESIAN_POINT ( 'NONE',  ( 200.2320358376919103, 270.9633186839029690, -11.45871590196247070 ) ) ;
#70824=CARTESIAN_POINT ( 'NONE',  ( 64.58612298413676456, 208.0958772461660544, -9.188101187500095079 ) ) ;
#70826=CARTESIAN_POINT ( 'NONE',  ( 202.7602807045765019, 279.4558873931827065, -15.90558713185497020 ) ) ;
#70827=CARTESIAN_POINT ( 'NONE',  ( 198.2114954873088948, 287.3346145022089786, 18.52864136173620935 ) ) ;
#70829=CARTESIAN_POINT ( 'NONE',  ( 153.8947951769603719, 264.0933910635359325, 16.60696150718446518 ) ) ;
#70831=CARTESIAN_POINT ( 'NONE',  ( 115.3478411848173835, 230.7365022471902023, 10.00000000000009592 ) ) ;
#70833=CARTESIAN_POINT ( 'NONE',  ( 164.2953672501826929, 246.0790718049323687, -2.576662677987826111 ) ) ;
#70839=CARTESIAN_POINT ( 'NONE',  ( 159.3995226465659982, 254.5589234043588078, -16.81133486613867234 ) ) ;
#70840=CARTESIAN_POINT ( 'NONE',  ( 194.2428668711552007, 293.6808394427342819, 14.33833691752719375 ) ) ;
#70842=ORIENTED_EDGE ( 'NONE', *, *, #39180, .T. ) ;
#70846=CARTESIAN_POINT ( 'NONE',  ( 167.4264173877831468, 247.7494294226382294, 3.562207888615490425 ) ) ;
#70850=ADVANCED_FACE ( 'NONE', ( #87107 ), #17645, .T. ) ;
#70851=AXIS2_PLACEMENT_3D ( 'NONE', #20026, #59985, #50900 ) ;
#70853=CARTESIAN_POINT ( 'NONE',  ( 21.87918239556003641, 194.9860189848785410, -2.679491924311252493 ) ) ;
#70856=ADVANCED_FACE ( 'NONE', ( #23223 ), #63233, .T. ) ;
#70861=CARTESIAN_POINT ( 'NONE',  ( 170.8150813163964585, 284.7511851418007609, 11.02223257947848012 ) ) ;
#70863=CARTESIAN_POINT ( 'NONE',  ( 162.9111130980074620, 284.4370125796830848, -2.463596310689824875 ) ) ;
#70866=CARTESIAN_POINT ( 'NONE',  ( 194.2764122224708103, 294.1503786489221284, 15.46903869661980835 ) ) ;
#70867=CARTESIAN_POINT ( 'NONE',  ( 160.8753431536632945, 265.5703843255740253, 17.74957321532883014 ) ) ;
#70868=CARTESIAN_POINT ( 'NONE',  ( 164.3157126687612504, 265.7538407082229241, -17.18074097244921816 ) ) ;
#70869=CARTESIAN_POINT ( 'NONE',  ( 133.4890956248536895, 254.0024278399161233, 9.188101187500095079 ) ) ;
#70871=CARTESIAN_POINT ( 'NONE',  ( 206.8217325168575371, 270.0045844243117017, 3.350393751014514532 ) ) ;
#70874=CARTESIAN_POINT ( 'NONE',  ( 77.73871025623044773, 221.8149278399160949, -9.188101187500095079 ) ) ;
#70879=CARTESIAN_POINT ( 'NONE',  ( 195.6782192648066427, 291.7223776291889408, -15.68068164243272022 ) ) ;
#70881=B_SPLINE_CURVE_WITH_KNOTS ( 'NONE', 3,
 ( #50451, #90505, #12981, #66652 ),
 .UNSPECIFIED., .F., .F.,
 ( 4, 4 ),
 ( 0.04313187872937399719, 0.04472034873244652015 ),
 .UNSPECIFIED. ) ;
#70888=CARTESIAN_POINT ( 'NONE',  ( 47.85994450909318232, 209.9860189848785410, -2.679491924311201423 ) ) ;
#70889=CARTESIAN_POINT ( 'NONE',  ( 207.5492168967516875, 271.1612065941299079, 2.279797467183042325 ) ) ;
#70891=CARTESIAN_POINT ( 'NONE',  ( 79.20030167299918844, 216.5333772461660544, 9.188101187500095079 ) ) ;
#70895=CARTESIAN_POINT ( 'NONE',  ( 163.2742264920156572, 247.8477394797576778, -9.850275379362519956 ) ) ;
#70896=EDGE_LOOP ( 'NONE', ( #94897, #97897, #93553, #80023 ) ) ;
#70903=CARTESIAN_POINT ( 'NONE',  ( 184.7820298688179719, 260.0036009586479508, 6.327424396724815381 ) ) ;
#70904=CARTESIAN_POINT ( 'NONE',  ( 206.3454060440500086, 273.2462681537123785, -9.268083217908118954 ) ) ;
#70905=CARTESIAN_POINT ( 'NONE',  ( 193.9866089479436368, 275.7653998617566913, 16.75281791482838400 ) ) ;
#70906=CARTESIAN_POINT ( 'NONE',  ( 174.6633675210554486, 283.9072383021423320, 13.76783388809871056 ) ) ;
#70907=( BOUNDED_CURVE ( )  B_SPLINE_CURVE ( 2, ( #70779, #38363, #69273, #62156, #47472, #93103, #30787 ),
 .UNSPECIFIED., .F., .T. ) 
 B_SPLINE_CURVE_WITH_KNOTS ( ( 3, 2, 2, 3 ),
 ( 0.9798387096774193727, 0.9811827956989247479, 0.9838709677419354982, 0.9855294979220013962 ),
 .UNSPECIFIED. ) 
 CURVE ( )  GEOMETRIC_REPRESENTATION_ITEM ( )  RATIONAL_B_SPLINE_CURVE ( ( 0.9330127018922194093, 0.9330127018922194093, 1.000000000000000000, 0.8660254037844387076, 1.000000000000000000, 0.9173412610389377608, 0.9366789799084298540 ) ) 
 REPRESENTATION_ITEM ( '' )  );
#70908=CYLINDRICAL_SURFACE ( 'NONE', #93732, 10.00000000000010658 ) ;
#70909=B_SPLINE_CURVE_WITH_KNOTS ( 'NONE', 3,
 ( #49820, #56415, #4212, #71647, #64528, #34133, #88893, #18943, #11351, #72141, #50311, #10336, #73142, #42207 ),
 .UNSPECIFIED., .F., .F.,
 ( 4, 2, 2, 2, 2, 2, 4 ),
 ( 0.0007774119382052871018, 0.001058953235776235405, 0.001340494533347183926, 0.001622035830918132230, 0.001903577128489080750, 0.002466659723631069515, 0.003029742318773058496 ),
 .UNSPECIFIED. ) ;
#70910=CARTESIAN_POINT ( 'NONE',  ( 195.5865870811380205, 279.6577477989692397, -17.40305323361667433 ) ) ;
#70911=VERTEX_POINT ( 'NONE', #57620 ) ;
#70912=CARTESIAN_POINT ( 'NONE',  ( 203.3892195006453107, 277.9383451777727032, -14.51582383987914149 ) ) ;
#70914=CARTESIAN_POINT ( 'NONE',  ( 181.1156277128715431, 292.7914473640799997, 9.490545386343454126 ) ) ;
#70916=CARTESIAN_POINT ( 'NONE',  ( 185.5597808477625961, 264.6293126611748789, -11.95344273703673466 ) ) ;
#70918=CARTESIAN_POINT ( 'NONE',  ( 153.7922915876480090, 270.4832132560703712, 14.01318345560697765 ) ) ;
#70924=CIRCLE ( 'NONE', #79045, 17.82106496071138935 ) ;
#70925=EDGE_CURVE ( 'NONE', #57797, #34618, #93983, .T. ) ;
#70926=CARTESIAN_POINT ( 'NONE',  ( 165.0509870607838252, 244.7702999017660375, -2.356357909806504392 ) ) ;
#70927=CARTESIAN_POINT ( 'NONE',  ( 180.2669822489033322, 266.6255696747526258, -14.77114471355729108 ) ) ;
#70931=CARTESIAN_POINT ( 'NONE',  ( 162.8496566865346438, 284.5585608631904506, -4.049346908545373047 ) ) ;
#70932=CARTESIAN_POINT ( 'NONE',  ( 160.1969820541083607, 255.1776831935258372, -16.37528374203482073 ) ) ;
#70933=CARTESIAN_POINT ( 'NONE',  ( 188.3509091528505905, 260.8885577967712379, 2.876703767957366598 ) ) ;
#70934=CARTESIAN_POINT ( 'NONE',  ( 195.3381664883222300, 265.3235058747017092, -7.510424545325947498 ) ) ;
#70936=CARTESIAN_POINT ( 'NONE',  ( 6.102605256642664067, 165.1423013555410080, -4.594050593750043987 ) ) ;
#70937=CARTESIAN_POINT ( 'NONE',  ( -27.42236680055714260, 166.5217562850347406, 1.224646799147364892E-15 ) ) ;
#70941=CARTESIAN_POINT ( 'NONE',  ( 160.2340067623557616, 254.0231382518209386, -15.28591403396486470 ) ) ;
#70942=DIRECTION ( 'NONE',  ( -0.8660254037844387076, -0.4999999999999998890, -0.000000000000000000 ) ) ;
#70944=CARTESIAN_POINT ( 'NONE',  ( 13.16551753867071461, 190.6589784336661637, -6.496448406907676862E-16 ) ) ;
#70945=CARTESIAN_POINT ( 'NONE',  ( 173.2322951681075551, 290.9646578649885669, 3.668310523228456965 ) ) ;
#70948=CARTESIAN_POINT ( 'NONE',  ( 189.4090321304425970, 263.6681562366250091, -10.67085280218717003 ) ) ;
#70949=CARTESIAN_POINT ( 'NONE',  ( 147.2592533090473239, 275.5864867145116932, -0.3770461397900867762 ) ) ;
#70952=B_SPLINE_SURFACE_WITH_KNOTS ( 'NONE', 3, 1, ( 
 ( #21949, #22449 ),
 ( #53345, #76652 ),
 ( #45730, #7241 ),
 ( #44732, #28055 ),
 ( #58930, #20479 ),
 ( #82318, #43746 ),
 ( #5268, #13375 ),
 ( #67051, #97974 ),
 ( #20986, #51869 ),
 ( #29073, #59938 ),
 ( #75668, #68050 ),
 ( #6252, #16347 ),
 ( #70540, #46743 ),
 ( #40127, #8748 ),
 ( #71066, #70035 ),
 ( #15837, #93384 ),
 ( #23937, #55328 ),
 ( #86305, #84787 ),
 ( #78160, #54835 ),
 ( #648, #16839 ),
 ( #47241, #94385 ),
 ( #61437, #15326 ),
 ( #69546, #79195 ),
 ( #85818, #32551 ),
 ( #53827, #9769 ),
 ( #47730, #7749 ),
 ( #30554, #78663 ),
 ( #77670, #151 ),
 ( #31535, #55815 ),
 ( #24938, #93893 ),
 ( #39619, #69039 ),
 ( #86808, #22937 ),
 ( #31040, #99969 ),
 ( #1668, #92391 ) ),
 .UNSPECIFIED., .T., .F., .F.,
 ( 4, 2, 2, 2, 2, 2, 2, 2, 2, 2, 2, 2, 2, 2, 2, 2, 4 ),
 ( 2, 2 ),
 ( 0.000000000000000000, 0.06250000000000000000, 0.1250000000000000000, 0.1875000000000000000, 0.2500000000000000000, 0.3125000000000000000, 0.3750000000000000000, 0.4375000000000000000, 0.5000000000000000000, 0.5625000000000000000, 0.6250000000000000000, 0.6875000000000000000, 0.7500000000000000000, 0.8125000000000000000, 0.8750000000000000000, 0.9375000000000000000, 1.000000000000000000 ),
 ( 0.000000000000000000, 1.000000000000000000 ),
 .UNSPECIFIED. ) ;
#70953=CARTESIAN_POINT ( 'NONE',  ( 186.9530661741948450, 295.9748403543025574, -7.697179163675227365 ) ) ;
#70954=CARTESIAN_POINT ( 'NONE',  ( 190.7500944235871998, 261.9717678648361812, -0.8447403391411513196 ) ) ;
#70955=CARTESIAN_POINT ( 'NONE',  ( 74.64464720694877542, 207.2365022471902023, -10.00000000000009059 ) ) ;
#70958=DIRECTION ( 'NONE',  ( -0.4999999999999987788, 0.8660254037844392627, 0.000000000000000000 ) ) ;
#70959=B_SPLINE_CURVE_WITH_KNOTS ( 'NONE', 3,
 ( #51468, #59042, #12999, #81419 ),
 .UNSPECIFIED., .F., .F.,
 ( 4, 4 ),
 ( 0.03583253215054491014, 0.04455304000076568821 ),
 .UNSPECIFIED. ) ;
#70960=FACE_OUTER_BOUND ( 'NONE', #12933, .T. ) ;
#70961=CARTESIAN_POINT ( 'NONE',  ( 29.51209413086700906, 187.8458772461660544, 9.188101187500095079 ) ) ;
#70962=CARTESIAN_POINT ( 'NONE',  ( 159.2303255284352304, 254.8519814094557603, 16.39103317446447150 ) ) ;
#70968=CARTESIAN_POINT ( 'NONE',  ( 80.56248746614238598, 223.9865022471902876, 10.00000000000009415 ) ) ;
#70970=CARTESIAN_POINT ( 'NONE',  ( 163.2169812233754840, 281.0183292176826626, -10.13472441872696805 ) ) ;
#70971=LINE ( 'NONE', #62841, #61712 ) ;
#70973=CARTESIAN_POINT ( 'NONE',  ( 163.2437751800324293, 247.9004826992694461, 9.806027032984305336 ) ) ;
#70974=CARTESIAN_POINT ( 'NONE',  ( 197.0226655822963551, 289.3937282992477549, -17.28982543158101493 ) ) ;
#70976=CARTESIAN_POINT ( 'NONE',  ( 185.5122645235197467, 267.6225438542603570, -14.65295725662480386 ) ) ;
#70978=CARTESIAN_POINT ( 'NONE',  ( 185.5535017383455454, 290.7975388464344064, 12.55098773011679469 ) ) ;
#70983=CARTESIAN_POINT ( 'NONE',  ( 25.50001727096127979, 173.9824982072973967, 3.021315404115420679E-15 ) ) ;
#70985=CARTESIAN_POINT ( 'NONE',  ( 191.4044787581200069, 299.1247133251352466, 7.435199718141230818 ) ) ;
#70986=CARTESIAN_POINT ( 'NONE',  ( 181.0633185409454597, 257.6960604115657816, -7.513758380418855687 ) ) ;
#70988=ORIENTED_EDGE ( 'NONE', *, *, #50326, .F. ) ;
#70989=CARTESIAN_POINT ( 'NONE',  ( 148.3010860587701814, 276.5068540982774721, -3.904121881399305050 ) ) ;
#70992=CARTESIAN_POINT ( 'NONE',  ( 200.9445292274600092, 282.6008612054670266, -16.62830946367346741 ) ) ;
#70997=CARTESIAN_POINT ( 'NONE',  ( 204.9658583905037688, 275.6357147811169170, -12.57240504404813564 ) ) ;
#70998=CARTESIAN_POINT ( 'NONE',  ( 100.7430306879021060, 216.7202760586659167, -5.415160957724236172E-17 ) ) ;
#71000=AXIS2_PLACEMENT_3D ( 'NONE', #9151, #17239, #2567 ) ;
#71001=CARTESIAN_POINT ( 'NONE',  ( 181.5074763156532072, 287.3577042999648370, -13.30743195732708450 ) ) ;
#71002=ORIENTED_EDGE ( 'NONE', *, *, #74554, .T. ) ;
#71004=CARTESIAN_POINT ( 'NONE',  ( 162.1885223555109974, 266.5710106843741869, 17.09332258216276657 ) ) ;
#71005=EDGE_LOOP ( 'NONE', ( #75112, #93549, #67487, #27348 ) ) ;
#71007=CARTESIAN_POINT ( 'NONE',  ( 157.2469855225926381, 258.6801040481246332, 16.82957450039010538 ) ) ;
#71009=CARTESIAN_POINT ( 'NONE',  ( 59.17381130624904984, 192.7202760586659451, -5.415160957724236172E-17 ) ) ;
#71013=CARTESIAN_POINT ( 'NONE',  ( 150.2982063762752603, 270.3228656002555681, 14.90512853129094495 ) ) ;
#71014=CARTESIAN_POINT ( 'NONE',  ( 176.6036273517752875, 273.2589018324615608, 17.10821691637876540 ) ) ;
#71016=ORIENTED_EDGE ( 'NONE', *, *, #27450, .F. ) ;
#71018=CARTESIAN_POINT ( 'NONE',  ( 190.7573459890224683, 299.4656496600463242, 6.232719852847871778 ) ) ;
#71020=CARTESIAN_POINT ( 'NONE',  ( 147.2443490232117256, 275.6123016948292275, 5.226063659459642352 ) ) ;
#71023=CARTESIAN_POINT ( 'NONE',  ( 174.5672763864540968, 261.0320004397244702, -14.05403048710671854 ) ) ;
#71024=CARTESIAN_POINT ( 'NONE',  ( 170.6811438746260592, 275.2999556018212388, -16.27734202032215904 ) ) ;
#71025=CARTESIAN_POINT ( 'NONE',  ( 207.7320178805681508, 270.8445860024863237, -5.379955943374661764 ) ) ;
#71026=CARTESIAN_POINT ( 'NONE',  ( 147.4824818982269790, 275.1998434563504929, -4.972419998968698351 ) ) ;
#71027=CARTESIAN_POINT ( 'NONE',  ( 190.8138402884741254, 300.1477291634665789, 4.037153726988762514 ) ) ;
#71028=CARTESIAN_POINT ( 'NONE',  ( 180.5385023393456834, 271.2514381441214368, 16.52379068675051599 ) ) ;
#71029=CYLINDRICAL_SURFACE ( 'NONE', #9445, 17.82106496071139645 ) ;
#71032=CARTESIAN_POINT ( 'NONE',  ( 163.7038023771459052, 247.1036922210055025, -6.448491958542482472 ) ) ;
#71033=CARTESIAN_POINT ( 'NONE',  ( 112.2171730965159071, 247.8464784336661353, 1.353441290958777327E-15 ) ) ;
#71035=CARTESIAN_POINT ( 'NONE',  ( 191.2111338740054975, 299.4595964878050154, -9.718193530796334301 ) ) ;
#71037=CARTESIAN_POINT ( 'NONE',  ( 155.6281496932864457, 261.0911329737299980, -18.07904265579665548 ) ) ;
#71038=CARTESIAN_POINT ( 'NONE',  ( 163.7239493340838123, 247.0687966679708438, 6.286946239157660266 ) ) ;
#71039=DIRECTION ( 'NONE',  ( -0.8660254037844387076, -0.4999999999999998890, -0.000000000000000000 ) ) ;
#71040=CARTESIAN_POINT ( 'NONE',  ( 177.9425579050794965, 255.3610639913140972, 4.864846912946482860 ) ) ;
#71042=CARTESIAN_POINT ( 'NONE',  ( 207.5959034698703078, 271.0803430774575418, -1.830000129038042544 ) ) ;
#71044=CARTESIAN_POINT ( 'NONE',  ( 158.4807356281016553, 274.9683795502273824, -12.52945643738231674 ) ) ;
#71045=CARTESIAN_POINT ( 'NONE',  ( 182.4400702163412404, 260.6821622823035227, 9.500263120530494376 ) ) ;
#71046=CARTESIAN_POINT ( 'NONE',  ( 206.4738852556816369, 273.0237356314501085, -9.746110091792012042 ) ) ;
#71047=CARTESIAN_POINT ( 'NONE',  ( 134.7341806906763395, 248.5958772461660544, -9.188101187500095079 ) ) ;
#71048=CARTESIAN_POINT ( 'NONE',  ( 189.8764391022526183, 294.5890629899907935, -12.42416005126432310 ) ) ;
#71049=CARTESIAN_POINT ( 'NONE',  ( -22.42236680055709641, 157.8615022471902591, 0.000000000000000000 ) ) ;
#71050=CARTESIAN_POINT ( 'NONE',  ( 196.3341081413628899, 290.5863447708742342, 16.12390540996472410 ) ) ;
#71051=CYLINDRICAL_SURFACE ( 'NONE', #9456, 10.00000000000010658 ) ;
#71052=CARTESIAN_POINT ( 'NONE',  ( 51.43353571204313823, 194.3768266524159856, -9.188101187500091527 ) ) ;
#71055=ADVANCED_FACE ( 'NONE', ( #26736 ), #1390, .F. ) ;
#71057=CARTESIAN_POINT ( 'NONE',  ( 171.5539035853818746, 260.2959543727399705, 14.72132304298182248 ) ) ;
#71058=CARTESIAN_POINT ( 'NONE',  ( 151.4588969340128983, 278.2628330447197982, -1.654564867966292319 ) ) ;
#71059=CARTESIAN_POINT ( 'NONE',  ( 178.8787720380167912, 291.7606112093855018, -6.206199073717809434 ) ) ;
#71061=CARTESIAN_POINT ( 'NONE',  ( 153.7185388398659711, 269.2090732872851504, -15.41358683631291271 ) ) ;
#71062=CARTESIAN_POINT ( 'NONE',  ( 127.5984922056368731, 231.1427522451417360, 1.119607411625061291E-15 ) ) ;
#71064=VERTEX_POINT ( 'NONE', #38679 ) ;
#71066=CARTESIAN_POINT ( 'NONE',  ( 202.3425522658138505, 280.1794142728863903, 15.86053073629060961 ) ) ;
#71068=CARTESIAN_POINT ( 'NONE',  ( 18.68642948779652002, 193.8464784336661637, 1.353441290958777327E-15 ) ) ;
#71069=AXIS2_PLACEMENT_3D ( 'NONE', #88788, #73047, #49718 ) ;
#71071=CARTESIAN_POINT ( 'NONE',  ( 188.7203383489409134, 290.4861718803290955, -14.87964105563550277 ) ) ;
#71074=CARTESIAN_POINT ( 'NONE',  ( 177.1262862392189845, 269.6057104283654553, 17.56656865388298172 ) ) ;
#71075=CARTESIAN_POINT ( 'NONE',  ( 58.38862868653046689, 194.5177522451417929, 5.000000000000051514 ) ) ;
#71077=CARTESIAN_POINT ( 'NONE',  ( 184.2320252568399894, 257.8019328292739374, 1.345153837617685255 ) ) ;
#71078=CARTESIAN_POINT ( 'NONE',  ( 204.9184781223158609, 275.7177798128946620, -12.59106622113254126 ) ) ;
#71082=AXIS2_PLACEMENT_3D ( 'NONE', #99875, #42781, #4297 ) ;
#71083=CARTESIAN_POINT ( 'NONE',  ( 161.4250356354754672, 267.9004136800010656, 17.49898951125957680 ) ) ;
#71084=CARTESIAN_POINT ( 'NONE',  ( 28.60096323907606219, 193.9865022471902876, 10.00000000000009237 ) ) ;
#71085=CARTESIAN_POINT ( 'NONE',  ( 39.40823858692152015, 186.8927522451417929, -10.00000000000009237 ) ) ;
#71086=CARTESIAN_POINT ( 'NONE',  ( 162.6626107288841467, 248.9070890562113902, 10.12509462564867313 ) ) ;
#71087=CARTESIAN_POINT ( 'NONE',  ( -7.997804718428996651, 172.3149278399160949, -9.188101187500095079 ) ) ;
#71090=CARTESIAN_POINT ( 'NONE',  ( 181.2305971022323661, 265.9781236237157032, -15.82518789413146010 ) ) ;
#71092=CARTESIAN_POINT ( 'NONE',  ( 187.8353293621520663, 261.5626033622391446, 6.406781397797947086 ) ) ;
#71093=CARTESIAN_POINT ( 'NONE',  ( 205.7829192689729325, 274.2205238267313234, 11.21202327925415254 ) ) ;
#71094=CARTESIAN_POINT ( 'NONE',  ( 187.1283629995790250, 258.9907284234702161, -2.438144316879867990 ) ) ;
#71096=EDGE_LOOP ( 'NONE', ( #90696, #87396, #28003, #71202 ) ) ;
#71097=CYLINDRICAL_SURFACE ( 'NONE', #17999, 17.82106496071139645 ) ;
#71099=CARTESIAN_POINT ( 'NONE',  ( 178.4448961284112158, 285.5018398465763312, 12.98938652614517153 ) ) ;
#71100=CARTESIAN_POINT ( 'NONE',  ( 153.2952765687912802, 277.6672861512745385, -5.343879082789506185 ) ) ;
#71102=AXIS2_PLACEMENT_3D ( 'NONE', #27100, #10400, #64598 ) ;
#71103=CARTESIAN_POINT ( 'NONE',  ( 160.6541084136885615, 252.3859171132495476, 15.19188851725936118 ) ) ;
#71104=CARTESIAN_POINT ( 'NONE',  ( 159.2713554375903300, 254.7809155221686410, -15.70062444474382168 ) ) ;
#71105=CARTESIAN_POINT ( 'NONE',  ( 63.33450210234187239, 195.8262482093458061, 3.021315404115420679E-15 ) ) ;
#71107=CARTESIAN_POINT ( 'NONE',  ( 104.7876960802104946, 219.7592609112380160, 2.679491924311254714 ) ) ;
#71111=CARTESIAN_POINT ( 'NONE',  ( 155.7862279768771714, 277.0639705730557694, -10.34674495731000654 ) ) ;
#71112=FACE_OUTER_BOUND ( 'NONE', #1940, .T. ) ;
#71117=CARTESIAN_POINT ( 'NONE',  ( 146.5046981847821428, 276.8934145268504494, 0.02269072295920678689 ) ) ;
#71120=CARTESIAN_POINT ( 'NONE',  ( 176.0798903307563990, 267.4715319269637916, 17.29251186195777379 ) ) ;
#71121=ORIENTED_EDGE ( 'NONE', *, *, #64706, .T. ) ;
#71122=CARTESIAN_POINT ( 'NONE',  ( 161.0952649348064938, 251.6218116045831437, 13.81854265722852482 ) ) ;
#71124=CARTESIAN_POINT ( 'NONE',  ( 177.3946647576825910, 293.3261284689752415, 3.859629117064975468 ) ) ;
#71126=CARTESIAN_POINT ( 'NONE',  ( 151.3579658450212264, 274.9463947945409359, -8.627328198253888303 ) ) ;
#71127=ORIENTED_EDGE ( 'NONE', *, *, #33879, .F. ) ;
#71128=CARTESIAN_POINT ( 'NONE',  ( 193.2752197284765998, 263.9480352582601768, 7.898392093415175452 ) ) ;
#71139=CARTESIAN_POINT ( 'NONE',  ( 166.8502408137956081, 271.8018640180155217, 16.11660651124998367 ) ) ;
#71142=CARTESIAN_POINT ( 'NONE',  ( 194.3177355571849318, 294.0788045336591381, -15.93712594727561616 ) ) ;
#71145=CARTESIAN_POINT ( 'NONE',  ( 197.7108840479781122, 288.2016989499799138, -17.75818441575643902 ) ) ;
#71149=CARTESIAN_POINT ( 'NONE',  ( 205.7867067512454184, 274.2139637150027056, 10.62737868262404106 ) ) ;
#71150=CARTESIAN_POINT ( 'NONE',  ( 190.7404869014439726, 298.2747809567102308, -9.591077548819823662 ) ) ;
#71154=CARTESIAN_POINT ( 'NONE',  ( 190.9873456450184506, 299.8472090705463984, 5.391280221519696880 ) ) ;
#71155=CARTESIAN_POINT ( 'NONE',  ( 154.1396649810517090, 268.6945475872249744, 16.07262325421418936 ) ) ;
#71156=CARTESIAN_POINT ( 'NONE',  ( 159.7692415128758228, 253.9185515433934768, -16.85856106119654285 ) ) ;
#71157=DIRECTION ( 'NONE',  ( -0.8660254037844387076, -0.4999999999999998890, -0.000000000000000000 ) ) ;
#71158=CARTESIAN_POINT ( 'NONE',  ( 200.9111546617170916, 282.6586676490145464, 17.66063511622358106 ) ) ;
#71159=CARTESIAN_POINT ( 'NONE',  ( 112.7497649734640959, 229.2365022471902307, 10.00000000000009948 ) ) ;
#71162=CARTESIAN_POINT ( 'NONE',  ( 190.7982574810033611, 262.8194055429554510, 8.405793748174573921 ) ) ;
#71165=CARTESIAN_POINT ( 'NONE',  ( 126.0342816572616016, 255.1199935810940929, 2.679491924311251605 ) ) ;
#71167=CARTESIAN_POINT ( 'NONE',  ( 9.891206074601820220, 186.5177522451419065, 5.000000000000046185 ) ) ;
#71168=CARTESIAN_POINT ( 'NONE',  ( 86.94057726720511425, 214.8768266524160140, 9.188101187500096856 ) ) ;
#71172=CARTESIAN_POINT ( 'NONE',  ( 8.727484440040480962, 175.8458772461660828, 9.188101187500095079 ) ) ;
#71175=CARTESIAN_POINT ( 'NONE',  ( 161.5504728662519369, 250.8333683393111926, 12.94300825113363373 ) ) ;
#71178=CARTESIAN_POINT ( 'NONE',  ( 197.5198955408084487, 265.2020030822665717, -2.944437631376198183 ) ) ;
#71183=CARTESIAN_POINT ( 'NONE',  ( 105.5870131927823081, 241.7677522451419065, -5.000000000000047962 ) ) ;
#71185=CARTESIAN_POINT ( 'NONE',  ( 37.63108229134613225, 192.5333772461660544, 9.188101187500095079 ) ) ;
#71186=CARTESIAN_POINT ( 'NONE',  ( 73.90491717100159974, 220.1427522451418781, 10.00000000000009237 ) ) ;
#71187=CARTESIAN_POINT ( 'NONE',  ( 199.4661499282636044, 277.5283185301939284, 15.18718668142867934 ) ) ;
#71188=VERTEX_POINT ( 'NONE', #16387 ) ;
#71189=CARTESIAN_POINT ( 'NONE',  ( 152.1915498382297471, 272.9642279343270275, -11.71006468322317140 ) ) ;
#71190=CARTESIAN_POINT ( 'NONE',  ( 175.2874222581449430, 281.1428048220561777, -14.59610539211987401 ) ) ;
#71191=ADVANCED_FACE ( 'NONE', ( #86349 ), #54715, .F. ) ;
#71192=CARTESIAN_POINT ( 'NONE',  ( -13.97887943725652882, 171.9244531367911293, -4.594050593750046652 ) ) ;
#71193=CARTESIAN_POINT ( 'NONE',  ( 196.0395593785976018, 291.0965181932902510, 15.97855489120023087 ) ) ;
#71195=CARTESIAN_POINT ( 'NONE',  ( 151.2567985338353935, 268.6625352796243646, -15.71756535662528798 ) ) ;
#71196=CARTESIAN_POINT ( 'NONE',  ( 186.9138942552878575, 282.8138041189644696, 16.19480528300033839 ) ) ;
#71197=CARTESIAN_POINT ( 'NONE',  ( 194.9385458806846430, 293.0035295114944347, -15.70518692812489192 ) ) ;
#71198=CARTESIAN_POINT ( 'NONE',  ( 192.6098662181048553, 265.0933516837970956, 7.612540007641825035 ) ) ;
#71199=CARTESIAN_POINT ( 'NONE',  ( 204.3951397407346064, 276.6242284793436852, 14.79595971842109137 ) ) ;
#71200=CARTESIAN_POINT ( 'NONE',  ( 76.37669801451765750, 208.2365022471902023, 10.00000000000009948 ) ) ;
#71201=CARTESIAN_POINT ( 'NONE',  ( 190.5154909595809727, 300.6644853595138329, -0.04129855346138300298 ) ) ;
#71202=ORIENTED_EDGE ( 'NONE', *, *, #51635, .T. ) ;
#71203=( BOUNDED_CURVE ( )  B_SPLINE_CURVE ( 2, ( #14577, #46441, #29768, #99182, #83012, #61653, #60641, #91597, #75389 ),
 .UNSPECIFIED., .F., .T. ) 
 B_SPLINE_CURVE_WITH_KNOTS ( ( 3, 2, 2, 2, 3 ),
 ( 0.3346774193548386900, 0.3360215053763440651, 0.3387096774193548154, 0.3413978494623655657, 0.3427419354838709964 ),
 .UNSPECIFIED. ) 
 CURVE ( )  GEOMETRIC_REPRESENTATION_ITEM ( )  RATIONAL_B_SPLINE_CURVE ( ( 0.9330127018922194093, 0.9330127018922194093, 1.000000000000000000, 0.8660254037844387076, 1.000000000000000000, 0.8660254037844387076, 1.000000000000000000, 0.9330127018922179660, 0.9330127018922194093 ) ) 
 REPRESENTATION_ITEM ( '' )  );
#71204=CARTESIAN_POINT ( 'NONE',  ( 12.21864935082045456, 177.8615022471902591, -10.00000000000009592 ) ) ;
#71205=CARTESIAN_POINT ( 'NONE',  ( 100.3364738622893810, 237.9244531367911009, -4.594050593750046652 ) ) ;
#71211=CARTESIAN_POINT ( 'NONE',  ( 150.0916500121360286, 245.9155109091895781, 2.679491924311254714 ) ) ;
#71212=CARTESIAN_POINT ( 'NONE',  ( 204.5701216393242987, 272.9108463828269464, -9.751758126869200183 ) ) ;
#71214=CARTESIAN_POINT ( 'NONE',  ( 196.9319848161575806, 289.5507919934690335, -17.64330560362266453 ) ) ;
#71216=CARTESIAN_POINT ( 'NONE',  ( 173.0532909196153071, 289.8873365335254562, -1.653350512543673378 ) ) ;
#71218=ORIENTED_EDGE ( 'NONE', *, *, #34950, .T. ) ;
#71219=CARTESIAN_POINT ( 'NONE',  ( 131.1144086761837571, 258.0530062829863027, -4.648177544792955347E-16 ) ) ;
#71220=CARTESIAN_POINT ( 'NONE',  ( 200.5914588262792222, 282.7033700937254821, -16.73555027083989444 ) ) ;
#71221=CARTESIAN_POINT ( 'NONE',  ( 156.1857201963304362, 277.6936791020598889, 10.39727624116721749 ) ) ;
#71228=CARTESIAN_POINT ( 'NONE',  ( 153.3100492430090753, 265.1062007306585997, 16.32434963471121492 ) ) ;
#71231=B_SPLINE_SURFACE_WITH_KNOTS ( 'NONE', 3, 1, ( 
 ( #12020, #87082 ),
 ( #89085, #27220 ),
 ( #19634, #49504 ),
 ( #3912, #80459 ),
 ( #79458, #65209 ),
 ( #96150, #57594 ),
 ( #4403, #50494 ),
 ( #34793, #10023 ),
 ( #88575, #19137 ),
 ( #65696, #73809 ),
 ( #41396, #50010 ),
 ( #40885, #96650 ),
 ( #35300, #94649 ),
 ( #25204, #18117 ),
 ( #2432, #79953 ),
 ( #33308, #95160 ),
 ( #10520, #68185 ),
 ( #59579, #89559 ),
 ( #51497, #74334 ),
 ( #13518, #74830 ),
 ( #98629, #35801 ),
 ( #21608, #43891 ),
 ( #21125, #36293 ),
 ( #20616, #52488 ),
 ( #29209, #5410 ),
 ( #67194, #59072 ),
 ( #66695, #5899 ),
 ( #98117, #4922 ),
 ( #99115, #22093 ),
 ( #82945, #45386 ),
 ( #97631, #36790 ),
 ( #90043, #28196 ),
 ( #28703, #67701 ),
 ( #83436, #60078 ) ),
 .UNSPECIFIED., .T., .F., .F.,
 ( 4, 2, 2, 2, 2, 2, 2, 2, 2, 2, 2, 2, 2, 2, 2, 2, 4 ),
 ( 2, 2 ),
 ( 0.000000000000000000, 0.06250000000000000000, 0.1250000000000000000, 0.1875000000000000000, 0.2500000000000000000, 0.3125000000000000000, 0.3750000000000000000, 0.4375000000000000000, 0.5000000000000000000, 0.5625000000000000000, 0.6250000000000000000, 0.6875000000000000000, 0.7500000000000000000, 0.8125000000000000000, 0.8750000000000000000, 0.9375000000000000000, 1.000000000000000000 ),
 ( 0.000000000000000000, 1.000000000000000000 ),
 .UNSPECIFIED. ) ;
#71233=CARTESIAN_POINT ( 'NONE',  ( 195.1200766625154017, 290.1138218968723663, -16.44780575384534771 ) ) ;
#71235=CARTESIAN_POINT ( 'NONE',  ( 163.9638979413247171, 279.3640461705110738, 12.10115734641663821 ) ) ;
#71237=CARTESIAN_POINT ( 'NONE',  ( 196.5144060520763105, 263.7350746926370562, -1.323704968039587815 ) ) ;
#71238=ORIENTED_EDGE ( 'NONE', *, *, #476, .T. ) ;
#71240=CARTESIAN_POINT ( 'NONE',  ( 188.7230124823968254, 293.4391532799720608, 12.65699786571403784 ) ) ;
#71241=CARTESIAN_POINT ( 'NONE',  ( 204.3951397407346064, 276.6242284793436852, 14.79595971842109137 ) ) ;
#71243=CARTESIAN_POINT ( 'NONE',  ( 155.3513572141771704, 261.5705516107003064, -17.00592413546589299 ) ) ;
#71247=CARTESIAN_POINT ( 'NONE',  ( 103.4941184669699794, 223.8927522451417929, 10.00000000000009948 ) ) ;
#71251=EDGE_CURVE ( 'NONE', #21258, #88994, #60012, .T. ) ;
#71252=CARTESIAN_POINT ( 'NONE',  ( 173.1761264927225454, 270.8446349882100321, 16.51755988034715017 ) ) ;
#71254=VERTEX_POINT ( 'NONE', #54188 ) ;
#71255=CARTESIAN_POINT ( 'NONE',  ( 186.0894263339278609, 282.3892669566888571, -16.72715339669124290 ) ) ;
#71256=CARTESIAN_POINT ( 'NONE',  ( 190.7042836556221062, 300.3374868178723887, 2.564074060554762280 ) ) ;
#71259=CARTESIAN_POINT ( 'NONE',  ( 201.4214977800931763, 281.7747274386935601, -17.04225209925078133 ) ) ;
#71263=CARTESIAN_POINT ( 'NONE',  ( 127.1021582719434662, 250.3149278399161233, -9.188101187500095079 ) ) ;
#71265=CARTESIAN_POINT ( 'NONE',  ( 186.8567874311567039, 262.4816910035492015, -10.18088338104968393 ) ) ;
#71270=B_SPLINE_CURVE_WITH_KNOTS ( 'NONE', 3,
 ( #98336, #7106, #60782, #66912, #75041, #90773, #83152, #82677, #59290, #36009, #28930, #5617, #90269, #45108, #13720, #37987, #91748, #76043, #21323, #61301, #29420, #60289, #20843, #21812, #52698, #13242, #75529, #68899, #99826, #6623, #30410, #59804, #83659, #84648, #67919, #37498, #6114, #68404, #37009, #84165, #22309, #91249, #46089, #99332, #53212, #14711 ),
 .UNSPECIFIED., .F., .F.,
 ( 4, 2, 2, 2, 2, 2, 2, 2, 2, 2, 2, 2, 2, 2, 2, 2, 2, 2, 2, 2, 2, 2, 4 ),
 ( 0.001500548513609991329, 0.001965505369317757569, 0.002430462225025523809, 0.002662940652879392835, 0.002779179866806390665, 0.002895419080733388061, 0.003011658294660385024, 0.003127897508587382854, 0.003360375936441254915, 0.003825332792148934419, 0.004290289647856613056, 0.005220203359271819409, 0.006150117070687024894, 0.006615073926394628503, 0.007080030782102231246, 0.007196269996029148845, 0.007254389602992554302, 0.007312509209955960626, 0.007544987637809759395, 0.008009944493517464487, 0.008474901349225167843, 0.008707379777079013450, 0.008939858204932860791 ),
 .UNSPECIFIED. ) ;
#71271=CARTESIAN_POINT ( 'NONE',  ( 203.5349748457618944, 276.1682765948387441, 13.32875452130744875 ) ) ;
#71272=CARTESIAN_POINT ( 'NONE',  ( 181.2270729396664706, 255.5114031541049826, 0.5804978543035055338 ) ) ;
#71273=CARTESIAN_POINT ( 'NONE',  ( 172.3006544489366263, 288.5207632028400440, -4.638716040452800726 ) ) ;
#71274=CARTESIAN_POINT ( 'NONE',  ( 192.0554304829709906, 297.9972318644188931, 11.99356102654441614 ) ) ;
#71276=CARTESIAN_POINT ( 'NONE',  ( 201.0356089830534643, 282.4431064412383989, -18.18835788025466371 ) ) ;
#71277=CARTESIAN_POINT ( 'NONE',  ( 173.3498119174590215, 287.3205656585489578, -9.768182251902993940 ) ) ;
#71278=CARTESIAN_POINT ( 'NONE',  ( 153.5053096856745469, 266.9305189219332419, 16.59624669306388967 ) ) ;
#71281=CARTESIAN_POINT ( 'NONE',  ( 194.6943296385021824, 293.4265244509877562, -16.10917128197217352 ) ) ;
#71282=CARTESIAN_POINT ( 'NONE',  ( 164.8489450237687493, 247.1202469751449939, -7.123750760659631531 ) ) ;
#71285=CARTESIAN_POINT ( 'NONE',  ( 190.9541724464728247, 283.5919873151655679, -16.59114474495747515 ) ) ;
#71286=CARTESIAN_POINT ( 'NONE',  ( 191.7730772792068308, 298.4862819590180720, -10.97593358402262886 ) ) ;
#71287=CARTESIAN_POINT ( 'NONE',  ( 190.0896302098338424, 301.4020978150248311, 3.433521196325825642 ) ) ;
#71288=CARTESIAN_POINT ( 'NONE',  ( 162.7644741734472120, 248.7306563947940958, 9.865755277559742353 ) ) ;
#71289=CARTESIAN_POINT ( 'NONE',  ( 153.3780955418828285, 270.1760744682334803, 14.08076314294041964 ) ) ;
#71290=CARTESIAN_POINT ( 'NONE',  ( 154.5359630391655514, 276.9837356694303594, -8.741008087266880722 ) ) ;
#71291=CARTESIAN_POINT ( 'NONE',  ( 199.9376085384402586, 267.5739236585927188, 6.187416678158419003 ) ) ;
#71292=EDGE_LOOP ( 'NONE', ( #60841, #60893, #89619, #58473 ) ) ;
#71294=CARTESIAN_POINT ( 'NONE',  ( 164.0405138800869054, 280.4465961471673836, -11.50895991882478242 ) ) ;
#71295=CARTESIAN_POINT ( 'NONE',  ( 193.7609008727193043, 262.8443104439116951, 4.759103018491034121 ) ) ;
#71297=CARTESIAN_POINT ( 'NONE',  ( 32.84087927488953085, 179.7677522451417929, -5.000000000000041744 ) ) ;
#71298=CARTESIAN_POINT ( 'NONE',  ( 165.7068383116082657, 276.7076515144831887, 15.46715011107357718 ) ) ;
#71299=CARTESIAN_POINT ( 'NONE',  ( 190.0534303668326288, 269.9073674132432643, 15.26070177760127322 ) ) ;
#71303=DIRECTION ( 'NONE',  ( -0.8660254037844387076, -0.4999999999999998890, -0.000000000000000000 ) ) ;
#71304=CARTESIAN_POINT ( 'NONE',  ( 1.528821818964843482, 165.5643266524160140, 9.188101187500095079 ) ) ;
#71305=CARTESIAN_POINT ( 'NONE',  ( 88.50972766791686297, 234.1589784336661637, -6.496448406907675876E-16 ) ) ;
#71306=CARTESIAN_POINT ( 'NONE',  ( 155.6281496932864457, 261.0911329737299980, -18.07904265579665548 ) ) ;
#71313=DIRECTION ( 'NONE',  ( 0.4999999999999992784, -0.8660254037844390407, 0.000000000000000000 ) ) ;
#71315=CARTESIAN_POINT ( 'NONE',  ( 178.6117656011147972, 290.0031260663362787, 9.480844723140000596 ) ) ;
#71316=CARTESIAN_POINT ( 'NONE',  ( 195.3341046825671583, 268.5239226548773104, 12.14968905865328175 ) ) ;
#71317=CARTESIAN_POINT ( 'NONE',  ( 205.5585585089849303, 274.6091280622553086, -13.37199793655179825 ) ) ;
#71319=DIRECTION ( 'NONE',  ( 0.4999999999999998890, -0.8660254037844385966, 0.000000000000000000 ) ) ;
#71321=CARTESIAN_POINT ( 'NONE',  ( 161.3773209892555371, 251.1332761876949746, -14.50043705923759241 ) ) ;
#71322=CARTESIAN_POINT ( 'NONE',  ( 37.63108229134613225, 192.5333772461660544, 9.188101187500095079 ) ) ;
#71324=EDGE_CURVE ( 'NONE', #83705, #99407, #808, .T. ) ;
#71325=CARTESIAN_POINT ( 'NONE',  ( 73.21957404993666785, 203.8923013555409796, 4.594050593750050204 ) ) ;
#71326=CARTESIAN_POINT ( 'NONE',  ( 57.68498304950345812, 214.1115022471903444, -5.000000000000047962 ) ) ;
#71330=CARTESIAN_POINT ( 'NONE',  ( 176.6243488689623007, 270.1410765278557164, -16.80516242629813561 ) ) ;
#71333=CARTESIAN_POINT ( 'NONE',  ( 196.4170778717353585, 290.4426369823788718, -17.78762421190030452 ) ) ;
#71334=VERTEX_POINT ( 'NONE', #87188 ) ;
#71336=CARTESIAN_POINT ( 'NONE',  ( 65.53359859134977228, 199.4548013555410080, -4.594050593750042211 ) ) ;
#71338=CARTESIAN_POINT ( 'NONE',  ( 154.9067123643522734, 262.3406990819208886, -18.18534662427576265 ) ) ;
#71339=CARTESIAN_POINT ( 'NONE',  ( 172.9649338451820029, 290.0245193479112800, -0.4253077601802810470 ) ) ;
#71341=CARTESIAN_POINT ( 'NONE',  ( 154.0022440109411832, 263.9072842238671228, 16.76240413822421971 ) ) ;
#71342=CARTESIAN_POINT ( 'NONE',  ( 189.9590362446921858, 286.5603738525368840, 16.42061212002715465 ) ) ;
#71343=CARTESIAN_POINT ( 'NONE',  ( 125.2349645446897171, 243.1115022471902591, 10.00000000000009592 ) ) ;
#71344=CARTESIAN_POINT ( 'NONE',  ( 200.9110265982630779, 282.6588894614233141, 17.52479721249226685 ) ) ;
#71345=CARTESIAN_POINT ( 'NONE',  ( 207.5686001603237116, 271.1276337968068333, 7.659944433763431704 ) ) ;
#71347=CARTESIAN_POINT ( 'NONE',  ( 149.2522690271913746, 273.6402648190738205, -10.03091955270726032 ) ) ;
#71349=VERTEX_POINT ( 'NONE', #89656 ) ;
#71350=CARTESIAN_POINT ( 'NONE',  ( 206.8317058779879574, 272.4039721336197317, -10.41591514895975834 ) ) ;
#71351=CARTESIAN_POINT ( 'NONE',  ( 207.3988330342936877, 270.8564699888902396, -1.301389719878858875 ) ) ;
#71353=VERTEX_POINT ( 'NONE', #82051 ) ;
#71354=CARTESIAN_POINT ( 'NONE',  ( 176.8434924416465321, 253.2981294648533606, -0.2582399125330065992 ) ) ;
#71357=CARTESIAN_POINT ( 'NONE',  ( 147.8819534105757043, 274.5079385007862811, -9.338341377131436971 ) ) ;
#71358=CARTESIAN_POINT ( 'NONE',  ( 148.8636819117637629, 274.0699646975406836, 8.926834414297511344 ) ) ;
#71363=CARTESIAN_POINT ( 'NONE',  ( -27.42236680055714260, 166.5217562850347406, 1.224646799147364892E-15 ) ) ;
#71368=CARTESIAN_POINT ( 'NONE',  ( 175.0809028706871118, 261.2525943152746208, 15.25527675994286092 ) ) ;
#71369=ORIENTED_EDGE ( 'NONE', *, *, #49202, .T. ) ;
#71371=ORIENTED_EDGE ( 'NONE', *, *, #54076, .F. ) ;
#71372=CARTESIAN_POINT ( 'NONE',  ( 183.6038495250667211, 296.0503002337411544, 1.014586387891125652 ) ) ;
#71374=CARTESIAN_POINT ( 'NONE',  ( 148.3629184514745987, 273.6748826132846375, -8.219814532462343948 ) ) ;
#71375=CARTESIAN_POINT ( 'NONE',  ( 208.3764315856425640, 269.7284287242038658, -1.833640725398759441 ) ) ;
#71376=CARTESIAN_POINT ( 'NONE',  ( 193.8603219414924013, 294.8710681561126989, 15.36476279452078586 ) ) ;
#71378=CARTESIAN_POINT ( 'NONE',  ( 157.4805323096970255, 257.8827121670497036, -16.70238855805511591 ) ) ;
#71379=CARTESIAN_POINT ( 'NONE',  ( 164.7279764954933512, 245.3297706122307034, 5.346914787972785632 ) ) ;
#71383=CARTESIAN_POINT ( 'NONE',  ( 81.47361835793333285, 217.8458772461660544, 9.188101187500095079 ) ) ;
#71385=CARTESIAN_POINT ( 'NONE',  ( 150.6453220160077251, 269.7216436761371483, 14.94145576020818034 ) ) ;
#71389=CARTESIAN_POINT ( 'NONE',  ( 157.4450252842904092, 257.9442121390794682, -17.98854725065957183 ) ) ;
#71394=CARTESIAN_POINT ( 'NONE',  ( 164.1883108770558692, 249.9675975386064692, 10.18338785008276481 ) ) ;
#71396=CARTESIAN_POINT ( 'NONE',  ( 207.7679535393632477, 270.7823436156499497, 1.643001479255987274 ) ) ;
#71397=CARTESIAN_POINT ( 'NONE',  ( 73.73334276372743545, 219.5024278399160664, 9.188101187500095079 ) ) ;
#71398=ORIENTED_EDGE ( 'NONE', *, *, #89685, .T. ) ;
#71401=CARTESIAN_POINT ( 'NONE',  ( 161.7973860292566712, 250.4057021959295071, -14.21001024987457484 ) ) ;
#71405=CARTESIAN_POINT ( 'NONE',  ( 109.9838485029171267, 222.7592609112380160, 2.679491924311254714 ) ) ;
#71408=CARTESIAN_POINT ( 'NONE',  ( 188.7267243920021542, 295.1910411013678299, 11.79826141631466463 ) ) ;
#71409=CARTESIAN_POINT ( 'NONE',  ( 159.3969902868548161, 275.0432323227933580, 12.88213412656160095 ) ) ;
#71410=CARTESIAN_POINT ( 'NONE',  ( 159.3237119419271437, 254.6902313965507858, -15.56765445935501191 ) ) ;
#71411=CARTESIAN_POINT ( 'NONE',  ( 148.1846401255833996, 275.9836697316168284, -5.368268268079755323 ) ) ;
#71412=CARTESIAN_POINT ( 'NONE',  ( 180.6665526851674599, 287.6815954905284798, 14.11204521094005671 ) ) ;
#71416=CARTESIAN_POINT ( 'NONE',  ( 203.1577047574547805, 277.9875982410399047, -14.81633164762421195 ) ) ;
#71417=CARTESIAN_POINT ( 'NONE',  ( 200.8551880497955437, 282.7556046643899776, 18.00894873733387058 ) ) ;
#71419=CARTESIAN_POINT ( 'NONE',  ( 171.6080846817307872, 251.3649527223411724, 7.288243930487503519 ) ) ;
#71421=CARTESIAN_POINT ( 'NONE',  ( 175.0524379492280502, 290.1408238227680272, -6.332636328160596406 ) ) ;
#71422=CARTESIAN_POINT ( 'NONE',  ( 153.3702792842350107, 270.2708052652295123, 14.01565955641743422 ) ) ;
#71423=ORIENTED_EDGE ( 'NONE', *, *, #86359, .T. ) ;
#71424=EDGE_CURVE ( 'NONE', #31631, #82532, #86344, .T. ) ;
#71425=CARTESIAN_POINT ( 'NONE',  ( 164.4858674010174298, 245.7491158648375347, -2.958464974013825355 ) ) ;
#71426=CARTESIAN_POINT ( 'NONE',  ( 177.5003341694142307, 264.7901247500786894, -15.18634591033956305 ) ) ;
#71428=CARTESIAN_POINT ( 'NONE',  ( 176.1768359416886369, 285.1771366315132923, -12.84902834441190755 ) ) ;
#71429=ADVANCED_FACE ( 'NONE', ( #53583 ), #84537, .T. ) ;
#71432=CARTESIAN_POINT ( 'NONE',  ( 168.7693793741400725, 272.9564462316830600, 15.95584976162842494 ) ) ;
#71433=CARTESIAN_POINT ( 'NONE',  ( 180.5253698147535317, 273.0125201196690909, 17.27947222482116985 ) ) ;
#71435=CARTESIAN_POINT ( 'NONE',  ( 192.2066520969698615, 261.9360867464749276, 3.041693569932921726 ) ) ;
#71436=VECTOR ( 'NONE', #35847, 1000.000000000000000 ) ;
#71437=CARTESIAN_POINT ( 'NONE',  ( 195.4436462626574667, 265.1414692012189676, -7.795071168451356058 ) ) ;
#71438=CARTESIAN_POINT ( 'NONE',  ( 6.724974241671477060, 168.5643266524160424, 9.188101187500095079 ) ) ;
#71442=CARTESIAN_POINT ( 'NONE',  ( 175.0454162132552085, 255.3288691254335561, 8.248559459473627342 ) ) ;
#71444=CARTESIAN_POINT ( 'NONE',  ( 192.8292865579535658, 291.0864435001786887, 16.05090170841207353 ) ) ;
#71446=CARTESIAN_POINT ( 'NONE',  ( 14.70821206310299978, 188.4869531367911293, 4.594050593750046652 ) ) ;
#71449=CARTESIAN_POINT ( 'NONE',  ( 181.7837364184500188, 294.2830797998335584, 6.350600127774545633 ) ) ;
#71450=CARTESIAN_POINT ( 'NONE',  ( 173.6102056894289660, 272.6920272357795056, -16.35699099929867018 ) ) ;
#71451=CARTESIAN_POINT ( 'NONE',  ( 197.0456392842824016, 289.3539366801700794, 16.77178551838651188 ) ) ;
#71453=CARTESIAN_POINT ( 'NONE',  ( 171.6209549223533770, 276.3359157968284876, 16.92957725593318941 ) ) ;
#71454=CARTESIAN_POINT ( 'NONE',  ( 186.8199858043552410, 295.8404895034861397, -7.792751730412551758 ) ) ;
#71455=EDGE_CURVE ( 'NONE', #29993, #15150, #47992, .T. ) ;
#71456=CARTESIAN_POINT ( 'NONE',  ( 87.56285948006663489, 221.3615022471902591, -10.00000000000009592 ) ) ;
#71458=CARTESIAN_POINT ( 'NONE',  ( 192.8922210760480311, 295.5150220211069723, -12.92664670631823753 ) ) ;
#71459=CARTESIAN_POINT ( 'NONE',  ( 70.67536410627012344, 201.6115022471901739, -5.000000000000041744 ) ) ;
#71462=CARTESIAN_POINT ( 'NONE',  ( 203.3512397331466275, 270.1136130142050433, 6.392281993283416952 ) ) ;
#71463=CARTESIAN_POINT ( 'NONE',  ( 53.65289935712325331, 189.5327760586659451, 1.948934522072303157E-15 ) ) ;
#71464=CARTESIAN_POINT ( 'NONE',  ( 159.5284711081640125, 254.3355781173132755, 15.34104435652608522 ) ) ;
#71466=CARTESIAN_POINT ( 'NONE',  ( 190.8545714895799392, 300.0771806536980648, -5.516553996882049837 ) ) ;
#71468=ORIENTED_EDGE ( 'NONE', *, *, #87942, .T. ) ;
#71470=CARTESIAN_POINT ( 'NONE',  ( 167.7092726043314315, 282.4287604056521559, -12.24019139390664535 ) ) ;
#71471=CARTESIAN_POINT ( 'NONE',  ( 193.2853656402591014, 295.8669216819805001, 14.14801835725165091 ) ) ;
#71472=CARTESIAN_POINT ( 'NONE',  ( 206.1617103877918851, 269.9578652681285575, -1.313740177516645069 ) ) ;
#71474=CARTESIAN_POINT ( 'NONE',  ( 162.6774150396764469, 248.8814472377480911, 10.88033986792731689 ) ) ;
#71475=CARTESIAN_POINT ( 'NONE',  ( 196.9976074755333286, 289.4371302133026802, -16.79549473444794216 ) ) ;
#71476=CARTESIAN_POINT ( 'NONE',  ( 185.5618649715216861, 267.5775901627870894, -14.75789268656261122 ) ) ;
#71483=ORIENTED_EDGE ( 'NONE', *, *, #32427, .T. ) ;
#71487=CARTESIAN_POINT ( 'NONE',  ( 149.0323968763055689, 272.5153119669064949, 11.64231532207353403 ) ) ;
#71491=CARTESIAN_POINT ( 'NONE',  ( 189.7007398628852286, 274.3294530569783660, -15.69864028862395067 ) ) ;
#71492=CARTESIAN_POINT ( 'NONE',  ( 161.0515428782683500, 277.3244187559503189, -13.42420650014866368 ) ) ;
#71494=CARTESIAN_POINT ( 'NONE',  ( 201.0356089830534643, 282.4431064412383989, -18.18835788025466371 ) ) ;
#71498=CARTESIAN_POINT ( 'NONE',  ( 157.8811243250769110, 257.1888664433053009, -17.39256699147873064 ) ) ;
#71500=CARTESIAN_POINT ( 'NONE',  ( 104.0442318961827652, 237.0024278399160949, -9.188101187500093303 ) ) ;
#71501=ADVANCED_FACE ( 'NONE', ( #32787 ), #18609, .T. ) ;
#71502=CARTESIAN_POINT ( 'NONE',  ( 148.9285945872975390, 272.6951028054104427, -12.01265727652413240 ) ) ;
#71503=CARTESIAN_POINT ( 'NONE',  ( 180.9558116816610323, 287.1304582847630513, -13.41095839139118695 ) ) ;
#71504=ORIENTED_EDGE ( 'NONE', *, *, #73449, .F. ) ;
#71511=CARTESIAN_POINT ( 'NONE',  ( 55.05949644674294774, 214.8464784336662206, 1.353441290958777525E-15 ) ) ;
#71513=( BOUNDED_CURVE ( )  B_SPLINE_CURVE ( 1, ( #30985, #22883 ),
 .UNSPECIFIED., .F., .T. ) 
 B_SPLINE_CURVE_WITH_KNOTS ( ( 2, 2 ),
 ( 0.000000000000000000, 0.0009374999959032095671 ),
 .UNSPECIFIED. ) 
 CURVE ( )  GEOMETRIC_REPRESENTATION_ITEM ( )  RATIONAL_B_SPLINE_CURVE ( ( 0.9368410486966849415, 0.9368410486966849415 ) ) 
 REPRESENTATION_ITEM ( '' )  );
#71514=CARTESIAN_POINT ( 'NONE',  ( 151.3883635558152321, 268.4346579770563608, 15.44343517165679103 ) ) ;
#71515=CARTESIAN_POINT ( 'NONE',  ( 198.2555168952299027, 287.2583671870688704, 16.98288975666356748 ) ) ;
#71516=CARTESIAN_POINT ( 'NONE',  ( 172.8453781230440995, 271.4476526176509878, 16.48331706524980333 ) ) ;
#71521=CARTESIAN_POINT ( 'NONE',  ( 189.9925954911225290, 301.5701668779311717, 0.1154287172046158938 ) ) ;
#71523=CARTESIAN_POINT ( 'NONE',  ( 171.9840958472507566, 258.8842185260619431, -13.78362884886991679 ) ) ;
#71525=CARTESIAN_POINT ( 'NONE',  ( 207.8570869662935365, 270.6279599915536664, -5.669188455878507504 ) ) ;
#71527=CARTESIAN_POINT ( 'NONE',  ( 190.5477107455830321, 300.6086790531491033, 3.126266616601216963 ) ) ;
#71528=CARTESIAN_POINT ( 'NONE',  ( 177.7425752430770274, 269.7382505134228268, 16.10177396393870808 ) ) ;
#71529=CARTESIAN_POINT ( 'NONE',  ( 188.0757938802393312, 263.1534643581272803, 10.95204294997910033 ) ) ;
#71531=CARTESIAN_POINT ( 'NONE',  ( 153.9606011487479122, 264.3624140031040497, -16.52591424867165770 ) ) ;
#71532=CARTESIAN_POINT ( 'NONE',  ( 174.9193129510662459, 283.1525502601675726, 14.86735122827573718 ) ) ;
#71533=CARTESIAN_POINT ( 'NONE',  ( 119.3082767336485404, 233.5643266524159856, -9.188101187500093303 ) ) ;
#71535=CARTESIAN_POINT ( 'NONE',  ( 191.8456210280128005, 298.3606325003146367, -9.135603544929113085 ) ) ;
#71537=CARTESIAN_POINT ( 'NONE',  ( 155.6569868912636991, 261.0411854816857158, -17.75433477650897984 ) ) ;
#71538=CARTESIAN_POINT ( 'NONE',  ( 192.0117586784035097, 296.2629708079742841, 12.42531335008228588 ) ) ;
#71542=CARTESIAN_POINT ( 'NONE',  ( 155.6368094659423207, 263.0761338075079721, 17.69820953191020152 ) ) ;
#71543=CARTESIAN_POINT ( 'NONE',  ( 158.3005605714957937, 275.4539231493820353, -12.33454573515837893 ) ) ;
#71544=CARTESIAN_POINT ( 'NONE',  ( 185.6517645066024613, 262.0489465526635513, 9.793930467762132608 ) ) ;
#71545=CARTESIAN_POINT ( 'NONE',  ( 205.7627300303947209, 272.2554926137148072, 9.584172220806708609 ) ) ;
#71546=CARTESIAN_POINT ( 'NONE',  ( 130.5662598870812019, 252.3149278399160949, 9.188101187500093303 ) ) ;
#71547=CARTESIAN_POINT ( 'NONE',  ( 198.7357616895271804, 286.4265588032756114, -17.04018524297827497 ) ) ;
#71548=CARTESIAN_POINT ( 'NONE',  ( 185.8605417954027530, 296.7763049164376525, 4.522302630076449503 ) ) ;
#71550=CARTESIAN_POINT ( 'NONE',  ( 67.69866210081085001, 200.7048013555409796, 4.594050593750051981 ) ) ;
#71553=CARTESIAN_POINT ( 'NONE',  ( 157.4805323096970255, 257.8827121670497036, -16.70238855805511591 ) ) ;
#71557=CARTESIAN_POINT ( 'NONE',  ( 173.8165395728766498, 261.8204000554670188, 14.38043926846092724 ) ) ;
#71558=CARTESIAN_POINT ( 'NONE',  ( 152.7550266220043511, 278.4983035287039570, -1.611717572787890296 ) ) ;
#71559=CARTESIAN_POINT ( 'NONE',  ( 180.5721669215874101, 292.9178206186057878, -6.192220326497509753 ) ) ;
#71560=CARTESIAN_POINT ( 'NONE',  ( 155.5587153255869453, 261.2113968263770971, -18.30500480654006878 ) ) ;
#71561=CARTESIAN_POINT ( 'NONE',  ( 157.3673062317275537, 270.8922321708535037, -14.72387779267422658 ) ) ;
#71562=CARTESIAN_POINT ( 'NONE',  ( 128.5366863930700276, 235.0177522451417929, 5.000000000000051514 ) ) ;
#71566=CARTESIAN_POINT ( 'NONE',  ( 190.3691966041315311, 300.9178746160123410, 0.1783449565851275009 ) ) ;
#71567=CARTESIAN_POINT ( 'NONE',  ( -13.35616335646270691, 163.0958772461660544, -9.188101187500095079 ) ) ;
#71568=CARTESIAN_POINT ( 'NONE',  ( 47.67182463829572470, 189.1423013555410080, -4.594050593750043987 ) ) ;
#71574=CARTESIAN_POINT ( 'NONE',  ( 198.2717785813136402, 277.4294249212936734, -15.37832795003007114 ) ) ;
#71575=CARTESIAN_POINT ( 'NONE',  ( 60.04851071045064970, 192.1427522451417644, 1.119607411625061291E-15 ) ) ;
#71576=LINE ( 'NONE', #18370, #61149 ) ;
#71577=CARTESIAN_POINT ( 'NONE',  ( 183.0365768892434346, 257.4193572625480897, 1.324102024236442965 ) ) ;
#71579=CARTESIAN_POINT ( 'NONE',  ( 164.3036517873781008, 252.3706336020835579, 13.60069832213670082 ) ) ;
#71583=CARTESIAN_POINT ( 'NONE',  ( 161.4744130670923994, 267.8122197200463006, 16.81033864343086748 ) ) ;
#71584=CARTESIAN_POINT ( 'NONE',  ( 31.70422093597033353, 189.1115022471902591, 10.00000000000009592 ) ) ;
#71586=CARTESIAN_POINT ( 'NONE',  ( 202.3421728196210552, 280.1800714929709670, 16.85915999540957344 ) ) ;
#71587=CARTESIAN_POINT ( 'NONE',  ( -14.30363896367569509, 171.7369531367911293, -4.594050593750048428 ) ) ;
#71590=CARTESIAN_POINT ( 'NONE',  ( 183.1557134058521683, 266.6876041466057927, -15.64491608568827452 ) ) ;
#71593=CARTESIAN_POINT ( 'NONE',  ( 205.9240884482826175, 273.9760116357041966, 10.27504561427317142 ) ) ;
#71594=CARTESIAN_POINT ( 'NONE',  ( 187.0851743399334168, 258.9150848785300809, -2.444460235746602095 ) ) ;
#71596=ORIENTED_EDGE ( 'NONE', *, *, #13366, .F. ) ;
#71597=CARTESIAN_POINT ( 'NONE',  ( 189.8267730604733003, 261.5921186768457574, 7.234476395667181592 ) ) ;
#71600=CARTESIAN_POINT ( 'NONE',  ( 153.2953402526850937, 277.6774005532211049, -5.292706812873809064 ) ) ;
#71602=CARTESIAN_POINT ( 'NONE',  ( 207.2815143871675048, 271.6248809420436032, 8.741063757625067154 ) ) ;
#71603=CARTESIAN_POINT ( 'NONE',  ( 152.8593402092683959, 275.2840601128194749, 10.96293945604634068 ) ) ;
#71604=CARTESIAN_POINT ( 'NONE',  ( 159.3586121662929713, 254.6297824347537642, -15.50090345830412630 ) ) ;
#71608=CARTESIAN_POINT ( 'NONE',  ( 207.0548180518391916, 272.0175305127218053, 7.721676452263806389 ) ) ;
#71609=B_SPLINE_CURVE_WITH_KNOTS ( 'NONE', 3,
 ( #63700, #79446, #50000, #33296 ),
 .UNSPECIFIED., .F., .F.,
 ( 4, 4 ),
 ( 0.008552533699946726631, 0.01491633745239599393 ),
 .UNSPECIFIED. ) ;
#71614=ORIENTED_EDGE ( 'NONE', *, *, #31399, .F. ) ;
#71615=ADVANCED_FACE ( 'NONE', ( #66194 ), #62824, .F. ) ;
#71616=CARTESIAN_POINT ( 'NONE',  ( 157.7825643558039417, 277.5034979810923232, -9.893793770821909916 ) ) ;
#71620=CARTESIAN_POINT ( 'NONE',  ( 189.0276854369573698, 297.1328171424457310, 8.003537747434423366 ) ) ;
#71621=ORIENTED_EDGE ( 'NONE', *, *, #13600, .T. ) ;
#71627=ORIENTED_EDGE ( 'NONE', *, *, #34322, .F. ) ;
#71628=CARTESIAN_POINT ( 'NONE',  ( 200.3765029811139584, 283.5847115241710981, 16.85207472104531590 ) ) ;
#71629=CARTESIAN_POINT ( 'NONE',  ( 158.4485968073939546, 275.2084588272041401, -13.86993402366507944 ) ) ;
#71630=CARTESIAN_POINT ( 'NONE',  ( 204.7986527064648214, 275.9253235211867263, 14.74587861556245905 ) ) ;
#71631=CARTESIAN_POINT ( 'NONE',  ( 151.4212479147002171, 275.0370223182968061, -8.550850240198341723 ) ) ;
#71636=AXIS2_PLACEMENT_3D ( 'NONE', #18400, #96932, #4174 ) ;
#71641=CARTESIAN_POINT ( 'NONE',  ( 161.0794736472514614, 271.0204982161961880, 16.04590376577446165 ) ) ;
#71644=CARTESIAN_POINT ( 'NONE',  ( 168.4682619938861023, 272.6906211788349310, 15.98134908431772594 ) ) ;
#71647=CARTESIAN_POINT ( 'NONE',  ( 193.7951232862128848, 294.4761830863158707, 13.69151923843489094 ) ) ;
#71649=CARTESIAN_POINT ( 'NONE',  ( 177.9714937548455680, 255.7189482022137383, 8.882064279750110813 ) ) ;
#71650=DIRECTION ( 'NONE',  ( -0.8660254037844359321, -0.5000000000000051070, -0.000000000000000000 ) ) ;
#71652=ORIENTED_EDGE ( 'NONE', *, *, #91677, .T. ) ;
#71654=B_SPLINE_CURVE_WITH_KNOTS ( 'NONE', 3,
 ( #91539, #52497, #6418, #37298 ),
 .UNSPECIFIED., .F., .F.,
 ( 4, 4 ),
 ( 0.007320200878984583701, 0.01237002053563545159 ),
 .UNSPECIFIED. ) ;
#71656=CARTESIAN_POINT ( 'NONE',  ( 205.7668501412109663, 274.2483563724483133, 11.09689540819876896 ) ) ;
#71657=CARTESIAN_POINT ( 'NONE',  ( 191.2053780694017462, 298.1875778970886586, -9.406300816995585734 ) ) ;
#71658=CARTESIAN_POINT ( 'NONE',  ( 159.2511875226268216, 254.8158473755685520, 15.75855490706745599 ) ) ;
#71659=ORIENTED_EDGE ( 'NONE', *, *, #27885, .F. ) ;
#71661=DIRECTION ( 'NONE',  ( 0.4999999999999998890, -0.8660254037844385966, 0.000000000000000000 ) ) ;
#71662=B_SPLINE_CURVE_WITH_KNOTS ( 'NONE', 3,
 ( #84881, #8838, #93481, #70637 ),
 .UNSPECIFIED., .F., .F.,
 ( 4, 4 ),
 ( 0.03188865644562008383, 0.04088460837272645670 ),
 .UNSPECIFIED. ) ;
#71663=CARTESIAN_POINT ( 'NONE',  ( 168.5771703487694992, 257.4052341225797704, -14.27990518792410768 ) ) ;
#71664=CARTESIAN_POINT ( 'NONE',  ( 159.2289198208967775, 254.8544161663325838, -15.88961297684315888 ) ) ;
#71666=CARTESIAN_POINT ( 'NONE',  ( 161.8811854682448939, 250.2605573099562264, 13.51112293479948789 ) ) ;
#71671=CARTESIAN_POINT ( 'NONE',  ( 207.1122325394003951, 271.9180857031755636, 7.794245785756032774 ) ) ;
#71673=CARTESIAN_POINT ( 'NONE',  ( 14.65434579541623172, 189.2677522451419065, -5.000000000000047962 ) ) ;
#71674=CARTESIAN_POINT ( 'NONE',  ( 85.53293889029039576, 226.3149278399160949, -9.188101187500095079 ) ) ;
#71675=CARTESIAN_POINT ( 'NONE',  ( 196.2547452604713385, 269.4049120393308385, -11.95081354204263668 ) ) ;
#71676=CYLINDRICAL_SURFACE ( 'NONE', #53411, 10.00000000000010658 ) ;
#71677=CARTESIAN_POINT ( 'NONE',  ( 167.2251136787149335, 278.4273091872281043, -13.36331558781519568 ) ) ;
#71678=CARTESIAN_POINT ( 'NONE',  ( 7.942909239684589728, 166.2048013555410080, 4.594050593750051981 ) ) ;
#71680=CARTESIAN_POINT ( 'NONE',  ( 200.8769374536528858, 282.7179335918746688, 17.26928237494566787 ) ) ;
#71681=VERTEX_POINT ( 'NONE', #77275 ) ;
#71683=CARTESIAN_POINT ( 'NONE',  ( 197.9182972497701769, 265.0047853328303518, -3.008455722180424452 ) ) ;
#71686=CARTESIAN_POINT ( 'NONE',  ( 161.6127771116929921, 250.7254542206800352, -12.96229604595372464 ) ) ;
#71687=CARTESIAN_POINT ( 'NONE',  ( 181.8542211641277788, 285.1504725237182356, 15.60384829402828011 ) ) ;
#71689=CARTESIAN_POINT ( 'NONE',  ( 28.02335264628875677, 196.1744531367911293, 4.594050593750047540 ) ) ;
#71690=CARTESIAN_POINT ( 'NONE',  ( 83.43119661263050091, 205.6427522451417644, 1.119607411625061291E-15 ) ) ;
#71691=CARTESIAN_POINT ( 'NONE',  ( 195.9913908494966392, 275.3482408794030221, 15.54441459790748148 ) ) ;
#71692=ORIENTED_EDGE ( 'NONE', *, *, #4708, .F. ) ;
#71695=B_SPLINE_CURVE_WITH_KNOTS ( 'NONE', 3,
 ( #74394, #97687, #83495, #52059, #74880, #29266, #100172, #14565, #6464, #21179 ),
 .UNSPECIFIED., .F., .F.,
 ( 4, 3, 3, 4 ),
 ( 0.001342218634783023945, 0.001498044977018986789, 0.004494154408217571929, 0.006632416054833400326 ),
 .UNSPECIFIED. ) ;
#71696=B_SPLINE_CURVE_WITH_KNOTS ( 'NONE', 3,
 ( #33395, #35383, #19223, #57679, #11613, #96235, #10102, #88158, #65294, #18706, #40965, #18208, #27301, #42472, #72927, #49100, #71911, #80035, #81530, #12099, #27796, #72425, #80541, #73903, #10604, #2512, #41476, #42961, #11120, #4490, #95246, #25815, #41990, #97227, #3517, #34394, #22184, #5004, #6978, #91124, #29298, #59155, #91611, #82544, #83524, #30278, #67279, #51073 ),
 .UNSPECIFIED., .F., .F.,
 ( 4, 2, 2, 2, 2, 2, 2, 2, 2, 2, 2, 2, 2, 2, 2, 2, 2, 2, 2, 2, 2, 2, 2, 4 ),
 ( 0.001443219783669777217, 0.001907740669036624061, 0.002372261554403471123, 0.002604521997086893786, 0.002720652218428617260, 0.002836782439770340735, 0.002952912661112064643, 0.003069042882453788118, 0.003301303325137235067, 0.003765824210504130701, 0.004230345095871026334, 0.005159386866604723058, 0.006088428637338420650, 0.006552949522705311079, 0.007017470408072201508, 0.007133600629413924116, 0.007191665740084785853, 0.007249730850755647590, 0.007365861072097308615, 0.007481991293438970507, 0.007946512178805745577, 0.008411033064172518045, 0.008643293506855859176, 0.008875553949539200307 ),
 .UNSPECIFIED. ) ;
#71697=CARTESIAN_POINT ( 'NONE',  ( 198.2505066714982149, 285.2670451491296149, 0.000000000000000000 ) ) ;
#71699=CARTESIAN_POINT ( 'NONE',  ( -4.289699588770600869, 159.1423013555410080, -4.594050593750043987 ) ) ;
#71702=CARTESIAN_POINT ( 'NONE',  ( -22.42236680055709641, 157.8615022471902591, 0.000000000000000000 ) ) ;
#71703=CARTESIAN_POINT ( 'NONE',  ( 194.7900911235093133, 293.2606606935473792, -14.66228443412922999 ) ) ;
#71704=CIRCLE ( 'NONE', #5378, 17.82106496071138224 ) ;
#71706=CARTESIAN_POINT ( 'NONE',  ( 164.0777181605478745, 246.4560510864015441, 5.763760713451748785 ) ) ;
#71708=CARTESIAN_POINT ( 'NONE',  ( 191.8456210280128005, 298.3606325003146367, -9.135603544929113085 ) ) ;
#71709=CARTESIAN_POINT ( 'NONE',  ( 148.2980785574368952, 273.7871886041155562, 9.134436720559454770 ) ) ;
#71713=CARTESIAN_POINT ( 'NONE',  ( 113.2460989071574460, 230.0643266524160140, 9.188101187500095079 ) ) ;
#71716=CARTESIAN_POINT ( 'NONE',  ( 151.0249774166511827, 270.1664039458447064, 13.81320228137823491 ) ) ;
#71718=CARTESIAN_POINT ( 'NONE',  ( 157.1606030646430554, 258.4368458743103361, 17.96998724893680688 ) ) ;
#71719=CARTESIAN_POINT ( 'NONE',  ( 162.2336410148055279, 251.8862672885301492, -14.09881826716025799 ) ) ;
#71720=CARTESIAN_POINT ( 'NONE',  ( 191.0684812360443914, 299.7066781045875246, -8.010743411620572019 ) ) ;
#71721=CARTESIAN_POINT ( 'NONE',  ( 192.8225454482096666, 263.7804965554488490, -4.355381635346724067 ) ) ;
#71722=CARTESIAN_POINT ( 'NONE',  ( 197.0226655822963551, 289.3937282992477549, -17.28982543158101493 ) ) ;
#71723=CARTESIAN_POINT ( 'NONE',  ( 175.1758473867431292, 292.4163926228642936, -1.150070930579374151 ) ) ;
#71727=CARTESIAN_POINT ( 'NONE',  ( 175.5888903117697453, 278.5951473192365597, 15.44173524372987139 ) ) ;
#71728=CARTESIAN_POINT ( 'NONE',  ( 165.3957260903385134, 269.6996331764513002, -16.29327252992070996 ) ) ;
#71729=CARTESIAN_POINT ( 'NONE',  ( 200.1133476818314705, 272.1141633677412415, 12.87458617912082914 ) ) ;
#71732=CARTESIAN_POINT ( 'NONE',  ( 148.2247184032906375, 275.5581615573433396, 5.963085520373529569 ) ) ;
#71734=EDGE_CURVE ( 'NONE', #47543, #66560, #11783, .T. ) ;
#71735=CARTESIAN_POINT ( 'NONE',  ( 198.9721957120447655, 281.0613474150461570, 17.36564602955951386 ) ) ;
#71737=CARTESIAN_POINT ( 'NONE',  ( 174.0223458074996472, 272.1910991151906956, -17.55968156639984556 ) ) ;
#71740=CARTESIAN_POINT ( 'NONE',  ( 148.1829914015846157, 273.9865254053503349, -9.304102644963160529 ) ) ;
#71741=CARTESIAN_POINT ( 'NONE',  ( 21.76528272068881265, 171.8262482093457777, 3.021315404115420679E-15 ) ) ;
#71748=CARTESIAN_POINT ( 'NONE',  ( 154.9048824156581361, 262.3438686460345366, -17.40627786727128168 ) ) ;
#71751=CARTESIAN_POINT ( 'NONE',  ( 100.3908607700757187, 228.7677522451418497, 10.00000000000009592 ) ) ;
#71758=CARTESIAN_POINT ( 'NONE',  ( 185.6868470588481159, 282.1044346093191848, -16.51667675334077501 ) ) ;
#71760=CARTESIAN_POINT ( 'NONE',  ( 147.3161703957304667, 275.4879034285576722, -5.959278055987775602 ) ) ;
#71761=CARTESIAN_POINT ( 'NONE',  ( 196.9911704225566211, 284.9555270314510267, -17.17161694444654785 ) ) ;
#71763=CARTESIAN_POINT ( 'NONE',  ( 152.9607371460978129, 265.7112270302071124, -16.17698032818104537 ) ) ;
#71765=CARTESIAN_POINT ( 'NONE',  ( 201.3053657339852691, 274.7141922394133076, -14.27644254562359372 ) ) ;
#71766=CARTESIAN_POINT ( 'NONE',  ( 122.2847184155099995, 253.6589784336661069, -6.496448406907675876E-16 ) ) ;
#71769=ADVANCED_FACE ( 'NONE', ( #93513 ), #24070, .T. ) ;
#71770=VERTEX_POINT ( 'NONE', #40753 ) ;
#71774=CARTESIAN_POINT ( 'NONE',  ( 56.67693180720107193, 191.9824982072973967, 3.021315404115420679E-15 ) ) ;
#71775=CARTESIAN_POINT ( 'NONE',  ( 173.7213227573953986, 290.5666012884805696, -4.949759831816241906 ) ) ;
#71777=CARTESIAN_POINT ( 'NONE',  ( 152.7122812589697958, 277.9324518551267147, 6.933031942251369983 ) ) ;
#71779=CARTESIAN_POINT ( 'NONE',  ( 173.6700662098836290, 287.8081707173866448, -9.948204391775917088 ) ) ;
#71780=CARTESIAN_POINT ( 'NONE',  ( 171.5564966965742997, 280.0145032911023577, 13.85370006234987450 ) ) ;
#71781=CARTESIAN_POINT ( 'NONE',  ( 176.9521628696608104, 255.8834708374732543, -7.282453275594096276 ) ) ;
#71782=VERTEX_POINT ( 'NONE', #32167 ) ;
#71783=CARTESIAN_POINT ( 'NONE',  ( 147.9500839974939197, 274.3899328626944225, -9.375093207164509224 ) ) ;
#71788=CARTESIAN_POINT ( 'NONE',  ( 205.0978449570898476, 268.9670457764514708, -3.035070700556400158 ) ) ;
#71789=CARTESIAN_POINT ( 'NONE',  ( 152.4585818852530963, 266.5809854552784941, -16.62427189540569117 ) ) ;
#71790=CARTESIAN_POINT ( 'NONE',  ( 149.7166446726674565, 271.3301600186404698, 12.26048591517335495 ) ) ;
#71791=CARTESIAN_POINT ( 'NONE',  ( 202.9972156839127990, 279.0455039708822937, 16.77197898838388213 ) ) ;
#71792=CARTESIAN_POINT ( 'NONE',  ( 163.1953264782998758, 283.8895661455310915, -7.125257539458086598 ) ) ;
#71793=CARTESIAN_POINT ( 'NONE',  ( 160.3733185927383715, 282.5102941377067509, 6.606729549618552078 ) ) ;
#71794=CARTESIAN_POINT ( 'NONE',  ( 200.9061540366740246, 282.6673289856585143, -18.13083321883407351 ) ) ;
#71796=CARTESIAN_POINT ( 'NONE',  ( 167.8261084473395499, 282.2036296651569387, -10.70662813516634060 ) ) ;
#71798=CARTESIAN_POINT ( 'NONE',  ( 9.963374858250592325, 169.8927522451418213, 10.00000000000009948 ) ) ;
#71799=CARTESIAN_POINT ( 'NONE',  ( 193.1669738419331850, 275.7633846255446315, -16.84869157407539575 ) ) ;
#71800=CARTESIAN_POINT ( 'NONE',  ( 74.07275743019523873, 225.1199935810941213, 2.679491924311251605 ) ) ;
#71803=CARTESIAN_POINT ( 'NONE',  ( 192.0523540417460993, 298.0025604169266558, 12.03387399082417275 ) ) ;
#71805=( BOUNDED_CURVE ( )  B_SPLINE_CURVE ( 2, ( #94619, #9997, #78400, #70787, #63180, #17585, #25177, #38872, #56057 ),
 .UNSPECIFIED., .F., .T. ) 
 B_SPLINE_CURVE_WITH_KNOTS ( ( 3, 2, 2, 2, 3 ),
 ( 0.02822580645161290591, 0.02956989247311828106, 0.03225806451612903136, 0.03494623655913978166, 0.03629032258064516375 ),
 .UNSPECIFIED. ) 
 CURVE ( )  GEOMETRIC_REPRESENTATION_ITEM ( )  RATIONAL_B_SPLINE_CURVE ( ( 0.9330127018922192983, 0.9330127018922194093, 1.000000000000000000, 0.8660254037844387076, 1.000000000000000000, 0.8660254037844387076, 1.000000000000000000, 0.9330127018922191873, 0.9330127018922194093 ) ) 
 REPRESENTATION_ITEM ( '' )  );
#71806=CARTESIAN_POINT ( 'NONE',  ( 194.3799873100184641, 293.9709813348915191, 15.33105633561973669 ) ) ;
#71808=CARTESIAN_POINT ( 'NONE',  ( -12.86919761471646773, 169.5024278399161233, -9.188101187500093303 ) ) ;
#71809=CARTESIAN_POINT ( 'NONE',  ( 93.67942421434402434, 215.7048013555409796, 4.594050593750051981 ) ) ;
#71810=CARTESIAN_POINT ( 'NONE',  ( 202.7676489560256528, 279.4431252073101746, -16.04062356091568020 ) ) ;
#71812=CARTESIAN_POINT ( 'NONE',  ( -17.42236680055705023, 149.2012482093457777, 0.000000000000000000 ) ) ;
#71813=CARTESIAN_POINT ( 'NONE',  ( -10.37017993122367976, 171.4865022471902876, 10.00000000000009415 ) ) ;
#71815=CARTESIAN_POINT ( 'NONE',  ( 160.6677038066905823, 282.0210727026695849, 5.138757052024616634 ) ) ;
#71816=CARTESIAN_POINT ( 'NONE',  ( 190.4455119341017451, 300.3931655422463791, -0.7229603976562811729 ) ) ;
#71817=CARTESIAN_POINT ( 'NONE',  ( 208.3682389855799499, 269.7426187237583690, -1.431169231381201890 ) ) ;
#71818=CARTESIAN_POINT ( 'NONE',  ( 178.5259719646841745, 290.8553054119842045, 10.01277831063413437 ) ) ;
#71819=EDGE_CURVE ( 'NONE', #46780, #81902, #86941, .T. ) ;
#71822=CARTESIAN_POINT ( 'NONE',  ( 207.2167723318516153, 271.7370174712370954, -6.606038862010207957 ) ) ;
#71825=CARTESIAN_POINT ( 'NONE',  ( 48.29419362332453858, 192.5643266524160140, 9.188101187500095079 ) ) ;
#71827=ADVANCED_FACE ( 'NONE', ( #79820 ), #16962, .T. ) ;
#71829=CARTESIAN_POINT ( 'NONE',  ( 72.54290492928882372, 206.5643266524159571, -9.188101187500093303 ) ) ;
#71830=CARTESIAN_POINT ( 'NONE',  ( 207.1572261440131797, 271.8401544939704877, -5.633070628900782140 ) ) ;
#71832=CARTESIAN_POINT ( 'NONE',  ( 164.6052063594347032, 258.5370629776766123, 15.54664782134921097 ) ) ;
#71835=CARTESIAN_POINT ( 'NONE',  ( 173.8329535930888881, 268.6061503712382432, -16.29996300370038043 ) ) ;
#71838=CARTESIAN_POINT ( 'NONE',  ( 196.7130436017243653, 289.9300093007386749, -16.33278734947153765 ) ) ;
#71841=CARTESIAN_POINT ( 'NONE',  ( 80.01237403692960015, 210.8768266524159856, -9.188101187500093303 ) ) ;
#71843=CARTESIAN_POINT ( 'NONE',  ( 173.1031462479762411, 289.7790225637821209, -0.7365366526630715560 ) ) ;
#71846=EDGE_LOOP ( 'NONE', ( #474, #45518, #52911, #13928 ) ) ;
#71848=CARTESIAN_POINT ( 'NONE',  ( 189.9889038007835040, 286.7716972915182509, 16.94430205996046013 ) ) ;
#71849=CARTESIAN_POINT ( 'NONE',  ( 116.2138665886017606, 251.2365022471903444, 2.944929066748280225E-16 ) ) ;
#71852=ORIENTED_EDGE ( 'NONE', *, *, #53702, .T. ) ;
#71853=CARTESIAN_POINT ( 'NONE',  ( 188.6960043714797166, 272.5830035644334544, 16.09278530888001413 ) ) ;
#71855=CARTESIAN_POINT ( 'NONE',  ( 203.0507839702407580, 278.9527209772879814, 16.21318481136342626 ) ) ;
#71857=CARTESIAN_POINT ( 'NONE',  ( 153.2283961777204695, 265.2476279883323400, -17.66880461074566000 ) ) ;
#71859=CARTESIAN_POINT ( 'NONE',  ( 174.4814676270071345, 252.3592025919409991, -0.2517021329253662509 ) ) ;
#71863=CARTESIAN_POINT ( 'NONE',  ( 170.7889457633958727, 250.2325148129452259, 2.962128769278053131 ) ) ;
#71864=CARTESIAN_POINT ( 'NONE',  ( 206.9220859797902961, 271.2613808489912799, -5.355436660003541682 ) ) ;
#71870=CARTESIAN_POINT ( 'NONE',  ( 168.0746954366166506, 276.8294243769387890, 15.45034248799716714 ) ) ;
#71871=CARTESIAN_POINT ( 'NONE',  ( 86.71718800452170228, 209.3262482093457493, 3.021315404115420679E-15 ) ) ;
#71873=EDGE_LOOP ( 'NONE', ( #98561, #16223, #12339, #31456, #5141, #80381, #76449, #61651, #50160, #48172, #64416, #63797, #72882, #60006, #35844, #1979, #73550, #38956, #84102, #8361 ) ) ;
#71874=CARTESIAN_POINT ( 'NONE',  ( 184.0405880873563547, 296.3429400402605438, 1.017449987670831169 ) ) ;
#71876=CARTESIAN_POINT ( 'NONE',  ( 194.4032909867620447, 293.9306181827685123, -16.05392006271526384 ) ) ;
#71877=CARTESIAN_POINT ( 'NONE',  ( 208.3586375946586315, 269.7592488206576604, -1.970210487958146128 ) ) ;
#71878=CARTESIAN_POINT ( 'NONE',  ( 185.4035662733510605, 292.5150471097351783, -10.83705993876271201 ) ) ;
#71881=CARTESIAN_POINT ( 'NONE',  ( 177.5654003108776351, 286.5527965801844630, -13.65658207675519975 ) ) ;
#71882=CARTESIAN_POINT ( 'NONE',  ( 83.31357524521028779, 231.1589784336661637, -6.496448406907675876E-16 ) ) ;
#71885=CARTESIAN_POINT ( 'NONE',  ( 149.9104953625653991, 271.4222773149817840, 11.90972932297161080 ) ) ;
#71886=CARTESIAN_POINT ( 'NONE',  ( 159.3383002321867821, 278.1316173108193084, 11.89870031586311683 ) ) ;
#71893=CARTESIAN_POINT ( 'NONE',  ( 75.36633504343575396, 220.9865022471902876, 10.00000000000009415 ) ) ;
#71896=CARTESIAN_POINT ( 'NONE',  ( 182.5291792280718823, 296.7636338796572204, 0.3805386115670883473 ) ) ;
#71897=CARTESIAN_POINT ( 'NONE',  ( 162.6076392040105816, 249.0023025302617725, 11.70000256607044165 ) ) ;
#71900=CARTESIAN_POINT ( 'NONE',  ( 163.4055107321044318, 247.6203485056908846, -10.24153090796238530 ) ) ;
#71901=ORIENTED_EDGE ( 'NONE', *, *, #29907, .T. ) ;
#71905=CARTESIAN_POINT ( 'NONE',  ( -15.15136185149820847, 175.3927522451419350, 2.944929066748280225E-16 ) ) ;
#71907=ORIENTED_EDGE ( 'NONE', *, *, #334, .T. ) ;
#71909=CARTESIAN_POINT ( 'NONE',  ( 160.1349499500167894, 275.4254527969055744, 12.83854157865886236 ) ) ;
#71910=CARTESIAN_POINT ( 'NONE',  ( 159.9894443651313338, 253.5371490153152081, -16.36035038356864391 ) ) ;
#71911=CARTESIAN_POINT ( 'NONE',  ( 188.9935787721526594, 269.7997667481943722, 14.53618363141985448 ) ) ;
#71913=CARTESIAN_POINT ( 'NONE',  ( 198.9561107160696736, 285.0479304499367572, -17.31132130523259960 ) ) ;
#71917=CARTESIAN_POINT ( 'NONE',  ( 203.2378153033330932, 277.9981038445823174, -14.71139916435034323 ) ) ;
#71918=CARTESIAN_POINT ( 'NONE',  ( 161.8811854682448939, 250.2605573099562264, 13.51112293479948789 ) ) ;
#71922=CARTESIAN_POINT ( 'NONE',  ( 174.8635978287226180, 290.2966283512476480, -6.424262721924552721 ) ) ;
#71924=ORIENTED_EDGE ( 'NONE', *, *, #85845, .F. ) ;
#71926=CARTESIAN_POINT ( 'NONE',  ( 164.7694554770609159, 245.2579269087094076, -3.003635650077957742 ) ) ;
#71931=CARTESIAN_POINT ( 'NONE',  ( 171.2100401816418298, 274.3227513589740738, 16.12125467595794959 ) ) ;
#71932=CARTESIAN_POINT ( 'NONE',  ( 181.7118876060299328, 273.6476297288324417, 17.70437625449880414 ) ) ;
#71934=CARTESIAN_POINT ( 'NONE',  ( 188.5734885077569629, 260.2193828105671400, 3.781240722223853989 ) ) ;
#71935=CARTESIAN_POINT ( 'NONE',  ( 207.8718670335145475, 270.6023601641878713, -6.322166851501095586 ) ) ;
#71936=CARTESIAN_POINT ( 'NONE',  ( 0.4998960083233069396, 183.3464784336661353, 1.353441290958777327E-15 ) ) ;
#71938=EDGE_LOOP ( 'NONE', ( #92093, #38701, #63127, #68419 ) ) ;
#71940=CARTESIAN_POINT ( 'NONE',  ( 178.7827978530413020, 256.8763733133778828, 8.538386915803064525 ) ) ;
#71941=CARTESIAN_POINT ( 'NONE',  ( 148.4047294057049555, 273.6024639162449716, 0.000000000000000000 ) ) ;
#71942=CARTESIAN_POINT ( 'NONE',  ( 191.1302745162771259, 290.4652077767679543, 15.89733196130017134 ) ) ;
#71944=CARTESIAN_POINT ( 'NONE',  ( 32.89474554257621719, 198.9869531367911293, 4.594050593750046652 ) ) ;
#71945=CARTESIAN_POINT ( 'NONE',  ( 200.1102648775588193, 284.0458494464393198, 17.54251420653697835 ) ) ;
#71946=CARTESIAN_POINT ( 'NONE',  ( 190.1693911629507738, 301.2639477917662703, -5.112716700269980485 ) ) ;
#71948=CARTESIAN_POINT ( 'NONE',  ( 181.7126073594628224, 294.1164641284040044, 6.307844905921689005 ) ) ;
#71949=CARTESIAN_POINT ( 'NONE',  ( 173.2870411084388138, 273.4504758881469115, -16.94085204434761494 ) ) ;
#71951=CARTESIAN_POINT ( 'NONE',  ( 5.270092192305421364, 185.3967562850347122, -4.648177544792955347E-16 ) ) ;
#71952=CARTESIAN_POINT ( 'NONE',  ( 77.46154149802761424, 203.9824982072973967, 3.021315404115420679E-15 ) ) ;
#71953=CARTESIAN_POINT ( 'NONE',  ( 186.8150228009728835, 295.8650736363334204, -7.734513286467996629 ) ) ;
#71955=CARTESIAN_POINT ( 'NONE',  ( 87.63502826371536969, 214.7365022471901739, -10.00000000000009059 ) ) ;
#71958=CARTESIAN_POINT ( 'NONE',  ( 44.34243207491050498, 208.6589784336661637, -6.496448406907675876E-16 ) ) ;
#71959=CARTESIAN_POINT ( 'NONE',  ( 159.2111180226792726, 254.8852497853115722, 16.01057445397460910 ) ) ;
#71962=CARTESIAN_POINT ( 'NONE',  ( 198.5511052797322975, 286.7463930869835167, -17.24711022262289006 ) ) ;
#71966=CARTESIAN_POINT ( 'NONE',  ( 168.0929298412453079, 282.0018323245688521, -10.93335134749426096 ) ) ;
#71970=CARTESIAN_POINT ( 'NONE',  ( 162.7644741734472120, 248.7306563947940958, 9.865755277559742353 ) ) ;
#71971=CARTESIAN_POINT ( 'NONE',  ( 149.1939152435731728, 272.2355539484436235, -11.44223522189843933 ) ) ;
#71972=CARTESIAN_POINT ( 'NONE',  ( 171.4773364337628152, 255.5008831467121979, 12.42855810394174121 ) ) ;
#71975=CARTESIAN_POINT ( 'NONE',  ( 171.9826536606966272, 253.0931212146789733, 8.466246838993372492 ) ) ;
#71977=ORIENTED_EDGE ( 'NONE', *, *, #77665, .T. ) ;
#71980=CARTESIAN_POINT ( 'NONE',  ( 177.3283375316947286, 255.9921738663651354, -7.116718427656683943 ) ) ;
#71985=CARTESIAN_POINT ( 'NONE',  ( -22.42236680055709641, 157.8615022471902591, 0.000000000000000000 ) ) ;
#71986=CARTESIAN_POINT ( 'NONE',  ( 151.0575349784822947, 270.7509268893103354, -13.83753715545528173 ) ) ;
#71987=ORIENTED_EDGE ( 'NONE', *, *, #88248, .F. ) ;
#71988=CARTESIAN_POINT ( 'NONE',  ( 200.6680263064462792, 283.0797783131037022, -17.21821073473145347 ) ) ;
#71992=CARTESIAN_POINT ( 'NONE',  ( 205.4103625296683617, 274.8658110279089897, -13.38953657917851814 ) ) ;
#71994=CARTESIAN_POINT ( 'NONE',  ( 108.5637151982415389, 242.6744531367911293, 4.594050593750047540 ) ) ;
#71995=CARTESIAN_POINT ( 'NONE',  ( 79.15288444911743682, 228.0530062829863027, -4.648177544792955347E-16 ) ) ;
#71998=CARTESIAN_POINT ( 'NONE',  ( 208.1415148974628266, 270.1353163636768500, 3.453641150550738725 ) ) ;
#71999=ORIENTED_EDGE ( 'NONE', *, *, #57502, .F. ) ;
#72001=CARTESIAN_POINT ( 'NONE',  ( 157.1457301079645958, 258.8834783542900482, 16.87614098766286119 ) ) ;
#72004=CARTESIAN_POINT ( 'NONE',  ( 68.02342162723002161, 200.8923013555409796, 4.594050593750050204 ) ) ;
#72006=CARTESIAN_POINT ( 'NONE',  ( 191.4922467593309250, 298.9726946877590876, 7.604184559945784017 ) ) ;
#72007=CARTESIAN_POINT ( 'NONE',  ( 92.59663213601577070, 224.2677522451418497, 10.00000000000009592 ) ) ;
#72009=B_SPLINE_CURVE_WITH_KNOTS ( 'NONE', 3,
 ( #82055, #5018, #57696, #65311, #12116, #27319 ),
 .UNSPECIFIED., .F., .F.,
 ( 4, 2, 4 ),
 ( 0.01870777577402827491, 0.02322058015305604461, 0.02773338453208381085 ),
 .UNSPECIFIED. ) ;
#72011=CARTESIAN_POINT ( 'NONE',  ( 156.6812872898450735, 261.2670451491295012, 0.000000000000000000 ) ) ;
#72012=CARTESIAN_POINT ( 'NONE',  ( 177.8473680943169484, 288.5077986257637122, 10.80235352749306621 ) ) ;
#72015=CARTESIAN_POINT ( 'NONE',  ( 101.3989120123781191, 240.8967562850346837, -4.648177544792955347E-16 ) ) ;
#72016=CARTESIAN_POINT ( 'NONE',  ( 173.8371423854052580, 278.0697674778426176, -16.44858265900196770 ) ) ;
#72018=CARTESIAN_POINT ( 'NONE',  ( 161.0965315767822972, 251.6196177163260188, -13.76772246540905442 ) ) ;
#72019=CARTESIAN_POINT ( 'NONE',  ( 206.4708747408093643, 270.6173459074702805, 2.419506436698913188 ) ) ;
#72020=CARTESIAN_POINT ( 'NONE',  ( 149.3883679478359454, 271.8987519849911223, 12.99187507659642371 ) ) ;
#72021=CARTESIAN_POINT ( 'NONE',  ( 177.2096423064392070, 269.5159051785426527, 16.11451641950014491 ) ) ;
#72023=DIRECTION ( 'NONE',  ( -0.8660254037844387076, -0.4999999999999998890, -0.000000000000000000 ) ) ;
#72025=CARTESIAN_POINT ( 'NONE',  ( 167.9973872756363562, 255.7907068641800379, 13.67785959516219130 ) ) ;
#72026=CYLINDRICAL_SURFACE ( 'NONE', #90143, 17.82106496071139645 ) ;
#72027=CARTESIAN_POINT ( 'NONE',  ( 110.0256537107753161, 225.1423013555409796, -4.594050593750043987 ) ) ;
#72028=ORIENTED_EDGE ( 'NONE', *, *, #15084, .T. ) ;
#72030=CARTESIAN_POINT ( 'NONE',  ( 92.93397336236306217, 212.9155109091896065, 2.679491924311254714 ) ) ;
#72033=CARTESIAN_POINT ( 'NONE',  ( 183.2230023984259333, 284.8711938070701990, -14.93434685926643013 ) ) ;
#72038=CARTESIAN_POINT ( 'NONE',  ( 157.3661001067102916, 274.3687252322818040, -12.59994636575860838 ) ) ;
#72039=CARTESIAN_POINT ( 'NONE',  ( 185.8872707255410432, 262.0278434869816238, 9.890274748944476002 ) ) ;
#72041=CARTESIAN_POINT ( 'NONE',  ( 147.1836429658426368, 243.5327760586659451, 1.948934522072302763E-15 ) ) ;
#72044=DIRECTION ( 'NONE',  ( -0.5000000000000006661, 0.8660254037844382635, -1.877843081442121204E-16 ) ) ;
#72045=CARTESIAN_POINT ( 'NONE',  ( 54.35602435405059651, 208.3149278399161233, -9.188101187500095079 ) ) ;
#72046=CARTESIAN_POINT ( 'NONE',  ( 164.8670003495851404, 245.0889742334797177, -1.557028074864921674 ) ) ;
#72047=CARTESIAN_POINT ( 'NONE',  ( 191.5083466856444261, 297.3227120659499292, 10.96045759559922317 ) ) ;
#72050=CARTESIAN_POINT ( 'NONE',  ( 199.9134407114337364, 283.6250491837689651, 17.05367660732407842 ) ) ;
#72052=CARTESIAN_POINT ( 'NONE',  ( 169.4088087987535687, 285.0667569032603410, -8.267254425861240819 ) ) ;
#72053=CARTESIAN_POINT ( 'NONE',  ( 155.2922060645262263, 261.6730044072216401, -16.98884022075611355 ) ) ;
#72055=ADVANCED_FACE ( 'NONE', ( #12894 ), #19508, .T. ) ;
#72056=CARTESIAN_POINT ( 'NONE',  ( 131.1347626044233152, 236.5177522451417929, 5.000000000000051514 ) ) ;
#72057=B_SPLINE_SURFACE_WITH_KNOTS ( 'NONE', 3, 1, ( 
 ( #71946, #41516 ),
 ( #79578, #50610 ),
 ( #27826, #58702 ),
 ( #3550, #27337 ),
 ( #12135, #26833 ),
 ( #42997, #4521 ),
 ( #42024, #42506 ),
 ( #73442, #72958 ),
 ( #28312, #81080 ),
 ( #4026, #5033 ),
 ( #34428, #89197 ),
 ( #49623, #95785 ),
 ( #11646, #96267 ),
 ( #26339, #13141 ),
 ( #57215, #96771 ),
 ( #19745, #65328 ),
 ( #72460, #57711 ),
 ( #58218, #88691 ),
 ( #89676, #88190 ),
 ( #34912, #19261 ),
 ( #59190, #43514 ),
 ( #65810, #73935 ),
 ( #20237, #35422 ),
 ( #81564, #50128 ),
 ( #66327, #97259 ),
 ( #51109, #33951 ),
 ( #82074, #12644 ),
 ( #74453, #35915 ),
 ( #66816, #97744 ),
 ( #18739, #90166 ),
 ( #20739, #51626 ),
 ( #82578, #3065 ),
 ( #64838, #80577 ),
 ( #11157, #7504 ) ),
 .UNSPECIFIED., .T., .F., .F.,
 ( 4, 2, 2, 2, 2, 2, 2, 2, 2, 2, 2, 2, 2, 2, 2, 2, 4 ),
 ( 2, 2 ),
 ( 0.000000000000000000, 0.06250000000000000000, 0.1250000000000000000, 0.1875000000000000000, 0.2500000000000000000, 0.3125000000000000000, 0.3750000000000000000, 0.4375000000000000000, 0.5000000000000000000, 0.5625000000000000000, 0.6250000000000000000, 0.6875000000000000000, 0.7500000000000000000, 0.8125000000000000000, 0.8750000000000000000, 0.9375000000000000000, 1.000000000000000000 ),
 ( 0.000000000000000000, 1.000000000000000000 ),
 .UNSPECIFIED. ) ;
#72061=EDGE_CURVE ( 'NONE', #86304, #11813, #80721, .T. ) ;
#72065=CARTESIAN_POINT ( 'NONE',  ( 43.96406660440233338, 190.0643266524159571, -9.188101187500093303 ) ) ;
#72067=CARTESIAN_POINT ( 'NONE',  ( 41.14028939449039513, 187.8927522451418213, 10.00000000000009948 ) ) ;
#72069=CARTESIAN_POINT ( 'NONE',  ( 190.8957779480239765, 300.0058089740729770, -4.541438514207768229 ) ) ;
#72073=CARTESIAN_POINT ( 'NONE',  ( 53.62548896571601631, 201.7677522451418781, 10.00000000000009592 ) ) ;
#72075=CARTESIAN_POINT ( 'NONE',  ( 174.5898090886373097, 289.3010444735929809, 7.825388048759662318 ) ) ;
#72077=CARTESIAN_POINT ( 'NONE',  ( 157.8239779013331372, 257.2878469527003062, -17.92251383114021479 ) ) ;
#72078=CARTESIAN_POINT ( 'NONE',  ( 162.1762925668143396, 251.9858117565144084, -13.16816576803558014 ) ) ;
#72079=( BOUNDED_CURVE ( )  B_SPLINE_CURVE ( 2, ( #80553, #42000, #49110, #33406, #46208, #32405, #63804, #3039, #33929 ),
 .UNSPECIFIED., .F., .T. ) 
 B_SPLINE_CURVE_WITH_KNOTS ( ( 3, 2, 2, 2, 3 ),
 ( 0.7862903225806451291, 0.7876344086021505042, 0.7903225806451612545, 0.7930107526881720048, 0.7943548387096773800 ),
 .UNSPECIFIED. ) 
 CURVE ( )  GEOMETRIC_REPRESENTATION_ITEM ( )  RATIONAL_B_SPLINE_CURVE ( ( 0.9330127018922194093, 0.9330127018922194093, 1.000000000000000000, 0.8660254037844387076, 1.000000000000000000, 0.8660254037844387076, 1.000000000000000000, 0.9330127018922194093, 0.9330127018922194093 ) ) 
 REPRESENTATION_ITEM ( '' )  );
#72080=CARTESIAN_POINT ( 'NONE',  ( 38.99326808448932979, 199.9865022471902876, 10.00000000000009237 ) ) ;
#72081=CARTESIAN_POINT ( 'NONE',  ( 156.6812872898450735, 261.2670451491295012, 0.000000000000000000 ) ) ;
#72082=CARTESIAN_POINT ( 'NONE',  ( 202.5245888501533216, 279.8641176599742266, 15.60152447840272494 ) ) ;
#72083=CARTESIAN_POINT ( 'NONE',  ( -7.619092152155812592, 178.6589784336661637, -6.496448406907675876E-16 ) ) ;
#72086=CARTESIAN_POINT ( 'NONE',  ( 200.4065898033495046, 283.0201594895918333, 16.80763448860258791 ) ) ;
#72087=CARTESIAN_POINT ( 'NONE',  ( 192.0331311261993790, 298.0358554833232461, 11.82583305898340953 ) ) ;
#72089=CARTESIAN_POINT ( 'NONE',  ( 155.5606021264401875, 261.5901729271447493, -16.99161892237499671 ) ) ;
#72090=CARTESIAN_POINT ( 'NONE',  ( 183.8754313647489198, 256.5225093191261294, -2.022205659181245174 ) ) ;
#72093=DIRECTION ( 'NONE',  ( 0.4999999999999998890, -0.8660254037844385966, 0.000000000000000000 ) ) ;
#72096=CARTESIAN_POINT ( 'NONE',  ( 153.5867603639496508, 277.8595165095850916, -5.207415017408751901 ) ) ;
#72098=CARTESIAN_POINT ( 'NONE',  ( 75.87151652897675547, 204.6115022471901739, -5.000000000000041744 ) ) ;
#72101=CARTESIAN_POINT ( 'NONE',  ( 159.6962080797732710, 254.0450491601782232, -15.33973334987084947 ) ) ;
#72102=VERTEX_POINT ( 'NONE', #26586 ) ;
#72103=( BOUNDED_CURVE ( )  B_SPLINE_CURVE ( 2, ( #64455, #62428, #25449, #17869, #63453, #17346, #40131, #1672, #56338 ),
 .UNSPECIFIED., .F., .T. ) 
 B_SPLINE_CURVE_WITH_KNOTS ( ( 3, 2, 2, 2, 3 ),
 ( 0.5524193548387096309, 0.5537634408602150060, 0.5564516129032257563, 0.5591397849462365066, 0.5604838709677418818 ),
 .UNSPECIFIED. ) 
 CURVE ( )  GEOMETRIC_REPRESENTATION_ITEM ( )  RATIONAL_B_SPLINE_CURVE ( ( 0.9330127018922194093, 0.9330127018922194093, 1.000000000000000000, 0.8660254037844387076, 1.000000000000000000, 0.8660254037844387076, 1.000000000000000000, 0.9330127018922194093, 0.9330127018922194093 ) ) 
 REPRESENTATION_ITEM ( '' )  );
#72104=CARTESIAN_POINT ( 'NONE',  ( 192.5254593562406171, 297.1831179748913314, 11.00703791256144015 ) ) ;
#72105=CARTESIAN_POINT ( 'NONE',  ( 164.2953672501826929, 246.0790718049323687, -2.576662677987826111 ) ) ;
#72109=CARTESIAN_POINT ( 'NONE',  ( 154.9683083969241011, 262.2340116239618055, 18.33261662430134109 ) ) ;
#72122=CARTESIAN_POINT ( 'NONE',  ( 200.4403816905005158, 283.4740703539914648, 16.81798557643505987 ) ) ;
#72123=CARTESIAN_POINT ( 'NONE',  ( 166.8997956679749564, 274.6136247820161316, -15.18620604814603503 ) ) ;
#72126=ORIENTED_EDGE ( 'NONE', *, *, #19669, .F. ) ;
#72127=CARTESIAN_POINT ( 'NONE',  ( 173.8258004643798245, 257.2059766620726009, -11.79308939057215255 ) ) ;
#72128=FACE_OUTER_BOUND ( 'NONE', #83627, .T. ) ;
#72131=CARTESIAN_POINT ( 'NONE',  ( 159.8820994310810022, 268.4908852645613706, -16.43388976517952571 ) ) ;
#72133=ORIENTED_EDGE ( 'NONE', *, *, #3337, .F. ) ;
#72137=CARTESIAN_POINT ( 'NONE',  ( 193.9762986263216646, 294.6701906454947562, 14.66460157377692042 ) ) ;
#72138=CARTESIAN_POINT ( 'NONE',  ( 176.9659610627589359, 289.4039066173891115, -10.56313750161503151 ) ) ;
#72139=B_SPLINE_CURVE_WITH_KNOTS ( 'NONE', 3,
 ( #47184, #24886, #62884, #78612, #40575, #40071, #86755, #34017, #17288, #71014, #1616, #32987, #79640, #16788, #63393, #56786, #26404, #32502, #9720, #17807, #94333, #10207, #78105, #8695, #55270, #64396, #18308, #95359, #86250, #48192, #16290, #48707, #87277, #79139, #87770, #31980, #71516, #39564, #2106, #10705, #70488, #25914, #80140, #3132 ),
 .UNSPECIFIED., .F., .F.,
 ( 4, 2, 2, 2, 2, 2, 2, 2, 2, 2, 2, 2, 2, 2, 2, 2, 2, 2, 2, 2, 2, 4 ),
 ( 0.0004122447795833745587, 0.001425156861282679847, 0.001931612902132293650, 0.002184840922557164736, 0.002311454932769600387, 0.002438068942982036039, 0.002691296963406946807, 0.002944524983831857574, 0.003450981024681599313, 0.004463893106381080188, 0.005476805188080561063, 0.005983261228930296730, 0.006236489249355129001, 0.006489717269779959538, 0.006553024274886150476, 0.006616331279992340546, 0.006679638285098531483, 0.006742945290204721553, 0.006996173310629566836, 0.007502629351479299900, 0.008009085392329034700, 0.008515541433178768632 ),
 .UNSPECIFIED. ) ;
#72141=CARTESIAN_POINT ( 'NONE',  ( 193.3011194324739961, 295.0724505835075320, 13.25748537430616381 ) ) ;
#72143=CARTESIAN_POINT ( 'NONE',  ( 175.2538527669093753, 291.0550713335976525, 6.537906992358419878 ) ) ;
#72144=FACE_OUTER_BOUND ( 'NONE', #57516, .T. ) ;
#72148=CARTESIAN_POINT ( 'NONE',  ( 206.1932826529868805, 273.5097535960530877, 11.72208607728249241 ) ) ;
#72149=CARTESIAN_POINT ( 'NONE',  ( 206.3505875407052486, 273.2372935382459787, 11.62318091048137880 ) ) ;
#72153=B_SPLINE_CURVE_WITH_KNOTS ( 'NONE', 3,
 ( #61170, #22691, #45957, #76874 ),
 .UNSPECIFIED., .F., .F.,
 ( 4, 4 ),
 ( 0.01224253334696489767, 0.01843315522474755358 ),
 .UNSPECIFIED. ) ;
#72154=CARTESIAN_POINT ( 'NONE',  ( 146.7209331427380050, 276.5188845932982531, -2.966446756160787679 ) ) ;
#72156=DIRECTION ( 'NONE',  ( -0.8660254037844387076, -0.4999999999999998890, -0.000000000000000000 ) ) ;
#72159=EDGE_CURVE ( 'NONE', #99538, #67236, #90409, .T. ) ;
#72160=CARTESIAN_POINT ( 'NONE',  ( 189.4381674897702794, 265.0040801212285828, 12.03645615491573828 ) ) ;
#72162=ORIENTED_EDGE ( 'NONE', *, *, #99095, .F. ) ;
#72163=CARTESIAN_POINT ( 'NONE',  ( -22.42236680055709641, 157.8615022471902591, 0.000000000000000000 ) ) ;
#72165=CARTESIAN_POINT ( 'NONE',  ( 49.80054343233477709, 192.8927522451417929, -10.00000000000009237 ) ) ;
#72166=CARTESIAN_POINT ( 'NONE',  ( 207.4285356523023154, 271.3702326410368642, 7.833982582429932506 ) ) ;
#72167=CARTESIAN_POINT ( 'NONE',  ( 16.02555268474158723, 193.3927522451419350, 2.944929066748280225E-16 ) ) ;
#72168=CARTESIAN_POINT ( 'NONE',  ( 97.84665082640911749, 236.4869531367911293, 4.594050593750046652 ) ) ;
#72170=CARTESIAN_POINT ( 'NONE',  ( 173.3920276507685401, 289.7572511702507541, -7.189583706006478891 ) ) ;
#72171=CARTESIAN_POINT ( 'NONE',  ( 207.6964130646365163, 270.9062553526738384, 2.975933372805272814 ) ) ;
#72172=CARTESIAN_POINT ( 'NONE',  ( 26.56245542105003210, 176.9548013555409796, -4.594050593750042211 ) ) ;
#72177=CARTESIAN_POINT ( 'NONE',  ( 200.4912881644965807, 267.5564725962747161, -2.850958659151126007 ) ) ;
#72179=VECTOR ( 'NONE', #65910, 1000.000000000000000 ) ;
#72181=CARTESIAN_POINT ( 'NONE',  ( 192.9756790785140765, 263.8394000145765972, -4.280765219900059648 ) ) ;
#72182=CARTESIAN_POINT ( 'NONE',  ( 161.2488013048736377, 251.3558788108169040, -13.10044423494716170 ) ) ;
#72184=CARTESIAN_POINT ( 'NONE',  ( 167.3696659777530158, 251.6663404442222713, 10.32696327628674915 ) ) ;
#72185=EDGE_CURVE ( 'NONE', #79646, #45796, #2669, .T. ) ;
#72186=CARTESIAN_POINT ( 'NONE',  ( 42.47567221558909267, 186.1423013555410080, -4.594050593750043987 ) ) ;
#72187=CARTESIAN_POINT ( 'NONE',  ( 82.70950877614343710, 211.8927522451418213, 10.00000000000009592 ) ) ;
#72188=ORIENTED_EDGE ( 'NONE', *, *, #31033, .T. ) ;
#72191=EDGE_CURVE ( 'NONE', #11457, #61620, #72103, .T. ) ;
#72192=CARTESIAN_POINT ( 'NONE',  ( 179.3683703725943417, 258.0455820962152984, -10.44019545301878082 ) ) ;
#72193=CARTESIAN_POINT ( 'NONE',  ( -5.237175195983594378, 167.7833772461660828, -9.188101187500095079 ) ) ;
#72196=CARTESIAN_POINT ( 'NONE',  ( 151.3898985249405200, 268.4319993325432847, -14.65018536945715510 ) ) ;
#72198=CARTESIAN_POINT ( 'NONE',  ( 186.1163208250084438, 283.4177454897106259, 16.70810301636890571 ) ) ;
#72199=CARTESIAN_POINT ( 'NONE',  ( 147.5381343315788172, 275.1034506142203782, -4.056595942992749393 ) ) ;
#72202=CARTESIAN_POINT ( 'NONE',  ( 164.2413944571582078, 246.1725554246774834, 7.304616466633322425 ) ) ;
#72203=CARTESIAN_POINT ( 'NONE',  ( 147.2592533090473239, 275.5864867145116932, -0.3770461397900867762 ) ) ;
#72204=CARTESIAN_POINT ( 'NONE',  ( 164.7243055739305078, 245.3361288348881999, -1.445094907380085170 ) ) ;
#72205=ORIENTED_EDGE ( 'NONE', *, *, #15399, .T. ) ;
#72207=CARTESIAN_POINT ( 'NONE',  ( 4.352251933111862314, 159.9865022471901739, 1.119607411625061291E-15 ) ) ;
#72208=CARTESIAN_POINT ( 'NONE',  ( 143.4214980241629576, 243.6115022471902023, -5.000000000000041744 ) ) ;
#72209=CARTESIAN_POINT ( 'NONE',  ( 132.2986577904150920, 241.0643266524159856, -9.188101187500093303 ) ) ;
#72212=CARTESIAN_POINT ( 'NONE',  ( 151.0474090540779741, 270.2368430214293653, 13.84391263241849934 ) ) ;
#72213=CARTESIAN_POINT ( 'NONE',  ( 195.8947060313465443, 291.3474115503753410, 16.07878593000791767 ) ) ;
#72214=CARTESIAN_POINT ( 'NONE',  ( 141.9699493749754140, 259.7505386000626686, -7.968025677899344572 ) ) ;
#72215=CARTESIAN_POINT ( 'NONE',  ( 191.0469974725420172, 299.7438890745112872, -6.451222553760779910 ) ) ;
#72217=CARTESIAN_POINT ( 'NONE',  ( 192.9845471803554346, 263.7469009655502532, -5.013485419990833414 ) ) ;
#72218=CARTESIAN_POINT ( 'NONE',  ( 196.8363552541316324, 289.7164272536036265, -17.80258609350122967 ) ) ;
#72219=CARTESIAN_POINT ( 'NONE',  ( 187.4784686605442232, 261.8693247467304559, 9.829215920296768161 ) ) ;
#72224=CARTESIAN_POINT ( 'NONE',  ( 175.1874290394435434, 279.2259713227149973, 15.64062928220176474 ) ) ;
#72225=CARTESIAN_POINT ( 'NONE',  ( 168.8736724576156405, 271.8586482977812011, -16.82536904539195532 ) ) ;
#72230=CARTESIAN_POINT ( 'NONE',  ( 153.1314981037513121, 265.4154603756023789, 17.73969815997475408 ) ) ;
#72232=B_SPLINE_CURVE_WITH_KNOTS ( 'NONE', 3,
 ( #9665, #30576, #45270, #46247 ),
 .UNSPECIFIED., .F., .F.,
 ( 4, 4 ),
 ( 6.208857164277751492E-15, 0.0007264857576706923751 ),
 .UNSPECIFIED. ) ;
#72235=CARTESIAN_POINT ( 'NONE',  ( 191.9438504840783821, 288.0378779041730013, -15.85995341028061389 ) ) ;
#72237=CARTESIAN_POINT ( 'NONE',  ( 163.8195406495391353, 279.5693214144951071, 12.35214766166425093 ) ) ;
#72239=CARTESIAN_POINT ( 'NONE',  ( 194.9220242159064185, 293.0321458743159724, -14.92681063007793263 ) ) ;
#72242=CARTESIAN_POINT ( 'NONE',  ( -22.42236680055709641, 157.8615022471902591, 0.000000000000000000 ) ) ;
#72243=CARTESIAN_POINT ( 'NONE',  ( 187.8752290710686452, 292.6574842239962209, 12.38629875236594557 ) ) ;
#72244=CARTESIAN_POINT ( 'NONE',  ( 191.4922467593309250, 298.9726946877590876, 7.604184559945784017 ) ) ;
#72253=CARTESIAN_POINT ( 'NONE',  ( 175.3253744491786676, 258.9757446337468991, 12.55620439745121608 ) ) ;
#72255=ORIENTED_EDGE ( 'NONE', *, *, #76246, .F. ) ;
#72256=CARTESIAN_POINT ( 'NONE',  ( 52.03546399666511491, 212.3967562850347122, -4.648177544792955347E-16 ) ) ;
#72259=FACE_OUTER_BOUND ( 'NONE', #77773, .T. ) ;
#72261=CARTESIAN_POINT ( 'NONE',  ( 186.1558086338376370, 282.4460829780409199, -16.80270888845420174 ) ) ;
#72264=CARTESIAN_POINT ( 'NONE',  ( 161.9353223911033410, 277.5374438971563222, -13.12909115375462576 ) ) ;
#72265=CARTESIAN_POINT ( 'NONE',  ( 147.3236643320416022, 275.4749235501183193, -5.185334239426818037 ) ) ;
#72266=CARTESIAN_POINT ( 'NONE',  ( 153.3544108199959908, 265.0293642254135307, -17.49105661178601423 ) ) ;
#72269=CARTESIAN_POINT ( 'NONE',  ( 157.9710662556744012, 281.0034536832922072, 2.292689402901011420 ) ) ;
#72270=CARTESIAN_POINT ( 'NONE',  ( 136.3040252829181327, 243.3768266524159856, 9.188101187500098632 ) ) ;
#72274=ORIENTED_EDGE ( 'NONE', *, *, #51316, .T. ) ;
#72276=CARTESIAN_POINT ( 'NONE',  ( 177.7342311040593756, 255.2532439957012684, -8.367404576774948310 ) ) ;
#72277=CARTESIAN_POINT ( 'NONE',  ( 178.9714194486930694, 253.6239517424200187, 1.422777586239305059 ) ) ;
#72278=CARTESIAN_POINT ( 'NONE',  ( 129.5390911288783684, 234.0494855054051584, -2.679491924311248496 ) ) ;
#72279=CARTESIAN_POINT ( 'NONE',  ( 147.2481089941287280, 275.6057892341661386, 4.088130380788767226 ) ) ;
#72280=CARTESIAN_POINT ( 'NONE',  ( 155.8801288042594990, 278.4237519192228660, 7.215275691167001071 ) ) ;
#72281=EDGE_CURVE ( 'NONE', #7878, #55188, #46750, .T. ) ;
#72282=CARTESIAN_POINT ( 'NONE',  ( 192.1779685593947420, 266.1842805242176269, 11.64530923862864142 ) ) ;
#72285=CARTESIAN_POINT ( 'NONE',  ( 170.9849025567062313, 280.9340470213971344, 14.23665144915766234 ) ) ;
#72288=CARTESIAN_POINT ( 'NONE',  ( 177.2393968558746735, 256.1135909324575550, -7.883863129844044693 ) ) ;
#72289=ORIENTED_EDGE ( 'NONE', *, *, #33031, .T. ) ;
#72290=CARTESIAN_POINT ( 'NONE',  ( 194.2900850603946310, 294.1266965989547657, -15.88613936555681505 ) ) ;
#72292=ORIENTED_EDGE ( 'NONE', *, *, #60788, .T. ) ;
#72293=CARTESIAN_POINT ( 'NONE',  ( 188.6301707762981152, 265.0060877223691591, -12.46499516475016733 ) ) ;
#72294=CARTESIAN_POINT ( 'NONE',  ( 201.4081090739200306, 268.0418142524571863, -2.853212221150517536 ) ) ;
#72295=CARTESIAN_POINT ( 'NONE',  ( 151.8037247284637488, 267.7152313225378180, -16.71686542126332853 ) ) ;
#72296=CARTESIAN_POINT ( 'NONE',  ( 190.8187029736043883, 300.1393067457597681, 3.941064102378585954 ) ) ;
#72297=CARTESIAN_POINT ( 'NONE',  ( 202.5511585997265911, 279.8180975037686835, 17.12781264818056925 ) ) ;
#72298=CARTESIAN_POINT ( 'NONE',  ( 161.4200482637542962, 281.4224831315765982, -7.121073954846943721 ) ) ;
#72299=CARTESIAN_POINT ( 'NONE',  ( 152.1281151080858933, 275.3594634850046532, -8.621110135100591876 ) ) ;
#72300=CARTESIAN_POINT ( 'NONE',  ( 111.2365322456207224, 223.4824982072973683, 3.021315404115420679E-15 ) ) ;
#72301=ORIENTED_EDGE ( 'NONE', *, *, #93944, .T. ) ;
#72305=CARTESIAN_POINT ( 'NONE',  ( 152.6656396574222754, 266.2223508737794759, 17.04346597795114349 ) ) ;
#72308=B_SPLINE_CURVE_WITH_KNOTS ( 'NONE', 3,
 ( #48045, #49547, #73364, #88117 ),
 .UNSPECIFIED., .F., .F.,
 ( 4, 4 ),
 ( 0.009486792614561130252, 0.01778295607789639327 ),
 .UNSPECIFIED. ) ;
#72309=EDGE_CURVE ( 'NONE', #96192, #14857, #68437, .T. ) ;
#72310=CARTESIAN_POINT ( 'NONE',  ( -14.60124842228533915, 168.5024278399160949, 9.188101187500095079 ) ) ;
#72311=CARTESIAN_POINT ( 'NONE',  ( 94.19319292813476352, 231.3149278399160664, 9.188101187500093303 ) ) ;
#72312=CARTESIAN_POINT ( 'NONE',  ( 155.6535436963908694, 261.0471492701456668, -17.87366571046205976 ) ) ;
#72313=CARTESIAN_POINT ( 'NONE',  ( 146.7842303614460207, 276.4092505945183689, -4.491116827832889236 ) ) ;
#72314=CARTESIAN_POINT ( 'NONE',  ( 147.8194150887063643, 275.1866381610261101, 4.566218682955557107 ) ) ;
#72318=CARTESIAN_POINT ( 'NONE',  ( 172.7264208856190919, 290.8582626858774347, 2.771863430787652849 ) ) ;
#72319=CIRCLE ( 'NONE', #15655, 10.00000000000007816 ) ;
#72320=CARTESIAN_POINT ( 'NONE',  ( 160.9539812394163221, 281.6746053238863965, 5.581094101012241460 ) ) ;
#72322=CARTESIAN_POINT ( 'NONE',  ( 163.3723087697842971, 247.6778559913402091, -10.08585062664141319 ) ) ;
#72323=CARTESIAN_POINT ( 'NONE',  ( 177.9561663662901765, 289.9063764978683935, 9.646858304667830453 ) ) ;
#72326=B_SPLINE_CURVE_WITH_KNOTS ( 'NONE', 3,
 ( #75441, #29334, #77305, #36415, #7912, #38787, #792, #69693, #62076, #44005, #93024, #15998, #74947, #77821, #8403, #85969, #54990, #16494, #62576, #67319, #93538, #98247, #47391, #78315, #39765, #70694, #32192, #63094, #94040, #2319, #73216, #33199, #33717, #64608, #2828, #95564, #26110, #56496, #25088, #56985, #11430, #9917, #34207, #26608, #10915, #87970, #80858, #42282, #63595, #32694 ),
 .UNSPECIFIED., .F., .F.,
 ( 4, 2, 2, 2, 2, 2, 2, 2, 2, 2, 2, 2, 2, 2, 2, 2, 2, 2, 2, 2, 2, 2, 2, 2, 4 ),
 ( 0.0002455370680951060418, 0.0007226616231845173211, 0.001199786178273928600, 0.001438348455818573958, 0.001557629594590812178, 0.001676910733363050614, 0.001796191872135289051, 0.001915473010907527271, 0.002154035288451925430, 0.002631159843540722184, 0.003108284398629518504, 0.004062533508807189206, 0.005016782618984860775, 0.005493907174073697428, 0.005732469451618076722, 0.005851750590390267237, 0.005971031729162457752, 0.006030672298548521784, 0.006090312867934584082, 0.006209594006706670513, 0.006448156284250841641, 0.006925280839339159611, 0.007163843116883351556, 0.007402405394427543500, 0.007879529949515927389 ),
 .UNSPECIFIED. ) ;
#72327=CARTESIAN_POINT ( 'NONE',  ( 164.5261241815984761, 245.6793890755219252, -5.756220888378682510 ) ) ;
#72330=CARTESIAN_POINT ( 'NONE',  ( 81.75096066047075283, 229.5530062829863027, -4.648177544792955347E-16 ) ) ;
#72332=CARTESIAN_POINT ( 'NONE',  ( 49.32242524243604720, 199.2833772461660828, -9.188101187500095079 ) ) ;
#72334=CARTESIAN_POINT ( 'NONE',  ( 65.45180129215621889, 220.8464784336661637, 1.353441290958777327E-15 ) ) ;
#72335=CARTESIAN_POINT ( 'NONE',  ( 207.2683629543511756, 271.6476598918739001, -6.694388351944108528 ) ) ;
#72340=CARTESIAN_POINT ( 'NONE',  ( 196.7338846360856337, 268.5824883939956180, -10.68874749315578399 ) ) ;
#72347=CARTESIAN_POINT ( 'NONE',  ( 72.54255783352381570, 218.8149278399160664, -9.188101187500095079 ) ) ;
#72348=CARTESIAN_POINT ( 'NONE',  ( 88.40853095561153907, 233.3967562850347122, -4.648177544792955347E-16 ) ) ;
#72350=DIRECTION ( 'NONE',  ( 0.4999999999999998890, -0.8660254037844385966, 0.000000000000000000 ) ) ;
#72351=CARTESIAN_POINT ( 'NONE',  ( 192.6247335881259630, 297.0111699613833594, -13.30158778996737290 ) ) ;
#72352=CARTESIAN_POINT ( 'NONE',  ( 202.1168934888335684, 280.5702667397902133, 16.99860635998273750 ) ) ;
#72355=CARTESIAN_POINT ( 'NONE',  ( 193.5890283099523401, 288.4767073959486652, 16.07932638873488074 ) ) ;
#72357=CARTESIAN_POINT ( 'NONE',  ( 135.1942566882107997, 238.8615022471902023, 5.000000000000051514 ) ) ;
#72358=CARTESIAN_POINT ( 'NONE',  ( 157.7733463334721478, 257.3755434007023268, -16.94489513499352995 ) ) ;
#72360=CARTESIAN_POINT ( 'NONE',  ( 188.2493976403605984, 273.3260856929751981, 15.61695768125983363 ) ) ;
#72361=EDGE_LOOP ( 'NONE', ( #75739, #40692, #11237, #32678, #83362, #61379, #67064, #24397, #84843, #57871, #8280, #78726, #53167, #43528, #14529, #51020, #40415, #43811, #50567, #84578 ) ) ;
#72362=CARTESIAN_POINT ( 'NONE',  ( 206.7893622945242385, 272.4773133715531230, -10.52881283832460291 ) ) ;
#72368=ORIENTED_EDGE ( 'NONE', *, *, #79165, .T. ) ;
#72369=CARTESIAN_POINT ( 'NONE',  ( 189.9629097242743399, 290.3047074849306455, 14.47560175050799813 ) ) ;
#72370=CARTESIAN_POINT ( 'NONE',  ( 167.4002430202556582, 247.6565219373602531, 3.576405092176313971 ) ) ;
#72371=CARTESIAN_POINT ( 'NONE',  ( 153.4542976351440302, 264.8563551865710224, -17.11782692037292009 ) ) ;
#72375=CARTESIAN_POINT ( 'NONE',  ( 168.1167649493694398, 276.7715220293193283, 15.30949590115454129 ) ) ;
#72378=ORIENTED_EDGE ( 'NONE', *, *, #11354, .F. ) ;
#72379=CARTESIAN_POINT ( 'NONE',  ( 186.1400847795470099, 298.1223424718040178, 1.048499119586248085 ) ) ;
#72380=CARTESIAN_POINT ( 'NONE',  ( 164.1224127655298730, 246.3786377597482158, 7.356982420601481998 ) ) ;
#72381=CARTESIAN_POINT ( 'NONE',  ( 194.8067605455144076, 293.2317884077015151, -16.00245909155922774 ) ) ;
#72383=CARTESIAN_POINT ( 'NONE',  ( 155.6559071247401960, 261.0430556921643870, 17.79853447468815375 ) ) ;
#72386=CARTESIAN_POINT ( 'NONE',  ( 164.4343973647912946, 245.8382645826486055, 4.228584463013169703 ) ) ;
#72387=CARTESIAN_POINT ( 'NONE',  ( 169.5474634885189005, 267.2654023188423480, 17.55852261903751099 ) ) ;
#72389=B_SPLINE_CURVE_WITH_KNOTS ( 'NONE', 3,
 ( #28734, #21153, #6918, #52032 ),
 .UNSPECIFIED., .F., .F.,
 ( 4, 4 ),
 ( 0.004231976529499276163, 0.009740177386616696159 ),
 .UNSPECIFIED. ) ;
#72390=CARTESIAN_POINT ( 'NONE',  ( 86.66977078063996487, 220.8458772461660544, 9.188101187500095079 ) ) ;
#72393=CARTESIAN_POINT ( 'NONE',  ( 163.2006102744146290, 276.5399316210059055, -13.88336064207830312 ) ) ;
#72394=AXIS2_PLACEMENT_3D ( 'NONE', #37772, #28691, #99106 ) ;
#72395=ORIENTED_EDGE ( 'NONE', *, *, #5956, .F. ) ;
#72397=ORIENTED_EDGE ( 'NONE', *, *, #77789, .T. ) ;
#72399=CARTESIAN_POINT ( 'NONE',  ( 191.0478321355427624, 299.7424433957868928, -9.006798842970001218 ) ) ;
#72400=B_SPLINE_SURFACE_WITH_KNOTS ( 'NONE', 3, 1, ( 
 ( #25251, #87132 ),
 ( #33881, #18163 ),
 ( #71876, #17664 ),
 ( #86615, #1963 ),
 ( #88120, #41441 ),
 ( #79997, #81012 ),
 ( #34354, #65250 ),
 ( #72381, #88616 ),
 ( #48047, #48562 ),
 ( #49549, #55630 ),
 ( #25775, #64255 ),
 ( #33355, #11076 ),
 ( #96196, #71374 ),
 ( #64766, #18669 ),
 ( #96693, #32848 ),
 ( #9575, #63757 ),
 ( #41952, #56650 ),
 ( #72887, #57139 ),
 ( #2991, #10566 ),
 ( #79503, #65739 ),
 ( #11574, #40929 ),
 ( #95715, #26263 ),
 ( #3479, #26757 ),
 ( #19184, #42432 ),
 ( #73366, #3954 ),
 ( #78990, #40439 ),
 ( #13071, #27262 ),
 ( #60122, #28748 ),
 ( #14049, #4447 ),
 ( #36338, #75874 ),
 ( #66256, #97191 ),
 ( #59117, #90090 ),
 ( #27758, #58630 ),
 ( #4965, #20658 ) ),
 .UNSPECIFIED., .T., .F., .F.,
 ( 4, 2, 2, 2, 2, 2, 2, 2, 2, 2, 2, 2, 2, 2, 2, 2, 4 ),
 ( 2, 2 ),
 ( 0.000000000000000000, 0.06250000000000000000, 0.1250000000000000000, 0.1875000000000000000, 0.2500000000000000000, 0.3125000000000000000, 0.3750000000000000000, 0.4375000000000000000, 0.5000000000000000000, 0.5625000000000000000, 0.6250000000000000000, 0.6875000000000000000, 0.7500000000000000000, 0.8125000000000000000, 0.8750000000000000000, 0.9375000000000000000, 1.000000000000000000 ),
 ( 0.000000000000000000, 1.000000000000000000 ),
 .UNSPECIFIED. ) ;
#72402=CARTESIAN_POINT ( 'NONE',  ( 159.2713554375903300, 254.7809155221686410, -15.70062444474382168 ) ) ;
#72405=CARTESIAN_POINT ( 'NONE',  ( 88.29356841273579448, 221.7833772461660544, -9.188101187500095079 ) ) ;
#72406=ORIENTED_EDGE ( 'NONE', *, *, #17188, .T. ) ;
#72409=( BOUNDED_CURVE ( )  B_SPLINE_CURVE ( 2, ( #39270, #78311, #16491, #70180, #40771, #788, #8892, #39761, #70690 ),
 .UNSPECIFIED., .F., .T. ) 
 B_SPLINE_CURVE_WITH_KNOTS ( ( 3, 2, 2, 2, 3 ),
 ( 0.7620967741935483764, 0.7634408602150537515, 0.7661290322580645018, 0.7688172043010752521, 0.7701612903225806273 ),
 .UNSPECIFIED. ) 
 CURVE ( )  GEOMETRIC_REPRESENTATION_ITEM ( )  RATIONAL_B_SPLINE_CURVE ( ( 0.9330127018922194093, 0.9330127018922194093, 1.000000000000000000, 0.8660254037844387076, 1.000000000000000000, 0.8660254037844387076, 1.000000000000000000, 0.9330127018922194093, 0.9330127018922194093 ) ) 
 REPRESENTATION_ITEM ( '' )  );
#72411=CARTESIAN_POINT ( 'NONE',  ( 208.2874212803407090, 269.8825990953837390, -1.143705256421198690 ) ) ;
#72418=CARTESIAN_POINT ( 'NONE',  ( -4.759057006084862707, 161.3927522451417929, -10.00000000000009059 ) ) ;
#72422=CARTESIAN_POINT ( 'NONE',  ( 204.2992694100975939, 276.7902807629455992, 13.99537586056731620 ) ) ;
#72424=CARTESIAN_POINT ( 'NONE',  ( 159.8946522441011382, 253.7013337850969492, -16.68230890105693121 ) ) ;
#72425=CARTESIAN_POINT ( 'NONE',  ( 190.0181636008472594, 270.5760841432478969, 14.27037020729528294 ) ) ;
#72426=FACE_OUTER_BOUND ( 'NONE', #90353, .T. ) ;
#72430=CARTESIAN_POINT ( 'NONE',  ( 202.9431782839550635, 277.8530662632501276, -15.10408699085403583 ) ) ;
#72431=CARTESIAN_POINT ( 'NONE',  ( 200.6097954076514895, 283.1806371883870383, 16.82611162221071766 ) ) ;
#72435=CARTESIAN_POINT ( 'NONE',  ( 178.8030382587059819, 291.7907898142459544, -6.050371113150406543 ) ) ;
#72436=CARTESIAN_POINT ( 'NONE',  ( 202.7185166046502331, 279.5282249361877120, -16.86058306256609640 ) ) ;
#72438=CARTESIAN_POINT ( 'NONE',  ( 165.0387478276132072, 244.7914988754632191, -2.473354058663827626 ) ) ;
#72439=CARTESIAN_POINT ( 'NONE',  ( 180.5277461560353913, 267.1741556918393599, -15.85281502895699290 ) ) ;
#72440=CARTESIAN_POINT ( 'NONE',  ( 182.0920134730108941, 264.0013790589371183, 13.94626246933171210 ) ) ;
#72441=CARTESIAN_POINT ( 'NONE',  ( 199.1791426384580745, 281.7616915630761127, -16.58245314267973214 ) ) ;
#72446=CARTESIAN_POINT ( 'NONE',  ( 158.9658060689105525, 271.8015287571203089, -14.71752948393448435 ) ) ;
#72448=CARTESIAN_POINT ( 'NONE',  ( 21.25804982287034406, 173.8923013555409796, 4.594050593750050204 ) ) ;
#72456=CARTESIAN_POINT ( 'NONE',  ( 28.37526224051742929, 193.3149278399160949, -9.188101187500095079 ) ) ;
#72459=CARTESIAN_POINT ( 'NONE',  ( 161.8289209813647176, 250.3510820566641257, 13.28523796267037937 ) ) ;
#72460=CARTESIAN_POINT ( 'NONE',  ( 190.9559560067148425, 299.9015775189195665, -4.895152914295826108 ) ) ;
#72462=CARTESIAN_POINT ( 'NONE',  ( 199.5639001218976887, 267.6271046904498121, -6.591559436455099785 ) ) ;
#72463=CARTESIAN_POINT ( 'NONE',  ( 146.5865263025993954, 276.7516840693029962, 0.4918294119671828835 ) ) ;
#72464=CARTESIAN_POINT ( 'NONE',  ( 196.8446868189476788, 289.7019965600358091, 16.40794635810030755 ) ) ;
#72465=CARTESIAN_POINT ( 'NONE',  ( 178.9488238674973388, 278.2840548466987798, -16.79158255535696043 ) ) ;
#72470=CARTESIAN_POINT ( 'NONE',  ( 78.90260544222221029, 226.3615022471903160, 5.000000000000046185 ) ) ;
#72473=CARTESIAN_POINT ( 'NONE',  ( 48.45674693441662129, 186.5327760586659451, 1.948934522072303157E-15 ) ) ;
#72478=CARTESIAN_POINT ( 'NONE',  ( 190.2236813008869660, 301.1699145145108218, -5.401374690107298093 ) ) ;
#72482=CARTESIAN_POINT ( 'NONE',  ( 171.2055318311769554, 286.8032793947884329, 8.461617862201846307 ) ) ;
#72483=CARTESIAN_POINT ( 'NONE',  ( 164.5416088356626290, 245.6525688679454618, -1.463507744092769292 ) ) ;
#72484=CARTESIAN_POINT ( 'NONE',  ( 159.6707594272863275, 278.7937339944729160, -10.98969969888871212 ) ) ;
#72485=CARTESIAN_POINT ( 'NONE',  ( 191.0785133773015332, 298.9844436051949401, -7.466887123898782619 ) ) ;
#72487=CARTESIAN_POINT ( 'NONE',  ( 203.0398866899141126, 278.9715956204779559, 16.57839218037009132 ) ) ;
#72488=CARTESIAN_POINT ( 'NONE',  ( 196.3286486926436680, 290.5958008134369948, -16.58330917766970458 ) ) ;
#72489=CARTESIAN_POINT ( 'NONE',  ( 204.6163864379986705, 276.2410179586759682, 14.66911174422491726 ) ) ;
#72494=DIRECTION ( 'NONE',  ( 0.8660254037844395958, 0.4999999999999985567, 0.000000000000000000 ) ) ;
#72495=ORIENTED_EDGE ( 'NONE', *, *, #16299, .F. ) ;
#72497=CARTESIAN_POINT ( 'NONE',  ( 151.3883635558152321, 268.4346579770563608, 15.44343517165679103 ) ) ;
#72498=CARTESIAN_POINT ( 'NONE',  ( 177.4109878776140761, 256.1497104635512869, -7.258573510546487917 ) ) ;
#72501=CARTESIAN_POINT ( 'NONE',  ( 161.8408514536557163, 250.3304178724980318, -14.12919723462510646 ) ) ;
#72503=CARTESIAN_POINT ( 'NONE',  ( 196.4808189786114951, 290.3322341467384717, -17.84817245450773271 ) ) ;
#72509=CARTESIAN_POINT ( 'NONE',  ( 157.1458804504438831, 258.4623461901232417, -17.08829597948888335 ) ) ;
#72510=CARTESIAN_POINT ( 'NONE',  ( 116.3314879560220163, 225.7202760586659167, -5.415160957724236172E-17 ) ) ;
#72511=B_SPLINE_CURVE_WITH_KNOTS ( 'NONE', 3,
 ( #15613, #43657, #30833, #81713 ),
 .UNSPECIFIED., .F., .F.,
 ( 4, 4 ),
 ( 0.005569629907708512073, 0.01055668864777740447 ),
 .UNSPECIFIED. ) ;
#72512=CARTESIAN_POINT ( 'NONE',  ( 184.1644723546534124, 288.8997711373874608, -13.10814152958829482 ) ) ;
#72513=VERTEX_POINT ( 'NONE', #32806 ) ;
#72514=CARTESIAN_POINT ( 'NONE',  ( 163.8947349411736525, 246.7729873192901664, -5.868803394723933309 ) ) ;
#72517=CARTESIAN_POINT ( 'NONE',  ( 197.9598023461055902, 287.7705598106892921, 18.23120408239484291 ) ) ;
#72518=CARTESIAN_POINT ( 'NONE',  ( 204.8580075507323102, 274.8627031754986092, -12.15300732346304358 ) ) ;
#72519=CARTESIAN_POINT ( 'NONE',  ( 64.74867629522887569, 202.0643266524159856, -9.188101187500093303 ) ) ;
#72521=CARTESIAN_POINT ( 'NONE',  ( 151.2455280670316711, 268.6820563007532314, 14.35914944935941229 ) ) ;
#72523=CARTESIAN_POINT ( 'NONE',  ( 147.7840609055601817, 276.6774932931532476, -0.9735537997635442808 ) ) ;
#72524=ORIENTED_EDGE ( 'NONE', *, *, #9111, .F. ) ;
#72526=CARTESIAN_POINT ( 'NONE',  ( 162.9254136962317148, 277.9293967287522946, 13.77390558128574760 ) ) ;
#72529=CARTESIAN_POINT ( 'NONE',  ( 109.6465072765698636, 224.1115022471901739, -5.000000000000041744 ) ) ;
#72530=CARTESIAN_POINT ( 'NONE',  ( 173.9076247008792393, 277.9417859016587045, -16.84130823774900776 ) ) ;
#72531=CARTESIAN_POINT ( 'NONE',  ( 161.1232569692349443, 251.5733279787459367, -14.02750397520710557 ) ) ;
#72534=CARTESIAN_POINT ( 'NONE',  ( 190.2318383114841254, 301.1557861577188078, 3.177919994438449525 ) ) ;
#72538=CARTESIAN_POINT ( 'NONE',  ( 97.33941792859064890, 238.5530062829863027, -4.648177544792955347E-16 ) ) ;
#72540=CARTESIAN_POINT ( 'NONE',  ( 208.3117541397001844, 269.8404533466799080, 2.895672523916592578 ) ) ;
#72542=CARTESIAN_POINT ( 'NONE',  ( 134.0307085979840167, 242.0643266524160140, 9.188101187500095079 ) ) ;
#72545=CARTESIAN_POINT ( 'NONE',  ( 93.04999876614748189, 212.9824982072973683, 3.021315404115420679E-15 ) ) ;
#72547=CARTESIAN_POINT ( 'NONE',  ( 204.6427704787179493, 276.1953194596412118, 13.28850621060895953 ) ) ;
#72549=CARTESIAN_POINT ( 'NONE',  ( 168.6156890688689884, 286.4116463664167895, -8.226575548882113509 ) ) ;
#72553=CARTESIAN_POINT ( 'NONE',  ( 158.4273715006077907, 275.2297750508094509, -12.38274785084877827 ) ) ;
#72554=CARTESIAN_POINT ( 'NONE',  ( 147.7077217681684260, 275.8739656668705038, 2.732453793621575588 ) ) ;
#72557=CARTESIAN_POINT ( 'NONE',  ( 136.8177939967088435, 258.9869531367911009, 4.594050593750046652 ) ) ;
#72561=CARTESIAN_POINT ( 'NONE',  ( 71.83943283659645829, 200.0327760586659451, 1.948934522072303157E-15 ) ) ;
#72562=CARTESIAN_POINT ( 'NONE',  ( 174.2379957965557651, 251.2590728793752248, 3.639292605338433795 ) ) ;
#72564=CARTESIAN_POINT ( 'NONE',  ( 190.7516742497373059, 300.2554039010641418, 4.342609251298632067 ) ) ;
#72565=CARTESIAN_POINT ( 'NONE',  ( 189.3883694580579800, 296.0778630567701839, -11.28578153020828800 ) ) ;
#72566=CARTESIAN_POINT ( 'NONE',  ( 169.2593199950322287, 285.3159198430261654, -8.952739639644439862 ) ) ;
#72567=CARTESIAN_POINT ( 'NONE',  ( 202.8549823380854491, 279.2918593523859272, -16.39745931995414807 ) ) ;
#72570=CARTESIAN_POINT ( 'NONE',  ( 123.7735466722555202, 252.2677522451419065, -5.000000000000047962 ) ) ;
#72573=CARTESIAN_POINT ( 'NONE',  ( 190.4744901378711290, 300.7355008658671522, 0.04566709859947504224 ) ) ;
#72574=CARTESIAN_POINT ( 'NONE',  ( -7.997804718428996651, 172.3149278399160949, -9.188101187500095079 ) ) ;
#72577=CARTESIAN_POINT ( 'NONE',  ( 40.98727782677583065, 182.2202760586659451, -5.415160957724236172E-17 ) ) ;
#72578=CARTESIAN_POINT ( 'NONE',  ( -22.42236680055709641, 157.8615022471902591, 0.000000000000000000 ) ) ;
#72581=CARTESIAN_POINT ( 'NONE',  ( 180.7928668231496658, 266.7588196529836182, -14.70969064882298127 ) ) ;
#72583=CARTESIAN_POINT ( 'NONE',  ( 190.5653282632609091, 300.5781646174276602, -5.775635208185608604 ) ) ;
#72585=CARTESIAN_POINT ( 'NONE',  ( 76.57516216600367898, 205.0177522451417929, 5.000000000000051514 ) ) ;
#72586=CARTESIAN_POINT ( 'NONE',  ( 57.59477206639472513, 197.3927522451418213, -10.00000000000009059 ) ) ;
#72587=CARTESIAN_POINT ( 'NONE',  ( 163.1764708121493470, 256.0176783961395017, -14.93589095490696650 ) ) ;
#72589=ADVANCED_FACE ( 'NONE', ( #72841 ), #78941, .T. ) ;
#72590=CARTESIAN_POINT ( 'NONE',  ( 161.7512311909553375, 267.3476107021334087, 16.49172225746472975 ) ) ;
#72591=CARTESIAN_POINT ( 'NONE',  ( 41.59134429584263870, 201.4865022471903160, 10.00000000000009237 ) ) ;
#72592=DIRECTION ( 'NONE',  ( -0.4999999999999987788, 0.8660254037844392627, 0.000000000000000000 ) ) ;
#72593=CARTESIAN_POINT ( 'NONE',  ( 202.9093905060991005, 279.1976216410395182, 16.97070083370504179 ) ) ;
#72595=CARTESIAN_POINT ( 'NONE',  ( 13.57207436428344316, 169.4548013555409796, -4.594050593750042211 ) ) ;
#72597=CARTESIAN_POINT ( 'NONE',  ( 163.8447499958178355, 252.4744309047850948, 13.22366909537081092 ) ) ;
#72599=CARTESIAN_POINT ( 'NONE',  ( 153.4389798490260262, 264.8828863703868137, 16.68923469758090761 ) ) ;
#72602=AXIS2_PLACEMENT_3D ( 'NONE', #54611, #69827, #8539 ) ;
#72603=CARTESIAN_POINT ( 'NONE',  ( 179.5007171280461478, 277.3276706483341627, 16.42695695674407830 ) ) ;
#72606=( NAMED_UNIT ( * ) PLANE_ANGLE_UNIT ( ) SI_UNIT ( $, .RADIAN. ) );
#72608=CARTESIAN_POINT ( 'NONE',  ( 168.3232405698885259, 288.2092820357482879, 0.5329914561559622177 ) ) ;
#72610=CARTESIAN_POINT ( 'NONE',  ( 207.0929546865518489, 271.9514759237700900, 9.422783993648820910 ) ) ;
#72611=CARTESIAN_POINT ( 'NONE',  ( 154.9683083969241011, 262.2340116239618055, 18.33261662430134109 ) ) ;
#72614=CARTESIAN_POINT ( 'NONE',  ( 206.8791291248445532, 272.3218326606039454, -10.16823074922856840 ) ) ;
#72615=VERTEX_POINT ( 'NONE', #2431 ) ;
#72616=CARTESIAN_POINT ( 'NONE',  ( 153.2964645303881923, 266.7684033456591806, 16.41629521975045236 ) ) ;
#72617=CARTESIAN_POINT ( 'NONE',  ( 164.3774690880109119, 245.9368672504194819, -2.805681983503304000 ) ) ;
#72620=VERTEX_POINT ( 'NONE', #95159 ) ;
#72627=CARTESIAN_POINT ( 'NONE',  ( 178.1953121367105837, 264.0555401404403142, 14.83908789417908913 ) ) ;
#72628=ORIENTED_EDGE ( 'NONE', *, *, #43687, .F. ) ;
#72630=CARTESIAN_POINT ( 'NONE',  ( 161.4397682720950797, 257.0206542164637540, -16.76434429226769041 ) ) ;
#72631=CARTESIAN_POINT ( 'NONE',  ( 149.2923684163597784, 272.0650280510108701, -12.99082738998495756 ) ) ;
#72635=CARTESIAN_POINT ( 'NONE',  ( 161.8873598795597388, 250.2498629158519350, 13.90822209621415873 ) ) ;
#72637=CARTESIAN_POINT ( 'NONE',  ( 150.8555837531579868, 276.0290483310748755, -8.437460036063264113 ) ) ;
#72638=B_SPLINE_SURFACE_WITH_KNOTS ( 'NONE', 3, 1, ( 
 ( #22002, #35712 ),
 ( #58980, #76230 ),
 ( #91440, #14413 ),
 ( #51918, #45296 ),
 ( #68597, #5320 ),
 ( #6805, #28602 ),
 ( #22502, #97539 ),
 ( #44788, #99520 ),
 ( #30104, #28107 ),
 ( #20527, #98532 ),
 ( #75724, #66611 ),
 ( #21036, #51406 ),
 ( #52897, #36197 ),
 ( #37200, #59484 ),
 ( #68102, #29609 ),
 ( #60482, #90466 ),
 ( #60986, #91952 ),
 ( #82369, #12940 ),
 ( #43799, #13429 ),
 ( #59989, #44297 ),
 ( #75226, #36693 ),
 ( #29123, #90959 ),
 ( #21515, #23479 ),
 ( #61973, #45779 ),
 ( #46274, #9302 ),
 ( #77197, #84838 ),
 ( #47288, #94435 ),
 ( #38690, #69595 ),
 ( #40178, #71117 ),
 ( #76701, #31580 ),
 ( #24990, #1718 ),
 ( #8798, #78212 ),
 ( #77720, #22987 ),
 ( #84345, #92440 ) ),
 .UNSPECIFIED., .T., .F., .F.,
 ( 4, 2, 2, 2, 2, 2, 2, 2, 2, 2, 2, 2, 2, 2, 2, 2, 4 ),
 ( 2, 2 ),
 ( 0.000000000000000000, 0.06250000000000000000, 0.1250000000000000000, 0.1875000000000000000, 0.2500000000000000000, 0.3125000000000000000, 0.3750000000000000000, 0.4375000000000000000, 0.5000000000000000000, 0.5625000000000000000, 0.6250000000000000000, 0.6875000000000000000, 0.7500000000000000000, 0.8125000000000000000, 0.8750000000000000000, 0.9375000000000000000, 1.000000000000000000 ),
 ( 0.000000000000000000, 1.000000000000000000 ),
 .UNSPECIFIED. ) ;
#72642=CARTESIAN_POINT ( 'NONE',  ( 171.0368701920845638, 254.8364417340256978, -11.42128868109841378 ) ) ;
#72643=CARTESIAN_POINT ( 'NONE',  ( 202.8167949821795446, 279.3580017930215149, 15.61966256214195070 ) ) ;
#72645=ORIENTED_EDGE ( 'NONE', *, *, #28684, .T. ) ;
#72646=CARTESIAN_POINT ( 'NONE',  ( 156.9842003858142334, 266.1501746981620045, -17.28325484864591743 ) ) ;
#72648=CARTESIAN_POINT ( 'NONE',  ( 160.1176491762495857, 270.3263959031288550, 15.73714383883323720 ) ) ;
#72651=CARTESIAN_POINT ( 'NONE',  ( 167.6595282994673539, 272.2419833626600507, 16.02614727597981670 ) ) ;
#72652=CARTESIAN_POINT ( 'NONE',  ( 194.0765626714293717, 294.4965282251961298, 14.23820788189426167 ) ) ;
#72653=CARTESIAN_POINT ( 'NONE',  ( 177.3343003988342446, 288.7990902974352707, -9.415208683635153619 ) ) ;
#72654=CARTESIAN_POINT ( 'NONE',  ( 161.4250356354754672, 267.9004136800010656, 17.49898951125957680 ) ) ;
#72657=EDGE_CURVE ( 'NONE', #84360, #59501, #85366, .T. ) ;
#72658=CARTESIAN_POINT ( 'NONE',  ( 158.4279782117914124, 256.2416877271991211, -17.37099813172751794 ) ) ;
#72662=CARTESIAN_POINT ( 'NONE',  ( 190.5851083282794320, 298.8997307812002191, -8.167350149732024889 ) ) ;
#72664=ORIENTED_EDGE ( 'NONE', *, *, #58301, .F. ) ;
#72665=ORIENTED_EDGE ( 'NONE', *, *, #87917, .T. ) ;
#72667=CARTESIAN_POINT ( 'NONE',  ( 191.0277618347450073, 299.7772061764919158, 6.528316324927639691 ) ) ;
#72670=CARTESIAN_POINT ( 'NONE',  ( 163.9070886935946874, 247.4979362769680620, 7.364863722913233879 ) ) ;
#72672=CARTESIAN_POINT ( 'NONE',  ( 160.5989244697666720, 252.4814985078845382, -15.88649589014268315 ) ) ;
#72673=CARTESIAN_POINT ( 'NONE',  ( 190.5937363720238977, 300.5289603297032954, -0.9120014529451631047 ) ) ;
#72675=FACE_OUTER_BOUND ( 'NONE', #69074, .T. ) ;
#72678=CARTESIAN_POINT ( 'NONE',  ( 164.2723164851102808, 246.1189969011916503, -1.993789335506892302 ) ) ;
#72679=CARTESIAN_POINT ( 'NONE',  ( 26.41785753015494009, 179.3927522451418213, -10.00000000000009059 ) ) ;
#72680=CARTESIAN_POINT ( 'NONE',  ( 110.8105760068962269, 222.5327760586659451, 1.948934522072302763E-15 ) ) ;
#72682=AXIS2_PLACEMENT_3D ( 'NONE', #71702, #39246, #70156 ) ;
#72684=CARTESIAN_POINT ( 'NONE',  ( 208.0941653616417852, 270.2173281654339689, 1.603026803260118704 ) ) ;
#72686=CARTESIAN_POINT ( 'NONE',  ( 19.39059577201889084, 175.8768266524160140, 9.188101187500098632 ) ) ;
#72687=CARTESIAN_POINT ( 'NONE',  ( 168.1589593212097498, 275.9390298053305628, -16.40258036402506647 ) ) ;
#72688=ORIENTED_EDGE ( 'NONE', *, *, #78282, .F. ) ;
#72690=ORIENTED_EDGE ( 'NONE', *, *, #48483, .T. ) ;
#72691=CARTESIAN_POINT ( 'NONE',  ( 188.2930696087533988, 261.4206402585738829, -5.929984520638014622 ) ) ;
#72695=CARTESIAN_POINT ( 'NONE',  ( 34.30229714732359980, 200.6115022471903160, -5.000000000000047962 ) ) ;
#72700=CARTESIAN_POINT ( 'NONE',  ( 48.29419362332453858, 192.5643266524160140, 9.188101187500095079 ) ) ;
#72701=CARTESIAN_POINT ( 'NONE',  ( 80.97745796857455503, 210.8927522451417929, -10.00000000000009059 ) ) ;
#72704=CARTESIAN_POINT ( 'NONE',  ( 158.4906987444244635, 282.4944243069865593, -1.669741222482398424 ) ) ;
#72705=B_SPLINE_CURVE_WITH_KNOTS ( 'NONE', 3,
 ( #55284, #40084, #40589, #88266, #16802, #17303, #56293, #25402, #63902, #48722, #33514, #48207, #79152, #18815, #64410, #79654, #71028, #34027, #26416, #1630, #11232, #33002, #9734, #62900, #93853, #71528, #9210, #95373, #63406, #2119, #87289, #10218, #47688, #80151, #72021, #56798, #10717, #78624, #41593, #57296, #80654, #42097, #1114, #27415, #5107, #42582, #58293, #50688, #19338, #65403 ),
 .UNSPECIFIED., .F., .F.,
 ( 4, 2, 2, 2, 2, 2, 2, 2, 2, 2, 2, 2, 2, 2, 2, 2, 2, 2, 2, 2, 2, 2, 2, 2, 4 ),
 ( 0.0001966302632834507791, 0.001208579006267713769, 0.001714553377759878887, 0.001967540563505931414, 0.002094034156378898372, 0.002220527749251865763, 0.002347021342124832721, 0.002473514934997800112, 0.002726502120743729256, 0.003232476492235519024, 0.004244425235219099861, 0.005256373978202681131, 0.005762348349694435337, 0.006015335535440235679, 0.006268322721186036887, 0.006331569517622465289, 0.006394816314058895425, 0.006458063110495323826, 0.006521309906931753962, 0.006774297092677275013, 0.007027284278422796064, 0.007280271464168316248, 0.007533258649913837299, 0.007786245835659358350, 0.008292220207150481984 ),
 .UNSPECIFIED. ) ;
#72708=CARTESIAN_POINT ( 'NONE',  ( 9.810363290536042058, 164.2202760586659736, -5.415160957724236172E-17 ) ) ;
#72710=CARTESIAN_POINT ( 'NONE',  ( 150.9115585710837877, 269.2605084359132093, -15.80434701481532578 ) ) ;
#72712=CARTESIAN_POINT ( 'NONE',  ( 147.3236643320416022, 275.4749235501183193, -5.185334239426818037 ) ) ;
#72713=EDGE_CURVE ( 'NONE', #20148, #96454, #63609, .T. ) ;
#72715=CARTESIAN_POINT ( 'NONE',  ( 163.7707306762541748, 246.9877690064858484, 7.021959502997312086 ) ) ;
#72716=CARTESIAN_POINT ( 'NONE',  ( 156.6812872898450735, 261.2670451491295012, 0.000000000000000000 ) ) ;
#72717=CARTESIAN_POINT ( 'NONE',  ( 147.6220714307702622, 274.9580672937808572, 8.392894244419288441 ) ) ;
#72719=CARTESIAN_POINT ( 'NONE',  ( 5.290446120544989306, 163.8615022471902023, 5.000000000000051514 ) ) ;
#72721=CARTESIAN_POINT ( 'NONE',  ( 127.7791744883563183, 235.3923013555409796, 4.594050593750050204 ) ) ;
#72724=ADVANCED_FACE ( 'NONE', ( #97630 ), #55553, .F. ) ;
#72725=DIRECTION ( 'NONE',  ( -0.4999999999999987788, 0.8660254037844392627, 0.000000000000000000 ) ) ;
#72726=CARTESIAN_POINT ( 'NONE',  ( 196.2255671652529259, 290.7743432561995860, 16.01325193769018185 ) ) ;
#72728=CARTESIAN_POINT ( 'NONE',  ( 190.8671785295675818, 300.0553446199063501, -7.998068249277817898 ) ) ;
#72730=CARTESIAN_POINT ( 'NONE',  ( 190.8264243556038195, 300.1259329198319961, 8.466983560044813117 ) ) ;
#72731=CARTESIAN_POINT ( 'NONE',  ( 149.5796913320911870, 271.5673701627850960, -12.80793412251569841 ) ) ;
#72733=CARTESIAN_POINT ( 'NONE',  ( 176.1322591638738118, 292.6111088397734648, -1.129813806047020863 ) ) ;
#72737=CARTESIAN_POINT ( 'NONE',  ( 176.2784824380131568, 278.9230878378185139, 15.47631285694224701 ) ) ;
#72738=CARTESIAN_POINT ( 'NONE',  ( 165.6403964848181829, 269.1609729818266032, -16.85820533882582595 ) ) ;
#72739=B_SPLINE_CURVE_WITH_KNOTS ( 'NONE', 3,
 ( #11043, #71848, #18640, #94662, #25743, #40900, #41410, #41920, #96662, #2446, #25220, #72856, #95687, #71342, #34325, #33326, #42403, #65222, #3925, #56623, #18132, #96165, #26726, #40409, #64736, #79967, #88589, #50024, #56107, #10535, #34807, #72355, #65709, #80979, #87095, #11545, #86583, #2959, #33851, #51008, #21140, #81959 ),
 .UNSPECIFIED., .F., .F.,
 ( 4, 2, 2, 2, 2, 2, 2, 2, 2, 2, 2, 2, 2, 2, 2, 2, 2, 2, 2, 2, 4 ),
 ( 0.003028838789308639992, 0.003226312173560616243, 0.003423785557812592060, 0.003522522249938576499, 0.003621258942064560938, 0.003719995634190545377, 0.003818732326316529382, 0.004016205710568453158, 0.004213679094820376933, 0.004608625863324152493, 0.005398519400331704479, 0.006188412937339255598, 0.007768200011354287580, 0.007866936703480216508, 0.007965673395606144569, 0.008015041741669108599, 0.008064410087732072629, 0.008163146779858087426, 0.008558093548362137939, 0.008953040316866188453, 0.009347987085370238966 ),
 .UNSPECIFIED. ) ;
#72741=EDGE_CURVE ( 'NONE', #48389, #21055, #40408, .T. ) ;
#72745=CARTESIAN_POINT ( 'NONE',  ( 148.0620100209659427, 274.6244786578839694, 6.173810397789149640 ) ) ;
#72746=DIRECTION ( 'NONE',  ( -0.8660254037844387076, -0.4999999999999998890, -0.000000000000000000 ) ) ;
#72748=CARTESIAN_POINT ( 'NONE',  ( 191.8314558436726145, 287.9551196214300148, -15.85916516023665856 ) ) ;
#72750=CARTESIAN_POINT ( 'NONE',  ( 163.8647661177941757, 279.6316184227941903, 12.38387626794212970 ) ) ;
#72751=CARTESIAN_POINT ( 'NONE',  ( 148.4042165687623083, 273.6033521758856750, -8.709765892313745539 ) ) ;
#72753=ORIENTED_EDGE ( 'NONE', *, *, #57438, .F. ) ;
#72756=CARTESIAN_POINT ( 'NONE',  ( 190.5217943342473745, 281.4870030958396683, 17.81127109971334121 ) ) ;
#72760=DIRECTION ( 'NONE',  ( -0.8660254037844387076, -0.4999999999999998890, -0.000000000000000000 ) ) ;
#72761=CARTESIAN_POINT ( 'NONE',  ( 155.6569868912636991, 261.0411854816857158, -17.75433477650897984 ) ) ;
#72765=CARTESIAN_POINT ( 'NONE',  ( 177.2385493374541454, 260.3943833094866136, 12.25215814848759699 ) ) ;
#72766=ORIENTED_EDGE ( 'NONE', *, *, #72741, .F. ) ;
#72768=ORIENTED_EDGE ( 'NONE', *, *, #95250, .T. ) ;
#72771=CARTESIAN_POINT ( 'NONE',  ( 203.0498946958275326, 278.9542612457532869, -15.11479947333269003 ) ) ;
#72776=CARTESIAN_POINT ( 'NONE',  ( 161.0515428782683500, 277.3244187559503189, -13.42420650014866368 ) ) ;
#72777=CARTESIAN_POINT ( 'NONE',  ( 147.5851099763508216, 275.0220864107570264, -4.372720440640867956 ) ) ;
#72778=CARTESIAN_POINT ( 'NONE',  ( 152.7691010214056462, 266.0431505347400503, -16.40662330462167162 ) ) ;
#72782=CARTESIAN_POINT ( 'NONE',  ( 143.4758849319492526, 244.4548013555409796, -4.594050593750042211 ) ) ;
#72784=ORIENTED_EDGE ( 'NONE', *, *, #21470, .T. ) ;
#72787=ADVANCED_FACE ( 'NONE', ( #30698 ), #76315, .T. ) ;
#72788=CARTESIAN_POINT ( 'NONE',  ( 200.2245315327614605, 270.3076691078479712, 9.266824258444575690 ) ) ;
#72789=ORIENTED_EDGE ( 'NONE', *, *, #2894, .T. ) ;
#72791=CARTESIAN_POINT ( 'NONE',  ( -0.7717317059461257234, 170.3615022471902591, -10.00000000000009592 ) ) ;
#72792=CARTESIAN_POINT ( 'NONE',  ( 162.6774150396764469, 248.8814472377480911, 10.88033986792731689 ) ) ;
#72793=CARTESIAN_POINT ( 'NONE',  ( 172.9698904924519240, 250.6642211707864476, -4.168778760986519671 ) ) ;
#72794=CARTESIAN_POINT ( 'NONE',  ( 146.6863996654837763, 276.5786983304647606, 3.619532364376333078 ) ) ;
#72797=CARTESIAN_POINT ( 'NONE',  ( 171.0847150063659683, 280.7602631364448484, 13.96071002983590859 ) ) ;
#72799=CARTESIAN_POINT ( 'NONE',  ( 177.2731322035851349, 256.0571359664338047, -8.025376214617153892 ) ) ;
#72805=CARTESIAN_POINT ( 'NONE',  ( 202.1068129883413746, 268.3794028533957317, -2.863715232315004133 ) ) ;
#72806=CARTESIAN_POINT ( 'NONE',  ( 152.4183529982803407, 266.6506639314469567, -16.73371844995563862 ) ) ;
#72807=CARTESIAN_POINT ( 'NONE',  ( 148.9232972370683399, 272.7042780851529642, 12.27045554427055940 ) ) ;
#72808=CARTESIAN_POINT ( 'NONE',  ( 202.4943568615953779, 279.9164810001701085, 17.09064351659286984 ) ) ;
#72809=CARTESIAN_POINT ( 'NONE',  ( 157.8667100161213739, 273.7629819761619956, 14.59697424305941382 ) ) ;
#72810=CARTESIAN_POINT ( 'NONE',  ( 151.3683638516007477, 275.1446189862357414, -9.648240976932610735 ) ) ;
#72812=ORIENTED_EDGE ( 'NONE', *, *, #27535, .T. ) ;
#72814=CARTESIAN_POINT ( 'NONE',  ( 190.2326078713353752, 273.4588640468538188, -15.98580255482095325 ) ) ;
#72815=CARTESIAN_POINT ( 'NONE',  ( 200.0313018224816801, 276.5939864008022369, 15.71640468486303099 ) ) ;
#72816=CARTESIAN_POINT ( 'NONE',  ( -6.583630525541995127, 178.5530062829863027, -4.648177544792955347E-16 ) ) ;
#72818=CARTESIAN_POINT ( 'NONE',  ( 52.05581792490468729, 190.8615022471902023, 5.000000000000051514 ) ) ;
#72819=CARTESIAN_POINT ( 'NONE',  ( 163.0171530587457767, 248.2930037274571191, 9.677214176418313940 ) ) ;
#72820=CARTESIAN_POINT ( 'NONE',  ( 10.86574497745707646, 167.8923013555410080, 4.594050593750050204 ) ) ;
#72821=CARTESIAN_POINT ( 'NONE',  ( 104.5854977735480560, 237.3149278399160664, 9.188101187500093303 ) ) ;
#72822=CARTESIAN_POINT ( 'NONE',  ( 89.31526421587503251, 210.8262482093457777, 3.021315404115420679E-15 ) ) ;
#72823=CARTESIAN_POINT ( 'NONE',  ( 186.7545291922311890, 295.9253793373928261, -7.587588941354818317 ) ) ;
#72827=CARTESIAN_POINT ( 'NONE',  ( 160.4265347487137205, 282.4329614563485507, 5.107902280202428535 ) ) ;
#72828=CARTESIAN_POINT ( 'NONE',  ( 189.5113466251651744, 300.6005995191865736, -1.615647776261078583 ) ) ;
#72829=CARTESIAN_POINT ( 'NONE',  ( 177.9124682818391250, 290.1927361200270070, 9.830732425089301785 ) ) ;
#72832=CARTESIAN_POINT ( 'NONE',  ( 185.6713631041849055, 258.9584525764907426, -6.747383155299178092 ) ) ;
#72836=CARTESIAN_POINT ( 'NONE',  ( 80.49933977867583224, 217.2833772461660544, -9.188101187500095079 ) ) ;
#72837=CARTESIAN_POINT ( 'NONE',  ( 161.6923300915171922, 250.5876644177310482, -14.43081872899884566 ) ) ;
#72841=FACE_OUTER_BOUND ( 'NONE', #42550, .T. ) ;
#72843=CARTESIAN_POINT ( 'NONE',  ( 173.2279903352282986, 268.2393894133472827, -16.29216417966541641 ) ) ;
#72846=CARTESIAN_POINT ( 'NONE',  ( 136.1966614240191689, 237.8932355074535678, -2.679491924311248496 ) ) ;
#72849=CARTESIAN_POINT ( 'NONE',  ( 75.49289073487081225, 205.2048013555409796, 4.594050593750051981 ) ) ;
#72850=CARTESIAN_POINT ( 'NONE',  ( 169.4774712875160390, 288.1570225834816483, -1.094182444139154775 ) ) ;
#72851=CARTESIAN_POINT ( 'NONE',  ( 147.2658550951450422, 275.5750520855697800, -5.215660180131691526 ) ) ;
#72852=CARTESIAN_POINT ( 'NONE',  ( 153.4767009694824367, 264.8175514732376996, 16.67166765953223617 ) ) ;
#72856=CARTESIAN_POINT ( 'NONE',  ( 189.8520780095588805, 286.5250076688263334, 16.49189287256407610 ) ) ;
#72859=CARTESIAN_POINT ( 'NONE',  ( 125.2349645446896886, 253.1115022471903160, -5.000000000000047962 ) ) ;
#72860=CARTESIAN_POINT ( 'NONE',  ( 157.1269483542914998, 258.4951375425532092, -17.15328932028234377 ) ) ;
#72862=ORIENTED_EDGE ( 'NONE', *, *, #34805, .T. ) ;
#72863=CARTESIAN_POINT ( 'NONE',  ( 165.7251599921764864, 247.0382640774007541, -1.865539601759665933 ) ) ;
#72864=VERTEX_POINT ( 'NONE', #8887 ) ;
#72865=CARTESIAN_POINT ( 'NONE',  ( 162.7644741734472120, 248.7306563947940958, 9.865755277559742353 ) ) ;
#72866=DIRECTION ( 'NONE',  ( -0.8660254037844387076, -0.4999999999999998890, -0.000000000000000000 ) ) ;
#72868=VERTEX_POINT ( 'NONE', #85960 ) ;
#72871=CARTESIAN_POINT ( 'NONE',  ( 192.8220505326807199, 292.3911712377218350, 15.11976871725602933 ) ) ;
#72872=CYLINDRICAL_SURFACE ( 'NONE', #8707, 5.000000000000058620 ) ;
#72874=CARTESIAN_POINT ( 'NONE',  ( 191.6148588865760871, 296.7603242537468873, -11.89382487812838995 ) ) ;
#72876=CARTESIAN_POINT ( 'NONE',  ( 102.2852913444020686, 239.8615022471903160, 5.000000000000046185 ) ) ;
#72879=CARTESIAN_POINT ( 'NONE',  ( 158.4316519640294132, 269.2869727094641235, -16.76269917448883717 ) ) ;
#72880=CARTESIAN_POINT ( 'NONE',  ( 44.12520995882072583, 207.8297689869269220, -2.679491924311252493 ) ) ;
#72881=ORIENTED_EDGE ( 'NONE', *, *, #37382, .F. ) ;
#72882=ORIENTED_EDGE ( 'NONE', *, *, #99831, .T. ) ;
#72883=CARTESIAN_POINT ( 'NONE',  ( 183.4103682618680295, 295.6271469934868605, 7.008542154348483599 ) ) ;
#72884=B_SPLINE_CURVE_WITH_KNOTS ( 'NONE', 3,
 ( #72526, #31985, #47681, #32993 ),
 .UNSPECIFIED., .F., .F.,
 ( 4, 4 ),
 ( 0.01401801354063230039, 0.02268410888174763121 ),
 .UNSPECIFIED. ) ;
#72885=EDGE_CURVE ( 'NONE', #33130, #56117, #8003, .T. ) ;
#72886=CARTESIAN_POINT ( 'NONE',  ( 163.9587364689194260, 246.6621334214722481, 5.816126667419880825 ) ) ;
#72887=CARTESIAN_POINT ( 'NONE',  ( 194.7900911235093133, 293.2606606935473792, -14.66228443412922999 ) ) ;
#72889=DIRECTION ( 'NONE',  ( -0.8660254037844359321, -0.5000000000000051070, -0.000000000000000000 ) ) ;
#72890=CARTESIAN_POINT ( 'NONE',  ( 131.9051165326627881, 235.4155109091896065, 2.679491924311254714 ) ) ;
#72892=CARTESIAN_POINT ( 'NONE',  ( 164.7632660535861930, 245.2686473046373692, 4.980011448959140274 ) ) ;
#72894=CARTESIAN_POINT ( 'NONE',  ( 169.7896959808458632, 267.4449072945214994, 17.07133255476025724 ) ) ;
#72896=EDGE_CURVE ( 'NONE', #46298, #85762, #32284, .T. ) ;
#72897=CARTESIAN_POINT ( 'NONE',  ( 110.8105760068962127, 222.5327760586659736, 1.948934522072303157E-15 ) ) ;
#72900=CARTESIAN_POINT ( 'NONE',  ( 166.2473226288001626, 277.8849993475402016, -13.37946549092444393 ) ) ;
#72903=CARTESIAN_POINT ( 'NONE',  ( 189.3775153017087973, 300.6355170167246911, -1.634152055493470757 ) ) ;
#72904=ADVANCED_FACE ( 'NONE', ( #16486 ), #9486, .F. ) ;
#72907=CARTESIAN_POINT ( 'NONE',  ( 206.1062572280473546, 273.6604860535989587, -9.773577984388410300 ) ) ;
#72908=CARTESIAN_POINT ( 'NONE',  ( 163.1685298068643988, 248.0308115086310465, 10.61953511350444046 ) ) ;
#72909=CARTESIAN_POINT ( 'NONE',  ( 100.2557178503908517, 222.5643266524160140, 9.188101187500095079 ) ) ;
#72910=ORIENTED_EDGE ( 'NONE', *, *, #62157, .T. ) ;
#72911=AXIS2_PLACEMENT_3D ( 'NONE', #66414, #97341, #58788 ) ;
#72913=DIRECTION ( 'NONE',  ( -0.8660254037844387076, -0.4999999999999998890, -0.000000000000000000 ) ) ;
#72916=CARTESIAN_POINT ( 'NONE',  ( 153.7130981888246026, 265.1850621614574948, 16.50407132121065246 ) ) ;
#72918=CARTESIAN_POINT ( 'NONE',  ( 143.0428722300570143, 244.2048013555409511, 4.594050593750051981 ) ) ;
#72919=CARTESIAN_POINT ( 'NONE',  ( -22.42236680055709641, 157.8615022471902591, 0.000000000000000000 ) ) ;
#72920=CARTESIAN_POINT ( 'NONE',  ( -11.83159780365783398, 170.6427522451419065, 10.00000000000009237 ) ) ;
#72922=ORIENTED_EDGE ( 'NONE', *, *, #88565, .F. ) ;
#72923=CARTESIAN_POINT ( 'NONE',  ( 157.0150015346687553, 258.6890351218854676, 16.85538724311808068 ) ) ;
#72925=B_SPLINE_CURVE_WITH_KNOTS ( 'NONE', 3,
 ( #87307, #95878, #47705, #78643, #9226, #9751, #10235, #25942, #70517, #32531, #72039, #41610, #64934, #40610, #71544, #62919, #63919, #94858, #2643, #17840, #40105, #18341, #49235, #80169, #33021, #10737, #71045, #8725, #1647, #63425, #94364, #33531, #3159, #86785, #55792, #39596, #48224, #2138, #25418, #64428, #95390, #34044, #26436, #57315, #32009, #93869, #24426, #55302 ),
 .UNSPECIFIED., .F., .F.,
 ( 4, 2, 2, 2, 2, 2, 2, 2, 2, 2, 2, 2, 2, 2, 2, 2, 2, 2, 2, 2, 2, 2, 2, 4 ),
 ( 0.0002174362994174117863, 0.001238585736266362711, 0.001749160454690868328, 0.002004447813903081996, 0.002132091493509117273, 0.002259735173115152550, 0.002387378852721187394, 0.002515022532327222671, 0.002770309891539291490, 0.003280884609963429562, 0.004302034046811783335, 0.005323183483660138410, 0.005833758202084277783, 0.006089045561296346602, 0.006344332920508415422, 0.006408154760311396414, 0.006471976600114376539, 0.006535798439917356664, 0.006599620279720337657, 0.006854907638932357904, 0.007365482357356391459, 0.007620769716568408236, 0.007876057075780427616, 0.008386631794204362292 ),
 .UNSPECIFIED. ) ;
#72927=CARTESIAN_POINT ( 'NONE',  ( 188.8786019601460282, 269.6712879289298144, 14.62574647380142778 ) ) ;
#72928=CARTESIAN_POINT ( 'NONE',  ( -22.42236680055709641, 157.8615022471902591, 0.000000000000000000 ) ) ;
#72930=FACE_OUTER_BOUND ( 'NONE', #54852, .T. ) ;
#72932=CARTESIAN_POINT ( 'NONE',  ( 153.5324998095718456, 266.8834243315761796, 16.61741842784684664 ) ) ;
#72934=CARTESIAN_POINT ( 'NONE',  ( 206.8106726053982811, 272.4404028303941914, -10.47827087991598560 ) ) ;
#72936=CARTESIAN_POINT ( 'NONE',  ( 175.0025046748339435, 290.6155586575834491, -6.507390672453347236 ) ) ;
#72938=CARTESIAN_POINT ( 'NONE',  ( -17.42236680055705023, 149.2012482093457777, 0.000000000000000000 ) ) ;
#72939=CARTESIAN_POINT ( 'NONE',  ( 207.6508796976096107, 270.9851214578045528, 6.713685698622268383 ) ) ;
#72941=CARTESIAN_POINT ( 'NONE',  ( 69.64695893572810803, 221.0177522451419065, 5.000000000000046185 ) ) ;
#72943=CARTESIAN_POINT ( 'NONE',  ( -22.42236680055709641, 157.8615022471902591, 0.000000000000000000 ) ) ;
#72944=FACE_OUTER_BOUND ( 'NONE', #50825, .T. ) ;
#72946=CARTESIAN_POINT ( 'NONE',  ( 160.9223551016720251, 273.3990656506861683, -15.46406356478478195 ) ) ;
#72948=CARTESIAN_POINT ( 'NONE',  ( 161.1492466472929266, 251.5283125358769212, -13.33353587056634915 ) ) ;
#72949=CARTESIAN_POINT ( 'NONE',  ( 23.85612603422365297, 175.3923013555409796, 4.594050593750050204 ) ) ;
#72954=CARTESIAN_POINT ( 'NONE',  ( 207.8302079587528794, 270.6745157982714431, 3.572475529330238153 ) ) ;
#72956=CARTESIAN_POINT ( 'NONE',  ( 36.52174756457106497, 182.7048013555409796, 4.594050593750051981 ) ) ;
#72957=CARTESIAN_POINT ( 'NONE',  ( 200.6097954076514895, 283.1806371883870383, 16.82611162221071766 ) ) ;
#72958=CARTESIAN_POINT ( 'NONE',  ( 147.2494378675467033, 275.6034875578896504, 3.639370109197119341 ) ) ;
#72960=CARTESIAN_POINT ( 'NONE',  ( 181.7502401732105000, 294.1801057147719121, 6.322034055514200723 ) ) ;
#72961=CARTESIAN_POINT ( 'NONE',  ( 146.6834825911944620, 276.5837508513432681, 0.6716460511724984261 ) ) ;
#72962=CARTESIAN_POINT ( 'NONE',  ( 178.7151539974932462, 270.9650308319119176, 17.63195993801104677 ) ) ;
#72964=CARTESIAN_POINT ( 'NONE',  ( 84.34903687182406884, 231.0530062829863027, -4.648177544792955347E-16 ) ) ;
#72969=CARTESIAN_POINT ( 'NONE',  ( 89.36707907128422335, 215.7365022471902023, 10.00000000000009592 ) ) ;
#72970=CARTESIAN_POINT ( 'NONE',  ( 13.51768745649711789, 178.6115022471902591, 10.00000000000009592 ) ) ;
#72971=CARTESIAN_POINT ( 'NONE',  ( 53.16558651961199899, 195.3768266524160140, 9.188101187500098632 ) ) ;
#72972=ORIENTED_EDGE ( 'NONE', *, *, #41389, .F. ) ;
#72974=CARTESIAN_POINT ( 'NONE',  ( 190.1858949294064871, 301.2353624297489887, -5.249932979468886707 ) ) ;
#72977=CARTESIAN_POINT ( 'NONE',  ( 167.4464793182998221, 285.4026007275220422, 7.926851182865696899 ) ) ;
#72979=LINE ( 'NONE', #42045, #65540 ) ;
#72981=CARTESIAN_POINT ( 'NONE',  ( 189.1222366604172294, 265.5048954663608924, 10.64636282005728596 ) ) ;
#72983=CARTESIAN_POINT ( 'NONE',  ( 171.3148662694858331, 255.7789367394895237, 12.02744102109133628 ) ) ;
#72986=CARTESIAN_POINT ( 'NONE',  ( 198.7634891777862549, 264.9856665559012185, 0.1351954043397823324 ) ) ;
#72987=CARTESIAN_POINT ( 'NONE',  ( 172.2873880799365338, 253.3886587257176473, 8.406275390072382336 ) ) ;
#72988=DIRECTION ( 'NONE',  ( -0.8660254037844387076, -0.4999999999999998890, -0.000000000000000000 ) ) ;
#72991=CARTESIAN_POINT ( 'NONE',  ( 151.4025156491502742, 268.4101458323662541, 14.71049357081981235 ) ) ;
#72994=ORIENTED_EDGE ( 'NONE', *, *, #43447, .F. ) ;
#72996=EDGE_CURVE ( 'NONE', #60981, #59884, #22523, .T. ) ;
#72997=CARTESIAN_POINT ( 'NONE',  ( 161.8750289368003621, 250.2712207352165592, -13.97436367953006098 ) ) ;
#72998=CARTESIAN_POINT ( 'NONE',  ( -22.42236680055709641, 157.8615022471902591, 0.000000000000000000 ) ) ;
#72999=CARTESIAN_POINT ( 'NONE',  ( 184.1482295286804458, 294.7143494075100421, -9.263004813192097231 ) ) ;
#73002=CARTESIAN_POINT ( 'NONE',  ( 197.9952413503812352, 287.7091776547143809, 17.17611241386010690 ) ) ;
#73006=CARTESIAN_POINT ( 'NONE',  ( 157.4805323096970255, 257.8827121670497036, -16.70238855805511591 ) ) ;
#73007=CARTESIAN_POINT ( 'NONE',  ( 121.9063529450018279, 235.0643266524160424, -9.188101187500093303 ) ) ;
#73008=CARTESIAN_POINT ( 'NONE',  ( 74.41009865654258704, 203.7677522451417929, -5.000000000000041744 ) ) ;
#73009=CARTESIAN_POINT ( 'NONE',  ( 207.5230514910949182, 271.2065264061283756, 2.678931747975364708 ) ) ;
#73014=CARTESIAN_POINT ( 'NONE',  ( 71.13526655237410523, 218.0024278399160664, 9.188101187500095079 ) ) ;
#73016=CARTESIAN_POINT ( 'NONE',  ( 150.6790040019602088, 269.6633047651677089, 15.38315204620803378 ) ) ;
#73017=CARTESIAN_POINT ( 'NONE',  ( 198.7606870255174272, 286.3833868549447743, 17.68329551240030284 ) ) ;
#73018=CARTESIAN_POINT ( 'NONE',  ( 175.5753062590537752, 278.4498914399613909, 15.48226569750622694 ) ) ;
#73019=VERTEX_POINT ( 'NONE', #73206 ) ;
#73023=VERTEX_POINT ( 'NONE', #34681 ) ;
#73024=CARTESIAN_POINT ( 'NONE',  ( 148.6879145481387638, 273.1119728616009752, 9.952982990420577991 ) ) ;
#73026=CARTESIAN_POINT ( 'NONE',  ( 161.8750289368003621, 250.2712207352165592, -13.97436367953006098 ) ) ;
#73028=CARTESIAN_POINT ( 'NONE',  ( 190.0445576990143195, 301.4801656937889902, 4.140328216824785912 ) ) ;
#73030=CARTESIAN_POINT ( 'NONE',  ( 206.0041637419966776, 273.8373171585603814, 11.66586596407113596 ) ) ;
#73031=CARTESIAN_POINT ( 'NONE',  ( 206.4695239676918845, 273.0312896038346366, 10.41704154450801667 ) ) ;
#73032=CARTESIAN_POINT ( 'NONE',  ( 125.8022308496927195, 254.9860189848785410, -2.679491924311252493 ) ) ;
#73033=CARTESIAN_POINT ( 'NONE',  ( 166.9567796355807729, 256.1732514150568818, 13.73539047231146171 ) ) ;
#73034=ORIENTED_EDGE ( 'NONE', *, *, #60928, .T. ) ;
#73035=CARTESIAN_POINT ( 'NONE',  ( 164.2647213391612979, 246.1321520798662164, -5.830872732487307530 ) ) ;
#73036=CARTESIAN_POINT ( 'NONE',  ( 128.2121871902485566, 235.6423013555409796, -4.594050593750043987 ) ) ;
#73037=ORIENTED_EDGE ( 'NONE', *, *, #43432, .F. ) ;
#73038=CARTESIAN_POINT ( 'NONE',  ( 146.5689048584090699, 276.7822053059436485, -0.4306668706573002492 ) ) ;
#73039=CARTESIAN_POINT ( 'NONE',  ( 90.50373741020339935, 216.3927522451418213, 10.00000000000009948 ) ) ;
#73040=CARTESIAN_POINT ( 'NONE',  ( 205.3549208985294001, 273.3626630250829521, -10.87845838788729758 ) ) ;
#73041=CARTESIAN_POINT ( 'NONE',  ( 164.2297246530060875, 246.1927681183832988, 5.803160395959773510 ) ) ;
#73043=CARTESIAN_POINT ( 'NONE',  ( 175.7520323455595417, 252.2218298946914388, 4.007223628156822315 ) ) ;
#73044=VERTEX_POINT ( 'NONE', #43769 ) ;
#73047=DIRECTION ( 'NONE',  ( -0.8660254037844387076, -0.4999999999999998890, -0.000000000000000000 ) ) ;
#73049=CARTESIAN_POINT ( 'NONE',  ( 164.9590787296926067, 244.9294898008548387, -2.278052160087662870 ) ) ;
#73050=CARTESIAN_POINT ( 'NONE',  ( 138.6312950077063135, 250.8458772461660260, 9.188101187500095079 ) ) ;
#73051=CARTESIAN_POINT ( 'NONE',  ( 184.9432817549989352, 285.0648861408565722, 16.61117941084251726 ) ) ;
#73053=CARTESIAN_POINT ( 'NONE',  ( 170.9566650728496882, 250.6362774811119891, 3.411191216732029297 ) ) ;
#73055=CARTESIAN_POINT ( 'NONE',  ( 149.4539134692060145, 271.7852238117696402, 12.95627816374690688 ) ) ;
#73058=CARTESIAN_POINT ( 'NONE',  ( 171.9374462982776492, 287.8333287246510963, -8.532231483866285160 ) ) ;
#73059=CARTESIAN_POINT ( 'NONE',  ( 159.3291946290163992, 279.0199804063916531, 10.96233109238993109 ) ) ;
#73060=CARTESIAN_POINT ( 'NONE',  ( 193.6579322423270355, 288.5700127970677045, 16.06830834735240643 ) ) ;
#73061=CARTESIAN_POINT ( 'NONE',  ( 128.9696990949622091, 245.2677522451418497, 10.00000000000009592 ) ) ;
#73064=CARTESIAN_POINT ( 'NONE',  ( 196.4677418905696129, 290.3548843276421394, 17.08610552292358520 ) ) ;
#73065=CARTESIAN_POINT ( 'NONE',  ( 148.3997536239841679, 273.6110822229926498, 8.713694244701960301 ) ) ;
#73066=CARTESIAN_POINT ( 'NONE',  ( -3.992090130160959482, 162.3768266524160140, 9.188101187500096856 ) ) ;
#73067=CARTESIAN_POINT ( 'NONE',  ( 43.09804120061789945, 189.5643266524160140, 9.188101187500095079 ) ) ;
#73068=CARTESIAN_POINT ( 'NONE',  ( 178.5061629747377765, 273.6775914088984223, -17.34296752049866086 ) ) ;
#73071=CARTESIAN_POINT ( 'NONE',  ( 157.0877926458200307, 258.5629572190321710, -17.40668770468195703 ) ) ;
#73073=CARTESIAN_POINT ( 'NONE',  ( 190.1813752874636805, 301.2431906792259042, -4.710625539811892359 ) ) ;
#73075=CARTESIAN_POINT ( 'NONE',  ( 168.1589593212097498, 275.9390298053305628, -16.40258036402506647 ) ) ;
#73076=CARTESIAN_POINT ( 'NONE',  ( 61.41971759977597145, 206.2677522451418781, 10.00000000000009592 ) ) ;
#73078=CARTESIAN_POINT ( 'NONE',  ( 204.7764732025852084, 275.9637395487929439, -14.02287343454361412 ) ) ;
#73079=CARTESIAN_POINT ( 'NONE',  ( 169.3846196238007735, 270.7800964535849744, -17.72459440982018108 ) ) ;
#73081=B_SPLINE_CURVE_WITH_KNOTS ( 'NONE', 3,
 ( #76422, #6511, #68293, #92635 ),
 .UNSPECIFIED., .F., .F.,
 ( 4, 4 ),
 ( 0.02105975151895524838, 0.02524676605399324425 ),
 .UNSPECIFIED. ) ;
#73082=EDGE_CURVE ( 'NONE', #99484, #17163, #12980, .T. ) ;
#73083=CARTESIAN_POINT ( 'NONE',  ( 179.7192414948235069, 294.1200435161542828, 1.033553133877518126 ) ) ;
#73084=CARTESIAN_POINT ( 'NONE',  ( 47.29267820409023670, 198.1115022471902591, 10.00000000000009592 ) ) ;
#73085=CARTESIAN_POINT ( 'NONE',  ( 184.9287284004330729, 293.9407481508790170, 9.651135569905934020 ) ) ;
#73086=CARTESIAN_POINT ( 'NONE',  ( 203.0398866899141126, 278.9715956204779559, 16.57839218037009132 ) ) ;
#73087=CARTESIAN_POINT ( 'NONE',  ( 6.887527552763561545, 162.5327760586659736, 1.948934522072303157E-15 ) ) ;
#73089=FACE_OUTER_BOUND ( 'NONE', #80378, .T. ) ;
#73091=CARTESIAN_POINT ( 'NONE',  ( 153.1745822862813498, 265.3408363824576668, 16.18092354043443493 ) ) ;
#73093=CARTESIAN_POINT ( 'NONE',  ( 84.11911179316838627, 207.8262482093457777, 3.021315404115420679E-15 ) ) ;
#73094=B_SPLINE_CURVE_WITH_KNOTS ( 'NONE', 3,
 ( #86367, #56400, #87395, #1215 ),
 .UNSPECIFIED., .F., .F.,
 ( 4, 4 ),
 ( 0.02632407315735414005, 0.03555975659152819934 ),
 .UNSPECIFIED. ) ;
#73095=CARTESIAN_POINT ( 'NONE',  ( 182.0984742165180705, 278.2391700500209026, 16.50274708701968862 ) ) ;
#73098=CARTESIAN_POINT ( 'NONE',  ( 176.6391464052069296, 260.6212487597024392, -13.24495383745690447 ) ) ;
#73101=CARTESIAN_POINT ( 'NONE',  ( 126.7089641099561845, 232.4155109091895781, 2.679491924311254714 ) ) ;
#73104=CARTESIAN_POINT ( 'NONE',  ( 189.5534384022301424, 269.0062095459838929, -14.92796778812864922 ) ) ;
#73106=CARTESIAN_POINT ( 'NONE',  ( 156.7117516780912183, 276.4586797656536419, 10.26618125257395242 ) ) ;
#73109=CARTESIAN_POINT ( 'NONE',  ( 152.7153488183568300, 266.1362520814392951, 17.33540622643059237 ) ) ;
#73110=CARTESIAN_POINT ( 'NONE',  ( 206.9059968923335475, 272.2752963222270068, 6.902135944297345560 ) ) ;
#73115=VERTEX_POINT ( 'NONE', #37657 ) ;
#73116=CARTESIAN_POINT ( 'NONE',  ( 159.7424789065890991, 278.4861631006231732, -9.771801590140540839 ) ) ;
#73121=CARTESIAN_POINT ( 'NONE',  ( 174.3220357038730128, 262.5849746787575327, 15.23774525505547395 ) ) ;
#73125=CARTESIAN_POINT ( 'NONE',  ( 196.9319848161575806, 289.5507919934690335, -17.64330560362266453 ) ) ;
#73126=CARTESIAN_POINT ( 'NONE',  ( 42.00631479827483616, 188.3927522451417929, -10.00000000000009237 ) ) ;
#73128=CARTESIAN_POINT ( 'NONE',  ( 200.7079229450794173, 283.0106753079404029, 16.90512463913211505 ) ) ;
#73129=CARTESIAN_POINT ( 'NONE',  ( 169.5268067963925205, 276.4064337483826534, -15.74407357586045464 ) ) ;
#73132=CARTESIAN_POINT ( 'NONE',  ( 174.6031362836316703, 276.7578777746297760, -16.67970167110237512 ) ) ;
#73133=CARTESIAN_POINT ( 'NONE',  ( 163.3854574543125580, 247.6550818016845597, 10.82482370245618775 ) ) ;
#73135=DIRECTION ( 'NONE',  ( -0.8660254037844387076, -0.4999999999999998890, -0.000000000000000000 ) ) ;
#73137=FACE_OUTER_BOUND ( 'NONE', #25772, .T. ) ;
#73138=ORIENTED_EDGE ( 'NONE', *, *, #11169, .F. ) ;
#73139=CARTESIAN_POINT ( 'NONE',  ( 147.9079810727873223, 274.4628572674334919, 6.305649893024213526 ) ) ;
#73140=CARTESIAN_POINT ( 'NONE',  ( 178.6359132194422727, 289.6913899023020917, -9.365969567067413237 ) ) ;
#73141=CARTESIAN_POINT ( 'NONE',  ( 192.5455529438217468, 269.1281655793299592, -13.93448690431165105 ) ) ;
#73142=CARTESIAN_POINT ( 'NONE',  ( 192.6030823458456780, 295.3171989905301871, 13.41425101105791384 ) ) ;
#73144=CARTESIAN_POINT ( 'NONE',  ( 197.2708468743591652, 288.9638656919068467, -16.67412905307064008 ) ) ;
#73146=ORIENTED_EDGE ( 'NONE', *, *, #87559, .T. ) ;
#73150=AXIS2_PLACEMENT_3D ( 'NONE', #62457, #75339, #23465 ) ;
#73153=CARTESIAN_POINT ( 'NONE',  ( 159.7897726928491409, 253.8829904965402875, 16.83923858130328810 ) ) ;
#73156=CARTESIAN_POINT ( 'NONE',  ( 147.1020895757533538, 275.8587022856839326, -2.572889012152433708 ) ) ;
#73159=CARTESIAN_POINT ( 'NONE',  ( 126.8249895137406043, 232.4824982072973683, 3.021315404115420679E-15 ) ) ;
#73161=CARTESIAN_POINT ( 'NONE',  ( 160.4075704321521130, 252.8129334232662586, -14.67865048504329906 ) ) ;
#73162=CARTESIAN_POINT ( 'NONE',  ( 148.5298631380253767, 273.3857259341252757, -8.957191713326388083 ) ) ;
#73164=DIRECTION ( 'NONE',  ( -0.8660254037844387076, -0.4999999999999998890, -0.000000000000000000 ) ) ;
#73166=CARTESIAN_POINT ( 'NONE',  ( 133.7328388157766312, 238.0177522451417929, 5.000000000000051514 ) ) ;
#73167=CARTESIAN_POINT ( 'NONE',  ( 164.8670003495851404, 245.0889742334797177, -1.557028074864921674 ) ) ;
#73169=CARTESIAN_POINT ( 'NONE',  ( 32.84087927488944558, 199.7677522451419350, -5.000000000000047962 ) ) ;
#73170=CARTESIAN_POINT ( 'NONE',  ( 99.66015183740654493, 228.3458772461660544, 9.188101187500095079 ) ) ;
#73171=CARTESIAN_POINT ( 'NONE',  ( 183.4553195968295256, 297.0403188216897661, -2.838562726794640056 ) ) ;
#73173=CARTESIAN_POINT ( 'NONE',  ( 163.8070446421170629, 255.0663642890118581, -15.42060242571707818 ) ) ;
#73174=CARTESIAN_POINT ( 'NONE',  ( 18.76822678699008051, 172.4548013555409796, -4.594050593750042211 ) ) ;
#73175=CARTESIAN_POINT ( 'NONE',  ( 171.9930234791391399, 277.2658286946252701, -16.71261851089754558 ) ) ;
#73176=ORIENTED_EDGE ( 'NONE', *, *, #24680, .F. ) ;
#73178=CARTESIAN_POINT ( 'NONE',  ( 185.3117431063705283, 259.6004929598439048, -5.362663101281642142 ) ) ;
#73180=CARTESIAN_POINT ( 'NONE',  ( 193.0451532016805913, 263.6626746619177766, -3.983151606634049990 ) ) ;
#73181=CARTESIAN_POINT ( 'NONE',  ( 161.1750406344237661, 251.4836360396366501, -14.21198410781773802 ) ) ;
#73182=DIRECTION ( 'NONE',  ( -0.8660254037844387076, -0.4999999999999998890, -0.000000000000000000 ) ) ;
#73183=CARTESIAN_POINT ( 'NONE',  ( 167.9816492369689911, 251.8180079618673233, 10.45878825870253159 ) ) ;
#73184=CARTESIAN_POINT ( 'NONE',  ( 39.09232661234986494, 199.5024278399160949, -9.188101187500093303 ) ) ;
#73185=CARTESIAN_POINT ( 'NONE',  ( 97.79278455872243114, 217.2677522451417644, -5.000000000000041744 ) ) ;
#73188=CARTESIAN_POINT ( 'NONE',  ( -6.807019788225388446, 173.0024278399160949, 9.188101187500095079 ) ) ;
#73190=CARTESIAN_POINT ( 'NONE',  ( 150.6626254231123880, 269.6916732958875969, -15.32062296289003811 ) ) ;
#73192=CARTESIAN_POINT ( 'NONE',  ( 192.4259603496955719, 297.3554553095298729, -12.40738485318142814 ) ) ;
#73195=CARTESIAN_POINT ( 'NONE',  ( 203.7159275419774360, 276.2629543621159769, 13.33400116652491718 ) ) ;
#73196=CARTESIAN_POINT ( 'NONE',  ( 78.80693396667733452, 204.7592609112379876, 2.679491924311254714 ) ) ;
#73197=CARTESIAN_POINT ( 'NONE',  ( 164.2600772519394923, 246.1401958748887182, -2.110785484364219311 ) ) ;
#73199=CARTESIAN_POINT ( 'NONE',  ( 1.826344505407192287, 171.8615022471902591, -10.00000000000009592 ) ) ;
#73201=CARTESIAN_POINT ( 'NONE',  ( 115.3025621453804490, 243.5024278399160949, 9.188101187500095079 ) ) ;
#73205=CARTESIAN_POINT ( 'NONE',  ( 151.1161590537679444, 269.2899787152654767, 13.95646909953505599 ) ) ;
#73206=CARTESIAN_POINT ( 'NONE',  ( 165.4473470637335879, 246.0837842385732301, 3.196113342258863899 ) ) ;
#73207=DIRECTION ( 'NONE',  ( -0.8660254037844387076, -0.4999999999999998890, -0.000000000000000000 ) ) ;
#73209=EDGE_LOOP ( 'NONE', ( #44291, #88016, #53376, #86535 ) ) ;
#73210=CARTESIAN_POINT ( 'NONE',  ( 150.6487462746963502, 269.7157126861102370, 15.18501655901553704 ) ) ;
#73211=CARTESIAN_POINT ( 'NONE',  ( 196.6317700900902139, 290.0707791521982131, -17.91116578096951883 ) ) ;
#73213=CARTESIAN_POINT ( 'NONE',  ( 203.9436454561111134, 276.7717721749480688, 13.76990199114231572 ) ) ;
#73215=ORIENTED_EDGE ( 'NONE', *, *, #76767, .T. ) ;
#73216=CARTESIAN_POINT ( 'NONE',  ( 189.3176312642889627, 265.7376729923254857, 10.75542669776848470 ) ) ;
#73218=CARTESIAN_POINT ( 'NONE',  ( 165.4318461280464874, 269.5429478206821159, -16.34563326180095189 ) ) ;
#73219=B_SPLINE_SURFACE_WITH_KNOTS ( 'NONE', 3, 1, ( 
 ( #79316, #48875 ),
 ( #16454, #85930 ),
 ( #55432, #40741 ),
 ( #87448, #63557 ),
 ( #95527, #25055 ),
 ( #86927, #70655 ),
 ( #87934, #49363 ),
 ( #17981, #33159 ),
 ( #1267, #71686 ),
 ( #26072, #64064 ),
 ( #32151, #94001 ),
 ( #79809, #10374 ),
 ( #3289, #72182 ),
 ( #56948, #18477 ),
 ( #80307, #54951 ),
 ( #63059, #41751 ),
 ( #62538, #93497 ),
 ( #24056, #11878 ),
 ( #49857, #89417 ),
 ( #75172, #57448 ),
 ( #97967, #42734 ),
 ( #57954, #73181 ),
 ( #73671, #82310 ),
 ( #11392, #19970 ),
 ( #4252, #42245 ),
 ( #97483, #81307 ),
 ( #50847, #20470 ),
 ( #88427, #18987 ),
 ( #96503, #81796 ),
 ( #28543, #34655 ),
 ( #12882, #35655 ),
 ( #35151, #20978 ),
 ( #51861, #43739 ),
 ( #74684, #28048 ) ),
 .UNSPECIFIED., .T., .F., .F.,
 ( 4, 2, 2, 2, 2, 2, 2, 2, 2, 2, 2, 2, 2, 2, 2, 2, 4 ),
 ( 2, 2 ),
 ( 0.000000000000000000, 0.06250000000000000000, 0.1250000000000000000, 0.1875000000000000000, 0.2500000000000000000, 0.3125000000000000000, 0.3750000000000000000, 0.4375000000000000000, 0.5000000000000000000, 0.5625000000000000000, 0.6250000000000000000, 0.6875000000000000000, 0.7500000000000000000, 0.8125000000000000000, 0.8750000000000000000, 0.9375000000000000000, 1.000000000000000000 ),
 ( 0.000000000000000000, 1.000000000000000000 ),
 .UNSPECIFIED. ) ;
#73222=CARTESIAN_POINT ( 'NONE',  ( 29.78943643340442549, 199.5530062829863027, -4.648177544792955347E-16 ) ) ;
#73224=CARTESIAN_POINT ( 'NONE',  ( 153.2712411579340426, 265.1734183057532732, 16.26687330118495467 ) ) ;
#73226=CARTESIAN_POINT ( 'NONE',  ( 194.5520723251022162, 283.0158833145478070, 17.60059791576126997 ) ) ;
#73228=CARTESIAN_POINT ( 'NONE',  ( 173.9008529106967558, 272.4049662731551962, -17.79092985220220058 ) ) ;
#73230=CARTESIAN_POINT ( 'NONE',  ( 167.8099530253072089, 271.3928698661641761, -17.53051755021046532 ) ) ;
#73232=CARTESIAN_POINT ( 'NONE',  ( 159.7188570120185034, 264.1459342443484957, -17.63143322946013214 ) ) ;
#73235=CARTESIAN_POINT ( 'NONE',  ( 185.3856663186220715, 291.1121785684215411, 12.07308616320444017 ) ) ;
#73237=ORIENTED_EDGE ( 'NONE', *, *, #46220, .F. ) ;
#73240=FACE_OUTER_BOUND ( 'NONE', #26103, .T. ) ;
#73243=CARTESIAN_POINT ( 'NONE',  ( 177.6456495537226772, 260.6504471429459500, 12.23025887897517983 ) ) ;
#73245=CARTESIAN_POINT ( 'NONE',  ( 173.9582802083413640, 250.9521034096781023, -3.022749797112575632 ) ) ;
#73248=CARTESIAN_POINT ( 'NONE',  ( 154.9048824156581361, 262.3438686460345366, -17.40627786727128168 ) ) ;
#73252=CARTESIAN_POINT ( 'NONE',  ( 163.0037873698800581, 255.9019164637528831, -14.93970584870495699 ) ) ;
#73253=CARTESIAN_POINT ( 'NONE',  ( 158.6202604900994686, 274.9997957384633764, -12.56136378133423470 ) ) ;
#73254=CARTESIAN_POINT ( 'NONE',  ( 152.7295469705997277, 266.1116601603806657, -17.40211458100010589 ) ) ;
#73257=CARTESIAN_POINT ( 'NONE',  ( 146.6963301283313967, 249.3768266524160140, 9.188101187500098632 ) ) ;
#73261=EDGE_CURVE ( 'NONE', #20256, #88849, #50335, .T. ) ;
#73265=CARTESIAN_POINT ( 'NONE',  ( 181.3414764931898162, 255.3117459804828400, 0.6552448166232091031 ) ) ;
#73267=CARTESIAN_POINT ( 'NONE',  ( 121.1754704609021900, 250.7677522451419065, -5.000000000000047962 ) ) ;
#73268=CARTESIAN_POINT ( 'NONE',  ( 153.1667354219324011, 277.1489508030442153, 6.793483612096318680 ) ) ;
#73270=CARTESIAN_POINT ( 'NONE',  ( 192.6772867332300621, 292.3908774927655259, -14.35745613815102928 ) ) ;
#73273=( BOUNDED_CURVE ( )  B_SPLINE_CURVE ( 2, ( #38677, #75712, #52885, #7283, #29597, #14879, #91938, #13896, #76216 ),
 .UNSPECIFIED., .F., .T. ) 
 B_SPLINE_CURVE_WITH_KNOTS ( ( 3, 2, 2, 2, 3 ),
 ( 0.6572580645161290036, 0.6586021505376343788, 0.6612903225806451291, 0.6639784946236558794, 0.6653225806451612545 ),
 .UNSPECIFIED. ) 
 CURVE ( )  GEOMETRIC_REPRESENTATION_ITEM ( )  RATIONAL_B_SPLINE_CURVE ( ( 0.9330127018922194093, 0.9330127018922194093, 1.000000000000000000, 0.8660254037844387076, 1.000000000000000000, 0.8660254037844387076, 1.000000000000000000, 0.9330127018922194093, 0.9330127018922194093 ) ) 
 REPRESENTATION_ITEM ( '' )  );
#73275=CARTESIAN_POINT ( 'NONE',  ( 184.9711235847237276, 272.9950566324947658, -17.00090985181319780 ) ) ;
#73280=CARTESIAN_POINT ( 'NONE',  ( 156.2648642422210514, 277.5543309471286193, 10.15725722932580410 ) ) ;
#73283=CARTESIAN_POINT ( 'NONE',  ( 202.9685995779611858, 279.0950685203052899, 16.84977534244423580 ) ) ;
#73285=CARTESIAN_POINT ( 'NONE',  ( 168.9285091408607684, 266.8905904589466900, 17.77692745299157195 ) ) ;
#73287=CARTESIAN_POINT ( 'NONE',  ( 200.3681102454790448, 268.1092862786254614, 6.092393729374322220 ) ) ;
#73288=ORIENTED_EDGE ( 'NONE', *, *, #25233, .T. ) ;
#73290=CARTESIAN_POINT ( 'NONE',  ( 117.8737486125219505, 248.8615022471903160, 5.000000000000046185 ) ) ;
#73291=AXIS2_PLACEMENT_3D ( 'NONE', #75972, #90697, #52131 ) ;
#73298=B_SPLINE_CURVE_WITH_KNOTS ( 'NONE', 3,
 ( #20987, #60935, #75181, #45245, #14359, #53346, #51870, #13376, #77145, #13856, #15327, #37634, #52347, #83795, #7242, #5753 ),
 .UNSPECIFIED., .F., .F.,
 ( 4, 2, 2, 2, 2, 2, 2, 4 ),
 ( 0.000000000000000000, 0.0003786681000626840776, 0.0007573362001253681553, 0.001136004300188052070, 0.001514672400250736311, 0.001893340500313420334, 0.002272008600376104141, 0.003029344800501419278 ),
 .UNSPECIFIED. ) ;
#73299=CARTESIAN_POINT ( 'NONE',  ( -2.098180203030011182, 181.8464784336661637, 1.353441290958777525E-15 ) ) ;
#73300=CARTESIAN_POINT ( 'NONE',  ( 108.7534185771431510, 233.5958772461660260, -9.188101187500095079 ) ) ;
#73301=CARTESIAN_POINT ( 'NONE',  ( 202.7602807045765019, 279.4558873931827065, -15.90558713185497020 ) ) ;
#73302=CARTESIAN_POINT ( 'NONE',  ( 192.4259603496955719, 297.3554553095298729, -12.40738485318142814 ) ) ;
#73303=CARTESIAN_POINT ( 'NONE',  ( 180.2803958731623197, 254.8946283151103955, -2.457077073020527358 ) ) ;
#73304=CARTESIAN_POINT ( 'NONE',  ( -1.617403181491035902, 158.3262482093458061, 3.021315404115420679E-15 ) ) ;
#73307=CARTESIAN_POINT ( 'NONE',  ( 160.8174585145418405, 281.7671747025778473, 5.344995675835433779 ) ) ;
#73308=CARTESIAN_POINT ( 'NONE',  ( 194.8432095198904221, 293.1686569321988145, -14.74101036184996616 ) ) ;
#73310=CARTESIAN_POINT ( 'NONE',  ( 182.7847760313759409, 280.0284915794045446, -17.53211380394024843 ) ) ;
#73314=EDGE_CURVE ( 'NONE', #8304, #87111, #49090, .T. ) ;
#73315=CARTESIAN_POINT ( 'NONE',  ( 172.5878269333680350, 263.4941563848159944, -15.40501487940348646 ) ) ;
#73316=CARTESIAN_POINT ( 'NONE',  ( 89.86341300497758766, 216.5643266524160140, 9.188101187500095079 ) ) ;
#73318=CARTESIAN_POINT ( 'NONE',  ( 161.2977680094314223, 251.2710659906439616, -13.03191437619249982 ) ) ;
#73319=CYLINDRICAL_SURFACE ( 'NONE', #41140, 10.00000000000010658 ) ;
#73321=CARTESIAN_POINT ( 'NONE',  ( 163.2942584940569191, 258.1478583562382028, 16.77787020301746779 ) ) ;
#73322=CARTESIAN_POINT ( 'NONE',  ( 157.0957870390718369, 258.5491105237443321, 17.69218919045495397 ) ) ;
#73324=CARTESIAN_POINT ( 'NONE',  ( 199.2299651681423143, 285.5705732690366858, -17.65328173313980642 ) ) ;
#73325=CARTESIAN_POINT ( 'NONE',  ( 173.1817746140479244, 268.1958027911921363, -16.29107544405880859 ) ) ;
#73326=EDGE_CURVE ( 'NONE', #68451, #13298, #62322, .T. ) ;
#73330=VERTEX_POINT ( 'NONE', #37693 ) ;
#73332=CARTESIAN_POINT ( 'NONE',  ( 74.03095222233704931, 222.7369531367911293, -4.594050593750048428 ) ) ;
#73333=CARTESIAN_POINT ( 'NONE',  ( 172.7158920701056957, 289.4533927640794673, -1.057531439601499201 ) ) ;
#73335=CARTESIAN_POINT ( 'NONE',  ( 188.3784916956350344, 286.3721210266486992, -16.81851773412965301 ) ) ;
#73336=ADVANCED_FACE ( 'NONE', ( #28113 ), #53074, .F. ) ;
#73340=CARTESIAN_POINT ( 'NONE',  ( 124.0080952226617796, 235.7365022471902023, -10.00000000000009059 ) ) ;
#73341=CARTESIAN_POINT ( 'NONE',  ( 157.8043799545718286, 257.3217915922150496, -17.97575562758749257 ) ) ;
#73343=ORIENTED_EDGE ( 'NONE', *, *, #68249, .F. ) ;
#73345=ORIENTED_EDGE ( 'NONE', *, *, #32416, .T. ) ;
#73346=CARTESIAN_POINT ( 'NONE',  ( 163.3706531435203146, 247.6807236201477735, 10.06957846017757241 ) ) ;
#73350=ORIENTED_EDGE ( 'NONE', *, *, #63690, .F. ) ;
#73351=CARTESIAN_POINT ( 'NONE',  ( 188.8058653551997566, 290.9426387842769373, 14.85089295608895021 ) ) ;
#73352=CARTESIAN_POINT ( 'NONE',  ( 158.4819084462915839, 256.1482778209808089, 16.21549387834203415 ) ) ;
#73359=AXIS2_PLACEMENT_3D ( 'NONE', #81207, #49762, #11291 ) ;
#73360=CARTESIAN_POINT ( 'NONE',  ( 164.0781508658037637, 275.4055464209769752, 15.63836535835214114 ) ) ;
#73362=VERTEX_POINT ( 'NONE', #15383 ) ;
#73364=CARTESIAN_POINT ( 'NONE',  ( 186.9477914209481355, 275.4121812026439216, 17.59542901063888820 ) ) ;
#73365=CARTESIAN_POINT ( 'NONE',  ( 204.6427704787179493, 276.1953194596412118, 13.28850621060895953 ) ) ;
#73366=CARTESIAN_POINT ( 'NONE',  ( 194.3011251241114508, 294.1075746476782342, -14.76047579547631905 ) ) ;
#73372=CARTESIAN_POINT ( 'NONE',  ( 207.4535553197589763, 271.3268973058138158, -4.905507205346139266 ) ) ;
#73373=CARTESIAN_POINT ( 'NONE',  ( 169.1799572416250612, 267.0414233079974338, 17.70411709586223736 ) ) ;
#73375=CARTESIAN_POINT ( 'NONE',  ( 178.5561507476227234, 255.7288023451889671, 4.885752237254268771 ) ) ;
#73376=CARTESIAN_POINT ( 'NONE',  ( 95.24857461505581568, 234.9869531367911293, 4.594050593750046652 ) ) ;
#73380=CARTESIAN_POINT ( 'NONE',  ( 166.8352072885147948, 278.2578104396429808, -13.33477771316318261 ) ) ;
#73381=ORIENTED_EDGE ( 'NONE', *, *, #546, .F. ) ;
#73384=DIRECTION ( 'NONE',  ( 0.4999999999999998890, -0.8660254037844385966, 0.000000000000000000 ) ) ;
#73385=CARTESIAN_POINT ( 'NONE',  ( 163.6378993367609382, 249.6457029564056711, 10.23770952667803691 ) ) ;
#73388=CARTESIAN_POINT ( 'NONE',  ( 95.57333414147498729, 235.1744531367911293, 4.594050593750047540 ) ) ;
#73390=ORIENTED_EDGE ( 'NONE', *, *, #39206, .T. ) ;
#73392=CARTESIAN_POINT ( 'NONE',  ( 208.3194307158603067, 269.8271571267425770, -2.120200867047394855 ) ) ;
#73393=ORIENTED_EDGE ( 'NONE', *, *, #62419, .T. ) ;
#73394=ADVANCED_FACE ( 'NONE', ( #30612 ), #93609, .F. ) ;
#73395=CARTESIAN_POINT ( 'NONE',  ( 191.6165807384784046, 263.6474570320527278, -8.167173469078569781 ) ) ;
#73396=CARTESIAN_POINT ( 'NONE',  ( 153.2087289474062572, 265.9906550880538134, 16.15720884485870812 ) ) ;
#73398=CARTESIAN_POINT ( 'NONE',  ( 135.6816562978893330, 239.9548013555409796, -4.594050593750042211 ) ) ;
#73400=CARTESIAN_POINT ( 'NONE',  ( -11.32641631811688221, 164.2677522451418781, 10.00000000000009592 ) ) ;
#73401=DIRECTION ( 'NONE',  ( -0.8660254037844392627, -0.4999999999999987232, 0.000000000000000000 ) ) ;
#73403=CARTESIAN_POINT ( 'NONE',  ( 204.9604304439480416, 275.6451162603322587, 13.28912526856024279 ) ) ;
#73404=B_SPLINE_CURVE_WITH_KNOTS ( 'NONE', 3,
 ( #36583, #35097, #42685, #20418, #5204, #43690, #74630, #67488, #12828, #20926, #66006, #51285, #82254, #89367, #36085, #59882, #12317, #50300, #82751, #73616, #66988, #19921, #21402, #19443, #51808, #97914, #35602, #81252, #80768, #11826, #28489, #59370, #90849, #13318, #96957, #27522, #98418, #44179, #75117, #5693, #11340, #29011, #42197, #73132, #27996, #3725, #34604, #43180 ),
 .UNSPECIFIED., .F., .F.,
 ( 4, 2, 2, 2, 2, 2, 2, 2, 2, 2, 2, 2, 2, 2, 2, 2, 2, 2, 2, 2, 2, 2, 2, 4 ),
 ( 0.0001333623287611991604, 0.001159685769147140652, 0.001672847489340077232, 0.001801137919388335175, 0.001929428349436593118, 0.002057718779484850845, 0.002186009209533108788, 0.002442590069629720084, 0.002699170929726331814, 0.003212332649919709231, 0.004238656090306530851, 0.005264979530693353338, 0.005778141250886801444, 0.006034722110983567998, 0.006291302971080335420, 0.006355448186104469162, 0.006419593401128602037, 0.006547883831177029983, 0.006804464691273848578, 0.007061045551370668041, 0.007317626411467486637, 0.007574207271564305233, 0.007830788131661124696, 0.008343949851854678620 ),
 .UNSPECIFIED. ) ;
#73406=CARTESIAN_POINT ( 'NONE',  ( 206.5237403681858552, 272.9373840435757188, -10.81420335655575116 ) ) ;
#73411=EDGE_CURVE ( 'NONE', #41871, #6045, #28542, .T. ) ;
#73415=CARTESIAN_POINT ( 'NONE',  ( 159.8732321751776624, 253.7384344327741132, -15.51998349828054202 ) ) ;
#73417=CARTESIAN_POINT ( 'NONE',  ( 208.1912724900461740, 270.0491336852600170, -0.9856800448607289100 ) ) ;
#73418=LINE ( 'NONE', #34405, #62460 ) ;
#73422=CARTESIAN_POINT ( 'NONE',  ( 185.2786651606941746, 266.4582656545080681, 13.16981717527268536 ) ) ;
#73423=CARTESIAN_POINT ( 'NONE',  ( 168.2694307985145770, 247.7137964094873439, -3.237542012886357234 ) ) ;
#73429=EDGE_CURVE ( 'NONE', #79972, #19414, #84221, .T. ) ;
#73430=CARTESIAN_POINT ( 'NONE',  ( 22.04262502322622908, 183.5333772461660544, 9.188101187500095079 ) ) ;
#73432=CARTESIAN_POINT ( 'NONE',  ( 207.3442821610807414, 271.1161826646066970, 2.723480558286873521 ) ) ;
#73433=ORIENTED_EDGE ( 'NONE', *, *, #16335, .T. ) ;
#73436=EDGE_CURVE ( 'NONE', #29477, #52312, #4758, .T. ) ;
#73438=DIRECTION ( 'NONE',  ( -0.8660254037844387076, -0.4999999999999998890, -0.000000000000000000 ) ) ;
#73440=CARTESIAN_POINT ( 'NONE',  ( 39.90439897628026955, 193.8458772461660544, 9.188101187500095079 ) ) ;
#73441=CARTESIAN_POINT ( 'NONE',  ( 161.5431944097339851, 250.8459749958011287, 14.52339846942414603 ) ) ;
#73442=CARTESIAN_POINT ( 'NONE',  ( 190.4976253092930278, 300.6954295735222900, -5.764807383508308902 ) ) ;
#73444=CARTESIAN_POINT ( 'NONE',  ( 178.5414132024961873, 291.6442548996461710, 6.015133232593436574 ) ) ;
#73445=CARTESIAN_POINT ( 'NONE',  ( 178.8763131426492521, 293.7076375770308800, 2.674743856691759181 ) ) ;
#73446=CARTESIAN_POINT ( 'NONE',  ( 179.0083614005145307, 278.2908046544912395, -16.68097254531133800 ) ) ;
#73448=B_SPLINE_SURFACE_WITH_KNOTS ( 'NONE', 3, 1, ( 
 ( #46380, #91541 ),
 ( #69197, #22106 ),
 ( #30710, #61590 ),
 ( #92541, #53002 ),
 ( #62080, #31189 ),
 ( #38791, #29222 ),
 ( #69697, #48280 ),
 ( #60089, #76802 ),
 ( #23088, #44893 ),
 ( #45397, #6902 ),
 ( #53980, #93027 ),
 ( #36802, #54475 ),
 ( #23583, #84938 ),
 ( #37300, #302 ),
 ( #17373, #85453 ),
 ( #37791, #91052 ),
 ( #21619, #52499 ),
 ( #53494, #83447 ),
 ( #14015, #68692 ),
 ( #7395, #92060 ),
 ( #75834, #30204 ),
 ( #61090, #84446 ),
 ( #14991, #45878 ),
 ( #57362, #35058 ),
 ( #3689, #94912 ),
 ( #56860, #49282 ),
 ( #42161, #87847 ),
 ( #64479, #95925 ),
 ( #25474, #65469 ),
 ( #49772, #65965 ),
 ( #58354, #81217 ),
 ( #88841, #10284 ),
 ( #79226, #80218 ),
 ( #89332, #33584 ) ),
 .UNSPECIFIED., .T., .F., .F.,
 ( 4, 2, 2, 2, 2, 2, 2, 2, 2, 2, 2, 2, 2, 2, 2, 2, 4 ),
 ( 2, 2 ),
 ( 0.000000000000000000, 0.06250000000000000000, 0.1250000000000000000, 0.1875000000000000000, 0.2500000000000000000, 0.3125000000000000000, 0.3750000000000000000, 0.4375000000000000000, 0.5000000000000000000, 0.5625000000000000000, 0.6250000000000000000, 0.6875000000000000000, 0.7500000000000000000, 0.8125000000000000000, 0.8750000000000000000, 0.9375000000000000000, 1.000000000000000000 ),
 ( 0.000000000000000000, 1.000000000000000000 ),
 .UNSPECIFIED. ) ;
#73449=EDGE_CURVE ( 'NONE', #38805, #30217, #24952, .T. ) ;
#73452=CARTESIAN_POINT ( 'NONE',  ( 72.04657099559535993, 225.7365022471903160, 2.944929066748280225E-16 ) ) ;
#73453=CARTESIAN_POINT ( 'NONE',  ( 16.62094515339138212, 173.7365022471902307, 10.00000000000009948 ) ) ;
#73456=CARTESIAN_POINT ( 'NONE',  ( 36.54820344085055694, 204.1589784336661637, -6.496448406907675876E-16 ) ) ;
#73458=CARTESIAN_POINT ( 'NONE',  ( 162.5280598625341497, 263.2215374870250457, 17.43915653070007110 ) ) ;
#73459=CARTESIAN_POINT ( 'NONE',  ( 190.6954410837624607, 300.3528026016029457, -5.728531842148099962 ) ) ;
#73461=EDGE_LOOP ( 'NONE', ( #27402, #11102, #69890, #8467, #57099 ) ) ;
#73462=CARTESIAN_POINT ( 'NONE',  ( 170.9080147460631736, 286.3543506222695783, 7.469236110414841256 ) ) ;
#73463=CARTESIAN_POINT ( 'NONE',  ( 164.4781197247689306, 245.7625352337404649, -1.511762618280499515 ) ) ;
#73466=CARTESIAN_POINT ( 'NONE',  ( 188.7940803133921577, 265.4288857401144810, 10.73849653901970491 ) ) ;
#73468=CARTESIAN_POINT ( 'NONE',  ( 171.2975384787696100, 255.8152646582991849, 11.65888598572620438 ) ) ;
#73472=CARTESIAN_POINT ( 'NONE',  ( 174.5500181047472381, 255.0162374629895226, 8.241104149140888069 ) ) ;
#73480=CARTESIAN_POINT ( 'NONE',  ( 161.0965315767822972, 251.6196177163260188, -13.76772246540905442 ) ) ;
#73489=CARTESIAN_POINT ( 'NONE',  ( 157.8043799545718286, 257.3217915922150496, -17.97575562758749257 ) ) ;
#73490=CARTESIAN_POINT ( 'NONE',  ( 106.6423081075360670, 238.5024278399160949, -9.188101187500093303 ) ) ;
#73491=CARTESIAN_POINT ( 'NONE',  ( 112.2445834879231086, 235.6115022471902307, 10.00000000000009592 ) ) ;
#73493=B_SPLINE_CURVE_WITH_KNOTS ( 'NONE', 3,
 ( #24069, #46870, #272, #86435 ),
 .UNSPECIFIED., .F., .F.,
 ( 4, 4 ),
 ( 0.01007082774348767168, 0.01841198851506076553 ),
 .UNSPECIFIED. ) ;
#73494=CARTESIAN_POINT ( 'NONE',  ( 163.9910908123517288, 246.6060940548019289, -7.333295033952830444 ) ) ;
#73497=CARTESIAN_POINT ( 'NONE',  ( 159.7953104873542145, 253.8733987550956783, 15.41928249285404107 ) ) ;
#73498=CARTESIAN_POINT ( 'NONE',  ( 165.2351475709818089, 262.2120121923977649, 17.49020206947767875 ) ) ;
#73499=CARTESIAN_POINT ( 'NONE',  ( 69.94482871793549350, 205.0643266524159856, -9.188101187500093303 ) ) ;
#73500=CARTESIAN_POINT ( 'NONE',  ( 19.85049821812290816, 182.2677522451418497, 10.00000000000009592 ) ) ;
#73501=CARTESIAN_POINT ( 'NONE',  ( 142.6123662252853421, 259.5780487066560340, -7.305945665944390655 ) ) ;
#73503=CARTESIAN_POINT ( 'NONE',  ( 175.1717403937841198, 278.2705980278694256, 15.46858508767819629 ) ) ;
#73509=CARTESIAN_POINT ( 'NONE',  ( 147.9505753669699857, 274.3890817857965772, 9.316607266155644496 ) ) ;
#73511=CARTESIAN_POINT ( 'NONE',  ( 163.5290595954285777, 260.2326466906550877, -16.19227360478010169 ) ) ;
#73512=CARTESIAN_POINT ( 'NONE',  ( 85.25577013208754806, 208.4824982072973967, 3.021315404115420679E-15 ) ) ;
#73514=EDGE_CURVE ( 'NONE', #16265, #78871, #47914, .T. ) ;
#73516=CARTESIAN_POINT ( 'NONE',  ( 205.7867067512454184, 274.2139637150027056, 10.62737868262404106 ) ) ;
#73517=CARTESIAN_POINT ( 'NONE',  ( 164.5813345449211624, 245.5837619211427523, 1.447064457712487373 ) ) ;
#73519=CARTESIAN_POINT ( 'NONE',  ( 164.1634658209742952, 254.0895655750726689, 14.32597737159830409 ) ) ;
#73520=CARTESIAN_POINT ( 'NONE',  ( 164.4414259850711915, 245.8260906552167171, -6.983224448873608381 ) ) ;
#73521=CARTESIAN_POINT ( 'NONE',  ( 124.1521724663614492, 251.6744531367911577, 4.594050593750047540 ) ) ;
#73523=CARTESIAN_POINT ( 'NONE',  ( 146.5046981847821428, 276.8934145268504494, 0.02269072295920678689 ) ) ;
#73525=CARTESIAN_POINT ( 'NONE',  ( 199.2985792285494995, 282.8172808829962150, -17.62369519561723408 ) ) ;
#73527=CARTESIAN_POINT ( 'NONE',  ( 164.3961040135806968, 245.9045906125373904, 7.095190383188031191 ) ) ;
#73528=EDGE_CURVE ( 'NONE', #78092, #31631, #54640, .T. ) ;
#73535=CARTESIAN_POINT ( 'NONE',  ( 205.9226911964632052, 273.9784317468465815, -10.54881836492553404 ) ) ;
#73536=CARTESIAN_POINT ( 'NONE',  ( 138.9828575061699496, 260.2369531367911009, -4.594050593750048428 ) ) ;
#73537=CARTESIAN_POINT ( 'NONE',  ( 190.1858949294064871, 301.2353624297489887, -5.249932979468886707 ) ) ;
#73539=CARTESIAN_POINT ( 'NONE',  ( 154.5458477507173143, 280.1990093249386859, 3.569508088704419713 ) ) ;
#73540=B_SPLINE_CURVE_WITH_KNOTS ( 'NONE', 3,
 ( #38355, #83018, #21195, #69265, #91604, #13588 ),
 .UNSPECIFIED., .F., .F.,
 ( 4, 2, 4 ),
 ( 0.000000000000000000, 0.0004057782954188846980, 0.0008115565908377693960 ),
 .UNSPECIFIED. ) ;
#73542=CARTESIAN_POINT ( 'NONE',  ( 149.7162292714551199, 271.3308795146458010, 12.12826134257344357 ) ) ;
#73544=CARTESIAN_POINT ( 'NONE',  ( 169.3669221716730533, 285.1312214744803555, -8.684624577439414850 ) ) ;
#73548=CARTESIAN_POINT ( 'NONE',  ( 128.9696990949621522, 255.2677522451419350, -5.000000000000047962 ) ) ;
#73549=CARTESIAN_POINT ( 'NONE',  ( 175.9525681479302932, 285.3181954580452953, -12.02530750686166705 ) ) ;
#73550=ORIENTED_EDGE ( 'NONE', *, *, #11905, .T. ) ;
#73551=CARTESIAN_POINT ( 'NONE',  ( 196.1613785401733878, 290.8855212161054737, 15.98157687694135021 ) ) ;
#73552=CARTESIAN_POINT ( 'NONE',  ( 190.1730848958311810, 301.2575500587478814, 0.2415986433272204748 ) ) ;
#73553=CARTESIAN_POINT ( 'NONE',  ( -5.399728507075681527, 173.8149278399160949, -9.188101187500095079 ) ) ;
#73554=CARTESIAN_POINT ( 'NONE',  ( 39.09232661234986494, 199.5024278399160664, -9.188101187500093303 ) ) ;
#73558=CARTESIAN_POINT ( 'NONE',  ( 157.8043799545718286, 257.3217915922150496, -17.97575562758749257 ) ) ;
#73560=CARTESIAN_POINT ( 'NONE',  ( 190.1693911629507738, 301.2639477917662703, -5.112716700269980485 ) ) ;
#73561=CARTESIAN_POINT ( 'NONE',  ( 148.3593702730603070, 275.6694849721874334, 3.735352563252699820 ) ) ;
#73562=CARTESIAN_POINT ( 'NONE',  ( 77.34551609424316609, 203.9155109091896065, 2.679491924311254714 ) ) ;
#73563=CARTESIAN_POINT ( 'NONE',  ( 80.83312040127718490, 204.1427522451417644, 1.119607411625061291E-15 ) ) ;
#73565=CARTESIAN_POINT ( 'NONE',  ( 204.6075833744878878, 276.2562653119390461, -13.34672481898815910 ) ) ;
#73567=CARTESIAN_POINT ( 'NONE',  ( 35.60133525300030755, 191.3615022471902591, -10.00000000000009592 ) ) ;
#73568=( BOUNDED_CURVE ( )  B_SPLINE_CURVE ( 2, ( #79970, #2962, #80982, #10539, #12537, #95176, #19154, #33856, #41413 ),
 .UNSPECIFIED., .F., .T. ) 
 B_SPLINE_CURVE_WITH_KNOTS ( ( 3, 2, 2, 2, 3 ),
 ( 0.1895161290322580627, 0.1908602150537634379, 0.1935483870967741882, 0.1962365591397849385, 0.1975806451612903136 ),
 .UNSPECIFIED. ) 
 CURVE ( )  GEOMETRIC_REPRESENTATION_ITEM ( )  RATIONAL_B_SPLINE_CURVE ( ( 0.9330127018922194093, 0.9330127018922194093, 1.000000000000000000, 0.8660254037844387076, 1.000000000000000000, 0.8660254037844387076, 1.000000000000000000, 0.9330127018922194093, 0.9330127018922194093 ) ) 
 REPRESENTATION_ITEM ( '' )  );
#73569=CARTESIAN_POINT ( 'NONE',  ( 181.1843555769024476, 292.6731038405765162, 9.241987700880018863 ) ) ;
#73570=CARTESIAN_POINT ( 'NONE',  ( 166.8033540930419463, 285.5752247180022323, -7.877208387440095549 ) ) ;
#73571=CARTESIAN_POINT ( 'NONE',  ( 2.394500126984267396, 178.3149278399160949, -9.188101187500095079 ) ) ;
#73572=CARTESIAN_POINT ( 'NONE',  ( 168.2746533154106316, 286.3035412645079418, 4.462338258111298472 ) ) ;
#73574=CARTESIAN_POINT ( 'NONE',  ( 192.3606619183491091, 297.4685555102766443, 10.99569063633359889 ) ) ;
#73576=CARTESIAN_POINT ( 'NONE',  ( 206.5508451493652444, 272.8904371854448527, 11.05407534521577695 ) ) ;
#73578=CARTESIAN_POINT ( 'NONE',  ( 164.7243055739305078, 245.3361288348881999, -1.445094907380085170 ) ) ;
#73579=CARTESIAN_POINT ( 'NONE',  ( 154.8556227199321427, 262.4291889417971788, 17.77326384500479861 ) ) ;
#73581=CARTESIAN_POINT ( 'NONE',  ( 179.7099650035556238, 262.7785925330675241, -12.85976170404427776 ) ) ;
#73587=CARTESIAN_POINT ( 'NONE',  ( 159.6001914315565955, 258.6705862423590361, 17.36259334898762319 ) ) ;
#73589=VERTEX_POINT ( 'NONE', #4455 ) ;
#73594=CARTESIAN_POINT ( 'NONE',  ( 153.1314981037513121, 265.4154603756023789, 17.73969815997475408 ) ) ;
#73595=CARTESIAN_POINT ( 'NONE',  ( 164.2672861321391053, 246.1277097281173667, -2.417001679502223777 ) ) ;
#73600=CARTESIAN_POINT ( 'NONE',  ( 164.5641499066685469, 246.8022252770303169, -5.664862832761055955 ) ) ;
#73602=CARTESIAN_POINT ( 'NONE',  ( 153.4619471835925708, 264.8431057800031567, 16.95044998314351758 ) ) ;
#73605=CARTESIAN_POINT ( 'NONE',  ( 178.2640794854746105, 263.8995157064278487, 15.14098684682329932 ) ) ;
#73606=ORIENTED_EDGE ( 'NONE', *, *, #56679, .F. ) ;
#73611=VERTEX_POINT ( 'NONE', #19190 ) ;
#73612=CARTESIAN_POINT ( 'NONE',  ( 203.3286960320409094, 267.8359400968079171, 2.569349860321338941 ) ) ;
#73613=CARTESIAN_POINT ( 'NONE',  ( 168.1589593212097498, 275.9390298053305628, -16.40258036402506647 ) ) ;
#73614=CARTESIAN_POINT ( 'NONE',  ( 151.2755745006645896, 275.3008544589386020, -8.292818474215351898 ) ) ;
#73616=CARTESIAN_POINT ( 'NONE',  ( 176.7827973027407040, 278.6576878780061861, -15.83051026523116533 ) ) ;
#73617=CARTESIAN_POINT ( 'NONE',  ( 169.1454831004496384, 261.3880614413394028, -16.47743258951610557 ) ) ;
#73619=CARTESIAN_POINT ( 'NONE',  ( 156.7634869529680373, 266.5784725184484500, -16.23112445323594244 ) ) ;
#73620=VERTEX_POINT ( 'NONE', #50061 ) ;
#73621=CARTESIAN_POINT ( 'NONE',  ( 157.3802686514316349, 269.1245054408723263, 15.58885404214087878 ) ) ;
#73623=CARTESIAN_POINT ( 'NONE',  ( 158.8270733235451075, 260.0119502166541565, 17.68969926203419618 ) ) ;
#73624=CARTESIAN_POINT ( 'NONE',  ( 147.7232839279827203, 274.7827621062478443, 5.908844693136329873 ) ) ;
#73627=CARTESIAN_POINT ( 'NONE',  ( 199.8071198270451703, 281.1414453001559082, -17.28171234339430029 ) ) ;
#73629=CARTESIAN_POINT ( 'NONE',  ( 158.9356049992396152, 255.3624523400558246, -16.15158836202271075 ) ) ;
#73630=ORIENTED_EDGE ( 'NONE', *, *, #52370, .F. ) ;
#73631=B_SPLINE_CURVE_WITH_KNOTS ( 'NONE', 3,
 ( #38175, #62998, #69093, #32084 ),
 .UNSPECIFIED., .F., .F.,
 ( 4, 4 ),
 ( 0.000000000000000000, 0.0001209126443684359120 ),
 .UNSPECIFIED. ) ;
#73634=CARTESIAN_POINT ( 'NONE',  ( 165.0565241268390366, 244.7607094220335568, 2.191926263411719589 ) ) ;
#73635=CARTESIAN_POINT ( 'NONE',  ( 206.4229368915142686, 273.1119807867502800, 10.31819530520674810 ) ) ;
#73639=CARTESIAN_POINT ( 'NONE',  ( 185.9583416565622258, 276.2403346773022577, 16.51595490223188278 ) ) ;
#73641=CARTESIAN_POINT ( 'NONE',  ( 188.2505817719666652, 300.0599093194876446, 0.6416181545256018914 ) ) ;
#73642=CARTESIAN_POINT ( 'NONE',  ( 181.1375824994216828, 258.0330255649733999, 9.585308223983551201 ) ) ;
#73643=EDGE_CURVE ( 'NONE', #75541, #31533, #68376, .T. ) ;
#73644=AXIS2_PLACEMENT_3D ( 'NONE', #23780, #48080, #69880 ) ;
#73645=CARTESIAN_POINT ( 'NONE',  ( 160.3446501917713931, 252.9219144764300893, -16.21746572878571158 ) ) ;
#73647=CARTESIAN_POINT ( 'NONE',  ( 148.4879991328100175, 273.4582365181666432, -8.909052134456917571 ) ) ;
#73649=CARTESIAN_POINT ( 'NONE',  ( 157.4655681218829670, 259.9086309006383431, -17.75190047967350893 ) ) ;
#73650=CARTESIAN_POINT ( 'NONE',  ( 205.7347617114599529, 273.8573068914000714, 10.24322677079193333 ) ) ;
#73651=CARTESIAN_POINT ( 'NONE',  ( 123.4362054459082572, 253.6199935810940929, 2.679491924311251605 ) ) ;
#73652=EDGE_CURVE ( 'NONE', #79145, #87147, #96238, .T. ) ;
#73655=CARTESIAN_POINT ( 'NONE',  ( 35.94413697178375600, 184.8927522451418213, 10.00000000000009592 ) ) ;
#73656=CARTESIAN_POINT ( 'NONE',  ( 113.4086522182495287, 224.0327760586659167, 1.948934522072302763E-15 ) ) ;
#73657=AXIS2_PLACEMENT_3D ( 'NONE', #38782, #30195, #85444 ) ;
#73658=CARTESIAN_POINT ( 'NONE',  ( 183.9912383556867610, 296.9911047963649935, -2.788240429904596862 ) ) ;
#73659=CARTESIAN_POINT ( 'NONE',  ( 167.7859171384422154, 281.8497203286631816, -10.91337641437639761 ) ) ;
#73660=CARTESIAN_POINT ( 'NONE',  ( 89.66121469831512059, 234.1199935810940929, 2.679491924311251605 ) ) ;
#73661=CARTESIAN_POINT ( 'NONE',  ( 208.2512496840233496, 269.9452501379965952, 1.821023623773176947 ) ) ;
#73662=CARTESIAN_POINT ( 'NONE',  ( 27.67213724359008964, 174.5327760586659451, 1.948934522072303157E-15 ) ) ;
#73664=ORIENTED_EDGE ( 'NONE', *, *, #96675, .T. ) ;
#73667=CARTESIAN_POINT ( 'NONE',  ( 185.5146895125434980, 259.2464410770732002, -5.300532970778875530 ) ) ;
#73668=CARTESIAN_POINT ( 'NONE',  ( 19.51315699177561314, 193.6199935810941213, 2.679491924311251605 ) ) ;
#73669=CARTESIAN_POINT ( 'NONE',  ( 190.7569505155522904, 300.2462651405980978, -5.670926626284815697 ) ) ;
#73671=CARTESIAN_POINT ( 'NONE',  ( 207.1432938686257046, 271.8642859028066141, -6.405155839440290322 ) ) ;
#73672=CARTESIAN_POINT ( 'NONE',  ( 181.8774662184618194, 285.1120569720015965, 15.89814067624403116 ) ) ;
#73673=DIRECTION ( 'NONE',  ( 0.4999999999999998890, -0.8660254037844385966, 0.000000000000000000 ) ) ;
#73674=CARTESIAN_POINT ( 'NONE',  ( 53.97765888354242492, 189.7202760586659451, -5.415160957724236172E-17 ) ) ;
#73675=CARTESIAN_POINT ( 'NONE',  ( 104.2158063034570290, 217.6427522451417360, 1.119607411625061291E-15 ) ) ;
#73679=CARTESIAN_POINT ( 'NONE',  ( 2.016134656476094023, 159.7202760586659736, -5.415160957724236172E-17 ) ) ;
#73681=CARTESIAN_POINT ( 'NONE',  ( 198.5201458116119397, 286.8000164587433005, -18.30276554821096013 ) ) ;
#73683=CARTESIAN_POINT ( 'NONE',  ( 193.1028332910263998, 296.1830769848763225, -12.04975758233223893 ) ) ;
#73685=CARTESIAN_POINT ( 'NONE',  ( 204.1633547645365638, 275.3510256380408237, 13.36249479004741580 ) ) ;
#73687=CARTESIAN_POINT ( 'NONE',  ( 189.8238368927809745, 301.8624653444729802, -0.3620111495846872751 ) ) ;
#73689=CARTESIAN_POINT ( 'NONE',  ( -0.7717317059461257234, 170.3615022471902591, -10.00000000000009592 ) ) ;
#73691=CARTESIAN_POINT ( 'NONE',  ( 123.3675972660055749, 242.0333772461660544, 9.188101187500095079 ) ) ;
#73698=CARTESIAN_POINT ( 'NONE',  ( 190.8003542858887158, 300.1710876051355399, -7.952726366508386491 ) ) ;
#73700=B_SPLINE_CURVE_WITH_KNOTS ( 'NONE', 3,
 ( #15183, #46083, #14705, #30902 ),
 .UNSPECIFIED., .F., .F.,
 ( 4, 4 ),
 ( 0.03034436796817569643, 0.03943245488163680396 ),
 .UNSPECIFIED. ) ;
#73701=CARTESIAN_POINT ( 'NONE',  ( 191.2645787786270262, 299.3670271975948367, 7.309947121636420242 ) ) ;
#73702=CARTESIAN_POINT ( 'NONE',  ( 164.0609569930187206, 246.4850822801560639, 8.623773733057504387 ) ) ;
#73703=ADVANCED_FACE ( 'NONE', ( #63641 ), #77858, .T. ) ;
#73704=CARTESIAN_POINT ( 'NONE',  ( 181.4283053378885597, 267.7238133557910373, 16.48022347432943135 ) ) ;
#73705=CARTESIAN_POINT ( 'NONE',  ( 169.5303480748956417, 265.9959136028709281, -17.12794529520477838 ) ) ;
#73709=CARTESIAN_POINT ( 'NONE',  ( 165.6547257697228588, 269.1390321728339359, -17.08687207675598430 ) ) ;
#73713=CARTESIAN_POINT ( 'NONE',  ( 185.8923765766539589, 296.7039355726019494, 5.058929278049905776 ) ) ;
#73718=CARTESIAN_POINT ( 'NONE',  ( 86.89529822776817980, 227.6427522451419065, 10.00000000000009415 ) ) ;
#73719=EDGE_LOOP ( 'NONE', ( #21473, #94951, #23881, #77844 ) ) ;
#73722=CARTESIAN_POINT ( 'NONE',  ( 194.1852025340051284, 294.3083584634874796, -15.46421316575964688 ) ) ;
#73723=CARTESIAN_POINT ( 'NONE',  ( 157.8749902780253365, 263.0387574327914422, -16.96638006302123713 ) ) ;
#73728=VERTEX_POINT ( 'NONE', #8942 ) ;
#73729=CARTESIAN_POINT ( 'NONE',  ( 86.72372382049401551, 227.0024278399160949, 9.188101187500095079 ) ) ;
#73732=CARTESIAN_POINT ( 'NONE',  ( 182.3576772462011206, 258.0377563476427554, -5.917524771864123068 ) ) ;
#73733=ORIENTED_EDGE ( 'NONE', *, *, #90750, .F. ) ;
#73734=ORIENTED_EDGE ( 'NONE', *, *, #17598, .T. ) ;
#73735=CARTESIAN_POINT ( 'NONE',  ( 194.5481722404243214, 283.9256704378062182, -17.81052777154215860 ) ) ;
#73738=ORIENTED_EDGE ( 'NONE', *, *, #29393, .F. ) ;
#73740=CARTESIAN_POINT ( 'NONE',  ( 203.5555343017997529, 278.0784677578903370, -15.71723084798551362 ) ) ;
#73741=ORIENTED_EDGE ( 'NONE', *, *, #99048, .T. ) ;
#73742=CARTESIAN_POINT ( 'NONE',  ( 207.4139425164918293, 271.3955086937027090, -6.918700682290102932 ) ) ;
#73748=CARTESIAN_POINT ( 'NONE',  ( 136.8177939967088435, 258.9869531367911009, 4.594050593750046652 ) ) ;
#73749=DIRECTION ( 'NONE',  ( 0.4999999999999998890, -0.8660254037844385966, 0.000000000000000000 ) ) ;
#73751=B_SPLINE_CURVE_WITH_KNOTS ( 'NONE', 3,
 ( #23352, #93300, #46144, #9171 ),
 .UNSPECIFIED., .F., .F.,
 ( 4, 4 ),
 ( 0.008808793980068530330, 0.01508001664632129327 ),
 .UNSPECIFIED. ) ;
#73757=ORIENTED_EDGE ( 'NONE', *, *, #57053, .T. ) ;
#73760=CARTESIAN_POINT ( 'NONE',  ( 202.8211298556536804, 279.3504935719197988, 17.07914446815911447 ) ) ;
#73762=CARTESIAN_POINT ( 'NONE',  ( 153.4389471588997651, 276.9034970075614410, 7.158391495164361906 ) ) ;
#73765=CARTESIAN_POINT ( 'NONE',  ( 171.6183182742749977, 280.0105497640429917, 13.87264028713023301 ) ) ;
#73769=CARTESIAN_POINT ( 'NONE',  ( 184.7835433439430801, 272.8597739924990151, -17.09939324130442273 ) ) ;
#73772=B_SPLINE_CURVE_WITH_KNOTS ( 'NONE', 3,
 ( #84857, #85365, #31105, #51558, #93460, #84363, #54910, #46816, #7826, #61993, #100041, #15912, #13082, #70104, #85889, #47309, #36349, #67252, #14910, #28760, #22521, #3246, #49325, #94455, #71139, #17415, #72651, #64018, #95968, #79270, #71644, #2238, #64524, #3733, #25523, #87406, #10332, #88385, #49816, #11347, #65511, #24514, #16910, #59379, #36593, #35105, #74640, #20936, #5215, #27530, #89851, #52295, #50802, #97923 ),
 .UNSPECIFIED., .F., .F.,
 ( 4, 2, 2, 2, 2, 2, 2, 2, 2, 2, 2, 2, 2, 2, 2, 2, 2, 2, 2, 2, 2, 2, 2, 2, 2, 2, 4 ),
 ( 0.0003707374380231760508, 0.0008344351438995525547, 0.001066283996837772601, 0.001298132849775992430, 0.001414057276245102345, 0.001529981702714212259, 0.001645906129183322391, 0.001761830555652432522, 0.001993679408590594022, 0.002225528261528755738, 0.002689225967405013250, 0.003152923673281270763, 0.004080319085033785355, 0.005007714496786301248, 0.005471412202662599526, 0.005703261055600751701, 0.005819185482069867688, 0.005877147695304387950, 0.005935109908538907346, 0.005993072121773427609, 0.006051034335007947872, 0.006166958761476983193, 0.006398807614415211696, 0.006862505320291640946, 0.007326203026168070197, 0.007558051879106252730, 0.007789900732044434395 ),
 .UNSPECIFIED. ) ;
#73773=CARTESIAN_POINT ( 'NONE',  ( 160.4213754921470922, 276.0766563818076520, 12.64007677385747996 ) ) ;
#73775=CARTESIAN_POINT ( 'NONE',  ( 156.8019257795724002, 276.6452858554906697, 10.13430466171780786 ) ) ;
#73778=CARTESIAN_POINT ( 'NONE',  ( 164.7211056338534547, 274.2655263718911556, 14.88749732853323593 ) ) ;
#73779=CARTESIAN_POINT ( 'NONE',  ( 161.3905752240380593, 281.4725768632542895, -7.270332528193686805 ) ) ;
#73781=CARTESIAN_POINT ( 'NONE',  ( 202.6672992768344841, 269.6846706196681680, 6.012455439154622994 ) ) ;
#73784=CARTESIAN_POINT ( 'NONE',  ( 189.8717058746474606, 274.3034288976620019, -15.65974089894849364 ) ) ;
#73791=CARTESIAN_POINT ( 'NONE',  ( 0.1211834420501121945, 177.0024278399160949, -9.188101187500093303 ) ) ;
#73792=CARTESIAN_POINT ( 'NONE',  ( 105.6408794604690797, 240.9869531367911293, 4.594050593750046652 ) ) ;
#73794=CARTESIAN_POINT ( 'NONE',  ( 186.1423004029541062, 295.4822973340021690, -7.680234142728118663 ) ) ;
#73796=CARTESIAN_POINT ( 'NONE',  ( 196.7523914512457281, 284.9123565375628573, 17.81558562320455508 ) ) ;
#73797=CARTESIAN_POINT ( 'NONE',  ( 160.8319974213378600, 281.7448561697519267, 5.375735037517149095 ) ) ;
#73798=CARTESIAN_POINT ( 'NONE',  ( 147.6884207308302450, 274.8431469350302336, -8.096293592099874203 ) ) ;
#73801=CARTESIAN_POINT ( 'NONE',  ( 48.51954752611815991, 205.4865022471903444, -10.00000000000009592 ) ) ;
#73802=CARTESIAN_POINT ( 'NONE',  ( 165.6450024763602755, 253.6044069627646991, -13.13053692596552047 ) ) ;
#73803=CARTESIAN_POINT ( 'NONE',  ( 176.0505323877982846, 265.6043802274069208, -15.93901269056853920 ) ) ;
#73804=CARTESIAN_POINT ( 'NONE',  ( 89.24104401994878799, 213.1423013555409796, -4.594050593750043987 ) ) ;
#73805=CARTESIAN_POINT ( 'NONE',  ( 207.3646600298985447, 271.4808684644054324, -5.284084612275558257 ) ) ;
#73808=CARTESIAN_POINT ( 'NONE',  ( 195.9359860111818250, 291.2759125279654882, 17.49638312768267312 ) ) ;
#73809=CARTESIAN_POINT ( 'NONE',  ( 151.7927911171883295, 267.7341688927767791, 15.72584582110084206 ) ) ;
#73810=B_SPLINE_CURVE_WITH_KNOTS ( 'NONE', 3,
 ( #71221, #63096, #24593, #15483 ),
 .UNSPECIFIED., .F., .F.,
 ( 4, 4 ),
 ( 0.007902357107153172230, 0.01373811809388502357 ),
 .UNSPECIFIED. ) ;
#73811=CARTESIAN_POINT ( 'NONE',  ( 198.8194531333411419, 286.2816009704309863, -17.01510935557533344 ) ) ;
#73812=CARTESIAN_POINT ( 'NONE',  ( 204.4092890902271904, 276.1033601826059112, -13.04005437736222106 ) ) ;
#73816=CARTESIAN_POINT ( 'NONE',  ( 192.5143468344189728, 297.2023654272867361, -12.06830393602581530 ) ) ;
#73817=CARTESIAN_POINT ( 'NONE',  ( 131.7301550730730071, 246.8615022471902591, -10.00000000000009592 ) ) ;
#73822=CARTESIAN_POINT ( 'NONE',  ( 164.3663504224794565, 247.9561253440330972, -9.019399920391260039 ) ) ;
#73823=CARTESIAN_POINT ( 'NONE',  ( 188.0428630768715834, 286.0956317496587644, -16.61304186841477559 ) ) ;
#73829=CARTESIAN_POINT ( 'NONE',  ( 202.9526507793443955, 267.5288703438144466, -1.989423397307486185 ) ) ;
#73831=CARTESIAN_POINT ( 'NONE',  ( 138.2253456014563255, 240.6115022471902023, -5.000000000000041744 ) ) ;
#73832=CARTESIAN_POINT ( 'NONE',  ( 157.8719920515997046, 257.2046840049564480, -17.69857783492101433 ) ) ;
#73834=VERTEX_POINT ( 'NONE', #47925 ) ;
#73835=CARTESIAN_POINT ( 'NONE',  ( 188.6826127332440421, 272.6057162039079458, 16.71479996418005243 ) ) ;
#73837=CARTESIAN_POINT ( 'NONE',  ( 196.9200716942098950, 264.9052758880268925, -4.632697318226754568 ) ) ;
#73843=CARTESIAN_POINT ( 'NONE',  ( 189.5277700490664472, 290.0407984534384127, 14.44961698594945609 ) ) ;
#73844=CARTESIAN_POINT ( 'NONE',  ( 158.7703600882743729, 255.6486649215402167, 17.63461153596049158 ) ) ;
#73845=CARTESIAN_POINT ( 'NONE',  ( 149.6191658661038559, 251.0643266524160140, 9.188101187500095079 ) ) ;
#73853=EDGE_CURVE ( 'NONE', #74497, #62997, #95523, .T. ) ;
#73854=CARTESIAN_POINT ( 'NONE',  ( 68.07728789491675059, 210.1115022471902591, 10.00000000000009592 ) ) ;
#73859=( BOUNDED_CURVE ( )  B_SPLINE_CURVE ( 2, ( #51578, #81040, #51064, #97218, #19212, #88148, #20194, #35372, #13098 ),
 .UNSPECIFIED., .F., .T. ) 
 B_SPLINE_CURVE_WITH_KNOTS ( ( 3, 2, 2, 2, 3 ),
 ( 0.1975806451612903136, 0.1989247311827956888, 0.2016129032258064391, 0.2043010752688172171, 0.2056451612903225923 ),
 .UNSPECIFIED. ) 
 CURVE ( )  GEOMETRIC_REPRESENTATION_ITEM ( )  RATIONAL_B_SPLINE_CURVE ( ( 0.9330127018922194093, 0.9330127018922194093, 1.000000000000000000, 0.8660254037844387076, 1.000000000000000000, 0.8660254037844387076, 1.000000000000000000, 0.9330127018922194093, 0.9330127018922194093 ) ) 
 REPRESENTATION_ITEM ( '' )  );
#73860=CARTESIAN_POINT ( 'NONE',  ( 204.1953342137782954, 276.9703018036655067, 13.84727111424505885 ) ) ;
#73863=CARTESIAN_POINT ( 'NONE',  ( 152.1671311979278016, 269.0857928536317445, 15.36489295260887822 ) ) ;
#73865=CARTESIAN_POINT ( 'NONE',  ( 164.2436631241379246, 246.1686259782033517, 4.255161687766976009 ) ) ;
#73866=CARTESIAN_POINT ( 'NONE',  ( 167.4183826251619678, 266.1184513312476270, 16.55919039627169909 ) ) ;
#73867=CARTESIAN_POINT ( 'NONE',  ( 181.1523296486749643, 256.9212113246534273, 4.964240719889960296 ) ) ;
#73868=CARTESIAN_POINT ( 'NONE',  ( 97.41363812451689341, 236.2369531367911009, -4.594050593750048428 ) ) ;
#73871=CARTESIAN_POINT ( 'NONE',  ( 163.5882744166410703, 276.6356449797434038, -13.72909506296926629 ) ) ;
#73877=CARTESIAN_POINT ( 'NONE',  ( 180.6484119781345328, 294.0070947715454395, -2.628133096437607730 ) ) ;
#73878=CARTESIAN_POINT ( 'NONE',  ( 157.6673516573649181, 257.5591315650518141, 16.79781451397666103 ) ) ;
#73879=CARTESIAN_POINT ( 'NONE',  ( 206.7923762329701276, 272.4720930770340033, -9.496103119940368487 ) ) ;
#73880=CARTESIAN_POINT ( 'NONE',  ( 207.1661313457130404, 271.3965419664068577, -4.352715553263532655 ) ) ;
#73881=CARTESIAN_POINT ( 'NONE',  ( 83.63833477162944519, 231.3464784336661637, 1.353441290958777327E-15 ) ) ;
#73885=CARTESIAN_POINT ( 'NONE',  ( 163.3409975114459485, 247.7320886816312111, -10.96358124877083640 ) ) ;
#73886=ORIENTED_EDGE ( 'NONE', *, *, #16914, .F. ) ;
#73889=CARTESIAN_POINT ( 'NONE',  ( 191.3867969386575680, 263.7415086189949989, -8.063185982860206380 ) ) ;
#73891=AXIS2_PLACEMENT_3D ( 'NONE', #90727, #85103, #21284 ) ;
#73892=CARTESIAN_POINT ( 'NONE',  ( 191.4738032422262677, 260.7793432447242594, -0.2951778641931921410 ) ) ;
#73893=CARTESIAN_POINT ( 'NONE',  ( 137.8467198073504107, 241.2048013555409796, 4.594050593750051981 ) ) ;
#73895=CARTESIAN_POINT ( 'NONE',  ( 177.6444986370304946, 293.6980009803469329, 2.770296639708824227 ) ) ;
#73898=CARTESIAN_POINT ( 'NONE',  ( 157.4725523017146429, 257.8965339463198916, 17.43710027717953892 ) ) ;
#73900=CARTESIAN_POINT ( 'NONE',  ( 52.92184332868904306, 211.3615022471903160, 5.000000000000046185 ) ) ;
#73903=CARTESIAN_POINT ( 'NONE',  ( 190.7986890213734625, 271.0762054634549258, 14.19875726436414176 ) ) ;
#73904=CARTESIAN_POINT ( 'NONE',  ( 114.2732676653602510, 248.3297689869269220, -2.679491924311252493 ) ) ;
#73908=DIRECTION ( 'NONE',  ( -0.8660254037844387076, -0.4999999999999998890, -0.000000000000000000 ) ) ;
#73909=CARTESIAN_POINT ( 'NONE',  ( 161.5431944097339851, 250.8459749958011287, 14.52339846942414603 ) ) ;
#73911=CARTESIAN_POINT ( 'NONE',  ( 206.6912923161529818, 272.6471755567893638, -9.325620632947922317 ) ) ;
#73913=CARTESIAN_POINT ( 'NONE',  ( 207.7625791259561652, 270.7916523727319031, -1.015623356719550063 ) ) ;
#73914=CARTESIAN_POINT ( 'NONE',  ( 168.4809247738020019, 252.9187805847961670, 12.05003015331094041 ) ) ;
#73917=CARTESIAN_POINT ( 'NONE',  ( 182.9064100835608144, 264.9912211263795143, 13.33838763049125831 ) ) ;
#73918=CARTESIAN_POINT ( 'NONE',  ( 77.51335635343683350, 208.8927522451418213, 10.00000000000009948 ) ) ;
#73925=CARTESIAN_POINT ( 'NONE',  ( 24.91150772114469092, 179.0643266524160140, 9.188101187500095079 ) ) ;
#73927=VERTEX_POINT ( 'NONE', #27154 ) ;
#73929=CARTESIAN_POINT ( 'NONE',  ( 182.9770351804424706, 269.0381230690315988, 16.62995593613592504 ) ) ;
#73931=CARTESIAN_POINT ( 'NONE',  ( 36.54820344085055694, 204.1589784336661637, -6.496448406907676862E-16 ) ) ;
#73933=CARTESIAN_POINT ( 'NONE',  ( 161.8016137473484548, 250.3983795733946636, 14.25000412375400316 ) ) ;
#73934=CARTESIAN_POINT ( 'NONE',  ( 174.6026413853588508, 289.1850952631716041, 7.771083852652256319 ) ) ;
#73935=CARTESIAN_POINT ( 'NONE',  ( 147.3023124603499809, 275.5119060767245287, 5.196938859334171212 ) ) ;
#73937=CARTESIAN_POINT ( 'NONE',  ( 202.9409128566982758, 270.0839114184054779, -6.625179921953246343 ) ) ;
#73938=CARTESIAN_POINT ( 'NONE',  ( 146.9235493515124062, 276.1679430252639804, 0.7994986043261682607 ) ) ;
#73941=CARTESIAN_POINT ( 'NONE',  ( 166.9032805970908839, 257.6634323422801458, -15.74477645480126142 ) ) ;
#73946=CARTESIAN_POINT ( 'NONE',  ( 100.6254093204819497, 222.2365022471902023, -10.00000000000009059 ) ) ;
#73948=CARTESIAN_POINT ( 'NONE',  ( 161.9624950439807094, 268.0139618835574424, -17.50977960935507127 ) ) ;
#73950=CARTESIAN_POINT ( 'NONE',  ( 63.01627839189497138, 213.3149278399160949, 9.188101187500093303 ) ) ;
#73951=ORIENTED_EDGE ( 'NONE', *, *, #8927, .T. ) ;
#73952=CARTESIAN_POINT ( 'NONE',  ( 162.6241144845578503, 263.2905756906662305, 17.26806262333970565 ) ) ;
#73953=CARTESIAN_POINT ( 'NONE',  ( 190.9335643195044838, 299.9403610588350944, -4.692880224846124548 ) ) ;
#73957=CARTESIAN_POINT ( 'NONE',  ( 171.3677841791904086, 286.5144775268977924, 7.813166782325457582 ) ) ;
#73958=CARTESIAN_POINT ( 'NONE',  ( 207.6727254509676186, 270.9472835030587703, 7.315149605389819953 ) ) ;
#73961=CARTESIAN_POINT ( 'NONE',  ( 188.9599767341003940, 265.5171183316097654, 10.73179992602947941 ) ) ;
#73962=CARTESIAN_POINT ( 'NONE',  ( 149.1429535397850827, 272.3238222086447990, -12.91457852089092384 ) ) ;
#73972=ORIENTED_EDGE ( 'NONE', *, *, #161, .F. ) ;
#73974=CARTESIAN_POINT ( 'NONE',  ( 191.5281967176683509, 298.9104275333885994, 7.715154960566919407 ) ) ;
#73975=EDGE_CURVE ( 'NONE', #24993, #77732, #46660, .T. ) ;
#73978=ORIENTED_EDGE ( 'NONE', *, *, #48031, .T. ) ;
#73980=CARTESIAN_POINT ( 'NONE',  ( 161.4143265314674522, 251.0691807084224365, -12.94469757303959234 ) ) ;
#73982=CARTESIAN_POINT ( 'NONE',  ( 149.1486417047969155, 272.3139700178423368, -11.47583619705022606 ) ) ;
#73983=VERTEX_POINT ( 'NONE', #80902 ) ;
#73989=CARTESIAN_POINT ( 'NONE',  ( 115.5733686319456126, 237.5333772461660544, 9.188101187500095079 ) ) ;
#73991=CARTESIAN_POINT ( 'NONE',  ( 205.4317452772315278, 270.7218421723977144, 7.456875539217049820 ) ) ;
#73994=AXIS2_PLACEMENT_3D ( 'NONE', #67516, #37113, #68016 ) ;
#73995=CARTESIAN_POINT ( 'NONE',  ( 207.8725590214046406, 270.6011616060040410, 1.988011721677743093 ) ) ;
#73996=ORIENTED_EDGE ( 'NONE', *, *, #98725, .F. ) ;
#74001=CARTESIAN_POINT ( 'NONE',  ( 71.40607303893924040, 212.0333772461660544, 9.188101187500095079 ) ) ;
#74002=CARTESIAN_POINT ( 'NONE',  ( 177.8222571804544430, 286.5223583772871621, 13.77940225188420875 ) ) ;
#74004=CARTESIAN_POINT ( 'NONE',  ( 198.5328126748496516, 286.7780768080430676, 18.48542741931266775 ) ) ;
#74005=CARTESIAN_POINT ( 'NONE',  ( 174.7265224105599657, 278.0225128774238215, 15.48253028248275065 ) ) ;
#74006=B_SPLINE_CURVE_WITH_KNOTS ( 'NONE', 3,
 ( #88021, #52932, #28640, #69127, #30133, #100053, #21550, #6834, #6348, #23018, #76262, #60025, #45329, #90989, #83885, #44330, #60516, #44828, #68629, #7329, #30641, #13464, #91988, #37719, #37235, #68133, #5847, #52432, #61528, #83379, #67638, #36732, #29643, #99550, #75262, #13945, #53425, #82411, #98571, #99061, #14447, #90501, #61016, #22540, #84375, #5354, #29154, #12976 ),
 .UNSPECIFIED., .F., .F.,
 ( 4, 2, 2, 2, 2, 2, 2, 2, 2, 2, 2, 2, 2, 2, 2, 2, 2, 2, 2, 2, 2, 2, 2, 4 ),
 ( 0.0003007692019500355176, 0.001319192577369706146, 0.001828404265079501372, 0.002083010108934399418, 0.002210313030861848008, 0.002337615952789296597, 0.002592221796644032447, 0.002846827640498767863, 0.003356039328208184486, 0.004374462703627130487, 0.005392886079046075622, 0.005902097766755467524, 0.006156703610610120107, 0.006411309454464772691, 0.006474960915428472699, 0.006538612376392171840, 0.006602263837355871849, 0.006665915298319570990, 0.006920521142174513272, 0.007429732829884467225, 0.007684338673739515325, 0.007938944517594562558, 0.008193550361449610658, 0.008448156205304658758 ),
 .UNSPECIFIED. ) ;
#74009=CARTESIAN_POINT ( 'NONE',  ( 112.8118497929261252, 247.4860189848785126, -2.679491924311252493 ) ) ;
#74010=CARTESIAN_POINT ( 'NONE',  ( 203.3349860717029571, 278.4604684979374838, -16.59553970625579566 ) ) ;
#74011=ORIENTED_EDGE ( 'NONE', *, *, #62187, .F. ) ;
#74012=CARTESIAN_POINT ( 'NONE',  ( 195.4137072836104494, 292.1805258198313027, 15.38860452967709413 ) ) ;
#74013=CARTESIAN_POINT ( 'NONE',  ( -16.52256874082355864, 171.2677522451419350, -5.000000000000047962 ) ) ;
#74014=CARTESIAN_POINT ( 'NONE',  ( 161.8408514536557163, 250.3304178724980318, -14.12919723462510646 ) ) ;
#74015=CARTESIAN_POINT ( 'NONE',  ( 192.4663556654298588, 297.2854885702906245, -12.98646995774174684 ) ) ;
#74017=B_SPLINE_CURVE_WITH_KNOTS ( 'NONE', 3,
 ( #87776, #49212, #80144, #18808 ),
 .UNSPECIFIED., .F., .F.,
 ( 4, 4 ),
 ( 0.04143897040461883702, 0.04887120950165265570 ),
 .UNSPECIFIED. ) ;
#74018=CARTESIAN_POINT ( 'NONE',  ( 199.8798371376168745, 283.2826252849788489, -17.21687883691964771 ) ) ;
#74021=CARTESIAN_POINT ( 'NONE',  ( 208.2764314485352770, 269.9016340424377063, 2.433736665191914117 ) ) ;
#74023=CARTESIAN_POINT ( 'NONE',  ( 118.5230073417626073, 248.4244531367911293, -4.594050593750046652 ) ) ;
#74027=CARTESIAN_POINT ( 'NONE',  ( 205.8688675895746201, 273.6846427845131871, -9.898080752049997599 ) ) ;
#74028=CARTESIAN_POINT ( 'NONE',  ( 164.4294002498235159, 245.8469198396639399, 6.098783631055905374 ) ) ;
#74031=EDGE_LOOP ( 'NONE', ( #15485, #43820, #47574, #82157, #60599, #80887, #7588, #28728, #34719, #87400, #90857, #74204, #6282, #15118, #67614, #77216, #84085, #48892, #50421, #12547 ) ) ;
#74033=CARTESIAN_POINT ( 'NONE',  ( 119.0104069514411123, 249.5177522451419065, 5.000000000000046185 ) ) ;
#74034=CARTESIAN_POINT ( 'NONE',  ( 164.7026013006809251, 246.9704538741483759, -5.638495517494114928 ) ) ;
#74035=CARTESIAN_POINT ( 'NONE',  ( 147.8331127587908043, 276.3582630845543804, 2.721914673797492412 ) ) ;
#74036=CARTESIAN_POINT ( 'NONE',  ( 29.67341102961999155, 199.4860189848785410, -2.679491924311252493 ) ) ;
#74037=CARTESIAN_POINT ( 'NONE',  ( 198.5699292022329416, 266.2780175646987573, 0.8405458176556424021 ) ) ;
#74038=CARTESIAN_POINT ( 'NONE',  ( 147.0670278774466908, 275.9194309285509235, 3.666898409139099257 ) ) ;
#74042=CARTESIAN_POINT ( 'NONE',  ( 172.8463378600133353, 251.6495383470449099, 3.423699583515463996 ) ) ;
#74043=B_SPLINE_SURFACE_WITH_KNOTS ( 'NONE', 3, 1, ( 
 ( #75396, #45463 ),
 ( #53563, #30781 ),
 ( #68765, #84516 ),
 ( #36875, #6972 ),
 ( #83519, #99689 ),
 ( #52076, #99192 ),
 ( #7465, #15059 ),
 ( #21684, #100196 ),
 ( #92131, #29777 ),
 ( #44967, #37364 ),
 ( #60650, #92612 ),
 ( #6486, #76867 ),
 ( #75906, #23158 ),
 ( #38357, #90634 ),
 ( #98706, #69267 ),
 ( #38861, #53071 ),
 ( #77383, #54049 ),
 ( #91606, #85007 ),
 ( #21197, #15551 ),
 ( #46452, #22178 ),
 ( #7985, #69767 ),
 ( #375, #83020 ),
 ( #60155, #1884 ),
 ( #870, #1387 ),
 ( #2392, #16569 ),
 ( #46972, #93606 ),
 ( #85527, #17573 ),
 ( #47955, #40849 ),
 ( #31749, #77891 ),
 ( #71794, #63671 ),
 ( #16070, #78898 ),
 ( #33272, #62654 ),
 ( #93096, #94610 ),
 ( #8971, #64175 ) ),
 .UNSPECIFIED., .T., .F., .F.,
 ( 4, 2, 2, 2, 2, 2, 2, 2, 2, 2, 2, 2, 2, 2, 2, 2, 4 ),
 ( 2, 2 ),
 ( 0.000000000000000000, 0.06250000000000000000, 0.1250000000000000000, 0.1875000000000000000, 0.2500000000000000000, 0.3125000000000000000, 0.3750000000000000000, 0.4375000000000000000, 0.5000000000000000000, 0.5625000000000000000, 0.6250000000000000000, 0.6875000000000000000, 0.7500000000000000000, 0.8125000000000000000, 0.8750000000000000000, 0.9375000000000000000, 1.000000000000000000 ),
 ( 0.000000000000000000, 1.000000000000000000 ),
 .UNSPECIFIED. ) ;
#74045=CARTESIAN_POINT ( 'NONE',  ( 149.5633513747893346, 271.5956717990251832, 12.83777201928511325 ) ) ;
#74046=FACE_OUTER_BOUND ( 'NONE', #60207, .T. ) ;
#74048=CARTESIAN_POINT ( 'NONE',  ( 159.3528137482544196, 254.6398255893999476, 16.73628156321660398 ) ) ;
#74049=CARTESIAN_POINT ( 'NONE',  ( 189.9879251633717558, 299.5782561228834879, -6.671532329245590809 ) ) ;
#74051=CARTESIAN_POINT ( 'NONE',  ( 132.0729567918564555, 240.3927522451418213, 10.00000000000009592 ) ) ;
#74052=CARTESIAN_POINT ( 'NONE',  ( 183.3367312544899619, 279.0378104038655351, 17.10307584900649402 ) ) ;
#74055=CARTESIAN_POINT ( 'NONE',  ( 157.3025066944120454, 258.1910615777721887, 18.21299529665260053 ) ) ;
#74056=CARTESIAN_POINT ( 'NONE',  ( 199.0756812798354645, 285.8378008023734083, -18.45377816087746936 ) ) ;
#74057=CARTESIAN_POINT ( 'NONE',  ( -11.27255005043015856, 173.4869531367911293, 4.594050593750046652 ) ) ;
#74058=CARTESIAN_POINT ( 'NONE',  ( 50.89226983467786170, 194.0643266524160424, 9.188101187500095079 ) ) ;
#74059=CARTESIAN_POINT ( 'NONE',  ( 178.6236953501245353, 259.1675616789437981, -10.33478249233844259 ) ) ;
#74063=CARTESIAN_POINT ( 'NONE',  ( 204.9658583905037688, 275.6357147811169170, -12.57240504404813564 ) ) ;
#74066=CARTESIAN_POINT ( 'NONE',  ( 171.2891392173955012, 258.0937863124287333, 14.46422458907198383 ) ) ;
#74067=CARTESIAN_POINT ( 'NONE',  ( 71.81202244518924260, 212.2677522451418497, 10.00000000000009592 ) ) ;
#74070=CARTESIAN_POINT ( 'NONE',  ( 150.6881537519499830, 269.6474569333088311, 15.31267828461696467 ) ) ;
#74071=CARTESIAN_POINT ( 'NONE',  ( 36.90037335867696555, 192.1115022471902591, 10.00000000000009592 ) ) ;
#74072=CARTESIAN_POINT ( 'NONE',  ( 181.7591720214631721, 291.6897925616224256, 9.200304531648196615 ) ) ;
#74075=CARTESIAN_POINT ( 'NONE',  ( -2.422939729449181012, 181.6589784336661637, -6.496448406907675876E-16 ) ) ;
#74076=CARTESIAN_POINT ( 'NONE',  ( 167.6502826215564994, 287.3877002845107995, 4.891367078714356609 ) ) ;
#74077=CARTESIAN_POINT ( 'NONE',  ( 152.7314557461996571, 266.1083540640618708, 17.39314074348802208 ) ) ;
#74082=CARTESIAN_POINT ( 'NONE',  ( 207.4285356523023154, 271.3702326410368642, 7.833982582429932506 ) ) ;
#74083=CARTESIAN_POINT ( 'NONE',  ( 155.0303156110108489, 262.1266119787277944, 17.11986653161320859 ) ) ;
#74084=CARTESIAN_POINT ( 'NONE',  ( 125.6883311748214425, 231.8262482093457493, 3.021315404115420679E-15 ) ) ;
#74085=CARTESIAN_POINT ( 'NONE',  ( 176.4522659647303442, 260.3536617702438889, -13.41910003846964550 ) ) ;
#74088=CARTESIAN_POINT ( 'NONE',  ( 159.5744557550824823, 258.7184754996998777, 17.16512081183459415 ) ) ;
#74089=CARTESIAN_POINT ( 'NONE',  ( 194.6820509838467785, 270.8910309865917156, -14.27696746312268239 ) ) ;
#74091=CARTESIAN_POINT ( 'NONE',  ( 156.8023757504856803, 276.4965331495019427, 10.27696673126826532 ) ) ;
#74096=CARTESIAN_POINT ( 'NONE',  ( 153.3920560952016956, 264.9641606960921649, 16.50453917291963535 ) ) ;
#74097=CARTESIAN_POINT ( 'NONE',  ( 81.52103558181507026, 206.3262482093457493, 3.021315404115420679E-15 ) ) ;
#74099=EDGE_CURVE ( 'NONE', #4549, #4372, #54599, .T. ) ;
#74100=CARTESIAN_POINT ( 'NONE',  ( 117.4407359106297264, 248.6115022471903160, -5.000000000000047962 ) ) ;
#74102=ORIENTED_EDGE ( 'NONE', *, *, #30863, .T. ) ;
#74103=CARTESIAN_POINT ( 'NONE',  ( 164.1745675548848737, 246.6954794637676116, -4.690626445906736386 ) ) ;
#74104=CARTESIAN_POINT ( 'NONE',  ( 163.7064929935861244, 247.0990319366274548, 6.401263337036986023 ) ) ;
#74105=CARTESIAN_POINT ( 'NONE',  ( 192.5049767439991513, 297.2185948999652965, 12.57567268027295881 ) ) ;
#74110=CARTESIAN_POINT ( 'NONE',  ( 174.4548664363482260, 262.3557869890522625, 15.65842366412776165 ) ) ;
#74114=CARTESIAN_POINT ( 'NONE',  ( 149.4908848037268001, 271.7211875819559737, -12.92288068979413573 ) ) ;
#74117=VERTEX_POINT ( 'NONE', #83873 ) ;
#74118=CARTESIAN_POINT ( 'NONE',  ( 177.1952554510797313, 269.3654139093299023, 16.08787487811796169 ) ) ;
#74119=CARTESIAN_POINT ( 'NONE',  ( 164.2801755739368446, 246.1053845600426087, 2.518777461081745717 ) ) ;
#74120=CIRCLE ( 'NONE', #28830, 17.82106496071138224 ) ;
#74121=CARTESIAN_POINT ( 'NONE',  ( 150.9278749657586900, 275.9046242529769870, -8.333285154183892374 ) ) ;
#74123=CARTESIAN_POINT ( 'NONE',  ( 148.9694607950094394, 272.6243204573405592, 11.81236034532910573 ) ) ;
#74124=CARTESIAN_POINT ( 'NONE',  ( 169.0457665943022505, 261.5072838169340343, -16.06598790874472726 ) ) ;
#74125=VERTEX_POINT ( 'NONE', #5341 ) ;
#74126=CARTESIAN_POINT ( 'NONE',  ( 156.7830287337671109, 266.5187050023503161, -16.25525341925989764 ) ) ;
#74130=ORIENTED_EDGE ( 'NONE', *, *, #70725, .F. ) ;
#74135=CARTESIAN_POINT ( 'NONE',  ( 191.2278159864466431, 297.4307022214792937, -10.96893880474589267 ) ) ;
#74138=CARTESIAN_POINT ( 'NONE',  ( 153.4389798490260262, 264.8828863703868137, 16.68923469758090761 ) ) ;
#74140=CARTESIAN_POINT ( 'NONE',  ( 196.9376666616535942, 289.5409507483896618, -17.49204032314444390 ) ) ;
#74142=EDGE_LOOP ( 'NONE', ( #92075, #44643, #35222, #78467 ) ) ;
#74147=CARTESIAN_POINT ( 'NONE',  ( -22.42236680055709641, 157.8615022471902591, 0.000000000000000000 ) ) ;
#74149=ORIENTED_EDGE ( 'NONE', *, *, #98412, .T. ) ;
#74150=CARTESIAN_POINT ( 'NONE',  ( 190.3695739790057075, 300.9172209835572858, 5.653673465233093332 ) ) ;
#74153=CYLINDRICAL_SURFACE ( 'NONE', #86814, 10.00000000000010658 ) ;
#74155=CARTESIAN_POINT ( 'NONE',  ( 160.4591988848097230, 252.7235103201471702, -16.13450096157204072 ) ) ;
#74156=CARTESIAN_POINT ( 'NONE',  ( 148.7027604483410528, 273.0862590081663939, -9.872652348069028250 ) ) ;
#74158=CARTESIAN_POINT ( 'NONE',  ( 208.0006710756887287, 270.3792650189220126, -0.8737665032493013850 ) ) ;
#74162=CARTESIAN_POINT ( 'NONE',  ( 207.5338226493333025, 271.1878702128032614, 6.432541580693135863 ) ) ;
#74163=CARTESIAN_POINT ( 'NONE',  ( 26.27351996285747049, 192.6427522451419634, -10.00000000000009415 ) ) ;
#74164=CARTESIAN_POINT ( 'NONE',  ( 101.9066655502961964, 220.4548013555409511, -4.594050593750042211 ) ) ;
#74165=B_SPLINE_CURVE_WITH_KNOTS ( 'NONE', 3,
 ( #57190, #88170, #26315, #60050 ),
 .UNSPECIFIED., .F., .F.,
 ( 4, 4 ),
 ( 0.04063817219314667939, 0.04887120950165274591 ),
 .UNSPECIFIED. ) ;
#74166=CARTESIAN_POINT ( 'NONE',  ( 183.0594061691496961, 295.7039273298110515, -2.683685864958768708 ) ) ;
#74167=CARTESIAN_POINT ( 'NONE',  ( 167.2887110157984125, 281.5736242869099897, -10.92832022129961977 ) ) ;
#74168=CARTESIAN_POINT ( 'NONE',  ( 190.1114827020009841, 297.9905665084500583, 9.484015614658840576 ) ) ;
#74170=CARTESIAN_POINT ( 'NONE',  ( 15.22267496842377099, 179.5958772461660544, -9.188101187500095079 ) ) ;
#74172=EDGE_LOOP ( 'NONE', ( #90342, #59150, #40906, #2971 ) ) ;
#74173=VERTEX_POINT ( 'NONE', #98557 ) ;
#74176=( BOUNDED_CURVE ( )  B_SPLINE_CURVE ( 2, ( #16199, #10607, #32890, #17189, #79549, #18211, #70393 ),
 .UNSPECIFIED., .F., .F. ) 
 B_SPLINE_CURVE_WITH_KNOTS ( ( 3, 2, 2, 3 ),
 ( 0.9717741935483871218, 0.9731182795698924970, 0.9758064516129032473, 0.9784858563273379772 ),
 .UNSPECIFIED. ) 
 CURVE ( )  GEOMETRIC_REPRESENTATION_ITEM ( )  RATIONAL_B_SPLINE_CURVE ( ( 0.9330127018922194093, 0.9330127018922194093, 1.000000000000000000, 0.8660254037844387076, 1.000000000000000000, 0.8664623547262191305, 0.9991289483004428540 ) ) 
 REPRESENTATION_ITEM ( '' )  );
#74177=DIRECTION ( 'NONE',  ( 0.4999999999999992784, -0.8660254037844390407, 0.000000000000000000 ) ) ;
#74178=CARTESIAN_POINT ( 'NONE',  ( 190.1858949294064871, 301.2353624297489887, -5.249932979468886707 ) ) ;
#74179=CARTESIAN_POINT ( 'NONE',  ( 205.6103970483690659, 272.1329265362093111, -9.537080485986734857 ) ) ;
#74180=ADVANCED_FACE ( 'NONE', ( #90488 ), #75735, .F. ) ;
#74182=CARTESIAN_POINT ( 'NONE',  ( 176.1186201279473096, 285.3276135723396578, -12.10217071624021123 ) ) ;
#74184=CARTESIAN_POINT ( 'NONE',  ( 51.92050145378936321, 200.7833772461660828, -9.188101187500095079 ) ) ;
#74185=CARTESIAN_POINT ( 'NONE',  ( 96.42157766939699570, 233.1427522451419065, -10.00000000000009415 ) ) ;
#74186=AXIS2_PLACEMENT_3D ( 'NONE', #23289, #29903, #8606 ) ;
#74190=CARTESIAN_POINT ( 'NONE',  ( 180.0250856602858960, 259.9265448933365974, -10.32933125829473830 ) ) ;
#74193=CARTESIAN_POINT ( 'NONE',  ( -7.294332625736644538, 178.8464784336661637, 1.353441290958777327E-15 ) ) ;
#74194=AXIS2_PLACEMENT_3D ( 'NONE', #49811, #73135, #27526 ) ;
#74195=CARTESIAN_POINT ( 'NONE',  ( 150.7133245577828689, 269.6038598187387834, -14.58664962216439598 ) ) ;
#74197=CARTESIAN_POINT ( 'NONE',  ( 146.9370072200009645, 276.1446333132804511, -3.799807221059707363 ) ) ;
#74199=CARTESIAN_POINT ( 'NONE',  ( 55.46605327235566563, 193.6423013555410080, -4.594050593750043987 ) ) ;
#74200=CARTESIAN_POINT ( 'NONE',  ( 164.3053959849042087, 246.0617015268593661, -7.251939739328854273 ) ) ;
#74201=CARTESIAN_POINT ( 'NONE',  ( 204.9768178125733016, 275.6167325052707611, 13.98665089523138505 ) ) ;
#74203=CARTESIAN_POINT ( 'NONE',  ( 189.8171280724701546, 301.8740853621098950, -0.4360232994423257624 ) ) ;
#74204=ORIENTED_EDGE ( 'NONE', *, *, #84985, .F. ) ;
#74205=VECTOR ( 'NONE', #31675, 1000.000000000000000 ) ;
#74206=CARTESIAN_POINT ( 'NONE',  ( -2.070769811622779510, 169.6115022471902591, 10.00000000000009592 ) ) ;
#74208=CARTESIAN_POINT ( 'NONE',  ( 114.8152493078691947, 249.3464784336661637, 1.353441290958777327E-15 ) ) ;
#74210=CARTESIAN_POINT ( 'NONE',  ( 164.2882413842225731, 246.0914141668236539, 1.641966415049095795 ) ) ;
#74212=CARTESIAN_POINT ( 'NONE',  ( 191.2104420009116836, 280.2857515794617598, 17.80337293751487593 ) ) ;
#74214=CARTESIAN_POINT ( 'NONE',  ( 186.5015629097202918, 288.3730187221656820, 14.57764263923063019 ) ) ;
#74215=B_SPLINE_CURVE_WITH_KNOTS ( 'NONE', 3,
 ( #71412, #18209, #24786, #18707 ),
 .UNSPECIFIED., .F., .F.,
 ( 4, 4 ),
 ( 0.03463969976448799670, 0.04344658197601434374 ),
 .UNSPECIFIED. ) ;
#74218=B_SPLINE_CURVE_WITH_KNOTS ( 'NONE', 3,
 ( #45816, #84877, #69131, #98576, #99555, #68138, #68634, #29159, #99066, #14926, #23518, #38215, #21556, #60030, #29648, #15417, #46314, #22042, #7844, #52937, #83890, #45333, #30138, #61022, #86397, #24030, #63035, #94475, #10353, #33656, #16929, #54929, #48344, #64544, #31617, #56927, #79788, #47816, #87914, #78754, #17437, #95505, #40722, #9341, #85907, #16433, #2766, #26053, #86902, #56433 ),
 .UNSPECIFIED., .F., .F.,
 ( 4, 2, 2, 2, 2, 2, 2, 2, 2, 2, 2, 2, 2, 2, 2, 2, 2, 2, 2, 2, 2, 2, 2, 2, 4 ),
 ( 0.0002266190613796248594, 0.0007024597989655380478, 0.001178300536551451236, 0.001416220905344407885, 0.001535181089740794052, 0.001654141274137180435, 0.001773101458533567036, 0.001892061642929953203, 0.002129982011722625791, 0.002605822749307888566, 0.003081663486893151341, 0.004033344962063676459, 0.004985026437234200275, 0.005460867174819500347, 0.005698787543612112219, 0.005817747728008340960, 0.005936707912404571436, 0.005996188004602654581, 0.006055668096800735992, 0.006174628281196945651, 0.006412548649989363234, 0.006888389387574264319, 0.007126309756366766904, 0.007364230125159267754, 0.007840070862744271188 ),
 .UNSPECIFIED. ) ;
#74219=CARTESIAN_POINT ( 'NONE',  ( 150.8167050463783312, 269.4247995599803289, 14.38040671671637938 ) ) ;
#74220=CARTESIAN_POINT ( 'NONE',  ( 208.3800376108834485, 269.7221829052733142, -1.355162556537697904 ) ) ;
#74221=CARTESIAN_POINT ( 'NONE',  ( 181.3897897703101023, 287.9624256778719200, 13.95846517440433310 ) ) ;
#74222=CARTESIAN_POINT ( 'NONE',  ( 172.3266757524851300, 267.7393374298979438, -16.32508309337648811 ) ) ;
#74223=CARTESIAN_POINT ( 'NONE',  ( 196.2038536313239661, 272.5484090068244427, -13.37539213265573146 ) ) ;
#74226=CARTESIAN_POINT ( 'NONE',  ( 171.2941760164128198, 284.5531234145211670, -11.44789784273924838 ) ) ;
#74229=CARTESIAN_POINT ( 'NONE',  ( 205.2127215196890120, 270.8542949291791047, -7.926103670997396655 ) ) ;
#74230=CARTESIAN_POINT ( 'NONE',  ( 185.8682827460642670, 296.7038206768884265, 4.702033971577086469 ) ) ;
#74243=CARTESIAN_POINT ( 'NONE',  ( 158.4984048909838634, 263.4026134211973726, -17.02607271676052392 ) ) ;
#74244=ORIENTED_EDGE ( 'NONE', *, *, #83368, .T. ) ;
#74245=FACE_OUTER_BOUND ( 'NONE', #36684, .T. ) ;
#74247=CARTESIAN_POINT ( 'NONE',  ( 164.4864504671816690, 245.7481059646165704, 6.337356894698421783 ) ) ;
#74248=CARTESIAN_POINT ( 'NONE',  ( 162.5887743522035294, 284.9919049736276975, -2.844505511527740005 ) ) ;
#74251=CARTESIAN_POINT ( 'NONE',  ( 83.09741599002914825, 218.7833772461660544, -9.188101187500095079 ) ) ;
#74252=CARTESIAN_POINT ( 'NONE',  ( 155.3607606009346398, 261.5542644670730965, 17.00535455698268095 ) ) ;
#74257=ORIENTED_EDGE ( 'NONE', *, *, #55587, .T. ) ;
#74258=LINE ( 'NONE', #96580, #83829 ) ;
#74259=VERTEX_POINT ( 'NONE', #88389 ) ;
#74260=CARTESIAN_POINT ( 'NONE',  ( 167.8099530253072089, 271.3928698661641761, -17.53051755021046532 ) ) ;
#74261=CARTESIAN_POINT ( 'NONE',  ( 156.6812872898450735, 261.2670451491295012, 0.000000000000000000 ) ) ;
#74262=VERTEX_POINT ( 'NONE', #65027 ) ;
#74263=B_SPLINE_CURVE_WITH_KNOTS ( 'NONE', 3,
 ( #86759, #56789, #87775, #2110, #17293, #48195, #95364, #25395, #79143, #32992, #63894, #94832, #56282, #87281, #17812, #48713, #79644, #10210, #41075, #72012, #2617, #8264, #31047, #99477, #39128, #54329, #15335, #52852, #75676, #91903, #59946, #91394, #61934, #7248, #98980, #22945, #60438, #92398, #6763, #76660, #22458, #46230, #83802, #30053, #84303, #83302, #38650, #14367, #90917, #29564, #21959, #70042 ),
 .UNSPECIFIED., .F., .F.,
 ( 4, 2, 2, 2, 2, 2, 2, 2, 2, 2, 2, 2, 2, 2, 2, 2, 2, 2, 2, 2, 2, 2, 2, 2, 2, 4 ),
 ( 0.0001479525476070201362, 0.0006328501284903549802, 0.001117747709373689878, 0.001360196499815357436, 0.001481420895036139824, 0.001602645290256922211, 0.001723869685477704815, 0.001845094080698487203, 0.001966318475919270024, 0.002087542871140052412, 0.002572440452022936499, 0.003057338032905820152, 0.004027133194671691542, 0.004996928356437562932, 0.005481825937320463499, 0.005724274727761836587, 0.005845499122982446803, 0.005966723518203056152, 0.006027335715813398991, 0.006087947913423741829, 0.006209172308644423169, 0.006451621099085631458, 0.006936518679968144314, 0.007178967470409401176, 0.007421416260850658038, 0.007906313841733193445 ),
 .UNSPECIFIED. ) ;
#74264=CARTESIAN_POINT ( 'NONE',  ( 207.5070909066002116, 271.2341709493916255, -7.107478141010028949 ) ) ;
#74265=EDGE_CURVE ( 'NONE', #84750, #4766, #34653, .T. ) ;
#74269=CARTESIAN_POINT ( 'NONE',  ( 152.8721808860877616, 265.8646109718731623, -17.65676496037632504 ) ) ;
#74273=CARTESIAN_POINT ( 'NONE',  ( 138.9021014942714487, 244.8768266524159856, 9.188101187500098632 ) ) ;
#74274=CARTESIAN_POINT ( 'NONE',  ( 168.1505723841142128, 267.0769752754364390, -17.55733195497056798 ) ) ;
#74275=ORIENTED_EDGE ( 'NONE', *, *, #22452, .T. ) ;
#74282=CARTESIAN_POINT ( 'NONE',  ( 200.2816180127317125, 270.3372598560825395, 9.268223811809287227 ) ) ;
#74284=CARTESIAN_POINT ( 'NONE',  ( 2.117331368781439682, 160.4824982072973683, 3.021315404115420679E-15 ) ) ;
#74285=CARTESIAN_POINT ( 'NONE',  ( 170.7320525446532713, 288.3325263888784207, -5.627708583524104746 ) ) ;
#74286=CARTESIAN_POINT ( 'NONE',  ( 160.6734846709049691, 282.6943762970620924, -6.583290857611773461 ) ) ;
#74288=CARTESIAN_POINT ( 'NONE',  ( 157.8323084318549547, 257.8542024558915955, 16.74327773638376726 ) ) ;
#74289=DIRECTION ( 'NONE',  ( -0.5000000000000006661, 0.8660254037844382635, -1.877843081442121204E-16 ) ) ;
#74293=CARTESIAN_POINT ( 'NONE',  ( 181.5913590924892560, 271.3060279288629317, -15.97644946730743598 ) ) ;
#74295=ORIENTED_EDGE ( 'NONE', *, *, #81114, .F. ) ;
#74296=CARTESIAN_POINT ( 'NONE',  ( 160.6982348739816757, 275.7565010011308004, 12.80364755394902687 ) ) ;
#74297=CARTESIAN_POINT ( 'NONE',  ( 173.4859908262079955, 280.5480941373698442, -14.23958667651489129 ) ) ;
#74301=CARTESIAN_POINT ( 'NONE',  ( 160.8321869569444971, 272.7815025554300519, 15.68266994514650214 ) ) ;
#74312=CARTESIAN_POINT ( 'NONE',  ( 192.7693357657653053, 296.7607116428271183, 12.22606306887835714 ) ) ;
#74315=CARTESIAN_POINT ( 'NONE',  ( 7.590999645455913658, 169.0643266524160140, -9.188101187500093303 ) ) ;
#74316=CARTESIAN_POINT ( 'NONE',  ( 98.90203251333015544, 240.1589784336661637, -6.496448406907675876E-16 ) ) ;
#74318=CARTESIAN_POINT ( 'NONE',  ( 186.6730029007337919, 295.8052390787480022, -7.682216135788281441 ) ) ;
#74321=FACE_OUTER_BOUND ( 'NONE', #39287, .T. ) ;
#74322=CARTESIAN_POINT ( 'NONE',  ( 194.6310785344323904, 293.5360785768717165, -14.54510914272505495 ) ) ;
#74324=CARTESIAN_POINT ( 'NONE',  ( 196.2517347386735480, 266.7219944345126237, 8.057602692514423737 ) ) ;
#74326=CARTESIAN_POINT ( 'NONE',  ( 66.95321124882991626, 197.9155109091896350, 2.679491924311254714 ) ) ;
#74327=CARTESIAN_POINT ( 'NONE',  ( 172.6066657261125101, 263.4582241914548604, -15.40626036171160607 ) ) ;
#74328=CARTESIAN_POINT ( 'NONE',  ( 75.46539357129627490, 220.5024278399160664, -9.188101187500093303 ) ) ;
#74330=CARTESIAN_POINT ( 'NONE',  ( 190.8443993347725325, 300.0947993426467519, 8.522468760355437212 ) ) ;
#74333=CARTESIAN_POINT ( 'NONE',  ( 196.4677418905696129, 290.3548843276421394, 17.08610552292358520 ) ) ;
#74334=CARTESIAN_POINT ( 'NONE',  ( 152.3580564471173489, 266.7551006215829261, 15.57995064934159046 ) ) ;
#74335=CARTESIAN_POINT ( 'NONE',  ( 197.0269530679106254, 289.3863021563271900, 16.70650816643942704 ) ) ;
#74336=CARTESIAN_POINT ( 'NONE',  ( 198.7357616895271804, 286.4265588032756114, -17.04018524297827497 ) ) ;
#74339=CARTESIAN_POINT ( 'NONE',  ( 147.2658550951450422, 275.5750520855697800, -5.215660180131691526 ) ) ;
#74340=CARTESIAN_POINT ( 'NONE',  ( -3.985554314188680003, 180.0530062829863311, 2.649461200531984646E-14 ) ) ;
#74344=CARTESIAN_POINT ( 'NONE',  ( 172.4419760422836134, 290.9306500000749907, -0.6531725299933459628 ) ) ;
#74345=CARTESIAN_POINT ( 'NONE',  ( 192.4259603496955719, 297.3554553095298729, -12.40738485318142814 ) ) ;
#74350=CARTESIAN_POINT ( 'NONE',  ( 198.2489255580726422, 287.2697837179150042, 18.53597557040773225 ) ) ;
#74351=CARTESIAN_POINT ( 'NONE',  ( 157.8111766759666068, 268.3688148911334110, 16.25763562993056510 ) ) ;
#74352=EDGE_CURVE ( 'NONE', #41536, #42536, #70909, .T. ) ;
#74353=CARTESIAN_POINT ( 'NONE',  ( 184.5341303888194773, 280.6061766946581315, -17.60036545423847087 ) ) ;
#74356=CARTESIAN_POINT ( 'NONE',  ( 136.8541387121308901, 256.4865022471902876, -10.00000000000009415 ) ) ;
#74357=CARTESIAN_POINT ( 'NONE',  ( 204.9658583905037688, 275.6357147811169170, -12.57240504404813564 ) ) ;
#74359=EDGE_LOOP ( 'NONE', ( #95098, #41048, #98669 ) ) ;
#74361=CARTESIAN_POINT ( 'NONE',  ( 167.3097680743688613, 247.9456010488782454, -1.868104155933442145 ) ) ;
#74362=ORIENTED_EDGE ( 'NONE', *, *, #58942, .T. ) ;
#74364=DIRECTION ( 'NONE',  ( -0.8660254037844387076, -0.4999999999999998890, -0.000000000000000000 ) ) ;
#74369=CARTESIAN_POINT ( 'NONE',  ( 190.2861294957589564, 290.5072236206235061, 14.49960583659686009 ) ) ;
#74370=CARTESIAN_POINT ( 'NONE',  ( 205.8468767641892043, 274.1097461954921073, 10.74163015103096797 ) ) ;
#74371=CARTESIAN_POINT ( 'NONE',  ( 157.5215017335775940, 258.4853116787141971, -16.92298772477023761 ) ) ;
#74376=DIRECTION ( 'NONE',  ( 0.4999999999999998890, -0.8660254037844385966, 0.000000000000000000 ) ) ;
#74379=ORIENTED_EDGE ( 'NONE', *, *, #71324, .F. ) ;
#74382=FACE_OUTER_BOUND ( 'NONE', #64031, .T. ) ;
#74383=CARTESIAN_POINT ( 'NONE',  ( 162.7122087945529927, 272.4192740586219657, -15.63422411579954563 ) ) ;
#74385=DIRECTION ( 'NONE',  ( 0.5000000000000048850, -0.8660254037844358210, 0.000000000000000000 ) ) ;
#74386=CARTESIAN_POINT ( 'NONE',  ( 160.9155581428462085, 282.2930683307629920, -7.657675304491033508 ) ) ;
#74388=CARTESIAN_POINT ( 'NONE',  ( 170.3564602903425111, 288.9689526880741823, -4.407563815828527964 ) ) ;
#74389=CARTESIAN_POINT ( 'NONE',  ( 159.2720798248943765, 273.8135256516483764, -15.04173180978755298 ) ) ;
#74390=CARTESIAN_POINT ( 'NONE',  ( 178.9144291139083975, 255.9268924588826621, 4.886238089006308627 ) ) ;
#74391=CARTESIAN_POINT ( 'NONE',  ( 102.5290345353249961, 223.8768266524159856, 9.188101187500098632 ) ) ;
#74394=CARTESIAN_POINT ( 'NONE',  ( 192.0603001030472683, 293.3461588932823929, -14.68827779892621344 ) ) ;
#74395=ORIENTED_EDGE ( 'NONE', *, *, #49575, .T. ) ;
#74397=CARTESIAN_POINT ( 'NONE',  ( 186.8003541658358984, 299.2222177555264011, -0.6103433986344138917 ) ) ;
#74399=CARTESIAN_POINT ( 'NONE',  ( 164.2183954753924979, 249.9265173926981163, 10.12780430522023423 ) ) ;
#74400=CARTESIAN_POINT ( 'NONE',  ( 159.3586121662929713, 254.6297824347537642, -15.50090345830412630 ) ) ;
#74401=CARTESIAN_POINT ( 'NONE',  ( 163.1611253217825492, 248.0436364529968216, 11.42797785440508029 ) ) ;
#74404=CARTESIAN_POINT ( 'NONE',  ( 163.3020905273760093, 247.7994775548095845, -11.05431316445765155 ) ) ;
#74408=CARTESIAN_POINT ( 'NONE',  ( 193.8703746310723943, 265.8671889252453866, -7.747450020969885109 ) ) ;
#74409=CARTESIAN_POINT ( 'NONE',  ( 153.2832131836460121, 266.4580806215291773, 16.33893799534572722 ) ) ;
#74410=ADVANCED_FACE ( 'NONE', ( #65515 ), #30433, .F. ) ;
#74412=CARTESIAN_POINT ( 'NONE',  ( 136.0332187963529975, 249.3458772461660544, 9.188101187500095079 ) ) ;
#74416=CARTESIAN_POINT ( 'NONE',  ( 190.6954410837624607, 300.3528026016029457, -5.728531842148099962 ) ) ;
#74417=CYLINDRICAL_SURFACE ( 'NONE', #77231, 10.00000000000010658 ) ;
#74418=CARTESIAN_POINT ( 'NONE',  ( 206.7408728089182546, 272.5612996242556960, -10.63134519248043475 ) ) ;
#74420=CARTESIAN_POINT ( 'NONE',  ( 39.49844957003027446, 193.6115022471902591, 10.00000000000009592 ) ) ;
#74422=ADVANCED_FACE ( 'NONE', ( #59383 ), #50806, .T. ) ;
#74423=CARTESIAN_POINT ( 'NONE',  ( 199.0467776771448882, 281.9810065596747108, -16.63176243157295175 ) ) ;
#74424=CYLINDRICAL_SURFACE ( 'NONE', #70542, 10.00000000000010658 ) ;
#74427=CARTESIAN_POINT ( 'NONE',  ( 55.22204975783502334, 208.8149278399160664, 9.188101187500093303 ) ) ;
#74428=CARTESIAN_POINT ( 'NONE',  ( 167.6185327982364015, 249.9494983323436088, 7.055657055613346884 ) ) ;
#74430=CARTESIAN_POINT ( 'NONE',  ( 162.9383752892161397, 248.4294508267893491, -11.25953730674605957 ) ) ;
#74431=EDGE_CURVE ( 'NONE', #42198, #54426, #10439, .T. ) ;
#74437=CARTESIAN_POINT ( 'NONE',  ( 172.9698904924519240, 250.6642211707864476, -4.168778760986519671 ) ) ;
#74440=CARTESIAN_POINT ( 'NONE',  ( 157.6510097567892501, 270.8399773495983709, -14.84913773220146993 ) ) ;
#74442=CARTESIAN_POINT ( 'NONE',  ( 161.0965315767822972, 251.6196177163260188, -13.76772246540905442 ) ) ;
#74443=CARTESIAN_POINT ( 'NONE',  ( 13.49027706508988267, 190.8464784336661637, 1.353441290958777327E-15 ) ) ;
#74447=CARTESIAN_POINT ( 'NONE',  ( 181.0686324902563911, 280.4193002135394295, 17.28172028329132104 ) ) ;
#74448=CARTESIAN_POINT ( 'NONE',  ( 208.1876422586379647, 270.0554214305024630, 3.377638779759113863 ) ) ;
#74450=CARTESIAN_POINT ( 'NONE',  ( 42.85403768609726427, 204.7369531367911293, -4.594050593750048428 ) ) ;
#74452=CARTESIAN_POINT ( 'NONE',  ( 199.2205425252482200, 285.5868937652708155, -18.05012564782189344 ) ) ;
#74453=CARTESIAN_POINT ( 'NONE',  ( 190.2648877593310317, 301.0985428348857340, -4.426259207433023590 ) ) ;
#74455=CARTESIAN_POINT ( 'NONE',  ( 203.0676174199914215, 269.8692695890372306, -7.319173559847955701 ) ) ;
#74456=CARTESIAN_POINT ( 'NONE',  ( 178.8150194001607360, 293.5229817246915331, 2.654719043459385031 ) ) ;
#74457=CARTESIAN_POINT ( 'NONE',  ( 180.0213682611045556, 276.4079177606270150, 16.56764346391123510 ) ) ;
#74458=CARTESIAN_POINT ( 'NONE',  ( 180.2261984326610218, 279.1782745765357276, -17.42438828499370729 ) ) ;
#74461=CARTESIAN_POINT ( 'NONE',  ( 167.0953271602620305, 257.8792139306702893, -15.57180271813312444 ) ) ;
#74463=CARTESIAN_POINT ( 'NONE',  ( 96.65612621980328356, 216.6115022471901739, -5.000000000000041744 ) ) ;
#74464=( BOUNDED_CURVE ( )  B_SPLINE_CURVE ( 2, ( #99315, #29894, #68880, #59789, #59276, #90253, #20826, #13225, #75022 ),
 .UNSPECIFIED., .F., .T. ) 
 B_SPLINE_CURVE_WITH_KNOTS ( ( 3, 2, 2, 2, 3 ),
 ( 0.06048387096774193727, 0.06182795698924731242, 0.06451612903225806273, 0.06720430107526881303, 0.06854838709677418818 ),
 .UNSPECIFIED. ) 
 CURVE ( )  GEOMETRIC_REPRESENTATION_ITEM ( )  RATIONAL_B_SPLINE_CURVE ( ( 0.9330127018922194093, 0.9330127018922194093, 1.000000000000000000, 0.8660254037844387076, 1.000000000000000000, 0.8660254037844387076, 1.000000000000000000, 0.9330127018922194093, 0.9330127018922194093 ) ) 
 REPRESENTATION_ITEM ( '' )  );
#74466=CARTESIAN_POINT ( 'NONE',  ( 165.2649712138198481, 269.7723956468109350, -16.27622833696107918 ) ) ;
#74468=CARTESIAN_POINT ( 'NONE',  ( 46.94050828626382099, 210.1589784336661637, -6.496448406907675876E-16 ) ) ;
#74469=ORIENTED_EDGE ( 'NONE', *, *, #33309, .F. ) ;
#74471=CARTESIAN_POINT ( 'NONE',  ( 190.4240181651484818, 300.8229208869809668, -4.214281362166949485 ) ) ;
#74474=EDGE_CURVE ( 'NONE', #70064, #33315, #35727, .T. ) ;
#74476=CARTESIAN_POINT ( 'NONE',  ( 59.82969263072505584, 216.8967562850347122, -4.648177544792955347E-16 ) ) ;
#74477=CARTESIAN_POINT ( 'NONE',  ( 207.1122325394003951, 271.9180857031755636, 7.794245785756032774 ) ) ;
#74482=CARTESIAN_POINT ( 'NONE',  ( 204.2956748066270620, 276.7965067987898919, 13.85972809245231119 ) ) ;
#74489=CARTESIAN_POINT ( 'NONE',  ( 182.5376139826708197, 283.9547259621338071, 16.22153700475692517 ) ) ;
#74490=CARTESIAN_POINT ( 'NONE',  ( 191.4685399627163633, 299.0137560639802814, 7.545791216288330716 ) ) ;
#74491=CARTESIAN_POINT ( 'NONE',  ( 159.8732321751776624, 253.7384344327741132, -15.51998349828054202 ) ) ;
#74493=EDGE_LOOP ( 'NONE', ( #64403, #82857, #73138, #76388 ) ) ;
#74494=CARTESIAN_POINT ( 'NONE',  ( 161.8807657183444064, 250.2612843381103573, -13.52770735624900311 ) ) ;
#74496=CARTESIAN_POINT ( 'NONE',  ( 181.4204268205617154, 259.5203828285251006, -11.17471347674236348 ) ) ;
#74497=VERTEX_POINT ( 'NONE', #99916 ) ;
#74499=CARTESIAN_POINT ( 'NONE',  ( 197.9552487813401456, 287.7784468162186613, 17.26493623863614602 ) ) ;
#74500=DIRECTION ( 'NONE',  ( -0.8660254037844387076, -0.4999999999999998890, -0.000000000000000000 ) ) ;
#74502=CARTESIAN_POINT ( 'NONE',  ( 125.6948669907937415, 249.5024278399160664, 9.188101187500095079 ) ) ;
#74506=CARTESIAN_POINT ( 'NONE',  ( 163.7038023771459052, 247.1036922210055025, -6.448491958542482472 ) ) ;
#74507=ORIENTED_EDGE ( 'NONE', *, *, #28717, .F. ) ;
#74509=CARTESIAN_POINT ( 'NONE',  ( 198.3075590527773784, 287.1682275260610027, 16.94807365630277118 ) ) ;
#74510=CARTESIAN_POINT ( 'NONE',  ( 170.3127733705114224, 263.9010670580030364, 17.23448983536806622 ) ) ;
#74511=CARTESIAN_POINT ( 'NONE',  ( 67.50895872190925218, 209.7833772461660544, -9.188101187500095079 ) ) ;
#74512=DIRECTION ( 'NONE',  ( -0.8660254037844387076, -0.4999999999999998890, -0.000000000000000000 ) ) ;
#74515=CARTESIAN_POINT ( 'NONE',  ( 175.8011943468589777, 278.1488512039077818, 16.59015806188801889 ) ) ;
#74520=CARTESIAN_POINT ( 'NONE',  ( 201.1060504099706350, 282.3210983108598384, -18.18000168485860257 ) ) ;
#74521=CARTESIAN_POINT ( 'NONE',  ( 203.3041373168503299, 278.5139001086923827, -16.61929732091214973 ) ) ;
#74522=ORIENTED_EDGE ( 'NONE', *, *, #29949, .T. ) ;
#74525=CARTESIAN_POINT ( 'NONE',  ( 174.0330057339203336, 253.5070743419241523, -7.570545654136764391 ) ) ;
#74526=CARTESIAN_POINT ( 'NONE',  ( 165.7625844681755325, 272.7524946119172569, 16.99070308655728923 ) ) ;
#74527=CARTESIAN_POINT ( 'NONE',  ( 164.7762319088960794, 245.2461897844768828, 2.994040459560653122 ) ) ;
#74529=CARTESIAN_POINT ( 'NONE',  ( 196.2293283710122012, 290.7678286567270902, -17.07152402978540096 ) ) ;
#74530=CARTESIAN_POINT ( 'NONE',  ( 45.19978347827786536, 190.2365022471902023, 10.00000000000009948 ) ) ;
#74531=CARTESIAN_POINT ( 'NONE',  ( 208.0045976720423084, 270.3724639545367836, 2.002128742561712471 ) ) ;
#74532=CARTESIAN_POINT ( 'NONE',  ( 135.5734031224162663, 239.8923013555409796, 4.594050593750050204 ) ) ;
#74533=ORIENTED_EDGE ( 'NONE', *, *, #46625, .T. ) ;
#74535=CARTESIAN_POINT ( 'NONE',  ( 183.5087089432283278, 257.8196472444194569, 6.855898145921591968 ) ) ;
#74538=CARTESIAN_POINT ( 'NONE',  ( 163.9587364689194260, 246.6621334214722481, 5.816126667419880825 ) ) ;
#74541=EDGE_LOOP ( 'NONE', ( #16407, #98420, #18195, #95217 ) ) ;
#74543=CARTESIAN_POINT ( 'NONE',  ( 182.0998708099376131, 275.6965794993143390, -16.43372495111283627 ) ) ;
#74545=CARTESIAN_POINT ( 'NONE',  ( 36.81016237556819704, 185.3927522451417929, -10.00000000000009237 ) ) ;
#74546=CARTESIAN_POINT ( 'NONE',  ( 202.5541353527785873, 267.6455170340615268, 0.8630784805652055303 ) ) ;
#74548=CARTESIAN_POINT ( 'NONE',  ( 199.0384395528189430, 265.2940482796883543, 0.1310837649599854438 ) ) ;
#74549=B_SPLINE_CURVE_WITH_KNOTS ( 'NONE', 3,
 ( #45325, #76259, #14444, #6344 ),
 .UNSPECIFIED., .F., .F.,
 ( 4, 4 ),
 ( 0.008293070909132364485, 0.01460849775743500514 ),
 .UNSPECIFIED. ) ;
#74550=CARTESIAN_POINT ( 'NONE',  ( 190.4976253092930278, 300.6954295735222900, -5.764807383508308902 ) ) ;
#74552=CARTESIAN_POINT ( 'NONE',  ( 204.7242223814549504, 276.0542406257275161, -13.93608974681376189 ) ) ;
#74553=CARTESIAN_POINT ( 'NONE',  ( 196.3531155526046632, 270.6521786943779375, 11.87296120750966466 ) ) ;
#74554=EDGE_CURVE ( 'NONE', #40233, #25756, #96687, .T. ) ;
#74557=CARTESIAN_POINT ( 'NONE',  ( 190.0259678364800493, 301.5123642802043946, 4.004183174499006626 ) ) ;
#74558=CARTESIAN_POINT ( 'NONE',  ( 205.0967303340277681, 274.5205728753008430, 11.66379712794152645 ) ) ;
#74560=CYLINDRICAL_SURFACE ( 'NONE', #70578, 10.00000000000010658 ) ;
#74562=CARTESIAN_POINT ( 'NONE',  ( 139.3620039403754731, 251.2677522451418497, 10.00000000000009592 ) ) ;
#74563=CARTESIAN_POINT ( 'NONE',  ( 172.5346649401163290, 284.2238562735757910, -12.87557711212363110 ) ) ;
#74566=CARTESIAN_POINT ( 'NONE',  ( 198.5511052797322975, 286.7463930869835167, -17.24711022262289006 ) ) ;
#74567=CARTESIAN_POINT ( 'NONE',  ( -12.81524457486244550, 175.6589784336661637, -6.496448406907676862E-16 ) ) ;
#74568=CARTESIAN_POINT ( 'NONE',  ( 56.08842225738448661, 197.0643266524160140, 9.188101187500095079 ) ) ;
#74569=CARTESIAN_POINT ( 'NONE',  ( 176.0198054981916869, 257.3513611390321216, -10.51569790059619791 ) ) ;
#74572=CARTESIAN_POINT ( 'NONE',  ( 205.4029933437358295, 274.8785748323546159, -13.50815392427034922 ) ) ;
#74573=CARTESIAN_POINT ( 'NONE',  ( 192.5606481657753761, 292.4750250043705933, -14.28755835911418082 ) ) ;
#74574=CARTESIAN_POINT ( 'NONE',  ( 150.0363948880720102, 276.4654116368551513, 3.707458508793961993 ) ) ;
#74575=EDGE_CURVE ( 'NONE', #79277, #86358, #16339, .T. ) ;
#74576=CARTESIAN_POINT ( 'NONE',  ( 167.4736906045900184, 256.7023835675479972, 14.85217472785100945 ) ) ;
#74578=CARTESIAN_POINT ( 'NONE',  ( 150.4319008355389542, 270.0913000041206260, 13.83804576328048697 ) ) ;
#74580=CARTESIAN_POINT ( 'NONE',  ( 65.04619898167126735, 198.3615022471901739, 5.000000000000051514 ) ) ;
#74581=CARTESIAN_POINT ( 'NONE',  ( 181.9590579474959213, 291.6908273499842039, 9.324365134751094075 ) ) ;
#74582=CARTESIAN_POINT ( 'NONE',  ( 202.6551236945213361, 279.6380246773706517, 15.55476940527561425 ) ) ;
#74583=CARTESIAN_POINT ( 'NONE',  ( 13.16551753867071461, 190.6589784336661921, -6.496448406907675876E-16 ) ) ;
#74584=CARTESIAN_POINT ( 'NONE',  ( 167.8811029522163096, 286.0887665112138052, 4.087334010221439939 ) ) ;
#74585=CARTESIAN_POINT ( 'NONE',  ( 2.672015980952107572, 183.8967562850347122, -4.648177544792955347E-16 ) ) ;
#74588=CARTESIAN_POINT ( 'NONE',  ( 144.8954975894293682, 242.9155109091896065, 2.679491924311254714 ) ) ;
#74589=CARTESIAN_POINT ( 'NONE',  ( 179.8745906151779081, 276.9455922838650395, 16.30155377088923885 ) ) ;
#74592=CARTESIAN_POINT ( 'NONE',  ( 148.9776469710554920, 275.4404107866210438, 7.585097431987186667 ) ) ;
#74593=B_SPLINE_CURVE_WITH_KNOTS ( 'NONE', 3,
 ( #40264, #56479, #1796, #33701, #95546, #24080, #54976, #85954, #32680, #39750, #1293, #32178 ),
 .UNSPECIFIED., .F., .F.,
 ( 4, 2, 2, 2, 2, 4 ),
 ( 0.001410800830378118077, 0.001612464706955823394, 0.001814128583533528927, 0.002217456336688934139, 0.002620784089844339568, 0.003024111842999744563 ),
 .UNSPECIFIED. ) ;
#74594=B_SPLINE_CURVE_WITH_KNOTS ( 'NONE', 3,
 ( #8408, #47395, #77824, #9921 ),
 .UNSPECIFIED., .F., .F.,
 ( 4, 4 ),
 ( 0.007261002233767476638, 0.01303800565229685030 ),
 .UNSPECIFIED. ) ;
#74595=CARTESIAN_POINT ( 'NONE',  ( 176.7509313491396483, 260.7307399239896313, -13.19623395499003848 ) ) ;
#74600=CARTESIAN_POINT ( 'NONE',  ( 159.5946725794669021, 258.6821552202987391, 17.29432174323186189 ) ) ;
#74601=EDGE_CURVE ( 'NONE', #76651, #69911, #59819, .T. ) ;
#74602=CARTESIAN_POINT ( 'NONE',  ( 193.7275870247597425, 295.1009717758319084, 14.48058678254265885 ) ) ;
#74603=ORIENTED_EDGE ( 'NONE', *, *, #78197, .F. ) ;
#74604=CARTESIAN_POINT ( 'NONE',  ( 181.5287477823910365, 289.3008137216033333, 12.67257242005390161 ) ) ;
#74605=CARTESIAN_POINT ( 'NONE',  ( 16.56913029798217352, 168.8262482093458061, 3.021315404115420679E-15 ) ) ;
#74606=EDGE_CURVE ( 'NONE', #30217, #49074, #94982, .T. ) ;
#74608=CARTESIAN_POINT ( 'NONE',  ( 169.5608527833963421, 251.6396950762901952, -9.960993533446050208 ) ) ;
#74609=ORIENTED_EDGE ( 'NONE', *, *, #98839, .T. ) ;
#74610=CARTESIAN_POINT ( 'NONE',  ( 196.3934922554618936, 290.0189000700918314, -16.29075131761187478 ) ) ;
#74613=CARTESIAN_POINT ( 'NONE',  ( 203.2369479875374623, 278.6302754407888074, -16.66242713208754367 ) ) ;
#74614=VERTEX_POINT ( 'NONE', #58773 ) ;
#74615=ORIENTED_EDGE ( 'NONE', *, *, #23716, .T. ) ;
#74617=CARTESIAN_POINT ( 'NONE',  ( 163.8990931530087494, 246.7654386749614162, 5.873176884778091633 ) ) ;
#74618=CARTESIAN_POINT ( 'NONE',  ( 153.4389798490260262, 264.8828863703868137, 16.68923469758090761 ) ) ;
#74619=ORIENTED_EDGE ( 'NONE', *, *, #6227, .F. ) ;
#74620=CARTESIAN_POINT ( 'NONE',  ( 150.6431064791187850, 269.7254810985950257, 15.11064854015152470 ) ) ;
#74622=CARTESIAN_POINT ( 'NONE',  ( 176.7010738378296253, 263.4434962957928406, 14.45361317776263910 ) ) ;
#74626=VERTEX_POINT ( 'NONE', #67385 ) ;
#74627=CARTESIAN_POINT ( 'NONE',  ( 206.5479446040613141, 272.8954610772809133, 10.74757481123993230 ) ) ;
#74628=DIRECTION ( 'NONE',  ( 0.4999999999999992784, -0.8660254037844390407, 0.000000000000000000 ) ) ;
#74630=CARTESIAN_POINT ( 'NONE',  ( 177.6723615241578216, 279.4491075471210593, -16.59050672443976282 ) ) ;
#74631=CARTESIAN_POINT ( 'NONE',  ( 168.9826911834654481, 261.4415967181243445, -16.13406239319744984 ) ) ;
#74632=ORIENTED_EDGE ( 'NONE', *, *, #54003, .T. ) ;
#74634=CARTESIAN_POINT ( 'NONE',  ( 146.8153075009282134, 276.3554234099810287, -4.113808735271278216 ) ) ;
#74635=ORIENTED_EDGE ( 'NONE', *, *, #23514, .T. ) ;
#74636=CARTESIAN_POINT ( 'NONE',  ( 157.4146825304236188, 269.0645323469553318, 15.58493267419004624 ) ) ;
#74640=CARTESIAN_POINT ( 'NONE',  ( 169.0638155539396905, 272.3808001447700917, 16.48807445323233623 ) ) ;
#74641=CARTESIAN_POINT ( 'NONE',  ( 147.3154503175461514, 275.4891506405583073, 3.671329888160011823 ) ) ;
#74642=CARTESIAN_POINT ( 'NONE',  ( 188.5163790307635168, 298.7479289875233235, -5.009957144413234253 ) ) ;
#74643=CARTESIAN_POINT ( 'NONE',  ( 190.0340467409721441, 301.4983712071542641, 4.077645795029533282 ) ) ;
#74644=CARTESIAN_POINT ( 'NONE',  ( 192.5049767439991513, 297.2185948999652965, 12.57567268027295881 ) ) ;
#74645=CARTESIAN_POINT ( 'NONE',  ( 178.4788175059835567, 291.5611646558071470, 6.106669723458193033 ) ) ;
#74646=CARTESIAN_POINT ( 'NONE',  ( 191.7934382699952494, 298.4510156884799699, -8.680100145728863126 ) ) ;
#74650=CARTESIAN_POINT ( 'NONE',  ( 164.9171241593586217, 245.0021572482830550, 1.622680932994367220 ) ) ;
#74651=CARTESIAN_POINT ( 'NONE',  ( 159.6898930778639283, 254.0559870643349143, 16.90891900388599822 ) ) ;
#74652=CARTESIAN_POINT ( 'NONE',  ( 171.5288823711526334, 289.0286466264677756, 4.266081008705642219 ) ) ;
#74656=CARTESIAN_POINT ( 'NONE',  ( 202.7310286658811265, 277.6365180286925352, 15.39425154460195699 ) ) ;
#74657=CARTESIAN_POINT ( 'NONE',  ( 126.3716228836089215, 233.7677522451417929, -5.000000000000041744 ) ) ;
#74658=B_SPLINE_CURVE_WITH_KNOTS ( 'NONE', 3,
 ( #20146, #81968, #36315, #4427, #13541, #73837, #67219, #82967, #5924, #35323, #43913, #12544, #74852, #43417, #5433, #97654, #98144, #75343, #67726, #29233, #60100, #33674, #56455, #10873, #10372, #66058, #35149, #97008, #96010, #87447, #42244, #64063, #88936, #11877, #64569, #72181, #18986, #34168, #3772, #18475, #19497, #41750, #73180, #34652, #11391, #65553, #96501, #65060, #95526, #27070 ),
 .UNSPECIFIED., .F., .F.,
 ( 4, 2, 2, 2, 2, 2, 2, 2, 2, 2, 2, 2, 2, 2, 2, 2, 2, 2, 2, 2, 2, 2, 2, 2, 4 ),
 ( 0.0003971087438474241605, 0.0008548896376937187465, 0.001083780084616804565, 0.001312670531539890384, 0.001427115755001357074, 0.001541560978462823764, 0.001656006201924290454, 0.001770451425385757144, 0.001999341872308679248, 0.002228232319231601352, 0.003143794106923289769, 0.004059355894614978186, 0.004974917682306666603, 0.005432698576152548975, 0.005661589023075452864, 0.005776034246536909146, 0.005833256858267558791, 0.005890479469998209303, 0.005947702081728858947, 0.006004924693459509459, 0.006119369916920820891, 0.006348260363843550441, 0.006806041257688862089, 0.007263822151534174605, 0.007721603045379487121 ),
 .UNSPECIFIED. ) ;
#74659=CARTESIAN_POINT ( 'NONE',  ( 199.4147421703242173, 285.2505301131875513, -17.63954444317369763 ) ) ;
#74660=CARTESIAN_POINT ( 'NONE',  ( 101.4192659406176915, 219.3615022471902023, 5.000000000000051514 ) ) ;
#74662=CARTESIAN_POINT ( 'NONE',  ( 162.9111474110223412, 248.4766108952035211, -9.702990628959184960 ) ) ;
#74663=CARTESIAN_POINT ( 'NONE',  ( 188.3784916956350344, 286.3721210266486992, -16.81851773412965301 ) ) ;
#74664=CARTESIAN_POINT ( 'NONE',  ( 152.7691010214056462, 266.0431505347400503, -16.40662330462167162 ) ) ;
#74665=CARTESIAN_POINT ( 'NONE',  ( 207.4764081617721843, 271.2873150223495600, 6.359972247200924578 ) ) ;
#74666=CARTESIAN_POINT ( 'NONE',  ( 28.14990833772381151, 180.3927522451418213, 10.00000000000009592 ) ) ;
#74667=CARTESIAN_POINT ( 'NONE',  ( 116.3854409958760385, 231.8768266524159856, -9.188101187500093303 ) ) ;
#74669=CARTESIAN_POINT ( 'NONE',  ( 183.7317734547368673, 297.0731768695540040, -2.820923390534820996 ) ) ;
#74670=CARTESIAN_POINT ( 'NONE',  ( 164.5864525486781531, 281.0963845696900307, -11.76674143703315600 ) ) ;
#74671=CARTESIAN_POINT ( 'NONE',  ( 96.65612621980318409, 236.6115022471902876, -5.000000000000047962 ) ) ;
#74672=CARTESIAN_POINT ( 'NONE',  ( 208.1583869480885483, 270.1060931147653719, 3.025867354224990979 ) ) ;
#74673=CARTESIAN_POINT ( 'NONE',  ( 44.31597619863101301, 187.2048013555409796, 4.594050593750051981 ) ) ;
#74675=B_SPLINE_CURVE_WITH_KNOTS ( 'NONE', 3,
 ( #25922, #41590, #87780, #3620, #80650, #26412, #89745, #89266, #64406, #57290, #11227, #42094, #80148, #10714, #33510, #34497, #26908, #81150, #73511, #34987, #20310, #51182, #65890, #96844, #50684, #12719, #67895, #90243, #91221, #21788, #37471, #14196, #75012, #99801, #68381, #98818, #92241, #29396, #53669, #36986 ),
 .UNSPECIFIED., .F., .F.,
 ( 4, 2, 2, 2, 2, 2, 2, 2, 2, 2, 2, 2, 2, 2, 2, 2, 2, 2, 2, 4 ),
 ( 0.0009206193881831178276, 0.001016370969008163153, 0.001112122549833208371, 0.001303625711483349329, 0.001495128873133490504, 0.001686632034783631679, 0.002452644681384161685, 0.003984669974585218662, 0.004750682621185713106, 0.005133688944485916526, 0.005325192106135940608, 0.005420943686960917086, 0.005516695267785893565, 0.005564571058198422571, 0.005612446848610951576, 0.005708198429435867340, 0.005899701591085861063, 0.006282707914385812081, 0.006665714237685763099, 0.007048720560985714118 ),
 .UNSPECIFIED. ) ;
#74680=CARTESIAN_POINT ( 'NONE',  ( -22.42236680055709641, 157.8615022471902591, 0.000000000000000000 ) ) ;
#74681=EDGE_CURVE ( 'NONE', #90285, #100061, #27428, .T. ) ;
#74682=CARTESIAN_POINT ( 'NONE',  ( 147.1249913145849177, 275.8190353104462815, 3.637773609013635223 ) ) ;
#74684=CARTESIAN_POINT ( 'NONE',  ( 207.8575108622103755, 270.6272257822888037, -6.381720258959569847 ) ) ;
#74685=CARTESIAN_POINT ( 'NONE',  ( 68.07728789491679322, 200.1115022471901739, -5.000000000000041744 ) ) ;
#74687=CARTESIAN_POINT ( 'NONE',  ( 92.16361943412358926, 214.0177522451417929, 5.000000000000051514 ) ) ;
#74688=ORIENTED_EDGE ( 'NONE', *, *, #4337, .T. ) ;
#74689=CARTESIAN_POINT ( 'NONE',  ( 198.1704809733372770, 267.8414693299324654, -7.977924972520448854 ) ) ;
#74690=CARTESIAN_POINT ( 'NONE',  ( 158.7268290693951087, 282.0671554313083789, -1.622909239661974423 ) ) ;
#74691=CARTESIAN_POINT ( 'NONE',  ( 207.9328781051891042, 270.4966858882232259, -0.8820402142964423042 ) ) ;
#74692=CARTESIAN_POINT ( 'NONE',  ( 10.35128207213630169, 176.7833772461660544, -9.188101187500095079 ) ) ;
#74697=CARTESIAN_POINT ( 'NONE',  ( 53.21953955946602122, 201.5333772461660544, 9.188101187500095079 ) ) ;
#74698=CARTESIAN_POINT ( 'NONE',  ( 207.5230514910949182, 271.2065264061283756, 2.678931747975364708 ) ) ;
#74699=CARTESIAN_POINT ( 'NONE',  ( 204.8762144138505903, 275.7909827032724479, 14.60855957933206817 ) ) ;
#74702=VERTEX_POINT ( 'NONE', #83126 ) ;
#74703=AXIS2_PLACEMENT_3D ( 'NONE', #26617, #34215, #65110 ) ;
#74706=CARTESIAN_POINT ( 'NONE',  ( 12.14648056717172686, 184.4865022471903444, -10.00000000000009415 ) ) ;
#74708=CARTESIAN_POINT ( 'NONE',  ( 147.5084024922618084, 243.7202760586659736, -5.415160957724236172E-17 ) ) ;
#74710=CARTESIAN_POINT ( 'NONE',  ( 164.4444695124895475, 245.8208191110937548, 1.054989284641946412 ) ) ;
#74717=ORIENTED_EDGE ( 'NONE', *, *, #81928, .F. ) ;
#74718=CARTESIAN_POINT ( 'NONE',  ( 159.0543278146147088, 283.1686167836548975, 1.246070035154647204 ) ) ;
#74719=CARTESIAN_POINT ( 'NONE',  ( 208.0240523230475276, 270.3387675105520884, -1.833813267351394494 ) ) ;
#74720=CARTESIAN_POINT ( 'NONE',  ( 173.9987591681438914, 277.1956714198441887, 17.06944903275143588 ) ) ;
#74728=CARTESIAN_POINT ( 'NONE',  ( 196.2046261908255929, 270.9293328135447041, 13.03164479674023291 ) ) ;
#74729=CARTESIAN_POINT ( 'NONE',  ( 182.4644955539734497, 295.0573375002295506, 4.739987455525070281 ) ) ;
#74731=CARTESIAN_POINT ( 'NONE',  ( 148.6717005876752182, 274.8950821652439345, -7.961084883142776292 ) ) ;
#74736=ORIENTED_EDGE ( 'NONE', *, *, #76532, .F. ) ;
#74742=CARTESIAN_POINT ( 'NONE',  ( 204.7817976169119163, 273.0227149632294754, -9.758020631165562619 ) ) ;
#74743=CARTESIAN_POINT ( 'NONE',  ( 164.0741338217690668, 246.4622593432776796, 7.359073626423302983 ) ) ;
#74744=CARTESIAN_POINT ( 'NONE',  ( 53.78786873247351252, 201.8615022471902307, -10.00000000000009592 ) ) ;
#74745=ORIENTED_EDGE ( 'NONE', *, *, #21336, .T. ) ;
#74746=CARTESIAN_POINT ( 'NONE',  ( 82.58295308470839302, 227.6744531367911293, 4.594050593750047540 ) ) ;
#74747=CARTESIAN_POINT ( 'NONE',  ( 155.3983691713044664, 261.4891245123925501, 17.00489288030859569 ) ) ;
#74748=CARTESIAN_POINT ( 'NONE',  ( 147.7917198021585534, 275.6304213403500398, -3.790807063116589770 ) ) ;
#74749=CARTESIAN_POINT ( 'NONE',  ( 185.0693321002852372, 259.9792428912778064, -5.919411351415631906 ) ) ;
#74750=ORIENTED_EDGE ( 'NONE', *, *, #66566, .T. ) ;
#74751=VERTEX_POINT ( 'NONE', #51181 ) ;
#74752=CARTESIAN_POINT ( 'NONE',  ( 207.3719924741569400, 270.9203590968859316, 1.937085497212718943 ) ) ;
#74757=CARTESIAN_POINT ( 'NONE',  ( 203.1526193585190470, 278.7763369107815379, -16.67658907091021447 ) ) ;
#74758=ORIENTED_EDGE ( 'NONE', *, *, #47342, .F. ) ;
#74761=B_SPLINE_CURVE_WITH_KNOTS ( 'NONE', 3,
 ( #13405, #74720, #52873, #60966 ),
 .UNSPECIFIED., .F., .F.,
 ( 4, 4 ),
 ( 0.008890319171618900340, 0.01510497574151875924 ),
 .UNSPECIFIED. ) ;
#74764=CARTESIAN_POINT ( 'NONE',  ( 10.35021921122761945, 188.3297689869269789, -2.679491924311252493 ) ) ;
#74766=CARTESIAN_POINT ( 'NONE',  ( 157.0064891765866832, 258.7037789585758105, -18.42258229807105963 ) ) ;
#74767=ORIENTED_EDGE ( 'NONE', *, *, #78116, .T. ) ;
#74771=CARTESIAN_POINT ( 'NONE',  ( 166.1232698191040527, 284.0209118141528961, 9.548314520813702799 ) ) ;
#74772=CARTESIAN_POINT ( 'NONE',  ( 199.9280821859048274, 270.2386370741994597, 9.410868133784870082 ) ) ;
#74774=CARTESIAN_POINT ( 'NONE',  ( 163.2442700311756596, 247.8996255919473697, 11.14021925110252020 ) ) ;
#74775=CARTESIAN_POINT ( 'NONE',  ( 159.9770824720811220, 253.5585604421560788, -16.42166711341322483 ) ) ;
#74776=CARTESIAN_POINT ( 'NONE',  ( 161.3512806983480914, 281.4835825935907110, -6.508326206231584976 ) ) ;
#74777=CARTESIAN_POINT ( 'NONE',  ( 164.8310825586143835, 246.4510164509542847, -1.875124838255799675 ) ) ;
#74778=( BOUNDED_CURVE ( )  B_SPLINE_CURVE ( 2, ( #99838, #92274, #34, #92755, #30423, #38000, #14724, #16222, #62812 ),
 .UNSPECIFIED., .F., .T. ) 
 B_SPLINE_CURVE_WITH_KNOTS ( ( 3, 2, 2, 2, 3 ),
 ( 0.5604838709677418818, 0.5618279569892472569, 0.5645161290322581182, 0.5672043010752688685, 0.5685483870967742437 ),
 .UNSPECIFIED. ) 
 CURVE ( )  GEOMETRIC_REPRESENTATION_ITEM ( )  RATIONAL_B_SPLINE_CURVE ( ( 0.9330127018922194093, 0.9330127018922194093, 1.000000000000000000, 0.8660254037844387076, 1.000000000000000000, 0.8660254037844387076, 1.000000000000000000, 0.9330127018922194093, 0.9330127018922194093 ) ) 
 REPRESENTATION_ITEM ( '' )  );
#74780=CARTESIAN_POINT ( 'NONE',  ( 168.0664690830419659, 253.0840726306553563, 11.72824221947031731 ) ) ;
#74782=ORIENTED_EDGE ( 'NONE', *, *, #34079, .F. ) ;
#74786=CARTESIAN_POINT ( 'NONE',  ( 160.0562591974253337, 276.7040562812561006, 12.99130222948419267 ) ) ;
#74788=B_SPLINE_CURVE_WITH_KNOTS ( 'NONE', 3,
 ( #46312, #38212, #61019, #53913 ),
 .UNSPECIFIED., .F., .F.,
 ( 4, 4 ),
 ( 0.01381869335794279167, 0.02017999936437927730 ),
 .UNSPECIFIED. ) ;
#74789=CARTESIAN_POINT ( 'NONE',  ( 171.3497015292133199, 279.8280180079489696, -15.00511433428560437 ) ) ;
#74790=CARTESIAN_POINT ( 'NONE',  ( 194.1260014150849145, 282.7392756228211397, -17.82763711395031692 ) ) ;
#74792=CARTESIAN_POINT ( 'NONE',  ( 164.7277326422747024, 274.2652274994892423, 16.02158536651776188 ) ) ;
#74793=CARTESIAN_POINT ( 'NONE',  ( -11.70556275232237908, 173.2369531367911293, -4.594050593750048428 ) ) ;
#74797=VERTEX_POINT ( 'NONE', #17633 ) ;
#74802=CARTESIAN_POINT ( 'NONE',  ( 175.5603300037018073, 290.9356092034950620, 2.583691617998545187 ) ) ;
#74803=FACE_OUTER_BOUND ( 'NONE', #51793, .T. ) ;
#74806=CARTESIAN_POINT ( 'NONE',  ( 44.18942050719596182, 202.9865022471903160, 10.00000000000009415 ) ) ;
#74807=CARTESIAN_POINT ( 'NONE',  ( -4.696256414383327638, 180.3464784336661637, 1.353441290958777525E-15 ) ) ;
#74808=CARTESIAN_POINT ( 'NONE',  ( 104.0717290597573026, 221.7048013555409796, 4.594050593750051981 ) ) ;
#74810=CARTESIAN_POINT ( 'NONE',  ( 181.6546199514925206, 256.8291319412630855, -2.317892941361705095 ) ) ;
#74812=CARTESIAN_POINT ( 'NONE',  ( 178.0467244306524890, 283.8085580107421038, -15.17727061845414660 ) ) ;
#74813=CIRCLE ( 'NONE', #34292, 17.82106496071138224 ) ;
#74816=CARTESIAN_POINT ( 'NONE',  ( 180.4555112726659445, 273.0096557832494568, 16.95796759167777523 ) ) ;
#74817=CARTESIAN_POINT ( 'NONE',  ( 194.6782745185928434, 293.4543327343926080, -14.56555309295305634 ) ) ;
#74819=CARTESIAN_POINT ( 'NONE',  ( 186.7579786969028817, 299.0471994399743494, -0.6060533366661751131 ) ) ;
#74820=CARTESIAN_POINT ( 'NONE',  ( 168.8563211758018099, 286.0187424789903048, -9.056861680415359217 ) ) ;
#74821=CARTESIAN_POINT ( 'NONE',  ( 184.3926338455641769, 268.4995540244821655, -15.66566532612987217 ) ) ;
#74824=CARTESIAN_POINT ( 'NONE',  ( 172.8992021874003342, 262.9442772269209740, -15.72255003995701195 ) ) ;
#74825=CARTESIAN_POINT ( 'NONE',  ( 88.29356841273579448, 221.7833772461660544, -9.188101187500095079 ) ) ;
#74827=DIRECTION ( 'NONE',  ( -0.4999999999999987788, 0.8660254037844392627, 0.000000000000000000 ) ) ;
#74829=CARTESIAN_POINT ( 'NONE',  ( 157.1606030646430554, 258.4368458743103361, 17.96998724893680688 ) ) ;
#74830=CARTESIAN_POINT ( 'NONE',  ( 152.4190720221992308, 266.6494185454878334, 15.69722907698042924 ) ) ;
#74832=CARTESIAN_POINT ( 'NONE',  ( 198.9832789858017463, 285.9978462703757600, -18.55676541969546278 ) ) ;
#74833=CARTESIAN_POINT ( 'NONE',  ( 204.0672213060390163, 276.0394433563056396, -13.55990476547925283 ) ) ;
#74835=CARTESIAN_POINT ( 'NONE',  ( 146.8153075009282134, 276.3554234099810287, -4.113808735271278216 ) ) ;
#74837=EDGE_LOOP ( 'NONE', ( #9857, #58897, #95610, #58812, #88420 ) ) ;
#74840=CARTESIAN_POINT ( 'NONE',  ( 116.4326846683273544, 226.4824982072973683, 3.021315404115420679E-15 ) ) ;
#74841=CARTESIAN_POINT ( 'NONE',  ( 189.9416213258632808, 286.8907125026590847, -15.86853789214096011 ) ) ;
#74845=CARTESIAN_POINT ( 'NONE',  ( 157.4612664356622815, 268.7406194900779610, 15.65006598224691281 ) ) ;
#74846=CARTESIAN_POINT ( 'NONE',  ( 169.9469112398214747, 250.9785751410766750, -8.718312767540300712 ) ) ;
#74847=CARTESIAN_POINT ( 'NONE',  ( 148.1846377449773513, 246.3615022471901739, 5.000000000000051514 ) ) ;
#74848=CARTESIAN_POINT ( 'NONE',  ( 205.2391015854675516, 275.1624436846170738, -14.01434138479280911 ) ) ;
#74849=ORIENTED_EDGE ( 'NONE', *, *, #49267, .F. ) ;
#74850=CARTESIAN_POINT ( 'NONE',  ( 189.9879251633717558, 299.5782561228834879, -6.671532329245590809 ) ) ;
#74851=ORIENTED_EDGE ( 'NONE', *, *, #21840, .T. ) ;
#74852=CARTESIAN_POINT ( 'NONE',  ( 196.9033078495128279, 265.2933406070572460, -4.538647946727325078 ) ) ;
#74855=CARTESIAN_POINT ( 'NONE',  ( 181.6377726600393316, 290.8352285560014252, -10.98690006892555004 ) ) ;
#74858=CARTESIAN_POINT ( 'NONE',  ( 158.9711380693753711, 255.3009072572319269, 16.19938186386990608 ) ) ;
#74859=CARTESIAN_POINT ( 'NONE',  ( 140.7960114214023974, 264.3464784336661637, 1.353441290958777327E-15 ) ) ;
#74860=CARTESIAN_POINT ( 'NONE',  ( 204.0783642268031031, 272.7229525204484162, 11.17834187752937325 ) ) ;
#74864=CARTESIAN_POINT ( 'NONE',  ( -22.42236680055709641, 157.8615022471902591, 0.000000000000000000 ) ) ;
#74865=CARTESIAN_POINT ( 'NONE',  ( 164.3152942664659690, 274.9982970269645648, 14.72102722954017118 ) ) ;
#74866=CARTESIAN_POINT ( 'NONE',  ( 189.3423859142968695, 300.6963629005612120, 0.4146017780601669589 ) ) ;
#74870=CARTESIAN_POINT ( 'NONE',  ( 204.9768178125733016, 275.6167325052707611, 13.98665089523138505 ) ) ;
#74871=CARTESIAN_POINT ( 'NONE',  ( 162.6368345399827433, 272.7197526209740772, -16.33568937601149784 ) ) ;
#74872=CARTESIAN_POINT ( 'NONE',  ( 206.0977829604818510, 273.6751639155793896, -9.820003938885891515 ) ) ;
#74876=CARTESIAN_POINT ( 'NONE',  ( 171.0255721845828418, 287.7745651417276349, -4.514413061350604828 ) ) ;
#74878=CARTESIAN_POINT ( 'NONE',  ( 178.3425427631553077, 255.6075038009615810, 4.888047764587837740 ) ) ;
#74880=CARTESIAN_POINT ( 'NONE',  ( 190.9928235942860795, 292.9214909438621817, -14.57390052809859249 ) ) ;
#74883=CIRCLE ( 'NONE', #18242, 17.82106496071138935 ) ;
#74887=CARTESIAN_POINT ( 'NONE',  ( 194.6050500505458842, 285.5465367126718093, -17.70104686455487553 ) ) ;
#74888=CARTESIAN_POINT ( 'NONE',  ( 195.8947060313465443, 291.3474115503753410, 16.07878593000791767 ) ) ;
#74889=CARTESIAN_POINT ( 'NONE',  ( 159.5221561062548972, 254.3465160214695118, -16.91023001054109542 ) ) ;
#74890=CARTESIAN_POINT ( 'NONE',  ( 195.6395968400605341, 272.4316657006998526, -14.88132701375339906 ) ) ;
#74896=CARTESIAN_POINT ( 'NONE',  ( 195.0706027375981080, 265.7742591254879017, -8.915832648898723178 ) ) ;
#74899=CARTESIAN_POINT ( 'NONE',  ( 127.1021582719434662, 250.3149278399161233, -9.188101187500095079 ) ) ;
#74903=CARTESIAN_POINT ( 'NONE',  ( 157.4843645388753544, 257.8760745514064183, 17.70049730742206862 ) ) ;
#74906=CARTESIAN_POINT ( 'NONE',  ( 170.8421116289723045, 249.9010192475012673, -0.2585453712269101811 ) ) ;
#74907=CARTESIAN_POINT ( 'NONE',  ( 121.4100190113084636, 234.2365022471901739, -10.00000000000009237 ) ) ;
#74912=FACE_OUTER_BOUND ( 'NONE', #23872, .T. ) ;
#74913=CARTESIAN_POINT ( 'NONE',  ( 155.6276701977099890, 261.0919634844306643, 17.49722577287685255 ) ) ;
#74917=CARTESIAN_POINT ( 'NONE',  ( 66.64328041388984047, 197.0327760586659736, 1.948934522072303157E-15 ) ) ;
#74918=CARTESIAN_POINT ( 'NONE',  ( 206.0930919633010774, 273.6832889610345774, -9.866500005465628220 ) ) ;
#74919=CARTESIAN_POINT ( 'NONE',  ( 178.1281481821618797, 292.9991590599575488, -6.064681374715556572 ) ) ;
#74920=CARTESIAN_POINT ( 'NONE',  ( 208.3863431123642727, 269.7112614563416173, -1.693909372230378851 ) ) ;
#74925=CARTESIAN_POINT ( 'NONE',  ( 71.30684095964828373, 218.6427522451419065, 10.00000000000009415 ) ) ;
#74928=CARTESIAN_POINT ( 'NONE',  ( 157.7698537200534190, 270.6225848554070126, -15.38064719042920103 ) ) ;
#74930=CARTESIAN_POINT ( 'NONE',  ( 29.48529115882250551, 178.6423013555409796, -4.594050593750043987 ) ) ;
#74931=B_SPLINE_CURVE_WITH_KNOTS ( 'NONE', 3,
 ( #40512, #70945, #32432, #78546 ),
 .UNSPECIFIED., .F., .F.,
 ( 4, 4 ),
 ( 0.008410254777844634877, 0.01479413815379926507 ),
 .UNSPECIFIED. ) ;
#74933=CARTESIAN_POINT ( 'NONE',  ( 185.0107362994922937, 259.8037357443623705, -8.917975770776131128 ) ) ;
#74934=CARTESIAN_POINT ( 'NONE',  ( 199.2838428981942229, 277.8941618483122511, 16.22077298392192191 ) ) ;
#74937=CARTESIAN_POINT ( 'NONE',  ( 46.39958950466356669, 197.5958772461660544, -9.188101187500095079 ) ) ;
#74939=CARTESIAN_POINT ( 'NONE',  ( 170.6536247108341513, 287.7753904406291667, 7.365555831541199971 ) ) ;
#74940=CARTESIAN_POINT ( 'NONE',  ( 149.7109319212262051, 271.3400547943878109, -12.38605961032017433 ) ) ;
#74942=CARTESIAN_POINT ( 'NONE',  ( 203.0033695482938185, 269.9821257774704009, -7.166763272130794782 ) ) ;
#74943=CARTESIAN_POINT ( 'NONE',  ( 175.8519086042108199, 291.1168019899661203, 2.550567897145465501 ) ) ;
#74944=CARTESIAN_POINT ( 'NONE',  ( 179.7328860548953458, 276.7974806922320568, 16.30745684656992722 ) ) ;
#74945=CARTESIAN_POINT ( 'NONE',  ( 182.2373335159190901, 280.9600371166583841, -17.30031729693378040 ) ) ;
#74947=CARTESIAN_POINT ( 'NONE',  ( 192.9510928534456298, 267.2000408598793797, 11.21941862815989488 ) ) ;
#74950=CARTESIAN_POINT ( 'NONE',  ( 91.89298649898879034, 233.8615022471903160, 5.000000000000046185 ) ) ;
#74951=CARTESIAN_POINT ( 'NONE',  ( 200.4116241316243645, 283.5238799070667142, 18.37703770054986663 ) ) ;
#74952=CARTESIAN_POINT ( 'NONE',  ( 194.7281770665802867, 285.5812223991454744, -17.42918990626452924 ) ) ;
#74954=CARTESIAN_POINT ( 'NONE',  ( 54.73473692032377613, 214.6589784336661637, -6.496448406907675876E-16 ) ) ;
#74955=EDGE_LOOP ( 'NONE', ( #7060, #10035, #6098, #67121 ) ) ;
#74957=CARTESIAN_POINT ( 'NONE',  ( 190.8957779480239765, 300.0058089740729770, -4.541438514207768229 ) ) ;
#74961=FACE_OUTER_BOUND ( 'NONE', #45536, .T. ) ;
#74964=B_SPLINE_CURVE_WITH_KNOTS ( 'NONE', 3,
 ( #67124, #97563, #13451, #58522 ),
 .UNSPECIFIED., .F., .F.,
 ( 4, 4 ),
 ( 0.01376344692898578796, 0.02004488622147810803 ),
 .UNSPECIFIED. ) ;
#74968=CARTESIAN_POINT ( 'NONE',  ( 205.0993130461165777, 275.4045645370890156, 13.92529057593422337 ) ) ;
#74969=ORIENTED_EDGE ( 'NONE', *, *, #62898, .F. ) ;
#74972=CARTESIAN_POINT ( 'NONE',  ( 164.8705138155180521, 286.2009910768602481, -3.373684704351256780 ) ) ;
#74973=CARTESIAN_POINT ( 'NONE',  ( 6.156471524329347744, 184.3615022471903160, 5.000000000000046185 ) ) ;
#74976=CARTESIAN_POINT ( 'NONE',  ( 167.3443243822065654, 261.7894444419548563, 16.27081549069046318 ) ) ;
#74977=CARTESIAN_POINT ( 'NONE',  ( 206.8317058779879574, 272.4039721336197317, -10.41591514895975834 ) ) ;
#74978=ORIENTED_EDGE ( 'NONE', *, *, #88443, .F. ) ;
#74979=CARTESIAN_POINT ( 'NONE',  ( 159.7396088078454852, 282.2794754784105749, -3.211990912219383709 ) ) ;
#74980=LINE ( 'NONE', #98282, #18405 ) ;
#74985=CARTESIAN_POINT ( 'NONE',  ( 163.5043721629895117, 264.4363120689758944, -16.70418041949503873 ) ) ;
#74987=CARTESIAN_POINT ( 'NONE',  ( 136.0064158243085046, 240.1423013555409796, -4.594050593750043987 ) ) ;
#74988=CARTESIAN_POINT ( 'NONE',  ( 10.46624461501205872, 188.3967562850346837, -4.648177544792955347E-16 ) ) ;
#74990=CARTESIAN_POINT ( 'NONE',  ( 170.1385426601652568, 264.1995677655418149, 16.47783103859512721 ) ) ;
#74993=B_SPLINE_CURVE_WITH_KNOTS ( 'NONE', 3,
 ( #53036, #52051, #99658, #14556 ),
 .UNSPECIFIED., .F., .F.,
 ( 4, 4 ),
 ( 2.780973288783981667E-17, 0.002844266532014441858 ),
 .UNSPECIFIED. ) ;
#74994=CARTESIAN_POINT ( 'NONE',  ( 83.21237853290490705, 230.3967562850347122, -4.648177544792955347E-16 ) ) ;
#74996=VERTEX_POINT ( 'NONE', #64487 ) ;
#74997=CARTESIAN_POINT ( 'NONE',  ( 198.6742831389107096, 286.5330427765190393, 17.60232614297041565 ) ) ;
#74999=CARTESIAN_POINT ( 'NONE',  ( 77.36034478572226192, 203.2202760586659167, -5.415160957724236172E-17 ) ) ;
#75001=CARTESIAN_POINT ( 'NONE',  ( 120.4921787521148246, 228.8262482093457777, 3.021315404115420679E-15 ) ) ;
#75002=CARTESIAN_POINT ( 'NONE',  ( 155.6435836392643637, 261.0644005951349982, 17.58841156286628049 ) ) ;
#75005=CARTESIAN_POINT ( 'NONE',  ( 183.3097982497011174, 257.4453907524014085, -6.291681649002233812 ) ) ;
#75007=CARTESIAN_POINT ( 'NONE',  ( 119.9486011388743236, 233.3927522451417360, -10.00000000000009237 ) ) ;
#75008=CARTESIAN_POINT ( 'NONE',  ( 152.9607371460978129, 265.7112270302071124, -16.17698032818104537 ) ) ;
#75009=CARTESIAN_POINT ( 'NONE',  ( 155.3513572141771704, 261.5705516107003064, -17.00592413546589299 ) ) ;
#75012=CARTESIAN_POINT ( 'NONE',  ( 163.8698660330890959, 260.7705462234230254, -16.30966607616605657 ) ) ;
#75014=CARTESIAN_POINT ( 'NONE',  ( 199.9852625142306977, 283.3066338628505036, -17.10789104304789277 ) ) ;
#75015=CARTESIAN_POINT ( 'NONE',  ( 164.5648480107187197, 245.6123174360222094, 3.015887571020871238 ) ) ;
#75017=CARTESIAN_POINT ( 'NONE',  ( 195.1869371033206164, 279.2024320103926129, 16.32474613100176342 ) ) ;
#75019=CARTESIAN_POINT ( 'NONE',  ( 207.5290616128274337, 271.1961165699281651, 2.604679844609484984 ) ) ;
#75020=CARTESIAN_POINT ( 'NONE',  ( 132.4608640057421667, 247.2833772461660544, -9.188101187500095079 ) ) ;
#75022=CARTESIAN_POINT ( 'NONE',  ( -7.720288864461156919, 177.8967562850347122, -4.648177544792955347E-16 ) ) ;
#75028=DIRECTION ( 'NONE',  ( -0.8660254037844387076, -0.4999999999999998890, -0.000000000000000000 ) ) ;
#75031=ORIENTED_EDGE ( 'NONE', *, *, #79719, .F. ) ;
#75033=CARTESIAN_POINT ( 'NONE',  ( 182.4489905826245888, 275.9573809634798636, -16.44186478306133736 ) ) ;
#75035=CARTESIAN_POINT ( 'NONE',  ( 167.2918192146199772, 248.9981393517354320, -5.482138639605560471 ) ) ;
#75041=CARTESIAN_POINT ( 'NONE',  ( 183.2023180053008673, 280.9201651122064618, 17.20581014854919744 ) ) ;
#75042=CARTESIAN_POINT ( 'NONE',  ( 193.1374568794722393, 268.2848186726958488, 12.69397648171735860 ) ) ;
#75045=CARTESIAN_POINT ( 'NONE',  ( 80.05961770938091604, 205.4824982072973967, 3.021315404115420679E-15 ) ) ;
#75047=FACE_OUTER_BOUND ( 'NONE', #78541, .T. ) ;
#75048=CARTESIAN_POINT ( 'NONE',  ( 207.2597638908594604, 271.6625539067387649, 6.169660687298267554 ) ) ;
#75049=( BOUNDED_CURVE ( )  B_SPLINE_CURVE ( 2, ( #48369, #15956, #47352, #78274, #16455, #70656, #1268, #70142, #38749 ),
 .UNSPECIFIED., .F., .T. ) 
 B_SPLINE_CURVE_WITH_KNOTS ( ( 3, 2, 2, 2, 3 ),
 ( 0.6411290322580645018, 0.6424731182795698770, 0.6451612903225806273, 0.6478494623655913776, 0.6491935483870967527 ),
 .UNSPECIFIED. ) 
 CURVE ( )  GEOMETRIC_REPRESENTATION_ITEM ( )  RATIONAL_B_SPLINE_CURVE ( ( 0.9330127018922194093, 0.9330127018922194093, 1.000000000000000000, 0.8660254037844387076, 1.000000000000000000, 0.8660254037844387076, 1.000000000000000000, 0.9330127018922194093, 0.9330127018922194093 ) ) 
 REPRESENTATION_ITEM ( '' )  );
#75050=CARTESIAN_POINT ( 'NONE',  ( 140.6610420460521311, 252.0177522451418213, -10.00000000000009592 ) ) ;
#75052=ORIENTED_EDGE ( 'NONE', *, *, #58561, .F. ) ;
#75054=CARTESIAN_POINT ( 'NONE',  ( 198.8194531333411419, 286.2816009704309863, -17.01510935557533344 ) ) ;
#75055=CARTESIAN_POINT ( 'NONE',  ( 5.777845730223497789, 164.9548013555410080, -4.594050593750042211 ) ) ;
#75056=CARTESIAN_POINT ( 'NONE',  ( 178.5612894430947790, 259.1195402287601723, -10.32338363706679019 ) ) ;
#75059=CARTESIAN_POINT ( 'NONE',  ( 157.1002372043759010, 258.5414026113353430, -17.73553732786789539 ) ) ;
#75061=CARTESIAN_POINT ( 'NONE',  ( 124.7297830591487724, 249.4865022471903160, 10.00000000000009415 ) ) ;
#75062=CARTESIAN_POINT ( 'NONE',  ( 200.1492870304027178, 271.0868101810378903, -11.33151401369217659 ) ) ;
#75063=CARTESIAN_POINT ( 'NONE',  ( 67.84273934451053378, 216.6427522451418781, -10.00000000000009415 ) ) ;
#75065=CARTESIAN_POINT ( 'NONE',  ( 150.9158774466703221, 269.2530279239659308, 15.11407781020157515 ) ) ;
#75066=CARTESIAN_POINT ( 'NONE',  ( 179.0995391845479503, 294.3117743827021400, 1.062652647630369485 ) ) ;
#75067=CARTESIAN_POINT ( 'NONE',  ( 54.58172535260923297, 208.9865022471903160, 10.00000000000009237 ) ) ;
#75068=DIRECTION ( 'NONE',  ( 0.4999999999999998890, -0.8660254037844385966, 0.000000000000000000 ) ) ;
#75069=CARTESIAN_POINT ( 'NONE',  ( 148.3837145175834280, 273.6388627701866767, 8.841971351370922605 ) ) ;
#75070=CARTESIAN_POINT ( 'NONE',  ( 11.32556065139379875, 177.3458772461660544, 9.188101187500095079 ) ) ;
#75071=CARTESIAN_POINT ( 'NONE',  ( 168.2809673467089624, 286.2893536684765081, 4.380497092391412828 ) ) ;
#75072=CARTESIAN_POINT ( 'NONE',  ( 13.85502868284443068, 167.2592609112379876, 2.679491924311228512 ) ) ;
#75074=CARTESIAN_POINT ( 'NONE',  ( 201.6770223052710946, 280.5522444021153206, -16.20575782718176328 ) ) ;
#75076=CARTESIAN_POINT ( 'NONE',  ( 188.2111106237954630, 267.2351608166093797, 14.29806277360018996 ) ) ;
#75077=CARTESIAN_POINT ( 'NONE',  ( 114.5053184729291189, 248.4637435831425023, 2.679491924311251605 ) ) ;
#75078=CARTESIAN_POINT ( 'NONE',  ( 160.1491107143660884, 280.2713282481162764, 9.384238864439979011 ) ) ;
#75083=CARTESIAN_POINT ( 'NONE',  ( 159.5589503240031206, 258.7431445789238751, 17.10287526337421227 ) ) ;
#75085=CARTESIAN_POINT ( 'NONE',  ( 194.1011995340913074, 294.4538559273262877, 13.93949783759920713 ) ) ;
#75087=CARTESIAN_POINT ( 'NONE',  ( 182.0723377230381743, 289.3047168942152325, 12.38573695971384048 ) ) ;
#75091=EDGE_CURVE ( 'NONE', #99571, #15352, #53818, .T. ) ;
#75092=EDGE_LOOP ( 'NONE', ( #14971, #89813, #59210, #85596, #55384, #23491, #81748, #44719, #15388, #91322, #30482, #25230, #79597, #10049, #711, #1682, #4806, #92864, #94412, #38546 ) ) ;
#75096=CARTESIAN_POINT ( 'NONE',  ( 155.1398527401465230, 261.9368881057492899, -17.02245700497956449 ) ) ;
#75100=CARTESIAN_POINT ( 'NONE',  ( 159.4050015888674920, 279.2435389297123152, -9.491234884881382783 ) ) ;
#75101=CARTESIAN_POINT ( 'NONE',  ( 204.3276935076901850, 276.7410487817560920, 13.46217427333259309 ) ) ;
#75102=CARTESIAN_POINT ( 'NONE',  ( 192.0523540417460993, 298.0025604169266558, 12.03387399082417275 ) ) ;
#75103=VERTEX_POINT ( 'NONE', #74605 ) ;
#75104=CARTESIAN_POINT ( 'NONE',  ( 151.4327733764141612, 268.3577379114237829, 14.90862905801242100 ) ) ;
#75106=CARTESIAN_POINT ( 'NONE',  ( 160.6574774401344428, 259.8181007787099475, -17.52623987902137515 ) ) ;
#75108=EDGE_CURVE ( 'NONE', #75612, #65702, #64993, .T. ) ;
#75111=CARTESIAN_POINT ( 'NONE',  ( 196.5475899070771675, 290.2165835061676944, -17.89382743182097002 ) ) ;
#75112=ORIENTED_EDGE ( 'NONE', *, *, #10578, .F. ) ;
#75113=CARTESIAN_POINT ( 'NONE',  ( 206.0041637419966776, 273.8373171585603814, 11.66586596407113596 ) ) ;
#75115=B_SPLINE_SURFACE_WITH_KNOTS ( 'NONE', 3, 1, ( 
 ( #73958, #50635 ),
 ( #20763, #19766 ),
 ( #88712, #58238 ),
 ( #19281, #12157 ),
 ( #42530, #50148 ),
 ( #18763, #10662 ),
 ( #89699, #41538 ),
 ( #97765, #72483 ),
 ( #3085, #73463 ),
 ( #74477, #33976 ),
 ( #82095, #12668 ),
 ( #57237, #65831 ),
 ( #96797, #64860 ),
 ( #43536, #95807 ),
 ( #4046, #43019 ),
 ( #81588, #5055 ),
 ( #4543, #26361 ),
 ( #3569, #35444 ),
 ( #81101, #66346 ),
 ( #88212, #49641 ),
 ( #97279, #27356 ),
 ( #26856, #57732 ),
 ( #11668, #27846 ),
 ( #51133, #80599 ),
 ( #11177, #58724 ),
 ( #42044, #34450 ),
 ( #65348, #20258 ),
 ( #35935, #28335 ),
 ( #59212, #90187 ),
 ( #21740, #29351 ),
 ( #7531, #92673 ),
 ( #30841, #99753 ),
 ( #90698, #7034 ),
 ( #37916, #30338 ) ),
 .UNSPECIFIED., .T., .F., .F.,
 ( 4, 2, 2, 2, 2, 2, 2, 2, 2, 2, 2, 2, 2, 2, 2, 2, 4 ),
 ( 2, 2 ),
 ( 0.000000000000000000, 0.06250000000000000000, 0.1250000000000000000, 0.1875000000000000000, 0.2500000000000000000, 0.3125000000000000000, 0.3750000000000000000, 0.4375000000000000000, 0.5000000000000000000, 0.5625000000000000000, 0.6250000000000000000, 0.6875000000000000000, 0.7500000000000000000, 0.8125000000000000000, 0.8750000000000000000, 0.9375000000000000000, 1.000000000000000000 ),
 ( 0.000000000000000000, 1.000000000000000000 ),
 .UNSPECIFIED. ) ;
#75116=ORIENTED_EDGE ( 'NONE', *, *, #93643, .F. ) ;
#75117=CARTESIAN_POINT ( 'NONE',  ( 174.5871134489742076, 276.7843657037444132, -16.02992603658275073 ) ) ;
#75118=CARTESIAN_POINT ( 'NONE',  ( 168.9751777291785402, 261.3521787389587985, -16.33135548124933223 ) ) ;
#75119=EDGE_LOOP ( 'NONE', ( #73996, #80782, #95874, #53174 ) ) ;
#75120=CARTESIAN_POINT ( 'NONE',  ( 158.6609831669983635, 274.8501997329411779, -12.75851027878984745 ) ) ;
#75125=ORIENTED_EDGE ( 'NONE', *, *, #37203, .T. ) ;
#75128=CARTESIAN_POINT ( 'NONE',  ( 190.9380839614473473, 299.9325328093580652, -5.232187664503159752 ) ) ;
#75131=CARTESIAN_POINT ( 'NONE',  ( 192.5254593562406171, 297.1831179748913314, 11.00703791256144015 ) ) ;
#75132=CARTESIAN_POINT ( 'NONE',  ( 191.7079280567292017, 298.5991237224230304, 9.677592105567574876 ) ) ;
#75133=CARTESIAN_POINT ( 'NONE',  ( 147.1447476476323004, 275.7848163378367872, 0.6373001129109078233 ) ) ;
#75139=CYLINDRICAL_SURFACE ( 'NONE', #88438, 17.82106496071139645 ) ;
#75141=CARTESIAN_POINT ( 'NONE',  ( 190.4155215753448829, 300.8376374122118477, -3.221041461475324219 ) ) ;
#75144=CARTESIAN_POINT ( 'NONE',  ( 202.8550299997861259, 277.8130222402279514, 15.22080692779638511 ) ) ;
#75146=CARTESIAN_POINT ( 'NONE',  ( 199.3292086366563467, 285.3986785392510797, -17.29754939996516683 ) ) ;
#75148=VERTEX_POINT ( 'NONE', #88345 ) ;
#75149=CARTESIAN_POINT ( 'NONE',  ( 163.4178923001155681, 247.5989030008181260, -10.38047187240561442 ) ) ;
#75152=CARTESIAN_POINT ( 'NONE',  ( 155.6368094659423207, 263.0761338075079721, 17.69820953191020152 ) ) ;
#75153=CARTESIAN_POINT ( 'NONE',  ( 43.23318412030271674, 205.7677522451419350, -5.000000000000047962 ) ) ;
#75154=B_SPLINE_CURVE_WITH_KNOTS ( 'NONE', 3,
 ( #77508, #16190, #39459, #54163 ),
 .UNSPECIFIED., .F., .F.,
 ( 4, 4 ),
 ( 0.04853114605566435924, 0.04887120950165265570 ),
 .UNSPECIFIED. ) ;
#75155=CARTESIAN_POINT ( 'NONE',  ( 120.1739550416679378, 246.3149278399160949, 9.188101187500093303 ) ) ;
#75156=CARTESIAN_POINT ( 'NONE',  ( 198.9590707264871412, 286.0397762054715827, -17.05306195936250191 ) ) ;
#75159=CARTESIAN_POINT ( 'NONE',  ( 97.88299554183114992, 233.9865022471902876, -10.00000000000009592 ) ) ;
#75160=CARTESIAN_POINT ( 'NONE',  ( 175.7329799467893849, 253.0876820653997186, -4.805701136885333291 ) ) ;
#75161=B_SPLINE_CURVE_WITH_KNOTS ( 'NONE', 3,
 ( #86790, #17323, #40614, #56317 ),
 .UNSPECIFIED., .F., .F.,
 ( 4, 4 ),
 ( 0.000000000000000000, 0.0003410592472882656044 ),
 .UNSPECIFIED. ) ;
#75162=CARTESIAN_POINT ( 'NONE',  ( 34.35668405510998724, 181.4548013555409796, -4.594050593750042211 ) ) ;
#75164=ORIENTED_EDGE ( 'NONE', *, *, #97028, .T. ) ;
#75167=CARTESIAN_POINT ( 'NONE',  ( 178.9149973514854537, 265.8180992141078605, 16.19802902779107967 ) ) ;
#75168=EDGE_CURVE ( 'NONE', #43311, #62454, #3102, .T. ) ;
#75172=CARTESIAN_POINT ( 'NONE',  ( 207.1019571622349815, 271.9358831784929293, -5.989975140547304733 ) ) ;
#75173=CARTESIAN_POINT ( 'NONE',  ( 177.2370279623645501, 286.0837832704111179, -12.08136213241702350 ) ) ;
#75174=CARTESIAN_POINT ( 'NONE',  ( 164.2180702684029825, 250.0262507739865043, 10.22535470056666540 ) ) ;
#75175=CARTESIAN_POINT ( 'NONE',  ( 91.22542524669036368, 230.1427522451419065, -10.00000000000009415 ) ) ;
#75176=B_SPLINE_SURFACE_WITH_KNOTS ( 'NONE', 3, 1, ( 
 ( #97388, #80217 ),
 ( #35057, #11790 ),
 ( #27956, #81707 ),
 ( #3688, #2692 ),
 ( #34567, #57861 ),
 ( #42647, #73579 ),
 ( #4161, #65964 ),
 ( #96916, #58353 ),
 ( #12279, #89331 ),
 ( #43140, #74083 ),
 ( #35563, #76085 ),
 ( #5656, #38537 ),
 ( #69934, #69444 ),
 ( #62838, #16247 ),
 ( #61832, #23334 ),
 ( #47138, #83529 ),
 ( #83031, #84036 ),
 ( #98718, #75916 ),
 ( #68280, #99202 ),
 ( #37866, #74913 ),
 ( #99699, #30286 ),
 ( #61173, #84527 ),
 ( #92141, #22694 ),
 ( #45960, #33281 ),
 ( #55559, #77901 ),
 ( #62162, #8981 ),
 ( #71806, #54063 ),
 ( #93111, #69777 ),
 ( #7997, #386 ),
 ( #8488, #63683 ),
 ( #9497, #77395 ),
 ( #23663, #31274 ),
 ( #40363, #93617 ),
 ( #1396, #54555 ) ),
 .UNSPECIFIED., .T., .F., .F.,
 ( 4, 2, 2, 2, 2, 2, 2, 2, 2, 2, 2, 2, 2, 2, 2, 2, 4 ),
 ( 2, 2 ),
 ( 0.000000000000000000, 0.06250000000000000000, 0.1250000000000000000, 0.1875000000000000000, 0.2500000000000000000, 0.3125000000000000000, 0.3750000000000000000, 0.4375000000000000000, 0.5000000000000000000, 0.5625000000000000000, 0.6250000000000000000, 0.6875000000000000000, 0.7500000000000000000, 0.8125000000000000000, 0.8750000000000000000, 0.9375000000000000000, 1.000000000000000000 ),
 ( 0.000000000000000000, 1.000000000000000000 ),
 .UNSPECIFIED. ) ;
#75177=ORIENTED_EDGE ( 'NONE', *, *, #41107, .F. ) ;
#75180=CARTESIAN_POINT ( 'NONE',  ( 157.3607188712925620, 280.8594552850489663, -1.588514201417627669 ) ) ;
#75181=CARTESIAN_POINT ( 'NONE',  ( 154.1399373542834326, 265.3127017963294634, 16.98476250194385884 ) ) ;
#75182=CARTESIAN_POINT ( 'NONE',  ( 5.317335864756744357, 180.0024278399160949, -9.188101187500093303 ) ) ;
#75184=CARTESIAN_POINT ( 'NONE',  ( 196.0836447532441014, 273.4668328341180654, 15.15126769363194015 ) ) ;
#75187=CARTESIAN_POINT ( 'NONE',  ( 54.00411475982191689, 211.1744531367911293, 4.594050593750047540 ) ) ;
#75188=CARTESIAN_POINT ( 'NONE',  ( 163.7085541710205234, 247.0954618725873217, -6.713544974106887331 ) ) ;
#75191=CARTESIAN_POINT ( 'NONE',  ( 165.0156970625405108, 244.8314239717225007, -1.890480716182876719 ) ) ;
#75192=ORIENTED_EDGE ( 'NONE', *, *, #94621, .F. ) ;
#75193=CARTESIAN_POINT ( 'NONE',  ( 164.7396270603856294, 269.0037874151494179, 17.61975801440670608 ) ) ;
#75194=CARTESIAN_POINT ( 'NONE',  ( 13.01250597095616612, 184.9865022471903160, 10.00000000000009237 ) ) ;
#75195=CARTESIAN_POINT ( 'NONE',  ( 164.4678285797544106, 245.7803600197737524, -6.875991496205872799 ) ) ;
#75196=CARTESIAN_POINT ( 'NONE',  ( 126.7502486777147794, 253.1744531367911009, 4.594050593750047540 ) ) ;
#75201=CARTESIAN_POINT ( 'NONE',  ( 189.4106793247880489, 289.8710049031299150, 14.49873233045173571 ) ) ;
#75205=CARTESIAN_POINT ( 'NONE',  ( 163.6302915796623267, 247.2310166571519687, 7.393723215219985434 ) ) ;
#75207=CARTESIAN_POINT ( 'NONE',  ( 169.9431595906827113, 266.1794658690906203, -17.47759505517880285 ) ) ;
#75208=CARTESIAN_POINT ( 'NONE',  ( 197.3266261510635786, 273.2354618366890691, -13.41124827380268236 ) ) ;
#75213=CARTESIAN_POINT ( 'NONE',  ( 20.85854946042532276, 194.3967562850347122, -4.648177544792955347E-16 ) ) ;
#75214=CARTESIAN_POINT ( 'NONE',  ( 181.9860418187968492, 295.0310787814198079, 4.802745342729399347 ) ) ;
#75217=CARTESIAN_POINT ( 'NONE',  ( 154.4470374439381146, 277.6591429590598068, -9.115886381272481742 ) ) ;
#75223=CARTESIAN_POINT ( 'NONE',  ( 159.6056220676521207, 264.0888561691485279, -17.76186630473194938 ) ) ;
#75224=ORIENTED_EDGE ( 'NONE', *, *, #93275, .F. ) ;
#75226=CARTESIAN_POINT ( 'NONE',  ( 191.6823192895500370, 298.6434794082964572, -8.424208857102787107 ) ) ;
#75228=CARTESIAN_POINT ( 'NONE',  ( 163.8990931530087494, 246.7654386749614162, 5.873176884778091633 ) ) ;
#75229=DIRECTION ( 'NONE',  ( -0.8660254037844387076, -0.4999999999999998890, -0.000000000000000000 ) ) ;
#75231=CARTESIAN_POINT ( 'NONE',  ( 89.86341300497758766, 216.5643266524160140, 9.188101187500095079 ) ) ;
#75232=CARTESIAN_POINT ( 'NONE',  ( 203.2845477157559060, 278.5478302930881682, 14.95601347903707889 ) ) ;
#75234=CARTESIAN_POINT ( 'NONE',  ( 177.9267046042368179, 268.9789068694544767, -16.81798070278933821 ) ) ;
#75237=EDGE_CURVE ( 'NONE', #7831, #81147, #92455, .T. ) ;
#75239=CARTESIAN_POINT ( 'NONE',  ( -5.625082409869304634, 160.8927522451418213, 10.00000000000009948 ) ) ;
#75241=ORIENTED_EDGE ( 'NONE', *, *, #48586, .T. ) ;
#75242=CYLINDRICAL_SURFACE ( 'NONE', #30412, 17.82106496071139645 ) ;
#75246=ORIENTED_EDGE ( 'NONE', *, *, #84816, .F. ) ;
#75250=CARTESIAN_POINT ( 'NONE',  ( 14.81672556217377235, 179.3615022471902591, -10.00000000000009592 ) ) ;
#75253=CARTESIAN_POINT ( 'NONE',  ( 168.2183573306309086, 267.1390863016062553, -17.06247922714877063 ) ) ;
#75254=EDGE_LOOP ( 'NONE', ( #73951, #96581 ) ) ;
#75257=ORIENTED_EDGE ( 'NONE', *, *, #43624, .F. ) ;
#75258=CARTESIAN_POINT ( 'NONE',  ( 166.2739464712248321, 282.9472121807791609, 8.907762031810820602 ) ) ;
#75261=CARTESIAN_POINT ( 'NONE',  ( 162.6220573360242270, 248.9773295930640131, 10.49878733418918486 ) ) ;
#75262=CARTESIAN_POINT ( 'NONE',  ( 188.2323859076021222, 260.7681868484680763, 2.706230261455492059 ) ) ;
#75263=CARTESIAN_POINT ( 'NONE',  ( 149.5706976103993782, 276.2301179004945197, -5.400069381014914960 ) ) ;
#75264=DIRECTION ( 'NONE',  ( -0.8660254037844387076, -0.4999999999999998890, -0.000000000000000000 ) ) ;
#75266=CARTESIAN_POINT ( 'NONE',  ( 168.1614549503004525, 252.8790457503890536, 11.93473075534227057 ) ) ;
#75268=VERTEX_POINT ( 'NONE', #13766 ) ;
#75269=CARTESIAN_POINT ( 'NONE',  ( 181.8129518053731033, 270.5384970965435514, -17.23398818032472946 ) ) ;
#75273=CARTESIAN_POINT ( 'NONE',  ( 11.37297787527554327, 165.8262482093457777, 3.021315404115420679E-15 ) ) ;
#75274=CARTESIAN_POINT ( 'NONE',  ( -3.532187684056895538, 158.7677522451418213, -5.000000000000041744 ) ) ;
#75275=EDGE_CURVE ( 'NONE', #100037, #99756, #90131, .T. ) ;
#75276=CARTESIAN_POINT ( 'NONE',  ( 193.1480066626644714, 267.5100469937302137, -10.98767188462725386 ) ) ;
#75278=CARTESIAN_POINT ( 'NONE',  ( 204.2488672143813346, 276.8775799267394291, -15.19253025301563831 ) ) ;
#75279=CARTESIAN_POINT ( 'NONE',  ( 172.0775005200765406, 286.7165937425170341, -10.58237651954697078 ) ) ;
#75280=CARTESIAN_POINT ( 'NONE',  ( 161.3261849411383650, 273.2032229615781489, 15.91718547624222957 ) ) ;
#75281=CARTESIAN_POINT ( 'NONE',  ( -9.107486540969064848, 174.7369531367911293, -4.594050593750048428 ) ) ;
#75284=CARTESIAN_POINT ( 'NONE',  ( 185.0535551050948868, 295.3960374749880771, 8.450267053739612066 ) ) ;
#75286=EDGE_CURVE ( 'NONE', #61039, #96078, #70701, .T. ) ;
#75291=CARTESIAN_POINT ( 'NONE',  ( 185.2824853868734181, 297.7695098558858149, 4.231266468330407093 ) ) ;
#75292=CARTESIAN_POINT ( 'NONE',  ( 175.4037125437872362, 291.3959072482493298, 3.423790665827645352 ) ) ;
#75294=CARTESIAN_POINT ( 'NONE',  ( 163.2084678683261814, 247.9616367570234559, -11.19269778657885972 ) ) ;
#75296=CARTESIAN_POINT ( 'NONE',  ( 153.5742155153078272, 278.9749726662499825, 3.791783021084301097 ) ) ;
#75297=CARTESIAN_POINT ( 'NONE',  ( 30.59497298136257726, 176.2202760586659736, -5.415160957724236172E-17 ) ) ;
#75298=CARTESIAN_POINT ( 'NONE',  ( 118.1982478153434357, 248.2369531367911293, -4.594050593750048428 ) ) ;
#75300=CARTESIAN_POINT ( 'NONE',  ( 182.9052583267165915, 257.6403021703982290, -2.314827183511977360 ) ) ;
#75302=CARTESIAN_POINT ( 'NONE',  ( 175.7813307086614714, 281.8375084945754452, -14.19557829653598979 ) ) ;
#75304=CARTESIAN_POINT ( 'NONE',  ( 182.7190055043868142, 259.1992038300794547, 9.912833159430794794 ) ) ;
#75305=CARTESIAN_POINT ( 'NONE',  ( 183.9464132997153456, 275.0587871046172950, 16.36209078982390963 ) ) ;
#75306=CARTESIAN_POINT ( 'NONE',  ( 194.1789525331299728, 294.3191837825503967, -15.34533909744314961 ) ) ;
#75310=CARTESIAN_POINT ( 'NONE',  ( 51.18979252112020362, 200.3615022471902307, -10.00000000000009592 ) ) ;
#75311=CARTESIAN_POINT ( 'NONE',  ( 183.2174363127404320, 268.2244215103378338, -14.94466466708451158 ) ) ;
#75313=CARTESIAN_POINT ( 'NONE',  ( 172.5095176311965872, 263.6581028672348452, -15.42591371060134264 ) ) ;
#75314=EDGE_CURVE ( 'NONE', #38232, #54274, #6102, .T. ) ;
#75315=CARTESIAN_POINT ( 'NONE',  ( 104.3964885861764600, 221.8923013555410080, 4.594050593750050204 ) ) ;
#75318=CARTESIAN_POINT ( 'NONE',  ( 190.8094645593471341, 300.1553081486349015, 8.399847186519689757 ) ) ;
#75320=CARTESIAN_POINT ( 'NONE',  ( 196.1613785401733878, 290.8855212161054737, 15.98157687694135021 ) ) ;
#75322=DIRECTION ( 'NONE',  ( 0.4999999999999992784, -0.8660254037844390407, 0.000000000000000000 ) ) ;
#75323=CARTESIAN_POINT ( 'NONE',  ( 151.2964716097791325, 268.5938194963972592, -15.66250187539618111 ) ) ;
#75324=CARTESIAN_POINT ( 'NONE',  ( 162.9254136962317148, 277.9293967287522946, 13.77390558128574760 ) ) ;
#75328=ORIENTED_EDGE ( 'NONE', *, *, #21916, .F. ) ;
#75331=CARTESIAN_POINT ( 'NONE',  ( 196.8537322840589070, 267.5011318901352411, 9.757633572797876909 ) ) ;
#75332=CARTESIAN_POINT ( 'NONE',  ( 191.6653133782924670, 287.8825534954372642, -15.84478586218862262 ) ) ;
#75334=CARTESIAN_POINT ( 'NONE',  ( 159.6978881494930249, 254.0421391940632532, 15.34888828951022610 ) ) ;
#75336=CARTESIAN_POINT ( 'NONE',  ( 169.4318521445344174, 252.1923235025763574, -8.759566905232736289 ) ) ;
#75337=CARTESIAN_POINT ( 'NONE',  ( 129.2042476453683264, 258.7365022471903444, 2.944929066748280225E-16 ) ) ;
#75339=DIRECTION ( 'NONE',  ( -0.8660254037844359321, -0.5000000000000051070, -0.000000000000000000 ) ) ;
#75342=EDGE_LOOP ( 'NONE', ( #46170, #51642, #8297, #21628 ) ) ;
#75343=CARTESIAN_POINT ( 'NONE',  ( 196.4555699717270159, 265.3045897231015147, -4.475125793179218547 ) ) ;
#75346=CARTESIAN_POINT ( 'NONE',  ( 181.5586684916292199, 291.2330295745708781, -11.30866533355154857 ) ) ;
#75350=CARTESIAN_POINT ( 'NONE',  ( 205.7652784884614618, 274.2510785548626586, 10.78649346335630632 ) ) ;
#75351=CARTESIAN_POINT ( 'NONE',  ( 190.8346167705416292, 278.0885925990914984, -16.91238342368501080 ) ) ;
#75352=CARTESIAN_POINT ( 'NONE',  ( 153.9376410758373197, 264.0191797897847437, -17.98316443701128264 ) ) ;
#75353=CARTESIAN_POINT ( 'NONE',  ( 200.9521687275011175, 282.5876292032514243, -18.16013154125647944 ) ) ;
#75364=ORIENTED_EDGE ( 'NONE', *, *, #14892, .T. ) ;
#75366=CARTESIAN_POINT ( 'NONE',  ( 174.5008544261717134, 257.2940615678410268, -12.04793888739825114 ) ) ;
#75367=CARTESIAN_POINT ( 'NONE',  ( 164.9505546126307820, 273.5171455901430591, -15.23424786856183211 ) ) ;
#75368=CARTESIAN_POINT ( 'NONE',  ( 179.3609674101392670, 270.6429099854789229, -17.53201452148147865 ) ) ;
#75369=CARTESIAN_POINT ( 'NONE',  ( 197.4318886344639168, 273.2323872680082104, -13.37235133448358582 ) ) ;
#75371=CARTESIAN_POINT ( 'NONE',  ( 167.5062897759243867, 286.2136144727477927, -4.753602936323340522 ) ) ;
#75373=CARTESIAN_POINT ( 'NONE',  ( 181.8753390830952981, 257.0193592213445868, 5.050065929983023949 ) ) ;
#75374=CARTESIAN_POINT ( 'NONE',  ( 111.1892885731694065, 228.8768266524159856, -9.188101187500091527 ) ) ;
#75377=CARTESIAN_POINT ( 'NONE',  ( 191.5502192675250797, 274.9178017426596057, 16.83841206479500840 ) ) ;
#75381=CARTESIAN_POINT ( 'NONE',  ( 164.4115384698665423, 246.2497411554974178, -2.154666020448770425 ) ) ;
#75382=CARTESIAN_POINT ( 'NONE',  ( 196.4677418905696129, 290.3548843276421394, 17.08610552292358520 ) ) ;
#75389=CARTESIAN_POINT ( 'NONE',  ( 37.58366506746438773, 204.0530062829863027, 1.101618078115930403E-13 ) ) ;
#75390=ORIENTED_EDGE ( 'NONE', *, *, #48031, .F. ) ;
#75391=CARTESIAN_POINT ( 'NONE',  ( 192.1803104008425009, 263.7327182331824815, -8.277698982533909344 ) ) ;
#75392=CARTESIAN_POINT ( 'NONE',  ( 156.0770925354950407, 262.0035003640769560, 17.00396438526712828 ) ) ;
#75394=CARTESIAN_POINT ( 'NONE',  ( 132.0211419364472363, 235.4824982072973683, 3.021315404115420679E-15 ) ) ;
#75396=CARTESIAN_POINT ( 'NONE',  ( 201.1060504099706350, 282.3210983108598384, -18.18000168485860257 ) ) ;
#75397=VERTEX_POINT ( 'NONE', #38310 ) ;
#75398=CARTESIAN_POINT ( 'NONE',  ( 147.2494378675467033, 275.6034875578896504, 3.639370109197119341 ) ) ;
#75403=CARTESIAN_POINT ( 'NONE',  ( 192.8280828621116143, 271.6925081571723695, -14.86971951722050989 ) ) ;
#75406=CARTESIAN_POINT ( 'NONE',  ( 122.0674962994202275, 252.8297689869269504, -2.679491924311252493 ) ) ;
#75407=CARTESIAN_POINT ( 'NONE',  ( 191.3433485266361060, 283.5098745242009386, -16.59037939125511230 ) ) ;
#75409=CARTESIAN_POINT ( 'NONE',  ( 83.72013207082297015, 209.9548013555409796, -4.594050593750042211 ) ) ;
#75410=CARTESIAN_POINT ( 'NONE',  ( 159.2713554375903300, 254.7809155221686410, -15.70062444474382168 ) ) ;
#75412=CARTESIAN_POINT ( 'NONE',  ( 162.7738416911812180, 248.7144313781379310, -11.09964294874192525 ) ) ;
#75413=ADVANCED_FACE ( 'NONE', ( #8922 ), #70721, .T. ) ;
#75415=CARTESIAN_POINT ( 'NONE',  ( 207.7320178805681508, 270.8445860024863237, -5.379955943374661764 ) ) ;
#75417=CARTESIAN_POINT ( 'NONE',  ( 185.9122197414204720, 265.5112680014551074, 13.45063299295054016 ) ) ;
#75418=CARTESIAN_POINT ( 'NONE',  ( 118.8119427999551476, 232.7365022471901739, -10.00000000000009237 ) ) ;
#75421=CARTESIAN_POINT ( 'NONE',  ( 157.7367892284080995, 270.6845674506320165, -15.10799881823672131 ) ) ;
#75430=CARTESIAN_POINT ( 'NONE',  ( 56.62968813474974894, 197.3768266524159856, -9.188101187500093303 ) ) ;
#75432=CARTESIAN_POINT ( 'NONE',  ( 171.3915261951946150, 286.6500415720103092, 7.434736897587270299 ) ) ;
#75433=CARTESIAN_POINT ( 'NONE',  ( -12.46307465703604400, 163.6115022471902591, 10.00000000000009592 ) ) ;
#75435=CARTESIAN_POINT ( 'NONE',  ( 202.9485587013432450, 270.0648872230868278, -6.527258153556268816 ) ) ;
#75438=CARTESIAN_POINT ( 'NONE',  ( 176.4777781830643733, 275.0219395333674584, 16.71559492492674437 ) ) ;
#75439=CARTESIAN_POINT ( 'NONE',  ( 182.1775460995084188, 281.0620400832397081, -16.66492851291912203 ) ) ;
#75441=CARTESIAN_POINT ( 'NONE',  ( 192.1779685593947420, 266.1842805242176269, 11.64530923862864142 ) ) ;
#75444=CARTESIAN_POINT ( 'NONE',  ( 103.0791479645378814, 216.9865022471901455, 1.119607411625061291E-15 ) ) ;
#75445=CARTESIAN_POINT ( 'NONE',  ( 200.7079229450794173, 283.0106753079404029, 16.90512463913211505 ) ) ;
#75446=CARTESIAN_POINT ( 'NONE',  ( 165.2257725011909599, 269.6626922470395016, -16.28745125698258889 ) ) ;
#75448=CARTESIAN_POINT ( 'NONE',  ( 55.49285624440017273, 202.8458772461660260, 9.188101187500095079 ) ) ;
#75450=CARTESIAN_POINT ( 'NONE',  ( 166.2024314945517744, 265.3097119368810581, 16.55270856133939006 ) ) ;
#75454=CARTESIAN_POINT ( 'NONE',  ( 175.5738744261513773, 288.6452583002058532, 10.69039192277817207 ) ) ;
#75456=B_SPLINE_CURVE_WITH_KNOTS ( 'NONE', 3,
 ( #9979, #41349, #8466, #25678 ),
 .UNSPECIFIED., .F., .F.,
 ( 4, 4 ),
 ( 0.006801831041879702333, 0.01491549308688025835 ),
 .UNSPECIFIED. ) ;
#75458=CARTESIAN_POINT ( 'NONE',  ( 175.8941769947522005, 273.9942606850552238, -16.49495549152694451 ) ) ;
#75459=CARTESIAN_POINT ( 'NONE',  ( 206.7093368940924449, 271.6371694531807748, -6.526174084559485777 ) ) ;
#75460=CARTESIAN_POINT ( 'NONE',  ( 204.2992694100975939, 276.7902807629455992, 13.99537586056731620 ) ) ;
#75461=ORIENTED_EDGE ( 'NONE', *, *, #86860, .F. ) ;
#75467=CARTESIAN_POINT ( 'NONE',  ( 182.1942909992290254, 284.0346785242947476, 14.95718866600176966 ) ) ;
#75470=EDGE_CURVE ( 'NONE', #39284, #79412, #5402, .T. ) ;
#75473=CARTESIAN_POINT ( 'NONE',  ( 159.2847755103654777, 282.3438696241352659, -3.266643173123188415 ) ) ;
#75474=CARTESIAN_POINT ( 'NONE',  ( 60.19284827774804114, 198.8927522451417644, -10.00000000000009237 ) ) ;
#75475=CARTESIAN_POINT ( 'NONE',  ( 162.7459776558209228, 248.7626933030860812, -9.895605163646791880 ) ) ;
#75476=CARTESIAN_POINT ( 'NONE',  ( 164.1224127655298730, 246.3786377597482158, 7.356982420601481998 ) ) ;
#75478=CARTESIAN_POINT ( 'NONE',  ( 159.9307118030769175, 253.6388767968520881, 16.60600887889890487 ) ) ;
#75480=CARTESIAN_POINT ( 'NONE',  ( 161.0194789840985550, 262.9636063602296758, -17.49589281607644864 ) ) ;
#75482=CARTESIAN_POINT ( 'NONE',  ( 125.6141109788952122, 234.1423013555409796, -4.594050593750043987 ) ) ;
#75483=CARTESIAN_POINT ( 'NONE',  ( 75.14063404487711750, 220.3149278399160664, -9.188101187500095079 ) ) ;
#75484=ORIENTED_EDGE ( 'NONE', *, *, #31894, .F. ) ;
#75485=CARTESIAN_POINT ( 'NONE',  ( 170.5242561500533895, 263.7951878494171183, 15.83046558349961863 ) ) ;
#75488=CARTESIAN_POINT ( 'NONE',  ( 160.3453973192849276, 253.3356115996859899, 14.63839832439733968 ) ) ;
#75491=ORIENTED_EDGE ( 'NONE', *, *, #89260, .T. ) ;
#75493=CARTESIAN_POINT ( 'NONE',  ( 195.2631479605611560, 291.6323043634218379, -15.73646530299744839 ) ) ;
#75494=CARTESIAN_POINT ( 'NONE',  ( -6.583630525541995127, 178.5530062829863027, -4.648177544792955347E-16 ) ) ;
#75495=CARTESIAN_POINT ( 'NONE',  ( 147.2405539530007559, 275.6188749492528132, 0.4306668706573002492 ) ) ;
#75497=CARTESIAN_POINT ( 'NONE',  ( 193.9844289374573520, 294.6561085335266625, 15.49818881749970245 ) ) ;
#75502=CARTESIAN_POINT ( 'NONE',  ( 153.3544108199959908, 265.0293642254135307, -17.49105661178601423 ) ) ;
#75503=CARTESIAN_POINT ( 'NONE',  ( 185.0684497205900527, 286.3477220876792444, 16.15350733335134237 ) ) ;
#75504=ORIENTED_EDGE ( 'NONE', *, *, #52812, .F. ) ;
#75505=CARTESIAN_POINT ( 'NONE',  ( -17.09196077473970021, 172.4860189848785410, -2.679491924311252049 ) ) ;
#75508=CARTESIAN_POINT ( 'NONE',  ( 165.0538309624641613, 244.7653741195639157, 2.311334310144196547 ) ) ;
#75509=CARTESIAN_POINT ( 'NONE',  ( 198.9303151507368170, 281.1112718272049165, 17.08711449059368803 ) ) ;
#75511=CARTESIAN_POINT ( 'NONE',  ( 136.3579783227721691, 249.5333772461660544, 9.188101187500095079 ) ) ;
#75515=CARTESIAN_POINT ( 'NONE',  ( 182.0583737030646319, 257.8139296662238280, 6.555026806704957743 ) ) ;
#75523=CARTESIAN_POINT ( 'NONE',  ( 185.1300216526354063, 277.5058458126731580, -16.84358915254627576 ) ) ;
#75524=CARTESIAN_POINT ( 'NONE',  ( 167.5907823061452291, 249.2350603960721855, -5.636120817613099909 ) ) ;
#75527=CARTESIAN_POINT ( 'NONE',  ( 195.1671348588630508, 263.5382602011624158, 0.8553596245369967654 ) ) ;
#75529=CARTESIAN_POINT ( 'NONE',  ( 185.8834930517967337, 282.2059964265092162, 16.17713989960437360 ) ) ;
#75530=ADVANCED_FACE ( 'NONE', ( #37747 ), #7351, .T. ) ;
#75531=CARTESIAN_POINT ( 'NONE',  ( 205.0994677818405023, 275.4042965269534307, -14.14519517703424789 ) ) ;
#75532=CARTESIAN_POINT ( 'NONE',  ( 193.3472389827650204, 268.3320133866042170, 12.76089158629410747 ) ) ;
#75535=CARTESIAN_POINT ( 'NONE',  ( 205.4925884257800988, 274.0740247280971857, 10.80283695292349222 ) ) ;
#75537=CARTESIAN_POINT ( 'NONE',  ( 159.7953104873542145, 253.8733987550956783, 15.41928249285404107 ) ) ;
#75538=CARTESIAN_POINT ( 'NONE',  ( 161.7101054567844187, 250.5568765819650707, 14.25969465237331235 ) ) ;
#75539=CARTESIAN_POINT ( 'NONE',  ( -2.124636079309504488, 160.3923013555410080, 4.594050593750050204 ) ) ;
#75540=CARTESIAN_POINT ( 'NONE',  ( 175.4324593603440974, 286.4533427740436196, -12.30467070008952213 ) ) ;
#75541=VERTEX_POINT ( 'NONE', #68654 ) ;
#75542=EDGE_CURVE ( 'NONE', #35189, #95819, #12590, .T. ) ;
#75545=CARTESIAN_POINT ( 'NONE',  ( 202.4876139799157500, 274.1054391224496953, -12.98901669480548016 ) ) ;
#75546=CARTESIAN_POINT ( 'NONE',  ( 199.0773057068961123, 285.8349872121713702, -17.17316764978006560 ) ) ;
#75547=CARTESIAN_POINT ( 'NONE',  ( 9.485603764116874004, 164.0327760586659451, 1.948934522072302763E-15 ) ) ;
#75551=CARTESIAN_POINT ( 'NONE',  ( 172.4538997260322617, 272.0033172842936438, -16.41376745784389968 ) ) ;
#75553=AXIS2_PLACEMENT_3D ( 'NONE', #19790, #51676, #12693 ) ;
#75554=CARTESIAN_POINT ( 'NONE',  ( 150.0749816411065183, 276.6459287350622844, 4.378659120374928548 ) ) ;
#75555=CARTESIAN_POINT ( 'NONE',  ( 178.4558349409154232, 255.0179201197129828, -3.920679784167997894 ) ) ;
#75556=CARTESIAN_POINT ( 'NONE',  ( 150.3774144590728952, 270.1856731764797814, 13.91914410364283938 ) ) ;
#75558=CARTESIAN_POINT ( 'NONE',  ( 58.91185237153143106, 211.4865022471903444, -10.00000000000009415 ) ) ;
#75560=CARTESIAN_POINT ( 'NONE',  ( 190.3049670482083684, 301.0291234702190764, 0.2225066852051815758 ) ) ;
#75561=CARTESIAN_POINT ( 'NONE',  ( 14.19444334931225349, 172.8768266524160140, 9.188101187500098632 ) ) ;
#75562=CARTESIAN_POINT ( 'NONE',  ( 168.1019601029094019, 286.2093627858199056, 4.093480230534757069 ) ) ;
#75565=CARTESIAN_POINT ( 'NONE',  ( 202.1602617260373336, 279.5841831652249425, -15.84922531218295383 ) ) ;
#75566=CARTESIAN_POINT ( 'NONE',  ( 164.9971748156432056, 244.8635054444190757, -1.825016704039769788 ) ) ;
#75567=CARTESIAN_POINT ( 'NONE',  ( 185.1770359163484159, 266.8001431404497907, 13.86940662139324765 ) ) ;
#75569=CARTESIAN_POINT ( 'NONE',  ( 163.9630091648389509, 281.4969130715203960, 8.857997127697792905 ) ) ;
#75572=DIRECTION ( 'NONE',  ( 0.5000000000000048850, -0.8660254037844358210, 0.000000000000000000 ) ) ;
#75576=ORIENTED_EDGE ( 'NONE', *, *, #47299, .F. ) ;
#75577=VECTOR ( 'NONE', #78007, 1000.000000000000000 ) ;
#75578=CARTESIAN_POINT ( 'NONE',  ( 183.2126764927348290, 289.7799306247588333, 12.21646338406959842 ) ) ;
#75579=CARTESIAN_POINT ( 'NONE',  ( 163.0804386853320125, 262.7275182220299712, -17.72388574752874746 ) ) ;
#75583=CARTESIAN_POINT ( 'NONE',  ( 196.0587100571994483, 289.0633482449420626, -17.27351923437598913 ) ) ;
#75586=CARTESIAN_POINT ( 'NONE',  ( 155.2193237801463113, 261.7992402267395846, -18.58295809893692407 ) ) ;
#75590=CARTESIAN_POINT ( 'NONE',  ( 202.3522217946735111, 279.7792213403169512, 15.59347206985308709 ) ) ;
#75592=ORIENTED_EDGE ( 'NONE', *, *, #79610, .F. ) ;
#75597=ORIENTED_EDGE ( 'NONE', *, *, #83416, .F. ) ;
#75598=CARTESIAN_POINT ( 'NONE',  ( -17.42236680055705023, 149.2012482093457777, 0.000000000000000000 ) ) ;
#75601=CARTESIAN_POINT ( 'NONE',  ( 205.8379285891498682, 274.1252448892948905, 10.44730901608240181 ) ) ;
#75603=ORIENTED_EDGE ( 'NONE', *, *, #38605, .T. ) ;
#75604=CARTESIAN_POINT ( 'NONE',  ( 148.9719199701866899, 272.6200610409887872, 12.59512981512031438 ) ) ;
#75605=CARTESIAN_POINT ( 'NONE',  ( 172.3369791656317034, 263.9050024373092924, -16.81851492143085025 ) ) ;
#75607=CARTESIAN_POINT ( 'NONE',  ( 158.5161842154787166, 275.0912836277667566, -13.81901676271391466 ) ) ;
#75611=VERTEX_POINT ( 'NONE', #30158 ) ;
#75612=VERTEX_POINT ( 'NONE', #23537 ) ;
#75613=CARTESIAN_POINT ( 'NONE',  ( 156.6195539527090546, 266.7731622753219654, -16.18964406384344912 ) ) ;
#75614=CARTESIAN_POINT ( 'NONE',  ( 190.9441801652054096, 299.9219738747156043, -4.765040093794296716 ) ) ;
#75617=CARTESIAN_POINT ( 'NONE',  ( 192.8132846206021611, 296.6845899933152850, 11.53748932578252351 ) ) ;
#75618=CARTESIAN_POINT ( 'NONE',  ( 191.1932856887581522, 299.4905104514762684, 9.694084360102674935 ) ) ;
#75619=CARTESIAN_POINT ( 'NONE',  ( 146.5502055023624735, 276.8145935406849389, 0.3770461397900869427 ) ) ;
#75622=CARTESIAN_POINT ( 'NONE',  ( 165.0297293518065658, 244.8071193337670195, 2.517333243890161665 ) ) ;
#75623=CARTESIAN_POINT ( 'NONE',  ( 196.8363552541316324, 289.7164272536036265, -17.80258609350122967 ) ) ;
#75626=CARTESIAN_POINT ( 'NONE',  ( 171.5288298918311511, 288.9004815652406251, 4.237906360154932273 ) ) ;
#75627=FACE_OUTER_BOUND ( 'NONE', #9901, .T. ) ;
#75630=CARTESIAN_POINT ( 'NONE',  ( 149.7482486646325412, 271.2754202988347743, -12.05835948757660958 ) ) ;
#75632=CARTESIAN_POINT ( 'NONE',  ( 149.3018356595837588, 273.4567121134075478, 10.20698179752245949 ) ) ;
#75634=CARTESIAN_POINT ( 'NONE',  ( 179.6164226443064535, 282.7900583135175339, -15.54602365610343107 ) ) ;
#75635=CARTESIAN_POINT ( 'NONE',  ( 189.9455075854687323, 301.6517255229458101, -1.253142702374338002 ) ) ;
#75637=CARTESIAN_POINT ( 'NONE',  ( 208.3829315663354862, 269.7171704273955015, -1.768817828503133072 ) ) ;
#75639=( BOUNDED_CURVE ( )  B_SPLINE_CURVE ( 2, ( #67676, #89542, #13007, #43867, #5387, #36273, #20103, #67172, #91019 ),
 .UNSPECIFIED., .F., .T. ) 
 B_SPLINE_CURVE_WITH_KNOTS ( ( 3, 2, 2, 2, 3 ),
 ( 0.3508064516129032473, 0.3521505376344086224, 0.3548387096774193727, 0.3575268817204301230, 0.3588709677419354982 ),
 .UNSPECIFIED. ) 
 CURVE ( )  GEOMETRIC_REPRESENTATION_ITEM ( )  RATIONAL_B_SPLINE_CURVE ( ( 0.9330127018922194093, 0.9330127018922194093, 1.000000000000000000, 0.8660254037844387076, 1.000000000000000000, 0.8660254037844387076, 1.000000000000000000, 0.9330127018922194093, 0.9330127018922194093 ) ) 
 REPRESENTATION_ITEM ( '' )  );
#75642=CARTESIAN_POINT ( 'NONE',  ( 36.81016237556811177, 205.3927522451419350, 2.944929066748280225E-16 ) ) ;
#75643=CARTESIAN_POINT ( 'NONE',  ( 105.6408794604690797, 240.9869531367911293, 4.594050593750046652 ) ) ;
#75644=CARTESIAN_POINT ( 'NONE',  ( 72.26538907532096800, 200.9824982072973967, 3.021315404115420679E-15 ) ) ;
#75646=CARTESIAN_POINT ( 'NONE',  ( 157.2168982216852555, 258.3393398020932636, 18.09635675623264106 ) ) ;
#75647=CARTESIAN_POINT ( 'NONE',  ( 175.2741237188109551, 253.4266919301918506, -3.879795126654972393 ) ) ;
#75649=CARTESIAN_POINT ( 'NONE',  ( 36.54820344085055694, 204.1589784336661637, -6.496448406907675876E-16 ) ) ;
#75655=CARTESIAN_POINT ( 'NONE',  ( 179.7777640920925535, 266.8932340374666978, 15.06726368060596144 ) ) ;
#75657=CARTESIAN_POINT ( 'NONE',  ( 147.1199024702499969, 275.8278494473859723, 5.224467159276165340 ) ) ;
#75658=CARTESIAN_POINT ( 'NONE',  ( 205.7872507830675204, 272.2130214242461079, -9.506855900917111413 ) ) ;
#75661=CARTESIAN_POINT ( 'NONE',  ( 177.5073464959093315, 286.2605698986350831, -12.10074426044735674 ) ) ;
#75664=CARTESIAN_POINT ( 'NONE',  ( 108.6902708896766114, 226.8927522451418213, 10.00000000000009592 ) ) ;
#75668=CARTESIAN_POINT ( 'NONE',  ( 202.2603678735342214, 280.3217618159037556, 16.49712126737133744 ) ) ;
#75669=CARTESIAN_POINT ( 'NONE',  ( 207.6523394534040392, 270.9825930866021508, -2.115019688068903392 ) ) ;
#75670=CARTESIAN_POINT ( 'NONE',  ( 3.097972219676621730, 184.8464784336661637, 1.353441290958777327E-15 ) ) ;
#75671=B_SPLINE_CURVE_WITH_KNOTS ( 'NONE', 3,
 ( #45382, #75818, #83433, #90039 ),
 .UNSPECIFIED., .F., .F.,
 ( 4, 4 ),
 ( 0.009406675354063229882, 0.01769731902523580952 ),
 .UNSPECIFIED. ) ;
#75675=DIRECTION ( 'NONE',  ( -0.8660254037844387076, -0.4999999999999998890, -0.000000000000000000 ) ) ;
#75676=CARTESIAN_POINT ( 'NONE',  ( 175.3741314181362725, 286.6665286446898904, 10.50185128592887018 ) ) ;
#75677=CARTESIAN_POINT ( 'NONE',  ( 58.68649846873780263, 198.5643266524160140, 9.188101187500095079 ) ) ;
#75678=CARTESIAN_POINT ( 'NONE',  ( 207.6932907333322191, 270.9116633891313199, 2.120963121341169710 ) ) ;
#75681=CARTESIAN_POINT ( 'NONE',  ( 207.6860335175200589, 270.9242332556395922, 6.913225035677485586 ) ) ;
#75682=VERTEX_POINT ( 'NONE', #85405 ) ;
#75683=CARTESIAN_POINT ( 'NONE',  ( 207.0624025450594843, 270.0043937851150417, -2.644299678167422840 ) ) ;
#75684=CARTESIAN_POINT ( 'NONE',  ( 8.754547735682661980, 185.8615022471903160, 5.000000000000046185 ) ) ;
#75685=FACE_OUTER_BOUND ( 'NONE', #47695, .T. ) ;
#75687=CARTESIAN_POINT ( 'NONE',  ( 138.1714793337695824, 241.3923013555409796, 4.594050593750050204 ) ) ;
#75689=CARTESIAN_POINT ( 'NONE',  ( 207.1023286545539861, 271.9352397349218791, -8.358798036041973134 ) ) ;
#75691=CARTESIAN_POINT ( 'NONE',  ( 69.21394623383592659, 210.7677522451418497, 10.00000000000009592 ) ) ;
#75693=CARTESIAN_POINT ( 'NONE',  ( 188.5998214029316102, 289.4849150055601399, 14.43259912634508524 ) ) ;
#75695=ORIENTED_EDGE ( 'NONE', *, *, #49962, .F. ) ;
#75696=CARTESIAN_POINT ( 'NONE',  ( 150.7530568467738590, 269.5350414755053521, 15.60317050893315916 ) ) ;
#75697=CYLINDRICAL_SURFACE ( 'NONE', #4073, 10.00000000000010658 ) ;
#75698=AXIS2_PLACEMENT_3D ( 'NONE', #9608, #25279, #56165 ) ;
#75700=CARTESIAN_POINT ( 'NONE',  ( 169.6285385964465604, 266.0829471737013705, -16.93693285811728799 ) ) ;
#75707=EDGE_CURVE ( 'NONE', #75268, #7831, #33013, .T. ) ;
#75709=B_SPLINE_SURFACE_WITH_KNOTS ( 'NONE', 3, 1, ( 
 ( #70276, #86548 ),
 ( #93622, #24189 ),
 ( #55072, #47480 ),
 ( #78404, #94127 ),
 ( #17079, #71306 ),
 ( #32778, #72312 ),
 ( #25701, #96133 ),
 ( #34288, #87568 ),
 ( #66188, #10491 ),
 ( #41373, #40863 ),
 ( #50475, #48995 ),
 ( #79931, #58085 ),
 ( #19114, #33285 ),
 ( #95647, #33810 ),
 ( #3414, #18602 ),
 ( #19617, #80945 ),
 ( #26194, #57073 ),
 ( #49481, #49990 ),
 ( #80437, #65185 ),
 ( #27701, #89541 ),
 ( #26687, #48495 ),
 ( #57575, #88548 ),
 ( #42367, #11513 ),
 ( #73301, #3892 ),
 ( #71810, #34774 ),
 ( #65675, #27196 ),
 ( #89065, #81428 ),
 ( #79436, #20102 ),
 ( #23046, #25310 ),
 ( #89661, #57199 ),
 ( #41503, #34413 ),
 ( #57699, #3537 ),
 ( #18725, #19249 ),
 ( #50114, #33938 ) ),
 .UNSPECIFIED., .T., .F., .F.,
 ( 4, 2, 2, 2, 2, 2, 2, 2, 2, 2, 2, 2, 2, 2, 2, 2, 4 ),
 ( 2, 2 ),
 ( 0.000000000000000000, 0.06250000000000000000, 0.1250000000000000000, 0.1875000000000000000, 0.2500000000000000000, 0.3125000000000000000, 0.3750000000000000000, 0.4375000000000000000, 0.5000000000000000000, 0.5625000000000000000, 0.6250000000000000000, 0.6875000000000000000, 0.7500000000000000000, 0.8125000000000000000, 0.8750000000000000000, 0.9375000000000000000, 1.000000000000000000 ),
 ( 0.000000000000000000, 1.000000000000000000 ),
 .UNSPECIFIED. ) ;
#75710=CARTESIAN_POINT ( 'NONE',  ( 200.6634772367119410, 281.5104481654628898, -17.03558376807434271 ) ) ;
#75711=CARTESIAN_POINT ( 'NONE',  ( 196.2305329650964723, 270.9041150931136031, 12.09698969586446538 ) ) ;
#75712=CARTESIAN_POINT ( 'NONE',  ( 98.36217659263859048, 216.0494855054051868, -2.679491924311248496 ) ) ;
#75714=CARTESIAN_POINT ( 'NONE',  ( 153.1983976505312626, 265.2995869615763809, -17.69657798691567763 ) ) ;
#75720=CARTESIAN_POINT ( 'NONE',  ( 149.6036070299368532, 271.5259469590175740, 11.63513718912356865 ) ) ;
#75724=CARTESIAN_POINT ( 'NONE',  ( 191.7247331938518187, 298.5700163710982338, -9.650650827884682315 ) ) ;
#75726=CARTESIAN_POINT ( 'NONE',  ( 181.4930680486588699, 260.3623518102999697, -11.98802389789063660 ) ) ;
#75727=CARTESIAN_POINT ( 'NONE',  ( 163.7136804588959649, 247.0865828815331042, 6.783386239354816105 ) ) ;
#75730=CARTESIAN_POINT ( 'NONE',  ( 97.03527265400872182, 217.6423013555409796, -4.594050593750043987 ) ) ;
#75731=CARTESIAN_POINT ( 'NONE',  ( 202.9416383086232543, 279.1417668086349977, 15.32562689463440364 ) ) ;
#75732=CARTESIAN_POINT ( 'NONE',  ( 177.9014365079093807, 268.9747928436916595, -16.77994175735417670 ) ) ;
#75735=B_SPLINE_SURFACE_WITH_KNOTS ( 'NONE', 3, 1, ( 
 ( #22525, #45801 ),
 ( #4856, #35738 ),
 ( #29143, #66633 ),
 ( #51939, #97564 ),
 ( #28131, #20553 ),
 ( #51431, #82396 ),
 ( #62493, #15914 ),
 ( #31107, #25011 ),
 ( #24517, #61514 ),
 ( #85892, #8817 ),
 ( #39686, #55394 ),
 ( #78237, #84859 ),
 ( #100043, #92947 ),
 ( #86381, #715 ),
 ( #222, #78734 ),
 ( #1227, #77741 ),
 ( #69617, #61995 ),
 ( #31601, #24015 ),
 ( #38709, #15403 ),
 ( #94457, #23500 ),
 ( #92462, #93463 ),
 ( #16912, #47801 ),
 ( #70614, #9325 ),
 ( #32109, #55890 ),
 ( #86884, #69117 ),
 ( #38198, #46295 ),
 ( #54392, #63018 ),
 ( #40198, #47311 ),
 ( #85368, #46819 ),
 ( #23007, #8326 ),
 ( #54912, #39191 ),
 ( #77223, #30629 ),
 ( #71142, #1742 ),
 ( #70106, #17417 ) ),
 .UNSPECIFIED., .T., .F., .F.,
 ( 4, 2, 2, 2, 2, 2, 2, 2, 2, 2, 2, 2, 2, 2, 2, 2, 4 ),
 ( 2, 2 ),
 ( 0.000000000000000000, 0.06250000000000000000, 0.1250000000000000000, 0.1875000000000000000, 0.2500000000000000000, 0.3125000000000000000, 0.3750000000000000000, 0.4375000000000000000, 0.5000000000000000000, 0.5625000000000000000, 0.6250000000000000000, 0.6875000000000000000, 0.7500000000000000000, 0.8125000000000000000, 0.8750000000000000000, 0.9375000000000000000, 1.000000000000000000 ),
 ( 0.000000000000000000, 1.000000000000000000 ),
 .UNSPECIFIED. ) ;
#75738=VERTEX_POINT ( 'NONE', #66551 ) ;
#75739=ORIENTED_EDGE ( 'NONE', *, *, #79862, .T. ) ;
#75743=ORIENTED_EDGE ( 'NONE', *, *, #54935, .T. ) ;
#75744=CARTESIAN_POINT ( 'NONE',  ( 208.3057440179679531, 269.8508631828800617, 2.969924427282375046 ) ) ;
#75747=CARTESIAN_POINT ( 'NONE',  ( 200.7694952279801157, 282.9040289856181403, -17.94628235092568502 ) ) ;
#75750=CARTESIAN_POINT ( 'NONE',  ( 171.2743479101317234, 254.4242377521371736, -11.94796457435898951 ) ) ;
#75752=DIRECTION ( 'NONE',  ( -0.8660254037844387076, -0.4999999999999998890, -0.000000000000000000 ) ) ;
#75754=EDGE_LOOP ( 'NONE', ( #74469, #6465, #19672, #56180 ) ) ;
#75755=CARTESIAN_POINT ( 'NONE',  ( 164.2963363950948690, 281.6989409824586801, 8.833678480319404613 ) ) ;
#75758=ORIENTED_EDGE ( 'NONE', *, *, #40455, .T. ) ;
#75760=CARTESIAN_POINT ( 'NONE',  ( 203.0535368433499457, 278.9479528611958585, 16.46202213522710167 ) ) ;
#75762=CARTESIAN_POINT ( 'NONE',  ( 161.3205084827974076, 281.4276874649026468, -6.572659893739726478 ) ) ;
#75763=CARTESIAN_POINT ( 'NONE',  ( 165.5366541472494362, 246.9067919256106620, -2.119420010412345956 ) ) ;
#75765=CARTESIAN_POINT ( 'NONE',  ( 200.1782072557437857, 283.9281697954355650, 18.05177561285849208 ) ) ;
#75766=CARTESIAN_POINT ( 'NONE',  ( 157.9927698565683727, 281.0302174119535721, 1.994413190729223739 ) ) ;
#75768=CARTESIAN_POINT ( 'NONE',  ( 181.5151252095495806, 271.0695012673220390, -15.95595848548451023 ) ) ;
#75770=AXIS2_PLACEMENT_3D ( 'NONE', #48140, #61822, #54215 ) ;
#75771=CARTESIAN_POINT ( 'NONE',  ( 3.125382611083808104, 182.6115022471903160, -5.000000000000047962 ) ) ;
#75772=CARTESIAN_POINT ( 'NONE',  ( 4.767222435543961190, 166.8927522451418213, 10.00000000000009592 ) ) ;
#75775=CARTESIAN_POINT ( 'NONE',  ( 188.1018771210319471, 260.4230313274653099, 6.875771660441075461 ) ) ;
#75777=CARTESIAN_POINT ( 'NONE',  ( 163.3365390452323425, 247.7398109716368424, -8.140084928332512959 ) ) ;
#75780=CARTESIAN_POINT ( 'NONE',  ( 164.5539697625973190, 274.3695635373503023, 14.76467764503104441 ) ) ;
#75781=CARTESIAN_POINT ( 'NONE',  ( -7.645548028435306342, 157.2048013555409796, 4.594050593750051981 ) ) ;
#75783=ADVANCED_FACE ( 'NONE', ( #88934 ), #6241, .T. ) ;
#75784=CARTESIAN_POINT ( 'NONE',  ( 162.8386403195304410, 249.0994062285972461, 10.29435687412694911 ) ) ;
#75792=CARTESIAN_POINT ( 'NONE',  ( 202.0980293819432916, 280.6029403313636408, -17.25107598010587751 ) ) ;
#75794=CARTESIAN_POINT ( 'NONE',  ( 153.5378496954705270, 279.2422976570009610, 3.847913014617606375 ) ) ;
#75795=CARTESIAN_POINT ( 'NONE',  ( 21.69106252476256458, 174.1423013555409796, -4.594050593750043987 ) ) ;
#75796=CARTESIAN_POINT ( 'NONE',  ( 108.2389556718223673, 242.4869531367911009, 4.594050593750046652 ) ) ;
#75800=CARTESIAN_POINT ( 'NONE',  ( 206.5615526473034151, 272.3516689047157229, -7.512841850187674808 ) ) ;
#75802=CARTESIAN_POINT ( 'NONE',  ( 175.5675097156527613, 281.7075564011171309, -14.18956677121689403 ) ) ;
#75804=CARTESIAN_POINT ( 'NONE',  ( 155.0303156110108489, 262.1266119787277944, 17.11986653161320859 ) ) ;
#75805=CARTESIAN_POINT ( 'NONE',  ( 184.0348397922024901, 275.0104453757304555, 16.36204107713549050 ) ) ;
#75807=EDGE_CURVE ( 'NONE', #49470, #57417, #54005, .T. ) ;
#75809=CARTESIAN_POINT ( 'NONE',  ( 195.5982822146934836, 266.5867291171349507, 7.946036122846243721 ) ) ;
#75811=CARTESIAN_POINT ( 'NONE',  ( 162.3854161007234609, 251.6213552765262875, -12.80540064494198838 ) ) ;
#75815=CARTESIAN_POINT ( 'NONE',  ( 181.6067143826203676, 267.9940397974941675, 15.00604427482618242 ) ) ;
#75816=CARTESIAN_POINT ( 'NONE',  ( 101.2839494695023603, 229.2833772461660544, -9.188101187500095079 ) ) ;
#75818=CARTESIAN_POINT ( 'NONE',  ( 162.5189332652596761, 275.0194079713638189, -15.39703335036588250 ) ) ;
#75819=CARTESIAN_POINT ( 'NONE',  ( 162.8751945631634612, 272.8900720096677333, -16.40198242748087054 ) ) ;
#75822=CARTESIAN_POINT ( 'NONE',  ( 201.5036534377215958, 270.3153034880852488, -10.25451236307256409 ) ) ;
#75823=CARTESIAN_POINT ( 'NONE',  ( 198.6894790592683080, 286.5067226703918095, -17.06774375037124614 ) ) ;
#75824=CARTESIAN_POINT ( 'NONE',  ( 173.5155000508206911, 267.4844645354696127, -16.73009763236219172 ) ) ;
#75831=B_SPLINE_CURVE_WITH_KNOTS ( 'NONE', 3,
 ( #39518, #54219, #61828, #25340, #15227, #32938, #16744, #93277, #2056, #8647, #63345, #17237, #24838, #93790, #70442, #23833, #94781, #85708, #47632, #39025, #38534, #77037, #54727, #7643, #78059, #78564, #46637, #30942, #9149, #24350, #47135, #55223 ),
 .UNSPECIFIED., .F., .F.,
 ( 4, 2, 2, 2, 2, 2, 2, 2, 2, 2, 2, 2, 2, 2, 2, 4 ),
 ( 0.001523115973120424535, 0.002198702639335023152, 0.002874289305549621986, 0.004225462637978878201, 0.004901049304193506526, 0.005238842637300820254, 0.005407739303854516150, 0.005449963470492883745, 0.005492187637131250473, 0.005534411803769618068, 0.005576635970407985664, 0.005745532636961396197, 0.005914429303514805863, 0.006252222636621627798, 0.006590015969728450600, 0.006927809302835272534 ),
 .UNSPECIFIED. ) ;
#75832=FACE_OUTER_BOUND ( 'NONE', #39045, .T. ) ;
#75833=CARTESIAN_POINT ( 'NONE',  ( 147.4824818982269790, 275.1998434563504929, -4.972419998968698351 ) ) ;
#75834=CARTESIAN_POINT ( 'NONE',  ( 196.5806080813426888, 290.1593943507663766, -16.31912166233602690 ) ) ;
#75835=ADVANCED_FACE ( 'NONE', ( #37136 ), #43736, .T. ) ;
#75836=VERTEX_POINT ( 'NONE', #81304 ) ;
#75838=CARTESIAN_POINT ( 'NONE',  ( 159.6898930778639283, 254.0559870643349143, 16.90891900388599822 ) ) ;
#75839=CARTESIAN_POINT ( 'NONE',  ( 153.6675463778983612, 266.9416252070789142, 16.49262662605783092 ) ) ;
#75841=CARTESIAN_POINT ( 'NONE',  ( 140.8234218128096131, 252.1115022471902591, 10.00000000000009592 ) ) ;
#75847=CARTESIAN_POINT ( 'NONE',  ( 202.9093905060991005, 279.1976216410395182, 16.97070083370504179 ) ) ;
#75849=CARTESIAN_POINT ( 'NONE',  ( 182.6217066138594305, 291.1375281399239157, -10.79417329231678302 ) ) ;
#75852=AXIS2_PLACEMENT_3D ( 'NONE', #52621, #37913, #83579 ) ;
#75853=CARTESIAN_POINT ( 'NONE',  ( 44.69460199273692069, 196.6115022471902591, 10.00000000000009592 ) ) ;
#75855=CARTESIAN_POINT ( 'NONE',  ( 158.6991807772081415, 256.2500756557278692, 16.19856017798593939 ) ) ;
#75856=CARTESIAN_POINT ( 'NONE',  ( 192.8453312832112090, 280.1102836227724424, -16.77340966031070835 ) ) ;
#75857=CARTESIAN_POINT ( 'NONE',  ( 153.4976680152657877, 264.7812354846562926, -17.98840356897177273 ) ) ;
#75858=B_SPLINE_CURVE_WITH_KNOTS ( 'NONE', 3,
 ( #98509, #23456, #21487, #52871 ),
 .UNSPECIFIED., .F., .F.,
 ( 4, 4 ),
 ( 0.04629403814142867696, 0.04887066958154943908 ),
 .UNSPECIFIED. ) ;
#75859=CARTESIAN_POINT ( 'NONE',  ( 152.6740002182599767, 266.2078699576288159, -17.16212636348624088 ) ) ;
#75861=EDGE_CURVE ( 'NONE', #56977, #88596, #16450, .T. ) ;
#75864=EDGE_CURVE ( 'NONE', #44309, #68820, #67593, .T. ) ;
#75868=ORIENTED_EDGE ( 'NONE', *, *, #78116, .F. ) ;
#75871=VECTOR ( 'NONE', #41179, 1000.000000000000000 ) ;
#75874=CARTESIAN_POINT ( 'NONE',  ( 147.7112127936102866, 274.8036699242858276, -9.124700685424272706 ) ) ;
#75876=CARTESIAN_POINT ( 'NONE',  ( 201.0150177425703077, 274.8767133061161303, -13.89391286736939612 ) ) ;
#75879=CARTESIAN_POINT ( 'NONE',  ( 187.7710022618638277, 277.0665775429750397, -17.72351784843695555 ) ) ;
#75881=CARTESIAN_POINT ( 'NONE',  ( 178.0655552872740088, 255.4621687460560508, 4.946877401895048543 ) ) ;
#75882=CARTESIAN_POINT ( 'NONE',  ( 111.3514947884964670, 235.0958772461660544, -9.188101187500095079 ) ) ;
#75883=ORIENTED_EDGE ( 'NONE', *, *, #55817, .T. ) ;
#75884=CARTESIAN_POINT ( 'NONE',  ( 183.4307448953204300, 260.0939146214054745, -9.483231343634749066 ) ) ;
#75886=CARTESIAN_POINT ( 'NONE',  ( 191.7218012215406304, 275.0451209121254124, 16.76516018751371107 ) ) ;
#75888=AXIS2_PLACEMENT_3D ( 'NONE', #97885, #58841, #59337 ) ;
#75890=CARTESIAN_POINT ( 'NONE',  ( 180.1168005803277481, 295.2192856762299016, -2.191971455912026467 ) ) ;
#75891=CARTESIAN_POINT ( 'NONE',  ( 157.2744851780909414, 258.2395962677452985, 18.17792129701959070 ) ) ;
#75892=CARTESIAN_POINT ( 'NONE',  ( 206.0930919633010774, 273.6832889610345774, -9.866500005465628220 ) ) ;
#75893=B_SPLINE_CURVE_WITH_KNOTS ( 'NONE', 3,
 ( #15627, #55126, #46526, #38932 ),
 .UNSPECIFIED., .F., .F.,
 ( 4, 4 ),
 ( 0.004991743399790857412, 0.009976538136425933123 ),
 .UNSPECIFIED. ) ;
#75894=CARTESIAN_POINT ( 'NONE',  ( 170.8463542321686077, 287.4393069310528972, -8.645854640182026429 ) ) ;
#75896=CARTESIAN_POINT ( 'NONE',  ( 195.0933678165431502, 292.7353700524613487, 15.12141487717723365 ) ) ;
#75900=CARTESIAN_POINT ( 'NONE',  ( 23.45662567177863167, 195.8967562850347122, -4.648177544792955347E-16 ) ) ;
#75901=CARTESIAN_POINT ( 'NONE',  ( 195.7200744708509887, 265.3358093963507827, 4.285174003455722413 ) ) ;
#75902=CARTESIAN_POINT ( 'NONE',  ( -11.77978294824862893, 175.5530062829863311, 1.347971487989956912E-14 ) ) ;
#75904=DIRECTION ( 'NONE',  ( 0.4999999999999992784, -0.8660254037844390407, 0.000000000000000000 ) ) ;
#75906=CARTESIAN_POINT ( 'NONE',  ( 201.3053499423511425, 281.9759013948520874, -16.75960365258566398 ) ) ;
#75908=CARTESIAN_POINT ( 'NONE',  ( 190.5653282632609091, 300.5781646174276602, -5.775635208185608604 ) ) ;
#75910=CARTESIAN_POINT ( 'NONE',  ( 190.5837197087969912, 264.0079844486248817, -9.604741279133001797 ) ) ;
#75911=CARTESIAN_POINT ( 'NONE',  ( 171.4692916405222718, 250.4214803585759626, -0.2564616657247425491 ) ) ;
#75912=CARTESIAN_POINT ( 'NONE',  ( 192.7848161478432303, 271.7584063516355855, -14.73987874102306961 ) ) ;
#75916=CARTESIAN_POINT ( 'NONE',  ( 155.5660013421004919, 261.1987770755905558, 17.28709111629370199 ) ) ;
#75918=CARTESIAN_POINT ( 'NONE',  ( 112.9278751967105450, 247.5530062829863311, -4.648177544792955347E-16 ) ) ;
#75920=CARTESIAN_POINT ( 'NONE',  ( 85.20852645963621796, 213.8768266524159856, -9.188101187500091527 ) ) ;
#75921=CARTESIAN_POINT ( 'NONE',  ( 159.2122473525774069, 254.8832937285494609, -16.22689353966294590 ) ) ;
#75922=CARTESIAN_POINT ( 'NONE',  ( 197.5333837132704673, 287.4243462569709209, 17.22026250574119288 ) ) ;
#75924=B_SPLINE_CURVE_WITH_KNOTS ( 'NONE', 3,
 ( #75784, #99078, #60538, #69145, #99570, #22558, #21570, #68649, #44352, #60042 ),
 .UNSPECIFIED., .F., .F.,
 ( 4, 2, 2, 2, 4 ),
 ( 0.001272943234969431620, 0.001710735386977082009, 0.002148527538984732616, 0.002586319690992383222, 0.003024111843000033394 ),
 .UNSPECIFIED. ) ;
#75927=CARTESIAN_POINT ( 'NONE',  ( 196.1749740761792111, 288.8619730569873809, -17.33086882175758703 ) ) ;
#75928=CARTESIAN_POINT ( 'NONE',  ( 207.1432938686257046, 271.8642859028066141, -6.405155839440290322 ) ) ;
#75932=CARTESIAN_POINT ( 'NONE',  ( 120.6082041558992586, 228.8932355074535394, -2.679491924311248496 ) ) ;
#75935=DIRECTION ( 'NONE',  ( -0.8660254037844387076, -0.4999999999999998890, -0.000000000000000000 ) ) ;
#75940=( BOUNDED_CURVE ( )  B_SPLINE_CURVE ( 1, ( #60527, #1250 ),
 .UNSPECIFIED., .F., .T. ) 
 B_SPLINE_CURVE_WITH_KNOTS ( ( 2, 2 ),
 ( 0.000000000000000000, 0.0009374999959032195417 ),
 .UNSPECIFIED. ) 
 CURVE ( )  GEOMETRIC_REPRESENTATION_ITEM ( )  RATIONAL_B_SPLINE_CURVE ( ( 0.9368410486966849415, 0.9368410486966849415 ) ) 
 REPRESENTATION_ITEM ( '' )  );
#75941=CARTESIAN_POINT ( 'NONE',  ( 28.53781555160951555, 187.2833772461660544, -9.188101187500095079 ) ) ;
#75942=CARTESIAN_POINT ( 'NONE',  ( 166.0506673010352472, 274.1027903476490337, -16.62009509085023851 ) ) ;
#75943=CARTESIAN_POINT ( 'NONE',  ( 199.5396699312275928, 277.5950600280153822, 15.20170681613290142 ) ) ;
#75946=CARTESIAN_POINT ( 'NONE',  ( 43.80151329331025067, 196.0958772461660544, -9.188101187500095079 ) ) ;
#75949=FACE_OUTER_BOUND ( 'NONE', #43462, .T. ) ;
#75950=CARTESIAN_POINT ( 'NONE',  ( 149.6564118588553924, 271.4344863124460971, -11.76165597393390172 ) ) ;
#75952=CARTESIAN_POINT ( 'NONE',  ( 204.6475128369918082, 276.1871054541632020, -13.72068618491070779 ) ) ;
#75953=CARTESIAN_POINT ( 'NONE',  ( 202.8126086360731222, 269.9569268784645146, -6.432707174703383046 ) ) ;
#75955=CARTESIAN_POINT ( 'NONE',  ( 178.1538850474519506, 275.9401529576537087, 16.36541506392882539 ) ) ;
#75957=CARTESIAN_POINT ( 'NONE',  ( 153.5689166488172646, 264.6578292313752740, 18.05965550300112099 ) ) ;
#75958=( BOUNDED_CURVE ( )  B_SPLINE_CURVE ( 2, ( #28301, #22583, #90154, #82568, #13131, #89666, #12633, #11638, #42989 ),
 .UNSPECIFIED., .F., .T. ) 
 B_SPLINE_CURVE_WITH_KNOTS ( ( 3, 2, 2, 2, 3 ),
 ( 0.3669354838709677491, 0.3682795698924731242, 0.3709677419354838745, 0.3736559139784946248, 0.3750000000000000000 ),
 .UNSPECIFIED. ) 
 CURVE ( )  GEOMETRIC_REPRESENTATION_ITEM ( )  RATIONAL_B_SPLINE_CURVE ( ( 0.9330127018922194093, 0.9330127018922194093, 1.000000000000000000, 0.8660254037844387076, 1.000000000000000000, 0.8660254037844387076, 1.000000000000000000, 0.9330127018922194093, 0.9330127018922194093 ) ) 
 REPRESENTATION_ITEM ( '' )  );
#75959=CARTESIAN_POINT ( 'NONE',  ( 153.0305350670531936, 277.3750776671890890, 8.290292975357761662 ) ) ;
#75961=CARTESIAN_POINT ( 'NONE',  ( 104.0173421519710217, 220.8615022471902023, 5.000000000000051514 ) ) ;
#75962=CARTESIAN_POINT ( 'NONE',  ( 161.4469036912142599, 251.0127554125742222, 12.93933463576739307 ) ) ;
#75964=CARTESIAN_POINT ( 'NONE',  ( 164.6958324620632368, 269.3431737359563272, -16.31609373033956345 ) ) ;
#75965=ORIENTED_EDGE ( 'NONE', *, *, #46768, .F. ) ;
#75966=CARTESIAN_POINT ( 'NONE',  ( 56.79189435007682363, 203.5958772461660544, -9.188101187500095079 ) ) ;
#75967=VERTEX_POINT ( 'NONE', #8738 ) ;
#75968=DIRECTION ( 'NONE',  ( 0.8660254037844395958, 0.4999999999999985567, 0.000000000000000000 ) ) ;
#75971=ORIENTED_EDGE ( 'NONE', *, *, #11169, .T. ) ;
#75972=CARTESIAN_POINT ( 'NONE',  ( 198.2505066714982149, 285.2670451491296149, 0.000000000000000000 ) ) ;
#75975=B_SPLINE_CURVE_WITH_KNOTS ( 'NONE', 3,
 ( #76547, #22831, #99849, #61322 ),
 .UNSPECIFIED., .F., .F.,
 ( 4, 4 ),
 ( 0.01071166683732669572, 0.01632733781203283066 ),
 .UNSPECIFIED. ) ;
#75977=CARTESIAN_POINT ( 'NONE',  ( 176.3483583558151508, 274.3708778633847487, -17.64881272765552822 ) ) ;
#75979=CARTESIAN_POINT ( 'NONE',  ( 156.6938127249734976, 259.2453504591003934, 17.44495368413245728 ) ) ;
#75986=CARTESIAN_POINT ( 'NONE',  ( 135.6272693901030095, 249.1115022471902591, 10.00000000000009592 ) ) ;
#75987=CARTESIAN_POINT ( 'NONE',  ( 159.2713554375903300, 254.7809155221686410, -15.70062444474382168 ) ) ;
#75988=ORIENTED_EDGE ( 'NONE', *, *, #1627, .F. ) ;
#75989=CARTESIAN_POINT ( 'NONE',  ( 159.2990852460085023, 282.6395706699606762, -3.314431380743207978 ) ) ;
#75992=CARTESIAN_POINT ( 'NONE',  ( 204.6780326111993986, 276.1342436545999703, 14.85609018352459287 ) ) ;
#75995=CARTESIAN_POINT ( 'NONE',  ( 204.1656981441084611, 271.5570760979641136, 9.881240885324146461 ) ) ;
#75996=CARTESIAN_POINT ( 'NONE',  ( 134.0307085979839883, 242.0643266524160140, 9.188101187500095079 ) ) ;
#75998=CARTESIAN_POINT ( 'NONE',  ( 177.5865089022509551, 268.7852845103913069, 17.37969943402860906 ) ) ;
#75999=CARTESIAN_POINT ( 'NONE',  ( 182.2689230490940986, 259.9811410596485075, 9.155893851718131415 ) ) ;
#76000=CARTESIAN_POINT ( 'NONE',  ( 68.83479979963041728, 219.7369531367911293, -4.594050593750048428 ) ) ;
#76002=CARTESIAN_POINT ( 'NONE',  ( 170.1373231016024477, 264.2063840763735243, 16.55828558264352424 ) ) ;
#76007=ORIENTED_EDGE ( 'NONE', *, *, #52189, .F. ) ;
#76010=CARTESIAN_POINT ( 'NONE',  ( 197.9367325884184083, 286.8643941967906130, 16.93519219127947295 ) ) ;
#76013=CARTESIAN_POINT ( 'NONE',  ( 194.4889937320412230, 293.7821766735966662, 14.99892588346621380 ) ) ;
#76022=CARTESIAN_POINT ( 'NONE',  ( 164.9356397357043704, 244.9700873293209042, 2.799217332519396972 ) ) ;
#76025=CARTESIAN_POINT ( 'NONE',  ( 195.0437424211503412, 279.4124847088495471, 16.44665416634688171 ) ) ;
#76026=CARTESIAN_POINT ( 'NONE',  ( 162.9364957791611630, 261.5460700938506875, 17.26453991925339082 ) ) ;
#76027=CARTESIAN_POINT ( 'NONE',  ( 144.4230134433972239, 248.0643266524160140, 9.188101187500095079 ) ) ;
#76035=ORIENTED_EDGE ( 'NONE', *, *, #37222, .F. ) ;
#76036=CARTESIAN_POINT ( 'NONE',  ( 199.1379133944519424, 266.8226340275038524, 4.550351456204111855 ) ) ;
#76039=CARTESIAN_POINT ( 'NONE',  ( 186.2798660816079632, 264.0713031700501006, -12.82791401631097550 ) ) ;
#76040=CARTESIAN_POINT ( 'NONE',  ( 202.6574465548223145, 267.4804609884895967, 0.8726363535044180386 ) ) ;
#76043=CARTESIAN_POINT ( 'NONE',  ( 183.3250138703919561, 280.8103892703075530, 16.49174253902363674 ) ) ;
#76044=CARTESIAN_POINT ( 'NONE',  ( 164.4781197247689306, 245.7625352337404649, -1.511762618280499515 ) ) ;
#76045=CARTESIAN_POINT ( 'NONE',  ( 193.0673848936551735, 268.2732046201192020, 12.66768335688180436 ) ) ;
#76049=CARTESIAN_POINT ( 'NONE',  ( 204.7200661083698776, 274.0614395018808978, 12.25436898028725530 ) ) ;
#76050=CARTESIAN_POINT ( 'NONE',  ( 151.3511865740561007, 278.6745403919405248, -1.693856907688049862 ) ) ;
#76051=CARTESIAN_POINT ( 'NONE',  ( 159.9014600375868440, 253.6895423408921886, 15.57825579621527368 ) ) ;
#76052=EDGE_CURVE ( 'NONE', #45778, #45450, #7715, .T. ) ;
#76054=CARTESIAN_POINT ( 'NONE',  ( -15.46727382606978374, 168.0024278399160664, -9.188101187500093303 ) ) ;
#76059=CARTESIAN_POINT ( 'NONE',  ( 178.2112680352368272, 255.9238100178365869, 8.848909479073256534 ) ) ;
#76061=CARTESIAN_POINT ( 'NONE',  ( 202.5775937153526627, 273.9552816370790538, -13.18159814775432181 ) ) ;
#76062=CARTESIAN_POINT ( 'NONE',  ( 151.1811967613751335, 268.7934813906678642, -15.79361349403328418 ) ) ;
#76063=CARTESIAN_POINT ( 'NONE',  ( 2.394500126984267840, 178.3149278399160949, -9.188101187500095079 ) ) ;
#76066=B_SPLINE_CURVE_WITH_KNOTS ( 'NONE', 3,
 ( #96773, #14126, #59711, #83059 ),
 .UNSPECIFIED., .F., .F.,
 ( 4, 4 ),
 ( 0.009172812625567213288, 0.01512212324709697256 ),
 .UNSPECIFIED. ) ;
#76067=CARTESIAN_POINT ( 'NONE',  ( 184.7894305693181138, 292.1317680087225881, 12.52679022050396895 ) ) ;
#76070=CARTESIAN_POINT ( 'NONE',  ( 149.9444379511524517, 276.8732903533755803, 4.578473933676738383 ) ) ;
#76071=CARTESIAN_POINT ( 'NONE',  ( 178.7534805286849178, 255.1052391757385749, -3.938431664117528541 ) ) ;
#76072=CARTESIAN_POINT ( 'NONE',  ( 151.0171360864231644, 269.0776428152087760, 14.21401713093731267 ) ) ;
#76074=CARTESIAN_POINT ( 'NONE',  ( 182.3197145248164190, 295.2660807675984529, 1.016087631068208097 ) ) ;
#76075=CARTESIAN_POINT ( 'NONE',  ( 49.89075441544350298, 209.6115022471903160, -5.000000000000047962 ) ) ;
#76078=CARTESIAN_POINT ( 'NONE',  ( 189.9925954911225290, 301.5701668779311717, 0.1154287172046158938 ) ) ;
#76079=CARTESIAN_POINT ( 'NONE',  ( 22.85469738715664434, 177.8768266524160140, -9.188101187500091527 ) ) ;
#76083=CARTESIAN_POINT ( 'NONE',  ( 118.1240276194171770, 250.5530062829863311, -4.648177544792955347E-16 ) ) ;
#76084=DIRECTION ( 'NONE',  ( 0.4999999999999998890, -0.8660254037844385966, 0.000000000000000000 ) ) ;
#76085=CARTESIAN_POINT ( 'NONE',  ( 155.0898745997320134, 262.0234527842152374, 17.05457557403769542 ) ) ;
#76086=CARTESIAN_POINT ( 'NONE',  ( 186.5969764575044394, 267.2136708933791169, 13.23504358057708430 ) ) ;
#76087=CARTESIAN_POINT ( 'NONE',  ( 120.0388121219830708, 240.1115022471902307, 10.00000000000009592 ) ) ;
#76088=CARTESIAN_POINT ( 'NONE',  ( 164.0149191615929851, 281.5227187913443458, 8.861377439193347527 ) ) ;
#76093=CARTESIAN_POINT ( 'NONE',  ( 194.5047661587782386, 293.7548580291293092, 14.86680123054176583 ) ) ;
#76095=CARTESIAN_POINT ( 'NONE',  ( 182.4138193503314653, 289.4190845564540950, 12.30891238242875829 ) ) ;
#76096=CARTESIAN_POINT ( 'NONE',  ( 161.0972336787313282, 260.9823377472601464, -17.65804059120327452 ) ) ;
#76103=CARTESIAN_POINT ( 'NONE',  ( 203.5258219653775313, 278.1299310341851765, -16.21052911601769608 ) ) ;
#76109=CARTESIAN_POINT ( 'NONE',  ( 151.3883635558152321, 268.4346579770563608, 15.44343517165679103 ) ) ;
#76112=CARTESIAN_POINT ( 'NONE',  ( 170.3127733705114224, 263.9010670580030364, 17.23448983536806622 ) ) ;
#76114=ORIENTED_EDGE ( 'NONE', *, *, #76769, .T. ) ;
#76118=CARTESIAN_POINT ( 'NONE',  ( 206.5571822944673670, 272.8794609281530938, 10.95833005210827515 ) ) ;
#76121=CARTESIAN_POINT ( 'NONE',  ( 190.1519139143167081, 301.2942192743771557, 4.481136594690903863 ) ) ;
#76126=CARTESIAN_POINT ( 'NONE',  ( 170.5373622343556690, 269.7751423367952270, 17.81562764448176850 ) ) ;
#76130=CARTESIAN_POINT ( 'NONE',  ( 156.3761965727711356, 267.2017284797204866, -16.34692893795439161 ) ) ;
#76132=CARTESIAN_POINT ( 'NONE',  ( 162.7435819479956933, 250.7668427907593411, -13.06080741167749082 ) ) ;
#76133=CARTESIAN_POINT ( 'NONE',  ( 190.4841013044967042, 300.7188538369516095, 4.682298117523464143 ) ) ;
#76134=DIRECTION ( 'NONE',  ( -0.8660254037844387076, -0.4999999999999998890, -0.000000000000000000 ) ) ;
#76136=CARTESIAN_POINT ( 'NONE',  ( 146.5665812168672915, 276.7862299711523519, -0.4280630669697406687 ) ) ;
#76137=CARTESIAN_POINT ( 'NONE',  ( 191.0481192767711036, 299.7419460525905492, -9.103377665618040737 ) ) ;
#76138=CARTESIAN_POINT ( 'NONE',  ( 163.9896819828944672, 256.9390232144978086, 16.08371068233360290 ) ) ;
#76140=CARTESIAN_POINT ( 'NONE',  ( 197.0226655822963551, 289.3937282992477549, -17.28982543158101493 ) ) ;
#76143=CARTESIAN_POINT ( 'NONE',  ( 171.0488218253813386, 288.2608493535105367, 4.157149925330108964 ) ) ;
#76145=CARTESIAN_POINT ( 'NONE',  ( 98.17141035282828909, 236.6744531367911293, 4.594050593750047540 ) ) ;
#76147=CARTESIAN_POINT ( 'NONE',  ( 190.7616931697327516, 300.2380506225948125, -4.491414918766103881 ) ) ;
#76151=CARTESIAN_POINT ( 'NONE',  ( 191.2278159864466431, 297.4307022214792937, -10.96893880474589267 ) ) ;
#76154=CARTESIAN_POINT ( 'NONE',  ( 165.5142259937072993, 283.5901604647961562, -8.273349223471056391 ) ) ;
#76156=CARTESIAN_POINT ( 'NONE',  ( 208.3863431123642727, 269.7112614563416173, -1.693909372230378851 ) ) ;
#76157=CARTESIAN_POINT ( 'NONE',  ( 160.0081047537594543, 253.5048282741223602, -16.11956848123596941 ) ) ;
#76159=CARTESIAN_POINT ( 'NONE',  ( 43.23318412030279489, 185.7677522451417929, -5.000000000000041744 ) ) ;
#76160=CARTESIAN_POINT ( 'NONE',  ( 111.3514947884964670, 235.0958772461660544, -9.188101187500095079 ) ) ;
#76163=CARTESIAN_POINT ( 'NONE',  ( 189.4827547918471851, 297.7068139993613727, 9.374012235039304031 ) ) ;
#76164=CARTESIAN_POINT ( 'NONE',  ( 173.5466779927756704, 252.2311758790288252, -3.912256498803678095 ) ) ;
#76165=CARTESIAN_POINT ( 'NONE',  ( 28.37526224051743284, 193.3149278399160949, -9.188101187500095079 ) ) ;
#76166=CARTESIAN_POINT ( 'NONE',  ( 147.6787290359179110, 275.8338687843527168, -2.569013399972302381 ) ) ;
#76169=CARTESIAN_POINT ( 'NONE',  ( 178.3855741922590994, 265.9601407903336394, 15.32162025640515068 ) ) ;
#76172=CARTESIAN_POINT ( 'NONE',  ( 147.2443490232117256, 275.6123016948292275, 5.226063659459642352 ) ) ;
#76173=DIRECTION ( 'NONE',  ( -0.8660254037844357100, -0.5000000000000049960, -0.000000000000000000 ) ) ;
#76176=CARTESIAN_POINT ( 'NONE',  ( 115.5463053363034476, 227.5177522451418213, 5.000000000000051514 ) ) ;
#76177=EDGE_CURVE ( 'NONE', #43169, #92570, #39092, .T. ) ;
#76181=CARTESIAN_POINT ( 'NONE',  ( 158.7695631051096257, 282.4121657607714155, -1.649238854537537158 ) ) ;
#76182=LINE ( 'NONE', #30046, #62530 ) ;
#76183=CARTESIAN_POINT ( 'NONE',  ( 10.89220085373657376, 189.3464784336661353, 1.353441290958777327E-15 ) ) ;
#76185=CARTESIAN_POINT ( 'NONE',  ( 196.2123514992661057, 273.6774763844528024, 14.95493983070488930 ) ) ;
#76188=CARTESIAN_POINT ( 'NONE',  ( 195.1313828796571386, 275.4209514540651185, -15.57016190239770914 ) ) ;
#76189=CARTESIAN_POINT ( 'NONE',  ( 74.76226857436894591, 201.7202760586659167, -5.415160957724236172E-17 ) ) ;
#76190=CARTESIAN_POINT ( 'NONE',  ( 207.8725590214046406, 270.6011616060040410, 1.988011721677743093 ) ) ;
#76192=CARTESIAN_POINT ( 'NONE',  ( 54.13067045125697518, 195.3927522451418213, 10.00000000000009948 ) ) ;
#76195=CARTESIAN_POINT ( 'NONE',  ( 13.51768745649715697, 168.6115022471901739, -5.000000000000041744 ) ) ;
#76196=CARTESIAN_POINT ( 'NONE',  ( 163.7038023771459052, 247.1036922210055025, -6.448491958542482472 ) ) ;
#76197=CARTESIAN_POINT ( 'NONE',  ( 137.1425535231280151, 259.1744531367911009, 4.594050593750047540 ) ) ;
#76199=CARTESIAN_POINT ( 'NONE',  ( 207.5386549290987546, 271.1795004587326048, -7.943787175633387321 ) ) ;
#76205=VERTEX_POINT ( 'NONE', #29310 ) ;
#76206=CARTESIAN_POINT ( 'NONE',  ( 64.47116044126103418, 196.4824982072973683, 3.021315404115420679E-15 ) ) ;
#76210=CARTESIAN_POINT ( 'NONE',  ( 194.1563733927635838, 270.7326105280735078, -14.10882362769777743 ) ) ;
#76211=ORIENTED_EDGE ( 'NONE', *, *, #18130, .F. ) ;
#76212=CARTESIAN_POINT ( 'NONE',  ( 160.0940723892081223, 253.3559279617186917, 16.15485901636618138 ) ) ;
#76214=FACE_OUTER_BOUND ( 'NONE', #3378, .T. ) ;
#76215=CARTESIAN_POINT ( 'NONE',  ( 206.1823507212516802, 271.5286882572439140, -8.119960357998227352 ) ) ;
#76216=CARTESIAN_POINT ( 'NONE',  ( 89.54518929453067244, 234.0530062829863027, -4.648177544792955347E-16 ) ) ;
#76217=CARTESIAN_POINT ( 'NONE',  ( 208.3863431123642727, 269.7112614563416173, -1.693909372230378851 ) ) ;
#76219=CARTESIAN_POINT ( 'NONE',  ( 200.8665851640556070, 282.7358642834317948, -16.69422397739980823 ) ) ;
#76220=VERTEX_POINT ( 'NONE', #90658 ) ;
#76221=CARTESIAN_POINT ( 'NONE',  ( 192.0331336666972391, 281.5685065300137353, 16.72509162371795099 ) ) ;
#76225=CARTESIAN_POINT ( 'NONE',  ( 149.6877696051026305, 271.3801731027346591, 11.89134584187677390 ) ) ;
#76227=CARTESIAN_POINT ( 'NONE',  ( 189.0590152237434154, 297.0845166239263335, 8.082612471021599632 ) ) ;
#76229=VERTEX_POINT ( 'NONE', #52094 ) ;
#76230=CARTESIAN_POINT ( 'NONE',  ( 146.6363376198206652, 276.6654083370839885, -0.5879280619134327202 ) ) ;
#76232=CARTESIAN_POINT ( 'NONE',  ( 204.6427704787179493, 276.1953194596412118, 13.28850621060895953 ) ) ;
#76233=EDGE_CURVE ( 'NONE', #77324, #74259, #78909, .T. ) ;
#76235=ORIENTED_EDGE ( 'NONE', *, *, #58254, .F. ) ;
#76236=CARTESIAN_POINT ( 'NONE',  ( 107.4275774994220001, 223.6423013555409796, -4.594050593750043987 ) ) ;
#76237=CARTESIAN_POINT ( 'NONE',  ( 155.2031798843469232, 261.8272022744961873, 18.50448283576785968 ) ) ;
#76239=CARTESIAN_POINT ( 'NONE',  ( 178.4381536407659894, 269.1936824936634594, -17.11615640515828574 ) ) ;
#76244=FACE_OUTER_BOUND ( 'NONE', #84852, .T. ) ;
#76246=EDGE_CURVE ( 'NONE', #51127, #33408, #16149, .T. ) ;
#76249=CARTESIAN_POINT ( 'NONE',  ( 163.7423057141168385, 247.0370024851108610, -6.909410042141566066 ) ) ;
#76250=CARTESIAN_POINT ( 'NONE',  ( 167.9307537431739661, 281.1416098987750729, 11.64201043039908434 ) ) ;
#76255=CARTESIAN_POINT ( 'NONE',  ( 196.6195079739135849, 274.6088269242578690, -15.71717729878580094 ) ) ;
#76257=CARTESIAN_POINT ( 'NONE',  ( 191.6779092374860625, 276.1752509429691145, -17.22939886907964890 ) ) ;
#76259=CARTESIAN_POINT ( 'NONE',  ( 180.7701619213715958, 282.8660957359396093, 16.53338994692317954 ) ) ;
#76261=CARTESIAN_POINT ( 'NONE',  ( 163.1691520398773321, 248.0297337694385931, 11.21816141384514331 ) ) ;
#76262=CARTESIAN_POINT ( 'NONE',  ( 184.9627711092587674, 258.1544921998163318, 2.978903034762152124 ) ) ;
#76263=DIRECTION ( 'NONE',  ( 0.4999999999999992784, -0.8660254037844390407, 0.000000000000000000 ) ) ;
#76264=CARTESIAN_POINT ( 'NONE',  ( 147.1270795744234476, 264.4111747905818675, -1.822351119449947324E-15 ) ) ;
#76265=CARTESIAN_POINT ( 'NONE',  ( 171.4292241046584877, 255.5488744981172431, 11.14177367849849887 ) ) ;
#76266=CARTESIAN_POINT ( 'NONE',  ( 159.9665222620925817, 282.2299347244568253, 2.085082827276235395 ) ) ;
#76268=CARTESIAN_POINT ( 'NONE',  ( 182.6715392610496735, 271.9296818901224242, -16.02872276298343834 ) ) ;
#76270=CARTESIAN_POINT ( 'NONE',  ( 160.1969820541083607, 255.1776831935258372, -16.37528374203482073 ) ) ;
#76271=CARTESIAN_POINT ( 'NONE',  ( 10.68506269473765258, 163.6427522451417644, 1.119607411625061291E-15 ) ) ;
#76272=CARTESIAN_POINT ( 'NONE',  ( 193.6071458082581955, 267.8835467034379008, -10.90750982005068259 ) ) ;
#76273=CARTESIAN_POINT ( 'NONE',  ( 201.4660993003597582, 266.8443734887555365, -2.250696924963314416 ) ) ;
#76274=CARTESIAN_POINT ( 'NONE',  ( 203.6076779758675741, 277.9881522651116370, -14.46320369641031256 ) ) ;
#76276=CARTESIAN_POINT ( 'NONE',  ( 161.5029716424245407, 251.3413373469583973, -13.00020995489466458 ) ) ;
#76277=CARTESIAN_POINT ( 'NONE',  ( -13.19395714113563045, 169.3149278399160949, -9.188101187500095079 ) ) ;
#76278=CARTESIAN_POINT ( 'NONE',  ( 106.4790390313002888, 243.8297689869268936, -2.679491924311252493 ) ) ;
#76279=CARTESIAN_POINT ( 'NONE',  ( 185.5618062172021894, 295.3137494393371298, 8.271460040209413833 ) ) ;
#76285=B_SPLINE_CURVE_WITH_KNOTS ( 'NONE', 3,
 ( #15965, #77791, #78283, #39242 ),
 .UNSPECIFIED., .F., .F.,
 ( 4, 4 ),
 ( 0.02265161601259375185, 0.02890507703157969843 ),
 .UNSPECIFIED. ) ;
#76288=CARTESIAN_POINT ( 'NONE',  ( 162.5387916653087927, 249.1215499652694234, -10.44916066063070126 ) ) ;
#76290=CARTESIAN_POINT ( 'NONE',  ( 150.1473662157767990, 276.5461327245939742, 3.629510331267637557 ) ) ;
#76291=CARTESIAN_POINT ( 'NONE',  ( 17.19803509898326510, 189.9244531367911293, -4.594050593750046652 ) ) ;
#76292=CARTESIAN_POINT ( 'NONE',  ( 127.8874276638293850, 235.4548013555409796, -4.594050593750042211 ) ) ;
#76293=CARTESIAN_POINT ( 'NONE',  ( 181.8839543305726068, 294.0754964817877521, -6.330318412758383140 ) ) ;
#76294=CARTESIAN_POINT ( 'NONE',  ( 172.0728039219370658, 285.9831811572526021, 11.38650458882361427 ) ) ;
#76298=CARTESIAN_POINT ( 'NONE',  ( 178.1976719649161964, 283.8584802497103396, -15.12167059147577675 ) ) ;
#76299=CARTESIAN_POINT ( 'NONE',  ( 61.41971759977592171, 216.2677522451419065, -5.000000000000047962 ) ) ;
#76301=CARTESIAN_POINT ( 'NONE',  ( 207.8792014703394671, 270.5896565469619759, -5.780233892547864905 ) ) ;
#76304=CARTESIAN_POINT ( 'NONE',  ( 167.7842790755206011, 278.3773043237077331, 14.72622960804143766 ) ) ;
#76305=CARTESIAN_POINT ( 'NONE',  ( 188.3964383979925401, 299.2957869059246718, -0.5852346544794374550 ) ) ;
#76307=CARTESIAN_POINT ( 'NONE',  ( 162.9294686138450459, 252.2324572554889812, -12.93311691499258309 ) ) ;
#76310=CARTESIAN_POINT ( 'NONE',  ( 189.7838259857693686, 299.9317662682615833, -5.554424272425116271 ) ) ;
#76311=CARTESIAN_POINT ( 'NONE',  ( 89.94416901687610277, 231.9244531367911009, -4.594050593750046652 ) ) ;
#76312=CARTESIAN_POINT ( 'NONE',  ( 207.7666684749232786, 270.7845694125510931, -6.630926507062123498 ) ) ;
#76313=CARTESIAN_POINT ( 'NONE',  ( 151.2455280670316711, 268.6820563007532314, 14.35914944935941229 ) ) ;
#76315=CYLINDRICAL_SURFACE ( 'NONE', #20966, 10.00000000000010658 ) ;
#76317=CARTESIAN_POINT ( 'NONE',  ( 201.1763559185644112, 270.5295643278437865, -10.00885884882298704 ) ) ;
#76318=CARTESIAN_POINT ( 'NONE',  ( 184.8303046393444049, 287.3399108598079579, -15.67031930442813348 ) ) ;
#76321=CARTESIAN_POINT ( 'NONE',  ( 123.7735466722555202, 252.2677522451419065, -5.000000000000047962 ) ) ;
#76325=CARTESIAN_POINT ( 'NONE',  ( 178.9095197733313114, 280.6377396294411710, 15.96141144708081860 ) ) ;
#76326=CARTESIAN_POINT ( 'NONE',  ( 193.2053309019613891, 296.0055459150826778, -12.79465285318189061 ) ) ;
#76328=VERTEX_POINT ( 'NONE', #14104 ) ;
#76329=B_SPLINE_SURFACE_WITH_KNOTS ( 'NONE', 3, 1, ( 
 ( #31841, #9065 ),
 ( #39932, #71379 ),
 ( #1968, #63762 ),
 ( #93700, #53645 ),
 ( #24263, #84600 ),
 ( #18673, #80002 ),
 ( #89130, #19682 ),
 ( #56655, #64771 ),
 ( #40934, #94694 ),
 ( #33360, #87640 ),
 ( #41446, #42437 ),
 ( #64260, #81500 ),
 ( #50543, #95211 ),
 ( #18168, #34842 ),
 ( #96201, #49554 ),
 ( #12068, #95720 ),
 ( #10571, #25256 ),
 ( #73372, #25780 ),
 ( #88621, #80507 ),
 ( #49068, #34359 ),
 ( #87137, #56139 ),
 ( #41957, #26763 ),
 ( #57645, #73865 ),
 ( #42925, #35352 ),
 ( #3959, #72386 ),
 ( #17669, #2996 ),
 ( #33886, #26268 ),
 ( #65745, #57144 ),
 ( #88126, #48567 ),
 ( #11081, #10069 ),
 ( #96699, #72892 ),
 ( #3484, #65256 ),
 ( #19189, #79508 ),
 ( #27267, #50060 ) ),
 .UNSPECIFIED., .T., .F., .F.,
 ( 4, 2, 2, 2, 2, 2, 2, 2, 2, 2, 2, 2, 2, 2, 2, 2, 4 ),
 ( 2, 2 ),
 ( 0.000000000000000000, 0.06250000000000000000, 0.1250000000000000000, 0.1875000000000000000, 0.2500000000000000000, 0.3125000000000000000, 0.3750000000000000000, 0.4375000000000000000, 0.5000000000000000000, 0.5625000000000000000, 0.6250000000000000000, 0.6875000000000000000, 0.7500000000000000000, 0.8125000000000000000, 0.8750000000000000000, 0.9375000000000000000, 1.000000000000000000 ),
 ( 0.000000000000000000, 1.000000000000000000 ),
 .UNSPECIFIED. ) ;
#76334=CARTESIAN_POINT ( 'NONE',  ( 173.2590479799806928, 253.7630292489582757, -9.109924965339219582 ) ) ;
#76336=CARTESIAN_POINT ( 'NONE',  ( 152.7618747630824885, 266.0556667813044101, 16.41480086888796919 ) ) ;
#76338=CARTESIAN_POINT ( 'NONE',  ( 187.2731080186762256, 278.8154626391448119, 17.13899673958438186 ) ) ;
#76341=CARTESIAN_POINT ( 'NONE',  ( 167.7069825692313429, 249.7662905202334969, 6.717005362718047934 ) ) ;
#76342=CARTESIAN_POINT ( 'NONE',  ( 184.5595156642797008, 292.1222730993646906, -10.69555203441723457 ) ) ;
#76346=CARTESIAN_POINT ( 'NONE',  ( 193.8837194332558056, 280.6698792847660684, -17.10338268821150720 ) ) ;
#76347=CARTESIAN_POINT ( 'NONE',  ( 153.9313804520737961, 264.0300235082304425, -16.64903060835773374 ) ) ;
#76348=CARTESIAN_POINT ( 'NONE',  ( 200.9445292274600092, 282.6008612054670266, -16.62830946367346741 ) ) ;
#76349=CARTESIAN_POINT ( 'NONE',  ( 169.0898264877448014, 257.6955085404131296, 15.20712983902550341 ) ) ;
#76350=ADVANCED_FACE ( 'NONE', ( #51605 ), #6508, .T. ) ;
#76355=VERTEX_POINT ( 'NONE', #55569 ) ;
#76356=CARTESIAN_POINT ( 'NONE',  ( 176.2398559119413051, 258.8095549018042334, 13.22354805979146697 ) ) ;
#76357=VERTEX_POINT ( 'NONE', #93629 ) ;
#76359=CARTESIAN_POINT ( 'NONE',  ( 198.0258880569907376, 286.7261629195996875, 16.96262172508392041 ) ) ;
#76360=CARTESIAN_POINT ( 'NONE',  ( 169.4301234034413426, 269.1242964454818889, 17.39485978491103069 ) ) ;
#76364=CARTESIAN_POINT ( 'NONE',  ( 201.1914266341661630, 274.9083111069574556, -13.97515993586548610 ) ) ;
#76366=CARTESIAN_POINT ( 'NONE',  ( 148.2159754900428936, 273.9293952882992471, 9.267836332806297150 ) ) ;
#76367=CARTESIAN_POINT ( 'NONE',  ( 167.0874653007571169, 286.5168870136799910, -4.892502125562864457 ) ) ;
#76369=CARTESIAN_POINT ( 'NONE',  ( 165.8866640751390094, 265.8956478032751534, 17.81115609982314751 ) ) ;
#76370=CARTESIAN_POINT ( 'NONE',  ( 183.5371895774011364, 284.7566254381118824, -15.01286450311582144 ) ) ;
#76371=CARTESIAN_POINT ( 'NONE',  ( 102.6097905472235539, 239.2369531367911009, -4.594050593750048428 ) ) ;
#76372=ORIENTED_EDGE ( 'NONE', *, *, #18772, .T. ) ;
#76375=CARTESIAN_POINT ( 'NONE',  ( 191.4296719636011517, 274.8339350444337583, 16.87517489376925539 ) ) ;
#76379=CARTESIAN_POINT ( 'NONE',  ( 180.7260405409376745, 294.0588039200300159, -2.607966119977916275 ) ) ;
#76380=CARTESIAN_POINT ( 'NONE',  ( 192.0670538266147958, 297.9770996426736929, 11.54736252216878256 ) ) ;
#76381=CARTESIAN_POINT ( 'NONE',  ( 206.7680519836501958, 272.5142239127119979, -10.57935479673322021 ) ) ;
#76382=CARTESIAN_POINT ( 'NONE',  ( 97.10949284993499475, 215.3262482093457493, 3.021315404115420679E-15 ) ) ;
#76383=ADVANCED_FACE ( 'NONE', ( #54565 ), #78921, .T. ) ;
#76388=ORIENTED_EDGE ( 'NONE', *, *, #87323, .F. ) ;
#76390=CARTESIAN_POINT ( 'NONE',  ( 191.8829787380248604, 267.6708518110137334, -12.49840204580878478 ) ) ;
#76391=CARTESIAN_POINT ( 'NONE',  ( 192.6073437551183645, 263.2194025587710939, 4.509002015703135413 ) ) ;
#76393=CARTESIAN_POINT ( 'NONE',  ( 163.1008115941903895, 248.1481028935802442, 11.25332017433677834 ) ) ;
#76394=CARTESIAN_POINT ( 'NONE',  ( 187.3716705114872809, 291.0127574213985895, -13.61402146762525334 ) ) ;
#76395=CARTESIAN_POINT ( 'NONE',  ( 156.9006073532037817, 280.5407770597218473, 5.988227030271738194 ) ) ;
#76396=CIRCLE ( 'NONE', #63434, 17.82106496071138224 ) ;
#76397=CARTESIAN_POINT ( 'NONE',  ( -22.42236680055709641, 157.8615022471902591, 0.000000000000000000 ) ) ;
#76399=CARTESIAN_POINT ( 'NONE',  ( 147.0670278774466908, 275.9194309285509235, 3.666898409139099257 ) ) ;
#76403=CARTESIAN_POINT ( 'NONE',  ( 172.7994643787747293, 251.3630591998880561, -0.2565247822977752556 ) ) ;
#76404=CARTESIAN_POINT ( 'NONE',  ( 192.5117867804768252, 271.3415924289031409, -15.10878263095346696 ) ) ;
#76407=CARTESIAN_POINT ( 'NONE',  ( 29.73762157799522399, 194.6427522451419065, 10.00000000000009415 ) ) ;
#76408=ADVANCED_FACE ( 'NONE', ( #61681 ), #36878, .F. ) ;
#76411=CARTESIAN_POINT ( 'NONE',  ( 81.74442484449845381, 211.8768266524159856, 9.188101187500098632 ) ) ;
#76413=CARTESIAN_POINT ( 'NONE',  ( 147.5749551500760788, 275.0396750858066639, -4.254929048021584670 ) ) ;
#76414=DIRECTION ( 'NONE',  ( -0.8660254037844387076, -0.4999999999999998890, -0.000000000000000000 ) ) ;
#76415=CARTESIAN_POINT ( 'NONE',  ( 196.8357460615746675, 288.9375519056556527, -16.76664714252133948 ) ) ;
#76417=CARTESIAN_POINT ( 'NONE',  ( 207.1019571622349815, 271.9358831784929293, -5.989975140547304733 ) ) ;
#76418=CARTESIAN_POINT ( 'NONE',  ( 167.5421813246326792, 287.5986610761024167, 3.969292590682533373 ) ) ;
#76419=CARTESIAN_POINT ( 'NONE',  ( 100.3908607700756619, 238.7677522451419065, -5.000000000000047962 ) ) ;
#76421=EDGE_CURVE ( 'NONE', #75268, #57662, #24574, .T. ) ;
#76422=CARTESIAN_POINT ( 'NONE',  ( 189.2845499996045930, 259.5340837477176024, -0.8149847707460528001 ) ) ;
#76424=CARTESIAN_POINT ( 'NONE',  ( 161.3697451762201922, 251.5394009270540607, 13.17726145763740853 ) ) ;
#76425=CARTESIAN_POINT ( 'NONE',  ( 189.7838259857693686, 299.9317662682615833, -5.554424272425116271 ) ) ;
#76427=CARTESIAN_POINT ( 'NONE',  ( 53.21953955946602122, 201.5333772461660544, 9.188101187500095079 ) ) ;
#76428=CARTESIAN_POINT ( 'NONE',  ( 196.2048238403250764, 290.8102717488927169, 17.53926796892840656 ) ) ;
#76429=CARTESIAN_POINT ( 'NONE',  ( 199.2752819598239000, 277.9111509360756145, 15.64615381322591681 ) ) ;
#76430=DIRECTION ( 'NONE',  ( -0.8660254037844387076, -0.4999999999999998890, -0.000000000000000000 ) ) ;
#76431=CARTESIAN_POINT ( 'NONE',  ( -18.88609640177068627, 173.2365022471903160, 2.944929066748280225E-16 ) ) ;
#76432=CARTESIAN_POINT ( 'NONE',  ( 50.02589733512838421, 205.8149278399161233, 9.188101187500093303 ) ) ;
#76434=CARTESIAN_POINT ( 'NONE',  ( 198.7829547491859330, 286.3448180261817129, -18.59838968157616179 ) ) ;
#76435=CARTESIAN_POINT ( 'NONE',  ( 196.8363552541316324, 289.7164272536036265, -17.80258609350122967 ) ) ;
#76437=CARTESIAN_POINT ( 'NONE',  ( 157.6500260163024620, 257.5891404556457474, -18.23450497588216379 ) ) ;
#76440=CARTESIAN_POINT ( 'NONE',  ( 179.8263126347392813, 276.7214098371354680, 16.33597602842999308 ) ) ;
#76442=CARTESIAN_POINT ( 'NONE',  ( 201.3598265928982869, 281.8815450682784558, 17.41054330225266966 ) ) ;
#76444=CARTESIAN_POINT ( 'NONE',  ( 107.4814437671086580, 242.8615022471903160, 5.000000000000046185 ) ) ;
#76445=CARTESIAN_POINT ( 'NONE',  ( 169.2681527202045118, 288.6954499571734800, 3.589104733571486516 ) ) ;
#76446=CARTESIAN_POINT ( 'NONE',  ( 165.2484375929805935, 269.8046256042021582, -16.27477966519025898 ) ) ;
#76449=ORIENTED_EDGE ( 'NONE', *, *, #62513, .F. ) ;
#76450=CARTESIAN_POINT ( 'NONE',  ( 166.5018518098672189, 264.8202169054221145, 16.82335354330060539 ) ) ;
#76451=CARTESIAN_POINT ( 'NONE',  ( 190.3620301733707834, 278.8805567241598169, -16.54082129631397891 ) ) ;
#76453=ORIENTED_EDGE ( 'NONE', *, *, #20347, .F. ) ;
#76454=CARTESIAN_POINT ( 'NONE',  ( 162.8756881843043516, 250.5380280774768949, 12.81046238701583029 ) ) ;
#76456=CARTESIAN_POINT ( 'NONE',  ( 194.4826705584825390, 293.7931287314651740, -16.11258321617245315 ) ) ;
#76458=AXIS2_PLACEMENT_3D ( 'NONE', #92676, #38928, #22748 ) ;
#76459=ORIENTED_EDGE ( 'NONE', *, *, #78233, .F. ) ;
#76462=CYLINDRICAL_SURFACE ( 'NONE', #5225, 10.00000000000010658 ) ;
#76467=ORIENTED_EDGE ( 'NONE', *, *, #39023, .F. ) ;
#76469=CARTESIAN_POINT ( 'NONE',  ( 170.8501576794184587, 284.6586050162820243, 10.94124936453461849 ) ) ;
#76470=CARTESIAN_POINT ( 'NONE',  ( 163.1241269448184710, 283.6514265758889906, -3.103922426645265187 ) ) ;
#76472=CARTESIAN_POINT ( 'NONE',  ( 163.1096928939807924, 248.1327200311062882, -9.690381021358412283 ) ) ;
#76473=CARTESIAN_POINT ( 'NONE',  ( 164.4761815919938215, 245.7658921781788592, 6.833796894895563412 ) ) ;
#76475=CARTESIAN_POINT ( 'NONE',  ( 164.6266891068947587, 265.1316493055271053, -16.62685662814512710 ) ) ;
#76476=B_SPLINE_CURVE_WITH_KNOTS ( 'NONE', 3,
 ( #83267, #6738, #14822, #21439 ),
 .UNSPECIFIED., .F., .F.,
 ( 4, 4 ),
 ( 0.01319540715386985363, 0.01956822373704288423 ),
 .UNSPECIFIED. ) ;
#76477=CARTESIAN_POINT ( 'NONE',  ( 134.8967340017684080, 242.5643266524160424, -9.188101187500093303 ) ) ;
#76479=CARTESIAN_POINT ( 'NONE',  ( 203.0230638682947699, 267.9133265956084529, 2.537566450392548134 ) ) ;
#76481=CARTESIAN_POINT ( 'NONE',  ( 179.5506826250896211, 257.8340240002441988, 10.21777184434937702 ) ) ;
#76482=CARTESIAN_POINT ( 'NONE',  ( 72.89481452351749624, 203.7048013555409796, 4.594050593750051981 ) ) ;
#76484=CARTESIAN_POINT ( 'NONE',  ( 176.4172214413987660, 252.1966103377273214, 1.934499474311637712 ) ) ;
#76490=CARTESIAN_POINT ( 'NONE',  ( 191.4738032422262677, 260.7793432447242594, -0.2951778641931921410 ) ) ;
#76494=CARTESIAN_POINT ( 'NONE',  ( 194.5047661587782386, 293.7548580291293092, 14.86680123054176583 ) ) ;
#76496=EDGE_CURVE ( 'NONE', #75612, #52858, #47891, .T. ) ;
#76497=ORIENTED_EDGE ( 'NONE', *, *, #69952, .F. ) ;
#76498=CARTESIAN_POINT ( 'NONE',  ( 200.9621566682951652, 282.5703295823330450, -16.90446154037251958 ) ) ;
#76502=CARTESIAN_POINT ( 'NONE',  ( 149.1429535397850827, 272.3238222086447990, -12.91457852089092384 ) ) ;
#76503=CARTESIAN_POINT ( 'NONE',  ( 194.9743901658331424, 279.5313095752043751, 16.57687009077668350 ) ) ;
#76504=CARTESIAN_POINT ( 'NONE',  ( 161.8358879837834365, 261.0030460270972412, 16.78525318079316264 ) ) ;
#76505=CARTESIAN_POINT ( 'NONE',  ( 140.4172988551291610, 258.0024278399160949, -9.188101187500093303 ) ) ;
#76510=CARTESIAN_POINT ( 'NONE',  ( 153.3939648708017387, 264.9608545997728015, -16.49556533540763681 ) ) ;
#76513=ORIENTED_EDGE ( 'NONE', *, *, #89036, .F. ) ;
#76514=CARTESIAN_POINT ( 'NONE',  ( 199.7315608606883757, 266.8161529887717620, 4.634410026811882410 ) ) ;
#76515=( BOUNDED_CURVE ( )  B_SPLINE_CURVE ( 2, ( #62787, #31881, #47587, #32397, #9620, #33398, #94730, #23789, #85658 ),
 .UNSPECIFIED., .F., .T. ) 
 B_SPLINE_CURVE_WITH_KNOTS ( ( 3, 2, 2, 2, 3 ),
 ( 0.7379032258064516236, 0.7392473118279569988, 0.7419354838709677491, 0.7446236559139784994, 0.7459677419354838745 ),
 .UNSPECIFIED. ) 
 CURVE ( )  GEOMETRIC_REPRESENTATION_ITEM ( )  RATIONAL_B_SPLINE_CURVE ( ( 0.9330127018922194093, 0.9330127018922194093, 1.000000000000000000, 0.8660254037844387076, 1.000000000000000000, 0.8660254037844387076, 1.000000000000000000, 0.9330127018922194093, 0.9330127018922194093 ) ) 
 REPRESENTATION_ITEM ( '' )  );
#76518=CARTESIAN_POINT ( 'NONE',  ( 25.20903040758703284, 185.3615022471902591, -10.00000000000009592 ) ) ;
#76519=CARTESIAN_POINT ( 'NONE',  ( 184.6202127605081387, 263.5949843424817800, -12.39504086723364651 ) ) ;
#76523=CARTESIAN_POINT ( 'NONE',  ( 146.9376205018946848, 276.1435710778808925, 5.066564108429441937 ) ) ;
#76526=EDGE_CURVE ( 'NONE', #11680, #37254, #97126, .T. ) ;
#76527=CARTESIAN_POINT ( 'NONE',  ( 207.3062152119541679, 271.5820978585240368, 7.879821064966149535 ) ) ;
#76528=CARTESIAN_POINT ( 'NONE',  ( 193.9204722154232741, 294.7668848255750049, 15.43855698596013859 ) ) ;
#76532=EDGE_CURVE ( 'NONE', #66560, #19653, #91190, .T. ) ;
#76536=CARTESIAN_POINT ( 'NONE',  ( 159.4285914931787431, 254.5085746851079023, 15.41072477910873673 ) ) ;
#76537=CARTESIAN_POINT ( 'NONE',  ( 144.5581563630820767, 254.2677522451418781, 10.00000000000009592 ) ) ;
#76542=CYLINDRICAL_SURFACE ( 'NONE', #53338, 17.82106496071139645 ) ;
#76543=CARTESIAN_POINT ( 'NONE',  ( 7.590652549690900308, 181.3149278399160949, -9.188101187500095079 ) ) ;
#76546=CARTESIAN_POINT ( 'NONE',  ( 170.7648842107952589, 271.0558799679138247, -16.70271480118435647 ) ) ;
#76547=CARTESIAN_POINT ( 'NONE',  ( 177.8222571804544430, 286.5223583772871621, 13.77940225188420875 ) ) ;
#76549=CARTESIAN_POINT ( 'NONE',  ( 175.6999050983589541, 253.1551923919900844, -3.327328156188026131 ) ) ;
#76551=CARTESIAN_POINT ( 'NONE',  ( 53.86003751612216917, 215.2365022471903444, 2.944929066748280225E-16 ) ) ;
#76553=CARTESIAN_POINT ( 'NONE',  ( 190.3691966041315311, 300.9178746160123410, 0.1783449565851275009 ) ) ;
#76554=CARTESIAN_POINT ( 'NONE',  ( 19.39059577201889084, 175.8768266524160140, 9.188101187500098632 ) ) ;
#76558=CARTESIAN_POINT ( 'NONE',  ( 164.2672861321391053, 246.1277097281173667, -2.417001679502223777 ) ) ;
#76559=CARTESIAN_POINT ( 'NONE',  ( 189.0332475110736823, 268.2270510816296110, 13.69286421477849380 ) ) ;
#76560=CARTESIAN_POINT ( 'NONE',  ( 160.1420032418522794, 278.6903965922204520, -9.786847659039947800 ) ) ;
#76561=CARTESIAN_POINT ( 'NONE',  ( 179.7070423342790662, 263.0192850531631734, -13.12411453645908743 ) ) ;
#76564=CARTESIAN_POINT ( 'NONE',  ( 190.6036479972031259, 300.5117928913073797, -0.6824572005520307405 ) ) ;
#76566=CARTESIAN_POINT ( 'NONE',  ( 194.4904290197884507, 293.7796906822950973, 14.50206953321744940 ) ) ;
#76568=CARTESIAN_POINT ( 'NONE',  ( 181.6021537782941948, 289.2296556448770843, 12.56736601662415787 ) ) ;
#76574=CARTESIAN_POINT ( 'NONE',  ( 153.8480465357228013, 265.0660884932569843, -16.61306390558784685 ) ) ;
#76577=CARTESIAN_POINT ( 'NONE',  ( 181.1649504240936324, 257.3422611971239462, -7.689218329250792294 ) ) ;
#76580=ORIENTED_EDGE ( 'NONE', *, *, #90388, .T. ) ;
#76581=CARTESIAN_POINT ( 'NONE',  ( 153.0444155045374544, 265.5662918618958201, -16.15173036748435109 ) ) ;
#76585=ORIENTED_EDGE ( 'NONE', *, *, #74601, .T. ) ;
#76586=CARTESIAN_POINT ( 'NONE',  ( 148.3519871123208986, 273.6938162480936398, 8.180046468253793890 ) ) ;
#76587=EDGE_CURVE ( 'NONE', #82896, #74751, #98163, .T. ) ;
#76589=CARTESIAN_POINT ( 'NONE',  ( 157.0957870390718369, 258.5491105237443321, 17.69218919045495397 ) ) ;
#76590=CARTESIAN_POINT ( 'NONE',  ( 158.0904712413047548, 265.1349370488131854, 17.45369701028249310 ) ) ;
#76592=CARTESIAN_POINT ( 'NONE',  ( 190.2389970918280540, 301.1433867864428748, 4.601241515604689525 ) ) ;
#76597=CARTESIAN_POINT ( 'NONE',  ( 159.5300091911712741, 255.0427242571105637, 15.76637448721640666 ) ) ;
#76604=CARTESIAN_POINT ( 'NONE',  ( 190.1813752874636805, 301.2431906792259042, -4.710625539811892359 ) ) ;
#76606=CARTESIAN_POINT ( 'NONE',  ( 190.3572031550745294, 300.9386478791372497, 3.093832330100951378 ) ) ;
#76608=CARTESIAN_POINT ( 'NONE',  ( 191.2740899065998121, 299.3505534407085520, 8.349120108963653308 ) ) ;
#76609=CARTESIAN_POINT ( 'NONE',  ( 191.7187529716733820, 298.5803744197520473, -8.487597704798396592 ) ) ;
#76612=FACE_OUTER_BOUND ( 'NONE', #96445, .T. ) ;
#76613=CARTESIAN_POINT ( 'NONE',  ( 196.9098758191317700, 289.5890858996224324, -16.54412079817003800 ) ) ;
#76614=DIRECTION ( 'NONE',  ( -0.8660254037844387076, -0.4999999999999998890, -0.000000000000000000 ) ) ;
#76616=CARTESIAN_POINT ( 'NONE',  ( 168.3793444054225290, 286.3781285656735349, 4.059011274220171828 ) ) ;
#76618=CARTESIAN_POINT ( 'NONE',  ( 108.5372593219620683, 221.2202760586659167, -5.415160957724236172E-17 ) ) ;
#76619=EDGE_LOOP ( 'NONE', ( #79140, #95463, #82881, #64999, #65265 ) ) ;
#76620=CARTESIAN_POINT ( 'NONE',  ( 190.8137524654443666, 300.1478812774159906, -3.757822530009682804 ) ) ;
#76622=CARTESIAN_POINT ( 'NONE',  ( 148.8152594325094640, 273.8656759551610094, 8.901672353312864772 ) ) ;
#76624=CARTESIAN_POINT ( 'NONE',  ( 179.6503533887556046, 282.9570081633805785, -15.82271799553900848 ) ) ;
#76626=CARTESIAN_POINT ( 'NONE',  ( 169.1676646093989973, 285.0513320500780878, -7.948105669459880396 ) ) ;
#76629=CARTESIAN_POINT ( 'NONE',  ( 206.7923762329701276, 272.4720930770340033, -9.496103119940368487 ) ) ;
#76630=ADVANCED_FACE ( 'NONE', ( #67096 ), #4824, .T. ) ;
#76632=CARTESIAN_POINT ( 'NONE',  ( 53.19247626382384908, 191.5177522451418213, 5.000000000000051514 ) ) ;
#76633=CARTESIAN_POINT ( 'NONE',  ( 113.0020953926368037, 245.2369531367911009, -4.594050593750048428 ) ) ;
#76634=CARTESIAN_POINT ( 'NONE',  ( 151.4188942279983223, 268.3817773016460251, -14.77302265413830895 ) ) ;
#76636=CARTESIAN_POINT ( 'NONE',  ( 157.5710319558766344, 257.7259621817996162, 18.28704422422941533 ) ) ;
#76637=CARTESIAN_POINT ( 'NONE',  ( 175.8738807006601235, 252.8402638148968720, -4.840734339853246304 ) ) ;
#76638=CARTESIAN_POINT ( 'NONE',  ( 38.06444208900335013, 180.5327760586659451, 1.948934522072303157E-15 ) ) ;
#76641=CARTESIAN_POINT ( 'NONE',  ( 9.795534599056948011, 164.9155109091896350, 2.679491924311254714 ) ) ;
#76642=CARTESIAN_POINT ( 'NONE',  ( 177.9052955790886870, 265.4696414361982306, 15.73918422437849074 ) ) ;
#76645=CARTESIAN_POINT ( 'NONE',  ( 190.6218339396177441, 300.4802939150614520, -4.178005820806754755 ) ) ;
#76646=CARTESIAN_POINT ( 'NONE',  ( 97.22339252480620075, 238.4860189848785410, -2.679491924311252493 ) ) ;
#76647=CARTESIAN_POINT ( 'NONE',  ( 188.2735287570237688, 299.1710073388255751, -5.251721556916531419 ) ) ;
#76648=CARTESIAN_POINT ( 'NONE',  ( 166.1961671434869174, 251.1444224861350563, 10.22506114935430155 ) ) ;
#76649=CARTESIAN_POINT ( 'NONE',  ( 104.2879750871056928, 231.0177522451418781, -10.00000000000009592 ) ) ;
#76651=VERTEX_POINT ( 'NONE', #90459 ) ;
#76652=CARTESIAN_POINT ( 'NONE',  ( 163.0683798854284703, 248.2042762609320903, 11.26611642476872710 ) ) ;
#76655=CARTESIAN_POINT ( 'NONE',  ( 14.51920287573142510, 173.0643266524160140, 9.188101187500095079 ) ) ;
#76657=CARTESIAN_POINT ( 'NONE',  ( 192.3965733967720269, 272.0314340560001938, 14.18959370928753572 ) ) ;
#76660=CARTESIAN_POINT ( 'NONE',  ( 174.6894609039457009, 286.3781494789058115, 10.38366818161665606 ) ) ;
#76661=CARTESIAN_POINT ( 'NONE',  ( 56.60219097117523290, 212.6744531367911293, 4.594050593750047540 ) ) ;
#76662=CARTESIAN_POINT ( 'NONE',  ( 200.5621507313343557, 283.2631601884785368, 16.81037192529623425 ) ) ;
#76668=CARTESIAN_POINT ( 'NONE',  ( 165.1220678389894090, 269.0795942023863745, 16.79297129081651363 ) ) ;
#76669=CARTESIAN_POINT ( 'NONE',  ( 11.42479273068475010, 170.7365022471902023, 10.00000000000009592 ) ) ;
#76671=CARTESIAN_POINT ( 'NONE',  ( 164.3890147726454813, 245.9168695380243435, -6.010262808998044548 ) ) ;
#76672=CARTESIAN_POINT ( 'NONE',  ( 140.2550926398021147, 251.7833772461660544, -9.188101187500095079 ) ) ;
#76674=CARTESIAN_POINT ( 'NONE',  ( 165.9273809406606688, 261.6126396426859628, -16.19544363369431750 ) ) ;
#76677=AXIS2_PLACEMENT_3D ( 'NONE', #8800, #62473, #87871 ) ;
#76682=CARTESIAN_POINT ( 'NONE',  ( 190.9501423151522772, 299.9116471280854626, 8.746938802470586083 ) ) ;
#76684=CARTESIAN_POINT ( 'NONE',  ( 196.6597737787374456, 289.2349992526956726, 16.68652926890371546 ) ) ;
#76687=CARTESIAN_POINT ( 'NONE',  ( 206.9158469655446879, 272.2582354949668684, 9.541657424068484161 ) ) ;
#76689=CYLINDRICAL_SURFACE ( 'NONE', #23059, 10.00000000000010658 ) ;
#76690=CARTESIAN_POINT ( 'NONE',  ( -22.42236680055709641, 157.8615022471902591, 0.000000000000000000 ) ) ;
#76693=CARTESIAN_POINT ( 'NONE',  ( 152.6621968174709991, 266.2283140474973493, -17.02835521334403168 ) ) ;
#76695=CARTESIAN_POINT ( 'NONE',  ( 173.8805019302338621, 250.6242863632701585, 0.4030408839048176262 ) ) ;
#76697=CARTESIAN_POINT ( 'NONE',  ( 190.0445576990143195, 301.4801656937889902, 4.140328216824785912 ) ) ;
#76700=EDGE_LOOP ( 'NONE', ( #85862, #2798, #97518, #58557 ) ) ;
#76701=CARTESIAN_POINT ( 'NONE',  ( 191.0478321355427624, 299.7424433957868928, -9.006798842970001218 ) ) ;
#76702=CARTESIAN_POINT ( 'NONE',  ( 174.8906308118707216, 255.9997517440984893, -11.44291824309870975 ) ) ;
#76703=B_SPLINE_CURVE_WITH_KNOTS ( 'NONE', 3,
 ( #4491, #35384, #37862, #91125 ),
 .UNSPECIFIED., .F., .F.,
 ( 4, 4 ),
 ( 0.01152314744103701688, 0.01766322936049247866 ),
 .UNSPECIFIED. ) ;
#76704=CARTESIAN_POINT ( 'NONE',  ( 196.8363552541316324, 289.7164272536036265, -17.80258609350122967 ) ) ;
#76707=CARTESIAN_POINT ( 'NONE',  ( 111.1353355333153843, 222.7202760586659167, -5.415160957724236172E-17 ) ) ;
#76709=CARTESIAN_POINT ( 'NONE',  ( 181.1618576654650212, 271.6441367243567697, -16.30549846865705277 ) ) ;
#76710=CARTESIAN_POINT ( 'NONE',  ( 132.0007880082076781, 257.0177522451418781, 5.000000000000046185 ) ) ;
#76711=VERTEX_POINT ( 'NONE', #97056 ) ;
#76713=EDGE_CURVE ( 'NONE', #85978, #20151, #53448, .T. ) ;
#76714=ORIENTED_EDGE ( 'NONE', *, *, #77280, .F. ) ;
#76716=ORIENTED_EDGE ( 'NONE', *, *, #85842, .T. ) ;
#76717=EDGE_CURVE ( 'NONE', #15906, #6168, #61113, .T. ) ;
#76720=CARTESIAN_POINT ( 'NONE',  ( 208.0287371622045782, 270.3306531311065442, 3.558879245883286746 ) ) ;
#76723=CARTESIAN_POINT ( 'NONE',  ( 170.8465782694706263, 283.6086715855652187, 12.33509960992013355 ) ) ;
#76728=CARTESIAN_POINT ( 'NONE',  ( 201.2591206913006658, 271.2044317791411459, -11.41792222164669113 ) ) ;
#76730=CARTESIAN_POINT ( 'NONE',  ( 202.0661878422603763, 279.1895584290143120, -16.02388874507808225 ) ) ;
#76732=CARTESIAN_POINT ( 'NONE',  ( 20.30386484825465132, 170.9824982072973967, 3.021315404115420679E-15 ) ) ;
#76734=CARTESIAN_POINT ( 'NONE',  ( 202.5245888501533216, 279.8641176599742266, 15.60152447840272494 ) ) ;
#76736=DIRECTION ( 'NONE',  ( -0.8660254037844387076, -0.4999999999999998890, -0.000000000000000000 ) ) ;
#76740=CARTESIAN_POINT ( 'NONE',  ( 160.9160827979327166, 283.0037893736308661, 2.110134644200618137 ) ) ;
#76742=CARTESIAN_POINT ( 'NONE',  ( 155.7106188756215204, 260.9482921598670373, -17.31404547047129938 ) ) ;
#76744=CARTESIAN_POINT ( 'NONE',  ( 1.663964738649655661, 181.7677522451419350, -5.000000000000047962 ) ) ;
#76747=CARTESIAN_POINT ( 'NONE',  ( 165.6131678205262290, 248.3344997053549434, 8.498622568436868363 ) ) ;
#76748=CARTESIAN_POINT ( 'NONE',  ( 163.8807549990905841, 246.7972012892647626, -8.911697419588444191 ) ) ;
#76750=CARTESIAN_POINT ( 'NONE',  ( 162.6383036806675193, 250.7589265055833323, -12.97350464324780184 ) ) ;
#76751=CARTESIAN_POINT ( 'NONE',  ( -2.016382903836450691, 160.4548013555409796, -4.594050593750042211 ) ) ;
#76755=ORIENTED_EDGE ( 'NONE', *, *, #82586, .F. ) ;
#76759=CARTESIAN_POINT ( 'NONE',  ( 202.7081908165554296, 279.5461097257963843, -16.92338847124122481 ) ) ;
#76761=CARTESIAN_POINT ( 'NONE',  ( 151.2757240218323886, 277.1518032949712165, 3.694889182893786650 ) ) ;
#76762=CARTESIAN_POINT ( 'NONE',  ( 14.59995888762994554, 188.4244531367911293, -4.594050593750046652 ) ) ;
#76763=CARTESIAN_POINT ( 'NONE',  ( 111.8924135700967355, 247.6589784336661069, -6.496448406907675876E-16 ) ) ;
#76764=CARTESIAN_POINT ( 'NONE',  ( 182.1055966411629186, 294.5202151697680506, -6.440452032333615406 ) ) ;
#76765=CARTESIAN_POINT ( 'NONE',  ( 196.2659867875262876, 275.2308177797455642, 16.04285008767656606 ) ) ;
#76766=CARTESIAN_POINT ( 'NONE',  ( 27.73493783529162116, 193.4865022471903160, -10.00000000000009592 ) ) ;
#76767=EDGE_CURVE ( 'NONE', #39680, #34226, #34104, .T. ) ;
#76768=CARTESIAN_POINT ( 'NONE',  ( 178.4166537163541193, 283.9060778229895163, -15.00412117590805572 ) ) ;
#76769=EDGE_CURVE ( 'NONE', #40898, #67853, #8786, .T. ) ;
#76770=CARTESIAN_POINT ( 'NONE',  ( 190.7246925096072516, 299.7733309290570674, -5.038784231807341918 ) ) ;
#76771=CARTESIAN_POINT ( 'NONE',  ( 195.8248271798537417, 291.4684452715354155, 17.35175160929494709 ) ) ;
#76772=CARTESIAN_POINT ( 'NONE',  ( 194.4263876777154394, 293.8906135405502482, 15.23185943445137802 ) ) ;
#76773=CARTESIAN_POINT ( 'NONE',  ( 161.1747502674735415, 251.4841389699472529, -13.25152330924089839 ) ) ;
#76776=CARTESIAN_POINT ( 'NONE',  ( 192.7415923820568082, 264.8708757276006622, 7.413265226357134807 ) ) ;
#76777=CARTESIAN_POINT ( 'NONE',  ( 169.3859977840389774, 278.7875771771462610, 14.01937899539775323 ) ) ;
#76778=CARTESIAN_POINT ( 'NONE',  ( 175.4391368986771340, 256.4972366567271251, -10.87669320986560528 ) ) ;
#76781=CARTESIAN_POINT ( 'NONE',  ( 151.7249709189835016, 274.7820922814796631, 10.79316925266204308 ) ) ;
#76782=ORIENTED_EDGE ( 'NONE', *, *, #68441, .T. ) ;
#76784=CARTESIAN_POINT ( 'NONE',  ( 184.7639518824382776, 269.2648697177924078, 16.06510220747506068 ) ) ;
#76786=CARTESIAN_POINT ( 'NONE',  ( 85.18102929606172324, 229.1744531367911293, 4.594050593750047540 ) ) ;
#76791=CARTESIAN_POINT ( 'NONE',  ( 191.7417035528519875, 277.0673726153275425, 16.68325300976718850 ) ) ;
#76792=CARTESIAN_POINT ( 'NONE',  ( 196.5464242819039384, 290.2186024281901950, 17.89341495589234654 ) ) ;
#76793=CARTESIAN_POINT ( 'NONE',  ( 198.7136873185829984, 286.4647927352960437, -18.57144721070432070 ) ) ;
#76794=CARTESIAN_POINT ( 'NONE',  ( 137.6559535675401094, 261.8297689869268652, -2.679491924311252493 ) ) ;
#76796=CARTESIAN_POINT ( 'NONE',  ( 192.4212750754384160, 297.3635704425909125, -12.73704185013552248 ) ) ;
#76797=FACE_OUTER_BOUND ( 'NONE', #84612, .T. ) ;
#76802=CARTESIAN_POINT ( 'NONE',  ( 149.6890529486499872, 271.3779502865075983, -12.51465682618088593 ) ) ;
#76803=( BOUNDED_CURVE ( )  B_SPLINE_CURVE ( 2, ( #78464, #24739, #951, #39918, #16640, #92198, #77959, #70853, #31827 ),
 .UNSPECIFIED., .F., .T. ) 
 B_SPLINE_CURVE_WITH_KNOTS ( ( 3, 2, 2, 2, 3 ),
 ( 0.2379032258064516236, 0.2392473118279569988, 0.2419354838709677491, 0.2446236559139784994, 0.2459677419354838745 ),
 .UNSPECIFIED. ) 
 CURVE ( )  GEOMETRIC_REPRESENTATION_ITEM ( )  RATIONAL_B_SPLINE_CURVE ( ( 0.9330127018922194093, 0.9330127018922194093, 1.000000000000000000, 0.8660254037844387076, 1.000000000000000000, 0.8660254037844387076, 1.000000000000000000, 0.9330127018922194093, 0.9330127018922194093 ) ) 
 REPRESENTATION_ITEM ( '' )  );
#76807=CARTESIAN_POINT ( 'NONE',  ( 171.2194629759952988, 253.1908842429618289, -8.786472813057685016 ) ) ;
#76813=ORIENTED_EDGE ( 'NONE', *, *, #11905, .F. ) ;
#76814=CARTESIAN_POINT ( 'NONE',  ( 168.1385646420976343, 249.0247310940818011, 6.544369751715001016 ) ) ;
#76815=CARTESIAN_POINT ( 'NONE',  ( 181.5035962553983211, 290.8403058601051612, -11.04694206434262682 ) ) ;
#76819=DIRECTION ( 'NONE',  ( -0.8660254037844387076, -0.4999999999999998890, -0.000000000000000000 ) ) ;
#76821=CARTESIAN_POINT ( 'NONE',  ( 200.8251833487811666, 282.8075743310126882, -16.74393672780000131 ) ) ;
#76822=LINE ( 'NONE', #7417, #17289 ) ;
#76823=DIRECTION ( 'NONE',  ( -0.8660254037844387076, -0.4999999999999998890, -0.000000000000000000 ) ) ;
#76824=CARTESIAN_POINT ( 'NONE',  ( 195.8961960204858599, 266.5302481932577621, 9.552191782196176817 ) ) ;
#76828=VERTEX_POINT ( 'NONE', #54365 ) ;
#76829=ORIENTED_EDGE ( 'NONE', *, *, #20706, .F. ) ;
#76830=CARTESIAN_POINT ( 'NONE',  ( 172.2043063819207021, 270.6962890225300953, 16.45290475606747549 ) ) ;
#76834=CARTESIAN_POINT ( 'NONE',  ( 200.9558679789573148, 274.8618586551609155, -13.87171223153703004 ) ) ;
#76837=CARTESIAN_POINT ( 'NONE',  ( 168.9820521491120360, 250.0049531100763716, -5.469593116480293560 ) ) ;
#76840=CARTESIAN_POINT ( 'NONE',  ( 178.0511205245788346, 255.4621034402314024, 4.984966428951989492 ) ) ;
#76841=CARTESIAN_POINT ( 'NONE',  ( 122.6912752411227103, 232.4548013555409796, -4.594050593750042211 ) ) ;
#76844=CARTESIAN_POINT ( 'NONE',  ( 187.9335791911229023, 273.9157097510401400, 16.49127241766424490 ) ) ;
#76851=EDGE_CURVE ( 'NONE', #21764, #78112, #81327, .T. ) ;
#76852=CARTESIAN_POINT ( 'NONE',  ( 146.6727924462101669, 276.6022667255962801, 3.481050673020940511 ) ) ;
#76853=CARTESIAN_POINT ( 'NONE',  ( 159.2651917302844993, 254.7915913763855258, -16.53922207549818424 ) ) ;
#76856=CARTESIAN_POINT ( 'NONE',  ( 148.3925088351605552, 273.6236305653253567, 10.42437868982396054 ) ) ;
#76862=CARTESIAN_POINT ( 'NONE',  ( 196.0526458812441035, 264.7804988895400697, 3.830367068405413189 ) ) ;
#76863=CARTESIAN_POINT ( 'NONE',  ( 158.3700511340344121, 263.3548805506079020, 17.43552943246885789 ) ) ;
#76865=CARTESIAN_POINT ( 'NONE',  ( 184.3332131814447621, 288.6360765898637624, -14.21508448381140965 ) ) ;
#76866=DIRECTION ( 'NONE',  ( -0.8660254037844387076, -0.4999999999999998890, -0.000000000000000000 ) ) ;
#76867=CARTESIAN_POINT ( 'NONE',  ( 153.2513309553138470, 265.2079037882803618, -16.24091495603130397 ) ) ;
#76868=VERTEX_POINT ( 'NONE', #61968 ) ;
#76869=CARTESIAN_POINT ( 'NONE',  ( 190.1635032421960148, 301.2741459696644029, -5.047660290019184259 ) ) ;
#76872=CARTESIAN_POINT ( 'NONE',  ( 33.41027130880567597, 178.5494855054051300, -2.679491924311248496 ) ) ;
#76873=CARTESIAN_POINT ( 'NONE',  ( 189.5354676446069391, 270.3341974172179221, -14.09206254053018270 ) ) ;
#76874=CARTESIAN_POINT ( 'NONE',  ( 177.9552638626009298, 260.7378092407702184, -13.94576028113082877 ) ) ;
#76876=CARTESIAN_POINT ( 'NONE',  ( 36.44700672854521883, 203.3967562850347122, 1.101618078115930403E-13 ) ) ;
#76878=CARTESIAN_POINT ( 'NONE',  ( 191.4168617962777148, 282.8041663340243872, -17.08726176923725149 ) ) ;
#76880=CARTESIAN_POINT ( 'NONE',  ( 68.83479979963041728, 219.7369531367911293, -4.594050593750048428 ) ) ;
#76881=CARTESIAN_POINT ( 'NONE',  ( 26.17072728691639583, 197.4637435831424739, 2.679491924311251605 ) ) ;
#76882=CARTESIAN_POINT ( 'NONE',  ( 192.8607783413999073, 296.6023284558532396, -11.80574095728561446 ) ) ;
#76884=CARTESIAN_POINT ( 'NONE',  ( 155.3716771045260714, 261.5353565282119348, -18.54934131471355840 ) ) ;
#76886=CARTESIAN_POINT ( 'NONE',  ( 161.8153478334749877, 250.3745914384277285, -14.21120979595050215 ) ) ;
#76887=CARTESIAN_POINT ( 'NONE',  ( -22.42236680055709641, 157.8615022471902591, 0.000000000000000000 ) ) ;
#76891=CARTESIAN_POINT ( 'NONE',  ( 204.8015065334591043, 275.9203805478366576, -12.93433564072899600 ) ) ;
#76892=CARTESIAN_POINT ( 'NONE',  ( 157.4656258344471098, 257.9085309395441641, 18.30485740784190796 ) ) ;
#76894=CARTESIAN_POINT ( 'NONE',  ( 32.43492986863949312, 189.5333772461660544, 9.188101187500095079 ) ) ;
#76896=CARTESIAN_POINT ( 'NONE',  ( 60.66220569506229765, 196.6423013555410080, -4.594050593750043987 ) ) ;
#76897=CARTESIAN_POINT ( 'NONE',  ( 157.5042325173297684, 257.8416622032797818, 16.70595240278738203 ) ) ;
#76899=DIRECTION ( 'NONE',  ( 0.4999999999999998890, -0.8660254037844385966, 0.000000000000000000 ) ) ;
#76900=CARTESIAN_POINT ( 'NONE',  ( 150.1604317434691325, 251.3768266524160140, -9.188101187500091527 ) ) ;
#76902=CARTESIAN_POINT ( 'NONE',  ( 200.1288169248181816, 270.7711892690550712, -11.55673819778957956 ) ) ;
#76905=CARTESIAN_POINT ( 'NONE',  ( 198.4427928769277969, 286.9339956717308837, -17.97122743692687763 ) ) ;
#76908=CARTESIAN_POINT ( 'NONE',  ( 60.68900866710680475, 205.8458772461660544, 9.188101187500095079 ) ) ;
#76910=B_SPLINE_CURVE_WITH_KNOTS ( 'NONE', 3,
 ( #27602, #97506, #89919, #98992, #29575, #91406 ),
 .UNSPECIFIED., .F., .F.,
 ( 4, 2, 4 ),
 ( 0.02165947195459741459, 0.02624956959626738653, 0.03083966723793735848 ),
 .UNSPECIFIED. ) ;
#76912=CARTESIAN_POINT ( 'NONE',  ( 159.5573297132660002, 254.2855935470410031, 16.91607698584599007 ) ) ;
#76914=CARTESIAN_POINT ( 'NONE',  ( 153.0920794520761206, 277.2686993117134762, 8.274819790008697495 ) ) ;
#76918=CARTESIAN_POINT ( 'NONE',  ( 111.0177141658951143, 248.2365022471903444, 2.944929066748280225E-16 ) ) ;
#76919=CARTESIAN_POINT ( 'NONE',  ( 200.1444820856229967, 283.9865835035790269, 17.93386694781497326 ) ) ;
#76920=CARTESIAN_POINT ( 'NONE',  ( 207.6918009085542849, 270.9142438413412037, 7.009114282139513818 ) ) ;
#76921=VERTEX_POINT ( 'NONE', #16886 ) ;
#76924=CARTESIAN_POINT ( 'NONE',  ( 159.9894443651313338, 253.5371490153152081, -16.36035038356864391 ) ) ;
#76925=CARTESIAN_POINT ( 'NONE',  ( 186.8956715526903167, 276.6081854589048135, -17.33659699395019516 ) ) ;
#76927=ORIENTED_EDGE ( 'NONE', *, *, #41114, .T. ) ;
#76928=ORIENTED_EDGE ( 'NONE', *, *, #89860, .F. ) ;
#76930=CARTESIAN_POINT ( 'NONE',  ( 194.1789525331299728, 294.3191837825503967, -15.34533909744314961 ) ) ;
#76931=CARTESIAN_POINT ( 'NONE',  ( 177.0218378549533327, 274.6764583735296696, -16.80540863426473308 ) ) ;
#76937=ADVANCED_FACE ( 'NONE', ( #71112 ), #78223, .F. ) ;
#76939=ORIENTED_EDGE ( 'NONE', *, *, #15028, .F. ) ;
#76940=CARTESIAN_POINT ( 'NONE',  ( 178.8595466249924755, 265.0989930076032124, -16.03772641351113748 ) ) ;
#76945=CARTESIAN_POINT ( 'NONE',  ( 174.7281960057983383, 286.2758036095501097, 11.50214825767278448 ) ) ;
#76949=CARTESIAN_POINT ( 'NONE',  ( 163.7239493340838123, 247.0687966679708438, 6.286946239157660266 ) ) ;
#76951=CARTESIAN_POINT ( 'NONE',  ( 164.6294852917785931, 265.1817657174682381, -16.63052033780461869 ) ) ;
#76952=CARTESIAN_POINT ( 'NONE',  ( 144.9103262809084924, 242.2202760586659167, -5.415160957724236172E-17 ) ) ;
#76954=CARTESIAN_POINT ( 'NONE',  ( 177.3466669983353938, 269.1945114843388751, 16.08467660924950593 ) ) ;
#76955=CARTESIAN_POINT ( 'NONE',  ( 181.2069392775523227, 259.9445122199059597, 9.505921896722259845 ) ) ;
#76956=CARTESIAN_POINT ( 'NONE',  ( 63.63864737692379236, 216.7369531367911293, -4.594050593750048428 ) ) ;
#76957=ORIENTED_EDGE ( 'NONE', *, *, #4123, .F. ) ;
#76958=CARTESIAN_POINT ( 'NONE',  ( 173.6315150813169623, 265.4685547730397843, 16.13185304422783162 ) ) ;
#76962=CARTESIAN_POINT ( 'NONE',  ( 157.3040537939580190, 258.1883819227538197, -18.30432891822131225 ) ) ;
#76963=ORIENTED_EDGE ( 'NONE', *, *, #96849, .T. ) ;
#76965=CARTESIAN_POINT ( 'NONE',  ( 79.15288444911743682, 228.0530062829863027, -4.648177544792955347E-16 ) ) ;
#76968=CARTESIAN_POINT ( 'NONE',  ( 197.8021188482492789, 286.7634004315060565, 16.92933056012654802 ) ) ;
#76969=CARTESIAN_POINT ( 'NONE',  ( 146.7373254022577100, 276.4904923669593586, -0.7242168585908188572 ) ) ;
#76971=CARTESIAN_POINT ( 'NONE',  ( 155.2098048002210930, 261.8157275836062468, 16.98811268941991059 ) ) ;
#76973=CARTESIAN_POINT ( 'NONE',  ( 76.87303194821100760, 209.0643266524160424, 9.188101187500095079 ) ) ;
#76981=CARTESIAN_POINT ( 'NONE',  ( 163.4520133936471495, 284.3138964249058631, 0.5061738602265062337 ) ) ;
#76983=CARTESIAN_POINT ( 'NONE',  ( 162.7485557827231446, 261.3830000631959365, 17.54795403777559670 ) ) ;
#76985=CARTESIAN_POINT ( 'NONE',  ( 158.8270733235451075, 260.0119502166541565, 17.68969926203419618 ) ) ;
#76986=CARTESIAN_POINT ( 'NONE',  ( 156.6857699971041029, 274.0622359378131137, 13.49643617979643118 ) ) ;
#76987=DIRECTION ( 'NONE',  ( -0.8660254037844387076, -0.4999999999999998890, -0.000000000000000000 ) ) ;
#76988=CARTESIAN_POINT ( 'NONE',  ( 153.0927037754837556, 265.4826541232073964, -16.15085267704102634 ) ) ;
#76990=CARTESIAN_POINT ( 'NONE',  ( 187.7710022618638277, 277.0665775429750397, -17.72351784843695555 ) ) ;
#76992=CARTESIAN_POINT ( 'NONE',  ( 199.7757112945883478, 266.5330615442240401, 4.708490324072631239 ) ) ;
#76994=CARTESIAN_POINT ( 'NONE',  ( 20.74252405664088172, 194.3297689869269220, -2.679491924311252493 ) ) ;
#76997=CARTESIAN_POINT ( 'NONE',  ( 156.0186942281396796, 271.8450601007914997, 14.11081356587844660 ) ) ;
#76998=VERTEX_POINT ( 'NONE', #48628 ) ;
#76999=CARTESIAN_POINT ( 'NONE',  ( 147.5813496936708020, 275.0285994114094592, 4.516581957185684004 ) ) ;
#77000=CARTESIAN_POINT ( 'NONE',  ( 202.8211298556536804, 279.3504935719197988, 17.07914446815911447 ) ) ;
#77001=EDGE_CURVE ( 'NONE', #55644, #23266, #47515, .T. ) ;
#77003=CARTESIAN_POINT ( 'NONE',  ( 164.2600772519394923, 246.1401958748887182, -2.110785484364219311 ) ) ;
#77004=CARTESIAN_POINT ( 'NONE',  ( 194.3799873100184641, 293.9709813348915191, 15.33105633561973669 ) ) ;
#77009=CARTESIAN_POINT ( 'NONE',  ( 165.4889794677011423, 286.4264833526404459, -3.351811820826717359 ) ) ;
#77010=CARTESIAN_POINT ( 'NONE',  ( 129.1320788617196911, 245.3615022471902591, -10.00000000000009592 ) ) ;
#77013=CARTESIAN_POINT ( 'NONE',  ( -12.49048504844327745, 175.8464784336661353, 1.353441290958777327E-15 ) ) ;
#77015=ORIENTED_EDGE ( 'NONE', *, *, #89670, .T. ) ;
#77020=CARTESIAN_POINT ( 'NONE',  ( 15.73713787374454043, 170.7048013555409796, 4.594050593750051981 ) ) ;
#77023=CARTESIAN_POINT ( 'NONE',  ( 181.1741292703470663, 294.4598225981704331, 6.531841373275609541 ) ) ;
#77024=CARTESIAN_POINT ( 'NONE',  ( 170.9037867558837718, 271.1323369732969013, -16.66440209927639415 ) ) ;
#77025=CARTESIAN_POINT ( 'NONE',  ( 154.9032082715209810, 280.6326124547101699, -2.389722542998433230 ) ) ;
#77026=CARTESIAN_POINT ( 'NONE',  ( 175.9272209172219164, 253.8149587822312014, -3.863606349031126097 ) ) ;
#77027=ADVANCED_FACE ( 'NONE', ( #25836 ), #11630, .T. ) ;
#77028=CARTESIAN_POINT ( 'NONE',  ( 188.6440864781562539, 260.6118655346156174, -0.7579459963146770729 ) ) ;
#77030=CARTESIAN_POINT ( 'NONE',  ( 182.9192744200266816, 296.0790939607076098, 1.760360045685976260 ) ) ;
#77031=CARTESIAN_POINT ( 'NONE',  ( 69.30415721694468800, 217.4865022471902876, -10.00000000000009415 ) ) ;
#77033=CARTESIAN_POINT ( 'NONE',  ( 148.3997536239841679, 273.6110822229926498, 8.713694244701960301 ) ) ;
#77034=CARTESIAN_POINT ( 'NONE',  ( 39.11982377592438809, 184.2048013555409796, 4.594050593750051981 ) ) ;
#77037=CARTESIAN_POINT ( 'NONE',  ( 203.0143287164872845, 269.9738428714081238, -6.283217384528930971 ) ) ;
#77038=CARTESIAN_POINT ( 'NONE',  ( 151.2646864780760723, 268.6488729594320830, -14.38346604407754548 ) ) ;
#77039=CARTESIAN_POINT ( 'NONE',  ( 207.6860335175200589, 270.9242332556395922, 6.913225035677485586 ) ) ;
#77040=CARTESIAN_POINT ( 'NONE',  ( 185.1815156408660812, 266.7917036737816261, 13.95118630758742917 ) ) ;
#77041=CARTESIAN_POINT ( 'NONE',  ( 163.1964476821512449, 280.9516185401507755, -10.10006455857531371 ) ) ;
#77044=DIRECTION ( 'NONE',  ( -0.8660254037844359321, -0.5000000000000051070, -0.000000000000000000 ) ) ;
#77046=CARTESIAN_POINT ( 'NONE',  ( 188.7841062153288192, 270.3218309834035153, -14.49186609326428687 ) ) ;
#77050=CARTESIAN_POINT ( 'NONE',  ( -22.42236680055709641, 157.8615022471902591, 0.000000000000000000 ) ) ;
#77054=CARTESIAN_POINT ( 'NONE',  ( 155.6483466250159893, 262.7148938034327443, -17.56146835583262344 ) ) ;
#77057=DIRECTION ( 'NONE',  ( -0.8660254037844387076, -0.4999999999999998890, -0.000000000000000000 ) ) ;
#77061=ORIENTED_EDGE ( 'NONE', *, *, #71734, .F. ) ;
#77067=CARTESIAN_POINT ( 'NONE',  ( 150.7530568467738590, 269.5350414755053521, 15.60317050893315916 ) ) ;
#77071=ORIENTED_EDGE ( 'NONE', *, *, #90152, .T. ) ;
#77072=CARTESIAN_POINT ( 'NONE',  ( 189.9462859318020946, 301.6503773875500087, -1.164147598593831656 ) ) ;
#77074=CARTESIAN_POINT ( 'NONE',  ( 196.5806080813426888, 290.1593943507663766, -16.31912166233602690 ) ) ;
#77077=CARTESIAN_POINT ( 'NONE',  ( 157.3988263959001870, 258.0242309610243865, 16.72376558639979294 ) ) ;
#77080=CARTESIAN_POINT ( 'NONE',  ( 158.6580134701507632, 265.3810918834140580, 16.98815342382654947 ) ) ;
#77084=VERTEX_POINT ( 'NONE', #52590 ) ;
#77087=CARTESIAN_POINT ( 'NONE',  ( 162.1260167985288376, 266.6785162637209510, 17.71249957499354366 ) ) ;
#77092=( BOUNDED_CURVE ( )  B_SPLINE_CURVE ( 2, ( #42328, #58042, #4341, #34246, #89023, #19574, #65143, #28133, #50434 ),
 .UNSPECIFIED., .F., .T. ) 
 B_SPLINE_CURVE_WITH_KNOTS ( ( 3, 2, 2, 2, 3 ),
 ( 0.1169354838709677491, 0.1182795698924731242, 0.1209677419354838745, 0.1236559139784946248, 0.1250000000000000000 ),
 .UNSPECIFIED. ) 
 CURVE ( )  GEOMETRIC_REPRESENTATION_ITEM ( )  RATIONAL_B_SPLINE_CURVE ( ( 0.9330127018922192983, 0.9330127018922196314, 1.000000000000000000, 0.8660254037844387076, 1.000000000000000000, 0.8660254037844387076, 1.000000000000000000, 0.9330127018922194093, 0.9330127018922194093 ) ) 
 REPRESENTATION_ITEM ( '' )  );
#77094=CARTESIAN_POINT ( 'NONE',  ( 77.57756690181206238, 204.0494855054051868, -2.679491924311248496 ) ) ;
#77095=CARTESIAN_POINT ( 'NONE',  ( 147.7870527676176948, 274.6723112360602386, 9.257357958194809555 ) ) ;
#77096=CARTESIAN_POINT ( 'NONE',  ( 148.9517569034208009, 272.6549844970639924, 12.50737104496728236 ) ) ;
#77097=CARTESIAN_POINT ( 'NONE',  ( 173.0421597889786369, 276.4496783815933441, -15.69011261309027638 ) ) ;
#77098=CARTESIAN_POINT ( 'NONE',  ( 147.3026092797766182, 275.5113919703970851, -0.02371565180376775453 ) ) ;
#77099=CARTESIAN_POINT ( 'NONE',  ( 147.1034852426517148, 275.8562849197056153, -3.648177088342072327 ) ) ;
#77107=CARTESIAN_POINT ( 'NONE',  ( 149.7004146199789147, 271.3582712945064941, -12.74589670383119433 ) ) ;
#77111=CARTESIAN_POINT ( 'NONE',  ( 180.6066648745947134, 283.7006809008031496, -16.18202752516933174 ) ) ;
#77113=CARTESIAN_POINT ( 'NONE',  ( 168.7558045253416310, 286.1749812365729326, -7.730637050109386621 ) ) ;
#77115=CARTESIAN_POINT ( 'NONE',  ( 163.1369207721744772, 248.0855599626920593, -11.24692769914530110 ) ) ;
#77116=B_SPLINE_CURVE_WITH_KNOTS ( 'NONE', 3,
 ( #5809, #34710, #35713, #59485, #66612, #80878, #26626, #44298, #74742, #82370, #96564, #51407, #98028, #90467 ),
 .UNSPECIFIED., .F., .F.,
 ( 4, 2, 2, 2, 2, 2, 4 ),
 ( 0.0002339632422484184916, 0.0009086598472604706872, 0.001246008149766496785, 0.001414682301019510972, 0.001499019376646056230, 0.001541187914459328859, 0.001583356452272601488 ),
 .UNSPECIFIED. ) ;
#77118=CARTESIAN_POINT ( 'NONE',  ( 39.33606980327277824, 193.5177522451418781, -10.00000000000009592 ) ) ;
#77119=CARTESIAN_POINT ( 'NONE',  ( 130.8370663736463655, 246.3458772461660544, 9.188101187500095079 ) ) ;
#77120=CARTESIAN_POINT ( 'NONE',  ( 180.3598775736073776, 294.8113545327539669, -3.562513127318830186 ) ) ;
#77121=CARTESIAN_POINT ( 'NONE',  ( 108.6384560342674064, 221.9824982072973967, 3.021315404115420679E-15 ) ) ;
#77122=CARTESIAN_POINT ( 'NONE',  ( 157.3363371328520088, 258.1324655395517311, 18.24585617226787093 ) ) ;
#77124=CARTESIAN_POINT ( 'NONE',  ( 54.03161192339643293, 195.8768266524159856, -9.188101187500091527 ) ) ;
#77126=CARTESIAN_POINT ( 'NONE',  ( 178.7926337964088361, 291.8428451618758572, -5.965102354984807675 ) ) ;
#77132=B_SPLINE_SURFACE_WITH_KNOTS ( 'NONE', 3, 1, ( 
 ( #5127, #97351 ),
 ( #27915, #12237 ),
 ( #73537, #42118 ),
 ( #3644, #96367 ),
 ( #4119, #35014 ),
 ( #43096, #74038 ),
 ( #65914, #82171 ),
 ( #74550, #35521 ),
 ( #96871, #58314 ),
 ( #4627, #58799 ),
 ( #12747, #36008 ),
 ( #53691, #67918 ),
 ( #30409, #59802 ),
 ( #60288, #28929 ),
 ( #6113, #76999 ),
 ( #83658, #92262 ),
 ( #98838, #5616 ),
 ( #51733, #60781 ),
 ( #7607, #84647 ),
 ( #22811, #61300 ),
 ( #37008, #69411 ),
 ( #22308, #38494 ),
 ( #91747, #29419 ),
 ( #45594, #91248 ),
 ( #83151, #21811 ),
 ( #90772, #76523 ),
 ( #15189, #46088 ),
 ( #52697, #22 ),
 ( #59289, #13241 ),
 ( #52201, #53211 ),
 ( #14710, #99331 ),
 ( #90268, #44593 ),
 ( #20841, #82675 ),
 ( #21322, #44095 ) ),
 .UNSPECIFIED., .T., .F., .F.,
 ( 4, 2, 2, 2, 2, 2, 2, 2, 2, 2, 2, 2, 2, 2, 2, 2, 4 ),
 ( 2, 2 ),
 ( 0.000000000000000000, 0.06250000000000000000, 0.1250000000000000000, 0.1875000000000000000, 0.2500000000000000000, 0.3125000000000000000, 0.3750000000000000000, 0.4375000000000000000, 0.5000000000000000000, 0.5625000000000000000, 0.6250000000000000000, 0.6875000000000000000, 0.7500000000000000000, 0.8125000000000000000, 0.8750000000000000000, 0.9375000000000000000, 1.000000000000000000 ),
 ( 0.000000000000000000, 1.000000000000000000 ),
 .UNSPECIFIED. ) ;
#77137=CARTESIAN_POINT ( 'NONE',  ( 206.9985020284622408, 270.1150727264914053, 3.388313042214953441 ) ) ;
#77138=CARTESIAN_POINT ( 'NONE',  ( 16.02555268474166539, 173.3927522451417929, -10.00000000000009237 ) ) ;
#77139=CARTESIAN_POINT ( 'NONE',  ( 101.6898988757523625, 229.5177522451418781, -10.00000000000009592 ) ) ;
#77142=B_SPLINE_CURVE_WITH_KNOTS ( 'NONE', 3,
 ( #34162, #49851, #57945, #65054 ),
 .UNSPECIFIED., .F., .F.,
 ( 4, 4 ),
 ( 0.02967357326668309050, 0.03879524988894693383 ),
 .UNSPECIFIED. ) ;
#77144=CARTESIAN_POINT ( 'NONE',  ( 189.8314329296643450, 301.8493086226544619, -0.8085564604676659384 ) ) ;
#77145=CARTESIAN_POINT ( 'NONE',  ( 153.9562949345533980, 264.3674845922398049, 16.52332238502633288 ) ) ;
#77147=CARTESIAN_POINT ( 'NONE',  ( 28.53781555160951555, 187.2833772461660544, -9.188101187500095079 ) ) ;
#77150=CARTESIAN_POINT ( 'NONE',  ( 192.1381319048448972, 272.2822842022381451, 14.66302914414172776 ) ) ;
#77151=CARTESIAN_POINT ( 'NONE',  ( 32.93109025799825673, 196.4865022471903160, -10.00000000000009592 ) ) ;
#77154=CARTESIAN_POINT ( 'NONE',  ( 194.9277292273816329, 275.2606802342018568, -15.65310477115430032 ) ) ;
#77155=CARTESIAN_POINT ( 'NONE',  ( 76.25066296318219372, 205.6423013555409796, -4.594050593750043987 ) ) ;
#77156=CARTESIAN_POINT ( 'NONE',  ( 200.3765029811139584, 283.5847115241710981, 16.85207472104531590 ) ) ;
#77163=EDGE_CURVE ( 'NONE', #79381, #25119, #35340, .T. ) ;
#77164=CARTESIAN_POINT ( 'NONE',  ( 26.50806851326369440, 186.1115022471902591, 10.00000000000009592 ) ) ;
#77165=CARTESIAN_POINT ( 'NONE',  ( 163.7587049410067266, 247.0085981909329576, -6.137518685179130351 ) ) ;
#77166=CARTESIAN_POINT ( 'NONE',  ( -12.05712525078605069, 163.8458772461660544, 9.188101187500095079 ) ) ;
#77168=CARTESIAN_POINT ( 'NONE',  ( 185.2932492178748873, 260.3554632076975963, 6.449134693235576421 ) ) ;
#77169=CARTESIAN_POINT ( 'NONE',  ( 164.7297297678022403, 245.3267338555121455, 3.020078936458732599 ) ) ;
#77175=CARTESIAN_POINT ( 'NONE',  ( 177.8222571804544430, 286.5223583772871621, 13.77940225188420875 ) ) ;
#77176=CARTESIAN_POINT ( 'NONE',  ( 156.0333632674501700, 279.4506186462613755, -5.256414494794261927 ) ) ;
#77179=CARTESIAN_POINT ( 'NONE',  ( 206.7942001012778235, 272.4689340444584786, 9.528356049623848634 ) ) ;
#77181=CARTESIAN_POINT ( 'NONE',  ( 204.9463377925012253, 275.6695254486514841, -14.15865086131798378 ) ) ;
#77182=CARTESIAN_POINT ( 'NONE',  ( 148.7536333930846979, 273.6080040564672231, -8.868003689723101601 ) ) ;
#77185=CARTESIAN_POINT ( 'NONE',  ( 162.8480293090835005, 248.5859346546387769, -9.753154585358942086 ) ) ;
#77186=CARTESIAN_POINT ( 'NONE',  ( 201.0732166862245549, 282.3779679885897167, -18.18766936363638820 ) ) ;
#77187=ORIENTED_EDGE ( 'NONE', *, *, #28573, .T. ) ;
#77190=CARTESIAN_POINT ( 'NONE',  ( 190.6023296602558901, 281.3493246229567717, 16.84671144084375172 ) ) ;
#77193=CARTESIAN_POINT ( 'NONE',  ( 149.1903793729515257, 272.2416782560088677, 12.95958987445043675 ) ) ;
#77197=CARTESIAN_POINT ( 'NONE',  ( 191.2211340522693774, 299.4422756709672626, -8.405362570633277741 ) ) ;
#77205=CARTESIAN_POINT ( 'NONE',  ( 97.73839765093606502, 236.4244531367911009, -4.594050593750046652 ) ) ;
#77206=CARTESIAN_POINT ( 'NONE',  ( 155.7553667887436859, 260.8707865008068438, 18.13952515356204032 ) ) ;
#77209=CARTESIAN_POINT ( 'NONE',  ( 191.0170959869219303, 299.7956799668270946, 7.353346939903929069 ) ) ;
#77212=ADVANCED_FACE ( 'NONE', ( #44990 ), #21220, .T. ) ;
#77214=ORIENTED_EDGE ( 'NONE', *, *, #97028, .F. ) ;
#77216=ORIENTED_EDGE ( 'NONE', *, *, #14840, .F. ) ;
#77217=CARTESIAN_POINT ( 'NONE',  ( 160.0499875548515263, 257.7887348395778986, -17.19135428511508579 ) ) ;
#77219=CARTESIAN_POINT ( 'NONE',  ( 208.2777459429579210, 269.8993572713111462, 3.129643751043610589 ) ) ;
#77222=CARTESIAN_POINT ( 'NONE',  ( 171.0295563763983751, 283.5921888939291193, 12.22847014256639042 ) ) ;
#77223=CARTESIAN_POINT ( 'NONE',  ( 194.2900850603946310, 294.1266965989547657, -15.88613936555681505 ) ) ;
#77227=DIRECTION ( 'NONE',  ( -0.8660254037844387076, -0.4999999999999998890, -0.000000000000000000 ) ) ;
#77229=CARTESIAN_POINT ( 'NONE',  ( 200.2093391412865060, 269.7417714514684803, 10.46510648850140157 ) ) ;
#77231=AXIS2_PLACEMENT_3D ( 'NONE', #28276, #13106, #35381 ) ;
#77232=CARTESIAN_POINT ( 'NONE',  ( 170.6243390796742858, 258.8588259563213683, -13.92090666709099622 ) ) ;
#77233=CARTESIAN_POINT ( 'NONE',  ( 206.8313602288537538, 272.4045708154811791, -9.607337080360906612 ) ) ;
#77237=CARTESIAN_POINT ( 'NONE',  ( 171.9118178377493109, 254.7376308715724633, 11.11564670839499769 ) ) ;
#77238=CARTESIAN_POINT ( 'NONE',  ( 157.9648847355622650, 281.0502099387495605, 1.885049730135211821 ) ) ;
#77240=CARTESIAN_POINT ( 'NONE',  ( 155.6699570996827617, 261.0187204217189674, -17.22644539015238863 ) ) ;
#77241=AXIS2_PLACEMENT_3D ( 'NONE', #56859, #18892, #95924 ) ;
#77244=ADVANCED_FACE ( 'NONE', ( #97245 ), #27811, .T. ) ;
#77245=CARTESIAN_POINT ( 'NONE',  ( 10.82940026203503336, 170.3927522451418213, -10.00000000000009059 ) ) ;
#77246=CARTESIAN_POINT ( 'NONE',  ( 93.16496130902324069, 224.5958772461660260, -9.188101187500095079 ) ) ;
#77247=CARTESIAN_POINT ( 'NONE',  ( 192.8095291656202619, 267.1346876124251253, -11.12116723929773698 ) ) ;
#77249=CARTESIAN_POINT ( 'NONE',  ( 203.4661181658017597, 278.2333410484554861, -14.92553451795532204 ) ) ;
#77251=CARTESIAN_POINT ( 'NONE',  ( 11.32556065139379875, 177.3458772461660544, 9.188101187500095079 ) ) ;
#77253=CARTESIAN_POINT ( 'NONE',  ( 161.8948331661419218, 250.2369188037922356, 13.64419044796309777 ) ) ;
#77254=EDGE_LOOP ( 'NONE', ( #97987, #3461, #18428, #12046 ) ) ;
#77256=CARTESIAN_POINT ( 'NONE',  ( 161.3981413584396876, 253.0972142504356270, -15.11937522241654719 ) ) ;
#77257=CARTESIAN_POINT ( 'NONE',  ( 198.2712628870943661, 265.0502820922010869, -3.032086182221595649 ) ) ;
#77259=CARTESIAN_POINT ( 'NONE',  ( 205.2660270307054304, 275.1158074454486382, -13.97598661256119179 ) ) ;
#77262=CARTESIAN_POINT ( 'NONE',  ( 149.6449510338218829, 277.3920198197748164, 3.114130954607317925 ) ) ;
#77263=CARTESIAN_POINT ( 'NONE',  ( 15.54743449484293372, 179.7833772461660544, -9.188101187500095079 ) ) ;
#77264=CARTESIAN_POINT ( 'NONE',  ( 114.1117772151768577, 242.8149278399161233, -9.188101187500095079 ) ) ;
#77265=CARTESIAN_POINT ( 'NONE',  ( 181.9627339888420465, 294.6573541485591932, -6.516454160791068873 ) ) ;
#77266=CARTESIAN_POINT ( 'NONE',  ( 183.1055844247790958, 257.7654091154714706, -2.368402100318311110 ) ) ;
#77268=CARTESIAN_POINT ( 'NONE',  ( 153.2819058590468160, 274.2512448977743134, -12.24885634829186287 ) ) ;
#77270=CARTESIAN_POINT ( 'NONE',  ( 151.7685526703961614, 270.8433852370800423, 14.21420454866266248 ) ) ;
#77271=CARTESIAN_POINT ( 'NONE',  ( 157.3988263959001870, 258.0242309610243865, 16.72376558639979294 ) ) ;
#77273=CARTESIAN_POINT ( 'NONE',  ( 155.0197698005585494, 262.1448778582381465, 18.42918111182112284 ) ) ;
#77274=CARTESIAN_POINT ( 'NONE',  ( 161.0974665087481981, 251.6179983666593216, -13.69252715295363210 ) ) ;
#77275=CARTESIAN_POINT ( 'NONE',  ( 189.4308808934198680, 289.8491723414206831, 15.72891001903047048 ) ) ;
#77276=CARTESIAN_POINT ( 'NONE',  ( 147.6264044922760377, 274.9505622111005323, -8.841872555777701592 ) ) ;
#77277=CARTESIAN_POINT ( 'NONE',  ( 189.3717192525180337, 262.4809367720384898, 8.181044353032417504 ) ) ;
#77278=CARTESIAN_POINT ( 'NONE',  ( 164.2214870300199152, 249.7080052763175217, -10.41861459481195595 ) ) ;
#77279=DIRECTION ( 'NONE',  ( -0.8660254037844387076, -0.4999999999999998890, -0.000000000000000000 ) ) ;
#77280=EDGE_CURVE ( 'NONE', #60835, #17038, #48631, .T. ) ;
#77282=CARTESIAN_POINT ( 'NONE',  ( 147.6618183892331331, 274.8892235422768522, 8.990680574201936892 ) ) ;
#77284=VERTEX_POINT ( 'NONE', #37880 ) ;
#77285=CARTESIAN_POINT ( 'NONE',  ( 152.3599525993681709, 267.1668075756145981, -15.39918555524012334 ) ) ;
#77286=ADVANCED_FACE ( 'NONE', ( #84053 ), #31266, .F. ) ;
#77288=CARTESIAN_POINT ( 'NONE',  ( 185.1220358696202481, 269.6591034785776628, 15.69820767156324770 ) ) ;
#77289=ADVANCED_FACE ( 'NONE', ( #65198 ), #55576, .T. ) ;
#77291=CARTESIAN_POINT ( 'NONE',  ( 94.43719644265542001, 216.1423013555410080, -4.594050593750043987 ) ) ;
#77293=CARTESIAN_POINT ( 'NONE',  ( 150.6571681785161445, 269.7011255207979730, 15.24894850018880454 ) ) ;
#77295=VECTOR ( 'NONE', #82728, 1000.000000000000000 ) ;
#77296=CARTESIAN_POINT ( 'NONE',  ( 145.1275483969982645, 243.0494855054051584, -2.679491924311248496 ) ) ;
#77297=CARTESIAN_POINT ( 'NONE',  ( 195.2484836900998175, 279.0356495040737173, 16.29341914179182282 ) ) ;
#77298=CARTESIAN_POINT ( 'NONE',  ( 176.6943099527350682, 256.7931168052207340, -11.17617521364210731 ) ) ;
#77301=CARTESIAN_POINT ( 'NONE',  ( 47.72569090598240393, 208.3615022471902876, 5.000000000000046185 ) ) ;
#77305=CARTESIAN_POINT ( 'NONE',  ( 192.4264036352439575, 266.3794008020136630, 11.60644757818683637 ) ) ;
#77310=CARTESIAN_POINT ( 'NONE',  ( 153.1548001820517868, 274.9824320604590184, 10.64421219061565793 ) ) ;
#77312=CARTESIAN_POINT ( 'NONE',  ( 190.6688270659779221, 284.0946164064107506, -17.60360843008351495 ) ) ;
#77315=CARTESIAN_POINT ( 'NONE',  ( 192.0331311261993790, 298.0358554833232461, 11.82583305898340953 ) ) ;
#77317=ORIENTED_EDGE ( 'NONE', *, *, #98920, .F. ) ;
#77318=EDGE_CURVE ( 'NONE', #47320, #99135, #71609, .T. ) ;
#77322=CARTESIAN_POINT ( 'NONE',  ( 165.1852812139168520, 248.1429326983447652, 7.096218362256309753 ) ) ;
#77324=VERTEX_POINT ( 'NONE', #40874 ) ;
#77326=CARTESIAN_POINT ( 'NONE',  ( 159.0577544183932446, 255.1508833399667253, 16.37810164263070334 ) ) ;
#77328=CARTESIAN_POINT ( 'NONE',  ( 153.4436003264302144, 264.8748834687675071, -16.72600001480972765 ) ) ;
#77333=B_SPLINE_CURVE_WITH_KNOTS ( 'NONE', 3,
 ( #27138, #26133, #58023, #56519 ),
 .UNSPECIFIED., .F., .F.,
 ( 4, 4 ),
 ( 0.008310172455301832045, 0.01464027962821165887 ),
 .UNSPECIFIED. ) ;
#77335=DIRECTION ( 'NONE',  ( -0.8660254037844387076, -0.4999999999999998890, -0.000000000000000000 ) ) ;
#77336=ORIENTED_EDGE ( 'NONE', *, *, #5156, .F. ) ;
#77337=VERTEX_POINT ( 'NONE', #41384 ) ;
#77339=ORIENTED_EDGE ( 'NONE', *, *, #52208, .F. ) ;
#77342=CARTESIAN_POINT ( 'NONE',  ( 154.9032082715209810, 280.6326124547101699, -2.389722542998433230 ) ) ;
#77346=B_SPLINE_CURVE_WITH_KNOTS ( 'NONE', 3,
 ( #1557, #47128, #78051, #39509, #63338, #63835, #55705, #79080, #40523, #71458, #94773, #42516, #65819, #4034 ),
 .UNSPECIFIED., .F., .F.,
 ( 4, 2, 2, 2, 2, 2, 4 ),
 ( 0.001312137252800617574, 0.001526837886047112489, 0.001741538519293607404, 0.001956239152540102319, 0.002170939785786597017, 0.002600341052279644960, 0.003029742318772693337 ),
 .UNSPECIFIED. ) ;
#77347=CARTESIAN_POINT ( 'NONE',  ( 167.6777283665894629, 249.2378510193953502, -5.459661846318103251 ) ) ;
#77348=CARTESIAN_POINT ( 'NONE',  ( 54.65389413625798909, 192.3615022471901739, 5.000000000000051514 ) ) ;
#77349=CARTESIAN_POINT ( 'NONE',  ( 183.5065578787086622, 284.7368108013639016, -15.01251262284198162 ) ) ;
#77350=CARTESIAN_POINT ( 'NONE',  ( 112.6505328941731108, 235.8458772461660544, 9.188101187500095079 ) ) ;
#77351=CARTESIAN_POINT ( 'NONE',  ( 183.5457472072443750, 260.5072762062756055, -9.285272734760553703 ) ) ;
#77353=CARTESIAN_POINT ( 'NONE',  ( 177.3471610734995068, 288.7557762509717350, -9.520805881307069285 ) ) ;
#77361=CARTESIAN_POINT ( 'NONE',  ( 164.4854433269806577, 246.2060377238486808, -1.879056492287135116 ) ) ;
#77362=CARTESIAN_POINT ( 'NONE',  ( 157.2744851780909414, 258.2395962677452985, 18.17792129701959070 ) ) ;
#77364=CARTESIAN_POINT ( 'NONE',  ( 152.7691010214056462, 266.0431505347400503, -16.40662330462167162 ) ) ;
#77365=CARTESIAN_POINT ( 'NONE',  ( 177.1970037392277391, 288.7997655633063232, -9.298457205910423795 ) ) ;
#77368=CARTESIAN_POINT ( 'NONE',  ( 175.4537718564577631, 254.8713487546767169, -7.339328112761260847 ) ) ;
#77371=CARTESIAN_POINT ( 'NONE',  ( 194.9636675848471441, 292.9600174435121289, -15.57898232594655319 ) ) ;
#77375=CARTESIAN_POINT ( 'NONE',  ( 191.8392821121727536, 267.5768712655535637, -12.56012087630908169 ) ) ;
#77377=CARTESIAN_POINT ( 'NONE',  ( 190.9710483804310854, 283.5610905854780981, -16.58407571954575488 ) ) ;
#77378=CARTESIAN_POINT ( 'NONE',  ( 192.4246011695004768, 262.9676472730263868, 4.544249788418587954 ) ) ;
#77381=CARTESIAN_POINT ( 'NONE',  ( 184.5344485499420273, 288.9945769638181901, -13.19104496679712213 ) ) ;
#77382=CARTESIAN_POINT ( 'NONE',  ( 157.3376867920517554, 280.1474045426916177, 5.786264004936231942 ) ) ;
#77383=CARTESIAN_POINT ( 'NONE',  ( 201.0468719883840265, 282.4235983437597497, -16.59631526626950659 ) ) ;
#77385=CARTESIAN_POINT ( 'NONE',  ( 190.9586609929293104, 299.8968923453624598, -4.970176667899034229 ) ) ;
#77386=B_SPLINE_SURFACE_WITH_KNOTS ( 'NONE', 3, 1, ( 
 ( #88445, #80840 ),
 ( #58460, #27091 ),
 ( #87951, #42262 ),
 ( #96521, #26591 ),
 ( #11896, #50371 ),
 ( #33183, #72204 ),
 ( #27596, #35169 ),
 ( #3306, #80324 ),
 ( #89434, #33697 ),
 ( #95027, #19987 ),
 ( #56476, #34186 ),
 ( #17997, #96029 ),
 ( #57464, #73197 ),
 ( #50867, #48891 ),
 ( #64590, #64082 ),
 ( #42753, #57974 ),
 ( #88958, #18495 ),
 ( #10894, #79825 ),
 ( #10393, #4271 ),
 ( #41770, #19004 ),
 ( #41261, #66080 ),
 ( #3791, #97026 ),
 ( #2809, #95543 ),
 ( #49381, #26090 ),
 ( #6267, #98494 ),
 ( #43757, #82819 ),
 ( #45743, #60950 ),
 ( #53359, #58941 ),
 ( #12901, #90922 ),
 ( #75681, #5766 ),
 ( #20999, #97500 ),
 ( #36655, #75191 ),
 ( #66574, #67562 ),
 ( #29086, #21472 ) ),
 .UNSPECIFIED., .T., .F., .F.,
 ( 4, 2, 2, 2, 2, 2, 2, 2, 2, 2, 2, 2, 2, 2, 2, 2, 4 ),
 ( 2, 2 ),
 ( 0.000000000000000000, 0.06250000000000000000, 0.1250000000000000000, 0.1875000000000000000, 0.2500000000000000000, 0.3125000000000000000, 0.3750000000000000000, 0.4375000000000000000, 0.5000000000000000000, 0.5625000000000000000, 0.6250000000000000000, 0.6875000000000000000, 0.7500000000000000000, 0.8125000000000000000, 0.8750000000000000000, 0.9375000000000000000, 1.000000000000000000 ),
 ( 0.000000000000000000, 1.000000000000000000 ),
 .UNSPECIFIED. ) ;
#77387=CARTESIAN_POINT ( 'NONE',  ( 168.3509053677366296, 264.6512997888990526, -17.59019591919307146 ) ) ;
#77388=CARTESIAN_POINT ( 'NONE',  ( 187.0383423799210902, 262.1832919597250111, -8.674447465982201066 ) ) ;
#77389=CARTESIAN_POINT ( 'NONE',  ( 182.6565686206717771, 276.0795042466008908, -16.45052173798808326 ) ) ;
#77391=CARTESIAN_POINT ( 'NONE',  ( 192.8314823969449492, 271.7167918609114849, -14.83780806620786485 ) ) ;
#77394=CARTESIAN_POINT ( 'NONE',  ( 188.0775634319173832, 267.1413101313072502, 14.31780989748781252 ) ) ;
#77395=CARTESIAN_POINT ( 'NONE',  ( 155.0929244053699847, 262.0181703658971628, 18.51426604808664678 ) ) ;
#77396=CARTESIAN_POINT ( 'NONE',  ( 192.6881117187585062, 284.3071375317443881, -16.71636262633107606 ) ) ;
#77398=CARTESIAN_POINT ( 'NONE',  ( 78.09096694622414248, 206.7048013555409796, 4.594050593750051981 ) ) ;
#77400=CARTESIAN_POINT ( 'NONE',  ( 147.3236643320416022, 275.4749235501183193, -5.185334239426818037 ) ) ;
#77401=CARTESIAN_POINT ( 'NONE',  ( 60.62040048720410823, 194.2592609112380160, 2.679491924311254714 ) ) ;
#77402=CARTESIAN_POINT ( 'NONE',  ( 203.0498946958275326, 278.9542612457532869, -15.11479947333269003 ) ) ;
#77405=CARTESIAN_POINT ( 'NONE',  ( 161.0974665087481981, 251.6179983666593216, -13.69252715295363210 ) ) ;
#77407=DIRECTION ( 'NONE',  ( -0.8660254037844387076, -0.4999999999999998890, -0.000000000000000000 ) ) ;
#77410=CARTESIAN_POINT ( 'NONE',  ( 168.9707749765159690, 251.9125659635931243, -8.781273530211780809 ) ) ;
#77411=CARTESIAN_POINT ( 'NONE',  ( 161.3691267615756431, 251.8145564780636221, 13.54285799199859675 ) ) ;
#77414=CARTESIAN_POINT ( 'NONE',  ( 157.5042325173297684, 257.8416622032797818, 16.70595240278738203 ) ) ;
#77418=CARTESIAN_POINT ( 'NONE',  ( 33.73396797431614402, 190.2833772461660544, -9.188101187500095079 ) ) ;
#77421=CARTESIAN_POINT ( 'NONE',  ( 61.28457468009112574, 200.0643266524160424, 9.188101187500095079 ) ) ;
#77422=CARTESIAN_POINT ( 'NONE',  ( 180.6161154953664152, 256.8960555319623609, 8.355174764559180289 ) ) ;
#77425=CARTESIAN_POINT ( 'NONE',  ( 96.20275958967147290, 237.8967562850346837, -4.648177544792955347E-16 ) ) ;
#77426=CARTESIAN_POINT ( 'NONE',  ( -13.83428154636143503, 169.4865022471903160, -10.00000000000009415 ) ) ;
#77429=CARTESIAN_POINT ( 'NONE',  ( 198.9154154329768573, 270.8075422652725024, -11.00997099090270481 ) ) ;
#77431=CARTESIAN_POINT ( 'NONE',  ( 198.7136873185829984, 286.4647927352960437, -18.57144721070432070 ) ) ;
#77434=CARTESIAN_POINT ( 'NONE',  ( 62.15025298811053744, 212.8149278399160949, -9.188101187500095079 ) ) ;
#77437=AXIS2_PLACEMENT_3D ( 'NONE', #92323, #60853, #61366 ) ;
#77438=CARTESIAN_POINT ( 'NONE',  ( 159.7953104873542145, 253.8733987550956783, 15.41928249285404107 ) ) ;
#77439=CARTESIAN_POINT ( 'NONE',  ( 58.38862868653046689, 194.5177522451417929, 5.000000000000051514 ) ) ;
#77440=CARTESIAN_POINT ( 'NONE',  ( 153.2550847801022087, 276.9870336669021640, 8.088704299435450551 ) ) ;
#77442=CIRCLE ( 'NONE', #37002, 17.82106496071138935 ) ;
#77444=CARTESIAN_POINT ( 'NONE',  ( 119.6057994200909036, 229.8615022471901739, 5.000000000000051514 ) ) ;
#77445=CARTESIAN_POINT ( 'NONE',  ( 161.5431944097339851, 250.8459749958011287, 14.52339846942414603 ) ) ;
#77446=CARTESIAN_POINT ( 'NONE',  ( 207.3062152119541679, 271.5820978585240368, 7.879821064966149535 ) ) ;
#77451=CARTESIAN_POINT ( 'NONE',  ( 159.3451320108506764, 254.6531307488737355, -16.72997986213134425 ) ) ;
#77452=CARTESIAN_POINT ( 'NONE',  ( 194.2091819726834103, 293.8763763881810291, 14.13354809719834826 ) ) ;
#77454=ORIENTED_EDGE ( 'NONE', *, *, #19445, .F. ) ;
#77455=CARTESIAN_POINT ( 'NONE',  ( 173.2985268944221104, 251.6510046717872910, -0.07099267305675936723 ) ) ;
#77458=CARTESIAN_POINT ( 'NONE',  ( 147.9791529310278122, 274.3395839928920168, -7.789432462804474433 ) ) ;
#77460=AXIS2_PLACEMENT_3D ( 'NONE', #71941, #62816, #63323 ) ;
#77469=CARTESIAN_POINT ( 'NONE',  ( 159.9647205790309101, 253.5799718689968927, -16.48298384325780219 ) ) ;
#77471=CARTESIAN_POINT ( 'NONE',  ( 174.7250473363198751, 286.2220955514192156, 10.55014635880517559 ) ) ;
#77473=CARTESIAN_POINT ( 'NONE',  ( 207.6163508138795635, 271.0449272387537576, -1.385071889578343152 ) ) ;
#77474=CARTESIAN_POINT ( 'NONE',  ( 163.9704062730716032, 246.6419207277664327, 7.317582738093436845 ) ) ;
#77475=CARTESIAN_POINT ( 'NONE',  ( 185.4517836755765643, 292.6420132580468589, -10.71622804994104605 ) ) ;
#77476=FACE_OUTER_BOUND ( 'NONE', #54650, .T. ) ;
#77477=CARTESIAN_POINT ( 'NONE',  ( 144.1522069568320887, 254.0333772461660260, 9.188101187500095079 ) ) ;
#77479=CARTESIAN_POINT ( 'NONE',  ( 178.7522638060953852, 257.9681842698315108, 9.852045485592459073 ) ) ;
#77480=CARTESIAN_POINT ( 'NONE',  ( 80.68904315757745849, 208.2048013555409796, 4.594050593750051981 ) ) ;
#77481=ORIENTED_EDGE ( 'NONE', *, *, #14715, .T. ) ;
#77482=B_SPLINE_CURVE_WITH_KNOTS ( 'NONE', 3,
 ( #776, #31662, #85431, #93520 ),
 .UNSPECIFIED., .F., .F.,
 ( 4, 4 ),
 ( 0.003345072186823920199, 0.01130424824522063658 ),
 .UNSPECIFIED. ) ;
#77483=CARTESIAN_POINT ( 'NONE',  ( 191.5281967176683509, 298.9104275333885994, 7.715154960566919407 ) ) ;
#77484=CARTESIAN_POINT ( 'NONE',  ( 185.7372650184451857, 257.4645284076796656, -2.264991511946413505E-12 ) ) ;
#77485=EDGE_CURVE ( 'NONE', #28084, #99896, #7513, .T. ) ;
#77491=CARTESIAN_POINT ( 'NONE',  ( 197.9324133593710542, 286.8504239745568043, 16.93537766679494894 ) ) ;
#77496=CARTESIAN_POINT ( 'NONE',  ( 82.55649720842890815, 206.2202760586659167, -5.415160957724236172E-17 ) ) ;
#77498=EDGE_CURVE ( 'NONE', #86016, #43672, #84894, .T. ) ;
#77501=CARTESIAN_POINT ( 'NONE',  ( 200.8466324750363299, 282.7704233545608190, -16.77580403217666927 ) ) ;
#77503=ADVANCED_FACE ( 'NONE', ( #41259 ), #79076, .F. ) ;
#77505=CARTESIAN_POINT ( 'NONE',  ( 183.6917392022668309, 275.6525662950718356, 17.55237957418163930 ) ) ;
#77507=CARTESIAN_POINT ( 'NONE',  ( 205.8030308266901898, 274.1856895869457844, 10.55961490432110317 ) ) ;
#77508=CARTESIAN_POINT ( 'NONE',  ( 206.8711744556208885, 269.6661967102621702, -5.660351959544826712E-12 ) ) ;
#77509=CARTESIAN_POINT ( 'NONE',  ( 207.1061707122464099, 270.1598718182783614, -2.616480830523119305 ) ) ;
#77514=CARTESIAN_POINT ( 'NONE',  ( 185.3548632422784976, 260.1969484205714025, 6.113967884209870363 ) ) ;
#77516=CARTESIAN_POINT ( 'NONE',  ( 200.6737073311291795, 283.0699384897140476, -17.61533935526990291 ) ) ;
#77519=ORIENTED_EDGE ( 'NONE', *, *, #61638, .T. ) ;
#77520=CARTESIAN_POINT ( 'NONE',  ( 185.1491161497484370, 292.9437783688060222, -11.97406807593424993 ) ) ;
#77524=CARTESIAN_POINT ( 'NONE',  ( 171.3649617487770911, 251.0102673366500596, 7.372720983288576946 ) ) ;
#77528=CARTESIAN_POINT ( 'NONE',  ( 202.7041331321765938, 279.5531378413010657, 17.14708438049711248 ) ) ;
#77529=CARTESIAN_POINT ( 'NONE',  ( 40.18174127881769664, 205.5530062829863027, -4.648177544792955347E-16 ) ) ;
#77532=CARTESIAN_POINT ( 'NONE',  ( 176.1242821188019718, 285.3583729749952909, -12.07621089340971920 ) ) ;
#77535=B_SPLINE_CURVE_WITH_KNOTS ( 'NONE', 3,
 ( #23708, #54602, #85586, #16127 ),
 .UNSPECIFIED., .F., .F.,
 ( 4, 4 ),
 ( 0.01081206089262459064, 0.01921137274017016561 ),
 .UNSPECIFIED. ) ;
#77538=CARTESIAN_POINT ( 'NONE',  ( 188.2526772805193502, 260.8404435756410180, 2.927908703176840266 ) ) ;
#77539=CARTESIAN_POINT ( 'NONE',  ( 139.3620039403753879, 261.2677522451419350, -5.000000000000047962 ) ) ;
#77540=CARTESIAN_POINT ( 'NONE',  ( 190.2505983465532324, 296.1737925351780518, -11.69656242540844282 ) ) ;
#77544=CARTESIAN_POINT ( 'NONE',  ( 178.5588389885454319, 256.8987037950940362, 8.463150697600209327 ) ) ;
#77547=CARTESIAN_POINT ( 'NONE',  ( 19.11978928545374501, 181.8458772461660544, 9.188101187500095079 ) ) ;
#77548=CARTESIAN_POINT ( 'NONE',  ( 181.9657388339318231, 275.7813954516299191, -16.43665191748776877 ) ) ;
#77551=CARTESIAN_POINT ( 'NONE',  ( 171.0406735725552210, 271.3140026262360607, -17.70316094230177129 ) ) ;
#77553=B_SPLINE_CURVE_WITH_KNOTS ( 'NONE', 3,
 ( #43007, #90175, #20245, #75959 ),
 .UNSPECIFIED., .F., .F.,
 ( 4, 4 ),
 ( 0.03513230373696424325, 0.04390280448137185570 ),
 .UNSPECIFIED. ) ;
#77555=CARTESIAN_POINT ( 'NONE',  ( 187.6663016716853747, 259.1672013800106242, -0.7921523300642274723 ) ) ;
#77556=CARTESIAN_POINT ( 'NONE',  ( 72.84042761573121538, 202.8615022471901739, 5.000000000000051514 ) ) ;
#77558=DIRECTION ( 'NONE',  ( -0.8660254037844387076, -0.4999999999999998890, -0.000000000000000000 ) ) ;
#77559=CARTESIAN_POINT ( 'NONE',  ( 25.10051690851626560, 194.4869531367911293, 4.594050593750046652 ) ) ;
#77563=CARTESIAN_POINT ( 'NONE',  ( 199.2299651681423143, 285.5705732690366858, -17.65328173313980642 ) ) ;
#77566=CARTESIAN_POINT ( 'NONE',  ( 6.176825452568912134, 162.8262482093457777, 3.021315404115420679E-15 ) ) ;
#77567=CARTESIAN_POINT ( 'NONE',  ( 162.2342503670216729, 281.0091534512037583, -10.48921805985605538 ) ) ;
#77568=CARTESIAN_POINT ( 'NONE',  ( 163.8712475794395118, 282.0753919168961374, 10.04803168266247582 ) ) ;
#77571=CARTESIAN_POINT ( 'NONE',  ( 190.3144310910409445, 301.0127312671879167, -1.334877248546042949 ) ) ;
#77573=CARTESIAN_POINT ( 'NONE',  ( 188.9238571764875871, 270.0808980012285474, -15.37208702597789234 ) ) ;
#77576=CARTESIAN_POINT ( 'NONE',  ( 185.4211012460235395, 291.0283491078289444, 13.34097488155738631 ) ) ;
#77581=VERTEX_POINT ( 'NONE', #27088 ) ;
#77584=B_SPLINE_CURVE_WITH_KNOTS ( 'NONE', 3,
 ( #63670, #17063, #55549, #64174, #55057, #85526, #25164, #31748, #8475, #9482, #47464, #32764, #93605, #79918, #16568, #71290, #56047, #95633, #87039, #32266, #86533, #2391, #10480, #72299, #33799, #33271, #9987, #78389, #8970, #24665, #87553, #18086, #39840, #64683, #70771, #63169, #94113, #47954, #48982, #78897, #94609, #41357, #2906, #26181, #16069, #46971, #72810, #65169, #35767, #58555 ),
 .UNSPECIFIED., .F., .F.,
 ( 4, 2, 2, 2, 2, 2, 2, 2, 2, 2, 2, 2, 2, 2, 2, 2, 2, 2, 2, 2, 2, 2, 2, 2, 4 ),
 ( 0.002964269280204859160, 0.003162640838911195268, 0.003361012397617531809, 0.003460198176970720896, 0.003559383956323909984, 0.003658569735677099071, 0.003757755515030288158, 0.004154498632443132111, 0.004551241749855975197, 0.005344727984681663102, 0.006138214219507351008, 0.006931700454333038913, 0.007725186689158725084, 0.007824372468511853890, 0.007873965358188416558, 0.007923558247864980961, 0.007973151137541543629, 0.008022744027218108032, 0.008121929806571235103, 0.008320301365277530878, 0.008518672923983824918, 0.008717044482690120694, 0.008915416041396416469, 0.009113787600102712244, 0.009312159158809008019 ),
 .UNSPECIFIED. ) ;
#77586=CARTESIAN_POINT ( 'NONE',  ( 173.8665542827094725, 250.6399523573830095, -0.9454928766311748722 ) ) ;
#77587=ORIENTED_EDGE ( 'NONE', *, *, #55901, .T. ) ;
#77588=AXIS2_PLACEMENT_3D ( 'NONE', #14079, #44965, #75904 ) ;
#77589=EDGE_LOOP ( 'NONE', ( #48198, #24097, #91455, #35574, #73037, #51934, #32618, #98259, #86489, #6781, #30744, #66393, #20043, #47562, #17523, #76714, #24799, #51719, #86293, #86372, #46662, #8052, #47795, #96584, #94449, #66054, #53649, #11148, #24251, #67645, #17019, #36107, #75988, #26772, #43902, #26632, #82383, #52332, #63845, #27892, #7894, #35182, #56008, #96609, #58625, #71371, #43831, #95101, #20461, #61615 ) ) ;
#77590=CARTESIAN_POINT ( 'NONE',  ( 189.4681065570641749, 274.0997382612658271, -15.65967126434479617 ) ) ;
#77593=FACE_OUTER_BOUND ( 'NONE', #48659, .T. ) ;
#77594=CARTESIAN_POINT ( 'NONE',  ( -27.42236680055714260, 166.5217562850347406, 1.224646799147364892E-15 ) ) ;
#77597=CARTESIAN_POINT ( 'NONE',  ( 148.3997536239841679, 273.6110822229926498, 8.713694244701960301 ) ) ;
#77598=CARTESIAN_POINT ( 'NONE',  ( 196.7491951525289835, 289.8673929779723721, -16.35352603081977207 ) ) ;
#77601=EDGE_CURVE ( 'NONE', #35992, #62993, #57044, .T. ) ;
#77603=CARTESIAN_POINT ( 'NONE',  ( 195.7578697689113199, 291.5844189092309193, 17.18796537138345215 ) ) ;
#77604=CARTESIAN_POINT ( 'NONE',  ( 208.3117541397001844, 269.8404533466799080, 2.895672523916592578 ) ) ;
#77605=EDGE_LOOP ( 'NONE', ( #17561, #36074, #38937 ) ) ;
#77607=CARTESIAN_POINT ( 'NONE',  ( 190.0550686570564949, 301.4619601804237732, 4.203010638620038542 ) ) ;
#77612=CARTESIAN_POINT ( 'NONE',  ( 150.6571681785161445, 269.7011255207979730, 15.24894850018880454 ) ) ;
#77614=LINE ( 'NONE', #8198, #99736 ) ;
#77617=CARTESIAN_POINT ( 'NONE',  ( 190.8131867350074060, 299.6564803534650423, 5.431438511040964201 ) ) ;
#77619=CARTESIAN_POINT ( 'NONE',  ( 190.6036479972031259, 300.5117928913073797, -0.6824572005520307405 ) ) ;
#77620=ORIENTED_EDGE ( 'NONE', *, *, #43812, .T. ) ;
#77621=CARTESIAN_POINT ( 'NONE',  ( 149.4539134692060145, 271.7852238117696402, 12.95627816374690688 ) ) ;
#77622=CARTESIAN_POINT ( 'NONE',  ( 157.3604748455635729, 259.8466937948429063, -17.62934668591135079 ) ) ;
#77624=DIRECTION ( 'NONE',  ( -0.8660254037844387076, -0.4999999999999998890, -0.000000000000000000 ) ) ;
#77625=CARTESIAN_POINT ( 'NONE',  ( 192.4259603496955719, 297.3554553095298729, -12.40738485318142814 ) ) ;
#77626=CARTESIAN_POINT ( 'NONE',  ( 160.0613924909338550, 255.6058025510563709, 16.19881800728115095 ) ) ;
#77628=CARTESIAN_POINT ( 'NONE',  ( 102.5355703512972809, 241.5530062829863027, -4.648177544792955347E-16 ) ) ;
#77632=CARTESIAN_POINT ( 'NONE',  ( 104.9102572999672276, 237.5024278399160949, 9.188101187500095079 ) ) ;
#77634=CARTESIAN_POINT ( 'NONE',  ( 191.4852287632733123, 298.9848502134979071, -9.870565261052552941 ) ) ;
#77638=CARTESIAN_POINT ( 'NONE',  ( 203.3349860717029571, 278.4604684979374838, -16.59553970625579566 ) ) ;
#77640=CARTESIAN_POINT ( 'NONE',  ( 183.2719456501309594, 284.6370414458698974, -14.99201719159501422 ) ) ;
#77642=CARTESIAN_POINT ( 'NONE',  ( 168.8758384829626209, 284.8846904623786713, -7.958113118064016334 ) ) ;
#77647=CARTESIAN_POINT ( 'NONE',  ( 135.2486435959970947, 239.7048013555409796, 4.594050593750051981 ) ) ;
#77648=CARTESIAN_POINT ( 'NONE',  ( 190.9583202594226918, 294.9585867271870256, -12.20043999232385978 ) ) ;
#77651=CARTESIAN_POINT ( 'NONE',  ( 157.6335212189247557, 257.6177276032722716, 16.76495363836117036 ) ) ;
#77653=CARTESIAN_POINT ( 'NONE',  ( 52.89478003304684250, 201.3458772461660260, 9.188101187500095079 ) ) ;
#77658=EDGE_CURVE ( 'NONE', #28879, #75738, #57876, .T. ) ;
#77660=CARTESIAN_POINT ( 'NONE',  ( 147.4963928429778264, 275.1757489932608109, 4.929816573182678852 ) ) ;
#77661=CARTESIAN_POINT ( 'NONE',  ( 151.3511865740561007, 278.6745403919405248, -1.693856907688049862 ) ) ;
#77662=CARTESIAN_POINT ( 'NONE',  ( 154.9792334219179679, 262.2150889255981951, -17.21325849938693153 ) ) ;
#77663=AXIS2_PLACEMENT_3D ( 'NONE', #13976, #29181, #69151 ) ;
#77664=CARTESIAN_POINT ( 'NONE',  ( 178.5084147955354297, 261.1889675471575174, 12.22496176922636835 ) ) ;
#77665=EDGE_CURVE ( 'NONE', #30031, #35626, #71576, .T. ) ;
#77666=CARTESIAN_POINT ( 'NONE',  ( 113.3812418268422846, 236.2677522451418497, 10.00000000000009592 ) ) ;
#77667=CARTESIAN_POINT ( 'NONE',  ( 169.3422351861262882, 267.3027105831644690, -17.79115954374443476 ) ) ;
#77670=CARTESIAN_POINT ( 'NONE',  ( 203.0535368433499457, 278.9479528611958585, 16.46202213522710167 ) ) ;
#77674=CARTESIAN_POINT ( 'NONE',  ( 36.16983797034238535, 185.5643266524159856, -9.188101187500093303 ) ) ;
#77676=DIRECTION ( 'NONE',  ( -0.8660254037844387076, -0.4999999999999998890, -0.000000000000000000 ) ) ;
#77677=FACE_OUTER_BOUND ( 'NONE', #60274, .T. ) ;
#77679=EDGE_CURVE ( 'NONE', #62642, #54504, #62957, .T. ) ;
#77680=CARTESIAN_POINT ( 'NONE',  ( 197.1856892100024652, 276.7320907554435507, -15.32951477734549961 ) ) ;
#77681=CARTESIAN_POINT ( 'NONE',  ( 65.93911412966747321, 215.0024278399160949, 9.188101187500095079 ) ) ;
#77683=CARTESIAN_POINT ( 'NONE',  ( 200.1103929410127762, 284.0456276340304953, 17.67835211026828901 ) ) ;
#77688=CARTESIAN_POINT ( 'NONE',  ( 25.28119919123577475, 178.7365022471902023, -10.00000000000009059 ) ) ;
#77689=CARTESIAN_POINT ( 'NONE',  ( 162.6937333994314656, 248.8531830095558632, 10.02305144031113926 ) ) ;
#77690=CARTESIAN_POINT ( 'NONE',  ( 152.7045549149684405, 246.7202760586659736, -5.415160957724236172E-17 ) ) ;
#77692=CARTESIAN_POINT ( 'NONE',  ( 164.0807478505496988, 260.5315732147755625, -16.15795033331652775 ) ) ;
#77693=CARTESIAN_POINT ( 'NONE',  ( 188.3128329290244665, 261.7237649635724779, 6.448241612589410643 ) ) ;
#77694=CARTESIAN_POINT ( 'NONE',  ( 164.3939401533646958, 245.9083385283718712, 2.844462461176849200 ) ) ;
#77697=ORIENTED_EDGE ( 'NONE', *, *, #60859, .F. ) ;
#77699=CARTESIAN_POINT ( 'NONE',  ( 178.7584752446753669, 285.6265442481744685, 13.03273535059368093 ) ) ;
#77700=CARTESIAN_POINT ( 'NONE',  ( 196.6848264441626100, 289.2939774968210713, 16.62394592573511432 ) ) ;
#77702=ORIENTED_EDGE ( 'NONE', *, *, #49251, .F. ) ;
#77706=CARTESIAN_POINT ( 'NONE',  ( 192.5712965840290849, 297.1037255674836501, 11.03742858512898906 ) ) ;
#77707=CARTESIAN_POINT ( 'NONE',  ( 164.9779129355220562, 244.8968679994381148, -1.771286574179712803 ) ) ;
#77708=CARTESIAN_POINT ( 'NONE',  ( -22.42236680055709641, 157.8615022471902591, 0.000000000000000000 ) ) ;
#77710=CARTESIAN_POINT ( 'NONE',  ( 201.0844796915553161, 282.3584598911111812, -16.59562674965125950 ) ) ;
#77712=( BOUNDED_CURVE ( )  B_SPLINE_CURVE ( 2, ( #1761, #71165, #85389, #77762, #47819, #25550, #55415, #79297, #39216 ),
 .UNSPECIFIED., .F., .T. ) 
 B_SPLINE_CURVE_WITH_KNOTS ( ( 3, 2, 2, 2, 3 ),
 ( 0.8911290322580645018, 0.8924731182795698770, 0.8951612903225806273, 0.8978494623655913776, 0.8991935483870967527 ),
 .UNSPECIFIED. ) 
 CURVE ( )  GEOMETRIC_REPRESENTATION_ITEM ( )  RATIONAL_B_SPLINE_CURVE ( ( 0.9330127018922194093, 0.9330127018922194093, 1.000000000000000000, 0.8660254037844387076, 1.000000000000000000, 0.8660254037844387076, 1.000000000000000000, 0.9330127018922194093, 0.9330127018922194093 ) ) 
 REPRESENTATION_ITEM ( '' )  );
#77713=ORIENTED_EDGE ( 'NONE', *, *, #64009, .F. ) ;
#77714=CARTESIAN_POINT ( 'NONE',  ( 198.6444633007815810, 284.5846922512318997, -17.80363864581810418 ) ) ;
#77715=CARTESIAN_POINT ( 'NONE',  ( 164.2173609823407219, 248.5881690971583851, 10.00396525085479915 ) ) ;
#77718=CARTESIAN_POINT ( 'NONE',  ( 155.4152395589816251, 261.8557187948458704, -16.98081665858997624 ) ) ;
#77719=EDGE_LOOP ( 'NONE', ( #79090, #48315, #84850, #32391 ) ) ;
#77720=CARTESIAN_POINT ( 'NONE',  ( 191.0724301404414689, 299.6998384015373063, -9.342134220577969828 ) ) ;
#77724=ORIENTED_EDGE ( 'NONE', *, *, #21108, .T. ) ;
#77725=CARTESIAN_POINT ( 'NONE',  ( 200.5438717407500917, 283.2948203288816558, 18.39667691545567152 ) ) ;
#77726=CARTESIAN_POINT ( 'NONE',  ( 127.3796741259112792, 255.8967562850346553, -4.648177544792955347E-16 ) ) ;
#77727=CARTESIAN_POINT ( 'NONE',  ( 191.4941427383744781, 298.9694107557253346, 8.584406880462095657 ) ) ;
#77729=VERTEX_POINT ( 'NONE', #68307 ) ;
#77731=B_SPLINE_CURVE_WITH_KNOTS ( 'NONE', 3,
 ( #22114, #91546, #52505, #92548, #83454, #53007, #83958, #14522, #45404, #76334, #6427, #44404, #6908, #30715, #14020, #82960, #37304, #7401, #44899, #98137, #76807, #13534, #52021, #28722, #30212, #68204, #22614, #37796, #75336, #68701, #15489, #99630, #61094, #92065, #99131, #23095, #29715, #84454, #14995, #38293, #69203, #100129, #61597, #53985, #36309, #74846 ),
 .UNSPECIFIED., .F., .F.,
 ( 4, 2, 2, 2, 2, 2, 2, 2, 2, 2, 2, 2, 2, 2, 2, 2, 2, 2, 2, 2, 2, 2, 4 ),
 ( 0.002307665126650576288, 0.002732801707347156522, 0.002945369997695357518, 0.003051654142869509190, 0.003157938288043660863, 0.003264222433217812535, 0.003370506578391964207, 0.003583074868740191658, 0.004008211449436645257, 0.004858484610829631387, 0.005708757772222617516, 0.006559030933615603645, 0.006984167514312139211, 0.007409304095008673041, 0.007515588240182871985, 0.007568730312769972324, 0.007621872385357072663, 0.007675014457944171267, 0.007728156530531271606, 0.007834440675705392487, 0.008259577256402054687, 0.008684713837098716888, 0.009109850417795377353 ),
 .UNSPECIFIED. ) ;
#77732=VERTEX_POINT ( 'NONE', #29325 ) ;
#77736=CIRCLE ( 'NONE', #46984, 17.82106496071138935 ) ;
#77738=CARTESIAN_POINT ( 'NONE',  ( 164.1146561143383167, 246.3920726737087534, -7.362905700427413436 ) ) ;
#77740=CARTESIAN_POINT ( 'NONE',  ( 168.0039864032107459, 281.1839448478028771, 11.64247976579110144 ) ) ;
#77741=CARTESIAN_POINT ( 'NONE',  ( 148.1974503712686158, 273.9614817352322120, -7.884397846570731616 ) ) ;
#77742=B_SPLINE_CURVE_WITH_KNOTS ( 'NONE', 3,
 ( #85668, #86665, #17198, #78525, #55187, #9109, #46086, #48100, #1012, #7605, #16206, #23293, #38991, #39983, #93238, #76997, #62796, #32406, #79041, #20, #69407, #47098, #70918, #70400, #87182, #1526, #23797, #71422, #24797, #38492, #63304, #78020, #54180, #31890, #2013, #32898, #94739, #94245, #86170, #30905, #85148, #69896, #8610, #25301 ),
 .UNSPECIFIED., .F., .F.,
 ( 4, 2, 2, 2, 2, 2, 2, 2, 2, 2, 2, 2, 2, 2, 2, 2, 2, 2, 2, 2, 2, 4 ),
 ( 0.003093253362364405644, 0.003290131544961049769, 0.003487009727557693894, 0.003585448818856016174, 0.003683887910154338453, 0.003880766092751096203, 0.004274522457944560094, 0.004668278823138022685, 0.005455791553525046744, 0.006243304283912070804, 0.007030817014299093996, 0.007818329744686117189, 0.007916768835984536179, 0.008015207927282951700, 0.008064427472932161195, 0.008113647018581370690, 0.008212086109879786211, 0.008408964292476488883, 0.008605842475073191555, 0.008802720657669894228, 0.008999598840266596900, 0.009393355205460038673 ),
 .UNSPECIFIED. ) ;
#77743=EDGE_CURVE ( 'NONE', #14532, #46006, #33699, .T. ) ;
#77744=CARTESIAN_POINT ( 'NONE',  ( 174.8312020576883299, 289.9788226860209193, 6.252573175169373165 ) ) ;
#77745=FACE_OUTER_BOUND ( 'NONE', #51055, .T. ) ;
#77748=CARTESIAN_POINT ( 'NONE',  ( 199.9740574423823887, 278.2632206211216612, -15.47992833812561564 ) ) ;
#77750=CARTESIAN_POINT ( 'NONE',  ( 198.0858447170796524, 287.5522480202560018, 18.44384186289807559 ) ) ;
#77751=ORIENTED_EDGE ( 'NONE', *, *, #80993, .F. ) ;
#77752=CARTESIAN_POINT ( 'NONE',  ( -22.42236680055709641, 157.8615022471902591, 0.000000000000000000 ) ) ;
#77753=CARTESIAN_POINT ( 'NONE',  ( 206.5237403681858552, 272.9373840435757188, -10.81420335655575116 ) ) ;
#77754=ADVANCED_FACE ( 'NONE', ( #75949 ), #84675, .F. ) ;
#77756=CARTESIAN_POINT ( 'NONE',  ( 153.2819058590468160, 274.2512448977743134, -12.24885634829186287 ) ) ;
#77760=VERTEX_POINT ( 'NONE', #85048 ) ;
#77761=CARTESIAN_POINT ( 'NONE',  ( 155.3559454620313147, 261.5626045322989626, -17.00790974192431548 ) ) ;
#77762=CARTESIAN_POINT ( 'NONE',  ( 128.4645176094212502, 251.6427522451419350, 10.00000000000009415 ) ) ;
#77764=CARTESIAN_POINT ( 'NONE',  ( 6.354935675815381657, 181.1427522451419350, 10.00000000000009237 ) ) ;
#77765=CARTESIAN_POINT ( 'NONE',  ( 98.87557663705065636, 218.7048013555409796, 4.594050593750051981 ) ) ;
#77768=CARTESIAN_POINT ( 'NONE',  ( 207.5492168967516875, 271.1612065941299079, 2.279797467183042325 ) ) ;
#77769=CARTESIAN_POINT ( 'NONE',  ( 8.890927067706668296, 164.3932355074535394, -2.679491924311248496 ) ) ;
#77770=CARTESIAN_POINT ( 'NONE',  ( 12.62459875707045143, 178.0958772461660544, -9.188101187500095079 ) ) ;
#77772=CARTESIAN_POINT ( 'NONE',  ( 186.8123841630082040, 258.3999256946553942, 3.104652050626591553 ) ) ;
#77773=EDGE_LOOP ( 'NONE', ( #62141, #96061, #22024, #4930 ) ) ;
#77777=CARTESIAN_POINT ( 'NONE',  ( 189.0259968054108128, 261.1256047311666180, -6.165518503103954551 ) ) ;
#77779=CARTESIAN_POINT ( 'NONE',  ( 160.2571224103306236, 275.9534525238444758, -14.07895364344611977 ) ) ;
#77781=CARTESIAN_POINT ( 'NONE',  ( 178.7215982705234012, 283.0458118805923391, -16.00884060594773217 ) ) ;
#77783=CARTESIAN_POINT ( 'NONE',  ( 34.27488675591641965, 202.8464784336661637, 1.353441290958777525E-15 ) ) ;
#77784=CARTESIAN_POINT ( 'NONE',  ( 121.2293367285889616, 249.9869531367911293, 4.594050593750046652 ) ) ;
#77785=CARTESIAN_POINT ( 'NONE',  ( 198.3441781175109497, 276.9090831475363075, 15.17843888428162735 ) ) ;
#77786=EDGE_LOOP ( 'NONE', ( #95165, #55374, #31982, #65380 ) ) ;
#77787=CARTESIAN_POINT ( 'NONE',  ( 150.2864214986432501, 271.8288624510125828, -11.67904241962729728 ) ) ;
#77788=EDGE_CURVE ( 'NONE', #10368, #2343, #81894, .T. ) ;
#77789=EDGE_CURVE ( 'NONE', #35626, #90703, #68223, .T. ) ;
#77790=CARTESIAN_POINT ( 'NONE',  ( 181.6873167589662330, 259.7205209471545118, -11.14285176367228836 ) ) ;
#77791=CARTESIAN_POINT ( 'NONE',  ( 168.4945589903323366, 288.0950524468156004, -4.184919968760112852 ) ) ;
#77794=CARTESIAN_POINT ( 'NONE',  ( 207.7666684749232786, 270.7845694125510931, -6.630926507062123498 ) ) ;
#77795=CARTESIAN_POINT ( 'NONE',  ( 147.8819534105757043, 274.5079385007862811, -9.338341377131436971 ) ) ;
#77796=CARTESIAN_POINT ( 'NONE',  ( 148.1974503712686158, 273.9614817352322120, -7.884397846570731616 ) ) ;
#77799=CARTESIAN_POINT ( 'NONE',  ( 189.3330452661960237, 262.4894502133154788, 8.166639359185952074 ) ) ;
#77800=CARTESIAN_POINT ( 'NONE',  ( 165.0066022244254498, 249.8389599805948080, -10.62953420576023511 ) ) ;
#77802=CARTESIAN_POINT ( 'NONE',  ( 190.5893431400089923, 300.5365696307625853, -0.3099240395267599535 ) ) ;
#77803=CARTESIAN_POINT ( 'NONE',  ( 181.0854462269685428, 266.2271372736428816, -14.79605532646364097 ) ) ;
#77804=VERTEX_POINT ( 'NONE', #9534 ) ;
#77805=CARTESIAN_POINT ( 'NONE',  ( 153.0234837362991698, 266.8886651207910177, -16.12888749788869447 ) ) ;
#77808=CARTESIAN_POINT ( 'NONE',  ( 102.3121810886138832, 236.0024278399160949, 9.188101187500095079 ) ) ;
#77810=CARTESIAN_POINT ( 'NONE',  ( 191.3375250863502970, 299.2406804863936145, 8.828791580707859410 ) ) ;
#77814=LINE ( 'NONE', #1803, #30308 ) ;
#77815=CARTESIAN_POINT ( 'NONE',  ( 198.4522155198218059, 286.9176751754968109, -17.57438352224490075 ) ) ;
#77816=CARTESIAN_POINT ( 'NONE',  ( 144.7927049134883077, 247.7365022471901739, -10.00000000000009237 ) ) ;
#77820=VERTEX_POINT ( 'NONE', #32810 ) ;
#77821=CARTESIAN_POINT ( 'NONE',  ( 192.8818986906848636, 267.2098981360021526, 11.18199646913336842 ) ) ;
#77823=CARTESIAN_POINT ( 'NONE',  ( 196.5239536785732923, 267.5882975073278089, 9.598076446533468697 ) ) ;
#77824=CARTESIAN_POINT ( 'NONE',  ( 187.0605947865943222, 282.7524552142733114, -17.49343033980654027 ) ) ;
#77827=CARTESIAN_POINT ( 'NONE',  ( 169.8745519614330419, 281.1702744907113356, -14.29939960421313039 ) ) ;
#77828=B_SPLINE_CURVE_WITH_KNOTS ( 'NONE', 3,
 ( #73075, #89786, #88823, #43123 ),
 .UNSPECIFIED., .F., .F.,
 ( 4, 4 ),
 ( 0.01763317218926846799, 0.02658475294366728983 ),
 .UNSPECIFIED. ) ;
#77829=EDGE_LOOP ( 'NONE', ( #26566, #46329, #88029, #27570, #81600, #43039, #82618, #93692, #75504, #84502, #9951, #87512, #79571, #98182, #73237, #96094, #16345, #47203, #85480, #56129 ) ) ;
#77833=CARTESIAN_POINT ( 'NONE',  ( 164.6836044745662377, 247.6625381034837403, 7.171422519083344049 ) ) ;
#77835=DIRECTION ( 'NONE',  ( -0.8660254037844387076, -0.4999999999999998890, -0.000000000000000000 ) ) ;
#77836=CARTESIAN_POINT ( 'NONE',  ( 157.2674082780516471, 258.2518538181732879, 18.34755329151241554 ) ) ;
#77840=CARTESIAN_POINT ( 'NONE',  ( 193.1926327199271327, 296.0275398115294934, -12.21752165518055833 ) ) ;
#77844=ORIENTED_EDGE ( 'NONE', *, *, #30650, .T. ) ;
#77845=CARTESIAN_POINT ( 'NONE',  ( 162.7020145476934090, 284.0983276010327359, 6.051621772638641872 ) ) ;
#77846=ORIENTED_EDGE ( 'NONE', *, *, #53213, .T. ) ;
#77848=EDGE_LOOP ( 'NONE', ( #19552, #83580, #62558 ) ) ;
#77849=CARTESIAN_POINT ( 'NONE',  ( 172.6226713180010961, 270.9341145373659856, 16.43373278848542540 ) ) ;
#77852=CARTESIAN_POINT ( 'NONE',  ( 164.5259176133158689, 246.1953198488120051, 1.882264443804981813 ) ) ;
#77854=CARTESIAN_POINT ( 'NONE',  ( 147.6272645182038161, 274.9490726024977789, -5.838234932324007254 ) ) ;
#77855=CARTESIAN_POINT ( 'NONE',  ( 190.0259678364800493, 301.5123642802043946, 4.004183174499006626 ) ) ;
#77857=CARTESIAN_POINT ( 'NONE',  ( 170.4391975808936479, 250.6982047760319858, -5.514033325473483238 ) ) ;
#77858=CYLINDRICAL_SURFACE ( 'NONE', #84177, 10.00000000000010658 ) ;
#77862=CARTESIAN_POINT ( 'NONE',  ( 124.1796696299359724, 236.3768266524159856, -9.188101187500091527 ) ) ;
#77863=CARTESIAN_POINT ( 'NONE',  ( 186.6174597086819631, 262.7463543296344142, -9.059254040013616560 ) ) ;
#77865=CARTESIAN_POINT ( 'NONE',  ( 177.4671251619221550, 288.9374044400234425, -9.330515757822047007 ) ) ;
#77868=CARTESIAN_POINT ( 'NONE',  ( 200.1964548776884101, 273.9920713698066379, 13.59980230080865837 ) ) ;
#77870=CARTESIAN_POINT ( 'NONE',  ( 174.2452046127573908, 290.2058683568998845, -4.780677047540736524 ) ) ;
#77871=CARTESIAN_POINT ( 'NONE',  ( 196.0034224882197975, 291.1591091234520263, 17.53794140922627776 ) ) ;
#77879=CARTESIAN_POINT ( 'NONE',  ( 174.0182248954802731, 253.4737597407804515, -7.581100471685894071 ) ) ;
#77881=CARTESIAN_POINT ( 'NONE',  ( 194.9455394410084921, 292.9914163096879065, -15.01116663483170655 ) ) ;
#77885=CARTESIAN_POINT ( 'NONE',  ( 160.2241445597728102, 279.1506239025324589, 10.70181301040688204 ) ) ;
#77886=CARTESIAN_POINT ( 'NONE',  ( 192.4441357708844578, 262.6530372631752925, 4.622430316263682393 ) ) ;
#77887=CARTESIAN_POINT ( 'NONE',  ( 190.5477107455830321, 300.6086790531491033, 3.126266616601216963 ) ) ;
#77888=CARTESIAN_POINT ( 'NONE',  ( 204.7130176219587554, 272.9107139802454753, -10.75958745166956909 ) ) ;
#77889=CARTESIAN_POINT ( 'NONE',  ( 153.4696322588327178, 270.0294559819171809, 15.09029231870687937 ) ) ;
#77890=CARTESIAN_POINT ( 'NONE',  ( 160.8497281054386576, 281.5906459864224871, 5.647281140516729359 ) ) ;
#77891=CARTESIAN_POINT ( 'NONE',  ( 152.9273493951901628, 265.7690563111299298, -17.70273273795505631 ) ) ;
#77893=CARTESIAN_POINT ( 'NONE',  ( 190.6218339396177441, 300.4802939150614520, -4.178005820806754755 ) ) ;
#77895=CARTESIAN_POINT ( 'NONE',  ( 187.2956951681344151, 261.7326779137165431, -8.891522745801257344 ) ) ;
#77897=CARTESIAN_POINT ( 'NONE',  ( 193.3429555150086685, 288.0943436124296113, -17.13583794773776248 ) ) ;
#77898=CARTESIAN_POINT ( 'NONE',  ( 167.7444804051520748, 288.1361480929475078, -1.744605501772117595 ) ) ;
#77900=CARTESIAN_POINT ( 'NONE',  ( 204.3548082856772794, 276.0577276202552071, 13.12054476288156302 ) ) ;
#77901=CARTESIAN_POINT ( 'NONE',  ( 155.5770330754656072, 261.1796695529068302, 18.26969263326161297 ) ) ;
#77904=CARTESIAN_POINT ( 'NONE',  ( -5.399381411310669066, 161.5643266524160140, -9.188101187500093303 ) ) ;
#77905=CARTESIAN_POINT ( 'NONE',  ( 88.13101510164371177, 227.8149278399160949, -9.188101187500095079 ) ) ;
#77906=CARTESIAN_POINT ( 'NONE',  ( 147.0314375879888757, 275.9810751181479986, -5.168577011192616588 ) ) ;
#77907=CARTESIAN_POINT ( 'NONE',  ( 208.2124092825819162, 270.0125236866795149, -2.339659020816897694 ) ) ;
#77908=CARTESIAN_POINT ( 'NONE',  ( 155.5066938333533528, 261.3015006940112244, -18.40036130547566273 ) ) ;
#77913=CARTESIAN_POINT ( 'NONE',  ( 207.5088755035018551, 271.2310799368871699, 6.444438407027963223 ) ) ;
#77915=DIRECTION ( 'NONE',  ( 0.4999999999999998890, -0.8660254037844385966, 0.000000000000000000 ) ) ;
#77916=CARTESIAN_POINT ( 'NONE',  ( 157.7365441389748923, 257.4392866714015895, 18.13124212464487073 ) ) ;
#77917=CYLINDRICAL_SURFACE ( 'NONE', #59198, 17.82106496071139645 ) ;
#77918=CARTESIAN_POINT ( 'NONE',  ( 38.38920161542251464, 180.7202760586659451, -5.415160957724236172E-17 ) ) ;
#77919=CARTESIAN_POINT ( 'NONE',  ( 69.59257202794182717, 220.1744531367911293, 4.594050593750047540 ) ) ;
#77923=CARTESIAN_POINT ( 'NONE',  ( -9.864998445682726214, 165.1115022471902591, 10.00000000000009592 ) ) ;
#77925=DIRECTION ( 'NONE',  ( -0.8660254037844387076, -0.4999999999999998890, -0.000000000000000000 ) ) ;
#77929=CARTESIAN_POINT ( 'NONE',  ( 198.7357616895271804, 286.4265588032756114, -17.04018524297827497 ) ) ;
#77932=CARTESIAN_POINT ( 'NONE',  ( 54.35602435405059651, 208.3149278399161233, -9.188101187500095079 ) ) ;
#77935=CARTESIAN_POINT ( 'NONE',  ( 159.9628729326222754, 253.5831720864507588, 15.75051413866357386 ) ) ;
#77937=CARTESIAN_POINT ( 'NONE',  ( 201.3854624970792599, 281.8371423797387934, 17.49239072403049988 ) ) ;
#77941=CARTESIAN_POINT ( 'NONE',  ( 111.0177141658951854, 228.2365022471901739, -10.00000000000009059 ) ) ;
#77942=CARTESIAN_POINT ( 'NONE',  ( 161.5056331467593225, 250.9110330116698435, 14.52719814064025528 ) ) ;
#77943=CARTESIAN_POINT ( 'NONE',  ( 164.7243055739305078, 245.3361288348881999, -1.445094907380085170 ) ) ;
#77946=CARTESIAN_POINT ( 'NONE',  ( 184.7502022281630047, 271.1445130452900685, 16.43725824281414560 ) ) ;
#77948=CARTESIAN_POINT ( 'NONE',  ( 206.0946696452135427, 273.6805563358039421, -10.19627505985792837 ) ) ;
#77949=CARTESIAN_POINT ( 'NONE',  ( 194.1728500316723967, 293.9464425811553383, 14.07605957608015501 ) ) ;
#77952=CARTESIAN_POINT ( 'NONE',  ( 173.5253749324791954, 251.2404134093094683, 0.4681658163635857850 ) ) ;
#77953=ORIENTED_EDGE ( 'NONE', *, *, #13954, .T. ) ;
#77955=CARTESIAN_POINT ( 'NONE',  ( 194.3541845315608612, 294.0156730581561533, -14.67567721756631016 ) ) ;
#77959=CARTESIAN_POINT ( 'NONE',  ( 22.44857442947618154, 193.7677522451419350, -5.000000000000047962 ) ) ;
#77962=CARTESIAN_POINT ( 'NONE',  ( 141.2767884429413243, 240.8262482093457777, 3.021315404115420679E-15 ) ) ;
#77964=EDGE_LOOP ( 'NONE', ( #61966, #85669, #62348, #31238 ) ) ;
#77965=CARTESIAN_POINT ( 'NONE',  ( 172.4923911848786702, 285.1025841718646916, 10.57918879521990618 ) ) ;
#77966=CARTESIAN_POINT ( 'NONE',  ( 163.2715301498190854, 283.7935623289845921, -2.937509578771470675 ) ) ;
#77968=CARTESIAN_POINT ( 'NONE',  ( 208.2912792141756029, 269.8759169579697641, -2.198672330625011995 ) ) ;
#77969=CARTESIAN_POINT ( 'NONE',  ( 155.0898745997320134, 262.0234527842152374, 17.05457557403769542 ) ) ;
#77970=CARTESIAN_POINT ( 'NONE',  ( 185.4923030054532092, 292.6699065248636202, -10.71444798707586621 ) ) ;
#77971=CARTESIAN_POINT ( 'NONE',  ( 205.3708847852691406, 274.9341884869767227, -13.70973585089674174 ) ) ;
#77972=CARTESIAN_POINT ( 'NONE',  ( 147.5084024922618084, 243.7202760586659167, -5.415160957724236172E-17 ) ) ;
#77973=CARTESIAN_POINT ( 'NONE',  ( 206.4627041557072573, 270.6281706969085121, 2.566430978744102198 ) ) ;
#77974=CARTESIAN_POINT ( 'NONE',  ( 182.6873171513263969, 259.2587024686063160, 9.588166490408216447 ) ) ;
#77975=CARTESIAN_POINT ( 'NONE',  ( 85.53293889029040997, 226.3149278399160949, -9.188101187500095079 ) ) ;
#77976=B_SPLINE_CURVE_WITH_KNOTS ( 'NONE', 3,
 ( #8147, #93272, #40020, #79589, #545, #69928, #31428, #62830, #63342, #17755, #93786, #54723, #92774, #24346, #48656, #8643, #56227, #40527, #23328, #86699, #86201, #10153, #85704, #41019, #71462, #16240, #32935, #24835, #16740, #47629, #47131, #55709 ),
 .UNSPECIFIED., .F., .F.,
 ( 4, 2, 2, 2, 2, 2, 2, 2, 2, 2, 2, 2, 2, 2, 2, 4 ),
 ( 0.0005803556464477676669, 0.001213002923345877972, 0.001845650200243988386, 0.003110944754040269496, 0.003743592030938444962, 0.004059915669387570425, 0.004138996578999795846, 0.004178537033805908990, 0.004218077488612021267, 0.004257617943418134411, 0.004297158398224247555, 0.004376239307836427006, 0.004692562946285125727, 0.005008886584733824449, 0.005325210223182522302, 0.005641533861631220156 ),
 .UNSPECIFIED. ) ;
#77978=CARTESIAN_POINT ( 'NONE',  ( 150.7254409736883645, 269.5828735707850683, 14.54962197351449049 ) ) ;
#77979=CARTESIAN_POINT ( 'NONE',  ( 162.0670251645566680, 279.3129746912387645, 12.26946893937585337 ) ) ;
#77981=ORIENTED_EDGE ( 'NONE', *, *, #76496, .F. ) ;
#77982=CARTESIAN_POINT ( 'NONE',  ( 157.4297042318662534, 257.9707489803037674, -17.23334323327960149 ) ) ;
#77983=ORIENTED_EDGE ( 'NONE', *, *, #17613, .T. ) ;
#77990=CARTESIAN_POINT ( 'NONE',  ( 48.42933654300934876, 208.7677522451419350, -5.000000000000047962 ) ) ;
#77993=CARTESIAN_POINT ( 'NONE',  ( 81.52757139778736928, 224.0024278399160949, 9.188101187500095079 ) ) ;
#78000=ADVANCED_FACE ( 'NONE', ( #29216 ), #86368, .F. ) ;
#78002=CARTESIAN_POINT ( 'NONE',  ( 200.5407427438653656, 272.3366537803537994, -12.86405620053299614 ) ) ;
#78003=CARTESIAN_POINT ( 'NONE',  ( 207.4163210057841127, 270.9512484179036278, -1.435526549205535130 ) ) ;
#78006=CARTESIAN_POINT ( 'NONE',  ( 189.0134143059085261, 294.9326290385585025, 11.47382056046370735 ) ) ;
#78007=DIRECTION ( 'NONE',  ( -0.8660254037844387076, -0.4999999999999998890, -0.000000000000000000 ) ) ;
#78008=CARTESIAN_POINT ( 'NONE',  ( 207.1181895030469491, 269.9077679394811753, 1.745611964362854929 ) ) ;
#78009=CARTESIAN_POINT ( 'NONE',  ( 153.4542976351440302, 264.8563551865710224, -17.11782692037292009 ) ) ;
#78011=CARTESIAN_POINT ( 'NONE',  ( 204.2143397907769611, 276.5280330293650195, 13.36303585211030054 ) ) ;
#78013=ORIENTED_EDGE ( 'NONE', *, *, #44813, .T. ) ;
#78014=CARTESIAN_POINT ( 'NONE',  ( 196.1671714888020972, 264.5940953169613294, 5.402994724792868020 ) ) ;
#78015=B_SPLINE_CURVE_WITH_KNOTS ( 'NONE', 3,
 ( #60332, #74592, #81708, #51249 ),
 .UNSPECIFIED., .F., .F.,
 ( 4, 4 ),
 ( 0.04823799508478943121, 0.04887066958154930724 ),
 .UNSPECIFIED. ) ;
#78016=CARTESIAN_POINT ( 'NONE',  ( 153.6323727466833873, 269.3172676078306154, -15.66543061290010641 ) ) ;
#78018=CARTESIAN_POINT ( 'NONE',  ( 187.9080819789693919, 266.1900786697327703, -11.89483730255598282 ) ) ;
#78019=CYLINDRICAL_SURFACE ( 'NONE', #36965, 17.82106496071139645 ) ;
#78020=CARTESIAN_POINT ( 'NONE',  ( 153.2977412669953310, 270.3394998157883720, 13.96444872914787716 ) ) ;
#78021=EDGE_LOOP ( 'NONE', ( #95736, #26744, #20404, #88043, #51397 ) ) ;
#78022=CARTESIAN_POINT ( 'NONE',  ( -22.42236680055709641, 157.8615022471902591, 0.000000000000000000 ) ) ;
#78023=CARTESIAN_POINT ( 'NONE',  ( 202.3894997978090373, 280.0980987621804275, 16.95659012541789323 ) ) ;
#78024=CARTESIAN_POINT ( 'NONE',  ( 164.8670003495851404, 245.0889742334797177, -1.557028074864921674 ) ) ;
#78025=CARTESIAN_POINT ( 'NONE',  ( 163.1218343930725894, 256.2508100442478849, -16.13596270478102923 ) ) ;
#78027=CARTESIAN_POINT ( 'NONE',  ( 199.1469736795485801, 281.8990786193456870, -16.60023204625315785 ) ) ;
#78029=CARTESIAN_POINT ( 'NONE',  ( 163.4339502362531675, 283.8181923016741166, -3.128993586085420553 ) ) ;
#78031=CARTESIAN_POINT ( 'NONE',  ( 188.6135346955672389, 260.1468269458595159, 3.785692842197046826 ) ) ;
#78032=CARTESIAN_POINT ( 'NONE',  ( 183.8301289239822722, 272.2411597453489662, -17.34995410509954183 ) ) ;
#78033=CARTESIAN_POINT ( 'NONE',  ( 0.9064528339360315989, 162.1423013555410080, -4.594050593750043987 ) ) ;
#78034=CARTESIAN_POINT ( 'NONE',  ( 153.3073463970432044, 273.0798447238802282, -13.25289232200638345 ) ) ;
#78035=VERTEX_POINT ( 'NONE', #85966 ) ;
#78037=B_SPLINE_CURVE_WITH_KNOTS ( 'NONE', 3,
 ( #37535, #60329, #5166, #6658, #66947, #97876, #75074, #28450, #5654, #36543, #67450, #98378, #28966, #21362, #75565, #38024, #53246, #21851 ),
 .UNSPECIFIED., .F., .F.,
 ( 4, 2, 2, 2, 2, 2, 2, 2, 4 ),
 ( 7.473417450352270646E-17, 0.0003311343341728208351, 0.0006622686683455668603, 0.0009934030025183129397, 0.001324537336691059127, 0.001655671670863805315, 0.001986806005036550853, 0.002317940339209297040, 0.002649074673382043228 ),
 .UNSPECIFIED. ) ;
#78038=CARTESIAN_POINT ( 'NONE',  ( 160.1656321119008624, 253.6529854836419133, -14.85229712523751466 ) ) ;
#78041=CARTESIAN_POINT ( 'NONE',  ( 12.78680497239753322, 184.3149278399160949, -9.188101187500095079 ) ) ;
#78046=CARTESIAN_POINT ( 'NONE',  ( 130.7684581937436405, 234.7592609112379876, 2.679491924311254714 ) ) ;
#78047=CARTESIAN_POINT ( 'NONE',  ( 173.6365052420643167, 272.7251026486088676, -16.35588217120040255 ) ) ;
#78048=CARTESIAN_POINT ( 'NONE',  ( 13.51768745649715697, 168.6115022471901739, -5.000000000000041744 ) ) ;
#78049=CARTESIAN_POINT ( 'NONE',  ( 189.9884492570354269, 298.3977273640915655, -7.992435462398296053 ) ) ;
#78050=CARTESIAN_POINT ( 'NONE',  ( 190.7539468448011064, 261.9718772365148425, -0.8656167993522486670 ) ) ;
#78051=CARTESIAN_POINT ( 'NONE',  ( 193.0242241521888502, 295.9312083549096428, -12.21184685123513347 ) ) ;
#78052=CARTESIAN_POINT ( 'NONE',  ( 69.44849478424214340, 204.2365022471902023, -10.00000000000009059 ) ) ;
#78053=CARTESIAN_POINT ( 'NONE',  ( 164.4654423005978288, 246.2001330526308323, 1.735427645011155873 ) ) ;
#78055=CARTESIAN_POINT ( 'NONE',  ( 23.17910981781079727, 190.3149278399161233, -9.188101187500095079 ) ) ;
#78056=CARTESIAN_POINT ( 'NONE',  ( 171.2743479101317234, 254.4242377521371736, -11.94796457435898951 ) ) ;
#78058=CARTESIAN_POINT ( 'NONE',  ( 135.1942566882107997, 238.8615022471902023, 5.000000000000051514 ) ) ;
#78059=CARTESIAN_POINT ( 'NONE',  ( 203.0856642093833671, 269.8431269742375775, -6.121545823302062317 ) ) ;
#78060=CARTESIAN_POINT ( 'NONE',  ( 177.9925615710933755, 254.8251403409008731, -7.350624415798725053 ) ) ;
#78064=CARTESIAN_POINT ( 'NONE',  ( 159.8982138663949399, 278.4101122861870863, -10.05609574519431071 ) ) ;
#78067=CARTESIAN_POINT ( 'NONE',  ( 163.1008115941903895, 248.1481028935802442, 11.25332017433677834 ) ) ;
#78068=CARTESIAN_POINT ( 'NONE',  ( 102.4837554958880759, 236.6427522451419350, 10.00000000000009415 ) ) ;
#78069=CARTESIAN_POINT ( 'NONE',  ( 186.4223700097188043, 267.8240592505130167, -15.11424446612579864 ) ) ;
#78076=ORIENTED_EDGE ( 'NONE', *, *, #34026, .F. ) ;
#78077=CARTESIAN_POINT ( 'NONE',  ( 30.47735161394240322, 181.7365022471901739, -10.00000000000009237 ) ) ;
#78079=CARTESIAN_POINT ( 'NONE',  ( 150.8757650385446993, 269.3225046528533539, 14.31332712971473953 ) ) ;
#78083=CARTESIAN_POINT ( 'NONE',  ( 186.9159192308579236, 272.5337820971376459, -15.87923880755278461 ) ) ;
#78086=CARTESIAN_POINT ( 'NONE',  ( 153.2906404175950854, 265.1398178023911782, -17.60231834963988007 ) ) ;
#78087=CARTESIAN_POINT ( 'NONE',  ( 189.7740653892032014, 260.9666063005456635, -5.939916383645439169 ) ) ;
#78090=CARTESIAN_POINT ( 'NONE',  ( 147.9710862514405960, 274.3535558917855042, 7.785500222159708272 ) ) ;
#78092=VERTEX_POINT ( 'NONE', #70691 ) ;
#78093=CARTESIAN_POINT ( 'NONE',  ( 195.7291534503633272, 291.6341570319625021, 16.44925029361851543 ) ) ;
#78094=CARTESIAN_POINT ( 'NONE',  ( 162.1614388314975486, 266.6158802597933004, 17.60528378688847795 ) ) ;
#78095=ORIENTED_EDGE ( 'NONE', *, *, #31857, .F. ) ;
#78098=CARTESIAN_POINT ( 'NONE',  ( 159.2111180226792726, 254.8852497853115722, 16.01057445397460910 ) ) ;
#78100=CARTESIAN_POINT ( 'NONE',  ( 56.08842225738447240, 197.0643266524160140, 9.188101187500095079 ) ) ;
#78104=CARTESIAN_POINT ( 'NONE',  ( 180.8890834033174713, 294.3766012452771861, 6.559837412958372305 ) ) ;
#78105=CARTESIAN_POINT ( 'NONE',  ( 173.7338896087951809, 271.5854767220461667, 16.43201141598054349 ) ) ;
#78107=ORIENTED_EDGE ( 'NONE', *, *, #93311, .T. ) ;
#78108=ORIENTED_EDGE ( 'NONE', *, *, #36509, .T. ) ;
#78109=CARTESIAN_POINT ( 'NONE',  ( 190.2020559385390470, 299.9191148095094377, 5.071379031179562347 ) ) ;
#78110=CARTESIAN_POINT ( 'NONE',  ( 68.76057960370418698, 222.0530062829863027, -4.648177544792955347E-16 ) ) ;
#78111=CARTESIAN_POINT ( 'NONE',  ( 190.5726849661229210, 300.5654224342945326, -0.2192718484028965964 ) ) ;
#78112=VERTEX_POINT ( 'NONE', #54468 ) ;
#78113=CARTESIAN_POINT ( 'NONE',  ( 174.5508403973756515, 260.3590064504865040, -14.93617697178709314 ) ) ;
#78115=CARTESIAN_POINT ( 'NONE',  ( 207.8996209429610360, 270.5542889829179103, -5.987818313449536411 ) ) ;
#78116=EDGE_CURVE ( 'NONE', #54626, #43956, #32189, .T. ) ;
#78117=CARTESIAN_POINT ( 'NONE',  ( 147.4271219180435253, 275.2957297547342819, -3.800519706258907782 ) ) ;
#78118=CARTESIAN_POINT ( 'NONE',  ( 190.0607312434325138, 301.4521522931182176, 3.538147641957853473 ) ) ;
#78126=CARTESIAN_POINT ( 'NONE',  ( 121.5276403787286483, 228.7202760586659736, -5.415160957724236172E-17 ) ) ;
#78128=CARTESIAN_POINT ( 'NONE',  ( 147.2592533090473239, 275.5864867145116932, -0.3770461397900867762 ) ) ;
#78132=CARTESIAN_POINT ( 'NONE',  ( 155.0304386007204016, 262.1263989543018056, -17.12961552904782181 ) ) ;
#78133=CARTESIAN_POINT ( 'NONE',  ( 163.7064929935861244, 247.0990319366274548, 6.401263337036986023 ) ) ;
#78136=ORIENTED_EDGE ( 'NONE', *, *, #1251, .F. ) ;
#78139=CARTESIAN_POINT ( 'NONE',  ( 206.3929371469040746, 272.7357536028613936, 8.215407031707147922 ) ) ;
#78140=CARTESIAN_POINT ( 'NONE',  ( 128.2389901622930495, 244.8458772461660544, 9.188101187500095079 ) ) ;
#78141=CARTESIAN_POINT ( 'NONE',  ( 198.8570476668614049, 286.2164853282868080, -17.01721544293231858 ) ) ;
#78143=CARTESIAN_POINT ( 'NONE',  ( 186.9854375150685257, 297.4581504985191032, 4.686305160240775258 ) ) ;
#78144=CARTESIAN_POINT ( 'NONE',  ( 187.4766440450278537, 281.3944037113421359, -17.42068772228976314 ) ) ;
#78146=CARTESIAN_POINT ( 'NONE',  ( 39.14627965220388006, 205.6589784336661637, -6.496448406907675876E-16 ) ) ;
#78152=CARTESIAN_POINT ( 'NONE',  ( 175.0900761532694219, 261.2389906071587689, 14.88021766879188412 ) ) ;
#78153=CARTESIAN_POINT ( 'NONE',  ( 84.79042978850567636, 219.7608392184588411, -2.428612866367529932E-12 ) ) ;
#78156=CARTESIAN_POINT ( 'NONE',  ( 118.0722127640079577, 245.6427522451419065, 10.00000000000009237 ) ) ;
#78157=CARTESIAN_POINT ( 'NONE',  ( 194.4648444083005359, 293.3692358227498289, -14.53531652569186150 ) ) ;
#78158=ORIENTED_EDGE ( 'NONE', *, *, #3619, .T. ) ;
#78159=B_SPLINE_CURVE_WITH_KNOTS ( 'NONE', 3,
 ( #77520, #1007, #31884, #62790 ),
 .UNSPECIFIED., .F., .F.,
 ( 4, 4 ),
 ( 0.006723087913367474522, 0.01173915425796831676 ),
 .UNSPECIFIED. ) ;
#78160=CARTESIAN_POINT ( 'NONE',  ( 202.5245888501533216, 279.8641176599742266, 15.60152447840272494 ) ) ;
#78162=EDGE_CURVE ( 'NONE', #81006, #68960, #78608, .T. ) ;
#78163=CARTESIAN_POINT ( 'NONE',  ( 24.36989474801440636, 191.0024278399160949, 9.188101187500095079 ) ) ;
#78169=CARTESIAN_POINT ( 'NONE',  ( 59.87693630317638593, 211.5024278399160949, -9.188101187500093303 ) ) ;
#78171=CARTESIAN_POINT ( 'NONE',  ( 126.6061714340151241, 237.2365022471902023, -10.00000000000009237 ) ) ;
#78174=CARTESIAN_POINT ( 'NONE',  ( 161.7988821920622513, 251.5333527145129437, -12.97904280059305293 ) ) ;
#78176=CARTESIAN_POINT ( 'NONE',  ( 30.47735161394240322, 181.7365022471901739, -10.00000000000009059 ) ) ;
#78177=DIRECTION ( 'NONE',  ( -0.8660254037844359321, -0.5000000000000051070, -0.000000000000000000 ) ) ;
#78178=CARTESIAN_POINT ( 'NONE',  ( 202.3139361598622372, 280.2289788223093865, 15.93832709035092421 ) ) ;
#78179=CARTESIAN_POINT ( 'NONE',  ( 151.5948730924283723, 249.1423013555410080, -4.594050593750043987 ) ) ;
#78181=CARTESIAN_POINT ( 'NONE',  ( 166.9114198365767550, 262.1412704778039142, -16.32394542780318858 ) ) ;
#78182=CARTESIAN_POINT ( 'NONE',  ( 170.5221306371715286, 263.5122761618970344, 15.79513009679484803 ) ) ;
#78184=CARTESIAN_POINT ( 'NONE',  ( 185.4455296801821476, 260.4024382772719264, 6.342364096776786475 ) ) ;
#78185=CARTESIAN_POINT ( 'NONE',  ( 206.2520115784021471, 273.4080321133600933, 11.69992874350409018 ) ) ;
#78186=CARTESIAN_POINT ( 'NONE',  ( 186.4709408934271266, 258.2127684368444989, -2.486660817739086315 ) ) ;
#78188=ORIENTED_EDGE ( 'NONE', *, *, #81421, .T. ) ;
#78189=CARTESIAN_POINT ( 'NONE',  ( 56.22356517706928969, 213.2677522451419350, -5.000000000000047962 ) ) ;
#78190=CARTESIAN_POINT ( 'NONE',  ( 178.3565173979539509, 285.6070500341613183, 12.91966154977564329 ) ) ;
#78196=AXIS2_PLACEMENT_3D ( 'NONE', #9787, #78177, #25981 ) ;
#78197=EDGE_CURVE ( 'NONE', #35992, #35860, #90827, .T. ) ;
#78198=CARTESIAN_POINT ( 'NONE',  ( 152.6992418905140028, 266.1641500988167763, 17.27767170937316621 ) ) ;
#78199=CARTESIAN_POINT ( 'NONE',  ( 81.06766895168330223, 227.6115022471903160, -5.000000000000047962 ) ) ;
#78201=CARTESIAN_POINT ( 'NONE',  ( 208.2912792141756029, 269.8759169579697641, -2.198672330625011995 ) ) ;
#78202=CARTESIAN_POINT ( 'NONE',  ( 154.8556227199321427, 262.4291889417971788, 17.77326384500479861 ) ) ;
#78205=CARTESIAN_POINT ( 'NONE',  ( 155.8645391177437887, 277.2735152180572982, -10.45080344275615758 ) ) ;
#78211=VERTEX_POINT ( 'NONE', #3808 ) ;
#78212=CARTESIAN_POINT ( 'NONE',  ( 146.5689048584090699, 276.7822053059436485, -0.4306668706573002492 ) ) ;
#78219=CARTESIAN_POINT ( 'NONE',  ( 155.6211605266461220, 261.1032385654538075, 17.14571743626555644 ) ) ;
#78220=CARTESIAN_POINT ( 'NONE',  ( 167.6711793886181852, 254.0238391605262223, -13.38728416657071563 ) ) ;
#78221=CARTESIAN_POINT ( 'NONE',  ( 190.7851751463332164, 300.1973786460605425, 8.237717828100052486 ) ) ;
#78223=B_SPLINE_SURFACE_WITH_KNOTS ( 'NONE', 3, 1, ( 
 ( #34589, #65488 ),
 ( #9297, #59869 ),
 ( #4183, #82736 ),
 ( #90835, #35084 ),
 ( #75102, #43676 ),
 ( #57885, #28996 ),
 ( #65988, #11812 ),
 ( #59357, #89353 ),
 ( #58377, #58858 ),
 ( #13307, #28476 ),
 ( #96941, #88864 ),
 ( #20910, #98402 ),
 ( #44166, #89827 ),
 ( #19429, #27979 ),
 ( #5680, #50285 ),
 ( #51797, #36569 ),
 ( #12814, #20403 ),
 ( #81238, #43164 ),
 ( #97411, #74618 ),
 ( #4699, #42669 ),
 ( #90333, #73602 ),
 ( #97901, #67476 ),
 ( #27507, #51272 ),
 ( #19906, #50778 ),
 ( #5191, #36073 ),
 ( #81728, #66974 ),
 ( #82238, #12305 ),
 ( #74105, #35589 ),
 ( #66484, #26325 ),
 ( #79563, #10121 ),
 ( #18226, #80560 ),
 ( #42491, #10625 ),
 ( #58206, #57198 ),
 ( #17726, #34896 ) ),
 .UNSPECIFIED., .T., .F., .F.,
 ( 4, 2, 2, 2, 2, 2, 2, 2, 2, 2, 2, 2, 2, 2, 2, 2, 4 ),
 ( 2, 2 ),
 ( 0.000000000000000000, 0.06250000000000000000, 0.1250000000000000000, 0.1875000000000000000, 0.2500000000000000000, 0.3125000000000000000, 0.3750000000000000000, 0.4375000000000000000, 0.5000000000000000000, 0.5625000000000000000, 0.6250000000000000000, 0.6875000000000000000, 0.7500000000000000000, 0.8125000000000000000, 0.8750000000000000000, 0.9375000000000000000, 1.000000000000000000 ),
 ( 0.000000000000000000, 1.000000000000000000 ),
 .UNSPECIFIED. ) ;
#78226=EDGE_CURVE ( 'NONE', #79518, #87939, #3769, .T. ) ;
#78228=ORIENTED_EDGE ( 'NONE', *, *, #7772, .T. ) ;
#78231=CARTESIAN_POINT ( 'NONE',  ( 177.5865089022509551, 268.7852845103913069, 17.37969943402860906 ) ) ;
#78233=EDGE_CURVE ( 'NONE', #20199, #30467, #60609, .T. ) ;
#78234=CARTESIAN_POINT ( 'NONE',  ( 208.3132655666949233, 269.8378354783333180, 2.688523655043302707 ) ) ;
#78235=CARTESIAN_POINT ( 'NONE',  ( -13.76211276271272865, 162.8615022471902307, 0.000000000000000000 ) ) ;
#78236=CARTESIAN_POINT ( 'NONE',  ( 171.0393489256058217, 283.3835579739524064, 12.04226256192440836 ) ) ;
#78237=CARTESIAN_POINT ( 'NONE',  ( 194.9819925439454664, 292.9282776833073285, -15.33279721168237586 ) ) ;
#78239=CARTESIAN_POINT ( 'NONE',  ( 197.7402002575066433, 288.1509217855910379, -17.43364815852810423 ) ) ;
#78240=CARTESIAN_POINT ( 'NONE',  ( 166.7979224981183108, 247.0939422667762813, 1.921831505315402477 ) ) ;
#78242=CARTESIAN_POINT ( 'NONE',  ( 195.6914848190668863, 279.7035040353765680, -17.46620344769279853 ) ) ;
#78243=CARTESIAN_POINT ( 'NONE',  ( 164.5648480107187197, 245.6123174360222094, 3.015887571020871238 ) ) ;
#78245=ORIENTED_EDGE ( 'NONE', *, *, #39078, .T. ) ;
#78247=CARTESIAN_POINT ( 'NONE',  ( 190.8086039075475071, 300.1567988412789987, 5.217942970589348306 ) ) ;
#78248=CARTESIAN_POINT ( 'NONE',  ( 152.7043854946215049, 268.1552411151685078, 15.94764448997051964 ) ) ;
#78250=CARTESIAN_POINT ( 'NONE',  ( 206.4640281786353171, 273.0408085897082060, -10.81921452789957883 ) ) ;
#78251=CYLINDRICAL_SURFACE ( 'NONE', #65120, 17.82106496071139645 ) ;
#78253=CARTESIAN_POINT ( 'NONE',  ( 161.6707029936031574, 250.6251236501384483, 14.45053103226186231 ) ) ;
#78254=CARTESIAN_POINT ( 'NONE',  ( 104.1130136275158975, 242.4637435831425023, 2.679491924311251605 ) ) ;
#78256=CARTESIAN_POINT ( 'NONE',  ( 193.9668281760451976, 294.6865939465442921, -14.27585970476158472 ) ) ;
#78259=CARTESIAN_POINT ( 'NONE',  ( 18.55146011244625370, 181.5177522451418497, -10.00000000000009592 ) ) ;
#78260=CARTESIAN_POINT ( 'NONE',  ( 84.85626976964255164, 228.9869531367911293, 4.594050593750046652 ) ) ;
#78262=CARTESIAN_POINT ( 'NONE',  ( 171.6481351228935353, 251.7782516689747183, -8.436504614365913923 ) ) ;
#78263=CARTESIAN_POINT ( 'NONE',  ( 166.9835885616171254, 278.1161903108272213, -13.50565314437992726 ) ) ;
#78264=CARTESIAN_POINT ( 'NONE',  ( 16.79251956066557128, 174.3768266524160140, 9.188101187500098632 ) ) ;
#78266=CLOSED_SHELL ( 'NONE', ( #35507, #52696, #46138, #48784 ) ) ;
#78267=CARTESIAN_POINT ( 'NONE',  ( 200.5621507313343557, 283.2631601884785368, 16.81037192529623425 ) ) ;
#78269=ORIENTED_EDGE ( 'NONE', *, *, #48245, .T. ) ;
#78270=CARTESIAN_POINT ( 'NONE',  ( 201.3911183001464451, 266.9640362439821502, -3.754059931952923534 ) ) ;
#78273=CARTESIAN_POINT ( 'NONE',  ( 42.54989241151534429, 183.8262482093457493, 3.021315404115420679E-15 ) ) ;
#78274=CARTESIAN_POINT ( 'NONE',  ( 92.83118068642198750, 217.7365022471901739, -10.00000000000009237 ) ) ;
#78276=CARTESIAN_POINT ( 'NONE',  ( 32.70573635520464251, 183.5643266524160140, 9.188101187500095079 ) ) ;
#78277=CARTESIAN_POINT ( 'NONE',  ( 94.68952686182812783, 232.1427522451419065, 10.00000000000009415 ) ) ;
#78279=CARTESIAN_POINT ( 'NONE',  ( 151.4434765650916859, 272.4879699064614442, -11.67392547022929783 ) ) ;
#78281=PLANE ( 'NONE',  #59836 ) ;
#78282=EDGE_CURVE ( 'NONE', #28585, #37573, #49687, .T. ) ;
#78283=CARTESIAN_POINT ( 'NONE',  ( 166.6782394145706974, 287.1526701389618665, -3.786997032746254988 ) ) ;
#78284=CARTESIAN_POINT ( 'NONE',  ( 157.2744851780909414, 258.2395962677452985, 18.17792129701959070 ) ) ;
#78286=CARTESIAN_POINT ( 'NONE',  ( 68.53065452504849020, 198.8262482093457777, 3.021315404115420679E-15 ) ) ;
#78288=CARTESIAN_POINT ( 'NONE',  ( 194.3442947553755005, 294.0328026529847421, -15.97648891113594871 ) ) ;
#78290=CARTESIAN_POINT ( 'NONE',  ( 192.4162201953099895, 265.1061942910134235, 7.764509510832549033 ) ) ;
#78291=CARTESIAN_POINT ( 'NONE',  ( 171.4174712912980567, 280.1694600568308147, 15.32434928890935133 ) ) ;
#78292=CYLINDRICAL_SURFACE ( 'NONE', #598, 17.82106496071139645 ) ;
#78293=CARTESIAN_POINT ( 'NONE',  ( 146.6363376198206652, 276.6654083370839885, -0.5879280619134327202 ) ) ;
#78294=CARTESIAN_POINT ( 'NONE',  ( 147.9710862514405960, 274.3535558917855042, 7.785500222159708272 ) ) ;
#78295=CARTESIAN_POINT ( 'NONE',  ( 180.9086552280229512, 266.9847810424545855, -14.76064602474076537 ) ) ;
#78298=( BOUNDED_CURVE ( )  B_SPLINE_CURVE ( 2, ( #69071, #1698, #15867, #32581, #69573, #39648, #45759 ),
 .UNSPECIFIED., .F., .T. ) 
 B_SPLINE_CURVE_WITH_KNOTS ( ( 3, 2, 2, 3 ),
 ( 0.9798387096774193727, 0.9811827956989247479, 0.9838709677419354982, 0.9855363728105643872 ),
 .UNSPECIFIED. ) 
 CURVE ( )  GEOMETRIC_REPRESENTATION_ITEM ( )  RATIONAL_B_SPLINE_CURVE ( ( 0.9330127018922194093, 0.9330127018922194093, 1.000000000000000000, 0.8660254037844387076, 1.000000000000000000, 0.9169986265629754829, 0.9368410486966849415 ) ) 
 REPRESENTATION_ITEM ( '' )  );
#78299=CARTESIAN_POINT ( 'NONE',  ( 207.5215400641004351, 271.2091442744748520, 2.886080616848571534 ) ) ;
#78300=CARTESIAN_POINT ( 'NONE',  ( 181.1695799106581148, 268.1689120071131924, 16.08932648799075338 ) ) ;
#78301=CARTESIAN_POINT ( 'NONE',  ( 100.7694865641816051, 238.1744531367911293, 4.594050593750047540 ) ) ;
#78303=CARTESIAN_POINT ( 'NONE',  ( 151.4361976351029000, 268.3518069213970421, 15.15218985681980612 ) ) ;
#78306=CARTESIAN_POINT ( 'NONE',  ( 157.5042325173297684, 257.8416622032797818, 16.70595240278738203 ) ) ;
#78307=CARTESIAN_POINT ( 'NONE',  ( 195.1777878793919854, 279.1127009034667594, 16.30558289032921948 ) ) ;
#78308=CARTESIAN_POINT ( 'NONE',  ( 150.6248456996347045, 269.7571096964470598, -15.31580666236335908 ) ) ;
#78310=CARTESIAN_POINT ( 'NONE',  ( 149.9417705975453430, 271.6836028715711677, -11.65547513120671219 ) ) ;
#78311=CARTESIAN_POINT ( 'NONE',  ( 105.2496719664350451, 243.1199935810941213, 2.679491924311251605 ) ) ;
#78312=CARTESIAN_POINT ( 'NONE',  ( 146.7943851877206214, 276.3916619194686746, -4.608908220452185844 ) ) ;
#78314=ORIENTED_EDGE ( 'NONE', *, *, #73449, .T. ) ;
#78315=CARTESIAN_POINT ( 'NONE',  ( 190.5690073685513255, 266.3856132956990450, 10.80116815030898003 ) ) ;
#78317=CARTESIAN_POINT ( 'NONE',  ( 196.6843777741297856, 267.5020668084886211, 9.700680000278353532 ) ) ;
#78318=EDGE_CURVE ( 'NONE', #31824, #69871, #8283, .T. ) ;
#78322=CARTESIAN_POINT ( 'NONE',  ( 179.8937413821747100, 262.8266594973790689, -12.81885310938439382 ) ) ;
#78323=CARTESIAN_POINT ( 'NONE',  ( 186.7554075434758545, 282.3000898601083577, 17.53539547572453827 ) ) ;
#78325=CARTESIAN_POINT ( 'NONE',  ( 192.0712386031329686, 297.9698513971258649, 12.12276320360788873 ) ) ;
#78327=B_SPLINE_CURVE_WITH_KNOTS ( 'NONE', 3,
 ( #1791, #31162, #62552, #93515 ),
 .UNSPECIFIED., .F., .F.,
 ( 4, 4 ),
 ( 0.04501900553147333839, 0.04887120950165264877 ),
 .UNSPECIFIED. ) ;
#78330=ORIENTED_EDGE ( 'NONE', *, *, #16335, .F. ) ;
#78332=DIRECTION ( 'NONE',  ( 0.4999999999999998890, -0.8660254037844385966, 0.000000000000000000 ) ) ;
#78336=DIRECTION ( 'NONE',  ( 0.4999999999999998890, -0.8660254037844385966, 0.000000000000000000 ) ) ;
#78337=CARTESIAN_POINT ( 'NONE',  ( 150.8555837531579868, 276.0290483310748755, -8.437460036063264113 ) ) ;
#78342=CARTESIAN_POINT ( 'NONE',  ( 203.5080190724872011, 278.1607665491929993, -15.47044080916498743 ) ) ;
#78344=ORIENTED_EDGE ( 'NONE', *, *, #79534, .T. ) ;
#78345=CARTESIAN_POINT ( 'NONE',  ( 162.6525385610000569, 249.3719130927429717, 10.67620540106957350 ) ) ;
#78349=ORIENTED_EDGE ( 'NONE', *, *, #68874, .T. ) ;
#78351=CARTESIAN_POINT ( 'NONE',  ( 164.8075539017095252, 280.4672370525465226, 12.63796469268613265 ) ) ;
#78352=EDGE_LOOP ( 'NONE', ( #55266, #82078, #3504, #90110 ) ) ;
#78354=CARTESIAN_POINT ( 'NONE',  ( 165.4979031618668444, 275.0437756392552160, -16.09671154009961569 ) ) ;
#78355=CARTESIAN_POINT ( 'NONE',  ( 165.0260329286864760, 244.8135217264176049, -2.114260670082726890 ) ) ;
#78356=CARTESIAN_POINT ( 'NONE',  ( 147.1659813806172110, 275.7480384334725159, -6.355065261369051477 ) ) ;
#78357=CARTESIAN_POINT ( 'NONE',  ( 196.0450415453838673, 284.4196233059693100, -17.59408283607186263 ) ) ;
#78361=AXIS2_PLACEMENT_3D ( 'NONE', #48132, #79075, #47624 ) ;
#78362=CARTESIAN_POINT ( 'NONE',  ( 154.0080725480042645, 280.0853259021857298, 2.227893399009504449 ) ) ;
#78363=EDGE_CURVE ( 'NONE', #43169, #346, #27972, .T. ) ;
#78364=CARTESIAN_POINT ( 'NONE',  ( 117.5758788303146076, 244.8149278399160664, 9.188101187500093303 ) ) ;
#78366=ORIENTED_EDGE ( 'NONE', *, *, #16550, .F. ) ;
#78369=ORIENTED_EDGE ( 'NONE', *, *, #35527, .T. ) ;
#78370=CARTESIAN_POINT ( 'NONE',  ( 200.3293654959697392, 273.7156512906800572, 13.98704503334941229 ) ) ;
#78371=CARTESIAN_POINT ( 'NONE',  ( 177.9052972741453971, 254.1236105787376687, 1.345436856673193127 ) ) ;
#78373=CARTESIAN_POINT ( 'NONE',  ( 190.1523655968549917, 300.2662179550520705, 3.189538939137619877 ) ) ;
#78376=CARTESIAN_POINT ( 'NONE',  ( 173.6157233020167610, 287.1844615712983568, -9.596145886780515610 ) ) ;
#78379=ORIENTED_EDGE ( 'NONE', *, *, #26480, .F. ) ;
#78380=CARTESIAN_POINT ( 'NONE',  ( 148.3625667886952044, 273.6754917110858401, -8.960758510948144462 ) ) ;
#78381=CARTESIAN_POINT ( 'NONE',  ( 150.1137873495230224, 271.7467049757541986, 11.69504156493408686 ) ) ;
#78382=EDGE_LOOP ( 'NONE', ( #2274, #21026, #83142, #96707 ) ) ;
#78383=CARTESIAN_POINT ( 'NONE',  ( 191.1909278266552974, 267.6859549916610490, -12.12569103935590675 ) ) ;
#78384=CARTESIAN_POINT ( 'NONE',  ( 190.6715059189721728, 283.1265308623420083, -16.56656797196155750 ) ) ;
#78385=CARTESIAN_POINT ( 'NONE',  ( 191.7031701327977657, 298.6073646884106552, -10.95670423068276200 ) ) ;
#78386=CARTESIAN_POINT ( 'NONE',  ( 149.3833831332874240, 271.9073859370555510, 11.40518020539810173 ) ) ;
#78387=CARTESIAN_POINT ( 'NONE',  ( 163.1002605973966126, 283.8590136238245236, 7.096359992437378139 ) ) ;
#78388=CARTESIAN_POINT ( 'NONE',  ( 161.5427656070157241, 281.5317803557720708, -6.609083002670620210 ) ) ;
#78389=CARTESIAN_POINT ( 'NONE',  ( 151.5633707495463227, 275.0466943824089299, -8.634966370009285797 ) ) ;
#78392=CARTESIAN_POINT ( 'NONE',  ( 190.9441801652054096, 299.9219738747156043, -4.765040093794296716 ) ) ;
#78393=CARTESIAN_POINT ( 'NONE',  ( 187.1508084581589344, 263.0214344965982036, -9.031509870500761039 ) ) ;
#78394=CARTESIAN_POINT ( 'NONE',  ( 190.1014290098027004, 274.4466737287558544, -15.67214041744576924 ) ) ;
#78397=CARTESIAN_POINT ( 'NONE',  ( 195.8285188278500470, 273.2427770020486832, 15.26130794574777383 ) ) ;
#78398=CARTESIAN_POINT ( 'NONE',  ( 153.3100492430090753, 265.1062007306585997, 16.32434963471121492 ) ) ;
#78400=CARTESIAN_POINT ( 'NONE',  ( -4.668846022976054222, 158.1115022471902023, -5.000000000000041744 ) ) ;
#78401=CARTESIAN_POINT ( 'NONE',  ( -22.42236680055709641, 157.8615022471902591, 0.000000000000000000 ) ) ;
#78402=CARTESIAN_POINT ( 'NONE',  ( 3.071516343397128423, 163.3923013555410080, 4.594050593750050204 ) ) ;
#78403=CARTESIAN_POINT ( 'NONE',  ( 86.94057726720511425, 214.8768266524160140, 9.188101187500098632 ) ) ;
#78404=CARTESIAN_POINT ( 'NONE',  ( 203.4357368910538355, 278.2859629599173559, -16.45855118664066197 ) ) ;
#78405=CARTESIAN_POINT ( 'NONE',  ( 146.8868584395697781, 276.2314935489248455, -3.891417269505058396 ) ) ;
#78406=CARTESIAN_POINT ( 'NONE',  ( 182.8360444305251349, 294.4420450557742583, -8.068983014621899486 ) ) ;
#78407=EDGE_CURVE ( 'NONE', #65018, #36928, #30304, .T. ) ;
#78408=CARTESIAN_POINT ( 'NONE',  ( 155.3250150347760723, 261.6161776038049425, -18.57420904020362684 ) ) ;
#78414=CARTESIAN_POINT ( 'NONE',  ( 180.9657615313112728, 291.1000814692523022, 9.328123854075322186 ) ) ;
#78416=CARTESIAN_POINT ( 'NONE',  ( 204.8040236202276674, 275.9160208256662941, -13.14144539090630204 ) ) ;
#78417=CARTESIAN_POINT ( 'NONE',  ( 157.2744851780909414, 258.2395962677452985, 18.17792129701959070 ) ) ;
#78420=CARTESIAN_POINT ( 'NONE',  ( 161.8839333999304415, 250.2557977526613229, -13.90128376743482441 ) ) ;
#78421=CARTESIAN_POINT ( 'NONE',  ( 41.52819660837609916, 194.7833772461660544, -9.188101187500095079 ) ) ;
#78422=B_SPLINE_CURVE_WITH_KNOTS ( 'NONE', 3,
 ( #42844, #88537, #65662, #12995 ),
 .UNSPECIFIED., .F., .F.,
 ( 4, 4 ),
 ( 0.003497155503932982204, 0.007366944115509544908 ),
 .UNSPECIFIED. ) ;
#78423=CARTESIAN_POINT ( 'NONE',  ( 67.67116493723634107, 216.0024278399160664, -9.188101187500093303 ) ) ;
#78431=CARTESIAN_POINT ( 'NONE',  ( 196.4451169242987305, 269.0860587627796576, -10.53632002257244338 ) ) ;
#78433=CARTESIAN_POINT ( 'NONE',  ( 198.7501991201633018, 286.4015524398827779, -18.58948563601804693 ) ) ;
#78434=CARTESIAN_POINT ( 'NONE',  ( 196.5806080813426888, 290.1593943507663766, -16.31912166233602690 ) ) ;
#78436=CARTESIAN_POINT ( 'NONE',  ( 73.32782722540972031, 203.9548013555409796, -4.594050593750042211 ) ) ;
#78438=CARTESIAN_POINT ( 'NONE',  ( 203.2732885619977026, 278.5673317194472247, -16.64305493556850024 ) ) ;
#78439=CARTESIAN_POINT ( 'NONE',  ( 160.0072461633487535, 253.5063153963366744, 16.23938890643736244 ) ) ;
#78440=CARTESIAN_POINT ( 'NONE',  ( 48.09199531666208571, 210.1199935810940929, 2.679491924311303119 ) ) ;
#78441=CARTESIAN_POINT ( 'NONE',  ( 154.0754981180030825, 263.7804043885726060, 17.67325968003652292 ) ) ;
#78442=EDGE_CURVE ( 'NONE', #99135, #68704, #37648, .T. ) ;
#78443=EDGE_CURVE ( 'NONE', #70599, #90346, #12628, .T. ) ;
#78445=CARTESIAN_POINT ( 'NONE',  ( 100.6254093204818645, 242.2365022471903444, 2.944929066748280225E-16 ) ) ;
#78446=CARTESIAN_POINT ( 'NONE',  ( 200.7897860911934913, 282.8688841796032420, 18.17522996445731920 ) ) ;
#78447=CARTESIAN_POINT ( 'NONE',  ( 206.9676408587583296, 272.1685258403992975, 7.544050792475608169 ) ) ;
#78450=CARTESIAN_POINT ( 'NONE',  ( 187.9837572234687002, 273.3093249989548212, 15.64228832037970562 ) ) ;
#78452=CARTESIAN_POINT ( 'NONE',  ( 159.2713554375903300, 254.7809155221686410, -15.70062444474382168 ) ) ;
#78453=CARTESIAN_POINT ( 'NONE',  ( 193.6538297768585153, 294.3106073703939387, 13.99927879369582406 ) ) ;
#78454=CARTESIAN_POINT ( 'NONE',  ( 167.4734756851294151, 275.5778401279644640, 16.39827101669492393 ) ) ;
#78456=CARTESIAN_POINT ( 'NONE',  ( 177.2715209000007235, 253.2106104779961981, -0.2627270112733235963 ) ) ;
#78457=VERTEX_POINT ( 'NONE', #3693 ) ;
#78459=CARTESIAN_POINT ( 'NONE',  ( 194.9455394410084921, 292.9914163096879065, -15.01116663483170655 ) ) ;
#78460=CARTESIAN_POINT ( 'NONE',  ( 148.5451600033913735, 273.7521268005480124, 8.257041405901727416 ) ) ;
#78461=ORIENTED_EDGE ( 'NONE', *, *, #37929, .F. ) ;
#78464=CARTESIAN_POINT ( 'NONE',  ( 30.69616969366791537, 176.9824982072973967, 3.021315404115420679E-15 ) ) ;
#78467=ORIENTED_EDGE ( 'NONE', *, *, #37924, .F. ) ;
#78469=CARTESIAN_POINT ( 'NONE',  ( -22.42236680055709641, 157.8615022471902591, 0.000000000000000000 ) ) ;
#78471=CARTESIAN_POINT ( 'NONE',  ( 174.2976836722478424, 286.0237415149990738, 10.49720334598133498 ) ) ;
#78474=CARTESIAN_POINT ( 'NONE',  ( 208.1612901671020381, 270.1010645919285480, -2.401583477149568768 ) ) ;
#78475=CARTESIAN_POINT ( 'NONE',  ( 194.4263876777154394, 293.8906135405502482, 15.23185943445137802 ) ) ;
#78477=CARTESIAN_POINT ( 'NONE',  ( 204.8878784573704195, 275.7707799872745795, -14.13380496213581594 ) ) ;
#78478=CARTESIAN_POINT ( 'NONE',  ( 148.9967968810750563, 247.6423013555410080, -4.594050593750043987 ) ) ;
#78480=CARTESIAN_POINT ( 'NONE',  ( 172.4171479096595476, 249.8244119910172572, -1.292277060833630919 ) ) ;
#78481=CARTESIAN_POINT ( 'NONE',  ( 81.82518085639701155, 227.2369531367911293, -4.594050593750048428 ) ) ;
#78483=CARTESIAN_POINT ( 'NONE',  ( 191.2056514706806070, 299.4690922889112699, 7.290007621276087590 ) ) ;
#78487=CARTESIAN_POINT ( 'NONE',  ( 195.3218463993883631, 292.3396335385324392, -16.35123038532568174 ) ) ;
#78488=EDGE_LOOP ( 'NONE', ( #38819, #61299, #55537, #93725 ) ) ;
#78493=CARTESIAN_POINT ( 'NONE',  ( 191.3413020738616410, 299.2341385521244774, -8.295023558158421295 ) ) ;
#78496=CARTESIAN_POINT ( 'NONE',  ( 162.5082079047825800, 249.1745225923870919, 11.52567592363465465 ) ) ;
#78497=CARTESIAN_POINT ( 'NONE',  ( 80.49933977867583224, 217.2833772461660544, -9.188101187500095079 ) ) ;
#78498=VERTEX_POINT ( 'NONE', #66955 ) ;
#78500=VERTEX_POINT ( 'NONE', #90316 ) ;
#78501=B_SPLINE_SURFACE_WITH_KNOTS ( 'NONE', 3, 1, ( 
 ( #84075, #37900 ),
 ( #97263, #94160 ),
 ( #70827, #92657 ),
 ( #61211, #93661 ),
 ( #8526, #85579 ),
 ( #23208, #31802 ),
 ( #54098, #38908 ),
 ( #86579, #39395 ),
 ( #1437, #32317 ),
 ( #16616, #23701 ),
 ( #69812, #93150 ),
 ( #54596, #24713 ),
 ( #63218, #85054 ),
 ( #92177, #24225 ),
 ( #70312, #16122 ),
 ( #15602, #62703 ),
 ( #46501, #422 ),
 ( #8035, #45994 ),
 ( #31311, #77438 ),
 ( #62200, #38406 ),
 ( #47020, #15103 ),
 ( #55596, #77935 ),
 ( #925, #55105 ),
 ( #47512, #69320 ),
 ( #86092, #78439 ),
 ( #9020, #39893 ),
 ( #17112, #48010 ),
 ( #78953, #61705 ),
 ( #9542, #68808 ),
 ( #99737, #30323 ),
 ( #22727, #53606 ),
 ( #84565, #76912 ),
 ( #7509, #100241 ),
 ( #30825, #10530 ) ),
 .UNSPECIFIED., .T., .F., .F.,
 ( 4, 2, 2, 2, 2, 2, 2, 2, 2, 2, 2, 2, 2, 2, 2, 2, 4 ),
 ( 2, 2 ),
 ( 0.000000000000000000, 0.06250000000000000000, 0.1250000000000000000, 0.1875000000000000000, 0.2500000000000000000, 0.3125000000000000000, 0.3750000000000000000, 0.4375000000000000000, 0.5000000000000000000, 0.5625000000000000000, 0.6250000000000000000, 0.6875000000000000000, 0.7500000000000000000, 0.8125000000000000000, 0.8750000000000000000, 0.9375000000000000000, 1.000000000000000000 ),
 ( 0.000000000000000000, 1.000000000000000000 ),
 .UNSPECIFIED. ) ;
#78502=CARTESIAN_POINT ( 'NONE',  ( 200.9599690715405984, 282.5741186110587364, -18.15734256570992855 ) ) ;
#78506=CARTESIAN_POINT ( 'NONE',  ( 161.8559746524236118, 283.8847177754445283, 0.5186945926108780247 ) ) ;
#78507=LINE ( 'NONE', #86155, #29938 ) ;
#78510=CARTESIAN_POINT ( 'NONE',  ( 189.8312826409137131, 295.2143506670603301, 11.32827604750477413 ) ) ;
#78512=CARTESIAN_POINT ( 'NONE',  ( 159.3995226465659982, 254.5589234043588078, -16.81133486613867234 ) ) ;
#78513=CARTESIAN_POINT ( 'NONE',  ( 155.5995420464182644, 262.6346450740109617, -17.48312782858739567 ) ) ;
#78514=CARTESIAN_POINT ( 'NONE',  ( 174.6073334282909570, 283.8159819771393018, 13.70195899965856690 ) ) ;
#78515=CARTESIAN_POINT ( 'NONE',  ( 198.9874128674464373, 285.2371454184261097, -17.19338160671415139 ) ) ;
#78520=CARTESIAN_POINT ( 'NONE',  ( 200.1102648775588193, 284.0458494464393198, 17.54251420653697835 ) ) ;
#78522=CARTESIAN_POINT ( 'NONE',  ( 188.0892524428953152, 265.9230919214824667, -13.13131459770854725 ) ) ;
#78525=CARTESIAN_POINT ( 'NONE',  ( 156.7822077518624440, 272.7230075932969839, 14.67370109713490933 ) ) ;
#78529=CARTESIAN_POINT ( 'NONE',  ( 164.9404048476745004, 244.9618339132846074, -2.801285734921658666 ) ) ;
#78530=CARTESIAN_POINT ( 'NONE',  ( 177.8817410463586555, 265.0886103430123057, -15.04724780127894412 ) ) ;
#78532=CARTESIAN_POINT ( 'NONE',  ( 199.5551099226704821, 281.1097900043435516, -17.04800700720547368 ) ) ;
#78534=CARTESIAN_POINT ( 'NONE',  ( 172.3227493250666953, 275.1189843839183027, 16.65430444194719684 ) ) ;
#78535=CARTESIAN_POINT ( 'NONE',  ( -22.42236680055709641, 157.8615022471902591, 0.000000000000000000 ) ) ;
#78536=CARTESIAN_POINT ( 'NONE',  ( 133.5985852126658529, 236.3932355074535963, -2.679491924311248496 ) ) ;
#78538=CARTESIAN_POINT ( 'NONE',  ( 207.8844858873204657, 270.5805036682629066, -6.251308616122969397 ) ) ;
#78539=CARTESIAN_POINT ( 'NONE',  ( -2.476892769303202790, 175.5024278399161233, -9.188101187500093303 ) ) ;
#78541=EDGE_LOOP ( 'NONE', ( #79243, #63501, #40700, #92247 ) ) ;
#78542=CARTESIAN_POINT ( 'NONE',  ( 178.8600085713521537, 256.7301307640913706, 8.633611849901967616 ) ) ;
#78543=FACE_OUTER_BOUND ( 'NONE', #34122, .T. ) ;
#78545=CARTESIAN_POINT ( 'NONE',  ( 19.39059577201889084, 175.8768266524160140, 9.188101187500096856 ) ) ;
#78546=CARTESIAN_POINT ( 'NONE',  ( 169.7005567072155259, 288.7155782076579271, 4.430715832634252394 ) ) ;
#78548=CARTESIAN_POINT ( 'NONE',  ( 122.1317068477954422, 247.9865022471903444, 10.00000000000009415 ) ) ;
#78549=CARTESIAN_POINT ( 'NONE',  ( 99.25420243115651431, 238.1115022471902876, -5.000000000000047962 ) ) ;
#78551=CYLINDRICAL_SURFACE ( 'NONE', #78361, 17.82106496071139645 ) ;
#78553=CARTESIAN_POINT ( 'NONE',  ( 187.5308134497532819, 259.4978860586243741, -0.7759764616068984822 ) ) ;
#78555=EDGE_CURVE ( 'NONE', #65763, #63007, #77442, .T. ) ;
#78557=CARTESIAN_POINT ( 'NONE',  ( 68.07728789491675059, 210.1115022471902591, 10.00000000000009592 ) ) ;
#78558=CARTESIAN_POINT ( 'NONE',  ( 164.5259176133158689, 246.1953198488120051, 1.882264443804981813 ) ) ;
#78560=ADVANCED_FACE ( 'NONE', ( #66 ), #60316, .F. ) ;
#78561=CARTESIAN_POINT ( 'NONE',  ( 24.04513522159523475, 190.8149278399161233, 9.188101187500093303 ) ) ;
#78562=CARTESIAN_POINT ( 'NONE',  ( 198.1300353965528984, 287.4757075181870505, 18.48278456664528946 ) ) ;
#78564=CARTESIAN_POINT ( 'NONE',  ( 203.1536195656275652, 269.7275029030552105, -6.026020274049146863 ) ) ;
#78565=CARTESIAN_POINT ( 'NONE',  ( 151.3999564459286375, 268.4145785023736153, -15.40574304386609050 ) ) ;
#78568=ORIENTED_EDGE ( 'NONE', *, *, #44182, .F. ) ;
#78570=CARTESIAN_POINT ( 'NONE',  ( 202.8096126329844253, 278.9917248286524796, -15.16107960898829532 ) ) ;
#78571=CARTESIAN_POINT ( 'NONE',  ( 205.6622124036295247, 269.3173564635357593, -1.337127560418800654 ) ) ;
#78573=CARTESIAN_POINT ( 'NONE',  ( 202.3894997978090373, 280.0980987621804275, 16.95659012541789323 ) ) ;
#78574=CARTESIAN_POINT ( 'NONE',  ( 149.3801359649374092, 271.9130101976182914, -11.41245530317637424 ) ) ;
#78575=CARTESIAN_POINT ( 'NONE',  ( 188.7310474590576632, 269.8941210489508080, -14.07782309740324500 ) ) ;
#78577=B_SPLINE_CURVE_WITH_KNOTS ( 'NONE', 3,
 ( #83992, #43935, #36843, #61626 ),
 .UNSPECIFIED., .F., .F.,
 ( 4, 4 ),
 ( 0.006037860917506979175, 0.01410894879655490500 ),
 .UNSPECIFIED. ) ;
#78583=CARTESIAN_POINT ( 'NONE',  ( 23.34060026799419063, 195.8297689869269504, -2.679491924311252493 ) ) ;
#78585=B_SPLINE_CURVE_WITH_KNOTS ( 'NONE', 3,
 ( #64114, #24114, #18034, #41805, #95580, #55987, #79370, #2845, #40796, #47895 ),
 .UNSPECIFIED., .F., .F.,
 ( 4, 2, 2, 2, 4 ),
 ( 0.000000000000000000, 0.0004220628552397187377, 0.0008441257104794374754, 0.001266188565719156105, 0.001688251420958874951 ),
 .UNSPECIFIED. ) ;
#78587=CARTESIAN_POINT ( 'NONE',  ( 178.1343968340341348, 256.5670189455112222, -7.272430892715192385 ) ) ;
#78588=ORIENTED_EDGE ( 'NONE', *, *, #21677, .F. ) ;
#78597=CARTESIAN_POINT ( 'NONE',  ( 148.2159754900428936, 273.9293952882992471, 9.267836332806297150 ) ) ;
#78598=CARTESIAN_POINT ( 'NONE',  ( 184.0730272687639513, 288.7302421887371793, -13.16879209019809061 ) ) ;
#78600=CARTESIAN_POINT ( 'NONE',  ( 157.2464636617698375, 258.2881309577184652, 18.14284729738657731 ) ) ;
#78602=ORIENTED_EDGE ( 'NONE', *, *, #28954, .T. ) ;
#78604=CARTESIAN_POINT ( 'NONE',  ( 197.9552487813401456, 287.7784468162186613, 17.26493623863614602 ) ) ;
#78606=CARTESIAN_POINT ( 'NONE',  ( 53.57110205792969282, 210.9244531367911577, -4.594050593750046652 ) ) ;
#78608=( BOUNDED_CURVE ( )  B_SPLINE_CURVE ( 2, ( #789, #23082, #53974, #52995, #83946, #45391, #76321, #6896, #31182 ),
 .UNSPECIFIED., .F., .T. ) 
 B_SPLINE_CURVE_WITH_KNOTS ( ( 3, 2, 2, 2, 3 ),
 ( 0.8669354838709677491, 0.8682795698924731242, 0.8709677419354838745, 0.8736559139784946248, 0.8750000000000000000 ),
 .UNSPECIFIED. ) 
 CURVE ( )  GEOMETRIC_REPRESENTATION_ITEM ( )  RATIONAL_B_SPLINE_CURVE ( ( 0.9330127018922194093, 0.9330127018922194093, 1.000000000000000000, 0.8660254037844387076, 1.000000000000000000, 0.8660254037844387076, 1.000000000000000000, 0.9330127018922194093, 0.9330127018922194093 ) ) 
 REPRESENTATION_ITEM ( '' )  );
#78612=CARTESIAN_POINT ( 'NONE',  ( 176.1305938586311299, 272.9992343613586741, 17.56359532786331457 ) ) ;
#78613=ORIENTED_EDGE ( 'NONE', *, *, #85122, .T. ) ;
#78616=CARTESIAN_POINT ( 'NONE',  ( 189.8533352240220893, 301.8113727360248504, -0.2033756396389863053 ) ) ;
#78617=ORIENTED_EDGE ( 'NONE', *, *, #13960, .T. ) ;
#78618=CARTESIAN_POINT ( 'NONE',  ( 171.7561557084762001, 259.2930754640176474, -13.77066962676198969 ) ) ;
#78619=CARTESIAN_POINT ( 'NONE',  ( 170.6581720520257761, 275.3793360666527974, -16.53181577443977446 ) ) ;
#78620=CARTESIAN_POINT ( 'NONE',  ( 207.7836085030675690, 270.7552284231231852, -5.468305433308493058 ) ) ;
#78621=CARTESIAN_POINT ( 'NONE',  ( 192.8301672656986341, 296.6553483942417415, -13.40355799340913556 ) ) ;
#78622=CARTESIAN_POINT ( 'NONE',  ( 190.7705347155322499, 300.2227366160529414, 3.504769718465625239 ) ) ;
#78624=CARTESIAN_POINT ( 'NONE',  ( 177.1099337379980625, 269.6391827967807444, 16.17709596969117669 ) ) ;
#78625=CARTESIAN_POINT ( 'NONE',  ( 164.5648480107187197, 245.6123174360222094, 3.015887571020871238 ) ) ;
#78626=CARTESIAN_POINT ( 'NONE',  ( 11.60290295393121696, 189.0530062829863027, -4.648177544792955347E-16 ) ) ;
#78628=CARTESIAN_POINT ( 'NONE',  ( 163.7323023463233937, 247.0543288263758086, -6.244751637846886361 ) ) ;
#78629=CARTESIAN_POINT ( 'NONE',  ( 113.2460989071574460, 230.0643266524160140, 9.188101187500095079 ) ) ;
#78633=CARTESIAN_POINT ( 'NONE',  ( 147.2180753513904961, 275.6578090293250511, 0.4909717733184589261 ) ) ;
#78636=AXIS2_PLACEMENT_3D ( 'NONE', #32, #30917, #61804 ) ;
#78637=CARTESIAN_POINT ( 'NONE',  ( 192.5672132233574700, 296.7161803602032819, 11.26440590052197521 ) ) ;
#78640=ORIENTED_EDGE ( 'NONE', *, *, #30157, .F. ) ;
#78641=CARTESIAN_POINT ( 'NONE',  ( 163.4178923001155681, 247.5989030008181260, -10.38047187240561442 ) ) ;
#78642=CARTESIAN_POINT ( 'NONE',  ( 154.5673665054800949, 273.4584833364699534, -13.30136609530668501 ) ) ;
#78643=CARTESIAN_POINT ( 'NONE',  ( 185.6000254797699256, 261.4070812443545151, 10.17022056266204011 ) ) ;
#78645=CARTESIAN_POINT ( 'NONE',  ( 139.3894143317826888, 239.0327760586659736, 1.948934522072302763E-15 ) ) ;
#78646=CARTESIAN_POINT ( 'NONE',  ( 198.7501991201633018, 286.4015524398827779, -18.58948563601804693 ) ) ;
#78647=CARTESIAN_POINT ( 'NONE',  ( 185.9018016517766796, 296.7470552638663435, 4.635871442932423925 ) ) ;
#78648=CARTESIAN_POINT ( 'NONE',  ( 157.8360072705708603, 257.2670114739976839, 17.12122855844125269 ) ) ;
#78649=DIRECTION ( 'NONE',  ( -0.8660254037844387076, -0.4999999999999998890, -0.000000000000000000 ) ) ;
#78650=CARTESIAN_POINT ( 'NONE',  ( 58.36173894231861681, 198.3768266524159856, 9.188101187500098632 ) ) ;
#78656=CARTESIAN_POINT ( 'NONE',  ( 171.1954379026365132, 259.7559371881407060, 15.23461156733691979 ) ) ;
#78657=DIRECTION ( 'NONE',  ( 0.8660254037844323793, 0.5000000000000108802, 1.093569679255778877E-14 ) ) ;
#78658=CARTESIAN_POINT ( 'NONE',  ( 155.6048174803203210, 261.1315455520403361, -17.38645169541727498 ) ) ;
#78659=CARTESIAN_POINT ( 'NONE',  ( 179.7248642212219920, 261.8487014404206548, 12.23902209130197782 ) ) ;
#78660=CARTESIAN_POINT ( 'NONE',  ( 118.5773942495488882, 249.2677522451419065, -5.000000000000047962 ) ) ;
#78663=CARTESIAN_POINT ( 'NONE',  ( 163.4216610345155800, 247.5923753613567442, 10.58669027323842826 ) ) ;
#78665=AXIS2_PLACEMENT_3D ( 'NONE', #97065, #75229, #59490 ) ;
#78666=CARTESIAN_POINT ( 'NONE',  ( 18.30771692152332975, 187.5024278399160949, -9.188101187500093303 ) ) ;
#78668=CARTESIAN_POINT ( 'NONE',  ( 188.7259824843985427, 290.5464306864724335, -14.95866673843798189 ) ) ;
#78673=CARTESIAN_POINT ( 'NONE',  ( 55.71838369152838766, 209.6427522451419350, 10.00000000000009237 ) ) ;
#78674=CARTESIAN_POINT ( 'NONE',  ( 173.5202059484193171, 289.2069962268759582, 8.056742666160944921 ) ) ;
#78676=CARTESIAN_POINT ( 'NONE',  ( 157.1458804504438831, 258.4623461901232417, -17.08829597948888335 ) ) ;
#78677=CARTESIAN_POINT ( 'NONE',  ( 162.2432041231853646, 251.8243937157151322, -12.96429670712563009 ) ) ;
#78679=AXIS2_PLACEMENT_3D ( 'NONE', #88388, #81755, #52299 ) ;
#78680=CARTESIAN_POINT ( 'NONE',  ( 161.4388948769270087, 267.8778111258301919, 16.93954275417836541 ) ) ;
#78681=CARTESIAN_POINT ( 'NONE',  ( 17.48697055717573789, 194.2365022471903728, 2.944929066748280225E-16 ) ) ;
#78682=DIRECTION ( 'NONE',  ( 0.4999999999999995559, -0.8660254037844389297, 0.000000000000000000 ) ) ;
#78683=CARTESIAN_POINT ( 'NONE',  ( 202.3425522658138505, 280.1794142728863903, 15.86053073629060961 ) ) ;
#78684=CARTESIAN_POINT ( 'NONE',  ( -4.262896616726100874, 168.3458772461660544, 9.188101187500095079 ) ) ;
#78686=CARTESIAN_POINT ( 'NONE',  ( 164.0691337515192174, 260.5160139313006766, -16.15666796438198460 ) ) ;
#78687=CARTESIAN_POINT ( 'NONE',  ( 170.8865616681041786, 262.8912071418242817, 16.88624067591380040 ) ) ;
#78690=CARTESIAN_POINT ( 'NONE',  ( 204.1633547645365638, 275.3510256380408237, 13.36249479004741580 ) ) ;
#78691=CARTESIAN_POINT ( 'NONE',  ( 183.2640056662122277, 257.8466347788053099, -2.285499766636972296 ) ) ;
#78694=CARTESIAN_POINT ( 'NONE',  ( 137.7201641159153098, 256.9865022471903444, 10.00000000000009415 ) ) ;
#78696=CARTESIAN_POINT ( 'NONE',  ( 178.4611519391757497, 285.4942648953933144, 12.99929199147914716 ) ) ;
#78697=CARTESIAN_POINT ( 'NONE',  ( 155.8136364298667331, 279.2791936157335044, -5.243594246769619716 ) ) ;
#78699=CARTESIAN_POINT ( 'NONE',  ( 160.6683587774825526, 252.3612347591322020, 15.32470308806421855 ) ) ;
#78702=CARTESIAN_POINT ( 'NONE',  ( 152.6945189806187955, 266.1723304187151484, 16.62409282110771613 ) ) ;
#78703=CARTESIAN_POINT ( 'NONE',  ( 191.8986733338516331, 296.2687432111309249, 12.49828825629462337 ) ) ;
#78705=CARTESIAN_POINT ( 'NONE',  ( 157.5215017335775940, 258.4853116787141971, -16.92298772477023761 ) ) ;
#78713=CARTESIAN_POINT ( 'NONE',  ( 8.953011887168695893, 182.6427522451419350, 10.00000000000009415 ) ) ;
#78715=ORIENTED_EDGE ( 'NONE', *, *, #88434, .F. ) ;
#78717=FACE_OUTER_BOUND ( 'NONE', #90730, .T. ) ;
#78720=CARTESIAN_POINT ( 'NONE',  ( 203.4846675955504907, 278.2012124936790087, 16.44718627781510634 ) ) ;
#78722=CARTESIAN_POINT ( 'NONE',  ( 190.8443993347725325, 300.0947993426467519, 8.522468760355437212 ) ) ;
#78725=LINE ( 'NONE', #80254, #29336 ) ;
#78726=ORIENTED_EDGE ( 'NONE', *, *, #88894, .F. ) ;
#78727=ORIENTED_EDGE ( 'NONE', *, *, #76587, .T. ) ;
#78734=CARTESIAN_POINT ( 'NONE',  ( 148.2670916631250861, 273.8408594794321971, -7.980554973576580835 ) ) ;
#78735=B_SPLINE_CURVE_WITH_KNOTS ( 'NONE', 3,
 ( #73892, #36365, #28778, #44964 ),
 .UNSPECIFIED., .F., .F.,
 ( 4, 4 ),
 ( 0.01084982095175494182, 0.01228877948971598445 ),
 .UNSPECIFIED. ) ;
#78737=CARTESIAN_POINT ( 'NONE',  ( 159.1305972428150710, 255.0247158671010084, -16.79903268104793312 ) ) ;
#78739=CARTESIAN_POINT ( 'NONE',  ( 167.0389919848387592, 247.0514236948299072, 1.939505287189084326 ) ) ;
#78745=CARTESIAN_POINT ( 'NONE',  ( 159.2077906806335932, 254.8910129107889588, 16.14624949541834553 ) ) ;
#78748=CARTESIAN_POINT ( 'NONE',  ( 190.6257723682618064, 300.4734723565479158, 5.229856753389036328 ) ) ;
#78750=CARTESIAN_POINT ( 'NONE',  ( 159.9770824720811220, 253.5585604421560788, -16.42166711341322483 ) ) ;
#78751=CARTESIAN_POINT ( 'NONE',  ( 161.1252381510204259, 272.2179608743590506, -16.27752944574491778 ) ) ;
#78752=EDGE_CURVE ( 'NONE', #73362, #24288, #92090, .T. ) ;
#78753=CARTESIAN_POINT ( 'NONE',  ( 161.8016137473484548, 250.3983795733946636, 14.25000412375400316 ) ) ;
#78754=CARTESIAN_POINT ( 'NONE',  ( 190.8174609004742592, 261.9199525876146595, -0.4327646785539380758 ) ) ;
#78756=CARTESIAN_POINT ( 'NONE',  ( 187.5197201530054656, 260.4900132203839576, 7.667313317775144021 ) ) ;
#78758=CARTESIAN_POINT ( 'NONE',  ( 164.8251969117060298, 245.1613799118173063, -1.508678420156898348 ) ) ;
#78759=ADVANCED_FACE ( 'NONE', ( #40319 ), #24829, .F. ) ;
#78760=CARTESIAN_POINT ( 'NONE',  ( 7.293129863248505984, 185.0177522451419065, 5.000000000000046185 ) ) ;
#78761=CARTESIAN_POINT ( 'NONE',  ( 92.62404252742300059, 212.0327760586659451, 1.948934522072302763E-15 ) ) ;
#78764=CARTESIAN_POINT ( 'NONE',  ( 168.2168545625571596, 279.0239035984992597, -13.38986689698590737 ) ) ;
#78765=CARTESIAN_POINT ( 'NONE',  ( 8.998290926605619688, 169.8768266524160140, 9.188101187500098632 ) ) ;
#78767=CARTESIAN_POINT ( 'NONE',  ( 161.1611771195837548, 251.5076483517112536, 14.17749514252127163 ) ) ;
#78773=CARTESIAN_POINT ( 'NONE',  ( 188.4359633627616404, 260.4672849544427322, -6.269197070210934974 ) ) ;
#78777=CARTESIAN_POINT ( 'NONE',  ( 38.19941146435361645, 192.8615022471902591, -10.00000000000009592 ) ) ;
#78780=CARTESIAN_POINT ( 'NONE',  ( 36.16983797034238535, 185.5643266524159856, -9.188101187500093303 ) ) ;
#78781=CARTESIAN_POINT ( 'NONE',  ( 76.50299338235490154, 221.6427522451419065, 10.00000000000009237 ) ) ;
#78782=CARTESIAN_POINT ( 'NONE',  ( 196.1813314310145415, 275.5097970061073056, 15.45116200187350586 ) ) ;
#78783=ORIENTED_EDGE ( 'NONE', *, *, #51113, .T. ) ;
#78784=CARTESIAN_POINT ( 'NONE',  ( 153.5359445101103404, 274.1292087801049888, -12.02885945652445976 ) ) ;
#78785=CARTESIAN_POINT ( 'NONE',  ( 175.1707756323828846, 281.3988818488836046, -14.22492014867428090 ) ) ;
#78786=CARTESIAN_POINT ( 'NONE',  ( -11.73236572436687730, 164.0333772461660544, 9.188101187500095079 ) ) ;
#78789=CARTESIAN_POINT ( 'NONE',  ( 151.1126408083691501, 268.9122237844355254, -15.82705194100464396 ) ) ;
#78790=CARTESIAN_POINT ( 'NONE',  ( 187.5768131394391958, 283.2038405381267125, 16.23894686413832034 ) ) ;
#78791=CARTESIAN_POINT ( 'NONE',  ( 194.4666154385731431, 293.8209370148700827, -14.56896502715340702 ) ) ;
#78794=CARTESIAN_POINT ( 'NONE',  ( 189.7252522328423368, 262.4931234074404642, 8.270058708727324515 ) ) ;
#78795=CARTESIAN_POINT ( 'NONE',  ( 163.9587364689194260, 246.6621334214722481, 5.816126667419880825 ) ) ;
#78796=CARTESIAN_POINT ( 'NONE',  ( 148.0389988358468827, 274.2359278451201590, 7.783622668412842671 ) ) ;
#78797=ORIENTED_EDGE ( 'NONE', *, *, #74352, .F. ) ;
#78798=CARTESIAN_POINT ( 'NONE',  ( 156.0916382163451601, 277.5285333452508212, -10.52960063827285886 ) ) ;
#78799=CARTESIAN_POINT ( 'NONE',  ( 208.2764314485352770, 269.9016340424377063, 2.433736665191914117 ) ) ;
#78800=CARTESIAN_POINT ( 'NONE',  ( 181.2716795336521329, 267.9920306002611028, 16.35033316730358877 ) ) ;
#78801=CARTESIAN_POINT ( 'NONE',  ( 106.9945647975297760, 223.3923013555410080, 4.594050593750050204 ) ) ;
#78803=CARTESIAN_POINT ( 'NONE',  ( 191.0900422946452011, 299.6693332556258724, 8.872191398975367349 ) ) ;
#78804=EDGE_CURVE ( 'NONE', #91470, #38315, #69054, .T. ) ;
#78806=CARTESIAN_POINT ( 'NONE',  ( 195.6974783896144174, 291.6890198465123945, 16.70600479393688431 ) ) ;
#78807=CARTESIAN_POINT ( 'NONE',  ( 166.5418805794664934, 264.7512503615053561, 17.71810435351582669 ) ) ;
#78808=FACE_OUTER_BOUND ( 'NONE', #11099, .T. ) ;
#78811=CARTESIAN_POINT ( 'NONE',  ( 196.8104339078508076, 289.7613243423628546, -16.40335862274955403 ) ) ;
#78812=AXIS2_PLACEMENT_3D ( 'NONE', #22658, #44942, #84004 ) ;
#78814=CARTESIAN_POINT ( 'NONE',  ( 173.2147484828852839, 289.7388750556115724, -1.099818896463917284 ) ) ;
#78820=CARTESIAN_POINT ( 'NONE',  ( 186.5128128464827455, 296.3652354721813822, -8.829210103799347564 ) ) ;
#78824=B_SPLINE_SURFACE_WITH_KNOTS ( 'NONE', 3, 1, ( 
 ( #52100, #44491 ),
 ( #82565, #98737 ),
 ( #29315, #85034 ),
 ( #99716, #8999 ),
 ( #403, #94139 ),
 ( #6997, #47985 ),
 ( #70808, #54573 ),
 ( #8505, #15580 ),
 ( #30305, #85557 ),
 ( #92639, #32296 ),
 ( #61687, #22711 ),
 ( #46483, #84545 ),
 ( #63199, #45975 ),
 ( #23681, #77414 ),
 ( #8017, #37881 ),
 ( #16099, #902 ),
 ( #86071, #62178 ),
 ( #23188, #38386 ),
 ( #53589, #68791 ),
 ( #15087, #100222 ),
 ( #54081, #55085 ),
 ( #39375, #61190 ),
 ( #24694, #69298 ),
 ( #70291, #17092 ),
 ( #39870, #30807 ),
 ( #47002, #38891 ),
 ( #31781, #77916 ),
 ( #55577, #86559 ),
 ( #62683, #92158 ),
 ( #69793, #76892 ),
 ( #31292, #93132 ),
 ( #93636, #24204 ),
 ( #16596, #7492 ),
 ( #47492, #78417 ) ),
 .UNSPECIFIED., .T., .F., .F.,
 ( 4, 2, 2, 2, 2, 2, 2, 2, 2, 2, 2, 2, 2, 2, 2, 2, 4 ),
 ( 2, 2 ),
 ( 0.000000000000000000, 0.06250000000000000000, 0.1250000000000000000, 0.1875000000000000000, 0.2500000000000000000, 0.3125000000000000000, 0.3750000000000000000, 0.4375000000000000000, 0.5000000000000000000, 0.5625000000000000000, 0.6250000000000000000, 0.6875000000000000000, 0.7500000000000000000, 0.8125000000000000000, 0.8750000000000000000, 0.9375000000000000000, 1.000000000000000000 ),
 ( 0.000000000000000000, 1.000000000000000000 ),
 .UNSPECIFIED. ) ;
#78826=CARTESIAN_POINT ( 'NONE',  ( 182.7235263772020346, 258.7439045234889932, -9.311915605583727995 ) ) ;
#78827=CARTESIAN_POINT ( 'NONE',  ( 189.2759868517105986, 283.1334299989923124, 17.63300985876514915 ) ) ;
#78828=CARTESIAN_POINT ( 'NONE',  ( 153.4242699508872647, 264.9083646613370320, 16.62000820703435267 ) ) ;
#78831=CARTESIAN_POINT ( 'NONE',  ( 161.6059911608744812, 269.3330164776378410, -17.24104619120290494 ) ) ;
#78833=CARTESIAN_POINT ( 'NONE',  ( 177.2074197889685365, 274.7965786531511867, -16.93324248537096111 ) ) ;
#78834=ORIENTED_EDGE ( 'NONE', *, *, #43523, .F. ) ;
#78835=CARTESIAN_POINT ( 'NONE',  ( 167.7018358744333000, 280.9558910960651019, 11.69324581573506805 ) ) ;
#78838=ORIENTED_EDGE ( 'NONE', *, *, #78804, .F. ) ;
#78840=FACE_OUTER_BOUND ( 'NONE', #73461, .T. ) ;
#78841=CARTESIAN_POINT ( 'NONE',  ( 66.61587002248261058, 209.2677522451418497, 10.00000000000009592 ) ) ;
#78845=CIRCLE ( 'NONE', #73994, 17.82106496071138935 ) ;
#78848=CARTESIAN_POINT ( 'NONE',  ( 155.6281496932864457, 261.0911329737299980, -18.07904265579665548 ) ) ;
#78850=ORIENTED_EDGE ( 'NONE', *, *, #16354, .T. ) ;
#78851=CARTESIAN_POINT ( 'NONE',  ( 178.9732493734400407, 260.1133086608659823, 12.29518698491872186 ) ) ;
#78859=CARTESIAN_POINT ( 'NONE',  ( 165.0803978706131545, 244.7193588848498678, -1.793249961207334486 ) ) ;
#78861=CARTESIAN_POINT ( 'NONE',  ( 196.4404618256887147, 284.6410079857341771, -17.31378922566917211 ) ) ;
#78863=CARTESIAN_POINT ( 'NONE',  ( 167.9449114283013955, 248.6326271889187751, -4.934543203145975276 ) ) ;
#78865=CARTESIAN_POINT ( 'NONE',  ( 153.8909117540673037, 279.9112642337403258, 2.216438095792761409 ) ) ;
#78866=B_SPLINE_CURVE_WITH_KNOTS ( 'NONE', 3,
 ( #2933, #33822, #50983, #4911 ),
 .UNSPECIFIED., .F., .F.,
 ( 4, 4 ),
 ( 0.008486201099387760682, 0.01670945231454646837 ),
 .UNSPECIFIED. ) ;
#78867=CARTESIAN_POINT ( 'NONE',  ( 124.8563387505838165, 233.7048013555409796, 4.594050593750051981 ) ) ;
#78868=B_SPLINE_CURVE_WITH_KNOTS ( 'NONE', 3,
 ( #22800, #53679, #6608, #20828 ),
 .UNSPECIFIED., .F., .F.,
 ( 4, 4 ),
 ( 0.01467339918438643684, 0.02339405670009707047 ),
 .UNSPECIFIED. ) ;
#78869=CARTESIAN_POINT ( 'NONE',  ( 183.4730159057174319, 260.4080488702623484, -9.317792726801004122 ) ) ;
#78871=VERTEX_POINT ( 'NONE', #98423 ) ;
#78875=CARTESIAN_POINT ( 'NONE',  ( 203.4267045473674500, 276.1086550667716324, 13.32450178018177844 ) ) ;
#78876=DIRECTION ( 'NONE',  ( 0.4999999999999998890, -0.8660254037844385966, 0.000000000000000000 ) ) ;
#78878=CARTESIAN_POINT ( 'NONE',  ( 173.8731466349179016, 289.7565554419105069, -4.721349978305271478 ) ) ;
#78879=CARTESIAN_POINT ( 'NONE',  ( 147.3488861203839235, 275.4312381312514049, 3.942095418248577676 ) ) ;
#78882=CARTESIAN_POINT ( 'NONE',  ( 173.8535554309253257, 287.2246996319072423, -9.538136335621828721 ) ) ;
#78883=CARTESIAN_POINT ( 'NONE',  ( 194.9515580553570260, 292.9809917638447132, 16.65666034366562798 ) ) ;
#78884=CARTESIAN_POINT ( 'NONE',  ( 177.1268731193232497, 255.9947964353676468, -7.287581347330274184 ) ) ;
#78885=ORIENTED_EDGE ( 'NONE', *, *, #16316, .F. ) ;
#78886=CARTESIAN_POINT ( 'NONE',  ( 147.6095889327917803, 274.9796876144846465, -8.460961150142429332 ) ) ;
#78890=EDGE_CURVE ( 'NONE', #15755, #66560, #60419, .T. ) ;
#78891=CARTESIAN_POINT ( 'NONE',  ( 191.0209356936215386, 283.3490554861720625, -16.57420257736403713 ) ) ;
#78892=CARTESIAN_POINT ( 'NONE',  ( 152.2897644507763459, 266.8733858289956515, -15.49661418983042083 ) ) ;
#78893=CARTESIAN_POINT ( 'NONE',  ( 148.9266665119372703, 272.6984423298952152, 12.06339424062075061 ) ) ;
#78895=CARTESIAN_POINT ( 'NONE',  ( 202.7599932440484451, 279.4563852894229967, 15.58249343055423353 ) ) ;
#78896=CARTESIAN_POINT ( 'NONE',  ( 153.4014598655621739, 270.1403366047916847, 14.11843096852130941 ) ) ;
#78897=CARTESIAN_POINT ( 'NONE',  ( 151.5138970483880030, 274.8970949040892719, -9.081682327913926045 ) ) ;
#78898=CARTESIAN_POINT ( 'NONE',  ( 153.0790963368640689, 265.5062228982576471, -17.74594954892339160 ) ) ;
#78900=CARTESIAN_POINT ( 'NONE',  ( 205.1662051911351057, 272.1315205505885046, -9.477979197527140798 ) ) ;
#78901=CARTESIAN_POINT ( 'NONE',  ( 187.4088158364907315, 261.5390839597025092, -9.233908393253857483 ) ) ;
#78902=CARTESIAN_POINT ( 'NONE',  ( 193.4438847740023846, 276.1245385600062718, -16.33226197978559213 ) ) ;
#78905=CARTESIAN_POINT ( 'NONE',  ( 188.0737869051473012, 299.5124861214166572, -3.734995909225475863 ) ) ;
#78908=CARTESIAN_POINT ( 'NONE',  ( -27.42236680055714260, 166.5217562850347406, 1.224646799147364892E-15 ) ) ;
#78909=CIRCLE ( 'NONE', #22251, 17.82106496071138224 ) ;
#78910=( BOUNDED_CURVE ( )  B_SPLINE_CURVE ( 2, ( #37388, #75932, #84539, #75418, #60176, #28806, #29801, #91141, #21217 ),
 .UNSPECIFIED., .F., .T. ) 
 B_SPLINE_CURVE_WITH_KNOTS ( ( 3, 2, 2, 2, 3 ),
 ( 0.8024193548387096309, 0.8037634408602150060, 0.8064516129032257563, 0.8091397849462365066, 0.8104838709677418818 ),
 .UNSPECIFIED. ) 
 CURVE ( )  GEOMETRIC_REPRESENTATION_ITEM ( )  RATIONAL_B_SPLINE_CURVE ( ( 0.9330127018922194093, 0.9330127018922194093, 1.000000000000000000, 0.8660254037844387076, 1.000000000000000000, 0.8660254037844387076, 1.000000000000000000, 0.9330127018922194093, 0.9330127018922194093 ) ) 
 REPRESENTATION_ITEM ( '' )  );
#78912=CARTESIAN_POINT ( 'NONE',  ( 166.2786170299253854, 246.9376851968044377, -4.638038840367427085 ) ) ;
#78913=CARTESIAN_POINT ( 'NONE',  ( -5.237175195983594378, 167.7833772461660828, -9.188101187500095079 ) ) ;
#78914=CARTESIAN_POINT ( 'NONE',  ( 83.31357524521028779, 231.1589784336661637, -6.496448406907675876E-16 ) ) ;
#78916=CARTESIAN_POINT ( 'NONE',  ( 182.2373335159190901, 280.9600371166583841, -17.30031729693378040 ) ) ;
#78918=CARTESIAN_POINT ( 'NONE',  ( 202.9490938173916561, 279.1288534886517709, -16.56031645010252973 ) ) ;
#78919=CIRCLE ( 'NONE', #35214, 17.82106496071138224 ) ;
#78921=CYLINDRICAL_SURFACE ( 'NONE', #4475, 17.82106496071139645 ) ;
#78923=CARTESIAN_POINT ( 'NONE',  ( 165.8866640751390094, 265.8956478032751534, 17.81115609982314751 ) ) ;
#78924=CARTESIAN_POINT ( 'NONE',  ( 190.0047355206681914, 300.4812981626290593, -1.397688852404484372 ) ) ;
#78925=CARTESIAN_POINT ( 'NONE',  ( 162.6541320028305506, 248.9217746405196294, -10.16950121496441817 ) ) ;
#78926=CARTESIAN_POINT ( 'NONE',  ( 178.2461545249785502, 289.9108068321567657, 9.551079046322911381 ) ) ;
#78933=CARTESIAN_POINT ( 'NONE',  ( 42.04265951369687571, 185.8923013555410080, 4.594050593750050204 ) ) ;
#78936=CARTESIAN_POINT ( 'NONE',  ( 66.56148311469628709, 218.4244531367911293, -4.594050593750046652 ) ) ;
#78937=CARTESIAN_POINT ( 'NONE',  ( 164.2137379661740795, 246.9428399464227937, -5.807035987355257944 ) ) ;
#78940=CARTESIAN_POINT ( 'NONE',  ( 166.6394175675808356, 259.6070987380002180, 15.76739866228208165 ) ) ;
#78941=CYLINDRICAL_SURFACE ( 'NONE', #82464, 17.82106496071139645 ) ;
#78943=CARTESIAN_POINT ( 'NONE',  ( 175.3932935011599170, 269.2958584618301643, -17.65833184418574930 ) ) ;
#78946=CARTESIAN_POINT ( 'NONE',  ( 198.4344074287054696, 286.9485196940960918, -17.83642855442570152 ) ) ;
#78947=CARTESIAN_POINT ( 'NONE',  ( 196.7491951525289835, 289.8673929779723721, -16.35352603081977207 ) ) ;
#78950=CARTESIAN_POINT ( 'NONE',  ( 63.63864737692379236, 216.7369531367911293, -4.594050593750048428 ) ) ;
#78952=CARTESIAN_POINT ( 'NONE',  ( 155.4810912439522212, 261.3458456796594760, -18.44218279064527266 ) ) ;
#78953=CARTESIAN_POINT ( 'NONE',  ( 198.6012358295098750, 286.6595644277572887, 18.21911298807435386 ) ) ;
#78955=CARTESIAN_POINT ( 'NONE',  ( 201.8747764691672728, 280.9896257192293660, 16.31383242165743042 ) ) ;
#78959=CARTESIAN_POINT ( 'NONE',  ( 123.9359264390130591, 242.3615022471902591, -10.00000000000009592 ) ) ;
#78961=CARTESIAN_POINT ( 'NONE',  ( 207.6900289502458179, 270.9173129631602706, 7.178327969100043227 ) ) ;
#78965=CARTESIAN_POINT ( 'NONE',  ( 188.1911093852794465, 273.3801814407030406, 15.63271712328260676 ) ) ;
#78967=CARTESIAN_POINT ( 'NONE',  ( 206.1408608592916494, 273.6005508061571732, -10.42739367433323494 ) ) ;
#78968=CARTESIAN_POINT ( 'NONE',  ( 153.3999530563582425, 279.9403317724381282, -0.6565603302638768346 ) ) ;
#78970=ORIENTED_EDGE ( 'NONE', *, *, #86343, .F. ) ;
#78974=CARTESIAN_POINT ( 'NONE',  ( 40.29776668260214478, 205.6199935810941213, 2.679491924311251605 ) ) ;
#78975=CARTESIAN_POINT ( 'NONE',  ( 148.7030012686772977, 273.8011336086232177, 8.646799806445988779 ) ) ;
#78978=AXIS2_PLACEMENT_3D ( 'NONE', #28598, #19544, #50405 ) ;
#78984=CARTESIAN_POINT ( 'NONE',  ( 206.6703863510205679, 272.6833857505801006, -10.72500664779635393 ) ) ;
#78985=ORIENTED_EDGE ( 'NONE', *, *, #41701, .F. ) ;
#78987=CARTESIAN_POINT ( 'NONE',  ( 186.2526055351975174, 298.2835612753726764, 1.053363499427862449 ) ) ;
#78990=CARTESIAN_POINT ( 'NONE',  ( 194.2223991963907963, 294.2439319543634610, -14.97294938100067441 ) ) ;
#78992=CARTESIAN_POINT ( 'NONE',  ( 185.4350764609872897, 292.4497694977334845, -11.01741108579075856 ) ) ;
#78993=CARTESIAN_POINT ( 'NONE',  ( 204.6713671561005299, 276.1457885614869951, -12.94307097876490431 ) ) ;
#78994=CARTESIAN_POINT ( 'NONE',  ( 145.9657079678295020, 245.8923013555409511, 4.594050593750050204 ) ) ;
#78997=CARTESIAN_POINT ( 'NONE',  ( 149.8050492866161392, 271.5723974896224604, -11.69608657949948061 ) ) ;
#78998=CARTESIAN_POINT ( 'NONE',  ( 85.37073267496330686, 220.0958772461660544, -9.188101187500095079 ) ) ;
#79000=CARTESIAN_POINT ( 'NONE',  ( 150.7226148805041817, 269.5877685077668957, 15.52819754351937576 ) ) ;
#79003=CARTESIAN_POINT ( 'NONE',  ( 195.3220404309544449, 292.3392974660017103, -16.60012830897328229 ) ) ;
#79008=CARTESIAN_POINT ( 'NONE',  ( 146.5865263025993954, 276.7516840693029962, 0.4918294119671828835 ) ) ;
#79009=CARTESIAN_POINT ( 'NONE',  ( 164.1514498073476034, 249.9675132558865016, 10.20859178390983324 ) ) ;
#79011=CARTESIAN_POINT ( 'NONE',  ( 162.5705829494080490, 249.0664858459717550, 10.39261705965051341 ) ) ;
#79012=CARTESIAN_POINT ( 'NONE',  ( 83.61187889534991768, 209.8923013555409796, 4.594050593750050204 ) ) ;
#79015=CARTESIAN_POINT ( 'NONE',  ( 161.2503778443652607, 251.3531481643174743, -13.44633621139661095 ) ) ;
#79016=ORIENTED_EDGE ( 'NONE', *, *, #53442, .F. ) ;
#79017=B_SPLINE_CURVE_WITH_KNOTS ( 'NONE', 3,
 ( #52946, #46321, #85393, #91484, #30145, #7338, #37246, #53921, #30654, #36745, #67653, #13959, #84884, #77247, #7853, #44839, #45341, #75276, #61538, #45823, #76272, #61030, #52446, #44345, #98584, #38735, #69639, #6846, #247, #31128, #62021, #37731, #60035, #22550, #53435, #5860, #29167, #23527, #54417, #84386, #14932, #92481, #54938, #71675, #55419, #64047, #85915, #93484 ),
 .UNSPECIFIED., .F., .F.,
 ( 4, 2, 2, 2, 2, 2, 2, 2, 2, 2, 2, 2, 2, 2, 2, 2, 2, 2, 2, 2, 2, 2, 2, 4 ),
 ( 0.001794995322932195925, 0.002245303848294032383, 0.002695612373655869275, 0.002808189504996264421, 0.002920766636336659568, 0.003033343767677054714, 0.003145920899017449427, 0.003371075161698240154, 0.003596229424379030447, 0.004046537949740726392, 0.004496846475102421470, 0.005397463525825844585, 0.006298080576549267701, 0.006748389101911021759, 0.007198697627272777552, 0.007311274758613178770, 0.007367563324283427084, 0.007423851889953675398, 0.007536429021294069677, 0.007649006152634463956, 0.008099314677995971684, 0.008549623203357479412, 0.008774777466038235010, 0.008999931728718987139 ),
 .UNSPECIFIED. ) ;
#79020=CARTESIAN_POINT ( 'NONE',  ( 164.9191543487298190, 285.0012716261463197, 0.5041077705605265802 ) ) ;
#79021=CARTESIAN_POINT ( 'NONE',  ( 104.4503548538631890, 231.1115022471902307, 10.00000000000009592 ) ) ;
#79024=CARTESIAN_POINT ( 'NONE',  ( 191.7321250286022121, 296.2108873932954225, 11.25078612220933927 ) ) ;
#79026=CARTESIAN_POINT ( 'NONE',  ( 206.1615484827472358, 273.5647187912443314, -9.556459874778100883 ) ) ;
#79027=CARTESIAN_POINT ( 'NONE',  ( 148.0706186424908140, 275.6441064196449702, -5.227547594756374316 ) ) ;
#79028=CARTESIAN_POINT ( 'NONE',  ( 175.0425229888917045, 283.7493962866749939, 13.34536946309205341 ) ) ;
#79029=EDGE_CURVE ( 'NONE', #43553, #98181, #89038, .T. ) ;
#79030=DIRECTION ( 'NONE',  ( 0.4999999999999992784, -0.8660254037844390407, 0.000000000000000000 ) ) ;
#79031=ADVANCED_FACE ( 'NONE', ( #25390 ), #47183, .T. ) ;
#79032=CARTESIAN_POINT ( 'NONE',  ( 195.4920518568790158, 279.6224761531880176, -17.31986585614815866 ) ) ;
#79033=ORIENTED_EDGE ( 'NONE', *, *, #41012, .F. ) ;
#79035=CARTESIAN_POINT ( 'NONE',  ( 161.8016137473484548, 250.3983795733946636, 14.25000412375400316 ) ) ;
#79038=CARTESIAN_POINT ( 'NONE',  ( 187.9510599096114163, 266.1630128281000793, -12.95057174692511204 ) ) ;
#79040=CARTESIAN_POINT ( 'NONE',  ( 177.5604642151115513, 291.0442495137150445, -6.142901185704334743 ) ) ;
#79041=CARTESIAN_POINT ( 'NONE',  ( 155.1439221426048505, 271.2780826592891685, 14.03075285333380862 ) ) ;
#79045=AXIS2_PLACEMENT_3D ( 'NONE', #16307, #24411, #86267 ) ;
#79047=CARTESIAN_POINT ( 'NONE',  ( 180.7542070542261854, 266.7828525480385338, -16.22133153096915947 ) ) ;
#79049=CARTESIAN_POINT ( 'NONE',  ( 199.4856116213349537, 281.2262712591287936, -16.83883655570358684 ) ) ;
#79051=CARTESIAN_POINT ( 'NONE',  ( 99.82359446507273049, 216.8932355074535394, -2.679491924311248496 ) ) ;
#79052=CARTESIAN_POINT ( 'NONE',  ( 168.8894219329319242, 272.9552995970117308, 15.96619431876584017 ) ) ;
#79053=CARTESIAN_POINT ( 'NONE',  ( 180.4080136573045365, 272.9691542711491365, 17.06805577271178365 ) ) ;
#79055=B_SPLINE_CURVE_WITH_KNOTS ( 'NONE', 3,
 ( #11706, #27398, #96833, #34975, #89255, #74002 ),
 .UNSPECIFIED., .F., .F.,
 ( 4, 2, 4 ),
 ( 0.02234597899312508462, 0.02694808822545060809, 0.03155019745777613155 ),
 .UNSPECIFIED. ) ;
#79056=CARTESIAN_POINT ( 'NONE',  ( 205.9449877905329345, 273.5527750745989692, -9.681680776101762476 ) ) ;
#79057=CARTESIAN_POINT ( 'NONE',  ( 207.8575108622103755, 270.6272257822888037, -6.381720258959569847 ) ) ;
#79060=CARTESIAN_POINT ( 'NONE',  ( -1.340060878953613477, 170.0333772461660828, 9.188101187500095079 ) ) ;
#79063=CARTESIAN_POINT ( 'NONE',  ( 178.7466306158354712, 256.8873838365522602, 8.522590757080182655 ) ) ;
#79064=EDGE_CURVE ( 'NONE', #74614, #77581, #88324, .T. ) ;
#79067=B_SPLINE_CURVE_WITH_KNOTS ( 'NONE', 3,
 ( #43480, #59160, #36380, #83032 ),
 .UNSPECIFIED., .F., .F.,
 ( 4, 4 ),
 ( 0.009153972151010242309, 0.01742534041516074009 ),
 .UNSPECIFIED. ) ;
#79068=CARTESIAN_POINT ( 'NONE',  ( 11.67712314985746858, 186.7369531367911293, -4.594050593750048428 ) ) ;
#79071=CARTESIAN_POINT ( 'NONE',  ( 178.7121136867105804, 291.7201401133655168, 6.070087115661351618 ) ) ;
#79072=CARTESIAN_POINT ( 'NONE',  ( 105.8215617431885534, 225.2365022471902023, -10.00000000000009237 ) ) ;
#79073=CARTESIAN_POINT ( 'NONE',  ( 148.9742902571590264, 272.6159555835243964, 12.12504745624938529 ) ) ;
#79074=CARTESIAN_POINT ( 'NONE',  ( 152.7122812589697958, 277.9324518551267147, 6.933031942251369983 ) ) ;
#79075=DIRECTION ( 'NONE',  ( -0.8660254037844387076, -0.4999999999999998890, -0.000000000000000000 ) ) ;
#79076=B_SPLINE_SURFACE_WITH_KNOTS ( 'NONE', 3, 1, ( 
 ( #95541, #40259 ),
 ( #95025, #72202 ),
 ( #88442, #17477 ),
 ( #86439, #19002 ),
 ( #32674, #80322 ),
 ( #47856, #2807 ),
 ( #33695, #10390 ),
 ( #71199, #55454 ),
 ( #8874, #72715 ),
 ( #48386, #57462 ),
 ( #70671, #16966 ),
 ( #10892, #79823 ),
 ( #48889, #1286 ),
 ( #32170, #41768 ),
 ( #64080, #87949 ),
 ( #63574, #3304 ),
 ( #79330, #63074 ),
 ( #94017, #78795 ),
 ( #94518, #64588 ),
 ( #1792, #71706 ),
 ( #26088, #87463 ),
 ( #9898, #56963 ),
 ( #18493, #34184 ),
 ( #2299, #65077 ),
 ( #33181, #25587 ),
 ( #96027, #56474 ),
 ( #49877, #98492 ),
 ( #74201, #35167 ),
 ( #36157, #3789 ),
 ( #65572, #4269 ),
 ( #89910, #51361 ),
 ( #11407, #34670 ),
 ( #74699, #12899 ),
 ( #96519, #59442 ) ),
 .UNSPECIFIED., .T., .F., .F.,
 ( 4, 2, 2, 2, 2, 2, 2, 2, 2, 2, 2, 2, 2, 2, 2, 2, 4 ),
 ( 2, 2 ),
 ( 0.000000000000000000, 0.06250000000000000000, 0.1250000000000000000, 0.1875000000000000000, 0.2500000000000000000, 0.3125000000000000000, 0.3750000000000000000, 0.4375000000000000000, 0.5000000000000000000, 0.5625000000000000000, 0.6250000000000000000, 0.6875000000000000000, 0.7500000000000000000, 0.8125000000000000000, 0.8750000000000000000, 0.9375000000000000000, 1.000000000000000000 ),
 ( 0.000000000000000000, 1.000000000000000000 ),
 .UNSPECIFIED. ) ;
#79078=CARTESIAN_POINT ( 'NONE',  ( 190.1127736092558962, 298.7324422743296850, -8.109491230568453446 ) ) ;
#79080=CARTESIAN_POINT ( 'NONE',  ( 193.0124118986755093, 295.6209498147566137, -12.68620708360851701 ) ) ;
#79081=CARTESIAN_POINT ( 'NONE',  ( 68.51030059680894624, 220.3615022471903160, 5.000000000000046185 ) ) ;
#79082=CARTESIAN_POINT ( 'NONE',  ( 203.7690284654797210, 275.7086850192775955, -13.99192714286714612 ) ) ;
#79083=CARTESIAN_POINT ( 'NONE',  ( 164.4706844205170171, 281.1311524026570510, 11.86625682173560925 ) ) ;
#79085=CARTESIAN_POINT ( 'NONE',  ( 30.64892602121659593, 182.3768266524159856, -9.188101187500091527 ) ) ;
#79086=CARTESIAN_POINT ( 'NONE',  ( 197.9952413503812352, 287.7091776547143809, 17.17611241386010690 ) ) ;
#79087=CARTESIAN_POINT ( 'NONE',  ( 64.90981964964726103, 219.8297689869269504, -2.679491924311252493 ) ) ;
#79090=ORIENTED_EDGE ( 'NONE', *, *, #23090, .F. ) ;
#79095=CARTESIAN_POINT ( 'NONE',  ( 202.4323889586180201, 280.0238125565655878, 15.69595176008160919 ) ) ;
#79096=CARTESIAN_POINT ( 'NONE',  ( 196.5114383562724072, 290.2791998289336561, -17.87308875047256862 ) ) ;
#79097=CARTESIAN_POINT ( 'NONE',  ( 185.5448903953628985, 267.7045173717977491, -14.56276892697053071 ) ) ;
#79098=ORIENTED_EDGE ( 'NONE', *, *, #84522, .F. ) ;
#79100=CARTESIAN_POINT ( 'NONE',  ( 189.7094295309238419, 300.0606247079692253, 5.078421157105148076 ) ) ;
#79104=CARTESIAN_POINT ( 'NONE',  ( 31.70422093597037616, 179.1115022471902023, -5.000000000000041744 ) ) ;
#79108=CARTESIAN_POINT ( 'NONE',  ( 149.2511585606875428, 272.1364056148075292, 11.40684181024752242 ) ) ;
#79109=ADVANCED_FACE ( 'NONE', ( #62883 ), #44126, .F. ) ;
#79110=ORIENTED_EDGE ( 'NONE', *, *, #15583, .T. ) ;
#79112=B_SPLINE_CURVE_WITH_KNOTS ( 'NONE', 3,
 ( #4406, #28705, #97153, #74833, #81944, #82948, #73812, #51500, #82469, #28199, #27719, #58587 ),
 .UNSPECIFIED., .F., .F.,
 ( 4, 2, 2, 2, 2, 4 ),
 ( 7.844548453170152250E-15, 0.0004651973059127275886, 0.0009303946118176106492, 0.001395591917722493547, 0.001628190570674949416, 0.001860789223627405285 ),
 .UNSPECIFIED. ) ;
#79113=CARTESIAN_POINT ( 'NONE',  ( 161.8926315922002743, 250.2407320417157166, -13.77020595223768495 ) ) ;
#79122=CARTESIAN_POINT ( 'NONE',  ( 204.9184781223158609, 275.7177798128946620, -12.59106622113254126 ) ) ;
#79123=CARTESIAN_POINT ( 'NONE',  ( 108.9159718882352479, 227.5643266524159856, -9.188101187500093303 ) ) ;
#79126=CARTESIAN_POINT ( 'NONE',  ( 184.1487307564388516, 288.9301599317471982, -13.09092302844920575 ) ) ;
#79127=ORIENTED_EDGE ( 'NONE', *, *, #62646, .F. ) ;
#79129=CARTESIAN_POINT ( 'NONE',  ( 161.8762453271136224, 267.0714273172965818, 16.50803258978729460 ) ) ;
#79132=DIRECTION ( 'NONE',  ( 0.4999999999999998890, -0.8660254037844385966, 0.000000000000000000 ) ) ;
#79134=CARTESIAN_POINT ( 'NONE',  ( 58.06412948370898164, 195.1423013555410080, -4.594050593750043987 ) ) ;
#79137=CARTESIAN_POINT ( 'NONE',  ( 191.4044787581200069, 299.1247133251352466, 7.435199718141230818 ) ) ;
#79138=CARTESIAN_POINT ( 'NONE',  ( 197.9812996484125449, 287.7333253908681741, 17.50297787674340455 ) ) ;
#79139=CARTESIAN_POINT ( 'NONE',  ( 172.9576090935003094, 271.2785582124699886, 16.43141609699088335 ) ) ;
#79140=ORIENTED_EDGE ( 'NONE', *, *, #13796, .T. ) ;
#79143=CARTESIAN_POINT ( 'NONE',  ( 177.7824965871422762, 288.9732240448931293, 11.16390339965338541 ) ) ;
#79145=VERTEX_POINT ( 'NONE', #19326 ) ;
#79148=CARTESIAN_POINT ( 'NONE',  ( 207.2707369601997982, 271.6435479931266173, -5.381413637561199614 ) ) ;
#79149=CARTESIAN_POINT ( 'NONE',  ( 147.2089949622447875, 275.6735367246781720, -3.633014386235353221 ) ) ;
#79151=CARTESIAN_POINT ( 'NONE',  ( 149.7128599965862463, 271.3367152699035501, 12.33532264622322394 ) ) ;
#79152=CARTESIAN_POINT ( 'NONE',  ( 180.8104799410488681, 271.3708678522607443, 16.68610488619162524 ) ) ;
#79154=CARTESIAN_POINT ( 'NONE',  ( 205.8918578537579833, 274.0318366629789466, 11.52627491423194250 ) ) ;
#79158=CARTESIAN_POINT ( 'NONE',  ( 108.5637151982415389, 242.6744531367911293, 4.594050593750047540 ) ) ;
#79160=CARTESIAN_POINT ( 'NONE',  ( 148.9665168016069288, 272.6294196034908737, -12.32906446557564806 ) ) ;
#79164=CARTESIAN_POINT ( 'NONE',  ( 183.2770270516915900, 284.7653891124718939, -14.95557695974454937 ) ) ;
#79165=EDGE_CURVE ( 'NONE', #99984, #49104, #20628, .T. ) ;
#79170=CARTESIAN_POINT ( 'NONE',  ( 158.3104460577808368, 274.8641074767056693, -12.54398958924856267 ) ) ;
#79173=CARTESIAN_POINT ( 'NONE',  ( 131.9738982639959488, 240.8768266524159856, -9.188101187500093303 ) ) ;
#79174=CARTESIAN_POINT ( 'NONE',  ( 191.1041001801271761, 295.0267033716904734, -12.18635420512492473 ) ) ;
#79175=CARTESIAN_POINT ( 'NONE',  ( 185.9833676731276171, 296.7909978881492066, 4.657551602822923797 ) ) ;
#79177=CARTESIAN_POINT ( 'NONE',  ( 45.37135788555205096, 190.8768266524159856, 9.188101187500098632 ) ) ;
#79179=CARTESIAN_POINT ( 'NONE',  ( 205.3704330671644414, 274.9349708856848338, -13.01557521325596944 ) ) ;
#79182=CARTESIAN_POINT ( 'NONE',  ( 174.3107956278732900, 262.1115639708946219, 14.35749921995197909 ) ) ;
#79185=CARTESIAN_POINT ( 'NONE',  ( 178.9474598655808109, 291.8225860576774267, -6.155819841034777973 ) ) ;
#79186=CARTESIAN_POINT ( 'NONE',  ( 203.4682009197399566, 278.2297336128146412, -15.36039508894693206 ) ) ;
#79187=CARTESIAN_POINT ( 'NONE',  ( 157.0611216476779077, 270.7214317481134458, -14.74200130514388007 ) ) ;
#79188=ADVANCED_FACE ( 'NONE', ( #57778 ), #47468, .F. ) ;
#79189=CARTESIAN_POINT ( 'NONE',  ( 123.7735466722555771, 232.2677522451417929, -5.000000000000041744 ) ) ;
#79192=VERTEX_POINT ( 'NONE', #6591 ) ;
#79195=CARTESIAN_POINT ( 'NONE',  ( 163.2919429874875448, 247.8170536094679903, 9.876785378511263147 ) ) ;
#79197=CARTESIAN_POINT ( 'NONE',  ( 26.96797095936772237, 192.5024278399160949, 9.188101187500095079 ) ) ;
#79198=AXIS2_PLACEMENT_3D ( 'NONE', #12837, #87015, #2367 ) ;
#79201=CARTESIAN_POINT ( 'NONE',  ( 190.2510882691990730, 301.1224442529128851, -5.480893437181090455 ) ) ;
#79204=CARTESIAN_POINT ( 'NONE',  ( 56.22356517706928969, 213.2677522451419350, -5.000000000000047962 ) ) ;
#79205=CARTESIAN_POINT ( 'NONE',  ( 174.5414916011210664, 289.0348056237772312, 7.720355924734928266 ) ) ;
#79206=CARTESIAN_POINT ( 'NONE',  ( 184.5160214038196500, 257.1200641698031859, 1.403992015128312287 ) ) ;
#79207=CARTESIAN_POINT ( 'NONE',  ( 6.292850856353352285, 162.8932355074535678, -2.679491924311248496 ) ) ;
#79210=( BOUNDED_CURVE ( )  B_SPLINE_CURVE ( 2, ( #17589, #76881, #86058, #7477, #8492, #47969, #23175, #93115, #31766 ),
 .UNSPECIFIED., .F., .T. ) 
 B_SPLINE_CURVE_WITH_KNOTS ( ( 3, 2, 2, 2, 3 ),
 ( 0.2782258064516128782, 0.2795698924731182533, 0.2822580645161290591, 0.2849462365591398094, 0.2862903225806451846 ),
 .UNSPECIFIED. ) 
 CURVE ( )  GEOMETRIC_REPRESENTATION_ITEM ( )  RATIONAL_B_SPLINE_CURVE ( ( 0.9330127018922194093, 0.9330127018922194093, 1.000000000000000000, 0.8660254037844387076, 1.000000000000000000, 0.8660254037844387076, 1.000000000000000000, 0.9330127018922194093, 0.9330127018922194093 ) ) 
 REPRESENTATION_ITEM ( '' )  );
#79211=CARTESIAN_POINT ( 'NONE',  ( 161.8434637317903935, 267.2159794866400944, 16.48508094337421070 ) ) ;
#79212=CARTESIAN_POINT ( 'NONE',  ( 31.70422093597037616, 179.1115022471902023, -5.000000000000041744 ) ) ;
#79214=CARTESIAN_POINT ( 'NONE',  ( 208.3135187673106543, 269.8373969220020285, 2.829653198597726682 ) ) ;
#79215=CARTESIAN_POINT ( 'NONE',  ( -3.992090130160959482, 162.3768266524160140, 9.188101187500098632 ) ) ;
#79219=CARTESIAN_POINT ( 'NONE',  ( 192.8325075361489382, 296.6512949269187516, 11.74553025762331515 ) ) ;
#79221=CARTESIAN_POINT ( 'NONE',  ( 205.7576124508049418, 274.2643565215761328, 10.88614016733041545 ) ) ;
#79222=B_SPLINE_CURVE_WITH_KNOTS ( 'NONE', 3,
 ( #69389, #6, #9092, #30890 ),
 .UNSPECIFIED., .F., .F.,
 ( 4, 4 ),
 ( 0.01340827837672923378, 0.01979442427779384839 ),
 .UNSPECIFIED. ) ;
#79223=CARTESIAN_POINT ( 'NONE',  ( 183.1953467321624203, 257.8017632849582697, -2.260499853111983537 ) ) ;
#79225=VERTEX_POINT ( 'NONE', #71896 ) ;
#79226=CARTESIAN_POINT ( 'NONE',  ( 196.4501996009505831, 290.3852684645433442, -17.82325615854289680 ) ) ;
#79228=ADVANCED_FACE ( 'NONE', ( #55648 ), #24770, .T. ) ;
#79230=CARTESIAN_POINT ( 'NONE',  ( 168.5795673232786669, 288.2161938891477462, 0.5292475961296263520 ) ) ;
#79233=CARTESIAN_POINT ( 'NONE',  ( 160.6659065328018130, 252.3654821715117862, 15.57355298855281411 ) ) ;
#79235=CARTESIAN_POINT ( 'NONE',  ( 206.8317058779879574, 272.4039721336197317, -10.41591514895975834 ) ) ;
#79237=( BOUNDED_CURVE ( )  B_SPLINE_CURVE ( 2, ( #32712, #49415, #24611, #9420, #94552, #25107, #17515, #95066, #71741 ),
 .UNSPECIFIED., .F., .T. ) 
 B_SPLINE_CURVE_WITH_KNOTS ( ( 3, 2, 2, 2, 3 ),
 ( 0.1814516129032258118, 0.1827956989247311870, 0.1854838709677419373, 0.1881720430107526876, 0.1895161290322580627 ),
 .UNSPECIFIED. ) 
 CURVE ( )  GEOMETRIC_REPRESENTATION_ITEM ( )  RATIONAL_B_SPLINE_CURVE ( ( 0.9330127018922194093, 0.9330127018922194093, 1.000000000000000000, 0.8660254037844387076, 1.000000000000000000, 0.8660254037844387076, 1.000000000000000000, 0.9330127018922194093, 0.9330127018922194093 ) ) 
 REPRESENTATION_ITEM ( '' )  );
#79239=CARTESIAN_POINT ( 'NONE',  ( 164.9404048476745004, 244.9618339132846074, -2.801285734921658666 ) ) ;
#79240=CARTESIAN_POINT ( 'NONE',  ( 148.2404373810095706, 275.8870260502966403, -5.709515531134017330 ) ) ;
#79241=CARTESIAN_POINT ( 'NONE',  ( 207.5959034698703078, 271.0803430774575418, -1.830000129038042544 ) ) ;
#79242=CARTESIAN_POINT ( 'NONE',  ( 193.7901930790854976, 294.9925349088783264, 14.24765323155741115 ) ) ;
#79243=ORIENTED_EDGE ( 'NONE', *, *, #12347, .T. ) ;
#79244=ORIENTED_EDGE ( 'NONE', *, *, #74099, .F. ) ;
#79245=CARTESIAN_POINT ( 'NONE',  ( 155.8886909462579524, 276.9667409604651880, -10.24749302008156171 ) ) ;
#79247=ORIENTED_EDGE ( 'NONE', *, *, #63629, .F. ) ;
#79249=CARTESIAN_POINT ( 'NONE',  ( 188.6351333907390710, 297.8094963952060539, 7.741002703549384023 ) ) ;
#79250=ORIENTED_EDGE ( 'NONE', *, *, #43789, .T. ) ;
#79255=CARTESIAN_POINT ( 'NONE',  ( 173.7393789614961861, 267.2768702419098759, 16.72977566464747312 ) ) ;
#79257=CARTESIAN_POINT ( 'NONE',  ( 128.2660534579352145, 254.8615022471902876, 5.000000000000046185 ) ) ;
#79258=CARTESIAN_POINT ( 'NONE',  ( 191.3375250863502970, 299.2406804863936145, 8.828791580707859410 ) ) ;
#79259=CARTESIAN_POINT ( 'NONE',  ( 151.4285566098263018, 275.0047588379541708, -8.595722058304710700 ) ) ;
#79261=CARTESIAN_POINT ( 'NONE',  ( 173.6868681682090312, 257.1546749658006661, -11.76848105503814601 ) ) ;
#79265=B_SPLINE_CURVE_WITH_KNOTS ( 'NONE', 3,
 ( #38587, #7695, #85764, #62889, #61386, #71018, #22888, #106, #23884, #94335, #77617, #30991, #16791, #78109, #39566, #47679 ),
 .UNSPECIFIED., .F., .F.,
 ( 4, 2, 2, 2, 2, 2, 2, 4 ),
 ( 2.809234570782672869E-17, 0.0003787177898467172050, 0.0007574355796934063292, 0.001136153369540095562, 0.001514871159386784686, 0.001893588949233473593, 0.002272306739080162934, 0.003029742318773669552 ),
 .UNSPECIFIED. ) ;
#79266=ORIENTED_EDGE ( 'NONE', *, *, #31776, .T. ) ;
#79267=DIRECTION ( 'NONE',  ( 0.4999999999999992784, -0.8660254037844390407, 0.000000000000000000 ) ) ;
#79270=CARTESIAN_POINT ( 'NONE',  ( 168.4007742750857517, 272.6532539270589268, 15.98367080703011567 ) ) ;
#79273=CARTESIAN_POINT ( 'NONE',  ( 152.7618747630824885, 266.0556667813044101, 16.41480086888796919 ) ) ;
#79276=DIRECTION ( 'NONE',  ( 0.5000000000000048850, -0.8660254037844358210, 0.000000000000000000 ) ) ;
#79277=VERTEX_POINT ( 'NONE', #1492 ) ;
#79282=CARTESIAN_POINT ( 'NONE',  ( 159.2111180226792726, 254.8852497853115722, 16.01057445397460910 ) ) ;
#79285=CARTESIAN_POINT ( 'NONE',  ( 191.1214701901826345, 299.6148985437802708, 6.122719862588978046 ) ) ;
#79286=CARTESIAN_POINT ( 'NONE',  ( 168.2186807742798464, 257.0030785273878564, -14.53950667589619350 ) ) ;
#79287=CARTESIAN_POINT ( 'NONE',  ( 206.3423291502491566, 273.2515974901050413, -10.76717883871977577 ) ) ;
#79290=CARTESIAN_POINT ( 'NONE',  ( 200.6097954076514895, 283.1806371883870383, 16.82611162221071766 ) ) ;
#79291=EDGE_CURVE ( 'NONE', #56261, #75967, #22951, .T. ) ;
#79294=VERTEX_POINT ( 'NONE', #58651 ) ;
#79295=DIRECTION ( 'NONE',  ( -0.8660254037844387076, -0.4999999999999998890, -0.000000000000000000 ) ) ;
#79297=CARTESIAN_POINT ( 'NONE',  ( 137.1012689553694486, 238.4155109091895781, 2.679491924311254714 ) ) ;
#79299=CARTESIAN_POINT ( 'NONE',  ( 207.2383675728608239, 271.6996134166075763, 7.873592648726489784 ) ) ;
#79301=CARTESIAN_POINT ( 'NONE',  ( 15.88121511744419756, 186.6427522451419350, -10.00000000000009415 ) ) ;
#79302=CARTESIAN_POINT ( 'NONE',  ( 93.67942421434402434, 215.7048013555409796, 4.594050593750051981 ) ) ;
#79303=CARTESIAN_POINT ( 'NONE',  ( 188.8544700204132880, 297.4231428397746413, 9.261439979758030461 ) ) ;
#79305=CARTESIAN_POINT ( 'NONE',  ( 162.9968728533147271, 248.3281300736514652, 11.73082768548638910 ) ) ;
#79306=CARTESIAN_POINT ( 'NONE',  ( 4.668163907683432257, 167.3768266524159856, -9.188101187500091527 ) ) ;
#79309=CARTESIAN_POINT ( 'NONE',  ( 161.5875797534026219, 250.7690973254556468, 12.95526170413129030 ) ) ;
#79310=ORIENTED_EDGE ( 'NONE', *, *, #64163, .F. ) ;
#79312=CARTESIAN_POINT ( 'NONE',  ( 200.9036115388549320, 267.7944843482957822, -2.996125407750229730 ) ) ;
#79316=CARTESIAN_POINT ( 'NONE',  ( 207.8575108622103755, 270.6272257822888037, -6.381720258959569847 ) ) ;
#79319=CARTESIAN_POINT ( 'NONE',  ( 33.73396797431614402, 190.2833772461660544, -9.188101187500095079 ) ) ;
#79320=CARTESIAN_POINT ( 'NONE',  ( 82.20432729060250665, 218.2677522451418497, 10.00000000000009592 ) ) ;
#79323=CARTESIAN_POINT ( 'NONE',  ( 175.1863726193077184, 281.4530106220159951, -14.19852717654378260 ) ) ;
#79326=CARTESIAN_POINT ( 'NONE',  ( 161.1232569692349443, 251.5733279787459367, -14.02750397520710557 ) ) ;
#79327=CARTESIAN_POINT ( 'NONE',  ( 186.1036463308693953, 283.4423093435331111, 16.91945572683130905 ) ) ;
#79328=CARTESIAN_POINT ( 'NONE',  ( 194.9220242159064185, 293.0321458743159724, -14.92681063007793263 ) ) ;
#79330=CARTESIAN_POINT ( 'NONE',  ( 204.2799274532736433, 276.8237820148827950, 13.55359442435934803 ) ) ;
#79331=CARTESIAN_POINT ( 'NONE',  ( 191.6723191112861855, 298.6608002251342100, -9.737039817265848995 ) ) ;
#79332=CARTESIAN_POINT ( 'NONE',  ( 190.3049670482083684, 301.0291234702190764, 0.2225066852051815758 ) ) ;
#79333=CARTESIAN_POINT ( 'NONE',  ( 135.6272693901029243, 259.1115022471903444, -5.000000000000047962 ) ) ;
#79334=CARTESIAN_POINT ( 'NONE',  ( 114.7887934315897382, 227.8923013555410080, 4.594050593750050204 ) ) ;
#79339=B_SPLINE_CURVE_WITH_KNOTS ( 'NONE', 3,
 ( #27954, #29947, #58835, #89801 ),
 .UNSPECIFIED., .F., .F.,
 ( 4, 4 ),
 ( 0.004601785012094098890, 0.01014120948868826866 ),
 .UNSPECIFIED. ) ;
#79341=CARTESIAN_POINT ( 'NONE',  ( 192.6361035247282985, 294.0892689374524593, 14.43747539422717630 ) ) ;
#79343=CARTESIAN_POINT ( 'NONE',  ( 150.7303054078841456, 269.5744481236075671, -15.29931087522330735 ) ) ;
#79344=DIRECTION ( 'NONE',  ( -0.8660254037844387076, -0.4999999999999998890, -0.000000000000000000 ) ) ;
#79345=CARTESIAN_POINT ( 'NONE',  ( 149.0203866098534888, 272.5361143586139860, -12.73049804737905255 ) ) ;
#79346=EDGE_CURVE ( 'NONE', #94303, #66081, #49492, .T. ) ;
#79348=CARTESIAN_POINT ( 'NONE',  ( 173.1762443375220926, 289.7177692896065651, -1.166275841582373296 ) ) ;
#79352=CARTESIAN_POINT ( 'NONE',  ( 176.8552821818880147, 279.2679361169009553, 15.50986861091530145 ) ) ;
#79354=B_SPLINE_CURVE_WITH_KNOTS ( 'NONE', 3,
 ( #87300, #71538, #1641, #63419, #1125, #17313, #54809, #70006, #621, #78637 ),
 .UNSPECIFIED., .F., .F.,
 ( 4, 2, 2, 2, 4 ),
 ( 0.000000000000000000, 0.0003983244503580934048, 0.0007966489007161868096, 0.001194973351074280106, 0.001593297801432373619 ),
 .UNSPECIFIED. ) ;
#79355=ORIENTED_EDGE ( 'NONE', *, *, #46022, .T. ) ;
#79358=CARTESIAN_POINT ( 'NONE',  ( 170.5993847053230468, 287.8722104901659691, 7.679145147933459370 ) ) ;
#79360=CARTESIAN_POINT ( 'NONE',  ( 182.1439385020048860, 290.0253507885926183, 13.01467259685074573 ) ) ;
#79362=CARTESIAN_POINT ( 'NONE',  ( 200.3804403721752578, 281.5778917628034606, 17.30444700233937994 ) ) ;
#79363=B_SPLINE_SURFACE_WITH_KNOTS ( 'NONE', 3, 1, ( 
 ( #26499, #60845 ),
 ( #90830, #29968 ),
 ( #6676, #99388 ),
 ( #20398, #21381 ),
 ( #45649, #89822 ),
 ( #76103, #97896 ),
 ( #53265, #36068 ),
 ( #91308, #6172 ),
 ( #84220, #37553 ),
 ( #98398, #27974 ),
 ( #90328, #12808 ),
 ( #68462, #36564 ),
 ( #83208, #4692 ),
 ( #60348, #82730 ),
 ( #59864, #75096 ),
 ( #59352, #21869 ),
 ( #37069, #13302 ),
 ( #5675, #28471 ),
 ( #67471, #28989 ),
 ( #44161, #43670 ),
 ( #91807, #22368 ),
 ( #52269, #14768 ),
 ( #58852, #52754 ),
 ( #20903, #51792 ),
 ( #35584, #66479 ),
 ( #67973, #83715 ),
 ( #66967, #14273 ),
 ( #13773, #97405 ),
 ( #44652, #75586 ),
 ( #51268, #98894 ),
 ( #5187, #82233 ),
 ( #74613, #29476 ),
 ( #45164, #47155 ),
 ( #92314, #70461 ) ),
 .UNSPECIFIED., .T., .F., .F.,
 ( 4, 2, 2, 2, 2, 2, 2, 2, 2, 2, 2, 2, 2, 2, 2, 2, 4 ),
 ( 2, 2 ),
 ( 0.000000000000000000, 0.06250000000000000000, 0.1250000000000000000, 0.1875000000000000000, 0.2500000000000000000, 0.3125000000000000000, 0.3750000000000000000, 0.4375000000000000000, 0.5000000000000000000, 0.5625000000000000000, 0.6250000000000000000, 0.6875000000000000000, 0.7500000000000000000, 0.8125000000000000000, 0.8750000000000000000, 0.9375000000000000000, 1.000000000000000000 ),
 ( 0.000000000000000000, 1.000000000000000000 ),
 .UNSPECIFIED. ) ;
#79365=CARTESIAN_POINT ( 'NONE',  ( 174.0778791619732715, 272.0937389636918056, -17.24785809618570909 ) ) ;
#79366=ORIENTED_EDGE ( 'NONE', *, *, #54268, .T. ) ;
#79368=ADVANCED_FACE ( 'NONE', ( #66764 ), #537, .F. ) ;
#79370=CARTESIAN_POINT ( 'NONE',  ( 164.5515570353740031, 246.1500442291780644, -1.332946268338321083 ) ) ;
#79373=CARTESIAN_POINT ( 'NONE',  ( 188.4650206215856088, 293.1607027833161396, 12.53756631082011630 ) ) ;
#79377=CARTESIAN_POINT ( 'NONE',  ( 154.9528145190857344, 262.2608478075840708, -17.26679351315302213 ) ) ;
#79378=ORIENTED_EDGE ( 'NONE', *, *, #39754, .T. ) ;
#79379=EDGE_LOOP ( 'NONE', ( #80797, #12966, #1449, #92328 ) ) ;
#79380=CARTESIAN_POINT ( 'NONE',  ( 176.1816596051692727, 259.6738327371759283, 12.35962930718384989 ) ) ;
#79381=VERTEX_POINT ( 'NONE', #91591 ) ;
#79386=ORIENTED_EDGE ( 'NONE', *, *, #61515, .T. ) ;
#79387=CARTESIAN_POINT ( 'NONE',  ( 164.3284847670581144, 246.0217105830841433, -2.055838629128057704 ) ) ;
#79388=CARTESIAN_POINT ( 'NONE',  ( 189.9967389050536610, 301.5629902744856281, 3.223574158822913205 ) ) ;
#79390=CARTESIAN_POINT ( 'NONE',  ( 146.7943851877206214, 276.3916619194686746, -4.608908220452185844 ) ) ;
#79391=CARTESIAN_POINT ( 'NONE',  ( 153.2513309553138470, 265.2079037882803618, -16.24091495603130397 ) ) ;
#79393=CARTESIAN_POINT ( 'NONE',  ( 203.3946109532447224, 276.3571951737117729, -14.55139583984842133 ) ) ;
#79394=CARTESIAN_POINT ( 'NONE',  ( 126.7777458412893026, 237.8768266524160140, -9.188101187500091527 ) ) ;
#79399=VERTEX_POINT ( 'NONE', #99674 ) ;
#79400=CARTESIAN_POINT ( 'NONE',  ( 203.5684408170273514, 276.3809927624695320, 13.51646973350518444 ) ) ;
#79401=CARTESIAN_POINT ( 'NONE',  ( 180.7033225138871444, 256.2122485056048617, 1.289357501824909935 ) ) ;
#79402=CARTESIAN_POINT ( 'NONE',  ( 171.2412005135090851, 287.8500574525499474, -4.635942788142338067 ) ) ;
#79403=CARTESIAN_POINT ( 'NONE',  ( 147.4632325565963527, 275.2331842940668594, 3.329760414512866085 ) ) ;
#79406=CARTESIAN_POINT ( 'NONE',  ( 176.8458400405337443, 288.5831395991251611, -9.313839573048495524 ) ) ;
#79407=CARTESIAN_POINT ( 'NONE',  ( 192.6700440564185044, 292.3860465289164381, -14.35732980996189845 ) ) ;
#79410=CARTESIAN_POINT ( 'NONE',  ( 147.8308140999695866, 274.5965143850199865, -7.866624397492971710 ) ) ;
#79412=VERTEX_POINT ( 'NONE', #59136 ) ;
#79413=EDGE_CURVE ( 'NONE', #83448, #29993, #37465, .T. ) ;
#79414=CARTESIAN_POINT ( 'NONE',  ( 163.4882229232755151, 278.1335026457492745, 13.64712021366251804 ) ) ;
#79416=CARTESIAN_POINT ( 'NONE',  ( 159.4766020264466420, 278.1878426662964330, 10.34255018954605276 ) ) ;
#79417=CARTESIAN_POINT ( 'NONE',  ( 191.4370491047775715, 299.0682998299044471, -9.862002456538565554 ) ) ;
#79418=CARTESIAN_POINT ( 'NONE',  ( 148.9228818358559749, 272.7049975811580680, 12.13823097167056275 ) ) ;
#79419=CARTESIAN_POINT ( 'NONE',  ( 162.6774150396764469, 248.8814472377480911, 10.88033986792731689 ) ) ;
#79420=CARTESIAN_POINT ( 'NONE',  ( 153.4150141106643161, 270.1174769024833040, 14.14566187613772641 ) ) ;
#79421=CARTESIAN_POINT ( 'NONE',  ( 160.8923266782674659, 281.5875368026315755, 5.746848696840308968 ) ) ;
#79422=CARTESIAN_POINT ( 'NONE',  ( 199.9222995550700261, 267.4785754008608478, 6.216224682353979070 ) ) ;
#79424=CARTESIAN_POINT ( 'NONE',  ( 164.0796711861443669, 280.3631140631478047, -11.42675980477452136 ) ) ;
#79425=CARTESIAN_POINT ( 'NONE',  ( 192.1412027652805534, 261.7830949532877298, 4.365074532660510265 ) ) ;
#79427=CYLINDRICAL_SURFACE ( 'NONE', #28693, 10.00000000000010658 ) ;
#79429=CARTESIAN_POINT ( 'NONE',  ( 152.6945189806187955, 266.1723304187151484, 16.62409282110771613 ) ) ;
#79434=CARTESIAN_POINT ( 'NONE',  ( -8.863483026448420787, 159.5643266524160140, 9.188101187500095079 ) ) ;
#79435=CARTESIAN_POINT ( 'NONE',  ( 81.82518085639701155, 227.2369531367911293, -4.594050593750048428 ) ) ;
#79436=CARTESIAN_POINT ( 'NONE',  ( 202.9490938173916561, 279.1288534886517709, -16.56031645010252973 ) ) ;
#79439=DIRECTION ( 'NONE',  ( -0.8660254037844387076, -0.4999999999999998890, -0.000000000000000000 ) ) ;
#79443=CARTESIAN_POINT ( 'NONE',  ( 163.2256942281324541, 247.9317998266098471, -9.780520296312531059 ) ) ;
#79444=CARTESIAN_POINT ( 'NONE',  ( 207.7267680070821427, 270.8536790500975826, 4.918728265708383063 ) ) ;
#79445=CARTESIAN_POINT ( 'NONE',  ( 169.2519802811189891, 252.1610067817271954, -8.894316421355656033 ) ) ;
#79446=CARTESIAN_POINT ( 'NONE',  ( 170.6278779686246878, 289.8994199495515431, -0.2720655136580445999 ) ) ;
#79447=CARTESIAN_POINT ( 'NONE',  ( 181.8509774751104544, 266.9677320091309412, 16.09658033613713712 ) ) ;
#79448=CARTESIAN_POINT ( 'NONE',  ( 165.9983592287585168, 253.7040021870680562, -13.23752916164668569 ) ) ;
#79451=CARTESIAN_POINT ( 'NONE',  ( 35.03300607999280913, 191.0333772461660544, 9.188101187500095079 ) ) ;
#79453=CARTESIAN_POINT ( 'NONE',  ( 66.96803994030899787, 197.2202760586659736, -5.415160957724236172E-17 ) ) ;
#79454=CARTESIAN_POINT ( 'NONE',  ( 207.5462191418491500, 271.1663988579299485, -5.239401497773396699 ) ) ;
#79458=CARTESIAN_POINT ( 'NONE',  ( 199.6718038460705031, 284.8052862301161667, 17.94500466126824989 ) ) ;
#79459=CARTESIAN_POINT ( 'NONE',  ( 176.7734426553208777, 270.1971082629633543, -16.99733951863274939 ) ) ;
#79463=CARTESIAN_POINT ( 'NONE',  ( 149.3141802193904368, 272.0272488999566463, -11.40332369054239336 ) ) ;
#79464=ORIENTED_EDGE ( 'NONE', *, *, #86538, .F. ) ;
#79466=CARTESIAN_POINT ( 'NONE',  ( 68.83479979963041728, 219.7369531367911293, -4.594050593750048428 ) ) ;
#79468=CARTESIAN_POINT ( 'NONE',  ( 172.4195363219592707, 289.2899927951424388, -1.060142233323475791 ) ) ;
#79474=CARTESIAN_POINT ( 'NONE',  ( 122.6368883333364010, 241.6115022471902591, 10.00000000000009592 ) ) ;
#79475=CARTESIAN_POINT ( 'NONE',  ( 20.41989025203908881, 171.0494855054051584, -2.679491924311248496 ) ) ;
#79479=ORIENTED_EDGE ( 'NONE', *, *, #13111, .T. ) ;
#79480=CARTESIAN_POINT ( 'NONE',  ( 202.9689790241539242, 279.0944113002206564, 15.85114608332523289 ) ) ;
#79485=CARTESIAN_POINT ( 'NONE',  ( 173.3282377161554848, 251.6955198918108749, -0.2234702318904273066 ) ) ;
#79488=CARTESIAN_POINT ( 'NONE',  ( 170.1765561332687184, 250.1434207139878652, 3.414147863577436048 ) ) ;
#79489=CARTESIAN_POINT ( 'NONE',  ( 206.9676577495037577, 271.5526395553730481, -5.460015649064563270 ) ) ;
#79490=ORIENTED_EDGE ( 'NONE', *, *, #15697, .F. ) ;
#79496=ADVANCED_FACE ( 'NONE', ( #31245 ), #40336, .T. ) ;
#79497=CYLINDRICAL_SURFACE ( 'NONE', #33538, 10.00000000000010658 ) ;
#79501=CARTESIAN_POINT ( 'NONE',  ( 183.1229191643124921, 295.7565714162242330, 0.9213203475738164228 ) ) ;
#79502=CARTESIAN_POINT ( 'NONE',  ( 162.6948115306194893, 284.8132865779174949, -2.619575048482838397 ) ) ;
#79503=CARTESIAN_POINT ( 'NONE',  ( 194.6782745185928434, 293.4543327343926080, -14.56555309295305634 ) ) ;
#79505=CARTESIAN_POINT ( 'NONE',  ( 155.2695601165254402, 261.7122283397445131, 16.98599069618989077 ) ) ;
#79507=CARTESIAN_POINT ( 'NONE',  ( 205.0520875136525376, 275.4863615587311756, -14.16385635411862509 ) ) ;
#79508=CARTESIAN_POINT ( 'NONE',  ( 164.7499588712500724, 245.2916960205490398, 5.222210624224128850 ) ) ;
#79511=CARTESIAN_POINT ( 'NONE',  ( 88.91628449352961638, 212.9548013555409796, -4.594050593750042211 ) ) ;
#79513=CARTESIAN_POINT ( 'NONE',  ( 190.8264243556038195, 300.1259329198319961, 8.466983560044813117 ) ) ;
#79514=CARTESIAN_POINT ( 'NONE',  ( 197.4151212697929907, 279.2547988841874371, -17.17267392321700470 ) ) ;
#79517=CARTESIAN_POINT ( 'NONE',  ( 164.9124716213052864, 264.7286630427709042, -16.72847895078608360 ) ) ;
#79518=VERTEX_POINT ( 'NONE', #1865 ) ;
#79520=CARTESIAN_POINT ( 'NONE',  ( 185.1252552835508425, 268.3045509528566299, -15.86481251201890608 ) ) ;
#79522=B_SPLINE_CURVE_WITH_KNOTS ( 'NONE', 3,
 ( #8424, #323, #24616, #46405 ),
 .UNSPECIFIED., .F., .F.,
 ( 4, 4 ),
 ( 0.000000000000000000, 0.007199726097782813139 ),
 .UNSPECIFIED. ) ;
#79523=CARTESIAN_POINT ( 'NONE',  ( 147.1447476476323004, 275.7848163378367872, 0.6373001129109078233 ) ) ;
#79524=DIRECTION ( 'NONE',  ( -0.4999999999999987232, 0.8660254037844394848, 0.000000000000000000 ) ) ;
#79526=CARTESIAN_POINT ( 'NONE',  ( 163.1177074157340030, 248.1188384722309195, 11.53923137679231026 ) ) ;
#79529=( BOUNDED_CURVE ( )  B_SPLINE_CURVE ( 2, ( #31934, #85713, #86706, #85189, #39521, #40535, #46641, #16747, #77566 ),
 .UNSPECIFIED., .F., .T. ) 
 B_SPLINE_CURVE_WITH_KNOTS ( ( 3, 2, 2, 2, 3 ),
 ( 0.08467741935483871774, 0.08602150537634409289, 0.08870967741935484319, 0.09139784946236559349, 0.09274193548387096864 ),
 .UNSPECIFIED. ) 
 CURVE ( )  GEOMETRIC_REPRESENTATION_ITEM ( )  RATIONAL_B_SPLINE_CURVE ( ( 0.9330127018922192983, 0.9330127018922196314, 1.000000000000000000, 0.8660254037844387076, 1.000000000000000000, 0.8660254037844387076, 1.000000000000000000, 0.9330127018922194093, 0.9330127018922194093 ) ) 
 REPRESENTATION_ITEM ( '' )  );
#79530=ORIENTED_EDGE ( 'NONE', *, *, #86236, .F. ) ;
#79531=CARTESIAN_POINT ( 'NONE',  ( 161.5872815829137608, 250.7696137718916134, -14.26133658251064951 ) ) ;
#79533=B_SPLINE_CURVE_WITH_KNOTS ( 'NONE', 3,
 ( #13590, #14585, #52563, #37856 ),
 .UNSPECIFIED., .F., .F.,
 ( 4, 4 ),
 ( 0.000000000000000000, 0.006921230768823173965 ),
 .UNSPECIFIED. ) ;
#79534=EDGE_CURVE ( 'NONE', #90906, #95819, #48431, .T. ) ;
#79536=CARTESIAN_POINT ( 'NONE',  ( 149.1653648461108617, 275.5304674000249179, 7.618651205328232479 ) ) ;
#79541=CARTESIAN_POINT ( 'NONE',  ( 205.0993130461165777, 275.4045645370890156, 13.92529057593422337 ) ) ;
#79542=EDGE_CURVE ( 'NONE', #71064, #37080, #67615, .T. ) ;
#79543=CARTESIAN_POINT ( 'NONE',  ( 158.6510112063557756, 274.6825264219753535, 12.95479408922676257 ) ) ;
#79544=CARTESIAN_POINT ( 'NONE',  ( 206.8313602288537538, 272.4045708154811791, -9.607337080360906612 ) ) ;
#79545=EDGE_CURVE ( 'NONE', #28883, #7026, #96738, .T. ) ;
#79548=DIRECTION ( 'NONE',  ( -0.8660254037844387076, -0.4999999999999998890, -0.000000000000000000 ) ) ;
#79549=CARTESIAN_POINT ( 'NONE',  ( 144.5581563630820767, 254.2677522451418781, 10.00000000000009592 ) ) ;
#79550=ORIENTED_EDGE ( 'NONE', *, *, #8433, .T. ) ;
#79552=CARTESIAN_POINT ( 'NONE',  ( 161.7587802986029999, 250.4725692828850754, 14.33336164792646450 ) ) ;
#79554=CARTESIAN_POINT ( 'NONE',  ( 168.7662487658844839, 250.5857779709543820, 6.949784551538230382 ) ) ;
#79556=CARTESIAN_POINT ( 'NONE',  ( 178.1182393013862395, 291.3468047747071523, -6.134831094139173935 ) ) ;
#79557=CARTESIAN_POINT ( 'NONE',  ( 202.6713589670606552, 279.6099043604578469, -16.15432042160254511 ) ) ;
#79558=ORIENTED_EDGE ( 'NONE', *, *, #12926, .T. ) ;
#79560=CARTESIAN_POINT ( 'NONE',  ( 181.9757784701835135, 264.1876005812737844, 13.64994279689907231 ) ) ;
#79563=CARTESIAN_POINT ( 'NONE',  ( 192.3401793061076717, 297.5040324353506094, 12.56432540404525611 ) ) ;
#79564=CARTESIAN_POINT ( 'NONE',  ( 168.6481342183708705, 273.1260240405907211, 15.95224985717143618 ) ) ;
#79566=CARTESIAN_POINT ( 'NONE',  ( 188.4534122740155624, 260.4225287015167396, 3.718312834711502202 ) ) ;
#79568=CARTESIAN_POINT ( 'NONE',  ( 162.6991225460172927, 284.8212170328912975, -3.897741803361528756 ) ) ;
#79569=CARTESIAN_POINT ( 'NONE',  ( 2.719259653403430121, 178.5024278399160949, -9.188101187500093303 ) ) ;
#79571=ORIENTED_EDGE ( 'NONE', *, *, #20648, .F. ) ;
#79572=CARTESIAN_POINT ( 'NONE',  ( 177.8840711869828510, 256.7301028248324997, 8.353015782577163151 ) ) ;
#79574=CARTESIAN_POINT ( 'NONE',  ( 164.4698008747318738, 245.7769439046653019, -6.272955660526681854 ) ) ;
#79576=CARTESIAN_POINT ( 'NONE',  ( 31.83936385565518279, 195.3149278399160664, 9.188101187500093303 ) ) ;
#79577=CARTESIAN_POINT ( 'NONE',  ( 164.3602934812760452, 245.9666162739349318, -7.171958108566009571 ) ) ;
#79578=CARTESIAN_POINT ( 'NONE',  ( 190.1752790837055045, 301.2537496138681945, -5.177773110520776711 ) ) ;
#79580=CARTESIAN_POINT ( 'NONE',  ( 181.1863822141313562, 293.5084475425986739, 6.203074340371671269 ) ) ;
#79581=CARTESIAN_POINT ( 'NONE',  ( 173.3588497307663374, 273.3242272104048993, -16.64521848681001259 ) ) ;
#79582=CARTESIAN_POINT ( 'NONE',  ( 196.9684447319790479, 289.4876415668271648, 17.73978044655682851 ) ) ;
#79585=CARTESIAN_POINT ( 'NONE',  ( 187.0591251360168883, 296.0433128962568503, -7.698390371408583732 ) ) ;
#79587=CARTESIAN_POINT ( 'NONE',  ( 87.49069069641797114, 207.9865022471901455, 1.119607411625061291E-15 ) ) ;
#79589=CARTESIAN_POINT ( 'NONE',  ( 205.9537632452105242, 271.2264420391654198, 6.128872511909795762 ) ) ;
#79590=CARTESIAN_POINT ( 'NONE',  ( 45.45211389745056607, 206.2369531367911293, -4.594050593750048428 ) ) ;
#79591=CARTESIAN_POINT ( 'NONE',  ( 159.4889735931715222, 254.4039898200529706, 16.88104032092801887 ) ) ;
#79594=CARTESIAN_POINT ( 'NONE',  ( 198.7501991201633018, 286.4015524398827779, -18.58948563601804693 ) ) ;
#79597=ORIENTED_EDGE ( 'NONE', *, *, #63333, .T. ) ;
#79599=CARTESIAN_POINT ( 'NONE',  ( -5.792922669062946284, 155.9155109091896065, 2.679491924311252937 ) ) ;
#79600=FACE_OUTER_BOUND ( 'NONE', #42887, .T. ) ;
#79603=CARTESIAN_POINT ( 'NONE',  ( 202.9689790241539242, 279.0944113002206564, 15.85114608332523289 ) ) ;
#79604=CARTESIAN_POINT ( 'NONE',  ( 149.6890529486499872, 271.3779502865075983, -12.51465682618088593 ) ) ;
#79605=CARTESIAN_POINT ( 'NONE',  ( 171.3306725491475504, 255.7550868248229960, 12.09612247527935125 ) ) ;
#79608=CARTESIAN_POINT ( 'NONE',  ( 15.66239703771868719, 191.3967562850346837, -4.648177544792955347E-16 ) ) ;
#79610=EDGE_CURVE ( 'NONE', #25756, #55485, #96925, .T. ) ;
#79613=CARTESIAN_POINT ( 'NONE',  ( 190.8001679306945277, 300.1714103817999444, 7.815449226872675403 ) ) ;
#79616=DIRECTION ( 'NONE',  ( -0.8660254037844387076, -0.4999999999999998890, -0.000000000000000000 ) ) ;
#79617=ORIENTED_EDGE ( 'NONE', *, *, #80161, .F. ) ;
#79618=EDGE_LOOP ( 'NONE', ( #65364, #36102, #33527, #6290 ) ) ;
#79619=CARTESIAN_POINT ( 'NONE',  ( 189.6306422694777893, 274.4800867691382678, -15.80158207961506278 ) ) ;
#79621=B_SPLINE_CURVE_WITH_KNOTS ( 'NONE', 3,
 ( #22481, #5296, #91416, #21979, #68079, #30079, #53373, #37663, #98002, #83322, #51382, #12916, #90443, #82348, #4810, #13884 ),
 .UNSPECIFIED., .F., .F.,
 ( 4, 2, 2, 2, 2, 2, 2, 4 ),
 ( 0.000000000000000000, 0.0005379944778325431451, 0.0008069917167488165066, 0.001075988955665089977, 0.001344986194581363446, 0.001613983433497636916, 0.001882980672413910386, 0.002151977911330183856 ),
 .UNSPECIFIED. ) ;
#79623=CARTESIAN_POINT ( 'NONE',  ( 152.7691010214056462, 266.0431505347400503, -16.40662330462167162 ) ) ;
#79627=CARTESIAN_POINT ( 'NONE',  ( 204.7764732025852084, 275.9637395487929439, -14.02287343454361412 ) ) ;
#79628=CARTESIAN_POINT ( 'NONE',  ( 105.9656389868882513, 241.1744531367911577, 4.594050593750047540 ) ) ;
#79629=CARTESIAN_POINT ( 'NONE',  ( 181.0301937916765667, 287.8052501752913486, -14.12606483171538052 ) ) ;
#79631=CARTESIAN_POINT ( 'NONE',  ( 161.7844122638997533, 267.0814880858553124, 16.49944467494395894 ) ) ;
#79634=CARTESIAN_POINT ( 'NONE',  ( 197.9002057575219453, 287.8737841300738296, 18.01270164875645818 ) ) ;
#79636=CARTESIAN_POINT ( 'NONE',  ( 47.26526781268299260, 210.3464784336661637, 1.353441290958777525E-15 ) ) ;
#79638=CARTESIAN_POINT ( 'NONE',  ( 150.6655900823359389, 269.6865383554857090, 15.31288044136207205 ) ) ;
#79639=CARTESIAN_POINT ( 'NONE',  ( 198.0167861310041530, 287.6718610000373246, 18.15276047493383160 ) ) ;
#79640=CARTESIAN_POINT ( 'NONE',  ( 176.4464654933624104, 273.1633176496665101, 16.93181923922713494 ) ) ;
#79641=ORIENTED_EDGE ( 'NONE', *, *, #16463, .F. ) ;
#79642=EDGE_CURVE ( 'NONE', #88756, #85510, #83449, .T. ) ;
#79644=CARTESIAN_POINT ( 'NONE',  ( 178.0221171495884676, 288.7633432952653152, 10.91361327765725342 ) ) ;
#79646=VERTEX_POINT ( 'NONE', #82222 ) ;
#79647=CARTESIAN_POINT ( 'NONE',  ( 172.2516114191509189, 258.4199449647830420, -14.42867330110744462 ) ) ;
#79649=CARTESIAN_POINT ( 'NONE',  ( 207.1158949475991164, 271.9117422260973740, -5.823035679195911918 ) ) ;
#79650=CARTESIAN_POINT ( 'NONE',  ( 206.7474862253485526, 270.1292977026819813, 1.793960490934114471 ) ) ;
#79653=CARTESIAN_POINT ( 'NONE',  ( 149.5633513747893346, 271.5956717990251832, 12.83777201928511325 ) ) ;
#79654=CARTESIAN_POINT ( 'NONE',  ( 180.6100108800816599, 271.2853514182555728, 16.55563358471784596 ) ) ;
#79655=CARTESIAN_POINT ( 'NONE',  ( 156.6812872898450735, 261.2670451491295012, 0.000000000000000000 ) ) ;
#79657=CARTESIAN_POINT ( 'NONE',  ( 165.3419214322780135, 255.1043459237804996, 13.90808614669940901 ) ) ;
#79659=ADVANCED_FACE ( 'NONE', ( #34098 ), #85530, .F. ) ;
#79660=CARTESIAN_POINT ( 'NONE',  ( 119.9849458542963561, 230.8923013555409796, 4.594050593750050204 ) ) ;
#79661=VERTEX_POINT ( 'NONE', #45154 ) ;
#79662=CARTESIAN_POINT ( 'NONE',  ( 191.3041230083617563, 299.2985345825480863, -9.819045872446528378 ) ) ;
#79664=EDGE_CURVE ( 'NONE', #44895, #27272, #28461, .T. ) ;
#79668=CARTESIAN_POINT ( 'NONE',  ( 177.6813079280251202, 255.2054228243137004, 4.880324467531951704 ) ) ;
#79671=CARTESIAN_POINT ( 'NONE',  ( 154.6163025329676088, 273.5610833407037035, -13.37509610506471702 ) ) ;
#79674=CARTESIAN_POINT ( 'NONE',  ( 164.4118148411678817, 245.8773786609274623, -1.109947685176164045 ) ) ;
#79676=CARTESIAN_POINT ( 'NONE',  ( 198.7829547491859330, 286.3448180261817129, -18.59838968157616179 ) ) ;
#79677=DIRECTION ( 'NONE',  ( 0.4999999999999992784, -0.8660254037844390407, 0.000000000000000000 ) ) ;
#79678=CARTESIAN_POINT ( 'NONE',  ( 190.7685386727469279, 298.2261938635710976, -9.678376712886644029 ) ) ;
#79679=CARTESIAN_POINT ( 'NONE',  ( 64.42391676880970408, 201.8768266524159856, -9.188101187500091527 ) ) ;
#79681=CARTESIAN_POINT ( 'NONE',  ( 164.9586510554008782, 244.9302305544571823, -1.717556444319656039 ) ) ;
#79682=CARTESIAN_POINT ( 'NONE',  ( 193.8354046899084153, 268.4885937380259406, 12.87375928640720524 ) ) ;
#79683=B_SPLINE_SURFACE_WITH_KNOTS ( 'NONE', 3, 1, ( 
 ( #87291, #47690 ),
 ( #17822, #48723 ),
 ( #85776, #23897 ),
 ( #62902, #64411 ),
 ( #10219, #47198 ),
 ( #86768, #41087 ),
 ( #39579, #78625 ),
 ( #93854, #49220 ),
 ( #24409, #33515 ),
 ( #79154, #95374 ),
 ( #56799, #70500 ),
 ( #1631, #87784 ),
 ( #41594, #86265 ),
 ( #610, #8710 ),
 ( #31492, #62384 ),
 ( #55285, #16803 ),
 ( #9211, #93341 ),
 ( #32515, #80655 ),
 ( #35499, #89271 ),
 ( #52557, #44960 ),
 ( #43075, #73517 ),
 ( #11234, #64915 ),
 ( #88770, #65404 ),
 ( #97329, #34028 ),
 ( #65894, #57297 ),
 ( #22171, #42098 ),
 ( #73031, #4100 ),
 ( #83513, #95860 ),
 ( #66401, #68259 ),
 ( #96850, #27417 ),
 ( #19820, #50690 ),
 ( #99184, #34502 ),
 ( #91111, #29283 ),
 ( #96345, #37358 ) ),
 .UNSPECIFIED., .T., .F., .F.,
 ( 4, 2, 2, 2, 2, 2, 2, 2, 2, 2, 2, 2, 2, 2, 2, 2, 4 ),
 ( 2, 2 ),
 ( 0.000000000000000000, 0.06250000000000000000, 0.1250000000000000000, 0.1875000000000000000, 0.2500000000000000000, 0.3125000000000000000, 0.3750000000000000000, 0.4375000000000000000, 0.5000000000000000000, 0.5625000000000000000, 0.6250000000000000000, 0.6875000000000000000, 0.7500000000000000000, 0.8125000000000000000, 0.8750000000000000000, 0.9375000000000000000, 1.000000000000000000 ),
 ( 0.000000000000000000, 1.000000000000000000 ),
 .UNSPECIFIED. ) ;
#79685=CARTESIAN_POINT ( 'NONE',  ( 174.8968804999455244, 261.5766033592863096, 14.34024671999864964 ) ) ;
#79686=CARTESIAN_POINT ( 'NONE',  ( 155.1231266014676180, 279.5326577215706152, -1.580077478444769534 ) ) ;
#79687=FACE_OUTER_BOUND ( 'NONE', #64521, .T. ) ;
#79688=CARTESIAN_POINT ( 'NONE',  ( 155.4661767250933622, 261.3716783840932294, -17.10192542004562810 ) ) ;
#79689=CARTESIAN_POINT ( 'NONE',  ( 193.5197837783914281, 288.6179979435178211, 16.03724552212410970 ) ) ;
#79690=CARTESIAN_POINT ( 'NONE',  ( 129.4748805805031395, 238.8927522451418781, 10.00000000000009592 ) ) ;
#79693=EDGE_CURVE ( 'NONE', #59645, #75836, #10947, .T. ) ;
#79694=CARTESIAN_POINT ( 'NONE',  ( 189.8171280724701546, 301.8740853621098950, -0.4360232994423257624 ) ) ;
#79695=CARTESIAN_POINT ( 'NONE',  ( -16.90171517502901466, 170.2369531367911293, -4.594050593750048428 ) ) ;
#79696=CARTESIAN_POINT ( 'NONE',  ( 46.72434903108273119, 197.7833772461660828, -9.188101187500095079 ) ) ;
#79700=CARTESIAN_POINT ( 'NONE',  ( 190.9335643195044838, 299.9403610588350944, -4.692880224846124548 ) ) ;
#79702=CARTESIAN_POINT ( 'NONE',  ( 195.8285188278500470, 273.2427770020486832, 15.26130794574777383 ) ) ;
#79703=CARTESIAN_POINT ( 'NONE',  ( 56.65657787896151376, 213.5177522451419065, 5.000000000000046185 ) ) ;
#79705=CARTESIAN_POINT ( 'NONE',  ( 180.8537919486467160, 256.3066541963624445, 1.346842808816189452 ) ) ;
#79706=CARTESIAN_POINT ( 'NONE',  ( 205.3704330671644414, 274.9349708856848338, -13.01557521325596944 ) ) ;
#79707=CARTESIAN_POINT ( 'NONE',  ( 162.1316038200447736, 252.0640768520765960, -13.69825752773376770 ) ) ;
#79708=CARTESIAN_POINT ( 'NONE',  ( 179.2389850949382151, 294.6081512498237771, 1.073768896970125786 ) ) ;
#79709=CARTESIAN_POINT ( 'NONE',  ( 49.89075441544358824, 189.6115022471902023, -5.000000000000041744 ) ) ;
#79710=CARTESIAN_POINT ( 'NONE',  ( 150.8371008641169908, 248.7048013555409511, 4.594050593750051981 ) ) ;
#79711=CARTESIAN_POINT ( 'NONE',  ( 202.4943568615953779, 279.9164810001701085, 17.09064351659286984 ) ) ;
#79712=CARTESIAN_POINT ( 'NONE',  ( 2.773212693257451900, 184.6589784336661637, -6.496448406907675876E-16 ) ) ;
#79716=CARTESIAN_POINT ( 'NONE',  ( 152.7618747630824885, 266.0556667813044101, 16.41480086888796919 ) ) ;
#79718=CARTESIAN_POINT ( 'NONE',  ( 156.3551087084618700, 261.3239775484371989, -17.56576820129662053 ) ) ;
#79719=EDGE_CURVE ( 'NONE', #90599, #66772, #84705, .T. ) ;
#79720=CARTESIAN_POINT ( 'NONE',  ( 186.8774594610050599, 259.3182782412434335, -2.380209424388837647 ) ) ;
#79723=CARTESIAN_POINT ( 'NONE',  ( 181.7505021599577333, 256.6548486136064753, -6.673752474138594515 ) ) ;
#79725=CARTESIAN_POINT ( 'NONE',  ( 166.3255300953076414, 285.8001061038755779, 0.4975669204057207584 ) ) ;
#79728=CARTESIAN_POINT ( 'NONE',  ( 153.0911466228407392, 274.9737743950042841, 10.66320493477942044 ) ) ;
#79730=CARTESIAN_POINT ( 'NONE',  ( 54.63354020801843092, 213.8967562850347122, -4.648177544792955347E-16 ) ) ;
#79733=CARTESIAN_POINT ( 'NONE',  ( 152.9920137376499838, 265.6570543845515431, 16.15798175643282164 ) ) ;
#79734=CARTESIAN_POINT ( 'NONE',  ( 165.0156970625405108, 244.8314239717225007, -1.890480716182876719 ) ) ;
#79736=EDGE_CURVE ( 'NONE', #81147, #30467, #14518, .T. ) ;
#79738=CARTESIAN_POINT ( 'NONE',  ( 155.5660013421004919, 261.1987770755905558, 17.28709111629370199 ) ) ;
#79739=ORIENTED_EDGE ( 'NONE', *, *, #43374, .T. ) ;
#79740=ORIENTED_EDGE ( 'NONE', *, *, #78752, .T. ) ;
#79751=ORIENTED_EDGE ( 'NONE', *, *, #30786, .F. ) ;
#79752=CARTESIAN_POINT ( 'NONE',  ( 200.6800100461949228, 283.0590218669948399, 18.32402613046234308 ) ) ;
#79753=CARTESIAN_POINT ( 'NONE',  ( 169.1532419530282141, 276.3814789465369586, -16.13320117031923573 ) ) ;
#79757=DIRECTION ( 'NONE',  ( -0.8660254037844387076, -0.4999999999999998890, -0.000000000000000000 ) ) ;
#79759=AXIS2_PLACEMENT_3D ( 'NONE', #9289, #24482, #39654 ) ;
#79760=ORIENTED_EDGE ( 'NONE', *, *, #91287, .T. ) ;
#79763=VERTEX_POINT ( 'NONE', #17771 ) ;
#79767=CARTESIAN_POINT ( 'NONE',  ( 159.1165150567399280, 259.5332163835566917, 16.70623555518022840 ) ) ;
#79768=CARTESIAN_POINT ( 'NONE',  ( 194.0370204994606524, 294.5650172760874170, 14.49136610471935604 ) ) ;
#79769=CARTESIAN_POINT ( 'NONE',  ( 177.5977857591645090, 289.0201305223690156, -9.328731151047037429 ) ) ;
#79772=CARTESIAN_POINT ( 'NONE',  ( 174.5517021171108638, 290.1645060665484266, 6.371634131280785596 ) ) ;
#79775=CARTESIAN_POINT ( 'NONE',  ( 165.0952264510788154, 281.4963861521250124, -11.84807672454148886 ) ) ;
#79777=CARTESIAN_POINT ( 'NONE',  ( 164.3754245770190039, 245.9404084473339083, 1.667926061651832992 ) ) ;
#79778=CARTESIAN_POINT ( 'NONE',  ( 206.4768661561222984, 273.0185725604343361, 11.39716120335626925 ) ) ;
#79779=CARTESIAN_POINT ( 'NONE',  ( 159.6610344727618269, 254.1059716346071866, 15.33388637456589620 ) ) ;
#79780=ORIENTED_EDGE ( 'NONE', *, *, #41389, .T. ) ;
#79782=CARTESIAN_POINT ( 'NONE',  ( 190.5278607951618710, 300.6430601758063403, 5.309934257482836095 ) ) ;
#79787=CARTESIAN_POINT ( 'NONE',  ( 200.6129772034685175, 283.1751261563724142, 18.36811917402039640 ) ) ;
#79788=CARTESIAN_POINT ( 'NONE',  ( 190.7970923485466699, 261.9842811066119452, -0.6382846533130664968 ) ) ;
#79794=CARTESIAN_POINT ( 'NONE',  ( 11.55108809852201013, 184.1427522451419350, 10.00000000000009237 ) ) ;
#79795=CARTESIAN_POINT ( 'NONE',  ( 100.7969837277561282, 222.8768266524159856, -9.188101187500093303 ) ) ;
#79797=CARTESIAN_POINT ( 'NONE',  ( 197.4842693130445923, 286.5942071846287149, -17.75505217046438489 ) ) ;
#79798=CARTESIAN_POINT ( 'NONE',  ( 167.0636792507274322, 277.9578970009563932, -14.05280382147244644 ) ) ;
#79799=ADVANCED_FACE ( 'NONE', ( #26861 ), #70094, .F. ) ;
#79800=CARTESIAN_POINT ( 'NONE',  ( 18.84898279888859918, 187.8149278399161233, 9.188101187500093303 ) ) ;
#79801=CARTESIAN_POINT ( 'NONE',  ( 174.6617384230121104, 289.1922761299584863, -9.320811169396549190 ) ) ;
#79802=ORIENTED_EDGE ( 'NONE', *, *, #40418, .T. ) ;
#79804=ORIENTED_EDGE ( 'NONE', *, *, #64033, .T. ) ;
#79805=CARTESIAN_POINT ( 'NONE',  ( 200.8942821848932851, 267.7847592425025027, -2.908898627582254370 ) ) ;
#79808=CARTESIAN_POINT ( 'NONE',  ( 205.4334751569798811, 272.0530277678294624, -9.567426915989852176 ) ) ;
#79809=CARTESIAN_POINT ( 'NONE',  ( 207.4218731373931632, 271.3817724553659332, -5.249531240730909154 ) ) ;
#79810=( BOUNDED_CURVE ( )  B_SPLINE_CURVE ( 2, ( #47375, #87954, #2812, #94026, #71204, #777, #2304, #10396, #49385 ),
 .UNSPECIFIED., .F., .T. ) 
 B_SPLINE_CURVE_WITH_KNOTS ( ( 3, 2, 2, 2, 3 ),
 ( 0.1572580645161290314, 0.1586021505376344065, 0.1612903225806451568, 0.1639784946236559071, 0.1653225806451612823 ),
 .UNSPECIFIED. ) 
 CURVE ( )  GEOMETRIC_REPRESENTATION_ITEM ( )  RATIONAL_B_SPLINE_CURVE ( ( 0.9330127018922194093, 0.9330127018922194093, 1.000000000000000000, 0.8660254037844387076, 1.000000000000000000, 0.8660254037844387076, 1.000000000000000000, 0.9330127018922194093, 0.9330127018922194093 ) ) 
 REPRESENTATION_ITEM ( '' )  );
#79811=CARTESIAN_POINT ( 'NONE',  ( 182.7656509685662343, 284.3849974448608577, 14.96600143269570182 ) ) ;
#79813=CARTESIAN_POINT ( 'NONE',  ( 40.98727782677583065, 182.2202760586659451, -5.415160957724236172E-17 ) ) ;
#79816=CARTESIAN_POINT ( 'NONE',  ( 179.4361089452441433, 259.6094657833778001, -10.31148828265781603 ) ) ;
#79817=CARTESIAN_POINT ( 'NONE',  ( -3.938137090306929711, 168.5333772461660828, 9.188101187500095079 ) ) ;
#79819=CARTESIAN_POINT ( 'NONE',  ( 198.9832789858017463, 285.9978462703757600, -18.55676541969546278 ) ) ;
#79820=FACE_OUTER_BOUND ( 'NONE', #92108, .T. ) ;
#79821=AXIS2_PLACEMENT_3D ( 'NONE', #63465, #33063, #78682 ) ;
#79823=CARTESIAN_POINT ( 'NONE',  ( 163.7064929935861244, 247.0990319366274548, 6.401263337036986023 ) ) ;
#79824=CARTESIAN_POINT ( 'NONE',  ( 146.5865263025993954, 276.7516840693029962, 0.4918294119671828835 ) ) ;
#79825=CARTESIAN_POINT ( 'NONE',  ( 164.3524132573224392, 245.9802652221976587, -2.749586949851067441 ) ) ;
#79826=EDGE_LOOP ( 'NONE', ( #17908, #49810, #86644, #69209 ) ) ;
#79827=CARTESIAN_POINT ( 'NONE',  ( 148.2390246527636748, 247.2048013555409511, 4.594050593750051981 ) ) ;
#79828=CARTESIAN_POINT ( 'NONE',  ( 181.3453648331101817, 267.8634245393459423, 16.44187752845164141 ) ) ;
#79829=CARTESIAN_POINT ( 'NONE',  ( 106.4801018922090066, 232.2833772461660544, -9.188101187500095079 ) ) ;
#79835=CARTESIAN_POINT ( 'NONE',  ( 157.1135969804030310, 258.5182628004787944, 17.19660297500358226 ) ) ;
#79837=CARTESIAN_POINT ( 'NONE',  ( 150.4620166971273534, 270.0391378017355919, -15.22190817129291673 ) ) ;
#79839=CARTESIAN_POINT ( 'NONE',  ( 192.9140677929238166, 263.8636187812822982, -4.540140315059590925 ) ) ;
#79840=CARTESIAN_POINT ( 'NONE',  ( 196.4501996009505831, 290.3852684645433442, -17.82325615854289680 ) ) ;
#79841=CARTESIAN_POINT ( 'NONE',  ( 189.7709616952058695, 300.0996391715700611, 4.806025422203243025 ) ) ;
#79842=CARTESIAN_POINT ( 'NONE',  ( 173.4032705993685965, 289.8532102436319633, -1.071672375802585675 ) ) ;
#79844=ORIENTED_EDGE ( 'NONE', *, *, #20682, .T. ) ;
#79846=CARTESIAN_POINT ( 'NONE',  ( 175.0839093973710305, 279.4057055686774902, 15.99633660845799987 ) ) ;
#79847=CARTESIAN_POINT ( 'NONE',  ( 191.9986677257686836, 264.8169910582080888, -10.25568683636180189 ) ) ;
#79849=EDGE_CURVE ( 'NONE', #93478, #38611, #68812, .T. ) ;
#79854=CARTESIAN_POINT ( 'NONE',  ( 148.6023484834014425, 275.2601776331305814, 7.517535991345212665 ) ) ;
#79855=VERTEX_POINT ( 'NONE', #10934 ) ;
#79859=CARTESIAN_POINT ( 'NONE',  ( 194.7451511902013124, 289.8320772759159354, -16.28529254116144287 ) ) ;
#79862=EDGE_CURVE ( 'NONE', #34753, #87476, #78585, .T. ) ;
#79863=CARTESIAN_POINT ( 'NONE',  ( 194.3442947553755005, 294.0328026529847421, -15.97648891113594871 ) ) ;
#79864=CYLINDRICAL_SURFACE ( 'NONE', #67811, 17.82106496071139645 ) ;
#79867=CARTESIAN_POINT ( 'NONE',  ( 187.2435932563332415, 292.1887571869974636, 12.29041050614439001 ) ) ;
#79868=CARTESIAN_POINT ( 'NONE',  ( 191.4685399627163633, 299.0137560639802814, 7.545791216288330716 ) ) ;
#79873=CARTESIAN_POINT ( 'NONE',  ( 202.9881971861223917, 279.0611244672630278, -15.16231470264511927 ) ) ;
#79876=CARTESIAN_POINT ( 'NONE',  ( 97.28760307318144385, 233.6427522451419065, 10.00000000000009415 ) ) ;
#79877=ORIENTED_EDGE ( 'NONE', *, *, #59265, .F. ) ;
#79879=ORIENTED_EDGE ( 'NONE', *, *, #69340, .F. ) ;
#79882=ORIENTED_EDGE ( 'NONE', *, *, #58549, .F. ) ;
#79883=CARTESIAN_POINT ( 'NONE',  ( 147.9167952901743206, 274.4475905950902188, -6.349683594314821100 ) ) ;
#79884=CARTESIAN_POINT ( 'NONE',  ( 189.7726967107949747, 264.4065126852114531, 11.24316165915873000 ) ) ;
#79885=CARTESIAN_POINT ( 'NONE',  ( 192.6170194583582429, 297.0245312260774995, -11.90166228306590490 ) ) ;
#79889=CARTESIAN_POINT ( 'NONE',  ( 131.9738982639959488, 240.8768266524160140, -9.188101187500091527 ) ) ;
#79891=CARTESIAN_POINT ( 'NONE',  ( 185.7372650184451857, 257.4645284076796656, -2.264991511946413505E-12 ) ) ;
#79895=CARTESIAN_POINT ( 'NONE',  ( 200.4137396061031211, 274.1951937318462456, 13.51466377508595507 ) ) ;
#79896=CARTESIAN_POINT ( 'NONE',  ( -22.42236680055709641, 157.8615022471902591, 0.000000000000000000 ) ) ;
#79898=CARTESIAN_POINT ( 'NONE',  ( 192.3158717363151595, 297.5461343812397104, 12.57290801860991003 ) ) ;
#79899=CARTESIAN_POINT ( 'NONE',  ( 156.0982710278114496, 278.5911654470725125, 7.232040771136105661 ) ) ;
#79902=CARTESIAN_POINT ( 'NONE',  ( 171.6386966857738230, 280.0180265567518063, 13.87489842761215009 ) ) ;
#79904=CARTESIAN_POINT ( 'NONE',  ( 177.5869845173387773, 255.5126858138248451, -8.405682457315087674 ) ) ;
#79907=CARTESIAN_POINT ( 'NONE',  ( 152.5049231584100653, 273.3283623610165023, 11.85969823726709826 ) ) ;
#79912=CARTESIAN_POINT ( 'NONE',  ( 205.0859877718122561, 268.9368413191317586, -3.038556538008958974 ) ) ;
#79913=CARTESIAN_POINT ( 'NONE',  ( 152.3230865050459784, 266.8156703379880810, -15.53149103319956303 ) ) ;
#79916=CARTESIAN_POINT ( 'NONE',  ( 202.8167949821795446, 279.3580017930215149, 15.61966256214195070 ) ) ;
#79918=CARTESIAN_POINT ( 'NONE',  ( 154.8138742624348367, 277.2620699001403750, -8.801558155086558699 ) ) ;
#79919=DIRECTION ( 'NONE',  ( -0.8660254037844387076, -0.4999999999999998890, -0.000000000000000000 ) ) ;
#79920=ORIENTED_EDGE ( 'NONE', *, *, #89482, .T. ) ;
#79921=B_SPLINE_SURFACE_WITH_KNOTS ( 'NONE', 3, 1, ( 
 ( #60360, #67482 ),
 ( #37081, #67986 ),
 ( #84719, #39053 ),
 ( #7680, #38057 ),
 ( #86237, #54248 ),
 ( #40057, #38567 ),
 ( #77072, #60856 ),
 ( #91821, #78090 ),
 ( #47167, #16771 ),
 ( #8679, #29979 ),
 ( #45662, #62867 ),
 ( #16273, #47663 ),
 ( #23867, #76586 ),
 ( #92326, #68970 ),
 ( #15258, #69966 ),
 ( #84232, #61861 ),
 ( #24382, #77597 ),
 ( #14779, #8185 ),
 ( #85221, #61369 ),
 ( #99401, #89 ),
 ( #69476, #22380 ),
 ( #580, #78597 ),
 ( #85745, #31464 ),
 ( #23364, #46155 ),
 ( #53278, #39548 ),
 ( #99893, #31963 ),
 ( #93823, #30479 ),
 ( #7171, #9182 ),
 ( #55254, #62356 ),
 ( #93310, #22874 ),
 ( #53759, #30972 ),
 ( #92810, #54759 ),
 ( #15766, #46671 ),
 ( #70471, #1086 ) ),
 .UNSPECIFIED., .T., .F., .F.,
 ( 4, 2, 2, 2, 2, 2, 2, 2, 2, 2, 2, 2, 2, 2, 2, 2, 4 ),
 ( 2, 2 ),
 ( 0.000000000000000000, 0.06250000000000000000, 0.1250000000000000000, 0.1875000000000000000, 0.2500000000000000000, 0.3125000000000000000, 0.3750000000000000000, 0.4375000000000000000, 0.5000000000000000000, 0.5625000000000000000, 0.6250000000000000000, 0.6875000000000000000, 0.7500000000000000000, 0.8125000000000000000, 0.8750000000000000000, 0.9375000000000000000, 1.000000000000000000 ),
 ( 0.000000000000000000, 1.000000000000000000 ),
 .UNSPECIFIED. ) ;
#79922=B_SPLINE_CURVE_WITH_KNOTS ( 'NONE', 3,
 ( #1315, #63100, #40282, #94046, #55481, #24599 ),
 .UNSPECIFIED., .F., .F.,
 ( 4, 2, 4 ),
 ( 0.01862806261678935302, 0.02313791776344208823, 0.02764777291009481996 ),
 .UNSPECIFIED. ) ;
#79924=CARTESIAN_POINT ( 'NONE',  ( 152.7122812589697958, 277.9324518551267147, 6.933031942251369983 ) ) ;
#79926=CARTESIAN_POINT ( 'NONE',  ( 152.7153488183568300, 266.1362520814392951, 17.33540622643059237 ) ) ;
#79929=CARTESIAN_POINT ( 'NONE',  ( -13.54586673536430830, 172.1744531367911293, 4.594050593750047540 ) ) ;
#79930=CARTESIAN_POINT ( 'NONE',  ( 91.59511671678144751, 229.8149278399160664, 9.188101187500093303 ) ) ;
#79931=CARTESIAN_POINT ( 'NONE',  ( 203.3740894404336927, 278.3927394765486838, -15.19753795879846869 ) ) ;
#79934=EDGE_CURVE ( 'NONE', #31705, #98801, #36211, .T. ) ;
#79936=CARTESIAN_POINT ( 'NONE',  ( 205.7872507830675204, 272.2130214242461079, -9.506855900917111413 ) ) ;
#79937=CARTESIAN_POINT ( 'NONE',  ( 164.1570551735447623, 284.3421986849189693, 5.865652139141318777 ) ) ;
#79938=CARTESIAN_POINT ( 'NONE',  ( 189.8897621674675804, 300.5079289680896864, -1.468582484996752147 ) ) ;
#79939=CARTESIAN_POINT ( 'NONE',  ( 208.3863431123642727, 269.7112614563416173, -1.693909372230378851 ) ) ;
#79940=CARTESIAN_POINT ( 'NONE',  ( 178.0890608223913603, 290.4326850333343373, 9.911865951459251534 ) ) ;
#79941=CARTESIAN_POINT ( 'NONE',  ( -22.42236680055709641, 157.8615022471902591, 0.000000000000000000 ) ) ;
#79944=CARTESIAN_POINT ( 'NONE',  ( 83.43119661263041564, 225.6427522451419065, -10.00000000000009592 ) ) ;
#79946=CARTESIAN_POINT ( 'NONE',  ( 50.62146334811270521, 200.0333772461660544, 9.188101187500095079 ) ) ;
#79948=CARTESIAN_POINT ( 'NONE',  ( 71.05451054047556170, 202.6423013555409796, -4.594050593750043987 ) ) ;
#79949=CARTESIAN_POINT ( 'NONE',  ( 207.6129110656513035, 271.0508850574501025, -5.265106572941297358 ) ) ;
#79951=CARTESIAN_POINT ( 'NONE',  ( 163.5572657305692132, 257.9363112301150522, 15.55976473370433766 ) ) ;
#79953=CARTESIAN_POINT ( 'NONE',  ( 152.1502187761652749, 267.1150860273985472, 15.41609850895314615 ) ) ;
#79954=CARTESIAN_POINT ( 'NONE',  ( 176.4985344937902880, 269.9855544425572020, -17.33307642928837566 ) ) ;
#79957=LINE ( 'NONE', #43397, #68493 ) ;
#79958=ORIENTED_EDGE ( 'NONE', *, *, #36443, .T. ) ;
#79960=CARTESIAN_POINT ( 'NONE',  ( 79.14634863314513780, 210.3768266524160140, 9.188101187500096856 ) ) ;
#79964=CARTESIAN_POINT ( 'NONE',  ( 201.8494044615141547, 281.0335713255741439, 17.80331436090332176 ) ) ;
#79965=ORIENTED_EDGE ( 'NONE', *, *, #31281, .T. ) ;
#79967=CARTESIAN_POINT ( 'NONE',  ( 193.3835840830572295, 288.4008497395175254, 16.05775961610054026 ) ) ;
#79969=CARTESIAN_POINT ( 'NONE',  ( 130.4311169673963775, 246.1115022471902591, 10.00000000000009592 ) ) ;
#79970=CARTESIAN_POINT ( 'NONE',  ( 21.76528272068881265, 171.8262482093457777, 3.021315404115420679E-15 ) ) ;
#79972=VERTEX_POINT ( 'NONE', #1830 ) ;
#79973=CARTESIAN_POINT ( 'NONE',  ( 184.7218640569926720, 271.1400913308660279, 16.40603036354897171 ) ) ;
#79975=CARTESIAN_POINT ( 'NONE',  ( 162.6774150396764469, 248.8814472377480911, 10.88033986792731689 ) ) ;
#79977=CARTESIAN_POINT ( 'NONE',  ( 201.1388841337167435, 282.2642286331299601, -18.17233400608081340 ) ) ;
#79978=ADVANCED_FACE ( 'NONE', ( #8913 ), #79864, .T. ) ;
#79979=VERTEX_POINT ( 'NONE', #86984 ) ;
#79983=CARTESIAN_POINT ( 'NONE',  ( 188.9102852820520582, 290.7616905290360023, 14.53875897011772445 ) ) ;
#79984=CARTESIAN_POINT ( 'NONE',  ( 171.0307695606911125, 249.8159844473073861, 2.774073808362228721 ) ) ;
#79985=CARTESIAN_POINT ( 'NONE',  ( 178.9281327940277606, 284.0931116521168747, -15.58854622419240243 ) ) ;
#79986=ORIENTED_EDGE ( 'NONE', *, *, #71734, .T. ) ;
#79994=ORIENTED_EDGE ( 'NONE', *, *, #57821, .F. ) ;
#79995=CARTESIAN_POINT ( 'NONE',  ( 183.0367609120576162, 295.8830680031519478, 0.5753348830509616985 ) ) ;
#79996=CARTESIAN_POINT ( 'NONE',  ( 163.7707306762541748, 246.9877690064858484, 7.021959502997312086 ) ) ;
#79997=CARTESIAN_POINT ( 'NONE',  ( 194.6356465353167948, 293.5281665672507643, -16.13180903283129197 ) ) ;
#79999=CARTESIAN_POINT ( 'NONE',  ( 194.3562588153086779, 294.0120802933159325, 14.11474987148825200 ) ) ;
#80001=CARTESIAN_POINT ( 'NONE',  ( 167.2638507335506688, 272.3832265362266867, -17.29346045784080133 ) ) ;
#80002=CARTESIAN_POINT ( 'NONE',  ( 164.5410109126144960, 245.6536045010434748, 5.739447577850491200 ) ) ;
#80003=CARTESIAN_POINT ( 'NONE',  ( 166.2521479564098854, 265.4651998704476341, 16.55286243553473469 ) ) ;
#80005=CARTESIAN_POINT ( 'NONE',  ( 82.25819355828922141, 227.4869531367911293, 4.594050593750046652 ) ) ;
#80007=CARTESIAN_POINT ( 'NONE',  ( 183.6422324172568210, 264.5785696717482551, 14.31652553825990104 ) ) ;
#80009=ORIENTED_EDGE ( 'NONE', *, *, #89430, .T. ) ;
#80011=CARTESIAN_POINT ( 'NONE',  ( 165.8785007526746540, 265.8076673077522969, -16.62180286104441507 ) ) ;
#80012=ORIENTED_EDGE ( 'NONE', *, *, #26555, .F. ) ;
#80017=CARTESIAN_POINT ( 'NONE',  ( 206.2313482792274328, 273.4438219973828268, -9.403385562213845361 ) ) ;
#80018=CARTESIAN_POINT ( 'NONE',  ( 160.3733185927383715, 282.5102941377067509, 6.606729549618552078 ) ) ;
#80019=CARTESIAN_POINT ( 'NONE',  ( 92.19068272976576850, 224.0333772461660544, 9.188101187500095079 ) ) ;
#80022=CARTESIAN_POINT ( 'NONE',  ( 161.9020140854683234, 250.2244810866738760, -14.08518779869104343 ) ) ;
#80023=ORIENTED_EDGE ( 'NONE', *, *, #14602, .F. ) ;
#80024=B_SPLINE_CURVE_WITH_KNOTS ( 'NONE', 3,
 ( #41209, #42214, #66026, #27038 ),
 .UNSPECIFIED., .F., .F.,
 ( 4, 4 ),
 ( 0.006155465570655065458, 0.01116048267587303570 ),
 .UNSPECIFIED. ) ;
#80026=EDGE_CURVE ( 'NONE', #4372, #82839, #79237, .T. ) ;
#80027=CARTESIAN_POINT ( 'NONE',  ( 165.5845933190392998, 285.3686551174989745, 0.6228737942997026877 ) ) ;
#80029=CARTESIAN_POINT ( 'NONE',  ( -15.29569941879559281, 168.6427522451418781, -10.00000000000009415 ) ) ;
#80032=CARTESIAN_POINT ( 'NONE',  ( 204.3227106360847927, 276.7496793685443208, 13.60086062244164573 ) ) ;
#80033=CARTESIAN_POINT ( 'NONE',  ( 160.5595428929208310, 275.8229991552611864, 14.13237683250033605 ) ) ;
#80035=CARTESIAN_POINT ( 'NONE',  ( 189.1550430427957110, 269.9471506065882522, 14.45832818640694484 ) ) ;
#80036=CARTESIAN_POINT ( 'NONE',  ( 174.6413940958611875, 283.8768656314015857, 13.74801433323937694 ) ) ;
#80040=DIRECTION ( 'NONE',  ( 0.4999999999999998890, -0.8660254037844385966, 0.000000000000000000 ) ) ;
#80042=CARTESIAN_POINT ( 'NONE',  ( 203.3946109532447224, 276.3571951737117729, -14.55139583984842133 ) ) ;
#80043=CARTESIAN_POINT ( 'NONE',  ( 200.1385401540174769, 283.9968752310148830, 17.30012534137638625 ) ) ;
#80045=CARTESIAN_POINT ( 'NONE',  ( 193.5910456581822814, 274.5466812142672097, -16.41199759748324283 ) ) ;
#80047=CARTESIAN_POINT ( 'NONE',  ( 174.9064783932017235, 290.1930726575905055, -6.379950440565356651 ) ) ;
#80049=FACE_OUTER_BOUND ( 'NONE', #75092, .T. ) ;
#80053=CARTESIAN_POINT ( 'NONE',  ( 180.6167065349397944, 266.8569723307038544, -14.77775250061756296 ) ) ;
#80054=CARTESIAN_POINT ( 'NONE',  ( 184.9023284419889137, 266.2659532107462041, 13.18801441717285883 ) ) ;
#80055=CARTESIAN_POINT ( 'NONE',  ( 199.1341087029324513, 281.8436105099906968, -16.59105901670938010 ) ) ;
#80060=CARTESIAN_POINT ( 'NONE',  ( 159.4413293807720606, 272.0932757909793622, -14.74450807601864888 ) ) ;
#80062=CARTESIAN_POINT ( 'NONE',  ( 207.1770866921659717, 271.8057550155037347, -5.569195235244989384 ) ) ;
#80063=CARTESIAN_POINT ( 'NONE',  ( -0.9884983804899494242, 179.4244531367911577, -4.594050593750046652 ) ) ;
#80069=CARTESIAN_POINT ( 'NONE',  ( 30.81113223654366706, 188.5958772461660544, -9.188101187500095079 ) ) ;
#80070=CARTESIAN_POINT ( 'NONE',  ( 161.1884843536000744, 251.4603508349806873, 13.21272898143761942 ) ) ;
#80073=CARTESIAN_POINT ( 'NONE',  ( 199.5204482824095464, 267.4377498580035422, -6.650170480489714819 ) ) ;
#80074=CARTESIAN_POINT ( 'NONE',  ( 191.3610003135137276, 299.2000202002271294, -9.855749861282104618 ) ) ;
#80075=CARTESIAN_POINT ( 'NONE',  ( 196.3076213506950296, 290.6322212380402448, 17.33673088264725592 ) ) ;
#80079=EDGE_CURVE ( 'NONE', #62092, #66923, #86876, .T. ) ;
#80083=CARTESIAN_POINT ( 'NONE',  ( 182.7078241176633639, 296.4455565966184167, 1.853464302320349200 ) ) ;
#80084=CARTESIAN_POINT ( 'NONE',  ( 82.43887584100873767, 211.7365022471901739, -10.00000000000009059 ) ) ;
#80087=CARTESIAN_POINT ( 'NONE',  ( 33.95012722949724093, 202.6589784336661637, -6.496448406907675876E-16 ) ) ;
#80088=CARTESIAN_POINT ( 'NONE',  ( 197.8809552785519656, 287.9071269377202498, 17.61728046362068412 ) ) ;
#80091=CARTESIAN_POINT ( 'NONE',  ( 198.4782858197754649, 286.8725200914082620, -17.44895083299520522 ) ) ;
#80095=CARTESIAN_POINT ( 'NONE',  ( 170.0073542471708947, 285.8791242548903142, 7.485010625345761781 ) ) ;
#80096=CARTESIAN_POINT ( 'NONE',  ( 168.2008345946905479, 248.1884056956802453, -5.064766917302788052 ) ) ;
#80097=CARTESIAN_POINT ( 'NONE',  ( 147.1485523687439070, 275.7782263675629792, 6.742590758227570369 ) ) ;
#80100=CARTESIAN_POINT ( 'NONE',  ( 163.1691520398773321, 248.0297337694385931, 11.21816141384514331 ) ) ;
#80101=CARTESIAN_POINT ( 'NONE',  ( 149.0598351764325002, 272.4677874370131576, -11.59078276432863674 ) ) ;
#80102=CARTESIAN_POINT ( 'NONE',  ( 174.6566889969473948, 257.2801211409499160, 11.41830854748823221 ) ) ;
#80103=ORIENTED_EDGE ( 'NONE', *, *, #16510, .F. ) ;
#80106=CARTESIAN_POINT ( 'NONE',  ( 171.6197681575868899, 252.4849835280233492, 8.664910895864313289 ) ) ;
#80108=EDGE_CURVE ( 'NONE', #68153, #26850, #27616, .T. ) ;
#80109=ORIENTED_EDGE ( 'NONE', *, *, #79165, .F. ) ;
#80110=CARTESIAN_POINT ( 'NONE',  ( 179.5754329387666246, 282.6374756363382517, 15.15522646414435926 ) ) ;
#80111=CARTESIAN_POINT ( 'NONE',  ( 144.9899443387551798, 254.5170451491295296, 0.000000000000000000 ) ) ;
#80112=CARTESIAN_POINT ( 'NONE',  ( 177.3409152927461889, 255.9687924550131299, -7.086473103942450003 ) ) ;
#80113=CARTESIAN_POINT ( 'NONE',  ( 167.4035461121217736, 269.8829485561403771, 17.70625493734027600 ) ) ;
#80114=AXIS2_PLACEMENT_3D ( 'NONE', #74147, #65523, #19940 ) ;
#80115=ORIENTED_EDGE ( 'NONE', *, *, #12887, .F. ) ;
#80116=ORIENTED_EDGE ( 'NONE', *, *, #38962, .T. ) ;
#80117=CARTESIAN_POINT ( 'NONE',  ( 161.1150691641480535, 251.5875096731584506, -13.48836942566120101 ) ) ;
#80121=CARTESIAN_POINT ( 'NONE',  ( 152.6873874250818517, 266.1846826352417565, -16.66598363829485763 ) ) ;
#80125=CARTESIAN_POINT ( 'NONE',  ( 157.8719920515997046, 257.2046840049564480, -17.69857783492101433 ) ) ;
#80127=CARTESIAN_POINT ( 'NONE',  ( 115.3025621453804490, 243.5024278399160949, 9.188101187500095079 ) ) ;
#80128=CARTESIAN_POINT ( 'NONE',  ( 196.3507576896697344, 290.5575069072837664, -17.68249398312240928 ) ) ;
#80129=CARTESIAN_POINT ( 'NONE',  ( 79.03685904533298867, 227.9860189848785126, -2.679491924311252493 ) ) ;
#80131=CARTESIAN_POINT ( 'NONE',  ( 164.4678285797544106, 245.7803600197737524, -6.875991496205872799 ) ) ;
#80134=CARTESIAN_POINT ( 'NONE',  ( 157.4027210288906531, 258.5085945389839139, 16.84379666775977213 ) ) ;
#80136=CARTESIAN_POINT ( 'NONE',  ( 60.25564886944957976, 217.8464784336661637, 1.353441290958777525E-15 ) ) ;
#80140=CARTESIAN_POINT ( 'NONE',  ( 172.6733913832073597, 271.7377284239155415, 17.68482103120430438 ) ) ;
#80143=CARTESIAN_POINT ( 'NONE',  ( 199.3863224916975412, 265.3452568596479182, 0.1349916258391212209 ) ) ;
#80144=CARTESIAN_POINT ( 'NONE',  ( 189.0172135941854492, 296.3830391516955274, 10.71955688187805222 ) ) ;
#80146=CARTESIAN_POINT ( 'NONE',  ( 171.8062308653840660, 259.5681322378169398, -13.86186043045860394 ) ) ;
#80148=CARTESIAN_POINT ( 'NONE',  ( 161.1678764334604921, 258.7517053225153063, -16.56551366227781230 ) ) ;
#80149=CARTESIAN_POINT ( 'NONE',  ( 206.8409998872672020, 269.9682599439536261, 1.764008356409222156 ) ) ;
#80150=CARTESIAN_POINT ( 'NONE',  ( 190.6893905452545823, 300.3632824417117604, 3.294993852933539191 ) ) ;
#80151=CARTESIAN_POINT ( 'NONE',  ( 177.2279885846477328, 269.5037953214600179, 16.10890805395466785 ) ) ;
#80154=CARTESIAN_POINT ( 'NONE',  ( 126.3716228836088362, 253.7677522451419065, -5.000000000000047962 ) ) ;
#80155=CARTESIAN_POINT ( 'NONE',  ( 167.5316711859411214, 256.4999896070169143, 13.69272852843613819 ) ) ;
#80157=CARTESIAN_POINT ( 'NONE',  ( 123.0967907794404113, 248.0024278399161517, 9.188101187500095079 ) ) ;
#80161=EDGE_CURVE ( 'NONE', #20951, #68688, #24003, .T. ) ;
#80162=CARTESIAN_POINT ( 'NONE',  ( 164.9101359252495627, 286.5608941336866451, 1.040025780022917790 ) ) ;
#80165=CARTESIAN_POINT ( 'NONE',  ( 177.3593506507800441, 255.0021141411331200, 4.887753322990675997 ) ) ;
#80168=CARTESIAN_POINT ( 'NONE',  ( 158.2519735457114791, 274.8320027810396482, -12.54673606207468950 ) ) ;
#80169=CARTESIAN_POINT ( 'NONE',  ( 182.8880264097929000, 260.9253942413262735, 9.506296218588019542 ) ) ;
#80170=CARTESIAN_POINT ( 'NONE',  ( 165.0748171242677245, 244.7290250210644729, -1.867635796467185028 ) ) ;
#80173=CARTESIAN_POINT ( 'NONE',  ( 195.2233764540819152, 263.4883587362652975, 0.8587759651238419112 ) ) ;
#80174=CARTESIAN_POINT ( 'NONE',  ( 187.4912959212919361, 285.9308727613615133, 16.80547087661522809 ) ) ;
#80176=CARTESIAN_POINT ( 'NONE',  ( 67.18419919549008057, 209.5958772461660544, -9.188101187500095079 ) ) ;
#80177=CARTESIAN_POINT ( 'NONE',  ( 170.6644942104857989, 250.4764242134850463, 3.560033027948075190 ) ) ;
#80179=EDGE_CURVE ( 'NONE', #55644, #98181, #55864, .T. ) ;
#80180=CARTESIAN_POINT ( 'NONE',  ( 173.1676448813863374, 261.4169956538293036, 14.42742222810248620 ) ) ;
#80181=CARTESIAN_POINT ( 'NONE',  ( 152.2460257044392620, 278.3500712430857789, -1.624206099058958630 ) ) ;
#80182=CARTESIAN_POINT ( 'NONE',  ( 169.4020686296666156, 285.0774647284627576, -8.180577219304280945 ) ) ;
#80184=CARTESIAN_POINT ( 'NONE',  ( 203.2732885619977026, 278.5673317194472247, -16.64305493556850024 ) ) ;
#80185=CARTESIAN_POINT ( 'NONE',  ( 157.3056943055385659, 271.4195445804601263, -14.62320538668267922 ) ) ;
#80186=CARTESIAN_POINT ( 'NONE',  ( 117.2783561438722586, 238.5177522451418497, -10.00000000000009592 ) ) ;
#80189=CARTESIAN_POINT ( 'NONE',  ( 148.3707431749605234, 273.6613297946520902, 8.912574527564540716 ) ) ;
#80190=CARTESIAN_POINT ( 'NONE',  ( -11.70556275232237908, 173.2369531367911293, -4.594050593750048428 ) ) ;
#80191=CARTESIAN_POINT ( 'NONE',  ( 37.36027580478099708, 198.5024278399160664, 9.188101187500095079 ) ) ;
#80192=DIRECTION ( 'NONE',  ( 0.4999999999999998890, -0.8660254037844385966, 0.000000000000000000 ) ) ;
#80196=CARTESIAN_POINT ( 'NONE',  ( 192.6090810369716166, 292.3580219496548693, -14.34990427975804472 ) ) ;
#80197=CARTESIAN_POINT ( 'NONE',  ( 147.5492216329511166, 275.0842468449245644, 4.751613690710122739 ) ) ;
#80199=EDGE_CURVE ( 'NONE', #63065, #6345, #68670, .T. ) ;
#80201=CARTESIAN_POINT ( 'NONE',  ( 61.41971759977592171, 216.2677522451419065, -5.000000000000047962 ) ) ;
#80203=CARTESIAN_POINT ( 'NONE',  ( 180.8720737262704290, 256.3169785306307631, 1.340588092569421130 ) ) ;
#80204=CARTESIAN_POINT ( 'NONE',  ( 204.8057697639265768, 275.9129964160624695, -12.68356524114230766 ) ) ;
#80207=CARTESIAN_POINT ( 'NONE',  ( 32.93109025799825673, 196.4865022471903160, -10.00000000000009415 ) ) ;
#80208=CARTESIAN_POINT ( 'NONE',  ( 185.1158863356004076, 294.2829762544421328, 9.788930817016709085 ) ) ;
#80209=CARTESIAN_POINT ( 'NONE',  ( 202.9972156839127990, 279.0455039708822937, 16.77197898838388213 ) ) ;
#80210=CARTESIAN_POINT ( 'NONE',  ( 12.46239254174337852, 171.8768266524160140, -9.188101187500091527 ) ) ;
#80212=CARTESIAN_POINT ( 'NONE',  ( 164.0397259771397955, 252.5309334026060242, 13.28083819032488577 ) ) ;
#80213=CARTESIAN_POINT ( 'NONE',  ( 192.0645969571214096, 297.9813550654635605, 11.46542907566974812 ) ) ;
#80215=CARTESIAN_POINT ( 'NONE',  ( 187.1539397334955765, 259.1171307905131584, -2.424303653640247802 ) ) ;
#80217=CARTESIAN_POINT ( 'NONE',  ( 154.9683083969241011, 262.2340116239618055, 18.33261662430134109 ) ) ;
#80218=CARTESIAN_POINT ( 'NONE',  ( 149.2593905435863348, 272.1221474021800759, -12.98626158366800176 ) ) ;
#80221=CARTESIAN_POINT ( 'NONE',  ( 153.4346252566255373, 277.7752686862202154, -5.213536763656924755 ) ) ;
#80223=CARTESIAN_POINT ( 'NONE',  ( 68.07728789491670796, 220.1115022471903160, -5.000000000000047962 ) ) ;
#80225=CARTESIAN_POINT ( 'NONE',  ( 192.9765683580851885, 270.2547331158643829, -14.50234918781434423 ) ) ;
#80231=CARTESIAN_POINT ( 'NONE',  ( 152.8890098693866832, 266.6752310492291826, 15.93618651899761041 ) ) ;
#80232=CARTESIAN_POINT ( 'NONE',  ( 207.6918009085542849, 270.9142438413412037, 7.009114282139513818 ) ) ;
#80236=ORIENTED_EDGE ( 'NONE', *, *, #84522, .T. ) ;
#80238=CARTESIAN_POINT ( 'NONE',  ( 193.6564271169084464, 262.6014873983580742, -4.146719891036213745 ) ) ;
#80242=CARTESIAN_POINT ( 'NONE',  ( 174.3997061797743982, 262.4591641033748033, 14.57197903150277796 ) ) ;
#80248=ORIENTED_EDGE ( 'NONE', *, *, #16276, .T. ) ;
#80249=CARTESIAN_POINT ( 'NONE',  ( 174.0017767277458347, 267.4700837321790914, 16.54826822959725874 ) ) ;
#80250=CARTESIAN_POINT ( 'NONE',  ( 166.1418958215914188, 273.9600516718538756, -15.29462885050179644 ) ) ;
#80254=CARTESIAN_POINT ( 'NONE',  ( -17.42236680055705023, 149.2012482093457777, 0.000000000000000000 ) ) ;
#80255=CARTESIAN_POINT ( 'NONE',  ( 202.8499463704053198, 279.3005819042728604, 17.04674939340617001 ) ) ;
#80256=ORIENTED_EDGE ( 'NONE', *, *, #47166, .T. ) ;
#80257=ORIENTED_EDGE ( 'NONE', *, *, #79849, .F. ) ;
#80258=CARTESIAN_POINT ( 'NONE',  ( 156.9270364742972959, 266.2560578317317095, -16.47839810797669102 ) ) ;
#80261=ORIENTED_EDGE ( 'NONE', *, *, #23907, .T. ) ;
#80263=EDGE_LOOP ( 'NONE', ( #65128, #7974, #45349, #96107 ) ) ;
#80265=CARTESIAN_POINT ( 'NONE',  ( 147.9374661616566016, 274.4117875954463557, 6.504250773332477920 ) ) ;
#80266=CARTESIAN_POINT ( 'NONE',  ( 177.6634127208063205, 289.0610186271913449, -9.329510868619479425 ) ) ;
#80268=CARTESIAN_POINT ( 'NONE',  ( 200.0350729207520430, 281.2229895077505830, -17.27079589148639371 ) ) ;
#80269=CARTESIAN_POINT ( 'NONE',  ( 176.3782206303458224, 290.4613412261181793, 6.112157577772562078 ) ) ;
#80270=CARTESIAN_POINT ( 'NONE',  ( 146.6138605399200117, 276.7043397814778132, -0.5394499176159462950 ) ) ;
#80272=CARTESIAN_POINT ( 'NONE',  ( 100.8442274002074441, 217.4824982072973683, 3.021315404115420679E-15 ) ) ;
#80274=CARTESIAN_POINT ( 'NONE',  ( 206.3907062969896060, 273.1678058140250300, 11.56942460516550675 ) ) ;
#80276=CARTESIAN_POINT ( 'NONE',  ( 164.8849641302980444, 245.0578600525887794, 2.884140591399200648 ) ) ;
#80280=CARTESIAN_POINT ( 'NONE',  ( 147.4586881104295344, 275.2410555057202828, -3.245347276174700202 ) ) ;
#80281=CARTESIAN_POINT ( 'NONE',  ( 171.3429355605559294, 259.3079905075224474, -13.88314242353945360 ) ) ;
#80282=CARTESIAN_POINT ( 'NONE',  ( 163.6678477032174044, 247.6361333164444432, 7.542859481152206058 ) ) ;
#80284=CARTESIAN_POINT ( 'NONE',  ( 161.1238074876215478, 251.5723744529297505, 13.42537408252843179 ) ) ;
#80285=CARTESIAN_POINT ( 'NONE',  ( 190.5677878487744863, 300.5739044903526178, -1.037535106822473630 ) ) ;
#80287=CARTESIAN_POINT ( 'NONE',  ( -27.42236680055714260, 166.5217562850347406, 1.224646799147364892E-15 ) ) ;
#80289=CARTESIAN_POINT ( 'NONE',  ( 19.85049821812295079, 172.2677522451417929, -5.000000000000041744 ) ) ;
#80290=CARTESIAN_POINT ( 'NONE',  ( 103.5572661544365332, 230.5958772461660260, -9.188101187500095079 ) ) ;
#80292=CARTESIAN_POINT ( 'NONE',  ( 183.5238647517005006, 297.0535124292885598, -2.834911233012364473 ) ) ;
#80293=CARTESIAN_POINT ( 'NONE',  ( 99.95784806818352308, 218.5177522451417929, 5.000000000000051514 ) ) ;
#80294=CARTESIAN_POINT ( 'NONE',  ( 163.1306191313178431, 248.0964747248268338, 10.50682697533535048 ) ) ;
#80295=CARTESIAN_POINT ( 'NONE',  ( 16.25090658753528317, 186.3149278399161233, 9.188101187500093303 ) ) ;
#80297=CARTESIAN_POINT ( 'NONE',  ( 170.7981279722302190, 250.1199420982161996, 6.208364627926498791 ) ) ;
#80299=ORIENTED_EDGE ( 'NONE', *, *, #75237, .T. ) ;
#80304=EDGE_CURVE ( 'NONE', #35723, #39680, #45698, .T. ) ;
#80307=CARTESIAN_POINT ( 'NONE',  ( 207.2337123599961899, 271.7076764818092443, -5.443417788256701861 ) ) ;
#80308=CARTESIAN_POINT ( 'NONE',  ( 182.1091148644272550, 284.7077012260656375, 14.92368712289904487 ) ) ;
#80309=CARTESIAN_POINT ( 'NONE',  ( 97.45544333237508283, 238.6199935810941213, 2.679491924311251605 ) ) ;
#80310=CARTESIAN_POINT ( 'NONE',  ( 45.15450443884093090, 203.0024278399160949, 9.188101187500095079 ) ) ;
#80311=CARTESIAN_POINT ( 'NONE',  ( 72.24503514708140983, 222.5177522451419065, 5.000000000000046185 ) ) ;
#80312=VERTEX_POINT ( 'NONE', #54887 ) ;
#80314=CARTESIAN_POINT ( 'NONE',  ( 181.8515780981809371, 260.7328092829080219, -10.50361218802076024 ) ) ;
#80315=CARTESIAN_POINT ( 'NONE',  ( -5.074968980656518802, 174.0024278399160664, -9.188101187500093303 ) ) ;
#80317=CARTESIAN_POINT ( 'NONE',  ( 198.5954523381739989, 286.6695817285962562, -18.45134152028667174 ) ) ;
#80320=CARTESIAN_POINT ( 'NONE',  ( 192.7705129102570822, 296.7586727687594816, -13.39629674907774692 ) ) ;
#80322=CARTESIAN_POINT ( 'NONE',  ( 164.0741338217690668, 246.4622593432776796, 7.359073626423302983 ) ) ;
#80323=CARTESIAN_POINT ( 'NONE',  ( 191.0724301404414689, 299.6998384015373063, -9.342134220577969828 ) ) ;
#80324=CARTESIAN_POINT ( 'NONE',  ( 164.5416088356626290, 245.6525688679454618, -1.463507744092769292 ) ) ;
#80329=CARTESIAN_POINT ( 'NONE',  ( 1.032487885271483163, 164.7365022471902307, 10.00000000000009592 ) ) ;
#80330=CARTESIAN_POINT ( 'NONE',  ( 181.1229545130053111, 268.2492853531657602, 15.68939201437969899 ) ) ;
#80331=CARTESIAN_POINT ( 'NONE',  ( 129.7005815790617760, 239.5643266524159856, -9.188101187500093303 ) ) ;
#80334=DIRECTION ( 'NONE',  ( 0.8660254037844395958, 0.4999999999999985567, 0.000000000000000000 ) ) ;
#80335=CARTESIAN_POINT ( 'NONE',  ( 157.3988263959001870, 258.0242309610243865, 16.72376558639979294 ) ) ;
#80336=CARTESIAN_POINT ( 'NONE',  ( 113.8346084569740242, 224.9824982072974251, 3.021315404115420679E-15 ) ) ;
#80337=EDGE_CURVE ( 'NONE', #9864, #10695, #12009, .T. ) ;
#80338=CARTESIAN_POINT ( 'NONE',  ( 190.6912771110283131, 300.3600148139396993, -7.801888377467689040 ) ) ;
#80339=B_SPLINE_CURVE_WITH_KNOTS ( 'NONE', 3,
 ( #41996, #72932, #88663, #19230 ),
 .UNSPECIFIED., .F., .F.,
 ( 4, 4 ),
 ( 0.000000000000000000, 0.0002476878907693983085 ),
 .UNSPECIFIED. ) ;
#80341=CARTESIAN_POINT ( 'NONE',  ( 189.6628273826063378, 261.3601078589450708, -4.481571141829256533 ) ) ;
#80342=CARTESIAN_POINT ( 'NONE',  ( 196.3286486926436680, 290.5958008134369948, -16.58330917766970458 ) ) ;
#80343=CARTESIAN_POINT ( 'NONE',  ( 206.7596416265183734, 271.4678399409689291, 6.202658291405857227 ) ) ;
#80344=CARTESIAN_POINT ( 'NONE',  ( 176.3864270403830687, 292.4019977604870064, -1.109940439014482694 ) ) ;
#80346=VERTEX_POINT ( 'NONE', #18920 ) ;
#80348=CARTESIAN_POINT ( 'NONE',  ( 189.0689802957956260, 269.8288687927027354, -15.50864081522695415 ) ) ;
#80349=CARTESIAN_POINT ( 'NONE',  ( 167.8099530253072089, 271.3928698661641761, -17.53051755021046532 ) ) ;
#80351=CARTESIAN_POINT ( 'NONE',  ( 196.4217682013366186, 270.9315512130719981, 12.02672033859111700 ) ) ;
#80354=CARTESIAN_POINT ( 'NONE',  ( 192.8323852661406761, 296.6515067047851062, 11.86505947732313615 ) ) ;
#80356=CARTESIAN_POINT ( 'NONE',  ( 199.9108924079315841, 281.4061427919369294, 17.32562639834143781 ) ) ;
#80358=CARTESIAN_POINT ( 'NONE',  ( 173.9975664532395285, 272.8775942563314629, -16.35843707697202021 ) ) ;
#80361=CARTESIAN_POINT ( 'NONE',  ( 148.2670916631250861, 273.8408594794321971, -7.980554973576580835 ) ) ;
#80363=ORIENTED_EDGE ( 'NONE', *, *, #61906, .T. ) ;
#80366=CARTESIAN_POINT ( 'NONE',  ( 151.4159295687746294, 268.3869122420484814, 14.78076517566594106 ) ) ;
#80373=CARTESIAN_POINT ( 'NONE',  ( 203.3349860717029571, 278.4604684979374838, -16.59553970625579566 ) ) ;
#80378=EDGE_LOOP ( 'NONE', ( #42833, #75364, #82726, #76114 ) ) ;
#80381=ORIENTED_EDGE ( 'NONE', *, *, #24228, .T. ) ;
#80382=CARTESIAN_POINT ( 'NONE',  ( 172.9882089762378712, 271.0907866236487394, 16.42842503185412539 ) ) ;
#80383=CARTESIAN_POINT ( 'NONE',  ( 202.9547455376043672, 279.1190644220934018, -15.19669173352461478 ) ) ;
#80385=ADVANCED_BREP_SHAPE_REPRESENTATION ( '', ( #45023, #68784 ), #59069 ) ;
#80387=CARTESIAN_POINT ( 'NONE',  ( 161.0951265809451627, 254.6677910432329384, -15.15446908189199782 ) ) ;
#80389=CARTESIAN_POINT ( 'NONE',  ( 146.8312060062178830, 276.3278863910550172, -4.807241325481028227 ) ) ;
#80390=CARTESIAN_POINT ( 'NONE',  ( 201.3053499423511425, 281.9759013948520874, -16.75960365258566398 ) ) ;
#80391=EDGE_CURVE ( 'NONE', #49558, #43311, #83256, .T. ) ;
#80393=CARTESIAN_POINT ( 'NONE',  ( 157.6399499600617560, 280.8244316517132120, 2.084453808153418297 ) ) ;
#80394=CARTESIAN_POINT ( 'NONE',  ( 138.6312950077063135, 250.8458772461660260, 9.188101187500095079 ) ) ;
#80401=VECTOR ( 'NONE', #44953, 1000.000000000000000 ) ;
#80402=CARTESIAN_POINT ( 'NONE',  ( 202.4943568615953779, 279.9164810001701085, 17.09064351659286984 ) ) ;
#80404=CARTESIAN_POINT ( 'NONE',  ( 147.4541998938148026, 275.2488293249323874, 3.198773118013638950 ) ) ;
#80405=CARTESIAN_POINT ( 'NONE',  ( 152.9604666561868669, 277.5026710028543562, 6.707571967777091970 ) ) ;
#80406=CARTESIAN_POINT ( 'NONE',  ( 152.8721808860877616, 265.8646109718731623, -17.65676496037632504 ) ) ;
#80409=CARTESIAN_POINT ( 'NONE',  ( 172.3025413328323623, 280.3883983834500668, 13.89755669804951133 ) ) ;
#80412=( BOUNDED_CURVE ( )  B_SPLINE_CURVE ( 2, ( #21396, #11332, #42191, #73126, #88874, #34597, #65495, #50292, #81246 ),
 .UNSPECIFIED., .F., .T. ) 
 B_SPLINE_CURVE_WITH_KNOTS ( ( 3, 2, 2, 2, 3 ),
 ( 0.3185483870967741882, 0.3198924731182795633, 0.3225806451612903136, 0.3252688172043010639, 0.3266129032258064391 ),
 .UNSPECIFIED. ) 
 CURVE ( )  GEOMETRIC_REPRESENTATION_ITEM ( )  RATIONAL_B_SPLINE_CURVE ( ( 0.9330127018922194093, 0.9330127018922194093, 1.000000000000000000, 0.8660254037844387076, 1.000000000000000000, 0.8660254037844387076, 1.000000000000000000, 0.9330127018922194093, 0.9330127018922194093 ) ) 
 REPRESENTATION_ITEM ( '' )  );
#80416=VERTEX_POINT ( 'NONE', #6686 ) ;
#80418=CARTESIAN_POINT ( 'NONE',  ( 200.9436326478643764, 267.7579332533520073, -2.705820022176459005 ) ) ;
#80419=CARTESIAN_POINT ( 'NONE',  ( 152.0594748232699658, 267.2722591642930183, -15.41760623154783616 ) ) ;
#80420=CARTESIAN_POINT ( 'NONE',  ( 148.9517569034208009, 272.6549844970639924, 12.50737104496728236 ) ) ;
#80421=CARTESIAN_POINT ( 'NONE',  ( 162.7561251957091031, 248.7451172484279027, 11.07313294959361194 ) ) ;
#80426=CARTESIAN_POINT ( 'NONE',  ( 3.756859464462060760, 179.6427522451419350, 10.00000000000009415 ) ) ;
#80427=CARTESIAN_POINT ( 'NONE',  ( 189.9154251947152545, 274.3351997317865312, -15.66312253186087311 ) ) ;
#80435=CARTESIAN_POINT ( 'NONE',  ( 2.042590532755589994, 181.1744531367911577, 4.594050593750047540 ) ) ;
#80436=CARTESIAN_POINT ( 'NONE',  ( 103.0428032491157779, 239.4869531367911293, 4.594050593750046652 ) ) ;
#80437=CARTESIAN_POINT ( 'NONE',  ( 202.9547455376043672, 279.1190644220934018, -15.19669173352461478 ) ) ;
#80438=CARTESIAN_POINT ( 'NONE',  ( 176.2580550267919932, 278.7780497695933946, -16.99066290002705060 ) ) ;
#80439=CARTESIAN_POINT ( 'NONE',  ( 185.6624252266433359, 295.2092130351491051, -7.682468391986430056 ) ) ;
#80444=CARTESIAN_POINT ( 'NONE',  ( 163.2163199008810750, 283.1128886150968924, 5.650665759342564876 ) ) ;
#80446=CARTESIAN_POINT ( 'NONE',  ( 207.7086642703471568, 270.8850356419295053, 6.393550561233467100 ) ) ;
#80449=CARTESIAN_POINT ( 'NONE',  ( 166.1787379219248919, 253.5053611955299004, -13.54722061411465361 ) ) ;
#80452=CARTESIAN_POINT ( 'NONE',  ( 175.8597011290570435, 265.2696089897137313, -16.46207262707587304 ) ) ;
#80453=EDGE_CURVE ( 'NONE', #40327, #62030, #43666, .T. ) ;
#80454=CARTESIAN_POINT ( 'NONE',  ( 84.12564760914067108, 225.5024278399160664, 9.188101187500095079 ) ) ;
#80455=CARTESIAN_POINT ( 'NONE',  ( 207.1432938686257046, 271.8642859028066141, -6.405155839440290322 ) ) ;
#80459=CARTESIAN_POINT ( 'NONE',  ( 151.8083138175603892, 267.7072827870618994, 16.72399268212840084 ) ) ;
#80466=CARTESIAN_POINT ( 'NONE',  ( 78.60473566001486745, 222.3149278399160664, 9.188101187500093303 ) ) ;
#80468=AXIS2_PLACEMENT_3D ( 'NONE', #11965, #64664, #97575 ) ;
#80469=CARTESIAN_POINT ( 'NONE',  ( 169.2282880876609852, 288.2011917236219460, -1.104675944282350830 ) ) ;
#80470=DIRECTION ( 'NONE',  ( -0.8660254037844359321, -0.5000000000000051070, -0.000000000000000000 ) ) ;
#80471=CARTESIAN_POINT ( 'NONE',  ( 153.9523474978568913, 263.9937075196493197, 17.96576651779691147 ) ) ;
#80474=CARTESIAN_POINT ( 'NONE',  ( 204.3825393355489268, 268.3164202310341011, -1.666735346079931457 ) ) ;
#80475=CARTESIAN_POINT ( 'NONE',  ( 116.9355544250888101, 244.9865022471903160, 10.00000000000009237 ) ) ;
#80476=CARTESIAN_POINT ( 'NONE',  ( 204.8057697639265768, 275.9129964160624695, -12.68356524114230766 ) ) ;
#80478=VERTEX_POINT ( 'NONE', #76112 ) ;
#80481=CARTESIAN_POINT ( 'NONE',  ( 162.6220573360242270, 248.9773295930640131, 10.49878733418918486 ) ) ;
#80482=DIRECTION ( 'NONE',  ( 0.4999999999999992784, -0.8660254037844390407, 0.000000000000000000 ) ) ;
#80483=CARTESIAN_POINT ( 'NONE',  ( 201.2949053258274148, 281.9939920013367782, -18.04004790210578335 ) ) ;
#80484=ORIENTED_EDGE ( 'NONE', *, *, #45491, .T. ) ;
#80485=CARTESIAN_POINT ( 'NONE',  ( 173.8489725193828690, 250.6783042533247112, 0.4419843250852882877 ) ) ;
#80486=B_SPLINE_CURVE_WITH_KNOTS ( 'NONE', 3,
 ( #30390, #21306, #68876, #53191, #5109, #99311, #75509, #51715, #91227, #99805, #61281, #92245, #29890, #83639, #97823, #44078, #83132, #84146, #14692, #98319, #22795, #28910, #21794, #37475, #75017, #52183, #45575, #84628, #59785, #67900, #76025, #36490, #76503, #68386, #35988, #66893, #90754, #7084, #37968, #53674 ),
 .UNSPECIFIED., .F., .F.,
 ( 4, 2, 2, 2, 2, 2, 2, 2, 2, 2, 2, 2, 2, 2, 2, 2, 2, 2, 2, 4 ),
 ( 0.0008933001899280981805, 0.0009882263429314807734, 0.001083152495934863258, 0.001273004801941664006, 0.001652709413955309953, 0.002412118637982602065, 0.003930937086037185856, 0.004690346310064516348, 0.005070050922078181595, 0.005259903228085013351, 0.005354829381088430096, 0.005449755534091846841, 0.005497218610593546106, 0.005544681687095245372, 0.005639607840098596198, 0.005829460146105390657, 0.006019312452112185116, 0.006209164758118979575, 0.006588869370132517320, 0.006968573982146054197 ),
 .UNSPECIFIED. ) ;
#80488=CARTESIAN_POINT ( 'NONE',  ( 189.5552538188079268, 290.0568273660060186, 14.45120452257448029 ) ) ;
#80489=CARTESIAN_POINT ( 'NONE',  ( 167.4768688352648383, 247.4600260772554350, 3.619672341560728146 ) ) ;
#80490=CARTESIAN_POINT ( 'NONE',  ( 193.9727266537411765, 280.6520757818764196, -17.67061856767345063 ) ) ;
#80491=CARTESIAN_POINT ( 'NONE',  ( 153.3939648708017387, 264.9608545997728015, -16.49556533540763681 ) ) ;
#80497=CARTESIAN_POINT ( 'NONE',  ( 77.96441125478906997, 222.4865022471902876, 10.00000000000009415 ) ) ;
#80498=ORIENTED_EDGE ( 'NONE', *, *, #46941, .F. ) ;
#80499=EDGE_LOOP ( 'NONE', ( #41696, #98052, #8533, #76372 ) ) ;
#80501=CARTESIAN_POINT ( 'NONE',  ( 163.8670932201372352, 246.8208641845333773, 5.912697114930636211 ) ) ;
#80502=CARTESIAN_POINT ( 'NONE',  ( 175.0296968597178306, 264.6864531019056699, -16.70299667166197466 ) ) ;
#80504=CARTESIAN_POINT ( 'NONE',  ( 155.0197698005585494, 262.1448778582381465, 18.42918111182112284 ) ) ;
#80506=CARTESIAN_POINT ( 'NONE',  ( 187.5797606156519635, 291.4431286935292746, -13.96543404383497489 ) ) ;
#80507=CARTESIAN_POINT ( 'NONE',  ( 164.0179581270640199, 246.5595585006577153, 4.626773987940105748 ) ) ;
#80508=CARTESIAN_POINT ( 'NONE',  ( 166.0711008457315359, 265.5911104622053927, 16.59982951413131502 ) ) ;
#80509=CARTESIAN_POINT ( 'NONE',  ( 26.05470188313195123, 197.3967562850347122, -4.648177544792955347E-16 ) ) ;
#80510=CARTESIAN_POINT ( 'NONE',  ( 101.9874215621947258, 235.8149278399160664, 9.188101187500093303 ) ) ;
#80511=ORIENTED_EDGE ( 'NONE', *, *, #85775, .F. ) ;
#80512=CARTESIAN_POINT ( 'NONE',  ( 150.5224706509996793, 271.7355727819179378, 12.90524344130334455 ) ) ;
#80513=CARTESIAN_POINT ( 'NONE',  ( 164.0156888896406144, 276.7977823333153538, -13.62624241490914478 ) ) ;
#80514=AXIS2_PLACEMENT_3D ( 'NONE', #3949, #64249, #25244 ) ;
#80515=VERTEX_POINT ( 'NONE', #29000 ) ;
#80517=CARTESIAN_POINT ( 'NONE',  ( 176.7809350997679871, 292.5586354479191868, -2.749667827406846232 ) ) ;
#80518=B_SPLINE_SURFACE_WITH_KNOTS ( 'NONE', 3, 1, ( 
 ( #25272, #79526 ),
 ( #10587, #87153 ),
 ( #47074, #39450 ),
 ( #10087, #40950 ),
 ( #41460, #93720 ),
 ( #24281, #55157 ),
 ( #9082, #86635 ),
 ( #32871, #86144 ),
 ( #47568, #71897 ),
 ( #94710, #78496 ),
 ( #2493, #39952 ),
 ( #70889, #31370 ),
 ( #1493, #32376 ),
 ( #63275, #481 ),
 ( #56671, #64279 ),
 ( #33376, #87656 ),
 ( #24771, #18188 ),
 ( #71396, #17170 ),
 ( #48070, #79011 ),
 ( #62254, #9598 ),
 ( #40460, #1986 ),
 ( #17685, #48585 ),
 ( #26778, #43460 ),
 ( #65760, #96715 ),
 ( #35366, #12082 ),
 ( #97694, #3498 ),
 ( #34375, #72908 ),
 ( #4473, #26285 ),
 ( #82015, #27777 ),
 ( #11594, #81031 ),
 ( #42453, #27282 ),
 ( #12589, #74401 ),
 ( #81512, #66276 ),
 ( #4986, #58164 ) ),
 .UNSPECIFIED., .T., .F., .F.,
 ( 4, 2, 2, 2, 2, 2, 2, 2, 2, 2, 2, 2, 2, 2, 2, 2, 4 ),
 ( 2, 2 ),
 ( 0.000000000000000000, 0.06250000000000000000, 0.1250000000000000000, 0.1875000000000000000, 0.2500000000000000000, 0.3125000000000000000, 0.3750000000000000000, 0.4375000000000000000, 0.5000000000000000000, 0.5625000000000000000, 0.6250000000000000000, 0.6875000000000000000, 0.7500000000000000000, 0.8125000000000000000, 0.8750000000000000000, 0.9375000000000000000, 1.000000000000000000 ),
 ( 0.000000000000000000, 1.000000000000000000 ),
 .UNSPECIFIED. ) ;
#80522=CARTESIAN_POINT ( 'NONE',  ( 93.48972083544241229, 224.7833772461660260, -9.188101187500095079 ) ) ;
#80523=ORIENTED_EDGE ( 'NONE', *, *, #82612, .T. ) ;
#80526=CARTESIAN_POINT ( 'NONE',  ( 208.3586375946586315, 269.7592488206576604, -1.970210487958146128 ) ) ;
#80528=B_SPLINE_CURVE_WITH_KNOTS ( 'NONE', 3,
 ( #82441, #19110, #20591, #13004 ),
 .UNSPECIFIED., .F., .F.,
 ( 4, 4 ),
 ( 0.002465106009209366237, 0.007832036753820320954 ),
 .UNSPECIFIED. ) ;
#80530=CARTESIAN_POINT ( 'NONE',  ( 154.1661291110820002, 265.4451940853067526, 17.04838890951767283 ) ) ;
#80532=CARTESIAN_POINT ( 'NONE',  ( 133.4351425849996531, 247.8458772461660544, 9.188101187500095079 ) ) ;
#80533=CARTESIAN_POINT ( 'NONE',  ( 63.56442718099752653, 219.0530062829863027, -4.648177544792955347E-16 ) ) ;
#80535=CARTESIAN_POINT ( 'NONE',  ( 179.2808028007571295, 294.7024261520388109, 2.441722445006270892 ) ) ;
#80536=ORIENTED_EDGE ( 'NONE', *, *, #30034, .T. ) ;
#80539=CARTESIAN_POINT ( 'NONE',  ( 160.3800780026849395, 275.5550921561430755, 12.83098206889909854 ) ) ;
#80541=CARTESIAN_POINT ( 'NONE',  ( 190.2764353542772540, 270.7453569036100589, 14.24146154583773871 ) ) ;
#80542=CARTESIAN_POINT ( 'NONE',  ( 175.9516857479530074, 284.1058583014313967, 13.15626907755806840 ) ) ;
#80547=CARTESIAN_POINT ( 'NONE',  ( 148.8636819117637629, 274.0699646975406836, 8.926834414297511344 ) ) ;
#80548=CARTESIAN_POINT ( 'NONE',  ( 161.8873598795597388, 250.2498629158519350, 13.90822209621415873 ) ) ;
#80551=CARTESIAN_POINT ( 'NONE',  ( 167.6084812233214620, 249.9591548999696045, 7.104712731158297601 ) ) ;
#80553=CARTESIAN_POINT ( 'NONE',  ( 117.8941025407614802, 227.3262482093458061, 3.021315404115420679E-15 ) ) ;
#80557=CARTESIAN_POINT ( 'NONE',  ( 184.0314392521297577, 265.7402128651979751, 13.22062658568063576 ) ) ;
#80558=CARTESIAN_POINT ( 'NONE',  ( 167.4011299790239775, 281.5488363183706042, 12.98604958840868662 ) ) ;
#80560=CARTESIAN_POINT ( 'NONE',  ( 152.8134625983922490, 265.9663140294953791, 17.57333028169644251 ) ) ;
#80564=CARTESIAN_POINT ( 'NONE',  ( 205.8859833147073459, 272.4477355138645862, -9.370556367187116820 ) ) ;
#80565=CARTESIAN_POINT ( 'NONE',  ( 161.1747502674735415, 251.4841389699472529, -13.25152330924089839 ) ) ;
#80566=B_SPLINE_CURVE_WITH_KNOTS ( 'NONE', 3,
 ( #7820, #6325, #7312, #52914 ),
 .UNSPECIFIED., .F., .F.,
 ( 4, 4 ),
 ( 0.004697621459670930574, 0.009681921251354225211 ),
 .UNSPECIFIED. ) ;
#80567=CARTESIAN_POINT ( 'NONE',  ( 12.43489537816885537, 187.1744531367911293, 4.594050593750047540 ) ) ;
#80574=CARTESIAN_POINT ( 'NONE',  ( 33.95012722949724093, 202.6589784336661353, -6.496448406907676862E-16 ) ) ;
#80576=CARTESIAN_POINT ( 'NONE',  ( 200.7079229450794173, 283.0106753079404029, 16.90512463913211505 ) ) ;
#80577=CARTESIAN_POINT ( 'NONE',  ( 146.8201187048455267, 276.3470901603510015, 4.112223577763169047 ) ) ;
#80579=CARTESIAN_POINT ( 'NONE',  ( 178.5111704587965846, 291.6673396684018371, 5.951657379714801799 ) ) ;
#80581=CARTESIAN_POINT ( 'NONE',  ( 191.5893301551938350, 298.8045413135534432, -8.323356515452589477 ) ) ;
#80582=AXIS2_PLACEMENT_3D ( 'NONE', #58996, #4847, #28122 ) ;
#80583=CARTESIAN_POINT ( 'NONE',  ( 180.4708198263617760, 279.0196451454304452, -16.21208881180018579 ) ) ;
#80584=FACE_OUTER_BOUND ( 'NONE', #64921, .T. ) ;
#80588=CARTESIAN_POINT ( 'NONE',  ( 86.76900285993090733, 214.2365022471902023, 10.00000000000009592 ) ) ;
#80590=CARTESIAN_POINT ( 'NONE',  ( 161.7978640724907677, 267.9030138832445118, -17.43408704942576293 ) ) ;
#80591=CARTESIAN_POINT ( 'NONE',  ( 47.34706511187656020, 188.9548013555409796, -4.594050593750042211 ) ) ;
#80594=CARTESIAN_POINT ( 'NONE',  ( 146.8516045228164160, 276.2925551239072774, 3.995954059407343273 ) ) ;
#80596=VERTEX_POINT ( 'NONE', #99399 ) ;
#80599=CARTESIAN_POINT ( 'NONE',  ( 164.7694554770609159, 245.2579269087094076, -3.003635650077957742 ) ) ;
#80600=CARTESIAN_POINT ( 'NONE',  ( 147.2111107388217590, 275.6698720921492622, 6.171440615279542463 ) ) ;
#80603=CARTESIAN_POINT ( 'NONE',  ( 149.0203866098534888, 272.5361143586139860, -12.73049804737905255 ) ) ;
#80605=CARTESIAN_POINT ( 'NONE',  ( 175.2507534243562759, 257.3665654692601947, 11.62234696046220428 ) ) ;
#80608=CARTESIAN_POINT ( 'NONE',  ( 171.6446478921618279, 252.6468516832340185, 8.591079895564956104 ) ) ;
#80611=CARTESIAN_POINT ( 'NONE',  ( 179.0976111355799958, 282.8091739615130678, 15.98715785805552159 ) ) ;
#80612=CARTESIAN_POINT ( 'NONE',  ( 190.9501423151522772, 299.9116471280854626, 8.746938802470586083 ) ) ;
#80616=EDGE_LOOP ( 'NONE', ( #90936, #42060, #42281, #41172, #8576, #63384, #6730, #66979, #61153, #92706, #51787, #68048, #97913, #23579, #98695, #69474, #34703, #93035, #66844, #34136, #42945 ) ) ;
#80617=ORIENTED_EDGE ( 'NONE', *, *, #33966, .T. ) ;
#80619=CARTESIAN_POINT ( 'NONE',  ( 207.1158949475991164, 271.9117422260973740, -5.823035679195911918 ) ) ;
#80620=DIRECTION ( 'NONE',  ( 0.4999999999999998890, -0.8660254037844385966, 0.000000000000000000 ) ) ;
#80621=CARTESIAN_POINT ( 'NONE',  ( 149.1004267900891307, 272.3974806997987343, -12.86882154300063341 ) ) ;
#80622=VERTEX_POINT ( 'NONE', #62866 ) ;
#80623=CARTESIAN_POINT ( 'NONE',  ( 152.9251141908703175, 265.7729277985770864, -16.20110192949203309 ) ) ;
#80624=CARTESIAN_POINT ( 'NONE',  ( 159.4285914931787431, 254.5085746851079023, 15.41072477910873673 ) ) ;
#80628=CARTESIAN_POINT ( 'NONE',  ( 205.0716081116550527, 275.4525508911965517, -12.57761053684872188 ) ) ;
#80629=CARTESIAN_POINT ( 'NONE',  ( 114.7887934315897382, 227.8923013555410080, 4.594050593750050204 ) ) ;
#80631=CARTESIAN_POINT ( 'NONE',  ( 70.51298433951257039, 211.5177522451418497, -10.00000000000009592 ) ) ;
#80632=ORIENTED_EDGE ( 'NONE', *, *, #67984, .T. ) ;
#80633=CARTESIAN_POINT ( 'NONE',  ( 208.2175703429120688, 270.0035844679667889, 2.257951022351344150 ) ) ;
#80638=CARTESIAN_POINT ( 'NONE',  ( 69.07880331415105957, 204.5643266524160424, 9.188101187500095079 ) ) ;
#80640=CARTESIAN_POINT ( 'NONE',  ( 190.8860811105559208, 300.0226043892405414, 8.636347304323541252 ) ) ;
#80641=CARTESIAN_POINT ( 'NONE',  ( 198.1444248750829047, 287.4507842102791528, 18.42558436659502519 ) ) ;
#80642=CARTESIAN_POINT ( 'NONE',  ( 172.9572136869028611, 277.5233305075546468, 16.75252092567692230 ) ) ;
#80645=CARTESIAN_POINT ( 'NONE',  ( 189.8238368927809745, 301.8624653444729802, -0.3620111495846872751 ) ) ;
#80647=ORIENTED_EDGE ( 'NONE', *, *, #92560, .T. ) ;
#80648=CARTESIAN_POINT ( 'NONE',  ( 152.3249143222120381, 268.8125044657937792, -15.54600960379902297 ) ) ;
#80650=CARTESIAN_POINT ( 'NONE',  ( 160.4244049798018352, 258.1628759096047361, -17.08294313303711220 ) ) ;
#80651=CARTESIAN_POINT ( 'NONE',  ( 206.5208294064731547, 270.6477873296462349, 2.445619694122634247 ) ) ;
#80652=CARTESIAN_POINT ( 'NONE',  ( 190.4249800432324662, 300.8212548652687133, 3.085047376053959400 ) ) ;
#80654=CARTESIAN_POINT ( 'NONE',  ( 176.9795028420571441, 269.8566753081326510, 16.40411541806681583 ) ) ;
#80655=CARTESIAN_POINT ( 'NONE',  ( 164.4261001824251878, 245.8526357240660900, 1.583002802772015549 ) ) ;
#80656=CARTESIAN_POINT ( 'NONE',  ( 130.2687372006388671, 246.0177522451418497, -10.00000000000009592 ) ) ;
#80657=CARTESIAN_POINT ( 'NONE',  ( 165.7657002015311889, 255.3986422146142274, 13.84715179042893141 ) ) ;
#80658=ORIENTED_EDGE ( 'NONE', *, *, #78282, .T. ) ;
#80659=CYLINDRICAL_SURFACE ( 'NONE', #22132, 17.82106496071139645 ) ;
#80661=CARTESIAN_POINT ( 'NONE',  ( 130.3772506997096343, 236.8923013555409796, 4.594050593750050204 ) ) ;
#80662=ORIENTED_EDGE ( 'NONE', *, *, #24680, .T. ) ;
#80663=CARTESIAN_POINT ( 'NONE',  ( 191.2211340522693774, 299.4422756709672626, -8.405362570633277741 ) ) ;
#80667=CARTESIAN_POINT ( 'NONE',  ( 204.9768178125733016, 275.6167325052707611, 13.98665089523138505 ) ) ;
#80668=CARTESIAN_POINT ( 'NONE',  ( 0.8646476260778407363, 159.7592609112380444, 2.679491924311254714 ) ) ;
#80669=CARTESIAN_POINT ( 'NONE',  ( 178.0531015906397840, 255.3758172151866574, 4.758062337834783051 ) ) ;
#80673=CARTESIAN_POINT ( 'NONE',  ( 158.5045327573800478, 274.9905139280085109, -12.52208736651823884 ) ) ;
#80676=CARTESIAN_POINT ( 'NONE',  ( 164.3883575065421496, 245.9180079563093955, -2.230252308397467687 ) ) ;
#80678=CARTESIAN_POINT ( 'NONE',  ( 136.0332187963529975, 249.3458772461660544, 9.188101187500095079 ) ) ;
#80680=CARTESIAN_POINT ( 'NONE',  ( 29.44348595096431609, 176.2592609112380444, 2.679491924311254714 ) ) ;
#80682=CARTESIAN_POINT ( 'NONE',  ( 58.09093245575348874, 204.3458772461660544, 9.188101187500095079 ) ) ;
#80683=CARTESIAN_POINT ( 'NONE',  ( 205.3943609285979051, 274.8935266139653777, -13.14270440534009943 ) ) ;
#80684=CARTESIAN_POINT ( 'NONE',  ( 174.0516803220720021, 252.0920059681404553, 3.469221368822683615 ) ) ;
#80686=CARTESIAN_POINT ( 'NONE',  ( 149.3883679478359454, 271.8987519849911223, 12.99187507659642371 ) ) ;
#80687=CARTESIAN_POINT ( 'NONE',  ( 155.3185930247096280, 279.9023224415089999, -1.077172130989042520 ) ) ;
#80688=CARTESIAN_POINT ( 'NONE',  ( 171.7676654267511935, 286.7502147520581275, -8.058579322952500235 ) ) ;
#80689=CARTESIAN_POINT ( 'NONE',  ( 154.9903553346911735, 262.1958252075976361, -18.39016733948542637 ) ) ;
#80690=CARTESIAN_POINT ( 'NONE',  ( 157.4489004501168097, 270.9419718275721038, -14.71794672505381385 ) ) ;
#80692=CARTESIAN_POINT ( 'NONE',  ( 134.1658515176688127, 258.2677522451419350, -5.000000000000047962 ) ) ;
#80694=ORIENTED_EDGE ( 'NONE', *, *, #18828, .T. ) ;
#80696=CARTESIAN_POINT ( 'NONE',  ( 190.2476911738421848, 301.1283281946692796, -1.360079143321618611 ) ) ;
#80697=CARTESIAN_POINT ( 'NONE',  ( -2.449395605728673875, 160.2048013555409796, 4.594050593750051981 ) ) ;
#80699=CARTESIAN_POINT ( 'NONE',  ( 39.87759600423577666, 184.6423013555410080, -4.594050593750043987 ) ) ;
#80700=CARTESIAN_POINT ( 'NONE',  ( 178.7014608347196827, 259.1862871959719428, -11.32543599931723222 ) ) ;
#80703=CARTESIAN_POINT ( 'NONE',  ( 205.1300674467857164, 275.3512963525735131, -12.60245643603069610 ) ) ;
#80705=CARTESIAN_POINT ( 'NONE',  ( 146.8195026170398023, 276.3481572557323034, 4.765869558735466249 ) ) ;
#80707=CARTESIAN_POINT ( 'NONE',  ( 171.3866751883526831, 258.3865106268564773, 14.16928307686719712 ) ) ;
#80708=CARTESIAN_POINT ( 'NONE',  ( 48.86234924490155862, 209.0177522451419065, 5.000000000000046185 ) ) ;
#80714=CARTESIAN_POINT ( 'NONE',  ( 161.8918814713609891, 267.1929759636259405, 16.48806508481699140 ) ) ;
#80715=CARTESIAN_POINT ( 'NONE',  ( 44.18942050719595471, 202.9865022471903160, 10.00000000000009237 ) ) ;
#80717=CARTESIAN_POINT ( 'NONE',  ( 164.9959905715102479, 284.7368986600080234, -7.507006057201434324 ) ) ;
#80719=CARTESIAN_POINT ( 'NONE',  ( 2.746756816977958593, 163.2048013555410080, 4.594050593750051981 ) ) ;
#80721=B_SPLINE_CURVE_WITH_KNOTS ( 'NONE', 3,
 ( #65569, #42257, #4266, #28061 ),
 .UNSPECIFIED., .F., .F.,
 ( 4, 4 ),
 ( 0.03005457668816597858, 0.03915685978210869944 ),
 .UNSPECIFIED. ) ;
#80722=CARTESIAN_POINT ( 'NONE',  ( 164.6637257444425302, 246.8187871797005926, 5.850462324949956106 ) ) ;
#80723=CARTESIAN_POINT ( 'NONE',  ( 153.4578721839791342, 264.8501638863745029, 16.85421393845643223 ) ) ;
#80725=CARTESIAN_POINT ( 'NONE',  ( 73.95673202641080479, 225.0530062829863311, -4.648177544792955347E-16 ) ) ;
#80726=CARTESIAN_POINT ( 'NONE',  ( 183.2734392787317290, 278.9810903348750344, 16.96010398477730519 ) ) ;
#80729=CARTESIAN_POINT ( 'NONE',  ( 179.3470654816431136, 262.5477174050944882, -12.85649373009148277 ) ) ;
#80731=CIRCLE ( 'NONE', #53189, 17.82106496071138224 ) ;
#80733=CARTESIAN_POINT ( 'NONE',  ( 168.6642430148957885, 288.2074250805146107, 0.5276533672608759717 ) ) ;
#80735=CARTESIAN_POINT ( 'NONE',  ( 76.44090856289290059, 203.3932355074535963, -2.679491924311248496 ) ) ;
#80739=CARTESIAN_POINT ( 'NONE',  ( 156.6823154307097070, 276.4438179710489862, 10.26594267860235554 ) ) ;
#80740=CARTESIAN_POINT ( 'NONE',  ( 159.2122473525774069, 254.8832937285494609, -16.22689353966294590 ) ) ;
#80745=CARTESIAN_POINT ( 'NONE',  ( 164.2578067403839555, 246.1441285162624126, -2.322300236470859591 ) ) ;
#80751=CARTESIAN_POINT ( 'NONE',  ( 165.3118168859175796, 246.3185293925050701, -4.432402497422931020 ) ) ;
#80752=DIRECTION ( 'NONE',  ( 0.4999999999999992784, -0.8660254037844390407, 0.000000000000000000 ) ) ;
#80756=CARTESIAN_POINT ( 'NONE',  ( 174.4138743697411371, 262.4381095864849840, 14.53967419496388658 ) ) ;
#80762=ORIENTED_EDGE ( 'NONE', *, *, #66773, .T. ) ;
#80763=CARTESIAN_POINT ( 'NONE',  ( 161.7101619467568980, 250.5567787384628389, 13.05644392949610655 ) ) ;
#80764=CARTESIAN_POINT ( 'NONE',  ( 166.3426357552802983, 274.2843506083544298, -15.18163831355469107 ) ) ;
#80765=CARTESIAN_POINT ( 'NONE',  ( -17.42236680055705023, 149.2012482093457777, 0.000000000000000000 ) ) ;
#80766=B_SPLINE_SURFACE_WITH_KNOTS ( 'NONE', 3, 1, ( 
 ( #74520, #5099 ),
 ( #16055, #36980 ),
 ( #92595, #44068 ),
 ( #28898, #75502 ),
 ( #82651, #98309 ),
 ( #13210, #69748 ),
 ( #69251, #28382 ),
 ( #58770, #66883 ),
 ( #89741, #20305 ),
 ( #51178, #97814 ),
 ( #59261, #84990 ),
 ( #90239, #20810 ),
 ( #7969, #359 ),
 ( #67382, #62133 ),
 ( #85508, #51702 ),
 ( #31246, #75008 ),
 ( #82146, #43585 ),
 ( #23141, #54527 ),
 ( #23635, #5588 ),
 ( #54034, #77364 ),
 ( #6087, #36478 ),
 ( #90743, #21300 ),
 ( #46956, #8458 ),
 ( #52175, #83123 ),
 ( #44567, #64156 ),
 ( #56552, #55532 ),
 ( #57042, #95107 ),
 ( #33783, #80406 ),
 ( #64668, #41848 ),
 ( #48463, #26165 ),
 ( #32750, #25671 ),
 ( #71276, #10977 ),
 ( #87025, #95617 ),
 ( #86024, #853 ) ),
 .UNSPECIFIED., .T., .F., .F.,
 ( 4, 2, 2, 2, 2, 2, 2, 2, 2, 2, 2, 2, 2, 2, 2, 2, 4 ),
 ( 2, 2 ),
 ( 0.000000000000000000, 0.06250000000000000000, 0.1250000000000000000, 0.1875000000000000000, 0.2500000000000000000, 0.3125000000000000000, 0.3750000000000000000, 0.4375000000000000000, 0.5000000000000000000, 0.5625000000000000000, 0.6250000000000000000, 0.6875000000000000000, 0.7500000000000000000, 0.8125000000000000000, 0.8750000000000000000, 0.9375000000000000000, 1.000000000000000000 ),
 ( 0.000000000000000000, 1.000000000000000000 ),
 .UNSPECIFIED. ) ;
#80768=CARTESIAN_POINT ( 'NONE',  ( 174.5488994031076970, 277.2909221230937646, -15.64416576916768165 ) ) ;
#80770=ORIENTED_EDGE ( 'NONE', *, *, #30786, .T. ) ;
#80771=EDGE_CURVE ( 'NONE', #46611, #94086, #16830, .T. ) ;
#80772=CARTESIAN_POINT ( 'NONE',  ( 156.8809214077219281, 266.3341492759256539, -16.38455355822726389 ) ) ;
#80776=CARTESIAN_POINT ( 'NONE',  ( 147.1780374576129589, 275.7271566955758999, 6.941191638535834763 ) ) ;
#80777=CARTESIAN_POINT ( 'NONE',  ( 176.8917175299031896, 289.5346434493817469, -10.53293604869262978 ) ) ;
#80779=CARTESIAN_POINT ( 'NONE',  ( 199.7320992005288360, 281.1146086494965175, -17.28530500821910820 ) ) ;
#80780=CARTESIAN_POINT ( 'NONE',  ( 175.6385077117528226, 290.1657555888949673, 6.156910366948349811 ) ) ;
#80781=CARTESIAN_POINT ( 'NONE',  ( 197.3013163403698798, 288.9110910286968306, -18.25968461953811328 ) ) ;
#80782=ORIENTED_EDGE ( 'NONE', *, *, #68344, .T. ) ;
#80785=CARTESIAN_POINT ( 'NONE',  ( 206.3106310032756596, 273.3065002911688453, 10.17860425536756175 ) ) ;
#80787=CARTESIAN_POINT ( 'NONE',  ( 205.8379285891498682, 274.1252448892948905, 10.44730901608240181 ) ) ;
#80788=CARTESIAN_POINT ( 'NONE',  ( 159.9628729326222754, 253.5831720864507588, 15.75051413866357386 ) ) ;
#80789=ORIENTED_EDGE ( 'NONE', *, *, #99796, .T. ) ;
#80790=CARTESIAN_POINT ( 'NONE',  ( 146.7539121514467695, 276.4617632746314371, -2.866763085982500403 ) ) ;
#80792=CARTESIAN_POINT ( 'NONE',  ( 171.5798264516812424, 259.4877759030353559, -13.89750514209113064 ) ) ;
#80793=CARTESIAN_POINT ( 'NONE',  ( 164.3996301846870267, 247.3020492865104529, 7.248807534621905191 ) ) ;
#80795=CARTESIAN_POINT ( 'NONE',  ( 160.6390625115447222, 252.4119773802086968, -15.11156539429256362 ) ) ;
#80796=CARTESIAN_POINT ( 'NONE',  ( 91.89298649898879034, 233.8615022471903160, 5.000000000000046185 ) ) ;
#80797=ORIENTED_EDGE ( 'NONE', *, *, #92994, .F. ) ;
#80798=CARTESIAN_POINT ( 'NONE',  ( 182.2991478702006134, 275.2734891516705034, -17.80812521087705846 ) ) ;
#80799=EDGE_CURVE ( 'NONE', #941, #65003, #9492, .T. ) ;
#80804=CARTESIAN_POINT ( 'NONE',  ( 29.01593374150824189, 180.8927522451417929, -10.00000000000009059 ) ) ;
#80805=CARTESIAN_POINT ( 'NONE',  ( 103.0163473728362504, 218.0327760586659451, 1.948934522072302763E-15 ) ) ;
#80806=CARTESIAN_POINT ( 'NONE',  ( 180.7869751407568231, 294.0814949767770941, -2.848415450199388577 ) ) ;
#80808=ADVANCED_FACE ( 'NONE', ( #37444 ), #67869, .T. ) ;
#80810=CARTESIAN_POINT ( 'NONE',  ( 208.1864700626310025, 270.0574517335433598, 2.990990977286084096 ) ) ;
#80812=CARTESIAN_POINT ( 'NONE',  ( 17.98295739510416524, 187.3149278399160949, -9.188101187500095079 ) ) ;
#80813=EDGE_CURVE ( 'NONE', #80879, #44657, #20445, .T. ) ;
#80815=ORIENTED_EDGE ( 'NONE', *, *, #47859, .F. ) ;
#80818=ADVANCED_FACE ( 'NONE', ( #77476 ), #32093, .F. ) ;
#80819=CARTESIAN_POINT ( 'NONE',  ( 185.1518460011666889, 259.9031676633314873, -5.660721190095883593 ) ) ;
#80822=CARTESIAN_POINT ( 'NONE',  ( 205.2564848266901834, 271.9733254596621350, -9.597888780111448526 ) ) ;
#80824=CARTESIAN_POINT ( 'NONE',  ( 182.2583020200309818, 284.4576732326586921, 14.88072139987983711 ) ) ;
#80825=CARTESIAN_POINT ( 'NONE',  ( 106.0921946783233096, 225.3927522451418213, 10.00000000000009948 ) ) ;
#80826=CARTESIAN_POINT ( 'NONE',  ( 45.42531092540608029, 197.0333772461660828, 9.188101187500095079 ) ) ;
#80827=CARTESIAN_POINT ( 'NONE',  ( 82.20432729060244981, 228.2677522451419350, -5.000000000000047962 ) ) ;
#80829=CARTESIAN_POINT ( 'NONE',  ( 150.0694502760089222, 271.4680435213315945, -12.17790201236558545 ) ) ;
#80830=CARTESIAN_POINT ( 'NONE',  ( 158.7081735734057872, 282.4546237173937016, -1.655763827236318209 ) ) ;
#80832=CARTESIAN_POINT ( 'NONE',  ( -0.2032289886040369309, 164.5643266524160140, -9.188101187500093303 ) ) ;
#80834=CARTESIAN_POINT ( 'NONE',  ( 150.6438662863770332, 269.7241650738195631, -14.92510732909997628 ) ) ;
#80836=CARTESIAN_POINT ( 'NONE',  ( 147.2658550951450422, 275.5750520855697800, -5.215660180131691526 ) ) ;
#80838=CARTESIAN_POINT ( 'NONE',  ( 204.0890941988925817, 276.4630862285632702, 13.35479316431303687 ) ) ;
#80839=CARTESIAN_POINT ( 'NONE',  ( 147.1447476476323004, 275.7848163378367872, 0.6373001129109078233 ) ) ;
#80840=CARTESIAN_POINT ( 'NONE',  ( 164.9779129355220562, 244.8968679994381148, -1.771286574179712803 ) ) ;
#80842=CARTESIAN_POINT ( 'NONE',  ( -0.8439004895948557516, 176.9865022471903444, -10.00000000000009415 ) ) ;
#80844=CARTESIAN_POINT ( 'NONE',  ( 113.3268549190559753, 245.4244531367911293, -4.594050593750046652 ) ) ;
#80848=CARTESIAN_POINT ( 'NONE',  ( 184.5194340083631346, 296.1660737835977102, -7.201245168507500516 ) ) ;
#80849=CARTESIAN_POINT ( 'NONE',  ( -22.42236680055709641, 157.8615022471902591, 0.000000000000000000 ) ) ;
#80852=CARTESIAN_POINT ( 'NONE',  ( 151.0036289208911171, 269.1010379121764799, 14.24595189915657478 ) ) ;
#80853=CARTESIAN_POINT ( 'NONE',  ( 149.0164813726494799, 272.5428784278667536, -11.67305721329070423 ) ) ;
#80855=CARTESIAN_POINT ( 'NONE',  ( 173.1997439627015467, 289.7296588321038939, -1.111478199152324375 ) ) ;
#80857=ORIENTED_EDGE ( 'NONE', *, *, #25618, .T. ) ;
#80858=CARTESIAN_POINT ( 'NONE',  ( 189.1697036996914960, 265.4656734670753053, 11.91601115033013514 ) ) ;
#80859=CARTESIAN_POINT ( 'NONE',  ( 165.4340772170561991, 269.7433133579526157, -16.28799140846306415 ) ) ;
#80862=CARTESIAN_POINT ( 'NONE',  ( 199.9868610850537607, 272.4588406731110126, 12.49652601812552533 ) ) ;
#80865=CARTESIAN_POINT ( 'NONE',  ( 148.0808017092188607, 274.9439814809830409, 5.964600266013551533 ) ) ;
#80866=ORIENTED_EDGE ( 'NONE', *, *, #66320, .F. ) ;
#80871=CARTESIAN_POINT ( 'NONE',  ( 164.4183836189802435, 279.4556777148490028, 11.95241060903501484 ) ) ;
#80872=CARTESIAN_POINT ( 'NONE',  ( 147.6884207308302450, 274.8431469350302336, -8.096293592099874203 ) ) ;
#80873=CARTESIAN_POINT ( 'NONE',  ( 156.0226403810962097, 261.9271281158086140, -16.96797176191799394 ) ) ;
#80878=CARTESIAN_POINT ( 'NONE',  ( 204.9314961322898228, 273.1004059617595203, -9.763055590748432877 ) ) ;
#80879=VERTEX_POINT ( 'NONE', #50059 ) ;
#80884=CARTESIAN_POINT ( 'NONE',  ( 185.6713631041849055, 258.9584525764907426, -6.747383155299178092 ) ) ;
#80886=EDGE_CURVE ( 'NONE', #79277, #54166, #38526, .T. ) ;
#80887=ORIENTED_EDGE ( 'NONE', *, *, #4156, .T. ) ;
#80888=DIRECTION ( 'NONE',  ( -0.8660254037844387076, -0.4999999999999998890, -0.000000000000000000 ) ) ;
#80892=EDGE_LOOP ( 'NONE', ( #43778, #89148, #12973, #66162 ) ) ;
#80895=CARTESIAN_POINT ( 'NONE',  ( 202.8874463667715133, 279.2356300052831557, -15.29930322226033468 ) ) ;
#80896=ORIENTED_EDGE ( 'NONE', *, *, #32054, .T. ) ;
#80898=CARTESIAN_POINT ( 'NONE',  ( 147.1439969174920464, 275.7861166405825770, -6.562009323313376719 ) ) ;
#80899=CARTESIAN_POINT ( 'NONE',  ( 161.8890841478012135, 277.2149579922602243, -12.83564633500961882 ) ) ;
#80900=CARTESIAN_POINT ( 'NONE',  ( 147.3379027498079381, 275.4502618871274535, -3.695260257281167249 ) ) ;
#80901=CARTESIAN_POINT ( 'NONE',  ( 200.6583719735737645, 283.0965001081523269, -17.35266956530146132 ) ) ;
#80902=CARTESIAN_POINT ( 'NONE',  ( 205.2564848266901834, 271.9733254596621350, -9.597888780111448526 ) ) ;
#80904=CARTESIAN_POINT ( 'NONE',  ( 135.7624123097878623, 255.3149278399160949, 9.188101187500093303 ) ) ;
#80907=ORIENTED_EDGE ( 'NONE', *, *, #17792, .T. ) ;
#80912=CARTESIAN_POINT ( 'NONE',  ( -22.42236680055709641, 157.8615022471902591, 0.000000000000000000 ) ) ;
#80914=CARTESIAN_POINT ( 'NONE',  ( 170.8882927430364020, 288.0602046512401557, -5.525210371943358290 ) ) ;
#80915=CARTESIAN_POINT ( 'NONE',  ( 157.3345317626142048, 280.0779076120791160, -6.962135762735354838 ) ) ;
#80916=DIRECTION ( 'NONE',  ( -0.8660254037844387076, -0.4999999999999998890, -0.000000000000000000 ) ) ;
#80917=CARTESIAN_POINT ( 'NONE',  ( 171.3649617487770911, 251.0102673366500596, 7.372720983288576946 ) ) ;
#80918=CARTESIAN_POINT ( 'NONE',  ( 168.2134749413384327, 253.2945090417912866, 11.62816938842056125 ) ) ;
#80919=CARTESIAN_POINT ( 'NONE',  ( 195.0180713635390930, 292.4506560729497551, 15.11837988040635672 ) ) ;
#80925=CARTESIAN_POINT ( 'NONE',  ( 163.6306258414269621, 278.1771990602612163, 13.60634061194307520 ) ) ;
#80928=CARTESIAN_POINT ( 'NONE',  ( 201.0972691433344437, 267.4835988171084864, -2.316786570161582404 ) ) ;
#80930=CARTESIAN_POINT ( 'NONE',  ( 190.4163244163388242, 300.8362468508201459, 4.691083071570470331 ) ) ;
#80931=CARTESIAN_POINT ( 'NONE',  ( 163.3854574543125580, 247.6550818016845597, 10.82482370245618775 ) ) ;
#80932=CARTESIAN_POINT ( 'NONE',  ( 173.2337249902883798, 270.7486416191997023, 17.82094672905207133 ) ) ;
#80934=CARTESIAN_POINT ( 'NONE',  ( 203.3277680582037590, 270.0362633623805664, 6.010087534169584522 ) ) ;
#80943=CARTESIAN_POINT ( 'NONE',  ( 6.102605256642664067, 165.1423013555410080, -4.594050593750043987 ) ) ;
#80944=CARTESIAN_POINT ( 'NONE',  ( 112.2989703957094605, 226.4548013555409796, -4.594050593750042211 ) ) ;
#80945=CARTESIAN_POINT ( 'NONE',  ( 155.0619429961492983, 262.0718317407570339, -17.08853361476647592 ) ) ;
#80947=CARTESIAN_POINT ( 'NONE',  ( 186.7302140808759816, 295.8439017956092698, -7.678039062033136020 ) ) ;
#80951=B_SPLINE_CURVE_WITH_KNOTS ( 'NONE', 3,
 ( #93562, #54501, #99648, #77845 ),
 .UNSPECIFIED., .F., .F.,
 ( 4, 4 ),
 ( 0.009075473815016553078, 0.01512968392534322706 ),
 .UNSPECIFIED. ) ;
#80952=CARTESIAN_POINT ( 'NONE',  ( 162.9598982752141296, 282.9239241067374451, 5.638055053146040052 ) ) ;
#80953=CARTESIAN_POINT ( 'NONE',  ( 194.6943296385021824, 293.4265244509877562, -16.10917128197217352 ) ) ;
#80954=CARTESIAN_POINT ( 'NONE',  ( 181.8289026455834971, 291.5239361404854321, 9.451350534620820198 ) ) ;
#80957=CARTESIAN_POINT ( 'NONE',  ( 145.9293632524074553, 248.3927522451417929, -10.00000000000009237 ) ) ;
#80959=CARTESIAN_POINT ( 'NONE',  ( 172.5583743051683996, 263.7812420529770066, -15.44831042087596984 ) ) ;
#80960=EDGE_CURVE ( 'NONE', #58917, #53525, #64259, .T. ) ;
#80961=CARTESIAN_POINT ( 'NONE',  ( 76.60222546164588664, 215.0333772461660544, 9.188101187500095079 ) ) ;
#80962=CARTESIAN_POINT ( 'NONE',  ( 207.8844858873204657, 270.5805036682629066, -6.251308616122969397 ) ) ;
#80964=CARTESIAN_POINT ( 'NONE',  ( 163.3102869483862492, 258.1249230757383657, 15.76774596908120074 ) ) ;
#80965=CARTESIAN_POINT ( 'NONE',  ( 198.0502297282944824, 286.6154393603603694, -17.27411237049796355 ) ) ;
#80966=CARTESIAN_POINT ( 'NONE',  ( 151.1451503555562113, 268.8559155969762742, -15.81507177720227553 ) ) ;
#80967=CARTESIAN_POINT ( 'NONE',  ( 14.14916430987532969, 185.6427522451419350, 10.00000000000009415 ) ) ;
#80973=CARTESIAN_POINT ( 'NONE',  ( 77.57650404090335883, 215.5958772461660544, -9.188101187500095079 ) ) ;
#80974=CARTESIAN_POINT ( 'NONE',  ( 172.8631597400377018, 289.5366941478733338, -1.054817492037981141 ) ) ;
#80976=CARTESIAN_POINT ( 'NONE',  ( 191.3415583986349873, 288.7194663682888631, -16.11500851257928346 ) ) ;
#80977=B_SPLINE_CURVE_WITH_KNOTS ( 'NONE', 3,
 ( #29850, #53145, #84101, #52634, #46021, #8059 ),
 .UNSPECIFIED., .F., .F.,
 ( 4, 2, 4 ),
 ( 0.01929493135631588779, 0.02382575134946158385, 0.02835657134260728338 ),
 .UNSPECIFIED. ) ;
#80979=CARTESIAN_POINT ( 'NONE',  ( 193.6219581044664722, 288.4232849465348067, 16.10596218273157021 ) ) ;
#80981=CARTESIAN_POINT ( 'NONE',  ( 127.8330407560430473, 244.6115022471902591, 10.00000000000009592 ) ) ;
#80982=CARTESIAN_POINT ( 'NONE',  ( 21.31191609055711211, 173.1115022471901739, -5.000000000000041744 ) ) ;
#80984=VERTEX_POINT ( 'NONE', #2478 ) ;
#80985=CARTESIAN_POINT ( 'NONE',  ( 168.0032770494077283, 248.2778096739003502, -1.874811026054818308 ) ) ;
#80986=VERTEX_POINT ( 'NONE', #19681 ) ;
#80987=CARTESIAN_POINT ( 'NONE',  ( 163.1008115941903895, 248.1481028935802442, 11.25332017433677834 ) ) ;
#80988=CARTESIAN_POINT ( 'NONE',  ( 207.4369976298412155, 270.8980557713372832, -0.6764754127990474375 ) ) ;
#80992=ORIENTED_EDGE ( 'NONE', *, *, #78555, .F. ) ;
#80993=EDGE_CURVE ( 'NONE', #53916, #64894, #55386, .T. ) ;
#80994=CARTESIAN_POINT ( 'NONE',  ( 189.6374659733051260, 290.1052907212381911, 14.45593141723346342 ) ) ;
#80995=CARTESIAN_POINT ( 'NONE',  ( 205.7538280185135307, 274.2709113505826508, 12.26218269827389307 ) ) ;
#80996=CARTESIAN_POINT ( 'NONE',  ( 146.7502831681854332, 255.5333772461660260, 9.188101187500095079 ) ) ;
#80997=CARTESIAN_POINT ( 'NONE',  ( 193.3021154463603750, 295.8379101667960072, -12.81235253903514959 ) ) ;
#80999=CARTESIAN_POINT ( 'NONE',  ( 112.6979501180548766, 224.3262482093458061, 3.021315404115420679E-15 ) ) ;
#81002=CARTESIAN_POINT ( 'NONE',  ( 164.0586374769217741, 275.4376342846808257, 15.48247449835999312 ) ) ;
#81003=EDGE_CURVE ( 'NONE', #61940, #51575, #73540, .T. ) ;
#81006=VERTEX_POINT ( 'NONE', #75394 ) ;
#81010=( BOUNDED_CURVE ( )  B_SPLINE_CURVE ( 2, ( #83116, #98805, #62250, #71893, #40946, #62758, #32867, #18183, #86631 ),
 .UNSPECIFIED., .F., .T. ) 
 B_SPLINE_CURVE_WITH_KNOTS ( ( 3, 2, 2, 2, 3 ),
 ( 0.5685483870967742437, 0.5698924731182796188, 0.5725806451612903691, 0.5752688172043011194, 0.5766129032258064946 ),
 .UNSPECIFIED. ) 
 CURVE ( )  GEOMETRIC_REPRESENTATION_ITEM ( )  RATIONAL_B_SPLINE_CURVE ( ( 0.9330127018922194093, 0.9330127018922194093, 1.000000000000000000, 0.8660254037844387076, 1.000000000000000000, 0.8660254037844387076, 1.000000000000000000, 0.9330127018922194093, 0.9330127018922194093 ) ) 
 REPRESENTATION_ITEM ( '' )  );
#81011=CARTESIAN_POINT ( 'NONE',  ( 164.2297246530060875, 246.1927681183832988, 5.803160395959773510 ) ) ;
#81012=CARTESIAN_POINT ( 'NONE',  ( 148.1829914015846157, 273.9865254053503349, -9.304102644963160529 ) ) ;
#81014=CARTESIAN_POINT ( 'NONE',  ( 201.3053657339852691, 274.7141922394133076, -14.27644254562359372 ) ) ;
#81019=CARTESIAN_POINT ( 'NONE',  ( 156.9763224152064822, 271.9908631200777904, -15.29896765642516776 ) ) ;
#81020=CARTESIAN_POINT ( 'NONE',  ( 181.9878657410701237, 256.9700144498582972, 5.080659748315781599 ) ) ;
#81021=CARTESIAN_POINT ( 'NONE',  ( 101.9066655502961964, 220.4548013555409511, -4.594050593750042211 ) ) ;
#81023=CARTESIAN_POINT ( 'NONE',  ( 149.8275266058892896, 271.5268038298542592, 11.74484678564449780 ) ) ;
#81024=CARTESIAN_POINT ( 'NONE',  ( 114.6802799325189284, 237.0177522451418497, -10.00000000000009592 ) ) ;
#81026=EDGE_LOOP ( 'NONE', ( #7606, #11461, #27408, #54789 ) ) ;
#81027=DIRECTION ( 'NONE',  ( -0.8660254037844387076, -0.4999999999999998890, -0.000000000000000000 ) ) ;
#81028=CARTESIAN_POINT ( 'NONE',  ( 195.5855337169582242, 285.9052202549062258, -17.72130995818495336 ) ) ;
#81030=CARTESIAN_POINT ( 'NONE',  ( 159.9531724557437826, 253.5999738052623229, -15.71074128491364874 ) ) ;
#81031=CARTESIAN_POINT ( 'NONE',  ( 163.2109138634145609, 247.9574001692554077, 11.18215713980082171 ) ) ;
#81032=CARTESIAN_POINT ( 'NONE',  ( 89.94416901687610277, 231.9244531367911009, -4.594050593750046652 ) ) ;
#81033=ORIENTED_EDGE ( 'NONE', *, *, #64163, .T. ) ;
#81036=ADVANCED_FACE ( 'NONE', ( #52561 ), #83517, .T. ) ;
#81037=CARTESIAN_POINT ( 'NONE',  ( 163.4084407101100851, 247.6152736349200438, -10.68829614238923931 ) ) ;
#81039=CARTESIAN_POINT ( 'NONE',  ( 194.6615252313652888, 266.3370749013627687, -7.769244936135564217 ) ) ;
#81040=CARTESIAN_POINT ( 'NONE',  ( 13.18034623014981044, 189.9637435831424739, 2.679491924311251605 ) ) ;
#81042=CARTESIAN_POINT ( 'NONE',  ( 136.3847812948166336, 258.7369531367911009, -4.594050593750048428 ) ) ;
#81046=ORIENTED_EDGE ( 'NONE', *, *, #51635, .F. ) ;
#81047=CARTESIAN_POINT ( 'NONE',  ( 157.2014865449050660, 258.3660336093062142, 16.87758714513496017 ) ) ;
#81051=CARTESIAN_POINT ( 'NONE',  ( 178.4805428241997163, 285.3359289386864930, 13.12455424698817907 ) ) ;
#81054=LINE ( 'NONE', #13601, #9090 ) ;
#81055=CARTESIAN_POINT ( 'NONE',  ( 161.4726291907278721, 250.9681975403669867, 14.52346149734912117 ) ) ;
#81057=CARTESIAN_POINT ( 'NONE',  ( 206.8313602288537538, 272.4045708154811791, -9.607337080360906612 ) ) ;
#81059=CARTESIAN_POINT ( 'NONE',  ( 163.4139553296302267, 247.6057220337265505, -10.31482883765270842 ) ) ;
#81060=CARTESIAN_POINT ( 'NONE',  ( -22.42236680055709641, 157.8615022471902591, 0.000000000000000000 ) ) ;
#81061=CARTESIAN_POINT ( 'NONE',  ( 192.4380962356868281, 295.3344353383980661, 13.50754959408193656 ) ) ;
#81064=CARTESIAN_POINT ( 'NONE',  ( 182.0281585185019537, 264.2490478462352712, 13.61349246500957477 ) ) ;
#81065=CARTESIAN_POINT ( 'NONE',  ( 170.6241101913971079, 249.1812156342870708, -3.705643032328568953 ) ) ;
#81069=CARTESIAN_POINT ( 'NONE',  ( 160.8610131809898860, 273.3839308686426648, -15.49656964745045329 ) ) ;
#81071=CARTESIAN_POINT ( 'NONE',  ( 23.17945691357580529, 178.0643266524160424, -9.188101187500093303 ) ) ;
#81075=CARTESIAN_POINT ( 'NONE',  ( 200.6117230619925635, 269.0360104864248001, 9.242361455687714056 ) ) ;
#81076=CARTESIAN_POINT ( 'NONE',  ( 208.2777459429579210, 269.8993572713111462, 3.129643751043610589 ) ) ;
#81078=CARTESIAN_POINT ( 'NONE',  ( 37.57712925149209582, 186.3768266524160140, 9.188101187500096856 ) ) ;
#81079=CARTESIAN_POINT ( 'NONE',  ( 161.6673510627899191, 250.6309293646106653, 13.01175935005004192 ) ) ;
#81080=CARTESIAN_POINT ( 'NONE',  ( 147.3154503175461514, 275.4891506405583073, 3.671329888160011823 ) ) ;
#81082=CARTESIAN_POINT ( 'NONE',  ( 199.5198787286983872, 267.5021379205973631, -6.627115275362054803 ) ) ;
#81083=CARTESIAN_POINT ( 'NONE',  ( 178.6383753932449281, 293.9108930832058491, 2.721302933230898002 ) ) ;
#81084=CARTESIAN_POINT ( 'NONE',  ( 179.0373480721268038, 278.3843228141229815, -16.99121447468398216 ) ) ;
#81090=CARTESIAN_POINT ( 'NONE',  ( 74.64464720694869015, 227.2365022471903444, 2.944929066748280225E-16 ) ) ;
#81092=CARTESIAN_POINT ( 'NONE',  ( 179.7389585068036979, 283.2694176073634935, 16.15404047216739514 ) ) ;
#81094=CARTESIAN_POINT ( 'NONE',  ( 38.60536087060361154, 193.0958772461660544, -9.188101187500095079 ) ) ;
#81095=ORIENTED_EDGE ( 'NONE', *, *, #89498, .F. ) ;
#81097=CARTESIAN_POINT ( 'NONE',  ( 147.3154503175461514, 275.4891506405583073, 3.671329888160011823 ) ) ;
#81100=CARTESIAN_POINT ( 'NONE',  ( 171.0568157338405229, 286.4360392956926944, 7.470701674589402153 ) ) ;
#81101=CARTESIAN_POINT ( 'NONE',  ( 206.9408877595175511, 272.2148635675444552, 6.707071080545934372 ) ) ;
#81102=CYLINDRICAL_SURFACE ( 'NONE', #47665, 17.82106496071139645 ) ;
#81104=CARTESIAN_POINT ( 'NONE',  ( 189.1716578938339524, 265.4390178063673034, 10.58420148173503783 ) ) ;
#81106=CARTESIAN_POINT ( 'NONE',  ( 173.6854900591675346, 256.8832444864495983, 11.28848571671958467 ) ) ;
#81109=CARTESIAN_POINT ( 'NONE',  ( -12.82842912691854309, 163.4005647456539521, -9.594050593750095501 ) ) ;
#81110=CARTESIAN_POINT ( 'NONE',  ( 174.7340118358694951, 255.1271270684982824, 8.232752107466076552 ) ) ;
#81112=VERTEX_POINT ( 'NONE', #22176 ) ;
#81113=CARTESIAN_POINT ( 'NONE',  ( 178.6460525542210007, 282.3916330005288842, 15.69558721233099341 ) ) ;
#81114=EDGE_CURVE ( 'NONE', #76868, #27771, #4631, .T. ) ;
#81115=CARTESIAN_POINT ( 'NONE',  ( 191.5451565139252068, 298.8810523045859213, 7.782291334092181323 ) ) ;
#81116=DIRECTION ( 'NONE',  ( -0.8660254037844387076, -0.4999999999999998890, -0.000000000000000000 ) ) ;
#81117=EDGE_CURVE ( 'NONE', #34750, #100037, #21500, .T. ) ;
#81120=CARTESIAN_POINT ( 'NONE',  ( 207.7836085030675690, 270.7552284231231852, -5.468305433308493058 ) ) ;
#81122=CARTESIAN_POINT ( 'NONE',  ( 148.9194629746633893, 272.7109192224475009, -12.27648025871169679 ) ) ;
#81123=ORIENTED_EDGE ( 'NONE', *, *, #38899, .T. ) ;
#81126=CARTESIAN_POINT ( 'NONE',  ( 198.0858447170796524, 287.5522480202560018, 18.44384186289807559 ) ) ;
#81129=CARTESIAN_POINT ( 'NONE',  ( 157.8429099974857195, 257.2550556002704525, -17.85752049034686095 ) ) ;
#81130=EDGE_CURVE ( 'NONE', #67131, #89517, #23804, .T. ) ;
#81131=CARTESIAN_POINT ( 'NONE',  ( 111.1617914095948692, 244.1744531367911293, 4.594050593750047540 ) ) ;
#81132=CARTESIAN_POINT ( 'NONE',  ( 117.8941025407614802, 227.3262482093458061, 3.021315404115420679E-15 ) ) ;
#81134=CARTESIAN_POINT ( 'NONE',  ( 201.5248099939757651, 280.9651160740240812, 16.27600578877254733 ) ) ;
#81135=EDGE_LOOP ( 'NONE', ( #98149, #58943, #47520, #6584, #1730 ) ) ;
#81137=CARTESIAN_POINT ( 'NONE',  ( 159.9880386575927957, 253.5395837721924863, 15.85893018594752846 ) ) ;
#81139=CARTESIAN_POINT ( 'NONE',  ( 70.64795371486285092, 223.8464784336661353, 1.353441290958777525E-15 ) ) ;
#81140=CARTESIAN_POINT ( 'NONE',  ( 172.2305375516802144, 289.0099938022871129, 7.323606124671270479 ) ) ;
#81141=CARTESIAN_POINT ( 'NONE',  ( 151.4384131719918685, 268.3479694989391078, 14.98299707687648841 ) ) ;
#81142=CARTESIAN_POINT ( 'NONE',  ( 196.9080397933726942, 269.7016881256661804, 12.39056067425276630 ) ) ;
#81143=CARTESIAN_POINT ( 'NONE',  ( 171.8895305906860358, 276.7362633202488382, 16.33455527369717686 ) ) ;
#81144=ORIENTED_EDGE ( 'NONE', *, *, #39328, .T. ) ;
#81146=CARTESIAN_POINT ( 'NONE',  ( 155.6535436963908694, 261.0471492701456668, -17.87366571046205976 ) ) ;
#81147=VERTEX_POINT ( 'NONE', #27685 ) ;
#81148=CARTESIAN_POINT ( 'NONE',  ( 195.1612419366965128, 292.6178086278368369, 15.12635622767516352 ) ) ;
#81150=CARTESIAN_POINT ( 'NONE',  ( 163.4196212193596978, 260.1667154333714507, -16.20002750279465431 ) ) ;
#81151=CARTESIAN_POINT ( 'NONE',  ( 79.03898477424621660, 204.8932355074535963, -2.679491924311248496 ) ) ;
#81154=CARTESIAN_POINT ( 'NONE',  ( 152.1095568868906298, 269.8383682962399348, -14.43354909618994419 ) ) ;
#81156=CARTESIAN_POINT ( 'NONE',  ( 167.5740236991643712, 256.4854641017122958, 13.67099374824216973 ) ) ;
#81158=CARTESIAN_POINT ( 'NONE',  ( 207.6471633721571379, 270.9915583223058206, 2.196965492132801678 ) ) ;
#81159=CARTESIAN_POINT ( 'NONE',  ( 128.5637496887121927, 245.0333772461660544, 9.188101187500095079 ) ) ;
#81161=CARTESIAN_POINT ( 'NONE',  ( 191.3413020738616410, 299.2341385521244774, -8.295023558158421295 ) ) ;
#81165=CARTESIAN_POINT ( 'NONE',  ( 204.7610021263893429, 275.9905362388115577, 13.36619428527026976 ) ) ;
#81171=CARTESIAN_POINT ( 'NONE',  ( 165.8535204196604695, 247.9869754089129970, -5.534111939223802068 ) ) ;
#81172=CARTESIAN_POINT ( 'NONE',  ( 206.3559632282955647, 273.2279825742143089, -11.28941701449801904 ) ) ;
#81178=CARTESIAN_POINT ( 'NONE',  ( 204.6470611188870521, 276.1878878528713130, -13.02652554726987866 ) ) ;
#81179=CARTESIAN_POINT ( 'NONE',  ( 174.4045371546278886, 252.1404095536752834, 3.497397249627876459 ) ) ;
#81181=CARTESIAN_POINT ( 'NONE',  ( 149.4491471355718772, 271.7934793437897270, 11.43912701239353780 ) ) ;
#81182=CARTESIAN_POINT ( 'NONE',  ( 153.7448948813404570, 278.8794451890384494, -1.595968573229418874 ) ) ;
#81183=CARTESIAN_POINT ( 'NONE',  ( 172.5430877045778288, 287.8837544777731523, -8.388212238523923503 ) ) ;
#81185=CARTESIAN_POINT ( 'NONE',  ( 193.6779244371759603, 288.5814230932801365, 16.06948571431362893 ) ) ;
#81186=CARTESIAN_POINT ( 'NONE',  ( 127.7428297729341580, 257.8927522451419918, 2.944929066748280225E-16 ) ) ;
#81188=ORIENTED_EDGE ( 'NONE', *, *, #94341, .T. ) ;
#81190=CARTESIAN_POINT ( 'NONE',  ( 196.0034224882197975, 291.1591091234520263, 17.53794140922627776 ) ) ;
#81191=CARTESIAN_POINT ( 'NONE',  ( 189.8763472015711216, 301.7715148217271803, -0.1184663095182975079 ) ) ;
#81192=CARTESIAN_POINT ( 'NONE',  ( -9.107486540969064848, 174.7369531367911293, -4.594050593750048428 ) ) ;
#81193=CARTESIAN_POINT ( 'NONE',  ( 32.16412338207434374, 195.5024278399160949, 9.188101187500095079 ) ) ;
#81196=CARTESIAN_POINT ( 'NONE',  ( 189.6855683962509147, 268.4063607128787794, 14.53388648619876378 ) ) ;
#81197=CARTESIAN_POINT ( 'NONE',  ( 204.8057697639265768, 275.9129964160624695, -12.68356524114230766 ) ) ;
#81198=CARTESIAN_POINT ( 'NONE',  ( 192.5978738290548051, 292.4115197693782875, -14.32134620733571495 ) ) ;
#81199=CARTESIAN_POINT ( 'NONE',  ( 146.7879906441258129, 276.4027375938661635, 4.347255311287614887 ) ) ;
#81202=CARTESIAN_POINT ( 'NONE',  ( 71.81202244518927102, 202.2677522451417929, -5.000000000000041744 ) ) ;
#81205=CARTESIAN_POINT ( 'NONE',  ( 174.3103273403459070, 251.6799977031412539, 4.969826440491621256 ) ) ;
#81206=CARTESIAN_POINT ( 'NONE',  ( 39.49844957003027446, 193.6115022471902591, 10.00000000000009592 ) ) ;
#81207=CARTESIAN_POINT ( 'NONE',  ( 199.1165320752825494, 285.7670451491295580, 0.000000000000000000 ) ) ;
#81208=CARTESIAN_POINT ( 'NONE',  ( 163.2835940097493790, 247.8315144631017404, 11.08416305054517359 ) ) ;
#81209=CARTESIAN_POINT ( 'NONE',  ( 7.266240119036749157, 168.8768266524159856, -9.188101187500091527 ) ) ;
#81210=CARTESIAN_POINT ( 'NONE',  ( 166.6849293799611758, 285.4799480694566682, 4.101407758763460976 ) ) ;
#81211=CARTESIAN_POINT ( 'NONE',  ( 164.2873127220971128, 252.5483806906220252, 13.40952729246955677 ) ) ;
#81212=CARTESIAN_POINT ( 'NONE',  ( 153.4242699508872647, 264.9083646613370320, 16.62000820703435267 ) ) ;
#81215=CARTESIAN_POINT ( 'NONE',  ( 179.6991264753519317, 277.0039691112309015, 16.29786852896214100 ) ) ;
#81217=CARTESIAN_POINT ( 'NONE',  ( 149.1429535397850827, 272.3238222086447990, -12.91457852089092384 ) ) ;
#81218=CARTESIAN_POINT ( 'NONE',  ( 177.2089533061429734, 260.4205850299505300, -13.82133967672870511 ) ) ;
#81223=CARTESIAN_POINT ( 'NONE',  ( 154.8596847415876994, 262.4221533139083817, 17.65401077761399762 ) ) ;
#81224=EDGE_LOOP ( 'NONE', ( #42239, #77846, #49616, #83983 ) ) ;
#81225=CARTESIAN_POINT ( 'NONE',  ( 156.8182864210080538, 276.5001846890115758, 10.28252859274006248 ) ) ;
#81226=CARTESIAN_POINT ( 'NONE',  ( 206.6268150440956504, 272.7588534679261443, -10.76664753678610609 ) ) ;
#81229=CARTESIAN_POINT ( 'NONE',  ( 153.3703256797887775, 265.0017988796566897, 16.44314709207578318 ) ) ;
#81230=CARTESIAN_POINT ( 'NONE',  ( 206.9408877595175511, 272.2148635675444552, 6.707071080545934372 ) ) ;
#81235=ORIENTED_EDGE ( 'NONE', *, *, #31033, .F. ) ;
#81237=CARTESIAN_POINT ( 'NONE',  ( 204.6780326111993986, 276.1342436545999703, 14.85609018352459287 ) ) ;
#81238=CARTESIAN_POINT ( 'NONE',  ( 192.7259387352017939, 296.8358775046606297, 11.24705370801146209 ) ) ;
#81239=ORIENTED_EDGE ( 'NONE', *, *, #29360, .T. ) ;
#81241=CARTESIAN_POINT ( 'NONE',  ( 177.7988474914041035, 263.9390705747547941, 14.66591618048462209 ) ) ;
#81246=CARTESIAN_POINT ( 'NONE',  ( 34.98558885611105751, 202.5530062829863027, -4.648177544792955347E-16 ) ) ;
#81247=ORIENTED_EDGE ( 'NONE', *, *, #34866, .T. ) ;
#81249=CARTESIAN_POINT ( 'NONE',  ( 168.1388140323589937, 275.3731239741051127, -15.27220439302207211 ) ) ;
#81250=CYLINDRICAL_SURFACE ( 'NONE', #41286, 10.00000000000010658 ) ;
#81252=CARTESIAN_POINT ( 'NONE',  ( 174.6227982317619478, 277.3332904828302503, -15.64528549635424071 ) ) ;
#81253=CARTESIAN_POINT ( 'NONE',  ( 202.9689790241539242, 279.0944113002206564, 15.85114608332523289 ) ) ;
#81255=CARTESIAN_POINT ( 'NONE',  ( 159.7740173431952542, 268.4189001149085811, -16.40494236134203376 ) ) ;
#81258=ORIENTED_EDGE ( 'NONE', *, *, #20214, .T. ) ;
#81259=CARTESIAN_POINT ( 'NONE',  ( 158.8346295283509733, 260.0021606417885778, 17.18667582297067042 ) ) ;
#81261=CARTESIAN_POINT ( 'NONE',  ( 147.8921479301010038, 274.4902810750095341, 6.237421762629938193 ) ) ;
#81264=CARTESIAN_POINT ( 'NONE',  ( 152.7153488183568300, 266.1362520814392951, 17.33540622643059237 ) ) ;
#81265=CARTESIAN_POINT ( 'NONE',  ( 29.53915742650918830, 197.8615022471903160, 5.000000000000046185 ) ) ;
#81266=CARTESIAN_POINT ( 'NONE',  ( 196.3956310503436953, 264.1850728776087180, 4.154333235580330630 ) ) ;
#81267=ORIENTED_EDGE ( 'NONE', *, *, #9042, .T. ) ;
#81270=CARTESIAN_POINT ( 'NONE',  ( 150.6217811227348875, 274.8790014839793230, -9.901424828548254453 ) ) ;
#81272=CARTESIAN_POINT ( 'NONE',  ( 164.6869624841032191, 245.4008089637804346, 1.435659848726088317 ) ) ;
#81274=EDGE_LOOP ( 'NONE', ( #197, #63448, #14576, #26377 ) ) ;
#81275=ORIENTED_EDGE ( 'NONE', *, *, #40418, .F. ) ;
#81276=CARTESIAN_POINT ( 'NONE',  ( 186.2313097042465699, 276.3922763046537057, 16.55972454784547310 ) ) ;
#81277=CARTESIAN_POINT ( 'NONE',  ( 171.5203192281751967, 259.6685845591893553, -14.08447829917957073 ) ) ;
#81280=CARTESIAN_POINT ( 'NONE',  ( 199.4224781028189000, 285.2371310850626287, -17.75806834606089168 ) ) ;
#81281=CARTESIAN_POINT ( 'NONE',  ( 148.3108110047529919, 273.7651353584593608, -10.43768245379277104 ) ) ;
#81282=ORIENTED_EDGE ( 'NONE', *, *, #74431, .F. ) ;
#81283=CARTESIAN_POINT ( 'NONE',  ( 167.3067612288924124, 252.8339271406035493, -12.30798038737281175 ) ) ;
#81287=CYLINDRICAL_SURFACE ( 'NONE', #16009, 10.00000000000010658 ) ;
#81288=CARTESIAN_POINT ( 'NONE',  ( 35.00594278435062989, 181.0177522451417929, 5.000000000000051514 ) ) ;
#81290=CARTESIAN_POINT ( 'NONE',  ( 107.4543804714665072, 232.8458772461660544, 9.188101187500095079 ) ) ;
#81291=CARTESIAN_POINT ( 'NONE',  ( 6.176825452568912134, 162.8262482093457777, 3.021315404115420679E-15 ) ) ;
#81292=CARTESIAN_POINT ( 'NONE',  ( 167.8847406357959358, 281.9191505512837352, -10.89945309425706021 ) ) ;
#81293=CARTESIAN_POINT ( 'NONE',  ( -22.42236680055709641, 157.8615022471902591, 0.000000000000000000 ) ) ;
#81294=CARTESIAN_POINT ( 'NONE',  ( 208.0366075493969902, 270.3170212206142082, 1.570844709476715284 ) ) ;
#81295=CARTESIAN_POINT ( 'NONE',  ( 21.98867198337220685, 177.3768266524160140, 9.188101187500098632 ) ) ;
#81301=CARTESIAN_POINT ( 'NONE',  ( 185.1558638909941408, 259.8922561614027700, -5.643363702243105351 ) ) ;
#81303=( BOUNDED_CURVE ( )  B_SPLINE_CURVE ( 2, ( #23985, #87864, #94429, #40172, #41678, #62991, #54883, #93935, #64498 ),
 .UNSPECIFIED., .F., .T. ) 
 B_SPLINE_CURVE_WITH_KNOTS ( ( 3, 2, 2, 2, 3 ),
 ( 0.9153225806451612545, 0.9166666666666666297, 0.9193548387096773800, 0.9220430107526881303, 0.9233870967741935054 ),
 .UNSPECIFIED. ) 
 CURVE ( )  GEOMETRIC_REPRESENTATION_ITEM ( )  RATIONAL_B_SPLINE_CURVE ( ( 0.9330127018922194093, 0.9330127018922194093, 1.000000000000000000, 0.8660254037844387076, 1.000000000000000000, 0.8660254037844387076, 1.000000000000000000, 0.9330127018922194093, 0.9330127018922194093 ) ) 
 REPRESENTATION_ITEM ( '' )  );
#81304=CARTESIAN_POINT ( 'NONE',  ( 203.6925490392534925, 269.5270927311577793, 7.084861529579629114 ) ) ;
#81305=CARTESIAN_POINT ( 'NONE',  ( 147.3154503175461514, 275.4891506405583073, 3.671329888160011823 ) ) ;
#81306=DIRECTION ( 'NONE',  ( 0.4999999999999992784, -0.8660254037844390407, 0.000000000000000000 ) ) ;
#81307=CARTESIAN_POINT ( 'NONE',  ( 161.5083988044524119, 250.9062427520286178, -14.53522982831775856 ) ) ;
#81308=CARTESIAN_POINT ( 'NONE',  ( 183.7164175811012115, 284.9638087483388063, 15.03005855678972047 ) ) ;
#81310=CARTESIAN_POINT ( 'NONE',  ( 36.87296296726972855, 204.3464784336661637, 1.353441290958777525E-15 ) ) ;
#81311=CARTESIAN_POINT ( 'NONE',  ( 99.09182266439904652, 228.0177522451418781, -10.00000000000009592 ) ) ;
#81315=CARTESIAN_POINT ( 'NONE',  ( 180.3229202803501323, 260.0783157291148200, -10.34379025228027338 ) ) ;
#81316=CARTESIAN_POINT ( 'NONE',  ( 0.4998960083233069396, 183.3464784336661353, 1.353441290958777327E-15 ) ) ;
#81318=CARTESIAN_POINT ( 'NONE',  ( 199.1526122334580862, 285.7045524820243259, -17.32174362185583050 ) ) ;
#81320=CARTESIAN_POINT ( 'NONE',  ( 192.4212750754384160, 297.3635704425909125, -12.73704185013552248 ) ) ;
#81322=CARTESIAN_POINT ( 'NONE',  ( 203.7037101912997059, 276.1473598535747556, 13.26654772282832973 ) ) ;
#81324=CARTESIAN_POINT ( 'NONE',  ( 147.6207754342248961, 274.9603120256437592, 8.795690793376332195 ) ) ;
#81325=EDGE_CURVE ( 'NONE', #59759, #79145, #51636, .T. ) ;
#81327=B_SPLINE_CURVE_WITH_KNOTS ( 'NONE', 3,
 ( #14884, #45289, #32079, #70078, #77715, #23986, #85338 ),
 .UNSPECIFIED., .F., .F.,
 ( 4, 3, 4 ),
 ( 0.0009084163136891124438, 0.001498048609634153143, 0.001783312035702471800 ),
 .UNSPECIFIED. ) ;
#81328=CARTESIAN_POINT ( 'NONE',  ( -11.09186776771074001, 177.7365022471903444, 2.944929066748280225E-16 ) ) ;
#81329=CARTESIAN_POINT ( 'NONE',  ( 199.9642529041454395, 269.6475505498956977, -10.52657023967446470 ) ) ;
#81330=CARTESIAN_POINT ( 'NONE',  ( 118.5230073417626073, 248.4244531367911293, -4.594050593750046652 ) ) ;
#81334=CARTESIAN_POINT ( 'NONE',  ( 157.4656258344471098, 257.9085309395441641, 18.30485740784190796 ) ) ;
#81338=CARTESIAN_POINT ( 'NONE',  ( 195.3619008497734058, 263.0282990088426800, -0.5392206530015204446 ) ) ;
#81339=CARTESIAN_POINT ( 'NONE',  ( 163.4778819063952540, 247.4949979548153465, 8.784095219806332011 ) ) ;
#81340=CARTESIAN_POINT ( 'NONE',  ( 192.9343601389454932, 263.4285982009681106, -7.324792422444850182 ) ) ;
#81341=CARTESIAN_POINT ( 'NONE',  ( 172.8644463536523972, 268.0606821319897790, -16.30213415373016517 ) ) ;
#81343=VERTEX_POINT ( 'NONE', #3877 ) ;
#81347=ADVANCED_FACE ( 'NONE', ( #34760 ), #59929, .T. ) ;
#81348=EDGE_CURVE ( 'NONE', #5719, #90285, #22617, .T. ) ;
#81349=B_SPLINE_SURFACE_WITH_KNOTS ( 'NONE', 3, 1, ( 
 ( #38195, #69111 ),
 ( #7823, #83870 ),
 ( #75744, #45799 ),
 ( #77219, #100038 ),
 ( #85361, #31103 ),
 ( #39188, #15397 ),
 ( #52917, #14433 ),
 ( #76720, #99539 ),
 ( #6328, #91973 ),
 ( #53413, #93456 ),
 ( #7314, #31597 ),
 ( #84855, #30626 ),
 ( #37219, #61002 ),
 ( #46290, #61511 ),
 ( #46814, #69614 ),
 ( #712, #91458 ),
 ( #23004, #62490 ),
 ( #45314, #76249 ),
 ( #92459, #53897 ),
 ( #30120, #6822 ),
 ( #219, #22520 ),
 ( #61990, #92943 ),
 ( #23497, #37706 ),
 ( #84361, #77738 ),
 ( #54387, #24009 ),
 ( #15909, #8323 ),
 ( #70102, #54907 ),
 ( #68119, #99044 ),
 ( #29627, #60501 ),
 ( #63014, #16412 ),
 ( #70610, #1223 ),
 ( #78234, #32103 ),
 ( #24512, #8814 ),
 ( #93960, #85887 ) ),
 .UNSPECIFIED., .T., .F., .F.,
 ( 4, 2, 2, 2, 2, 2, 2, 2, 2, 2, 2, 2, 2, 2, 2, 2, 4 ),
 ( 2, 2 ),
 ( 0.000000000000000000, 0.06250000000000000000, 0.1250000000000000000, 0.1875000000000000000, 0.2500000000000000000, 0.3125000000000000000, 0.3750000000000000000, 0.4375000000000000000, 0.5000000000000000000, 0.5625000000000000000, 0.6250000000000000000, 0.6875000000000000000, 0.7500000000000000000, 0.8125000000000000000, 0.8750000000000000000, 0.9375000000000000000, 1.000000000000000000 ),
 ( 0.000000000000000000, 1.000000000000000000 ),
 .UNSPECIFIED. ) ;
#81351=CARTESIAN_POINT ( 'NONE',  ( 200.1567857842741773, 272.1619586071154799, 12.85406770604015492 ) ) ;
#81352=CARTESIAN_POINT ( 'NONE',  ( 185.8939863203812308, 296.6946888721068945, 4.888489570743712598 ) ) ;
#81354=CARTESIAN_POINT ( 'NONE',  ( 147.4771206202524354, 275.6046823160672830, -0.001107820683494442279 ) ) ;
#81356=DIRECTION ( 'NONE',  ( -0.8660254037844387076, -0.4999999999999998890, -0.000000000000000000 ) ) ;
#81358=CARTESIAN_POINT ( 'NONE',  ( 173.8858844611855829, 272.4353729945644318, -16.46099354089476563 ) ) ;
#81359=ORIENTED_EDGE ( 'NONE', *, *, #90152, .F. ) ;
#81361=CARTESIAN_POINT ( 'NONE',  ( 194.8067605455144076, 293.2317884077015151, -16.00245909155922774 ) ) ;
#81363=B_SPLINE_CURVE_WITH_KNOTS ( 'NONE', 3,
 ( #15816, #32012, #24430, #32534, #87310, #9229, #10238, #85270, #71048, #63922, #85795, #94367, #630, #48227, #94861, #77648, #79174, #25421, #48744, #46721 ),
 .UNSPECIFIED., .F., .F.,
 ( 4, 2, 2, 2, 2, 2, 2, 2, 2, 4 ),
 ( 0.003680063676163143182, 0.003801481233049108874, 0.003922898789935074133, 0.004044316346821039826, 0.004165733903707005518, 0.004408569017478878790, 0.004651404131250752062, 0.005137074358794497739, 0.005622744586338243415, 0.007565425496513157599 ),
 .UNSPECIFIED. ) ;
#81367=CARTESIAN_POINT ( 'NONE',  ( 185.0905594003060060, 291.6090161883107044, 11.96356110993400002 ) ) ;
#81371=CARTESIAN_POINT ( 'NONE',  ( 84.39645409570583467, 219.5333772461660544, 9.188101187500095079 ) ) ;
#81374=CARTESIAN_POINT ( 'NONE',  ( 185.5992489932250464, 259.0872182414688609, -6.824291053258027873 ) ) ;
#81375=EDGE_CURVE ( 'NONE', #14896, #47944, #52882, .T. ) ;
#81376=ORIENTED_EDGE ( 'NONE', *, *, #52749, .F. ) ;
#81380=ORIENTED_EDGE ( 'NONE', *, *, #29047, .T. ) ;
#81382=CARTESIAN_POINT ( 'NONE',  ( 202.7973612924478743, 279.3916619310153919, -15.54732529288344089 ) ) ;
#81383=EDGE_LOOP ( 'NONE', ( #97644, #81, #59132, #40507 ) ) ;
#81385=CARTESIAN_POINT ( 'NONE',  ( 161.9514198990980560, 255.2405834741430226, -15.02415447469453724 ) ) ;
#81386=CARTESIAN_POINT ( 'NONE',  ( 162.0346552423833941, 277.4622592605515479, -12.99750001863938031 ) ) ;
#81387=CARTESIAN_POINT ( 'NONE',  ( 201.1060504099706350, 282.3210983108598384, -18.18000168485860257 ) ) ;
#81390=CARTESIAN_POINT ( 'NONE',  ( 140.4447960187037552, 242.7048013555409796, 4.594050593750051981 ) ) ;
#81399=CARTESIAN_POINT ( 'NONE',  ( -17.42236680055705023, 149.2012482093457777, 0.000000000000000000 ) ) ;
#81404=CARTESIAN_POINT ( 'NONE',  ( 185.1126663572763675, 273.1539052423648286, -16.71538631548864018 ) ) ;
#81407=CARTESIAN_POINT ( 'NONE',  ( 194.3193926313213638, 293.6800862088419422, -14.28503170336555428 ) ) ;
#81408=CARTESIAN_POINT ( 'NONE',  ( 200.9494940653346191, 267.7474625779211124, -2.675924154422841816 ) ) ;
#81411=CARTESIAN_POINT ( 'NONE',  ( 164.6805913154744587, 274.3217421407699703, 14.82948928037302672 ) ) ;
#81416=CARTESIAN_POINT ( 'NONE',  ( 200.0126145424869719, 267.7195842788145228, 6.153478395924335764 ) ) ;
#81419=CARTESIAN_POINT ( 'NONE',  ( 191.9824032073976241, 287.6194387751458521, -17.05427143794285882 ) ) ;
#81421=EDGE_CURVE ( 'NONE', #89705, #1456, #23590, .T. ) ;
#81423=CARTESIAN_POINT ( 'NONE',  ( 152.9489295551198893, 265.7316783776963121, 17.71675637597311237 ) ) ;
#81425=CARTESIAN_POINT ( 'NONE',  ( 50.39593590098449738, 193.2365022471902307, 10.00000000000009948 ) ) ;
#81426=CARTESIAN_POINT ( 'NONE',  ( 8.267668766103758671, 166.3923013555410080, 4.594050593750050204 ) ) ;
#81427=CARTESIAN_POINT ( 'NONE',  ( 114.4640339051705666, 227.7048013555410080, 4.594050593750051981 ) ) ;
#81428=CARTESIAN_POINT ( 'NONE',  ( 155.0453531195792038, 262.1005662498678817, -18.46987289964740953 ) ) ;
#81430=CARTESIAN_POINT ( 'NONE',  ( 186.1869626216079894, 296.9195626386382969, -7.441086137094660380 ) ) ;
#81433=AXIS2_PLACEMENT_3D ( 'NONE', #29239, #83465, #44419 ) ;
#81434=CARTESIAN_POINT ( 'NONE',  ( -27.42236680055714260, 166.5217562850347406, 1.224646799147364892E-15 ) ) ;
#81435=CARTESIAN_POINT ( 'NONE',  ( 163.9287928004966375, 283.7425982196886594, 5.719485170213416403 ) ) ;
#81436=CARTESIAN_POINT ( 'NONE',  ( 148.4042165687623083, 273.6033521758856750, -8.709765892313745539 ) ) ;
#81437=ADVANCED_FACE ( 'NONE', ( #1318 ), #16733, .F. ) ;
#81440=FACE_OUTER_BOUND ( 'NONE', #23148, .T. ) ;
#81441=EDGE_CURVE ( 'NONE', #11960, #24507, #28664, .T. ) ;
#81442=CARTESIAN_POINT ( 'NONE',  ( 172.8108118737807786, 263.0936288908736174, -15.55104684167783091 ) ) ;
#81443=CARTESIAN_POINT ( 'NONE',  ( 80.33713356334875755, 211.0643266524159856, -9.188101187500093303 ) ) ;
#81444=CARTESIAN_POINT ( 'NONE',  ( 207.8575108622103755, 270.6272257822888037, -6.381720258959569847 ) ) ;
#81447=CARTESIAN_POINT ( 'NONE',  ( 196.3519702320103590, 290.5554067223432639, 17.39042812051341969 ) ) ;
#81449=CARTESIAN_POINT ( 'NONE',  ( 151.1230807375396807, 268.8941412966845519, -14.26613110909109849 ) ) ;
#81452=CARTESIAN_POINT ( 'NONE',  ( 193.1169444172380167, 296.1586357973259283, -13.13373377033755318 ) ) ;
#81456=EDGE_CURVE ( 'NONE', #35189, #89364, #22756, .T. ) ;
#81457=CARTESIAN_POINT ( 'NONE',  ( 173.0357146759456271, 289.9031501978675465, -0.5316909439790075131 ) ) ;
#81459=CARTESIAN_POINT ( 'NONE',  ( 188.0020763875417629, 286.0549491211741042, -16.57088730622232120 ) ) ;
#81463=CARTESIAN_POINT ( 'NONE',  ( 143.9266795097038596, 247.2365022471902023, 10.00000000000009592 ) ) ;
#81465=EDGE_CURVE ( 'NONE', #49648, #46249, #54124, .T. ) ;
#81467=EDGE_LOOP ( 'NONE', ( #11247, #1076, #88607 ) ) ;
#81468=CARTESIAN_POINT ( 'NONE',  ( 165.7517492418863014, 246.5407772836408355, -1.235758156293855103 ) ) ;
#81470=CARTESIAN_POINT ( 'NONE',  ( 162.6264071486809542, 248.9697954965390920, 10.36322805486644683 ) ) ;
#81472=VERTEX_POINT ( 'NONE', #50400 ) ;
#81475=VERTEX_POINT ( 'NONE', #13418 ) ;
#81476=CARTESIAN_POINT ( 'NONE',  ( 191.5566566914955331, 291.3450863069615480, 14.65428652378087371 ) ) ;
#81479=CARTESIAN_POINT ( 'NONE',  ( 145.4512450625087467, 254.7833772461660544, -9.188101187500095079 ) ) ;
#81481=CARTESIAN_POINT ( 'NONE',  ( 202.3879523842396111, 275.1512786724707098, -14.15337613030473918 ) ) ;
#81483=CARTESIAN_POINT ( 'NONE',  ( 43.68655075043449898, 184.4824982072973967, 3.021315404115420679E-15 ) ) ;
#81484=ADVANCED_FACE ( 'NONE', ( #82847 ), #11924, .T. ) ;
#81488=DIRECTION ( 'NONE',  ( 0.8660254037844395958, 0.4999999999999985567, 0.000000000000000000 ) ) ;
#81489=CARTESIAN_POINT ( 'NONE',  ( 44.69460199273685674, 206.6115022471903160, -5.000000000000047962 ) ) ;
#81491=ORIENTED_EDGE ( 'NONE', *, *, #21677, .T. ) ;
#81493=CARTESIAN_POINT ( 'NONE',  ( 163.7136804588959649, 247.0865828815331042, 6.783386239354816105 ) ) ;
#81498=CARTESIAN_POINT ( 'NONE',  ( 147.7840666256145425, 276.6774833857293174, 0.9737628777943441172 ) ) ;
#81500=CARTESIAN_POINT ( 'NONE',  ( 164.0303808347895256, 246.5380417397093140, 5.465094127736859875 ) ) ;
#81501=CARTESIAN_POINT ( 'NONE',  ( 168.8523083975146903, 266.9327454831334876, 16.71699773333943284 ) ) ;
#81505=CARTESIAN_POINT ( 'NONE',  ( 190.8443993347725325, 300.0947993426467519, 8.522468760355437212 ) ) ;
#81506=CARTESIAN_POINT ( 'NONE',  ( 163.3750637014402400, 276.5743216800318010, -13.80359379715451773 ) ) ;
#81509=CARTESIAN_POINT ( 'NONE',  ( 177.8737369365807410, 292.6277481362276944, -2.671055768360467209 ) ) ;
#81510=CARTESIAN_POINT ( 'NONE',  ( 196.2255671652529259, 290.7743432561995860, 16.01325193769018185 ) ) ;
#81512=CARTESIAN_POINT ( 'NONE',  ( 208.1864700626310025, 270.0574517335433598, 2.990990977286084096 ) ) ;
#81515=ORIENTED_EDGE ( 'NONE', *, *, #42742, .F. ) ;
#81516=CARTESIAN_POINT ( 'NONE',  ( 207.6067494229581314, 271.0615573356529353, -1.924113146155245868 ) ) ;
#81519=CARTESIAN_POINT ( 'NONE',  ( 194.6851553498462124, 266.4313783899017380, -7.994026154862396538 ) ) ;
#81522=CARTESIAN_POINT ( 'NONE',  ( 140.4447960187037552, 242.7048013555409796, 4.594050593750051981 ) ) ;
#81523=DIRECTION ( 'NONE',  ( -0.8660254037844387076, -0.4999999999999998890, -0.000000000000000000 ) ) ;
#81524=CARTESIAN_POINT ( 'NONE',  ( -10.89340361622470610, 174.5177522451419350, 5.000000000000046185 ) ) ;
#81525=CARTESIAN_POINT ( 'NONE',  ( 180.9226702965857783, 295.6987777469875027, 2.116087624927042388 ) ) ;
#81526=ORIENTED_EDGE ( 'NONE', *, *, #91560, .T. ) ;
#81527=CARTESIAN_POINT ( 'NONE',  ( 156.8993174718108605, 258.8894057963813680, 16.93179113901802069 ) ) ;
#81530=CARTESIAN_POINT ( 'NONE',  ( 189.2738920610548803, 270.0414595828373763, 14.42171763143272756 ) ) ;
#81531=CARTESIAN_POINT ( 'NONE',  ( 42.60170726692454224, 188.7365022471902023, 10.00000000000009948 ) ) ;
#81534=DIRECTION ( 'NONE',  ( 0.4999999999999998890, -0.8660254037844385966, 0.000000000000000000 ) ) ;
#81536=CYLINDRICAL_SURFACE ( 'NONE', #18804, 17.82106496071139645 ) ;
#81537=CARTESIAN_POINT ( 'NONE',  ( 160.0081047537594543, 253.5048282741223602, -16.11956848123596941 ) ) ;
#81539=CARTESIAN_POINT ( 'NONE',  ( 208.2874212803407090, 269.8825990953837390, -1.143705256421198690 ) ) ;
#81541=EDGE_CURVE ( 'NONE', #58155, #32950, #39590, .T. ) ;
#81542=VECTOR ( 'NONE', #28452, 1000.000000000000000 ) ;
#81545=CARTESIAN_POINT ( 'NONE',  ( 185.4417336918466219, 266.3141122328166830, 13.06621773694827837 ) ) ;
#81555=CARTESIAN_POINT ( 'NONE',  ( 11.65032017781297036, 177.5333772461660544, 9.188101187500095079 ) ) ;
#81556=DIRECTION ( 'NONE',  ( -0.8660254037844387076, -0.4999999999999998890, -0.000000000000000000 ) ) ;
#81560=CARTESIAN_POINT ( 'NONE',  ( 28.53675269070083331, 198.8297689869269220, -2.679491924311252493 ) ) ;
#81562=CARTESIAN_POINT ( 'NONE',  ( 38.44315465527655107, 186.8768266524159856, -9.188101187500093303 ) ) ;
#81564=CARTESIAN_POINT ( 'NONE',  ( 190.6218339396177441, 300.4802939150614520, -4.178005820806754755 ) ) ;
#81566=CARTESIAN_POINT ( 'NONE',  ( 202.9297445357156278, 270.0237240353077937, -6.443924261151921407 ) ) ;
#81567=CARTESIAN_POINT ( 'NONE',  ( 147.1447476476323004, 275.7848163378367872, 0.6373001129109078233 ) ) ;
#81571=CARTESIAN_POINT ( 'NONE',  ( 166.8565011125344597, 257.6213196747827965, -15.76983133553760297 ) ) ;
#81573=CARTESIAN_POINT ( 'NONE',  ( 200.2362722391634975, 283.4274695507068600, 16.82377321601456899 ) ) ;
#81575=CARTESIAN_POINT ( 'NONE',  ( 80.63465624979117763, 207.3615022471901739, 5.000000000000051514 ) ) ;
#81576=( BOUNDED_CURVE ( )  B_SPLINE_CURVE ( 2, ( #70253, #62641, #32756, #10472, #9474, #2383, #93598, #63660, #40343 ),
 .UNSPECIFIED., .F., .T. ) 
 B_SPLINE_CURVE_WITH_KNOTS ( ( 3, 2, 2, 2, 3 ),
 ( 0.1250000000000000000, 0.1263440860215053752, 0.1290322580645161255, 0.1317204301075268758, 0.1330645161290322509 ),
 .UNSPECIFIED. ) 
 CURVE ( )  GEOMETRIC_REPRESENTATION_ITEM ( )  RATIONAL_B_SPLINE_CURVE ( ( 0.9330127018922194093, 0.9330127018922194093, 1.000000000000000000, 0.8660254037844387076, 1.000000000000000000, 0.8660254037844387076, 1.000000000000000000, 0.9330127018922194093, 0.9330127018922194093 ) ) 
 REPRESENTATION_ITEM ( '' )  );
#81577=CARTESIAN_POINT ( 'NONE',  ( 183.5953950971229744, 289.9057545191589043, -13.74357891376704544 ) ) ;
#81581=CARTESIAN_POINT ( 'NONE',  ( 44.82974491242176640, 202.8149278399160664, 9.188101187500093303 ) ) ;
#81584=CARTESIAN_POINT ( 'NONE',  ( 190.3791419447713906, 300.9006487807255326, -5.688668718458480988 ) ) ;
#81587=CARTESIAN_POINT ( 'NONE',  ( 170.8851693353173005, 287.3571709677545982, 8.586156227924460538 ) ) ;
#81588=CARTESIAN_POINT ( 'NONE',  ( 206.8986117509267899, 272.2880877623646825, 6.975890063856878598 ) ) ;
#81593=CARTESIAN_POINT ( 'NONE',  ( 171.6154833087297789, 255.2606305366970503, 12.53362356821959978 ) ) ;
#81597=CARTESIAN_POINT ( 'NONE',  ( 174.8904491429100574, 255.1896265538727846, 8.186123047353046189 ) ) ;
#81600=ORIENTED_EDGE ( 'NONE', *, *, #96875, .F. ) ;
#81601=CARTESIAN_POINT ( 'NONE',  ( 180.2906877376209138, 282.9895530604892997, 15.04284179662483645 ) ) ;
#81602=CARTESIAN_POINT ( 'NONE',  ( 191.3375250863502970, 299.2406804863936145, 8.828791580707859410 ) ) ;
#81605=CARTESIAN_POINT ( 'NONE',  ( 161.1232569692349443, 251.5733279787459367, -14.02750397520710557 ) ) ;
#81607=CARTESIAN_POINT ( 'NONE',  ( 196.3286486926436680, 290.5958008134369948, -16.58330917766970458 ) ) ;
#81614=CARTESIAN_POINT ( 'NONE',  ( 107.5083335113205578, 239.0024278399160949, 9.188101187500095079 ) ) ;
#81618=CARTESIAN_POINT ( 'NONE',  ( 208.0287371622045782, 270.3306531311065442, 3.558879245883286746 ) ) ;
#81623=CARTESIAN_POINT ( 'NONE',  ( 65.93911412966745900, 215.0024278399160664, 9.188101187500095079 ) ) ;
#81624=ORIENTED_EDGE ( 'NONE', *, *, #52578, .F. ) ;
#81626=CARTESIAN_POINT ( 'NONE',  ( 119.6057994200909036, 229.8615022471901739, 5.000000000000051514 ) ) ;
#81627=CARTESIAN_POINT ( 'NONE',  ( 154.8838596469624349, 262.3802811495310152, 18.07457254681616021 ) ) ;
#81628=CARTESIAN_POINT ( 'NONE',  ( 172.2631232552246843, 276.7629437217855752, 15.87404649013240210 ) ) ;
#81632=B_SPLINE_CURVE_WITH_KNOTS ( 'NONE', 3,
 ( #46642, #7648, #77567, #53249, #62840, #84205, #92297, #9154, #16249, #40030, #22848, #68939, #70970, #77041, #84690, #8155, #99865, #31935, #1572, #15735, #53731, #46127, #92782, #69446, #8651, #63352, #22353, #70447, #76560, #554, #30449, #23336, #47139, #63, #30946, #54224, #85190, #39029, #78064, #69937, #31436, #93282, #23838, #54731, #26857, #56239, #11669, #72484, #25346, #10163 ),
 .UNSPECIFIED., .F., .F.,
 ( 4, 2, 2, 2, 2, 2, 2, 2, 2, 2, 2, 2, 2, 2, 2, 2, 2, 2, 2, 2, 2, 2, 2, 2, 4 ),
 ( 0.001466970120733069325, 0.001928437086138543640, 0.002389904051544017739, 0.002620637534246755655, 0.002736004275598119193, 0.002851371016949482730, 0.002966737758300846267, 0.003082104499652209804, 0.003312837982354939481, 0.003774304947760222760, 0.004235771913165505172, 0.005158705843975971983, 0.006081639774786438794, 0.006543106740191636204, 0.007004573705596833615, 0.007119940446948069650, 0.007177623817623719760, 0.007235307188299369870, 0.007350673929650749887, 0.007466040671002129904, 0.007696774153704884734, 0.007927507636407640432, 0.008158241119110395262, 0.008388974601813150092, 0.008850441567218573016 ),
 .UNSPECIFIED. ) ;
#81633=CARTESIAN_POINT ( 'NONE',  ( 121.6288370910339864, 229.4824982072973398, 3.021315404115420679E-15 ) ) ;
#81635=CARTESIAN_POINT ( 'NONE',  ( 155.5211745099813356, 261.2764194263634749, -17.18163098020766810 ) ) ;
#81637=CARTESIAN_POINT ( 'NONE',  ( 148.7149237849385770, 273.0651914911900917, 9.533111688205226031 ) ) ;
#81639=EDGE_CURVE ( 'NONE', #85118, #66481, #66180, .T. ) ;
#81640=CARTESIAN_POINT ( 'NONE',  ( 207.1007598919583472, 271.9379569114424271, -6.086525981869248092 ) ) ;
#81644=CARTESIAN_POINT ( 'NONE',  ( 153.0305350670531936, 277.3750776671890890, 8.290292975357761662 ) ) ;
#81645=CARTESIAN_POINT ( 'NONE',  ( 152.3606757194620229, 270.2396459880571342, -14.76350148286496555 ) ) ;
#81647=CARTESIAN_POINT ( 'NONE',  ( 208.0692320075777957, 270.2605140014760536, 2.043861372130216569 ) ) ;
#81648=CARTESIAN_POINT ( 'NONE',  ( 129.8627877943888791, 245.7833772461660544, -9.188101187500095079 ) ) ;
#81649=VERTEX_POINT ( 'NONE', #31946 ) ;
#81651=CARTESIAN_POINT ( 'NONE',  ( 84.29722201641486379, 226.1427522451419065, 10.00000000000009415 ) ) ;
#81652=CARTESIAN_POINT ( 'NONE',  ( 205.5208005306483017, 273.6775489442410390, -10.63251936667145081 ) ) ;
#81653=CARTESIAN_POINT ( 'NONE',  ( 204.5831314780710954, 276.2986172388744421, 13.28075685133257089 ) ) ;
#81658=CARTESIAN_POINT ( 'NONE',  ( 167.5947507133649310, 249.2327294981003263, -5.855345954056704549 ) ) ;
#81659=CARTESIAN_POINT ( 'NONE',  ( 147.6281730237836882, 275.3355110443876583, 3.207598580681599643 ) ) ;
#81660=CARTESIAN_POINT ( 'NONE',  ( 206.7156906810202770, 272.6049163492177740, -10.59685249612386571 ) ) ;
#81661=CARTESIAN_POINT ( 'NONE',  ( 166.2786698706664765, 279.3007919285489606, -14.16120680810289301 ) ) ;
#81662=CARTESIAN_POINT ( 'NONE',  ( 196.0043407458614126, 263.5071561960751865, 0.8773891917627181236 ) ) ;
#81663=B_SPLINE_CURVE_WITH_KNOTS ( 'NONE', 3,
 ( #46008, #14640, #30836, #8538, #85068, #24726, #76925, #7526, #61722, #38921, #31326, #38418, #69333, #22741, #55116, #39410, #39907, #62716, #45520, #69826, #62213, #15114, #1451, #23222, #54111, #99749, #61224, #437, #86103, #93165, #100254, #94175, #23715, #76451, #84089, #53620, #7028, #70325, #54610, #16629, #85593, #30334, #47032, #92188, #16134, #31815 ),
 .UNSPECIFIED., .F., .F.,
 ( 4, 2, 2, 2, 2, 2, 2, 2, 2, 2, 2, 2, 2, 2, 2, 2, 2, 2, 2, 2, 2, 2, 4 ),
 ( 0.001735191271250833937, 0.002191273913610610868, 0.002647356555970387798, 0.002875397877150307271, 0.002989418537740283922, 0.003103439198330260572, 0.003331480519510220811, 0.003559521840690181918, 0.004015604483050082447, 0.004471687125409982977, 0.005383852410129784036, 0.006296017694849584227, 0.006752100337209405827, 0.007208182979569228294, 0.007322203640159166346, 0.007379213970454106750, 0.007436224300749048888, 0.007550244961338901939, 0.007664265621928754990, 0.008120348264288413526, 0.008576430906648068592, 0.008804472227827903064, 0.009032513549007735801 ),
 .UNSPECIFIED. ) ;
#81664=CARTESIAN_POINT ( 'NONE',  ( 182.4004271739244700, 284.1903799708203451, 16.39187655311515002 ) ) ;
#81666=CARTESIAN_POINT ( 'NONE',  ( 204.7237927799493775, 276.0549847173622879, -12.81020997223575364 ) ) ;
#81667=CARTESIAN_POINT ( 'NONE',  ( 174.5969907055684018, 251.7067686988808077, 3.596065318713836945 ) ) ;
#81670=CARTESIAN_POINT ( 'NONE',  ( 190.2318383114841254, 301.1557861577188078, 3.177919994438449525 ) ) ;
#81671=CARTESIAN_POINT ( 'NONE',  ( 168.8563211758018099, 286.0187424789903048, -9.056861680415359217 ) ) ;
#81672=CARTESIAN_POINT ( 'NONE',  ( 155.4810912439522212, 261.3458456796594760, -18.44218279064527266 ) ) ;
#81674=CARTESIAN_POINT ( 'NONE',  ( 193.2549072042652938, 289.0724932029194747, 16.12968917536251112 ) ) ;
#81675=CARTESIAN_POINT ( 'NONE',  ( 131.0625938207745662, 253.1427522451419350, 10.00000000000009237 ) ) ;
#81677=CARTESIAN_POINT ( 'NONE',  ( 182.0338464029501040, 278.3680066549227945, 17.69288446120480174 ) ) ;
#81679=EDGE_CURVE ( 'NONE', #73728, #56977, #60519, .T. ) ;
#81681=CARTESIAN_POINT ( 'NONE',  ( 148.4049257185216106, 273.6021238924720365, 8.639190357831699529 ) ) ;
#81682=CARTESIAN_POINT ( 'NONE',  ( 2.070087696330116689, 165.8768266524159856, -9.188101187500093303 ) ) ;
#81683=CARTESIAN_POINT ( 'NONE',  ( 46.20988612576196175, 206.6744531367911009, 4.594050593750047540 ) ) ;
#81684=CARTESIAN_POINT ( 'NONE',  ( 178.3284622040489182, 258.9725433493954938, -10.32068595145413070 ) ) ;
#81687=CARTESIAN_POINT ( 'NONE',  ( 205.3943609285979051, 274.8935266139653777, -13.14270440534009943 ) ) ;
#81689=CARTESIAN_POINT ( 'NONE',  ( 147.5813496936708020, 275.0285994114094592, 4.516581957185684004 ) ) ;
#81690=CARTESIAN_POINT ( 'NONE',  ( 149.8523222352334585, 276.3723033856174993, 3.703967980727939757 ) ) ;
#81691=CARTESIAN_POINT ( 'NONE',  ( 66.27852879613530490, 220.6199935810940644, 2.679491924311251605 ) ) ;
#81692=CARTESIAN_POINT ( 'NONE',  ( 72.31720393073018727, 205.8927522451418213, 10.00000000000009592 ) ) ;
#81695=CARTESIAN_POINT ( 'NONE',  ( 198.0384979254556015, 287.6342550689238351, 17.28192639992792579 ) ) ;
#81697=CARTESIAN_POINT ( 'NONE',  ( 34.73530984921583098, 200.8615022471903160, 5.000000000000046185 ) ) ;
#81698=CARTESIAN_POINT ( 'NONE',  ( 183.0123155676400017, 292.3663792116327045, 9.373780817324643522 ) ) ;
#81699=CARTESIAN_POINT ( 'NONE',  ( 149.7247407264208618, 272.0633196944937140, -11.44969454563192279 ) ) ;
#81700=CARTESIAN_POINT ( 'NONE',  ( 9.485603764116877556, 164.0327760586659451, 1.948934522072303157E-15 ) ) ;
#81701=CARTESIAN_POINT ( 'NONE',  ( 167.8403557585028238, 287.0638538939059572, 5.056128628522604807 ) ) ;
#81704=CARTESIAN_POINT ( 'NONE',  ( 82.43887584100872346, 211.7365022471901455, -10.00000000000009237 ) ) ;
#81706=CARTESIAN_POINT ( 'NONE',  ( 164.4781197247689306, 245.7625352337404649, -1.511762618280499515 ) ) ;
#81707=CARTESIAN_POINT ( 'NONE',  ( 154.9226727788713731, 262.3130548330639726, 18.22497199616848818 ) ) ;
#81708=CARTESIAN_POINT ( 'NONE',  ( 148.7899746831494951, 275.3503135630597285, 7.551395034694676767 ) ) ;
#81713=CARTESIAN_POINT ( 'NONE',  ( 204.1541407990405332, 272.6956988606675623, 11.22829397770025395 ) ) ;
#81715=CARTESIAN_POINT ( 'NONE',  ( 152.7451086342026372, 277.4192470735611664, -5.215848642440160887 ) ) ;
#81717=CARTESIAN_POINT ( 'NONE',  ( 156.9269804116493674, 276.4015752635256717, 10.91086647732385906 ) ) ;
#81718=CARTESIAN_POINT ( 'NONE',  ( 206.7408728089182546, 272.5612996242556960, -10.63134519248043475 ) ) ;
#81720=CARTESIAN_POINT ( 'NONE',  ( 192.6773196027083372, 296.9200883123592689, 11.15745042875121484 ) ) ;
#81725=ORIENTED_EDGE ( 'NONE', *, *, #79664, .F. ) ;
#81726=CARTESIAN_POINT ( 'NONE',  ( 159.7739451486069129, 278.5727107813384578, -9.701063066010021885 ) ) ;
#81727=CARTESIAN_POINT ( 'NONE',  ( 204.5730103890532519, 276.3161474792809145, 14.88139715235883109 ) ) ;
#81728=CARTESIAN_POINT ( 'NONE',  ( 192.6797324865049745, 296.9159090750308110, 12.42053959885222625 ) ) ;
#81731=CARTESIAN_POINT ( 'NONE',  ( 176.1222898868072377, 263.1452895647582295, 14.39881833071060591 ) ) ;
#81740=CARTESIAN_POINT ( 'NONE',  ( 203.0389248067080814, 268.2143839803633227, 2.500499824216583011 ) ) ;
#81741=CARTESIAN_POINT ( 'NONE',  ( 164.9103019330012216, 245.0139736909548560, 2.841678961959298810 ) ) ;
#81744=CARTESIAN_POINT ( 'NONE',  ( 148.9498507103374152, 272.6582861203333437, 11.90061892622094852 ) ) ;
#81745=CARTESIAN_POINT ( 'NONE',  ( 168.9465774574146053, 261.3817357245186486, -16.22414195487736777 ) ) ;
#81747=CARTESIAN_POINT ( 'NONE',  ( 156.8020845273852615, 266.4781374791638768, -16.27585026529224521 ) ) ;
#81748=ORIENTED_EDGE ( 'NONE', *, *, #86935, .T. ) ;
#81755=DIRECTION ( 'NONE',  ( -0.8660254037844387076, -0.4999999999999998890, -0.000000000000000000 ) ) ;
#81756=CARTESIAN_POINT ( 'NONE',  ( 153.3100492430090753, 265.1062007306585997, 16.32434963471121492 ) ) ;
#81757=CARTESIAN_POINT ( 'NONE',  ( 34.30229714732364954, 190.6115022471902591, 10.00000000000009592 ) ) ;
#81758=CARTESIAN_POINT ( 'NONE',  ( 197.5317255130193246, 288.5120106351379832, -18.16135075925290465 ) ) ;
#81761=CARTESIAN_POINT ( 'NONE',  ( 206.5280879940269756, 272.9298537347264642, 11.21709153681466731 ) ) ;
#81762=CARTESIAN_POINT ( 'NONE',  ( 149.3253462891332219, 272.0079086998416074, -12.99539319630191336 ) ) ;
#81763=CARTESIAN_POINT ( 'NONE',  ( 164.4261001824251878, 245.8526357240660900, 1.583002802772015549 ) ) ;
#81764=CYLINDRICAL_SURFACE ( 'NONE', #80114, 10.00000000000010658 ) ;
#81767=CARTESIAN_POINT ( 'NONE',  ( 184.5921257832661126, 275.4691417599202055, 16.38528715067328179 ) ) ;
#81773=CARTESIAN_POINT ( 'NONE',  ( 160.2441359297705219, 253.0960102851007605, -14.63485326429217537 ) ) ;
#81774=CARTESIAN_POINT ( 'NONE',  ( 148.3276789103558997, 273.7359192889379074, -8.831907802783907968 ) ) ;
#81775=ORIENTED_EDGE ( 'NONE', *, *, #28208, .T. ) ;
#81776=CARTESIAN_POINT ( 'NONE',  ( 170.5504771200006076, 255.5552483777219095, -11.63320334257268840 ) ) ;
#81777=CARTESIAN_POINT ( 'NONE',  ( 205.7578342874187740, 273.6337450154945827, 10.12066660866375400 ) ) ;
#81779=CARTESIAN_POINT ( 'NONE',  ( 165.0387478276132072, 244.7914988754632191, -2.473354058663827626 ) ) ;
#81780=CARTESIAN_POINT ( 'NONE',  ( 34.13991738056614622, 190.5177522451418497, -10.00000000000009592 ) ) ;
#81781=CARTESIAN_POINT ( 'NONE',  ( 95.92524373570365981, 232.3149278399160949, -9.188101187500095079 ) ) ;
#81784=CARTESIAN_POINT ( 'NONE',  ( 162.8265537361057795, 249.1312387917435558, -10.34784883127201915 ) ) ;
#81787=CARTESIAN_POINT ( 'NONE',  ( 30.64892602121659593, 182.3768266524159856, -9.188101187500091527 ) ) ;
#81788=CARTESIAN_POINT ( 'NONE',  ( 204.6350011963004647, 275.7068757420208271, -12.64342396695018245 ) ) ;
#81796=CARTESIAN_POINT ( 'NONE',  ( 161.7412967960748915, 250.5028515975580774, -14.36228887024421041 ) ) ;
#81800=CARTESIAN_POINT ( 'NONE',  ( 47.23881193640350062, 188.8923013555410080, 4.594050593750050204 ) ) ;
#81801=CARTESIAN_POINT ( 'NONE',  ( 93.10181362155671536, 217.8927522451418213, 10.00000000000009592 ) ) ;
#81802=ORIENTED_EDGE ( 'NONE', *, *, #58549, .T. ) ;
#81803=CARTESIAN_POINT ( 'NONE',  ( 197.3520635096637648, 267.5934713644667795, -7.874698761606322428 ) ) ;
#81808=CARTESIAN_POINT ( 'NONE',  ( 2.557053438076354990, 172.2833772461660828, -9.188101187500095079 ) ) ;
#81809=CARTESIAN_POINT ( 'NONE',  ( 150.9003228897357189, 269.2799692068659283, -14.30003212299500781 ) ) ;
#81811=CARTESIAN_POINT ( 'NONE',  ( 192.6679047218190135, 296.9363953644068488, -13.34486378385621386 ) ) ;
#81813=CARTESIAN_POINT ( 'NONE',  ( 58.06412948370898164, 195.1423013555410080, -4.594050593750043987 ) ) ;
#81814=CARTESIAN_POINT ( 'NONE',  ( 208.2777459429579210, 269.8993572713111462, 3.129643751043610589 ) ) ;
#81815=CARTESIAN_POINT ( 'NONE',  ( 203.7776468208327003, 276.2971780117193248, 13.33764639693685616 ) ) ;
#81817=CARTESIAN_POINT ( 'NONE',  ( 147.6140518775699491, 274.9719575673779559, 8.457032797753797126 ) ) ;
#81818=ORIENTED_EDGE ( 'NONE', *, *, #23403, .T. ) ;
#81820=CARTESIAN_POINT ( 'NONE',  ( -0.6995629222974718564, 183.7365022471903444, 2.944929066748280225E-16 ) ) ;
#81822=CARTESIAN_POINT ( 'NONE',  ( 124.1521724663614492, 251.6744531367911577, 4.594050593750047540 ) ) ;
#81824=CARTESIAN_POINT ( 'NONE',  ( 206.9146873713863783, 272.2602439709654618, -8.162908012510746047 ) ) ;
#81825=CARTESIAN_POINT ( 'NONE',  ( 150.9988863956583600, 269.5412616643368438, 13.78873124909360293 ) ) ;
#81828=CARTESIAN_POINT ( 'NONE',  ( 190.6426292480107350, 300.4442753843661080, -6.777079808125155758 ) ) ;
#81829=ORIENTED_EDGE ( 'NONE', *, *, #63047, .T. ) ;
#81830=CARTESIAN_POINT ( 'NONE',  ( 191.3638605175971747, 299.1950661814348678, 7.382965314423603154 ) ) ;
#81831=CARTESIAN_POINT ( 'NONE',  ( 208.2584889301005546, 269.9327113959824374, -1.669397994094046211 ) ) ;
#81832=CARTESIAN_POINT ( 'NONE',  ( 185.2961235551778714, 291.2460235572835927, 13.48139818756336616 ) ) ;
#81833=CARTESIAN_POINT ( 'NONE',  ( 170.4818684897218759, 266.4664816474689246, -17.63139018167740701 ) ) ;
#81841=AXIS2_PLACEMENT_3D ( 'NONE', #27658, #66142, #73749 ) ;
#81842=CARTESIAN_POINT ( 'NONE',  ( 184.5043411789232266, 295.9227417631768731, 4.662132045941501879 ) ) ;
#81846=CARTESIAN_POINT ( 'NONE',  ( 193.8615474287298355, 282.6207621793728322, 17.07927997190257940 ) ) ;
#81848=CARTESIAN_POINT ( 'NONE',  ( 191.9828369562736441, 287.6126897466953665, -16.13172383425306933 ) ) ;
#81851=CARTESIAN_POINT ( 'NONE',  ( 194.7576540903134799, 293.3168432830895540, -14.62421624641040196 ) ) ;
#81854=CARTESIAN_POINT ( 'NONE',  ( 185.4551394198477681, 291.0484231367762504, 12.14165578421975233 ) ) ;
#81855=CARTESIAN_POINT ( 'NONE',  ( 204.9780665305064531, 275.6145696623662502, 14.10615427165218883 ) ) ;
#81856=EDGE_CURVE ( 'NONE', #63287, #70064, #16646, .T. ) ;
#81858=EDGE_LOOP ( 'NONE', ( #42305, #79558, #60586, #80617, #88261 ) ) ;
#81859=CARTESIAN_POINT ( 'NONE',  ( 86.20995510670323370, 211.3923013555409796, 4.594050593750050204 ) ) ;
#81860=CARTESIAN_POINT ( 'NONE',  ( 202.8905955564125065, 279.2301754488222514, 15.56958316349127358 ) ) ;
#81861=CARTESIAN_POINT ( 'NONE',  ( 189.4199209167946663, 300.3895034224956930, 3.306026617473488027 ) ) ;
#81863=VERTEX_POINT ( 'NONE', #21261 ) ;
#81866=ORIENTED_EDGE ( 'NONE', *, *, #29720, .F. ) ;
#81867=CARTESIAN_POINT ( 'NONE',  ( 192.7041411452173918, 293.9924959157295916, 14.27507663239260971 ) ) ;
#81869=EDGE_CURVE ( 'NONE', #21409, #87939, #43184, .T. ) ;
#81871=CARTESIAN_POINT ( 'NONE',  ( 155.4495868485232108, 261.4004128932040203, -18.48326470492642315 ) ) ;
#81873=CARTESIAN_POINT ( 'NONE',  ( 165.0633574835339346, 244.7488737010519628, 1.949578632198007977 ) ) ;
#81875=CARTESIAN_POINT ( 'NONE',  ( 147.1692232402260174, 275.7424233679190593, -6.897157937245698811 ) ) ;
#81878=CARTESIAN_POINT ( 'NONE',  ( 170.2835531134608686, 278.8928912914798275, -15.69417418368842654 ) ) ;
#81880=CARTESIAN_POINT ( 'NONE',  ( 147.1836429658426084, 243.5327760586659451, 1.948934522072303157E-15 ) ) ;
#81881=CARTESIAN_POINT ( 'NONE',  ( 164.9790521326853536, 265.2878599192118827, -16.61474165352627352 ) ) ;
#81884=ORIENTED_EDGE ( 'NONE', *, *, #19895, .F. ) ;
#81886=CARTESIAN_POINT ( 'NONE',  ( 167.3703416170141338, 284.2892190735486224, 9.299199617839436272 ) ) ;
#81887=CARTESIAN_POINT ( 'NONE',  ( 201.8432742760849123, 271.0906551529850503, 9.350329334099363621 ) ) ;
#81892=CARTESIAN_POINT ( 'NONE',  ( 153.3922461054063433, 276.8823880860896338, 7.152063237113233996 ) ) ;
#81894=( BOUNDED_CURVE ( )  B_SPLINE_CURVE ( 2, ( #99730, #92651, #30317, #61204, #100235, #84558, #61699, #15097, #15595 ),
 .UNSPECIFIED., .F., .T. ) 
 B_SPLINE_CURVE_WITH_KNOTS ( ( 3, 2, 2, 2, 3 ),
 ( 0.02016129032258064807, 0.02150537634408602322, 0.02419354838709677352, 0.02688172043010752729, 0.02822580645161290591 ),
 .UNSPECIFIED. ) 
 CURVE ( )  GEOMETRIC_REPRESENTATION_ITEM ( )  RATIONAL_B_SPLINE_CURVE ( ( 0.9330127018922192983, 0.9330127018922194093, 1.000000000000000000, 0.8660254037844387076, 1.000000000000000000, 0.8660254037844387076, 1.000000000000000000, 0.9330127018922191873, 0.9330127018922192983 ) ) 
 REPRESENTATION_ITEM ( '' )  );
#81899=ORIENTED_EDGE ( 'NONE', *, *, #57951, .F. ) ;
#81900=CARTESIAN_POINT ( 'NONE',  ( 185.0763070350663781, 273.0824188773292462, -16.90268598921084120 ) ) ;
#81902=VERTEX_POINT ( 'NONE', #16145 ) ;
#81903=CARTESIAN_POINT ( 'NONE',  ( 160.1979016687359092, 276.4615463954939401, 12.73367540184897351 ) ) ;
#81904=CARTESIAN_POINT ( 'NONE',  ( 156.5654777510188183, 277.0389622341601807, 9.949659676293464372 ) ) ;
#81905=CARTESIAN_POINT ( 'NONE',  ( 190.1758200331204876, 279.2204749713225169, -17.78067544974210890 ) ) ;
#81907=CARTESIAN_POINT ( 'NONE',  ( 160.8137364596917109, 272.7584256728402465, 15.66121798818901567 ) ) ;
#81910=CARTESIAN_POINT ( 'NONE',  ( 200.1347818429666177, 267.8741717063466581, 6.125758183920250843 ) ) ;
#81913=ORIENTED_EDGE ( 'NONE', *, *, #67764, .T. ) ;
#81916=CARTESIAN_POINT ( 'NONE',  ( 125.7401460302306759, 236.7365022471902307, 10.00000000000009948 ) ) ;
#81919=CARTESIAN_POINT ( 'NONE',  ( 171.9101151227116020, 289.4071025166348932, 2.638113784258313554 ) ) ;
#81923=CARTESIAN_POINT ( 'NONE',  ( 4.614210867829411811, 161.2202760586659451, -5.415160957724236172E-17 ) ) ;
#81924=CARTESIAN_POINT ( 'NONE',  ( 98.52331994705694740, 233.8149278399160949, -9.188101187500095079 ) ) ;
#81926=CARTESIAN_POINT ( 'NONE',  ( 179.9282632979647474, 254.9894960794134136, -2.420314024967571864 ) ) ;
#81928=EDGE_CURVE ( 'NONE', #57417, #41328, #76803, .T. ) ;
#81930=CARTESIAN_POINT ( 'NONE',  ( 167.6146168596400514, 252.8497314824998909, -12.44459218179994231 ) ) ;
#81931=CARTESIAN_POINT ( 'NONE',  ( 194.1852025340051284, 294.3083584634874796, -15.46421316575964688 ) ) ;
#81934=CARTESIAN_POINT ( 'NONE',  ( 182.0171333322937528, 267.6076494233564063, -14.80649776740987278 ) ) ;
#81935=CARTESIAN_POINT ( 'NONE',  ( 172.5499481646635331, 263.5659312731885962, -15.40879909798235836 ) ) ;
#81936=CARTESIAN_POINT ( 'NONE',  ( 83.09741599002914825, 218.7833772461660544, -9.188101187500095079 ) ) ;
#81938=CARTESIAN_POINT ( 'NONE',  ( 191.4685399627163633, 299.0137560639802814, 7.545791216288330716 ) ) ;
#81940=CARTESIAN_POINT ( 'NONE',  ( 157.6335212189247557, 257.6177276032722716, 16.76495363836117036 ) ) ;
#81942=CARTESIAN_POINT ( 'NONE',  ( 149.1585757751420829, 272.2967637032783728, 11.60936825230297842 ) ) ;
#81943=CARTESIAN_POINT ( 'NONE',  ( 151.3681950933278983, 268.4695907787949523, -15.50699599486383917 ) ) ;
#81944=CARTESIAN_POINT ( 'NONE',  ( 204.1506106421540494, 276.0852532772063341, -13.43628313753478487 ) ) ;
#81947=CARTESIAN_POINT ( 'NONE',  ( 147.5851099763508216, 275.0220864107570264, -4.372720440640867956 ) ) ;
#81951=CARTESIAN_POINT ( 'NONE',  ( 181.8509774751104544, 266.9677320091309412, 16.09658033613713712 ) ) ;
#81953=CARTESIAN_POINT ( 'NONE',  ( 192.4335622838504207, 297.3422883733380786, -12.83044365323471325 ) ) ;
#81954=CARTESIAN_POINT ( 'NONE',  ( 65.04619898167126735, 198.3615022471901739, 5.000000000000051514 ) ) ;
#81955=ORIENTED_EDGE ( 'NONE', *, *, #37382, .T. ) ;
#81959=CARTESIAN_POINT ( 'NONE',  ( 193.8003511027313550, 288.1208047801705447, 17.19107869180001913 ) ) ;
#81960=CARTESIAN_POINT ( 'NONE',  ( 182.7847760313759409, 280.0284915794045446, -17.53211380394024843 ) ) ;
#81961=CARTESIAN_POINT ( 'NONE',  ( 133.0291931787496367, 257.6115022471902876, -5.000000000000047962 ) ) ;
#81962=CARTESIAN_POINT ( 'NONE',  ( 204.6713671561005299, 276.1457885614869951, -12.94307097876490431 ) ) ;
#81965=CARTESIAN_POINT ( 'NONE',  ( 190.8228695072887149, 299.3521595973184617, -6.560059525124882995 ) ) ;
#81966=CARTESIAN_POINT ( 'NONE',  ( 169.4432399169915016, 248.6629731721966436, -1.917647540753971480 ) ) ;
#81968=CARTESIAN_POINT ( 'NONE',  ( 196.5171250811640675, 264.4500657306584230, -4.685409136380966899 ) ) ;
#81974=CARTESIAN_POINT ( 'NONE',  ( 158.3301009428178361, 256.4112161299673858, 16.93297520252109933 ) ) ;
#81977=CARTESIAN_POINT ( 'NONE',  ( 202.8483755843326719, 275.3371640334334529, -14.10040576359822317 ) ) ;
#81978=DIRECTION ( 'NONE',  ( 0.4999999999999998890, -0.8660254037844385966, 0.000000000000000000 ) ) ;
#81979=EDGE_CURVE ( 'NONE', #34461, #40710, #22752, .T. ) ;
#81985=DIRECTION ( 'NONE',  ( 0.4999999999999998890, -0.8660254037844385966, 0.000000000000000000 ) ) ;
#81988=VERTEX_POINT ( 'NONE', #7539 ) ;
#81989=VERTEX_POINT ( 'NONE', #62728 ) ;
#81991=CARTESIAN_POINT ( 'NONE',  ( 163.8990931530087494, 246.7654386749614162, 5.873176884778091633 ) ) ;
#81992=CARTESIAN_POINT ( 'NONE',  ( 162.2535035907551730, 272.2911684813469151, -15.91294751376331007 ) ) ;
#81994=DIRECTION ( 'NONE',  ( -0.4999999999999987788, 0.8660254037844392627, 0.000000000000000000 ) ) ;
#81995=CARTESIAN_POINT ( 'NONE',  ( 154.4470374439381146, 277.6591429590598068, -9.115886381272481742 ) ) ;
#81997=CARTESIAN_POINT ( 'NONE',  ( 169.4077006606329405, 286.8755356998590855, -4.641866896595598924 ) ) ;
#81999=CARTESIAN_POINT ( 'NONE',  ( 169.2387200762215684, 267.1480446973579888, 16.80865198575004982 ) ) ;
#82000=CARTESIAN_POINT ( 'NONE',  ( 181.7124919110368921, 257.0325072718674164, 5.021470642198736734 ) ) ;
#82001=CARTESIAN_POINT ( 'NONE',  ( 104.0717290597573026, 221.7048013555409796, 4.594050593750051981 ) ) ;
#82005=CARTESIAN_POINT ( 'NONE',  ( 166.7216842753552157, 278.1553442122267370, -13.35919087224943880 ) ) ;
#82007=ORIENTED_EDGE ( 'NONE', *, *, #73429, .T. ) ;
#82011=CARTESIAN_POINT ( 'NONE',  ( 179.2777005192219235, 293.2395681535716108, -2.642785613701771563 ) ) ;
#82012=CARTESIAN_POINT ( 'NONE',  ( 196.3341081413628899, 290.5863447708742342, 16.12390540996472410 ) ) ;
#82013=CARTESIAN_POINT ( 'NONE',  ( 159.5050723400634638, 254.3761059724978679, -15.34938048045353298 ) ) ;
#82015=CARTESIAN_POINT ( 'NONE',  ( 208.3379394461497895, 269.7950990654974817, 2.541397148058371691 ) ) ;
#82018=VERTEX_POINT ( 'NONE', #24249 ) ;
#82019=CARTESIAN_POINT ( 'NONE',  ( 189.5534384022301424, 269.0062095459838929, -14.92796778812864922 ) ) ;
#82020=CARTESIAN_POINT ( 'NONE',  ( 207.8446715390582540, 270.6494641423232679, -2.429516028743652800 ) ) ;
#82021=ORIENTED_EDGE ( 'NONE', *, *, #49370, .T. ) ;
#82023=DIRECTION ( 'NONE',  ( 0.4999999999999998890, -0.8660254037844385966, 0.000000000000000000 ) ) ;
#82025=DIRECTION ( 'NONE',  ( -0.8660254037844387076, -0.4999999999999998890, -0.000000000000000000 ) ) ;
#82026=CARTESIAN_POINT ( 'NONE',  ( 130.5662598870812019, 252.3149278399160664, 9.188101187500093303 ) ) ;
#82027=CARTESIAN_POINT ( 'NONE',  ( 199.9289737974172567, 283.7008907154707344, 17.00951001457953637 ) ) ;
#82029=VERTEX_POINT ( 'NONE', #85080 ) ;
#82031=CARTESIAN_POINT ( 'NONE',  ( 69.55128746018320385, 199.4155109091896065, 2.679491924311254714 ) ) ;
#82033=EDGE_CURVE ( 'NONE', #31533, #94451, #75893, .T. ) ;
#82034=CARTESIAN_POINT ( 'NONE',  ( 206.7893622945242385, 272.4773133715531230, -10.52881283832460291 ) ) ;
#82035=CARTESIAN_POINT ( 'NONE',  ( 170.0332508499076312, 248.8708985649008696, -0.2654087898054893757 ) ) ;
#82036=CARTESIAN_POINT ( 'NONE',  ( 33.96495592097634386, 201.9637435831425023, 2.679491924311251605 ) ) ;
#82039=CARTESIAN_POINT ( 'NONE',  ( 199.0897609194714164, 281.8722272735701040, -16.59838435980774562 ) ) ;
#82040=CARTESIAN_POINT ( 'NONE',  ( 136.4265865026747804, 261.1199935810940360, 2.679491924311251605 ) ) ;
#82043=CARTESIAN_POINT ( 'NONE',  ( 206.7925996035142759, 272.0411403573240818, 6.555066398942419603 ) ) ;
#82044=CARTESIAN_POINT ( 'NONE',  ( 167.6018919913909428, 249.9623704280710967, 7.441045516060340148 ) ) ;
#82046=CARTESIAN_POINT ( 'NONE',  ( 207.6837091943624785, 270.9282591014416539, -1.156610046911421552 ) ) ;
#82051=CARTESIAN_POINT ( 'NONE',  ( 177.5665759502285539, 275.7863988818428993, 17.69313789786682989 ) ) ;
#82055=CARTESIAN_POINT ( 'NONE',  ( 187.0083344850037008, 268.0836409071914090, -15.22627500120235133 ) ) ;
#82063=CARTESIAN_POINT ( 'NONE',  ( 207.2337123599961899, 271.7076764818092443, -5.443417788256701861 ) ) ;
#82064=CARTESIAN_POINT ( 'NONE',  ( 22.80074434730262567, 171.7202760586659736, -5.415160957724236172E-17 ) ) ;
#82069=CARTESIAN_POINT ( 'NONE',  ( 164.3890147726454813, 245.9168695380243435, -6.010262808998044548 ) ) ;
#82071=CARTESIAN_POINT ( 'NONE',  ( 55.49285624440017273, 202.8458772461660260, 9.188101187500095079 ) ) ;
#82072=CARTESIAN_POINT ( 'NONE',  ( 84.34903687182406884, 231.0530062829863027, -4.648177544792955347E-16 ) ) ;
#82074=CARTESIAN_POINT ( 'NONE',  ( 190.3625087333586521, 300.9294583479858147, -4.271886578030237303 ) ) ;
#82076=CARTESIAN_POINT ( 'NONE',  ( 199.6805176955043066, 267.7911124590283976, -6.556812613813658430 ) ) ;
#82077=CARTESIAN_POINT ( 'NONE',  ( 191.0933613939813540, 299.6635844069401173, -8.689828987424775164 ) ) ;
#82078=ORIENTED_EDGE ( 'NONE', *, *, #25902, .F. ) ;
#82084=CARTESIAN_POINT ( 'NONE',  ( 92.75901190277325270, 224.3615022471902591, -10.00000000000009592 ) ) ;
#82087=VERTEX_POINT ( 'NONE', #90536 ) ;
#82088=CARTESIAN_POINT ( 'NONE',  ( 60.68900866710680475, 205.8458772461660544, 9.188101187500095079 ) ) ;
#82090=CARTESIAN_POINT ( 'NONE',  ( 166.0118957362736012, 265.2928580242756880, 16.55930147465089064 ) ) ;
#82091=CARTESIAN_POINT ( 'NONE',  ( 161.5400823882263808, 251.2469044075661486, 12.89492200680558120 ) ) ;
#82094=CARTESIAN_POINT ( 'NONE',  ( 167.8036517631731215, 285.0360000349990628, 7.673623445836456725 ) ) ;
#82095=CARTESIAN_POINT ( 'NONE',  ( 207.0548180518391916, 272.0175305127218053, 7.721676452263806389 ) ) ;
#82098=CARTESIAN_POINT ( 'NONE',  ( 186.3038661936600704, 263.7620536213361788, 10.91854419716388769 ) ) ;
#82101=CARTESIAN_POINT ( 'NONE',  ( 205.0302908362115772, 275.5241145114948154, 13.44798751587103425 ) ) ;
#82109=CARTESIAN_POINT ( 'NONE',  ( 181.1411778180677175, 283.4433145892596144, 14.97450737243938157 ) ) ;
#82111=CARTESIAN_POINT ( 'NONE',  ( 206.1408608592916494, 273.6005508061571732, -10.42739367433323494 ) ) ;
#82112=ORIENTED_EDGE ( 'NONE', *, *, #40123, .F. ) ;
#82115=CARTESIAN_POINT ( 'NONE',  ( 161.6923300915171922, 250.5876644177310482, -14.43081872899884566 ) ) ;
#82117=CARTESIAN_POINT ( 'NONE',  ( 196.2878005184348353, 290.6665519265632724, -16.69183432842427806 ) ) ;
#82118=ORIENTED_EDGE ( 'NONE', *, *, #863, .F. ) ;
#82123=CARTESIAN_POINT ( 'NONE',  ( 117.4133255192225391, 250.8464784336661353, 1.353441290958777525E-15 ) ) ;
#82125=CARTESIAN_POINT ( 'NONE',  ( 190.9501423151522772, 299.9116471280854626, 8.746938802470586083 ) ) ;
#82126=CARTESIAN_POINT ( 'NONE',  ( 67.84273934451053378, 216.6427522451419065, -10.00000000000009592 ) ) ;
#82127=VERTEX_POINT ( 'NONE', #13501 ) ;
#82129=CARTESIAN_POINT ( 'NONE',  ( 207.5215400641004351, 271.2091442744748520, 2.886080616848571534 ) ) ;
#82130=VERTEX_POINT ( 'NONE', #14958 ) ;
#82131=ORIENTED_EDGE ( 'NONE', *, *, #38048, .F. ) ;
#82133=CARTESIAN_POINT ( 'NONE',  ( 204.8370930553071503, 274.7064833943479698, -12.16292712972826706 ) ) ;
#82134=CARTESIAN_POINT ( 'NONE',  ( 76.25066296318219372, 205.6423013555409796, -4.594050593750043987 ) ) ;
#82137=CARTESIAN_POINT ( 'NONE',  ( 22.95375591501717594, 177.3927522451418497, 10.00000000000009948 ) ) ;
#82139=CARTESIAN_POINT ( 'NONE',  ( 198.6416989287814943, 286.5894802839873137, 18.33538993684147300 ) ) ;
#82140=CARTESIAN_POINT ( 'NONE',  ( 173.3845174282522237, 277.2994966234552408, 15.60446512967379284 ) ) ;
#82141=ADVANCED_FACE ( 'NONE', ( #91510 ), #53460, .T. ) ;
#82146=CARTESIAN_POINT ( 'NONE',  ( 201.0468719883840265, 282.4235983437597497, -16.59631526626950659 ) ) ;
#82147=CARTESIAN_POINT ( 'NONE',  ( -27.42236680055714260, 166.5217562850347406, 1.224646799147364892E-15 ) ) ;
#82149=CARTESIAN_POINT ( 'NONE',  ( 156.6812872898450735, 261.2670451491295012, 0.000000000000000000 ) ) ;
#82150=CARTESIAN_POINT ( 'NONE',  ( 161.1093323826042933, 251.5974460702646809, -13.93502574894237078 ) ) ;
#82151=CARTESIAN_POINT ( 'NONE',  ( 164.2618602210349934, 246.6285193662782547, 4.483609632043464188 ) ) ;
#82153=CARTESIAN_POINT ( 'NONE',  ( 164.8849641302980444, 245.0578600525887794, 2.884140591399200648 ) ) ;
#82154=ORIENTED_EDGE ( 'NONE', *, *, #42742, .T. ) ;
#82156=CARTESIAN_POINT ( 'NONE',  ( 128.2929432021470859, 251.0024278399160949, 9.188101187500095079 ) ) ;
#82157=ORIENTED_EDGE ( 'NONE', *, *, #34026, .T. ) ;
#82160=CARTESIAN_POINT ( 'NONE',  ( 205.2706556652093752, 273.1077904153184477, -10.97544480913108167 ) ) ;
#82163=CARTESIAN_POINT ( 'NONE',  ( 200.6117230619925635, 269.0360104864248001, 9.242361455687714056 ) ) ;
#82164=ORIENTED_EDGE ( 'NONE', *, *, #60528, .F. ) ;
#82167=EDGE_CURVE ( 'NONE', #49046, #45423, #17724, .T. ) ;
#82168=CARTESIAN_POINT ( 'NONE',  ( 167.6380257754661045, 249.1599301665656867, -6.117841082608373782 ) ) ;
#82169=CARTESIAN_POINT ( 'NONE',  ( 205.9580306612148490, 273.9172219983844911, -10.82161348643986720 ) ) ;
#82171=CARTESIAN_POINT ( 'NONE',  ( 147.1249913145849177, 275.8190353104462815, 3.637773609013635223 ) ) ;
#82173=CARTESIAN_POINT ( 'NONE',  ( 165.5918197702007433, 245.8335501706607147, 2.182451016153225905E-15 ) ) ;
#82174=VECTOR ( 'NONE', #57858, 1000.000000000000000 ) ;
#82175=CARTESIAN_POINT ( 'NONE',  ( 195.0636388027741930, 270.1460199898987184, 12.01487925370120990 ) ) ;
#82176=EDGE_CURVE ( 'NONE', #22854, #69571, #48514, .T. ) ;
#82179=CARTESIAN_POINT ( 'NONE',  ( 149.0761751337341821, 272.4394858007734683, 11.56094486755886130 ) ) ;
#82182=CARTESIAN_POINT ( 'NONE',  ( 188.0361769804965206, 281.7550819701144746, -17.70093714309158983 ) ) ;
#82185=( BOUNDED_CURVE ( )  B_SPLINE_CURVE ( 2, ( #25084, #1305, #77301, #32188, #30703, #61583, #15476, #31674, #92534 ),
 .UNSPECIFIED., .F., .T. ) 
 B_SPLINE_CURVE_WITH_KNOTS ( ( 3, 2, 2, 2, 3 ),
 ( 0.4072580645161290591, 0.4086021505376344343, 0.4112903225806451846, 0.4139784946236559349, 0.4153225806451613100 ),
 .UNSPECIFIED. ) 
 CURVE ( )  GEOMETRIC_REPRESENTATION_ITEM ( )  RATIONAL_B_SPLINE_CURVE ( ( 0.9330127018922194093, 0.9330127018922207416, 1.000000000000000000, 0.8660254037844387076, 1.000000000000000000, 0.8660254037844387076, 1.000000000000000000, 0.9330127018922194093, 0.9330127018922194093 ) ) 
 REPRESENTATION_ITEM ( '' )  );
#82186=CARTESIAN_POINT ( 'NONE',  ( 138.1351346183475357, 243.8927522451417929, -10.00000000000009059 ) ) ;
#82187=CARTESIAN_POINT ( 'NONE',  ( 175.9837504787562636, 285.3457777721278603, -12.01839870738883143 ) ) ;
#82188=EDGE_LOOP ( 'NONE', ( #51971, #56162, #56005, #75597 ) ) ;
#82191=CARTESIAN_POINT ( 'NONE',  ( 151.0388915836658725, 269.0399611886400635, -14.24896787280406585 ) ) ;
#82192=CARTESIAN_POINT ( 'NONE',  ( -8.674473839076844328, 174.9869531367911293, 4.594050593750046652 ) ) ;
#82193=CARTESIAN_POINT ( 'NONE',  ( 53.49034604603116350, 195.5643266524160140, 9.188101187500095079 ) ) ;
#82197=AXIS2_PLACEMENT_3D ( 'NONE', #36339, #52049, #92579 ) ;
#82198=CARTESIAN_POINT ( 'NONE',  ( 157.8239779013331372, 257.2878469527003062, -17.92251383114021479 ) ) ;
#82199=CARTESIAN_POINT ( 'NONE',  ( 189.5693900039456707, 290.6981618181056888, -14.49310309556349274 ) ) ;
#82201=CARTESIAN_POINT ( 'NONE',  ( 168.7281583638259121, 257.2268137270143029, 13.70307109309566940 ) ) ;
#82203=CARTESIAN_POINT ( 'NONE',  ( 198.0542955016221924, 287.6068928643675804, 18.26164672886581997 ) ) ;
#82204=CARTESIAN_POINT ( 'NONE',  ( 179.2120688271028541, 294.1024010724993332, 1.048020959340867364 ) ) ;
#82205=CARTESIAN_POINT ( 'NONE',  ( 60.28305926085680966, 205.6115022471902591, 10.00000000000009592 ) ) ;
#82208=CARTESIAN_POINT ( 'NONE',  ( 147.6857584380539095, 274.8477581613835810, 8.112022437684441201 ) ) ;
#82209=CARTESIAN_POINT ( 'NONE',  ( 27.67213724359008964, 174.5327760586659451, 1.948934522072303157E-15 ) ) ;
#82210=CARTESIAN_POINT ( 'NONE',  ( 164.4201679284129227, 284.8060357136131415, 4.241341315168992487 ) ) ;
#82211=EDGE_CURVE ( 'NONE', #34226, #27863, #27546, .T. ) ;
#82215=CARTESIAN_POINT ( 'NONE',  ( 179.9844968997953174, 277.0016935229651267, 16.30433957883684570 ) ) ;
#82216=CARTESIAN_POINT ( 'NONE',  ( 175.4507454171546783, 278.7747778411292643, 15.41403683019787962 ) ) ;
#82218=CARTESIAN_POINT ( 'NONE',  ( 177.5011205626351227, 261.3373948018718238, -13.00779142369327523 ) ) ;
#82222=CARTESIAN_POINT ( 'NONE',  ( 13.06432082636536762, 189.8967562850346837, -4.648177544792955347E-16 ) ) ;
#82223=EDGE_LOOP ( 'NONE', ( #18592, #55980, #80009, #26077 ) ) ;
#82227=CARTESIAN_POINT ( 'NONE',  ( 206.1798448551755598, 273.5330285446045195, -10.53862763475382813 ) ) ;
#82228=B_SPLINE_CURVE_WITH_KNOTS ( 'NONE', 3,
 ( #81014, #11576, #3956, #34839, #58147, #89127, #61625, #76364, #21652, #75876, #76834, #44436, #99158, #92580, #92101, #84972, #38824, #23122, #83485, #83991, #13564, #37332, #36842, #54015, #15517, #46419, #22145, #75369, #68734, #21169, #15024, #38325, #91087, #98675, #45430, #60618, #30243, #44929, #45915, #61124, #22646, #99657, #37825, #53531, #84482, #91573, #60124, #7432 ),
 .UNSPECIFIED., .F., .F.,
 ( 4, 2, 2, 2, 2, 2, 2, 2, 2, 2, 2, 2, 2, 2, 2, 2, 2, 2, 2, 2, 2, 2, 2, 4 ),
 ( 0.0008680554427910739442, 0.001061939928173833824, 0.001158882170865213872, 0.001255824413556593921, 0.001449708898939420804, 0.001643593384322248122, 0.002031362355087858087, 0.002419131325853468052, 0.003970207208915833320, 0.004745745150447016822, 0.005133514121212644568, 0.005327398606595498340, 0.005424340849286961655, 0.005472811970632649077, 0.005521283091978336499, 0.005569754213324024789, 0.005618225334669713078, 0.005715167577361120882, 0.005909052062743800314, 0.006102936548126478011, 0.006296821033509157443, 0.006490705518891836008, 0.006684590004274514573, 0.007072358975039798844 ),
 .UNSPECIFIED. ) ;
#82229=ORIENTED_EDGE ( 'NONE', *, *, #96342, .F. ) ;
#82230=CARTESIAN_POINT ( 'NONE',  ( 152.8134625983922490, 265.9663140294953791, 17.57333028169644251 ) ) ;
#82231=LINE ( 'NONE', #83713, #77295 ) ;
#82233=CARTESIAN_POINT ( 'NONE',  ( 155.3716771045260714, 261.5353565282119348, -18.54934131471355840 ) ) ;
#82234=VERTEX_POINT ( 'NONE', #9891 ) ;
#82236=CARTESIAN_POINT ( 'NONE',  ( 159.2244323577040177, 279.5560594508606300, -9.704040566180836436 ) ) ;
#82237=CARTESIAN_POINT ( 'NONE',  ( 204.4325665793906524, 276.5594032932251594, 13.33817701435311598 ) ) ;
#82238=CARTESIAN_POINT ( 'NONE',  ( 192.6224552386041182, 297.0151161785129261, 12.49354144254605181 ) ) ;
#82239=ORIENTED_EDGE ( 'NONE', *, *, #9942, .T. ) ;
#82243=CARTESIAN_POINT ( 'NONE',  ( 177.5782878460544225, 263.8519546370548028, 14.60380941168531166 ) ) ;
#82247=ADVANCED_FACE ( 'NONE', ( #15963 ), #78281, .F. ) ;
#82250=EDGE_LOOP ( 'NONE', ( #25004, #79266, #3935 ) ) ;
#82251=CARTESIAN_POINT ( 'NONE',  ( 205.7639495959071212, 274.2533802642843170, 10.79039487422292432 ) ) ;
#82254=CARTESIAN_POINT ( 'NONE',  ( 177.8323663984979532, 279.4302167523874232, -16.28584057845160515 ) ) ;
#82255=CARTESIAN_POINT ( 'NONE',  ( 199.3359313799735162, 277.8054090533971134, 16.38672730308284997 ) ) ;
#82258=CARTESIAN_POINT ( 'NONE',  ( 149.0240550263898740, 274.5270876550541743, 9.114866661042729135 ) ) ;
#82260=EDGE_CURVE ( 'NONE', #37254, #705, #96356, .T. ) ;
#82261=CARTESIAN_POINT ( 'NONE',  ( 157.4876528856866287, 268.9475409797686325, 15.59749454131434732 ) ) ;
#82264=CARTESIAN_POINT ( 'NONE',  ( 154.5269387696429533, 265.4077020348397014, -16.45718875575290951 ) ) ;
#82268=CARTESIAN_POINT ( 'NONE',  ( 192.3606619183491091, 297.4685555102766443, 10.99569063633359889 ) ) ;
#82270=CARTESIAN_POINT ( 'NONE',  ( 194.6737116153428246, 263.0965258421714452, 3.813308892523692872 ) ) ;
#82275=CARTESIAN_POINT ( 'NONE',  ( 149.7072529793668707, 271.3464269086063041, -11.98883662638834657 ) ) ;
#82276=CARTESIAN_POINT ( 'NONE',  ( 205.9642072045669465, 273.9065239114831911, 10.22128930895731536 ) ) ;
#82277=CARTESIAN_POINT ( 'NONE',  ( 198.4264492142971221, 286.9623037257889564, 17.00126466006521397 ) ) ;
#82278=CARTESIAN_POINT ( 'NONE',  ( 171.3375887344810735, 288.5721954326351124, 4.189121038472729097 ) ) ;
#82284=CARTESIAN_POINT ( 'NONE',  ( 159.9019937409323688, 253.6886179395814622, -15.75542456264497559 ) ) ;
#82285=CARTESIAN_POINT ( 'NONE',  ( 148.1086267770833729, 274.1153287132722198, -10.31239854325041705 ) ) ;
#82287=CARTESIAN_POINT ( 'NONE',  ( 168.7890239821780085, 254.3732592748322361, -11.73109540831163500 ) ) ;
#82288=CARTESIAN_POINT ( 'NONE',  ( 205.5320288733365146, 274.0930176087748578, 10.72952057639821000 ) ) ;
#82291=CARTESIAN_POINT ( 'NONE',  ( 201.4617167010348737, 281.7050662241970826, -17.43131506460443703 ) ) ;
#82292=CARTESIAN_POINT ( 'NONE',  ( 164.9971748156432056, 244.8635054444190757, -1.825016704039769788 ) ) ;
#82293=EDGE_CURVE ( 'NONE', #57499, #64644, #83066, .T. ) ;
#82294=CARTESIAN_POINT ( 'NONE',  ( 31.54184116921283376, 189.0177522451418497, -10.00000000000009592 ) ) ;
#82295=CARTESIAN_POINT ( 'NONE',  ( 109.2943373587434195, 246.1589784336661069, -6.496448406907676862E-16 ) ) ;
#82296=CARTESIAN_POINT ( 'NONE',  ( 181.7371966266162815, 294.7030870310439923, -2.651400403382340176 ) ) ;
#82297=CARTESIAN_POINT ( 'NONE',  ( 165.5402849709041959, 280.7227082719551277, -11.05355863872715361 ) ) ;
#82298=B_SPLINE_CURVE_WITH_KNOTS ( 'NONE', 3,
 ( #17501, #79847, #48405, #10413 ),
 .UNSPECIFIED., .F., .F.,
 ( 4, 4 ),
 ( 0.02996210580220542985, 0.03907057961704281379 ),
 .UNSPECIFIED. ) ;
#82299=CARTESIAN_POINT ( 'NONE',  ( 195.8248271798537417, 291.4684452715354155, 17.35175160929494709 ) ) ;
#82300=CARTESIAN_POINT ( 'NONE',  ( 163.1685298068643988, 248.0308115086310465, 10.61953511350444046 ) ) ;
#82301=CARTESIAN_POINT ( 'NONE',  ( 32.38097682878547090, 183.3768266524159856, 9.188101187500098632 ) ) ;
#82305=CARTESIAN_POINT ( 'NONE',  ( 9.911560002841389050, 164.9824982072973967, 3.021315404115420679E-15 ) ) ;
#82307=CARTESIAN_POINT ( 'NONE',  ( 29.80979036164399432, 178.0177522451417929, 5.000000000000051514 ) ) ;
#82308=CARTESIAN_POINT ( 'NONE',  ( 146.9324727656309335, 276.1524872186338371, 3.813717745456558728 ) ) ;
#82310=CARTESIAN_POINT ( 'NONE',  ( 161.2133744761260061, 251.4172398781588811, -14.30368667312104058 ) ) ;
#82313=CARTESIAN_POINT ( 'NONE',  ( 99.16399144804778132, 221.3927522451417929, -10.00000000000009059 ) ) ;
#82315=ORIENTED_EDGE ( 'NONE', *, *, #8906, .T. ) ;
#82316=CARTESIAN_POINT ( 'NONE',  ( 196.8199239667486609, 267.3837811503672697, -7.829876893548646244 ) ) ;
#82318=CARTESIAN_POINT ( 'NONE',  ( 202.5511585997265911, 279.8180975037686835, 17.12781264818056925 ) ) ;
#82319=CARTESIAN_POINT ( 'NONE',  ( 163.0424334805279045, 248.2492167524936804, -9.671494865076915914 ) ) ;
#82321=EDGE_CURVE ( 'NONE', #29501, #44538, #12033, .T. ) ;
#82322=CARTESIAN_POINT ( 'NONE',  ( 14.59995888762994554, 188.4244531367911293, -4.594050593750046652 ) ) ;
#82323=AXIS2_PLACEMENT_3D ( 'NONE', #40795, #77835, #85469 ) ;
#82328=CARTESIAN_POINT ( 'NONE',  ( 51.75829523846228852, 194.5643266524159856, -9.188101187500093303 ) ) ;
#82334=CARTESIAN_POINT ( 'NONE',  ( -6.833909532437232315, 176.8615022471903160, 5.000000000000046185 ) ) ;
#82335=B_SPLINE_CURVE_WITH_KNOTS ( 'NONE', 3,
 ( #2653, #47719, #9760, #48237, #85809, #33544, #86797, #86298, #78656, #64440, #25954, #32542, #87319, #95399, #48753, #17332, #63441, #40117, #49243, #71057, #40620, #56826, #87812, #70026, #1658, #80180, #94376, #71557, #70531, #54826, #33033, #79182, #24930, #2154, #55804, #63932, #641, #94871, #31522, #62415, #39610, #25433, #93376, #56324, #1148, #17851, #79685, #23928, #47234, #78152, #93884, #8739, #32023, #62932 ),
 .UNSPECIFIED., .F., .F.,
 ( 4, 2, 2, 2, 2, 2, 2, 2, 2, 2, 2, 2, 2, 2, 2, 2, 2, 2, 2, 2, 2, 2, 2, 2, 2, 2, 4 ),
 ( 0.0003929596557535101030, 0.0008568129670863414366, 0.001088739622752727667, 0.001320666278419114006, 0.001436629606252273024, 0.001552592934085432041, 0.001668556261918591058, 0.001784519589751749858, 0.002016446245418110177, 0.002248372901084470712, 0.002712226212417150582, 0.003176079523749829586, 0.004103786146415284303, 0.005031492769080740321, 0.005495346080413547260, 0.005727272736079950730, 0.005843236063913116035, 0.005901217727829699555, 0.005959199391746281341, 0.006017181055662863126, 0.006075162719579446646, 0.006191126047412610217, 0.006423052703078795111, 0.006886906014411166635, 0.007350759325743539893, 0.007582685981409723053, 0.007814612637075906212 ),
 .UNSPECIFIED. ) ;
#82337=CARTESIAN_POINT ( 'NONE',  ( 132.9753269110629503, 238.3923013555409796, 4.594050593750050204 ) ) ;
#82339=CARTESIAN_POINT ( 'NONE',  ( 207.5409781303276588, 271.1754765561682348, -7.231270017877110767 ) ) ;
#82343=CARTESIAN_POINT ( 'NONE',  ( 189.4247981172279367, 289.8473999775135894, 14.52074419908731961 ) ) ;
#82346=CARTESIAN_POINT ( 'NONE',  ( 150.8757650385446993, 269.3225046528533539, 14.31332712971473953 ) ) ;
#82347=CARTESIAN_POINT ( 'NONE',  ( 208.2570380151932170, 269.9352244543189272, -0.4063029386674604782 ) ) ;
#82348=CARTESIAN_POINT ( 'NONE',  ( 151.3417120142295289, 269.1063531457227214, -14.26574085409202652 ) ) ;
#82349=CARTESIAN_POINT ( 'NONE',  ( 166.7436140395748225, 253.3389855339687244, 13.27779792997078090 ) ) ;
#82350=CARTESIAN_POINT ( 'NONE',  ( 197.2826717042014479, 273.3494898236381800, -13.53960516259263613 ) ) ;
#82352=ORIENTED_EDGE ( 'NONE', *, *, #49866, .F. ) ;
#82356=CARTESIAN_POINT ( 'NONE',  ( 193.1030321335636586, 294.1827325794992021, -14.54662778306917481 ) ) ;
#82357=CARTESIAN_POINT ( 'NONE',  ( 181.8573685214958573, 295.1748175033092139, 4.857304733903339944 ) ) ;
#82363=CARTESIAN_POINT ( 'NONE',  ( 192.0177730709008301, 287.5582357824112023, -16.95470262859629784 ) ) ;
#82367=CARTESIAN_POINT ( 'NONE',  ( 159.7028767715829929, 264.1383856807740358, -17.65718168856439618 ) ) ;
#82368=ORIENTED_EDGE ( 'NONE', *, *, #98027, .F. ) ;
#82369=CARTESIAN_POINT ( 'NONE',  ( 191.7934382699952494, 298.4510156884799699, -8.680100145728863126 ) ) ;
#82370=CARTESIAN_POINT ( 'NONE',  ( 204.7444193837539501, 273.0031821285110709, -9.756915323793542427 ) ) ;
#82371=CARTESIAN_POINT ( 'NONE',  ( 164.2851776226980860, 246.0967207574460929, 5.847738044744511754 ) ) ;
#82374=ORIENTED_EDGE ( 'NONE', *, *, #61776, .F. ) ;
#82375=CARTESIAN_POINT ( 'NONE',  ( 85.85769841670955316, 226.5024278399160949, -9.188101187500093303 ) ) ;
#82376=CARTESIAN_POINT ( 'NONE',  ( 155.0271965705274795, 262.1320143153159847, 17.46223432386462093 ) ) ;
#82377=CARTESIAN_POINT ( 'NONE',  ( 181.2624089752565624, 271.4720694466574287, -17.37114438570441521 ) ) ;
#82378=CARTESIAN_POINT ( 'NONE',  ( 181.8338920363375735, 257.2967203629509072, -6.061067647267480929 ) ) ;
#82381=ADVANCED_FACE ( 'NONE', ( #34663 ), #12380, .T. ) ;
#82383=ORIENTED_EDGE ( 'NONE', *, *, #94225, .F. ) ;
#82385=ORIENTED_EDGE ( 'NONE', *, *, #5103, .T. ) ;
#82386=EDGE_CURVE ( 'NONE', #36946, #4581, #95221, .T. ) ;
#82388=CARTESIAN_POINT ( 'NONE',  ( 155.2922060645262263, 261.6730044072216401, -16.98884022075611355 ) ) ;
#82390=CARTESIAN_POINT ( 'NONE',  ( 164.8768953149048286, 245.0718356508067188, 2.399905317103016689 ) ) ;
#82392=ADVANCED_FACE ( 'NONE', ( #91896 ), #70952, .F. ) ;
#82393=AXIS2_PLACEMENT_3D ( 'NONE', #80111, #56252, #1587 ) ;
#82394=CARTESIAN_POINT ( 'NONE',  ( 201.0732166862245549, 282.3779679885897167, -18.18766936363638820 ) ) ;
#82395=ADVANCED_FACE ( 'NONE', ( #63449 ), #40186, .F. ) ;
#82396=CARTESIAN_POINT ( 'NONE',  ( 148.1829914015846157, 273.9865254053503349, -9.304102644963160529 ) ) ;
#82398=CARTESIAN_POINT ( 'NONE',  ( 157.5735440838707007, 281.7061173120971489, 2.965151850968649416 ) ) ;
#82399=CARTESIAN_POINT ( 'NONE',  ( 168.3667151233534014, 267.2158819435744590, -17.25990780505111744 ) ) ;
#82404=ORIENTED_EDGE ( 'NONE', *, *, #81130, .T. ) ;
#82405=CARTESIAN_POINT ( 'NONE',  ( 167.2558879808692609, 284.3031459148808722, 9.343441084002181540 ) ) ;
#82407=CARTESIAN_POINT ( 'NONE',  ( 168.2356071464602962, 248.8554872198452301, 6.669745218284529820 ) ) ;
#82409=CARTESIAN_POINT ( 'NONE',  ( -3.441976700948170542, 175.4865022471903160, -10.00000000000009592 ) ) ;
#82411=CARTESIAN_POINT ( 'NONE',  ( 188.3691292746556769, 260.5545915045569245, 2.351640140481156216 ) ) ;
#82412=CARTESIAN_POINT ( 'NONE',  ( 160.7870188850188526, 282.4993610488249942, -6.291640665936681032 ) ) ;
#82414=CARTESIAN_POINT ( 'NONE',  ( 157.4627203480516755, 258.4629190429250798, 16.86169483958236626 ) ) ;
#82418=VERTEX_POINT ( 'NONE', #10256 ) ;
#82419=CARTESIAN_POINT ( 'NONE',  ( 181.5093725072136976, 271.2422899577236421, -15.97233562208454138 ) ) ;
#82421=ORIENTED_EDGE ( 'NONE', *, *, #54175, .T. ) ;
#82422=CARTESIAN_POINT ( 'NONE',  ( 158.4995706392118393, 280.6444534788661258, 8.122523594373102895 ) ) ;
#82424=CARTESIAN_POINT ( 'NONE',  ( 164.1107196200280782, 246.3988908818576249, -7.889078953360578517 ) ) ;
#82425=CARTESIAN_POINT ( 'NONE',  ( 191.4420812244453600, 260.8157448279923187, -1.331758356259544085 ) ) ;
#82426=CARTESIAN_POINT ( 'NONE',  ( 164.8178548836487778, 274.1146863845406187, 15.79208962134384642 ) ) ;
#82427=CARTESIAN_POINT ( 'NONE',  ( -5.399728507075681527, 173.8149278399160949, -9.188101187500095079 ) ) ;
#82430=CARTESIAN_POINT ( 'NONE',  ( 203.3947719899915683, 270.0274960689384898, 5.925299578284906055 ) ) ;
#82433=ORIENTED_EDGE ( 'NONE', *, *, #63334, .F. ) ;
#82435=CARTESIAN_POINT ( 'NONE',  ( 189.9728169475564528, 273.9113149598638870, -15.63390733120380638 ) ) ;
#82436=B_SPLINE_CURVE_WITH_KNOTS ( 'NONE', 3,
 ( #36561, #20899, #7155, #83205 ),
 .UNSPECIFIED., .F., .F.,
 ( 4, 4 ),
 ( 0.000000000000000000, 0.003361958963760078647 ),
 .UNSPECIFIED. ) ;
#82438=CARTESIAN_POINT ( 'NONE',  ( 175.4168235025557578, 290.8539856576853708, 2.566641252103732285 ) ) ;
#82439=CARTESIAN_POINT ( 'NONE',  ( 153.4389798490260262, 264.8828863703868137, 16.68923469758090761 ) ) ;
#82441=CARTESIAN_POINT ( 'NONE',  ( 193.8003511027313550, 288.1208047801705447, 17.19107869180001913 ) ) ;
#82442=CARTESIAN_POINT ( 'NONE',  ( 11.65032017781297036, 177.5333772461660544, 9.188101187500095079 ) ) ;
#82443=CARTESIAN_POINT ( 'NONE',  ( 103.0163473728362504, 218.0327760586659451, 1.948934522072303157E-15 ) ) ;
#82445=CARTESIAN_POINT ( 'NONE',  ( 180.4917861999344950, 255.8997540221662916, -2.348914290984229325 ) ) ;
#82447=CARTESIAN_POINT ( 'NONE',  ( 178.2349067178215307, 283.5087980138422381, -14.56972715175360733 ) ) ;
#82451=CARTESIAN_POINT ( 'NONE',  ( 180.8580557430661315, 273.1824778245191396, 17.46595093170893520 ) ) ;
#82452=CARTESIAN_POINT ( 'NONE',  ( 194.9757425430702824, 292.9391030023704161, -15.21392314336593365 ) ) ;
#82453=B_SPLINE_CURVE_WITH_KNOTS ( 'NONE', 3,
 ( #4418, #89573, #36308, #75839, #97163, #66226, #27728, #59088, #59595, #5918, #50510, #12534, #52019, #21623, #6426, #20631, #51514, #42889, #43905, #74845, #90572, #83452, #20135, #36807, #67719, #98643, #5425, #29226, #58598, #89097, #43406, #74351, #4939, #28721, #60094, #66711 ),
 .UNSPECIFIED., .F., .F.,
 ( 4, 2, 2, 2, 2, 2, 2, 2, 2, 2, 2, 2, 2, 2, 2, 2, 2, 4 ),
 ( 0.0009418892082754573266, 0.001034195886821434552, 0.001126502565367411886, 0.001311115922459314947, 0.001680342636643120851, 0.002418796065010804866, 0.003895702921746029782, 0.004634156350113681488, 0.005003383064297432098, 0.005372609778481181840, 0.005418763117754132885, 0.005464916457027083063, 0.005511069796300034108, 0.005557223135572984286, 0.005741836492664717344, 0.006111063206848219888, 0.006480289921031722432, 0.006849516635215224108 ),
 .UNSPECIFIED. ) ;
#82455=CARTESIAN_POINT ( 'NONE',  ( 193.6585565783151424, 265.7726264491872143, 7.804970366182538477 ) ) ;
#82457=CARTESIAN_POINT ( 'NONE',  ( 162.3075208383741312, 251.8437974874645420, -12.94720210134591376 ) ) ;
#82459=CARTESIAN_POINT ( 'NONE',  ( 175.7396758166374013, 265.4884659434268883, -15.79124167090947850 ) ) ;
#82460=EDGE_CURVE ( 'NONE', #3492, #79294, #30983, .T. ) ;
#82461=CARTESIAN_POINT ( 'NONE',  ( 75.84410613756948294, 226.8464784336661353, 1.353441290958777327E-15 ) ) ;
#82464=AXIS2_PLACEMENT_3D ( 'NONE', #3433, #57593, #87081 ) ;
#82465=CARTESIAN_POINT ( 'NONE',  ( 159.0966864002964769, 259.3073909472009291, -17.37488020174250636 ) ) ;
#82466=CARTESIAN_POINT ( 'NONE',  ( 157.1135969804030310, 258.5182628004787944, 17.19660297500358226 ) ) ;
#82469=CARTESIAN_POINT ( 'NONE',  ( 204.5540905216327303, 275.9620748824726775, -12.79967422555914958 ) ) ;
#82471=CARTESIAN_POINT ( 'NONE',  ( 147.0456760057551833, 275.9564134551570760, -3.678503029046952033 ) ) ;
#82473=VERTEX_POINT ( 'NONE', #10756 ) ;
#82476=CARTESIAN_POINT ( 'NONE',  ( 192.9633865298379476, 296.4246058602058156, -11.85717392250713864 ) ) ;
#82479=CARTESIAN_POINT ( 'NONE',  ( 198.5612432604688991, 286.7288335892616260, 18.30793681285053509 ) ) ;
#82480=CARTESIAN_POINT ( 'NONE',  ( 183.8210692855788864, 257.9504670327482927, 6.873620218444065344 ) ) ;
#82483=CARTESIAN_POINT ( 'NONE',  ( 139.4522149234842061, 257.9865022471903444, -10.00000000000009415 ) ) ;
#82484=( BOUNDED_CURVE ( )  B_SPLINE_CURVE ( 2, ( #99208, #85024, #15568, #46471, #62168, #23669, #46992, #77401, #69783 ),
 .UNSPECIFIED., .F., .T. ) 
 B_SPLINE_CURVE_WITH_KNOTS ( ( 3, 2, 2, 2, 3 ),
 ( 0.4233870967741935609, 0.4247311827956989361, 0.4274193548387096864, 0.4301075268817204367, 0.4314516129032258118 ),
 .UNSPECIFIED. ) 
 CURVE ( )  GEOMETRIC_REPRESENTATION_ITEM ( )  RATIONAL_B_SPLINE_CURVE ( ( 0.9330127018922194093, 0.9330127018922194093, 1.000000000000000000, 0.8660254037844387076, 1.000000000000000000, 0.8660254037844387076, 1.000000000000000000, 0.9330127018922194093, 0.9330127018922194093 ) ) 
 REPRESENTATION_ITEM ( '' )  );
#82488=B_SPLINE_SURFACE_WITH_KNOTS ( 'NONE', 3, 1, ( 
 ( #13676, #50663 ),
 ( #43047, #12187 ),
 ( #71630, #2225 ),
 ( #45052, #75476 ),
 ( #75992, #67866 ),
 ( #21757, #77474 ),
 ( #8068, #7053 ),
 ( #53642, #6061 ),
 ( #23244, #6569 ),
 ( #30359, #45541 ),
 ( #29860, #30859 ),
 ( #84597, #15135 ),
 ( #46032, #76949 ),
 ( #37442, #7549 ),
 ( #60730, #54131 ),
 ( #61744, #38441 ),
 ( #31351, #83599 ),
 ( #98788, #92693 ),
 ( #85094, #15640 ),
 ( #84113, #46537 ),
 ( #69355, #38943 ),
 ( #61244, #91197 ),
 ( #36955, #99768 ),
 ( #52644, #29370 ),
 ( #14165, #69848 ),
 ( #461, #14665 ),
 ( #60236, #92210 ),
 ( #62234, #37934 ),
 ( #100274, #76473 ),
 ( #93186, #22765 ),
 ( #23741, #68352 ),
 ( #68847, #54635 ),
 ( #85614, #16157 ),
 ( #22255, #99277 ) ),
 .UNSPECIFIED., .T., .F., .F.,
 ( 4, 2, 2, 2, 2, 2, 2, 2, 2, 2, 2, 2, 2, 2, 2, 2, 4 ),
 ( 2, 2 ),
 ( 0.000000000000000000, 0.06250000000000000000, 0.1250000000000000000, 0.1875000000000000000, 0.2500000000000000000, 0.3125000000000000000, 0.3750000000000000000, 0.4375000000000000000, 0.5000000000000000000, 0.5625000000000000000, 0.6250000000000000000, 0.6875000000000000000, 0.7500000000000000000, 0.8125000000000000000, 0.8750000000000000000, 0.9375000000000000000, 1.000000000000000000 ),
 ( 0.000000000000000000, 1.000000000000000000 ),
 .UNSPECIFIED. ) ;
#82492=CARTESIAN_POINT ( 'NONE',  ( 184.1800646242121786, 291.9084716066498686, -10.70019971855618834 ) ) ;
#82493=ORIENTED_EDGE ( 'NONE', *, *, #84418, .F. ) ;
#82495=CARTESIAN_POINT ( 'NONE',  ( 194.1714003930522949, 280.7953645453140439, -17.43791269142986877 ) ) ;
#82497=CARTESIAN_POINT ( 'NONE',  ( 153.4361244163197000, 264.8878321249116539, -17.23169627811277493 ) ) ;
#82501=ADVANCED_FACE ( 'NONE', ( #49744 ), #28785, .F. ) ;
#82502=CARTESIAN_POINT ( 'NONE',  ( 164.6328405706842943, 274.5024593735440135, 14.72560760841240679 ) ) ;
#82506=ORIENTED_EDGE ( 'NONE', *, *, #89498, .T. ) ;
#82507=CARTESIAN_POINT ( 'NONE',  ( 182.8497346172418077, 296.2091331152387852, 0.3117783270952969032 ) ) ;
#82508=CARTESIAN_POINT ( 'NONE',  ( 204.9004517216375518, 275.7490024547470853, 14.55104398969427670 ) ) ;
#82514=CARTESIAN_POINT ( 'NONE',  ( 171.0161179014379798, 287.7422477288193932, -4.570675186747868324 ) ) ;
#82517=DIRECTION ( 'NONE',  ( -0.4999999999999987788, 0.8660254037844392627, 0.000000000000000000 ) ) ;
#82518=CARTESIAN_POINT ( 'NONE',  ( 107.1028179730028285, 223.4548013555409796, -4.594050593750042211 ) ) ;
#82519=ORIENTED_EDGE ( 'NONE', *, *, #91733, .F. ) ;
#82520=CARTESIAN_POINT ( 'NONE',  ( -0.4807448425718762741, 158.9824982072973683, 3.021315404115420679E-15 ) ) ;
#82521=CARTESIAN_POINT ( 'NONE',  ( 179.4404154152157105, 291.3709498135804097, -10.08759257512885199 ) ) ;
#82523=ORIENTED_EDGE ( 'NONE', *, *, #36387, .T. ) ;
#82525=CYLINDRICAL_SURFACE ( 'NONE', #68948, 17.82106496071139645 ) ;
#82526=CARTESIAN_POINT ( 'NONE',  ( 157.2464636617698375, 258.2881309577184652, 18.14284729738657731 ) ) ;
#82527=CARTESIAN_POINT ( 'NONE',  ( 206.2809287719926488, 273.3579460648492159, -10.70911012174624588 ) ) ;
#82531=CARTESIAN_POINT ( 'NONE',  ( -17.42236680055705023, 149.2012482093457777, 0.000000000000000000 ) ) ;
#82532=VERTEX_POINT ( 'NONE', #85170 ) ;
#82534=CARTESIAN_POINT ( 'NONE',  ( 191.7168775847123641, 264.3120571150079172, -7.888889122128393439 ) ) ;
#82535=FACE_OUTER_BOUND ( 'NONE', #43313, .T. ) ;
#82537=CARTESIAN_POINT ( 'NONE',  ( 141.5001777056247931, 246.3768266524160140, 9.188101187500098632 ) ) ;
#82539=CYLINDRICAL_SURFACE ( 'NONE', #57563, 2.471954595299370006 ) ;
#82540=ORIENTED_EDGE ( 'NONE', *, *, #43566, .F. ) ;
#82541=CARTESIAN_POINT ( 'NONE',  ( 190.3791419447713906, 300.9006487807255326, -5.688668718458480988 ) ) ;
#82544=CARTESIAN_POINT ( 'NONE',  ( 192.8798198427039665, 270.9848878250640496, 14.54342281811944027 ) ) ;
#82545=CARTESIAN_POINT ( 'NONE',  ( 178.2267749612124135, 285.2995087623953623, 13.03308732619244736 ) ) ;
#82547=CARTESIAN_POINT ( 'NONE',  ( 198.7849384794873231, 282.4363158398074916, -17.34911472281661204 ) ) ;
#82551=CARTESIAN_POINT ( 'NONE',  ( 60.95981515367195414, 199.8768266524160140, 9.188101187500098632 ) ) ;
#82552=LINE ( 'NONE', #53576, #54083 ) ;
#82554=CARTESIAN_POINT ( 'NONE',  ( 162.8480293090835005, 248.5859346546387769, -9.753154585358942086 ) ) ;
#82555=B_SPLINE_CURVE_WITH_KNOTS ( 'NONE', 3,
 ( #20786, #34960, #5078, #65860 ),
 .UNSPECIFIED., .F., .F.,
 ( 4, 4 ),
 ( 0.008944368131606707586, 0.01511703026669370883 ),
 .UNSPECIFIED. ) ;
#82556=CARTESIAN_POINT ( 'NONE',  ( 196.3345161992979229, 288.9417725351840431, -17.15029287748203757 ) ) ;
#82561=CARTESIAN_POINT ( 'NONE',  ( 174.3943357370370677, 284.3386801424128976, 13.92617907230369312 ) ) ;
#82562=ADVANCED_FACE ( 'NONE', ( #24821 ), #16229, .T. ) ;
#82564=CARTESIAN_POINT ( 'NONE',  ( 149.9060791885465846, 273.0020498124315509, -11.57482514211843849 ) ) ;
#82565=CARTESIAN_POINT ( 'NONE',  ( 195.9713281756800427, 291.2146981034049418, 17.52210387885178022 ) ) ;
#82567=CARTESIAN_POINT ( 'NONE',  ( 20.20266813594930611, 170.2202760586659736, -5.415160957724236172E-17 ) ) ;
#82568=CARTESIAN_POINT ( 'NONE',  ( 48.66388509341562241, 192.2365022471902023, -10.00000000000009237 ) ) ;
#82571=CARTESIAN_POINT ( 'NONE',  ( 196.3341081413628899, 290.5863447708742342, 16.12390540996472410 ) ) ;
#82572=CARTESIAN_POINT ( 'NONE',  ( 199.3468182655126100, 277.7844241296513701, 15.39279173571824266 ) ) ;
#82573=CYLINDRICAL_SURFACE ( 'NONE', #38597, 10.00000000000010658 ) ;
#82575=CARTESIAN_POINT ( 'NONE',  ( 42.23166870106845039, 201.3149278399161233, 9.188101187500093303 ) ) ;
#82577=CARTESIAN_POINT ( 'NONE',  ( 199.1944722252943905, 285.6320488493591938, -18.17555833707144686 ) ) ;
#82578=CARTESIAN_POINT ( 'NONE',  ( 190.1607982559816890, 301.2788311432216233, -4.972636536415983244 ) ) ;
#82580=CARTESIAN_POINT ( 'NONE',  ( 199.7244443182572979, 267.8419476567416950, -6.547629676957067879 ) ) ;
#82581=CARTESIAN_POINT ( 'NONE',  ( 193.6881582770097054, 289.9360790452486754, 16.66172979718519898 ) ) ;
#82582=CARTESIAN_POINT ( 'NONE',  ( 176.9920332807921568, 275.4403497717407276, 17.58608646401103215 ) ) ;
#82583=DIRECTION ( 'NONE',  ( 0.4999999999999998890, -0.8660254037844385966, 0.000000000000000000 ) ) ;
#82585=CARTESIAN_POINT ( 'NONE',  ( 163.3377027424940025, 255.8893630163459534, -14.85816214141254576 ) ) ;
#82586=EDGE_CURVE ( 'NONE', #59744, #50323, #3327, .T. ) ;
#82587=CARTESIAN_POINT ( 'NONE',  ( -13.76211276271269668, 162.8615022471902591, 0.000000000000000000 ) ) ;
#82588=CARTESIAN_POINT ( 'NONE',  ( 104.9555363394041336, 224.7365022471902307, 10.00000000000009592 ) ) ;
#82589=CARTESIAN_POINT ( 'NONE',  ( 200.1102648775588193, 284.0458494464393198, 17.54251420653697835 ) ) ;
#82590=CARTESIAN_POINT ( 'NONE',  ( 164.9127185089346028, 270.4126442277538445, -16.66829531255166330 ) ) ;
#82592=CARTESIAN_POINT ( 'NONE',  ( 54.35602435405059651, 208.3149278399161233, -9.188101187500095079 ) ) ;
#82594=CARTESIAN_POINT ( 'NONE',  ( -22.42236680055709641, 157.8615022471902591, 0.000000000000000000 ) ) ;
#82595=CARTESIAN_POINT ( 'NONE',  ( 175.0296968597178306, 264.6864531019056699, -16.70299667166197466 ) ) ;
#82598=ORIENTED_EDGE ( 'NONE', *, *, #38829, .F. ) ;
#82601=CARTESIAN_POINT ( 'NONE',  ( 155.7716105177659927, 262.8426515368366267, -17.72795275872529430 ) ) ;
#82603=CARTESIAN_POINT ( 'NONE',  ( 189.3285837834738174, 265.1763588534336122, 10.46335708403672626 ) ) ;
#82604=CARTESIAN_POINT ( 'NONE',  ( 196.2421909983451940, 290.7455499326673021, -17.31908925000307065 ) ) ;
#82605=CARTESIAN_POINT ( 'NONE',  ( 157.2014865449050660, 258.3660336093062142, 16.87758714513496017 ) ) ;
#82611=ADVANCED_FACE ( 'NONE', ( #46615 ), #76542, .T. ) ;
#82612=EDGE_CURVE ( 'NONE', #50052, #20654, #90371, .T. ) ;
#82615=CARTESIAN_POINT ( 'NONE',  ( 166.9403103669216648, 261.3810178180994512, 16.77684693550508754 ) ) ;
#82616=CARTESIAN_POINT ( 'NONE',  ( 206.7893622945242385, 272.4773133715531230, -10.52881283832460291 ) ) ;
#82618=ORIENTED_EDGE ( 'NONE', *, *, #23026, .F. ) ;
#82625=CARTESIAN_POINT ( 'NONE',  ( 159.2554912534056939, 254.8083930951974878, 16.49944922174842432 ) ) ;
#82626=CYLINDRICAL_SURFACE ( 'NONE', #43491, 10.00000000000010658 ) ;
#82627=CARTESIAN_POINT ( 'NONE',  ( 164.5858729372050675, 265.2716139154605344, -16.65117712114545512 ) ) ;
#82628=CARTESIAN_POINT ( 'NONE',  ( 124.8288415870092791, 249.0024278399161517, -9.188101187500093303 ) ) ;
#82630=CARTESIAN_POINT ( 'NONE',  ( 114.3374782137354799, 243.4865022471903160, 10.00000000000009415 ) ) ;
#82631=ORIENTED_EDGE ( 'NONE', *, *, #5964, .F. ) ;
#82632=CARTESIAN_POINT ( 'NONE',  ( 174.0587387296342854, 265.5211078058665066, 16.69357511762551383 ) ) ;
#82634=CARTESIAN_POINT ( 'NONE',  ( 36.00834752015899198, 180.0494855054051868, -2.679491924311248496 ) ) ;
#82636=CARTESIAN_POINT ( 'NONE',  ( 160.4722622339176041, 253.9870023085891830, 15.41922939303313811 ) ) ;
#82640=CARTESIAN_POINT ( 'NONE',  ( 159.9628729326222754, 253.5831720864507588, 15.75051413866357386 ) ) ;
#82643=CARTESIAN_POINT ( 'NONE',  ( 68.80799682758592439, 210.5333772461660544, 9.188101187500095079 ) ) ;
#82645=CARTESIAN_POINT ( 'NONE',  ( 176.9376637958658591, 282.2927093116995820, 15.89557571866741981 ) ) ;
#82646=CARTESIAN_POINT ( 'NONE',  ( 154.9344967692067598, 262.2925750810547356, 17.30210568643136781 ) ) ;
#82647=CARTESIAN_POINT ( 'NONE',  ( 175.7384777704949386, 278.2480916999407441, 15.65549428786727759 ) ) ;
#82651=CARTESIAN_POINT ( 'NONE',  ( 201.2949053258274148, 281.9939920013367782, -18.04004790210578335 ) ) ;
#82652=CARTESIAN_POINT ( 'NONE',  ( 203.5629025532486196, 278.0657055720176913, -15.85226727704602823 ) ) ;
#82658=CARTESIAN_POINT ( 'NONE',  ( 206.0691053506789387, 273.7248349927971844, 11.70564474658248422 ) ) ;
#82659=CARTESIAN_POINT ( 'NONE',  ( 163.7183543885751078, 247.0784873978576854, -6.786164904910574336 ) ) ;
#82660=CARTESIAN_POINT ( 'NONE',  ( 139.7141738582018604, 239.2202760586659736, -5.415160957724236172E-17 ) ) ;
#82665=B_SPLINE_CURVE_WITH_KNOTS ( 'NONE', 3,
 ( #62366, #99411, #45671, #61380 ),
 .UNSPECIFIED., .F., .F.,
 ( 4, 4 ),
 ( 0.01147170345886797983, 0.01992442707605523305 ),
 .UNSPECIFIED. ) ;
#82667=CYLINDRICAL_SURFACE ( 'NONE', #56315, 17.82106496071139645 ) ;
#82671=CARTESIAN_POINT ( 'NONE',  ( 182.2980163133740064, 275.2725943275962095, -16.61995625180471592 ) ) ;
#82672=CARTESIAN_POINT ( 'NONE',  ( 159.9950753608005130, 276.8117990079294373, 13.35014033362692487 ) ) ;
#82675=CARTESIAN_POINT ( 'NONE',  ( 146.8201187048455267, 276.3470901603510015, 4.112223577763169047 ) ) ;
#82676=B_SPLINE_CURVE_WITH_KNOTS ( 'NONE', 3,
 ( #65998, #96950, #60858, #61371, #84721, #91 ),
 .UNSPECIFIED., .F., .F.,
 ( 4, 2, 4 ),
 ( 0.02038262341263210459, 0.02494425553470808188, 0.02950588765678405917 ),
 .UNSPECIFIED. ) ;
#82677=CARTESIAN_POINT ( 'NONE',  ( 182.9080384886626973, 280.6966867911361305, 16.99481542840181092 ) ) ;
#82678=CARTESIAN_POINT ( 'NONE',  ( 157.2777284163744582, 258.2339788142568864, -16.82360006463426316 ) ) ;
#82684=CARTESIAN_POINT ( 'NONE',  ( 159.9880386575927957, 253.5395837721924863, 15.85893018594752846 ) ) ;
#82685=CARTESIAN_POINT ( 'NONE',  ( 175.4039180538638050, 286.4985578832265105, -12.71199677751706503 ) ) ;
#82686=CARTESIAN_POINT ( 'NONE',  ( 130.2687372006388671, 246.0177522451418497, -10.00000000000009592 ) ) ;
#82687=CARTESIAN_POINT ( 'NONE',  ( 173.8366476056167755, 284.1819771225056002, -12.13474973978462579 ) ) ;
#82688=ORIENTED_EDGE ( 'NONE', *, *, #65463, .T. ) ;
#82691=CARTESIAN_POINT ( 'NONE',  ( 151.1699610800269511, 268.8129421616204695, -14.28929860221299286 ) ) ;
#82692=CARTESIAN_POINT ( 'NONE',  ( 15.22267496842377099, 179.5958772461660544, -9.188101187500095079 ) ) ;
#82693=CARTESIAN_POINT ( 'NONE',  ( 178.6505616879398985, 259.2469067511012213, -10.41651906039837527 ) ) ;
#82696=CARTESIAN_POINT ( 'NONE',  ( 204.6075833744878878, 276.2562653119390461, -13.34672481898815910 ) ) ;
#82699=CARTESIAN_POINT ( 'NONE',  ( 170.9894030905899456, 257.8110510375899480, 14.60046632396432109 ) ) ;
#82700=CARTESIAN_POINT ( 'NONE',  ( 178.8651605570578624, 254.1428845745818990, -4.151848116954283796 ) ) ;
#82702=CARTESIAN_POINT ( 'NONE',  ( 150.2950809960438221, 270.3282789176094525, 14.12607625385173193 ) ) ;
#82704=CARTESIAN_POINT ( 'NONE',  ( 47.29267820409018697, 208.1115022471903160, -5.000000000000047962 ) ) ;
#82705=CARTESIAN_POINT ( 'NONE',  ( 181.6690914948270574, 291.8339887612885946, 9.074948012314465018 ) ) ;
#82706=CARTESIAN_POINT ( 'NONE',  ( 148.0389988358468827, 274.2359278451201590, 7.783622668412842671 ) ) ;
#82707=CARTESIAN_POINT ( 'NONE',  ( 22.47598482088346117, 171.5327760586659451, 1.948934522072303157E-15 ) ) ;
#82708=CARTESIAN_POINT ( 'NONE',  ( 168.0427418980721939, 286.7126107662992922, 5.006243472136755912 ) ) ;
#82712=CARTESIAN_POINT ( 'NONE',  ( 179.8149668105232877, 276.9306161883004052, 16.29941506102614923 ) ) ;
#82713=CARTESIAN_POINT ( 'NONE',  ( 188.0775634319173832, 267.1413101313072502, 14.31780989748781252 ) ) ;
#82715=CARTESIAN_POINT ( 'NONE',  ( 164.1509177496182588, 281.5495894003347530, 8.939607256454412010 ) ) ;
#82721=CARTESIAN_POINT ( 'NONE',  ( 194.1493756275458793, 294.3704124857528655, 13.94613522129020744 ) ) ;
#82722=ORIENTED_EDGE ( 'NONE', *, *, #27823, .F. ) ;
#82723=DIRECTION ( 'NONE',  ( -0.8660254037844387076, -0.4999999999999998890, -0.000000000000000000 ) ) ;
#82724=CARTESIAN_POINT ( 'NONE',  ( 156.9346906984713144, 276.3858077937837834, 10.77862339299636574 ) ) ;
#82726=ORIENTED_EDGE ( 'NONE', *, *, #27951, .T. ) ;
#82727=CARTESIAN_POINT ( 'NONE',  ( 195.7705542948037021, 290.3450269424856742, -16.49291066975641229 ) ) ;
#82728=DIRECTION ( 'NONE',  ( -0.8660254037844387076, -0.4999999999999998890, -0.000000000000000000 ) ) ;
#82730=CARTESIAN_POINT ( 'NONE',  ( 155.1865148098964937, 261.8560670301561686, -16.99758927948949605 ) ) ;
#82732=ORIENTED_EDGE ( 'NONE', *, *, #26253, .F. ) ;
#82736=CARTESIAN_POINT ( 'NONE',  ( 152.6845319923753834, 266.1896283897672220, 17.20844521882669653 ) ) ;
#82738=CARTESIAN_POINT ( 'NONE',  ( 191.3638605175971747, 299.1950661814348678, 7.382965314423603154 ) ) ;
#82740=CARTESIAN_POINT ( 'NONE',  ( 162.2281535785777464, 260.3593638863677597, -17.46508937750856560 ) ) ;
#82747=CARTESIAN_POINT ( 'NONE',  ( 206.1932826529868805, 273.5097535960530877, 11.72208607728249241 ) ) ;
#82751=CARTESIAN_POINT ( 'NONE',  ( 177.1951107123421139, 278.9335273702716336, -15.93379266965202312 ) ) ;
#82752=CARTESIAN_POINT ( 'NONE',  ( 168.9995394412663927, 261.3531918911040179, -16.36193740910546168 ) ) ;
#82755=CARTESIAN_POINT ( 'NONE',  ( 192.4867975473904949, 297.2500821921321972, -13.04960750009181325 ) ) ;
#82759=CARTESIAN_POINT ( 'NONE',  ( 155.2084098882724845, 265.7658068242191689, -16.35003261853351830 ) ) ;
#82761=CARTESIAN_POINT ( 'NONE',  ( 188.6795480343751308, 298.6307287810504931, -4.269171661791919092 ) ) ;
#82762=CARTESIAN_POINT ( 'NONE',  ( 190.0259678364800493, 301.5123642802043946, 4.004183174499006626 ) ) ;
#82763=CARTESIAN_POINT ( 'NONE',  ( 157.1241657895010633, 258.9031910183524019, -16.87105681078169894 ) ) ;
#82764=CARTESIAN_POINT ( 'NONE',  ( 146.6805974831222841, 276.5887480051095508, -0.6663123207720742514 ) ) ;
#82765=CARTESIAN_POINT ( 'NONE',  ( 147.2405539530007559, 275.6188749492528132, 0.4306668706573002492 ) ) ;
#82766=ORIENTED_EDGE ( 'NONE', *, *, #69580, .T. ) ;
#82769=CARTESIAN_POINT ( 'NONE',  ( 164.9617201910520237, 244.9249146555742414, 2.745022583679548767 ) ) ;
#82771=CARTESIAN_POINT ( 'NONE',  ( 168.2709212779534482, 286.3625079078701674, 3.948410620585521613 ) ) ;
#82773=CARTESIAN_POINT ( 'NONE',  ( 100.3364738622893810, 237.9244531367911009, -4.594050593750046652 ) ) ;
#82775=CARTESIAN_POINT ( 'NONE',  ( 190.1544783179600415, 301.2897775969759664, -3.447215837936876248 ) ) ;
#82777=CARTESIAN_POINT ( 'NONE',  ( 202.5752970409983220, 279.0574324504058268, 15.43767528721618021 ) ) ;
#82779=CARTESIAN_POINT ( 'NONE',  ( 198.7409601489106592, 286.4175548075023698, -17.25928620176719974 ) ) ;
#82781=VERTEX_POINT ( 'NONE', #76876 ) ;
#82782=CARTESIAN_POINT ( 'NONE',  ( 170.5199279757401598, 255.7150289786715973, -11.87445405841454971 ) ) ;
#82783=( BOUNDED_CURVE ( )  B_SPLINE_CURVE ( 2, ( #44367, #82921, #50973, #90022, #4382, #66189, #59556, #20594, #27702 ),
 .UNSPECIFIED., .F., .T. ) 
 B_SPLINE_CURVE_WITH_KNOTS ( ( 3, 2, 2, 2, 3 ),
 ( 0.3346774193548386900, 0.3360215053763440651, 0.3387096774193548154, 0.3413978494623655657, 0.3427419354838709964 ),
 .UNSPECIFIED. ) 
 CURVE ( )  GEOMETRIC_REPRESENTATION_ITEM ( )  RATIONAL_B_SPLINE_CURVE ( ( 0.9330127018922194093, 0.9330127018922194093, 1.000000000000000000, 0.8660254037844387076, 1.000000000000000000, 0.8660254037844387076, 1.000000000000000000, 0.9330127018922179660, 0.9330127018922194093 ) ) 
 REPRESENTATION_ITEM ( '' )  );
#82785=CARTESIAN_POINT ( 'NONE',  ( 164.8329445879545290, 245.1479605429143760, -2.955380775890217304 ) ) ;
#82787=CARTESIAN_POINT ( 'NONE',  ( 31.61400995286148330, 202.3927522451419350, 2.944929066748280225E-16 ) ) ;
#82788=CARTESIAN_POINT ( 'NONE',  ( 119.3079296378835181, 245.8149278399160949, -9.188101187500095079 ) ) ;
#82789=CARTESIAN_POINT ( 'NONE',  ( 199.0363797504450929, 285.9058730480928716, -17.12190301149298222 ) ) ;
#82790=CARTESIAN_POINT ( 'NONE',  ( 164.1788121382481904, 280.3338528224191464, -11.36002433749857410 ) ) ;
#82792=CARTESIAN_POINT ( 'NONE',  ( 172.3688428511626967, 251.1033656833274677, -4.005216378610661820 ) ) ;
#82793=CARTESIAN_POINT ( 'NONE',  ( 38.76756708593069334, 199.3149278399161233, -9.188101187500095079 ) ) ;
#82796=CARTESIAN_POINT ( 'NONE',  ( -1.387478102835363769, 181.5530062829863596, 2.649461200531984646E-14 ) ) ;
#82797=CARTESIAN_POINT ( 'NONE',  ( 181.8871442283018212, 266.9089101108496038, 15.94309912413098473 ) ) ;
#82801=CARTESIAN_POINT ( 'NONE',  ( 178.6792603332878002, 287.1060177970853715, -12.25702117352004450 ) ) ;
#82802=CARTESIAN_POINT ( 'NONE',  ( 164.2020060191955793, 250.0206628281335668, 10.23082325107943191 ) ) ;
#82803=CARTESIAN_POINT ( 'NONE',  ( 94.76169564547690527, 215.5177522451417929, 5.000000000000051514 ) ) ;
#82805=CARTESIAN_POINT ( 'NONE',  ( 198.7498379103732304, 267.8340533398088610, -8.134651165626271663 ) ) ;
#82807=CARTESIAN_POINT ( 'NONE',  ( 155.1870085809113675, 280.1431070046639320, -2.400648766995867600 ) ) ;
#82808=CARTESIAN_POINT ( 'NONE',  ( 208.1612901671020381, 270.1010645919285480, -2.401583477149568768 ) ) ;
#82809=CARTESIAN_POINT ( 'NONE',  ( 16.06189740016370848, 170.8923013555409796, 4.594050593750050204 ) ) ;
#82811=CARTESIAN_POINT ( 'NONE',  ( 192.2441535563929733, 272.1090697265545373, 14.30193341551846586 ) ) ;
#82814=CARTESIAN_POINT ( 'NONE',  ( 52.46142023538963173, 213.3464784336661637, 1.353441290958777327E-15 ) ) ;
#82815=CARTESIAN_POINT ( 'NONE',  ( 207.6590484093196096, 270.9709728340903894, 3.402057849327809524 ) ) ;
#82817=EDGE_CURVE ( 'NONE', #62993, #35992, #100027, .T. ) ;
#82819=CARTESIAN_POINT ( 'NONE',  ( 164.9404048476745004, 244.9618339132846074, -2.801285734921658666 ) ) ;
#82821=EDGE_CURVE ( 'NONE', #3950, #4092, #49120, .T. ) ;
#82823=CARTESIAN_POINT ( 'NONE',  ( 1.898513289055842712, 185.2365022471903444, 2.944929066748280225E-16 ) ) ;
#82825=CARTESIAN_POINT ( 'NONE',  ( 139.7406297344813311, 260.6744531367911009, 4.594050593750047540 ) ) ;
#82827=CARTESIAN_POINT ( 'NONE',  ( 165.0826521866380006, 244.7154542949585050, 1.746033430215258475 ) ) ;
#82829=DIRECTION ( 'NONE',  ( -0.8660254037844387076, -0.4999999999999998890, -0.000000000000000000 ) ) ;
#82831=CARTESIAN_POINT ( 'NONE',  ( 188.2348408267917250, 289.2768701213889244, 14.43578146676328977 ) ) ;
#82834=CARTESIAN_POINT ( 'NONE',  ( 150.6431064791187850, 269.7254810985950257, 15.11064854015152470 ) ) ;
#82835=CARTESIAN_POINT ( 'NONE',  ( 163.4299912484447930, 247.5779470075939059, 8.687773149566549336 ) ) ;
#82836=CARTESIAN_POINT ( 'NONE',  ( 129.4230657250939203, 233.9824982072973683, 3.021315404115420679E-15 ) ) ;
#82837=CARTESIAN_POINT ( 'NONE',  ( 172.9592948101169725, 268.4257463397073593, -16.38380952890091891 ) ) ;
#82838=CARTESIAN_POINT ( 'NONE',  ( 197.3002854903134562, 273.1938965430982194, -13.39091482477390116 ) ) ;
#82839=VERTEX_POINT ( 'NONE', #56575 ) ;
#82841=CARTESIAN_POINT ( 'NONE',  ( 171.3274490369448415, 284.4986492857913163, -11.39081580260379134 ) ) ;
#82843=CARTESIAN_POINT ( 'NONE',  ( 80.05961770938091604, 205.4824982072973967, 3.021315404115420679E-15 ) ) ;
#82844=CARTESIAN_POINT ( 'NONE',  ( 196.1399273980812836, 271.0394808790050547, 12.45890580183448471 ) ) ;
#82845=CARTESIAN_POINT ( 'NONE',  ( 185.8152975361811912, 296.8366838734828548, 5.365625994531613152 ) ) ;
#82847=FACE_OUTER_BOUND ( 'NONE', #82250, .T. ) ;
#82849=EDGE_CURVE ( 'NONE', #22636, #51125, #58895, .T. ) ;
#82854=CARTESIAN_POINT ( 'NONE',  ( 166.7959447105422157, 276.3626885415273478, 15.91653206054683523 ) ) ;
#82857=ORIENTED_EDGE ( 'NONE', *, *, #32793, .F. ) ;
#82858=CARTESIAN_POINT ( 'NONE',  ( 163.5477118939200807, 267.5842859632946329, -17.71268400963646528 ) ) ;
#82859=CARTESIAN_POINT ( 'NONE',  ( 185.2241444343604257, 291.3773840544799896, 11.95617939456810674 ) ) ;
#82860=CARTESIAN_POINT ( 'NONE',  ( 163.7064929935861244, 247.0990319366274548, 6.401263337036986023 ) ) ;
#82862=ORIENTED_EDGE ( 'NONE', *, *, #62203, .F. ) ;
#82863=CARTESIAN_POINT ( 'NONE',  ( 75.84410613756948294, 226.8464784336661353, 1.353441290958777525E-15 ) ) ;
#82864=CARTESIAN_POINT ( 'NONE',  ( 155.0478382459045577, 262.0962618848092802, 18.21693143622618649 ) ) ;
#82865=CARTESIAN_POINT ( 'NONE',  ( 180.1013849714563833, 270.4519419265931788, -16.02035677620936482 ) ) ;
#82867=VERTEX_POINT ( 'NONE', #25175 ) ;
#82868=ADVANCED_FACE ( 'NONE', ( #8486 ), #98364, .F. ) ;
#82870=CARTESIAN_POINT ( 'NONE',  ( 207.3500332735622180, 270.8109745646875126, 1.847778963486053749 ) ) ;
#82871=VERTEX_POINT ( 'NONE', #72816 ) ;
#82875=ORIENTED_EDGE ( 'NONE', *, *, #52578, .T. ) ;
#82876=CARTESIAN_POINT ( 'NONE',  ( 165.0777597283848195, 244.7239282812269039, 1.811418920707685842 ) ) ;
#82877=CARTESIAN_POINT ( 'NONE',  ( 152.9273493951901628, 265.7690563111299298, -17.70273273795505631 ) ) ;
#82880=CARTESIAN_POINT ( 'NONE',  ( 164.7384773709341630, 265.0745892635314362, -16.62235727310338618 ) ) ;
#82881=ORIENTED_EDGE ( 'NONE', *, *, #97232, .T. ) ;
#82886=CARTESIAN_POINT ( 'NONE',  ( 166.9150765994704955, 283.4538441081094788, 8.983515016175676493 ) ) ;
#82887=CARTESIAN_POINT ( 'NONE',  ( 203.2792425030030188, 271.6204427260279317, 9.522413789076535906 ) ) ;
#82888=VERTEX_POINT ( 'NONE', #20097 ) ;
#82890=CARTESIAN_POINT ( 'NONE',  ( 160.0081047537594543, 253.5048282741223602, -16.11956848123596941 ) ) ;
#82891=CARTESIAN_POINT ( 'NONE',  ( 150.1843315557205756, 276.3611790585334802, -5.337065203306020855 ) ) ;
#82892=CARTESIAN_POINT ( 'NONE',  ( 165.4478602433182743, 246.8625711930905027, -1.873768097677063427 ) ) ;
#82894=CARTESIAN_POINT ( 'NONE',  ( 168.4809247738020019, 252.9187805847961670, 12.05003015331094041 ) ) ;
#82896=VERTEX_POINT ( 'NONE', #18596 ) ;
#82897=B_SPLINE_CURVE_WITH_KNOTS ( 'NONE', 3,
 ( #73335, #26724, #27230, #73823, #81459, #51510, #90568, #44397, #43901, #57606, #12531, #52014, #4415, #59083, #50022, #34321, #12030, #35310, #74841, #97642, #42886, #5421, #82955, #13529, #75332, #67207, #58114, #65219, #43402, #89095, #50505, #96161, #28714, #88587, #36303, #19644, #98130, #19148, #66223, #35813, #80976, #11541, #66707, #3922, #28207, #97161 ),
 .UNSPECIFIED., .F., .F.,
 ( 4, 2, 2, 2, 2, 2, 2, 2, 2, 2, 2, 2, 2, 2, 2, 2, 2, 2, 2, 2, 2, 2, 4 ),
 ( 0.002719413596635465377, 0.003132706262424970068, 0.003339352595319770335, 0.003442675761767165915, 0.003545998928214561929, 0.003752645261109377375, 0.003959291594004193254, 0.004372584259793886596, 0.005199169591373273280, 0.006025754922952659097, 0.006852340254532045781, 0.007678925586111432465, 0.007782248752558854933, 0.007833910335782613005, 0.007885571919006371944, 0.007937233502230130883, 0.007988895085453889822, 0.008092218251901553416, 0.008505510917692367390, 0.008712157250587838561, 0.008918803583483309733, 0.009125449916378780904, 0.009332096249274252076 ),
 .UNSPECIFIED. ) ;
#82898=CARTESIAN_POINT ( 'NONE',  ( 155.4266178972399359, 261.4401962838231839, -18.59384973550221076 ) ) ;
#82901=CARTESIAN_POINT ( 'NONE',  ( 160.1345624105295542, 276.5719778673294513, 12.81990450689413308 ) ) ;
#82902=ADVANCED_FACE ( 'NONE', ( #26189 ), #58079, .T. ) ;
#82903=CARTESIAN_POINT ( 'NONE',  ( 201.4015734403423323, 266.9510600575795820, -2.208871080923278107 ) ) ;
#82904=CARTESIAN_POINT ( 'NONE',  ( 164.0871364075242980, 246.4397382041199762, -7.779248982433414561 ) ) ;
#82907=CARTESIAN_POINT ( 'NONE',  ( -9.188242552867592394, 159.3768266524160140, 9.188101187500098632 ) ) ;
#82909=CARTESIAN_POINT ( 'NONE',  ( 19.34531673258195994, 188.6427522451419350, 10.00000000000009415 ) ) ;
#82910=ORIENTED_EDGE ( 'NONE', *, *, #39834, .T. ) ;
#82913=CARTESIAN_POINT ( 'NONE',  ( 169.1310403812000516, 286.3093371794724931, 8.868891257890425095 ) ) ;
#82915=CARTESIAN_POINT ( 'NONE',  ( 172.2401199401735710, 289.4450576335847813, 2.617625608981040575 ) ) ;
#82919=CARTESIAN_POINT ( 'NONE',  ( 18.68642948779652002, 193.8464784336661637, 1.353441290958777525E-15 ) ) ;
#82920=CARTESIAN_POINT ( 'NONE',  ( 116.5476472112030990, 238.0958772461660544, -9.188101187500095079 ) ) ;
#82921=CARTESIAN_POINT ( 'NONE',  ( 45.26399402665309424, 185.3932355074535678, -2.679491924311248496 ) ) ;
#82924=CARTESIAN_POINT ( 'NONE',  ( 178.3505713125701959, 283.6140345280227848, -14.62659922741302054 ) ) ;
#82925=AXIS2_PLACEMENT_3D ( 'NONE', #96198, #72889, #74385 ) ;
#82927=CARTESIAN_POINT ( 'NONE',  ( 193.7706395672514645, 295.0264025848412075, 15.16938698680137065 ) ) ;
#82928=CARTESIAN_POINT ( 'NONE',  ( 207.8844858873204657, 270.5805036682629066, -6.251308616122969397 ) ) ;
#82929=CARTESIAN_POINT ( 'NONE',  ( 194.3541845315608612, 294.0156730581561533, -14.67567721756631016 ) ) ;
#82934=CARTESIAN_POINT ( 'NONE',  ( 184.1241864019008858, 268.6134890520179397, -15.18471742826366722 ) ) ;
#82937=CARTESIAN_POINT ( 'NONE',  ( 172.7788321272523717, 263.1548091139151779, -15.50655718291449148 ) ) ;
#82940=CARTESIAN_POINT ( 'NONE',  ( 95.14032143958276322, 234.9244531367911009, -4.594050593750046652 ) ) ;
#82941=CARTESIAN_POINT ( 'NONE',  ( 190.7779368023172708, 300.2099158256590385, 8.142228434510803581 ) ) ;
#82944=CARTESIAN_POINT ( 'NONE',  ( 157.8092552871339365, 257.3133472685137235, 17.04082256169242626 ) ) ;
#82945=CARTESIAN_POINT ( 'NONE',  ( 199.9508427912207367, 284.3219765998254047, 18.49391385354404349 ) ) ;
#82946=CYLINDRICAL_SURFACE ( 'NONE', #22206, 10.00000000000010658 ) ;
#82947=CARTESIAN_POINT ( 'NONE',  ( 199.2383506163646132, 285.5560492466715345, -17.78808061564097898 ) ) ;
#82948=CARTESIAN_POINT ( 'NONE',  ( 204.3209023394900328, 276.1179509721322347, -13.17759910032226678 ) ) ;
#82950=CARTESIAN_POINT ( 'NONE',  ( 147.4824818982269790, 275.1998434563504929, -4.972419998968698351 ) ) ;
#82951=CYLINDRICAL_SURFACE ( 'NONE', #55540, 17.82106496071139645 ) ;
#82952=ORIENTED_EDGE ( 'NONE', *, *, #4440, .F. ) ;
#82954=CARTESIAN_POINT ( 'NONE',  ( 192.8011239859581849, 296.7056528303708660, -11.79847971295421694 ) ) ;
#82955=CARTESIAN_POINT ( 'NONE',  ( 191.3732078456864372, 287.7026800961180015, -15.83705375440161767 ) ) ;
#82956=ORIENTED_EDGE ( 'NONE', *, *, #1901, .T. ) ;
#82959=CARTESIAN_POINT ( 'NONE',  ( 175.6063544791335573, 254.0105997054014040, 8.344378697908656051 ) ) ;
#82960=CARTESIAN_POINT ( 'NONE',  ( 172.7840071827034478, 253.8156868574323255, -8.935542012173989690 ) ) ;
#82962=CARTESIAN_POINT ( 'NONE',  ( 136.9984762794282744, 263.2365022471902876, 2.944929066748280225E-16 ) ) ;
#82966=ORIENTED_EDGE ( 'NONE', *, *, #64947, .T. ) ;
#82967=CARTESIAN_POINT ( 'NONE',  ( 197.0006684375643715, 265.0764226805687827, -4.603465283812302467 ) ) ;
#82970=CARTESIAN_POINT ( 'NONE',  ( 183.1488928027059444, 291.3758770271683147, -10.74625559401416375 ) ) ;
#82973=CARTESIAN_POINT ( 'NONE',  ( 205.5156181057928677, 274.6835030222813998, 11.38452381065716068 ) ) ;
#82974=CARTESIAN_POINT ( 'NONE',  ( 193.4272026183557216, 280.4276906386824635, -16.92506342575424583 ) ) ;
#82975=CARTESIAN_POINT ( 'NONE',  ( 193.2107205041928353, 295.9962108501849229, -13.27437237753875721 ) ) ;
#82976=CARTESIAN_POINT ( 'NONE',  ( 201.3053499423511425, 281.9759013948520874, -16.75960365258566398 ) ) ;
#82977=FACE_OUTER_BOUND ( 'NONE', #68825, .T. ) ;
#82980=CARTESIAN_POINT ( 'NONE',  ( 170.9169832065359458, 256.6048082181670225, 13.90689315385514035 ) ) ;
#82983=ORIENTED_EDGE ( 'NONE', *, *, #24044, .F. ) ;
#82984=CARTESIAN_POINT ( 'NONE',  ( 183.8037341582430884, 275.4624792557407318, 17.77592483611231700 ) ) ;
#82985=CARTESIAN_POINT ( 'NONE',  ( 174.5258411212118972, 257.2153983152082333, -12.12657788165876838 ) ) ;
#82986=CARTESIAN_POINT ( 'NONE',  ( 163.1080940025530310, 272.5857820118623636, -15.50684756597832958 ) ) ;
#82988=CARTESIAN_POINT ( 'NONE',  ( 148.7819146692434629, 276.2864599824047218, -5.482525570765545808 ) ) ;
#82990=CARTESIAN_POINT ( 'NONE',  ( 189.8238368927809745, 301.8624653444729802, -0.3620111495846872751 ) ) ;
#82991=CARTESIAN_POINT ( 'NONE',  ( 170.9352951703182555, 287.6820827080605341, -4.605083712371007110 ) ) ;
#82993=CARTESIAN_POINT ( 'NONE',  ( 181.7635954225607406, 256.3719561854650237, 5.206822859736072395 ) ) ;
#82994=CARTESIAN_POINT ( 'NONE',  ( 101.5001087246834857, 241.6589784336661637, -6.496448406907675876E-16 ) ) ;
#82997=CARTESIAN_POINT ( 'NONE',  ( 191.8819534272594183, 275.1740554287606528, 16.67007678262692494 ) ) ;
#82998=EDGE_CURVE ( 'NONE', #27498, #44553, #90257, .T. ) ;
#83005=B_SPLINE_SURFACE_WITH_KNOTS ( 'NONE', 3, 1, ( 
 ( #16465, #78284 ),
 ( #31155, #39733 ),
 ( #70665, #94011 ),
 ( #30680, #1279 ),
 ( #76771, #45848 ),
 ( #63068, #55446 ),
 ( #86433, #23053 ),
 ( #92507, #47848 ),
 ( #6871, #53462 ),
 ( #37762, #99588 ),
 ( #53951, #30172 ),
 ( #61058, #15449 ),
 ( #46348, #77271 ),
 ( #65932, #5143 ),
 ( #71193, #26946 ),
 ( #3662, #57830 ),
 ( #73551, #12761 ),
 ( #58814, #66924 ),
 ( #42133, #89303 ),
 ( #49743, #18860 ),
 ( #11758, #58328 ),
 ( #65438, #26457 ),
 ( #34540, #9374 ),
 ( #27457, #12253 ),
 ( #95899, #4135 ),
 ( #73064, #89776 ),
 ( #51221, #96887 ),
 ( #42622, #43110 ),
 ( #19858, #36024 ),
 ( #3178, #88810 ),
 ( #96383, #19376 ),
 ( #50724, #97364 ),
 ( #50235, #74055 ),
 ( #81190, #35028 ) ),
 .UNSPECIFIED., .T., .F., .F.,
 ( 4, 2, 2, 2, 2, 2, 2, 2, 2, 2, 2, 2, 2, 2, 2, 2, 4 ),
 ( 2, 2 ),
 ( 0.000000000000000000, 0.06250000000000000000, 0.1250000000000000000, 0.1875000000000000000, 0.2500000000000000000, 0.3125000000000000000, 0.3750000000000000000, 0.4375000000000000000, 0.5000000000000000000, 0.5625000000000000000, 0.6250000000000000000, 0.6875000000000000000, 0.7500000000000000000, 0.8125000000000000000, 0.8750000000000000000, 0.9375000000000000000, 1.000000000000000000 ),
 ( 0.000000000000000000, 1.000000000000000000 ),
 .UNSPECIFIED. ) ;
#83006=CARTESIAN_POINT ( 'NONE',  ( 195.9920715006079490, 291.1787696107118677, 15.99608784761372071 ) ) ;
#83009=VERTEX_POINT ( 'NONE', #3887 ) ;
#83011=B_SPLINE_CURVE_WITH_KNOTS ( 'NONE', 3,
 ( #8888, #30699, #24086, #86453, #69185, #54982, #85961, #39266, #32184, #16978, #39757, #61579, #31178, #61078, #76791, #23077, #45866, #68682, #85441, #46367, #53969, #15989, #37780, #16487, #47383, #15472, #100114, #93016, #7904, #70176, #84926, #78307, #784, #31670, #77297, #7384, #38779, #69685, #62566, #290, #62068, #94032, #23570, #38273, #54462, #70685 ),
 .UNSPECIFIED., .F., .F.,
 ( 4, 2, 2, 2, 2, 2, 2, 2, 2, 2, 2, 2, 2, 2, 2, 2, 2, 2, 2, 2, 2, 2, 4 ),
 ( 0.002472027920451953277, 0.002893672058135126832, 0.003104494126976747436, 0.003209905161397578338, 0.003315316195818409240, 0.003420727230239240142, 0.003526138264660071044, 0.003736960333501726343, 0.004158604471184948470, 0.005001892746551547114, 0.005845181021918147493, 0.006688469297284747005, 0.007110113434968052398, 0.007531757572651357792, 0.007637168607072145760, 0.007689874124282577474, 0.007742579641493009188, 0.007847990675913931596, 0.007953401710334854005, 0.008375045848018541905, 0.008796689985702228071, 0.009007512054544076358, 0.009218334123385926379 ),
 .UNSPECIFIED. ) ;
#83012=CARTESIAN_POINT ( 'NONE',  ( 41.93414601462609426, 195.0177522451418781, -10.00000000000009592 ) ) ;
#83015=CARTESIAN_POINT ( 'NONE',  ( 194.6903171191896433, 266.4159511179065021, -7.916380833475905376 ) ) ;
#83018=CARTESIAN_POINT ( 'NONE',  ( 197.9793137651938935, 285.9304194886471464, 17.71000985939274841 ) ) ;
#83019=CARTESIAN_POINT ( 'NONE',  ( 199.8805116513159135, 284.0430704225434511, 16.91808164086238264 ) ) ;
#83020=CARTESIAN_POINT ( 'NONE',  ( 152.6873874250818517, 266.1846826352417565, -16.66598363829485763 ) ) ;
#83021=VERTEX_POINT ( 'NONE', #36267 ) ;
#83022=CARTESIAN_POINT ( 'NONE',  ( 157.1886094632603772, 258.3883373689681093, 18.40926891635499985 ) ) ;
#83023=B_SPLINE_SURFACE_WITH_KNOTS ( 'NONE', 3, 1, ( 
 ( #15437, #88796 ),
 ( #77259, #10742 ),
 ( #48234, #18847 ),
 ( #26445, #87315 ),
 ( #57321, #33540 ),
 ( #7868, #38747 ),
 ( #64438, #56824 ),
 ( #80683, #259 ),
 ( #79179, #63929 ),
 ( #88293, #11258 ),
 ( #2148, #31141 ),
 ( #92985, #71553 ),
 ( #33029, #94868 ),
 ( #25429, #56321 ),
 ( #50713, #82678 ),
 ( #27441, #4629 ),
 ( #35016, #19364 ),
 ( #51209, #97353 ),
 ( #81666, #50223 ),
 ( #21325, #35523 ),
 ( #81178, #96873 ),
 ( #44596, #59291 ),
 ( #66423, #37011 ),
 ( #90272, #51736 ),
 ( #58802, #12750 ),
 ( #74552, #11744 ),
 ( #28931, #36011 ),
 ( #83153, #66913 ),
 ( #13243, #36511 ),
 ( #59805, #90774 ),
 ( #75531, #67920 ),
 ( #98841, #42607 ),
 ( #8122, #52701 ),
 ( #30910, #15698 ) ),
 .UNSPECIFIED., .T., .F., .F.,
 ( 4, 2, 2, 2, 2, 2, 2, 2, 2, 2, 2, 2, 2, 2, 2, 2, 4 ),
 ( 2, 2 ),
 ( 0.000000000000000000, 0.06250000000000000000, 0.1250000000000000000, 0.1875000000000000000, 0.2500000000000000000, 0.3125000000000000000, 0.3750000000000000000, 0.4375000000000000000, 0.5000000000000000000, 0.5625000000000000000, 0.6250000000000000000, 0.6875000000000000000, 0.7500000000000000000, 0.8125000000000000000, 0.8750000000000000000, 0.9375000000000000000, 1.000000000000000000 ),
 ( 0.000000000000000000, 1.000000000000000000 ),
 .UNSPECIFIED. ) ;
#83026=CARTESIAN_POINT ( 'NONE',  ( 173.2276582641987659, 251.6345432004491443, -0.2848423752525459096 ) ) ;
#83027=CARTESIAN_POINT ( 'NONE',  ( 45.14796862286864609, 185.3262482093457209, 3.021315404115420679E-15 ) ) ;
#83031=CARTESIAN_POINT ( 'NONE',  ( 194.2669918475045279, 294.1666952169902629, 14.00965265288584050 ) ) ;
#83032=CARTESIAN_POINT ( 'NONE',  ( 178.2382707639212356, 285.7843550335422833, 14.43266090959460435 ) ) ;
#83034=CARTESIAN_POINT ( 'NONE',  ( 78.52397964811635234, 206.9548013555409796, -4.594050593750042211 ) ) ;
#83035=CARTESIAN_POINT ( 'NONE',  ( 159.4491226731523454, 254.4730136382542582, -15.39140229921534520 ) ) ;
#83037=CARTESIAN_POINT ( 'NONE',  ( 207.6050568035884680, 271.0644890383991310, -1.456818755242089702 ) ) ;
#83038=CARTESIAN_POINT ( 'NONE',  ( 197.1490659794403939, 288.7466081235293700, -16.65847605485208760 ) ) ;
#83039=CARTESIAN_POINT ( 'NONE',  ( 161.1492466472929266, 251.5283125358769212, -13.33353587056634915 ) ) ;
#83045=CARTESIAN_POINT ( 'NONE',  ( 157.6304115535352537, 270.8650229002738001, -16.00510772102553858 ) ) ;
#83047=( BOUNDED_CURVE ( )  B_SPLINE_CURVE ( 2, ( #48861, #64044, #9346, #32641, #42229, #87432, #57431, #56932, #3272 ),
 .UNSPECIFIED., .F., .T. ) 
 B_SPLINE_CURVE_WITH_KNOTS ( ( 3, 2, 2, 2, 3 ),
 ( 0.04435483870967742159, 0.04569892473118279674, 0.04838709677419354704, 0.05107526881720430428, 0.05241935483870967943 ),
 .UNSPECIFIED. ) 
 CURVE ( )  GEOMETRIC_REPRESENTATION_ITEM ( )  RATIONAL_B_SPLINE_CURVE ( ( 0.9330127018922194093, 0.9330127018922194093, 1.000000000000000000, 0.8660254037844387076, 1.000000000000000000, 0.8660254037844387076, 1.000000000000000000, 0.9330127018922194093, 0.9330127018922194093 ) ) 
 REPRESENTATION_ITEM ( '' )  );
#83048=CARTESIAN_POINT ( 'NONE',  ( 27.23877744593285755, 186.5333772461660544, 9.188101187500095079 ) ) ;
#83049=EDGE_CURVE ( 'NONE', #87772, #82029, #38237, .T. ) ;
#83054=CARTESIAN_POINT ( 'NONE',  ( 52.11020483269097525, 191.7048013555409796, 4.594050593750051981 ) ) ;
#83056=CARTESIAN_POINT ( 'NONE',  ( 151.1230807375396807, 268.8941412966845519, -14.26613110909109849 ) ) ;
#83059=CARTESIAN_POINT ( 'NONE',  ( 178.6317619811870259, 253.9327355832967612, -4.167451725846189170 ) ) ;
#83061=CARTESIAN_POINT ( 'NONE',  ( 176.6908210328434450, 275.1332777264201468, 16.63294263746914581 ) ) ;
#83063=CARTESIAN_POINT ( 'NONE',  ( 149.6148422561466305, 277.4437614652936190, 3.137689077364430368 ) ) ;
#83064=CARTESIAN_POINT ( 'NONE',  ( 163.4168112749207467, 255.7475448173238135, -14.83461233001398405 ) ) ;
#83066=B_SPLINE_CURVE_WITH_KNOTS ( 'NONE', 3,
 ( #46866, #77790, #8375, #39239, #70152, #31647, #1276, #47358, #39731, #8865, #761, #62545, #93505, #24064, #85937, #32160, #63067, #80314, #97016, #27081, #95533, #81315, #74190, #58452, #79816, #65563, #50359, #19504, #17988, #41251, #35160, #26081, #35662, #33684, #11398, #89424, #96511, #10383, #66563, #25578, #42744, #56464, #57962, #11885, #57455, #72192, #43246, #87456 ),
 .UNSPECIFIED., .F., .F.,
 ( 4, 2, 2, 2, 2, 2, 2, 2, 2, 2, 2, 2, 2, 2, 2, 2, 2, 2, 2, 2, 2, 2, 2, 4 ),
 ( 0.0005187678782849775710, 0.001523663581573160260, 0.002026111433217250846, 0.002151723396128240803, 0.002277335359039230761, 0.002402947321950220285, 0.002528559284861210243, 0.002779783210683136382, 0.003031007136505062087, 0.003533454988148913931, 0.004538350691436559073, 0.005543246394724203781, 0.006045694246368027436, 0.006296918172189937962, 0.006548142098011849356, 0.006610948079467326988, 0.006673754060922803752, 0.006736560042378281384, 0.006799366023833759015, 0.007050589949655808319, 0.007301813875477857624, 0.007553037801299906061, 0.008055485652944047170, 0.008557933504588185677 ),
 .UNSPECIFIED. ) ;
#83069=CARTESIAN_POINT ( 'NONE',  ( 95.28491933047786233, 232.4865022471902876, -10.00000000000009415 ) ) ;
#83070=CARTESIAN_POINT ( 'NONE',  ( 200.4592688079413847, 283.4413569069752725, 18.39277739746426832 ) ) ;
#83071=CARTESIAN_POINT ( 'NONE',  ( 165.0635501472802957, 269.5554238516661485, -16.29592778247673479 ) ) ;
#83074=CARTESIAN_POINT ( 'NONE',  ( 51.75794814269728050, 206.8149278399160949, -9.188101187500095079 ) ) ;
#83076=CYLINDRICAL_SURFACE ( 'NONE', #28725, 17.82106496071139645 ) ;
#83077=CARTESIAN_POINT ( 'NONE',  ( 162.6012440678564133, 250.5872267631778527, 12.68799555347811392 ) ) ;
#83081=DIRECTION ( 'NONE',  ( 0.4999999999999998890, -0.8660254037844385966, 0.000000000000000000 ) ) ;
#83084=CARTESIAN_POINT ( 'NONE',  ( 176.6079174955794429, 274.4222495781426687, -16.64941559833394180 ) ) ;
#83086=CARTESIAN_POINT ( 'NONE',  ( 157.1517242151937523, 258.4522244926691883, 18.42395718741238042 ) ) ;
#83093=DIRECTION ( 'NONE',  ( 0.4999999999999998890, -0.8660254037844385966, 0.000000000000000000 ) ) ;
#83094=CARTESIAN_POINT ( 'NONE',  ( 167.2310611304565953, 261.7083964245842935, 16.31600354341965087 ) ) ;
#83095=CARTESIAN_POINT ( 'NONE',  ( 159.3451320108506764, 254.6531307488737355, -16.72997986213134425 ) ) ;
#83099=CARTESIAN_POINT ( 'NONE',  ( 207.6875671281972870, 270.9215769640275653, -2.211577121115235300 ) ) ;
#83101=CARTESIAN_POINT ( 'NONE',  ( 188.6852239700973541, 295.1919775169639593, -11.19696146816310112 ) ) ;
#83103=CARTESIAN_POINT ( 'NONE',  ( 164.4977080725190319, 265.4334248489062702, -16.72650950839127049 ) ) ;
#83104=CARTESIAN_POINT ( 'NONE',  ( 119.6326891643026613, 246.0024278399160949, -9.188101187500093303 ) ) ;
#83107=CARTESIAN_POINT ( 'NONE',  ( 174.1098532474522642, 265.5656642385555983, 16.65038209508332301 ) ) ;
#83108=CARTESIAN_POINT ( 'NONE',  ( 182.5686778644665083, 296.6873302901632314, 1.787712280751329708 ) ) ;
#83113=ORIENTED_EDGE ( 'NONE', *, *, #57821, .T. ) ;
#83115=CARTESIAN_POINT ( 'NONE',  ( 195.0452099689448460, 291.6879811394439912, -15.84229188559630686 ) ) ;
#83116=CARTESIAN_POINT ( 'NONE',  ( 72.82007368749162879, 224.3967562850346837, -4.648177544792955347E-16 ) ) ;
#83119=CARTESIAN_POINT ( 'NONE',  ( 155.6518451030846961, 261.0500913200531841, 17.91778754207898317 ) ) ;
#83120=CARTESIAN_POINT ( 'NONE',  ( 72.82007368749162879, 224.3967562850346837, -4.648177544792955347E-16 ) ) ;
#83122=ADVANCED_FACE ( 'NONE', ( #74803 ), #52460, .T. ) ;
#83123=CARTESIAN_POINT ( 'NONE',  ( 152.6621968174709991, 266.2283140474973493, -17.02835521334403168 ) ) ;
#83126=CARTESIAN_POINT ( 'NONE',  ( 165.3929592122126451, 286.2279243276498732, 4.432946431554212197 ) ) ;
#83129=CARTESIAN_POINT ( 'NONE',  ( 174.0121777967311516, 253.3006934959134355, -7.652886187659225570 ) ) ;
#83130=CARTESIAN_POINT ( 'NONE',  ( 205.7829192689729325, 274.2205238267313234, 11.21202327925415254 ) ) ;
#83131=CARTESIAN_POINT ( 'NONE',  ( 196.4170778717353585, 290.4426369823788718, -17.78762421190030452 ) ) ;
#83132=CARTESIAN_POINT ( 'NONE',  ( 195.6729656511292035, 279.4309229103643020, 16.33979319762304883 ) ) ;
#83133=CARTESIAN_POINT ( 'NONE',  ( 164.4915767550571957, 245.7392269735623529, -6.407198159945809657 ) ) ;
#83134=CARTESIAN_POINT ( 'NONE',  ( 136.0871718362070339, 255.5024278399161233, 9.188101187500095079 ) ) ;
#83135=ORIENTED_EDGE ( 'NONE', *, *, #2405, .F. ) ;
#83138=CARTESIAN_POINT ( 'NONE',  ( 155.7413558407242533, 261.8087528638905610, -16.98101007095269210 ) ) ;
#83142=ORIENTED_EDGE ( 'NONE', *, *, #10456, .T. ) ;
#83144=CARTESIAN_POINT ( 'NONE',  ( 185.5970932491234748, 277.7727884765715771, -17.11431047842418707 ) ) ;
#83148=CARTESIAN_POINT ( 'NONE',  ( 199.7212432965426103, 266.8524737126543869, 0.8277979432595076181 ) ) ;
#83149=CARTESIAN_POINT ( 'NONE',  ( 195.1484500613037483, 263.5738921410981561, 0.8534460714690799144 ) ) ;
#83151=CARTESIAN_POINT ( 'NONE',  ( 190.5541309856500050, 300.5975588711562523, -4.167177996129430184 ) ) ;
#83152=CARTESIAN_POINT ( 'NONE',  ( 182.9775332447387655, 280.7556200032468610, 17.06854547713099990 ) ) ;
#83153=CARTESIAN_POINT ( 'NONE',  ( 204.8878784573704195, 275.7707799872745795, -14.13380496213581594 ) ) ;
#83154=CARTESIAN_POINT ( 'NONE',  ( 195.4470299022805762, 270.3734295143469808, 12.00835009477670390 ) ) ;
#83158=CARTESIAN_POINT ( 'NONE',  ( 190.1519139143167081, 301.2942192743771557, 4.481136594690903863 ) ) ;
#83161=CARTESIAN_POINT ( 'NONE',  ( 197.9552487813401456, 287.7784468162186613, 17.26493623863614602 ) ) ;
#83163=CARTESIAN_POINT ( 'NONE',  ( -6.265406815095104776, 161.0643266524160140, 9.188101187500095079 ) ) ;
#83164=CARTESIAN_POINT ( 'NONE',  ( 173.5307509579417342, 284.0411775505230594, -12.16872317665307079 ) ) ;
#83166=ADVANCED_FACE ( 'NONE', ( #23040 ), #6859, .T. ) ;
#83169=CARTESIAN_POINT ( 'NONE',  ( 151.0013883899287066, 269.1049186256390726, -14.25461351222133466 ) ) ;
#83170=CARTESIAN_POINT ( 'NONE',  ( 1.284818304444202530, 180.7369531367911293, -4.594050593750048428 ) ) ;
#83171=CARTESIAN_POINT ( 'NONE',  ( 181.6464193077049458, 276.3867670284828932, -17.07225131682299946 ) ) ;
#83174=CARTESIAN_POINT ( 'NONE',  ( 170.2422670303552081, 270.8252190829385881, -17.42252638875442017 ) ) ;
#83178=CARTESIAN_POINT ( 'NONE',  ( 196.3462811589356249, 269.2578400835121215, -10.58958620393924477 ) ) ;
#83179=CARTESIAN_POINT ( 'NONE',  ( 73.11106055086588640, 213.0177522451418497, -10.00000000000009592 ) ) ;
#83180=ADVANCED_FACE ( 'NONE', ( #53936 ), #83023, .F. ) ;
#83181=CARTESIAN_POINT ( 'NONE',  ( 177.0233654624311725, 254.4087770924622873, -3.874647819833805240 ) ) ;
#83182=CARTESIAN_POINT ( 'NONE',  ( 197.9679655381963244, 287.7564207472362341, 17.61949439995294497 ) ) ;
#83183=CARTESIAN_POINT ( 'NONE',  ( 180.8886826254641846, 294.5332475160486183, 1.019920492680034263 ) ) ;
#83184=CARTESIAN_POINT ( 'NONE',  ( 45.92147131476482969, 203.9865022471903444, -10.00000000000009415 ) ) ;
#83186=CARTESIAN_POINT ( 'NONE',  ( 190.5893431400089923, 300.5365696307625853, -0.3099240395267599535 ) ) ;
#83187=CARTESIAN_POINT ( 'NONE',  ( 23.53136650780448491, 175.2048013555409796, 4.594050593750051981 ) ) ;
#83188=CARTESIAN_POINT ( 'NONE',  ( 164.6285367961174870, 284.7931077284160892, 4.211549190166783418 ) ) ;
#83192=CARTESIAN_POINT ( 'NONE',  ( 189.1023583995641104, 268.2289247844391866, 13.73749984714365091 ) ) ;
#83194=CARTESIAN_POINT ( 'NONE',  ( 164.1193093486783710, 281.5602788190849424, 8.891021254689583486 ) ) ;
#83199=CARTESIAN_POINT ( 'NONE',  ( 193.7901930790854976, 294.9925349088783264, 14.24765323155741115 ) ) ;
#83200=VERTEX_POINT ( 'NONE', #77529 ) ;
#83201=CARTESIAN_POINT ( 'NONE',  ( 185.0212309258022856, 290.7568242972342887, 12.15772952871526336 ) ) ;
#83204=ORIENTED_EDGE ( 'NONE', *, *, #88763, .F. ) ;
#83205=CARTESIAN_POINT ( 'NONE',  ( 158.2129804214947058, 265.2348010298870236, 17.61986633405762603 ) ) ;
#83208=CARTESIAN_POINT ( 'NONE',  ( 203.3205561747472814, 278.4854618126124706, -15.14439614831292147 ) ) ;
#83212=CARTESIAN_POINT ( 'NONE',  ( 186.9124060917193333, 272.1944072449207965, -16.74496829271420850 ) ) ;
#83213=DIRECTION ( 'NONE',  ( -0.8660254037844387076, -0.4999999999999998890, -0.000000000000000000 ) ) ;
#83214=ORIENTED_EDGE ( 'NONE', *, *, #24624, .T. ) ;
#83215=CARTESIAN_POINT ( 'NONE',  ( 191.0170959869219303, 299.7956799668270946, 7.353346939903929069 ) ) ;
#83222=ORIENTED_EDGE ( 'NONE', *, *, #54183, .F. ) ;
#83223=CARTESIAN_POINT ( 'NONE',  ( 164.4573439719129340, 245.7985198932525748, 1.541132361166968501 ) ) ;
#83226=CARTESIAN_POINT ( 'NONE',  ( 149.0802055316563326, 272.4325049467973940, 12.84384348890831085 ) ) ;
#83227=CARTESIAN_POINT ( 'NONE',  ( 172.3329631802389201, 263.6870992125010389, -15.46481966459473689 ) ) ;
#83228=EDGE_CURVE ( 'NONE', #49659, #80879, #31093, .T. ) ;
#83230=CARTESIAN_POINT ( 'NONE',  ( -22.42236680055709641, 157.8615022471902591, 0.000000000000000000 ) ) ;
#83234=CARTESIAN_POINT ( 'NONE',  ( 153.8480465357228013, 265.0660884932569843, -16.61306390558784685 ) ) ;
#83235=CARTESIAN_POINT ( 'NONE',  ( 147.5492216329511166, 275.0842468449245644, 4.751613690710122739 ) ) ;
#83238=CARTESIAN_POINT ( 'NONE',  ( 153.1745822862813498, 265.3408363824576668, 16.18092354043443493 ) ) ;
#83240=CARTESIAN_POINT ( 'NONE',  ( 191.5641729352803395, 298.8481148966207570, 9.839145202254165667 ) ) ;
#83241=CARTESIAN_POINT ( 'NONE',  ( 191.6823192895500370, 298.6434794082964572, -8.424208857102787107 ) ) ;
#83244=CARTESIAN_POINT ( 'NONE',  ( 206.4943150373521803, 272.9883502116088039, 11.34100825923693101 ) ) ;
#83245=CARTESIAN_POINT ( 'NONE',  ( 196.7491951525289835, 289.8673929779723721, -16.35352603081977207 ) ) ;
#83248=CARTESIAN_POINT ( 'NONE',  ( 169.1455093422647167, 286.8367317026995238, 4.082882422040602144 ) ) ;
#83249=CARTESIAN_POINT ( 'NONE',  ( 177.0647803954294375, 289.2179056399639876, -8.988518407010369415 ) ) ;
#83251=CARTESIAN_POINT ( 'NONE',  ( 190.6733132232214984, 300.3911291803227641, -3.379496780928331390 ) ) ;
#83256=B_SPLINE_CURVE_WITH_KNOTS ( 'NONE', 3,
 ( #38055, #82740, #75106, #91818 ),
 .UNSPECIFIED., .F., .F.,
 ( 4, 4 ),
 ( 0.005284111372439467477, 0.01027133156736889999 ),
 .UNSPECIFIED. ) ;
#83258=CARTESIAN_POINT ( 'NONE',  ( 191.8935548119142425, 297.8494204854303007, -9.596788447830101987 ) ) ;
#83260=ORIENTED_EDGE ( 'NONE', *, *, #18696, .F. ) ;
#83261=CARTESIAN_POINT ( 'NONE',  ( 163.2742264920156572, 247.8477394797576778, -9.850275379362519956 ) ) ;
#83263=B_SPLINE_CURVE_WITH_KNOTS ( 'NONE', 3,
 ( #87129, #65248, #10563, #3477, #34352, #34835, #25249, #26755, #63755, #41439, #78987, #72379, #55628, #94688, #57638, #9574, #19181, #65737, #50053, #11571, #71874, #86613, #71372, #64764, #17662, #2988, #48560, #17146, #40437, #87633, #49061, #25773, #79501, #10062, #2472, #33353, #18161, #79995, #20165, #27756, #59624, #12563, #82507, #58143, #67746, #89123, #66253, #60120, #90600, #21648 ),
 .UNSPECIFIED., .F., .F.,
 ( 4, 2, 2, 2, 2, 2, 2, 2, 2, 2, 2, 2, 2, 2, 2, 2, 2, 2, 2, 2, 2, 2, 2, 2, 4 ),
 ( 0.0008342906553197565857, 0.001033266195178259104, 0.001132753965107476807, 0.001232241735036694727, 0.001431217274895130349, 0.001630192814753566189, 0.002028143894470437868, 0.002426094974187309114, 0.003221997133621052039, 0.004017899293054795831, 0.004813801452488538322, 0.005211752532205410002, 0.005410728072063810713, 0.005510215841993010635, 0.005609703611922210557, 0.005659447496886774523, 0.005709191381851337621, 0.005808679151780464685, 0.006007654691638748302, 0.006206630231497031920, 0.006405605771355314670, 0.006604581311213598288, 0.006803556851071881906, 0.007002532390930164656, 0.007201507930788447406 ),
 .UNSPECIFIED. ) ;
#83264=CARTESIAN_POINT ( 'NONE',  ( 207.6900289502458179, 270.9173129631602706, 7.178327969100043227 ) ) ;
#83265=CARTESIAN_POINT ( 'NONE',  ( 52.25428207639071587, 187.6427522451417644, 1.119607411625061291E-15 ) ) ;
#83266=CARTESIAN_POINT ( 'NONE',  ( 116.7098534265301737, 244.3149278399160949, -9.188101187500095079 ) ) ;
#83267=CARTESIAN_POINT ( 'NONE',  ( 172.7371573690596449, 271.6299009131761864, 17.79590902495428040 ) ) ;
#83269=CARTESIAN_POINT ( 'NONE',  ( 195.7578697689113199, 291.5844189092309193, 17.18796537138345215 ) ) ;
#83270=CARTESIAN_POINT ( 'NONE',  ( 174.2336437131566527, 252.7393380672576200, -3.889790898222944104 ) ) ;
#83271=CARTESIAN_POINT ( 'NONE',  ( 36.95476026646328194, 182.9548013555409796, -4.594050593750042211 ) ) ;
#83277=B_SPLINE_CURVE_WITH_KNOTS ( 'NONE', 3,
 ( #17751, #10146, #25332, #79078, #64337, #95298, #47126, #78049, #23823, #56218, #9140, #87216, #86693, #8639, #55703, #49145, #9660, #40520, #79585, #39505, #70953, #16734, #25856, #32438, #41014, #71953, #2556, #71454, #63335, #47625, #31921, #2045, #69923, #94274, #70432, #62825, #24830, #24340, #56732, #32930 ),
 .UNSPECIFIED., .F., .F.,
 ( 4, 2, 2, 2, 2, 2, 2, 2, 2, 2, 2, 2, 2, 2, 2, 2, 2, 2, 2, 4 ),
 ( 0.0009087385142839295420, 0.001001542006469175903, 0.001094345498654422048, 0.001279952483024912602, 0.001651166451765993456, 0.002393594389248154299, 0.003878450264212475983, 0.004620878201694636825, 0.004992092170435751507, 0.005177699154806264178, 0.005270502646991520948, 0.005363306139176776850, 0.005409707885269485900, 0.005456109631362194082, 0.005548913123547547996, 0.005734520107918297457, 0.006105734076659791176, 0.006476948045401284028, 0.006662555029771971907, 0.006848162014142659786 ),
 .UNSPECIFIED. ) ;
#83279=CARTESIAN_POINT ( 'NONE',  ( 190.8907028847385448, 300.0145992415348815, -5.421341690443150618 ) ) ;
#83285=EDGE_CURVE ( 'NONE', #29236, #70733, #77736, .T. ) ;
#83286=CARTESIAN_POINT ( 'NONE',  ( 95.62772104926125394, 236.0177522451419350, 5.000000000000046185 ) ) ;
#83287=B_SPLINE_SURFACE_WITH_KNOTS ( 'NONE', 3, 1, ( 
 ( #66244, #88606 ),
 ( #97181, #20157 ),
 ( #51025, #12554 ),
 ( #50044, #59106 ),
 ( #90078, #20647 ),
 ( #51535, #82497 ),
 ( #13062, #72371 ),
 ( #2977, #33869 ),
 ( #57125, #88108 ),
 ( #49537, #80491 ),
 ( #90592, #68719 ),
 ( #67736, #6922 ),
 ( #82976, #22630 ),
 ( #61610, #45416 ),
 ( #92564, #45899 ),
 ( #37317, #67228 ),
 ( #29243, #52036 ),
 ( #91559, #52521 ),
 ( #76348, #13550 ),
 ( #61109, #30225 ),
 ( #76821, #91075 ),
 ( #98659, #99643 ),
 ( #37809, #83470 ),
 ( #14034, #36827 ),
 ( #44914, #75859 ),
 ( #22128, #60109 ),
 ( #7416, #21638 ),
 ( #15009, #6440 ),
 ( #44424, #83974 ),
 ( #68218, #99143 ),
 ( #75353, #29730 ),
 ( #92082, #60604 ),
 ( #59612, #36326 ),
 ( #21157, #53516 ) ),
 .UNSPECIFIED., .T., .F., .F.,
 ( 4, 2, 2, 2, 2, 2, 2, 2, 2, 2, 2, 2, 2, 2, 2, 2, 4 ),
 ( 2, 2 ),
 ( 0.000000000000000000, 0.06250000000000000000, 0.1250000000000000000, 0.1875000000000000000, 0.2500000000000000000, 0.3125000000000000000, 0.3750000000000000000, 0.4375000000000000000, 0.5000000000000000000, 0.5625000000000000000, 0.6250000000000000000, 0.6875000000000000000, 0.7500000000000000000, 0.8125000000000000000, 0.8750000000000000000, 0.9375000000000000000, 1.000000000000000000 ),
 ( 0.000000000000000000, 1.000000000000000000 ),
 .UNSPECIFIED. ) ;
#83288=ORIENTED_EDGE ( 'NONE', *, *, #38385, .F. ) ;
#83292=CARTESIAN_POINT ( 'NONE',  ( 163.4222916751007801, 247.5912830598222172, -10.52132777929285012 ) ) ;
#83293=ADVANCED_FACE ( 'NONE', ( #62289 ), #52232, .F. ) ;
#83294=CARTESIAN_POINT ( 'NONE',  ( 15.54743449484293372, 179.7833772461660544, -9.188101187500095079 ) ) ;
#83296=CARTESIAN_POINT ( 'NONE',  ( 195.6045292168243463, 273.5821757523950168, 14.58780494107374359 ) ) ;
#83299=CARTESIAN_POINT ( 'NONE',  ( -27.42236680055714260, 166.5217562850347406, 1.224646799147364892E-15 ) ) ;
#83300=B_SPLINE_CURVE_WITH_KNOTS ( 'NONE', 3,
 ( #79912, #71788, #33266, #50458, #2386, #19597, #41352, #34756, #2900, #65656, #3873, #10475, #64678, #18081, #25681, #64169, #66167, #72805, #49463, #50953, #72294, #41863, #95117, #95628, #42837, #87548, #96614, #26176, #58065, #11981, #57054, #42349, #89048, #80418, #81408, #88036, #3394, #18584, #4364, #80928, #65163, #26669, #57554, #35260, #88531, #82903, #76273, #14460 ),
 .UNSPECIFIED., .F., .F.,
 ( 4, 2, 2, 2, 2, 2, 2, 2, 2, 2, 2, 2, 2, 2, 2, 2, 2, 2, 2, 2, 2, 2, 2, 4 ),
 ( 0.0008776508359081067320, 0.0009741453280959741544, 0.001070639820283841468, 0.001167134312471708891, 0.001263628804659576313, 0.001456617789035311375, 0.001649606773411046220, 0.002421562710914172082, 0.003965474585920503170, 0.004737430523423668931, 0.005123408492175214948, 0.005316397476551025687, 0.005412891968738894194, 0.005461139214832867045, 0.005509386460926840763, 0.005557633707020814481, 0.005605880953114787332, 0.005702375445302676656, 0.005895364429678470915, 0.006088353414054266041, 0.006281342398430060300, 0.006474331382805854559, 0.006667320367181648819, 0.007053298335933237337 ),
 .UNSPECIFIED. ) ;
#83302=CARTESIAN_POINT ( 'NONE',  ( 174.2608556768636561, 287.0962246304461587, 10.28298298902735830 ) ) ;
#83303=CARTESIAN_POINT ( 'NONE',  ( 44.28847903505648986, 202.5024278399160949, -9.188101187500093303 ) ) ;
#83309=CARTESIAN_POINT ( 'NONE',  ( 5.218277336896219865, 180.4865022471902876, 10.00000000000009237 ) ) ;
#83310=CARTESIAN_POINT ( 'NONE',  ( 163.7323023463233937, 247.0543288263758086, -6.244751637846886361 ) ) ;
#83311=CARTESIAN_POINT ( 'NONE',  ( 134.5444773117747275, 257.6744531367911577, 4.594050593750047540 ) ) ;
#83313=CARTESIAN_POINT ( 'NONE',  ( 165.0596455280890211, 244.7553029964778943, 1.410246537223424079 ) ) ;
#83315=CARTESIAN_POINT ( 'NONE',  ( 64.45080651302146180, 218.0177522451419065, 5.000000000000046185 ) ) ;
#83317=CARTESIAN_POINT ( 'NONE',  ( 189.5697419595462918, 289.6068222778108066, 15.26551028775433494 ) ) ;
#83319=VERTEX_POINT ( 'NONE', #623 ) ;
#83322=CARTESIAN_POINT ( 'NONE',  ( 151.5039520077037309, 268.6434754965026173, -14.46698723261350317 ) ) ;
#83327=CIRCLE ( 'NONE', #97909, 17.82106496071138224 ) ;
#83331=CARTESIAN_POINT ( 'NONE',  ( 196.1377568310088293, 271.0462798384791654, 12.65795514811142297 ) ) ;
#83332=CARTESIAN_POINT ( 'NONE',  ( 184.7485916865611557, 296.0552073707631848, 4.660200707592978553 ) ) ;
#83333=CARTESIAN_POINT ( 'NONE',  ( 208.3790849386676598, 269.7238329819538762, -1.525282248498321946 ) ) ;
#83339=CARTESIAN_POINT ( 'NONE',  ( 167.4841441875519763, 281.4071184892553106, 13.00054054298708905 ) ) ;
#83341=CARTESIAN_POINT ( 'NONE',  ( 191.2827847134780654, 298.6246597018299553, 8.274781095337747416 ) ) ;
#83344=CARTESIAN_POINT ( 'NONE',  ( 173.0842903984389807, 255.2088337646690661, -11.69841797509658399 ) ) ;
#83345=B_SPLINE_CURVE_WITH_KNOTS ( 'NONE', 3,
 ( #29726, #43918, #60600, #15005 ),
 .UNSPECIFIED., .F., .F.,
 ( 4, 4 ),
 ( 0.04023740652969061415, 0.04865954048918677555 ),
 .UNSPECIFIED. ) ;
#83346=CARTESIAN_POINT ( 'NONE',  ( 164.1259971043086239, 246.3724295028720519, 5.761669507629934905 ) ) ;
#83348=FACE_OUTER_BOUND ( 'NONE', #69632, .T. ) ;
#83350=CARTESIAN_POINT ( 'NONE',  ( 96.60225995211651195, 217.3923013555410080, 4.594050593750050204 ) ) ;
#83351=CARTESIAN_POINT ( 'NONE',  ( 176.6943099527350682, 256.7931168052207340, -11.17617521364210731 ) ) ;
#83356=EDGE_LOOP ( 'NONE', ( #52066, #20574, #77983, #3222 ) ) ;
#83360=CARTESIAN_POINT ( 'NONE',  ( -17.42236680055705023, 149.2012482093457777, 0.000000000000000000 ) ) ;
#83362=ORIENTED_EDGE ( 'NONE', *, *, #91115, .F. ) ;
#83364=( BOUNDED_CURVE ( )  B_SPLINE_CURVE ( 2, ( #1585, #1071, #79104, #78077, #63365, #47646, #46140, #78583, #16758 ),
 .UNSPECIFIED., .F., .T. ) 
 B_SPLINE_CURVE_WITH_KNOTS ( ( 3, 2, 2, 2, 3 ),
 ( 0.2540322580645161255, 0.2553763440860215006, 0.2580645161290322509, 0.2607526881720430012, 0.2620967741935483764 ),
 .UNSPECIFIED. ) 
 CURVE ( )  GEOMETRIC_REPRESENTATION_ITEM ( )  RATIONAL_B_SPLINE_CURVE ( ( 0.9330127018922194093, 0.9330127018922194093, 1.000000000000000000, 0.8660254037844387076, 1.000000000000000000, 0.8660254037844387076, 1.000000000000000000, 0.9330127018922194093, 0.9330127018922194093 ) ) 
 REPRESENTATION_ITEM ( '' )  );
#83368=EDGE_CURVE ( 'NONE', #99756, #32094, #86672, .T. ) ;
#83370=CARTESIAN_POINT ( 'NONE',  ( 165.0565896242556505, 264.4795236785039947, -17.06046605472587530 ) ) ;
#83375=CARTESIAN_POINT ( 'NONE',  ( 164.1511151698870492, 281.6580413806572096, 8.784358064721770276 ) ) ;
#83376=CARTESIAN_POINT ( 'NONE',  ( 11.55108809852201190, 184.1427522451419634, 10.00000000000009415 ) ) ;
#83378=CARTESIAN_POINT ( 'NONE',  ( 162.6264071486809542, 248.9697954965390920, 10.36322805486644683 ) ) ;
#83379=CARTESIAN_POINT ( 'NONE',  ( 188.1606188679294576, 260.7699807044755289, 2.827598859516843532 ) ) ;
#83380=CARTESIAN_POINT ( 'NONE',  ( 161.3495717744529259, 281.4625470895858257, -6.539439586222937528 ) ) ;
#83386=CARTESIAN_POINT ( 'NONE',  ( 157.3305006125302441, 282.1378183958786963, 1.589776369934247979 ) ) ;
#83387=ORIENTED_EDGE ( 'NONE', *, *, #42975, .T. ) ;
#83388=CARTESIAN_POINT ( 'NONE',  ( 194.5115483076113208, 293.7431110027661703, -15.44127576492984666 ) ) ;
#83389=CARTESIAN_POINT ( 'NONE',  ( 193.9664686127508730, 294.0370461807386278, -14.11319465475718182 ) ) ;
#83390=CARTESIAN_POINT ( 'NONE',  ( -6.130263895410292818, 177.2677522451419350, -5.000000000000047962 ) ) ;
#83392=CARTESIAN_POINT ( 'NONE',  ( 171.6998185013865736, 280.1550421627382548, -15.19015613463140646 ) ) ;
#83393=CARTESIAN_POINT ( 'NONE',  ( 164.0970344217799948, 246.4225943405349710, -8.491506243827155131 ) ) ;
#83395=CARTESIAN_POINT ( 'NONE',  ( 161.2114343358352926, 273.1184554557211754, 15.88516176658350254 ) ) ;
#83396=CARTESIAN_POINT ( 'NONE',  ( 2.070087696330116689, 165.8768266524159856, -9.188101187500091527 ) ) ;
#83399=CARTESIAN_POINT ( 'NONE',  ( 189.0928626679413185, 297.0040558712296956, 8.255658072684374460 ) ) ;
#83400=ORIENTED_EDGE ( 'NONE', *, *, #90708, .F. ) ;
#83404=CARTESIAN_POINT ( 'NONE',  ( 175.1581344279587711, 291.8196898309956850, 3.447612312626186615 ) ) ;
#83405=DIRECTION ( 'NONE',  ( 0.4999999999999992784, -0.8660254037844390407, 0.000000000000000000 ) ) ;
#83406=CARTESIAN_POINT ( 'NONE',  ( 162.4759493558299539, 249.2303960381514969, -10.61385178995842615 ) ) ;
#83408=CARTESIAN_POINT ( 'NONE',  ( 150.1431628338321786, 276.5498008164989869, 3.614034262083622551 ) ) ;
#83410=CARTESIAN_POINT ( 'NONE',  ( 22.82720022358212120, 193.1744531367911293, 4.594050593750047540 ) ) ;
#83411=CARTESIAN_POINT ( 'NONE',  ( 123.3136442261515526, 235.8768266524159856, 9.188101187500098632 ) ) ;
#83412=CARTESIAN_POINT ( 'NONE',  ( -17.42236680055705023, 149.2012482093457777, 0.000000000000000000 ) ) ;
#83414=B_SPLINE_CURVE_WITH_KNOTS ( 'NONE', 3,
 ( #95423, #42147, #73079, #64463 ),
 .UNSPECIFIED., .F., .F.,
 ( 4, 4 ),
 ( 0.01188302911889913341, 0.01804894381992137864 ),
 .UNSPECIFIED. ) ;
#83415=CARTESIAN_POINT ( 'NONE',  ( 206.4458344621057506, 272.2190885279491681, -7.771912452422065520 ) ) ;
#83416=EDGE_CURVE ( 'NONE', #88529, #19194, #2038, .T. ) ;
#83417=CARTESIAN_POINT ( 'NONE',  ( 176.3489251979494554, 282.1873958766605028, -14.22545077220611276 ) ) ;
#83419=CARTESIAN_POINT ( 'NONE',  ( 168.8785100482814698, 272.6966330010931756, 17.41127854651366391 ) ) ;
#83420=CARTESIAN_POINT ( 'NONE',  ( 184.3506428846281722, 274.4990011916261778, 17.60835909835985547 ) ) ;
#83425=CARTESIAN_POINT ( 'NONE',  ( 186.7645341827467291, 298.9987601547266536, -0.6044513963858351158 ) ) ;
#83427=CARTESIAN_POINT ( 'NONE',  ( 162.2966749516206733, 251.8041562247694287, -12.92595150436406293 ) ) ;
#83431=CARTESIAN_POINT ( 'NONE',  ( 98.68587325814904432, 227.7833772461660544, -9.188101187500095079 ) ) ;
#83433=CARTESIAN_POINT ( 'NONE',  ( 164.6115012019945425, 276.7995639496792819, -15.09699049157054418 ) ) ;
#83434=CARTESIAN_POINT ( 'NONE',  ( -22.42236680055709641, 157.8615022471902591, 0.000000000000000000 ) ) ;
#83436=CARTESIAN_POINT ( 'NONE',  ( 199.7779437056017571, 284.6214466006996417, 18.28733359541573478 ) ) ;
#83437=CARTESIAN_POINT ( 'NONE',  ( 194.5725374088679871, 291.6374747806817140, -16.23208319182986870 ) ) ;
#83438=CARTESIAN_POINT ( 'NONE',  ( 150.6386650955079176, 269.7331738006648720, -15.06054658539322766 ) ) ;
#83439=CARTESIAN_POINT ( 'NONE',  ( 168.2820353728258738, 287.7095463320123940, -5.019694092131335772 ) ) ;
#83441=CARTESIAN_POINT ( 'NONE',  ( 192.8011239859581849, 296.7056528303708660, -11.79847971295421694 ) ) ;
#83446=CARTESIAN_POINT ( 'NONE',  ( 192.4172326059820648, 297.3705722050773943, -12.52563289807247848 ) ) ;
#83447=CARTESIAN_POINT ( 'NONE',  ( 149.3141802193904368, 272.0272488999566463, -11.40332369054239336 ) ) ;
#83448=VERTEX_POINT ( 'NONE', #12738 ) ;
#83449=B_SPLINE_CURVE_WITH_KNOTS ( 'NONE', 3,
 ( #73104, #43659, #80225, #74089 ),
 .UNSPECIFIED., .F., .F.,
 ( 4, 4 ),
 ( 0.01057430845927626734, 0.01607705855292669225 ),
 .UNSPECIFIED. ) ;
#83452=CARTESIAN_POINT ( 'NONE',  ( 157.5046580301597032, 268.7583167102267794, 15.65051971689831589 ) ) ;
#83454=CARTESIAN_POINT ( 'NONE',  ( 173.1833192663806926, 253.4864516599578792, -9.233729552024655618 ) ) ;
#83455=CARTESIAN_POINT ( 'NONE',  ( 138.6583583033484786, 260.8615022471902876, 5.000000000000046185 ) ) ;
#83456=ORIENTED_EDGE ( 'NONE', *, *, #28685, .T. ) ;
#83459=CARTESIAN_POINT ( 'NONE',  ( 163.1691520398773321, 248.0297337694385931, 11.21816141384514331 ) ) ;
#83462=ORIENTED_EDGE ( 'NONE', *, *, #1452, .T. ) ;
#83463=CARTESIAN_POINT ( 'NONE',  ( 184.7176300103652125, 293.6802179342421937, -10.75420723427517977 ) ) ;
#83465=DIRECTION ( 'NONE',  ( -0.8660254037844387076, -0.4999999999999998890, -0.000000000000000000 ) ) ;
#83467=CARTESIAN_POINT ( 'NONE',  ( 190.8725948953614591, 278.0229128820462279, -17.51817159285709025 ) ) ;
#83468=DIRECTION ( 'NONE',  ( 0.4999999999999998890, -0.8660254037844385966, 0.000000000000000000 ) ) ;
#83469=B_SPLINE_CURVE_WITH_KNOTS ( 'NONE', 3,
 ( #83924, #91512, #60062, #75304 ),
 .UNSPECIFIED., .F., .F.,
 ( 4, 4 ),
 ( 0.01804370536616622250, 0.02702473640048589851 ),
 .UNSPECIFIED. ) ;
#83470=CARTESIAN_POINT ( 'NONE',  ( 152.6692142062575499, 266.2161595735824449, -16.77985299603479419 ) ) ;
#83474=CARTESIAN_POINT ( 'NONE',  ( 178.1281481821618797, 292.9991590599575488, -6.064681374715556572 ) ) ;
#83478=ORIENTED_EDGE ( 'NONE', *, *, #3177, .F. ) ;
#83483=CARTESIAN_POINT ( 'NONE',  ( 165.9617581993362023, 274.1071786095166090, -15.17248422297432420 ) ) ;
#83484=CARTESIAN_POINT ( 'NONE',  ( 206.1569797555946195, 273.5726320587986038, -9.753408447412784454 ) ) ;
#83485=CARTESIAN_POINT ( 'NONE',  ( 198.3132153568068929, 273.7169797895816714, -13.42874499935994237 ) ) ;
#83487=CARTESIAN_POINT ( 'NONE',  ( 147.6618183892331331, 274.8892235422768522, 8.990680574201936892 ) ) ;
#83488=CARTESIAN_POINT ( 'NONE',  ( 170.5177250007984640, 288.6921495108791760, -4.130607863702036475 ) ) ;
#83490=CARTESIAN_POINT ( 'NONE',  ( 186.6577945393187008, 286.8565254842017112, -15.55016485953022176 ) ) ;
#83491=CARTESIAN_POINT ( 'NONE',  ( 121.2028808523094767, 228.5327760586659451, 1.948934522072303157E-15 ) ) ;
#83493=CARTESIAN_POINT ( 'NONE',  ( 183.5821904726393825, 260.0513847542609938, -9.557056484130177054 ) ) ;
#83495=CARTESIAN_POINT ( 'NONE',  ( 191.9642392354410561, 293.3079686636485803, -14.67799312013193003 ) ) ;
#83500=CARTESIAN_POINT ( 'NONE',  ( 164.9359911487327963, 246.1719262986664489, -2.773572180244460839 ) ) ;
#83501=CARTESIAN_POINT ( 'NONE',  ( 195.8449251089225811, 291.4336346372613775, 16.14492769602857081 ) ) ;
#83506=AXIS2_PLACEMENT_3D ( 'NONE', #31034, #76173, #38629 ) ;
#83507=CARTESIAN_POINT ( 'NONE',  ( 148.7194274992590408, 273.0573908291643761, 9.629271269182392956 ) ) ;
#83508=EDGE_CURVE ( 'NONE', #44920, #50293, #24996, .T. ) ;
#83513=CARTESIAN_POINT ( 'NONE',  ( 206.5318754762992910, 272.9232936229979032, 10.63244694018452741 ) ) ;
#83514=CARTESIAN_POINT ( 'NONE',  ( 195.9012476844455364, 265.0396910272671676, 3.914111099667014759 ) ) ;
#83515=CARTESIAN_POINT ( 'NONE',  ( 158.4641270891539193, 263.4220271406156826, 17.63380002636472810 ) ) ;
#83517=CYLINDRICAL_SURFACE ( 'NONE', #77588, 10.00000000000010658 ) ;
#83519=CARTESIAN_POINT ( 'NONE',  ( 201.2949053258274148, 281.9939920013367782, -18.04004790210578335 ) ) ;
#83521=CARTESIAN_POINT ( 'NONE',  ( 146.8358616138309571, 276.3198226421291679, 4.054088818585255716 ) ) ;
#83522=CARTESIAN_POINT ( 'NONE',  ( 52.15148940044955594, 212.4637435831425307, 2.679491924311251605 ) ) ;
#83524=CARTESIAN_POINT ( 'NONE',  ( 192.8922468175501876, 270.9615889258991501, 14.61616359823144506 ) ) ;
#83525=CARTESIAN_POINT ( 'NONE',  ( 189.2695117162384122, 270.1846877967625460, -14.08055865318978839 ) ) ;
#83526=CARTESIAN_POINT ( 'NONE',  ( 154.6982851380984130, 273.6571292083216349, -13.42362762759460892 ) ) ;
#83528=CARTESIAN_POINT ( 'NONE',  ( 59.27500801855438795, 193.4824982072973683, 3.021315404115420679E-15 ) ) ;
#83529=CARTESIAN_POINT ( 'NONE',  ( 155.4917600441137324, 261.3273667757233056, 17.14261720787171939 ) ) ;
#83530=CARTESIAN_POINT ( 'NONE',  ( 191.4336085427262333, 282.7786862010840423, -17.53248462874352498 ) ) ;
#83531=EDGE_CURVE ( 'NONE', #19194, #92966, #93948, .T. ) ;
#83533=CARTESIAN_POINT ( 'NONE',  ( 73.95019621043853419, 207.3768266524160140, 9.188101187500098632 ) ) ;
#83534=CARTESIAN_POINT ( 'NONE',  ( 206.7680519836501958, 272.5142239127119979, -10.57935479673322021 ) ) ;
#83536=LINE ( 'NONE', #22195, #36510 ) ;
#83540=CARTESIAN_POINT ( 'NONE',  ( 207.1572261440131797, 271.8401544939704877, -5.633070628900782140 ) ) ;
#83546=CARTESIAN_POINT ( 'NONE',  ( 149.7503540259411068, 272.3885311082809153, -11.42439314646132509 ) ) ;
#83550=CARTESIAN_POINT ( 'NONE',  ( 26.10194555558328133, 192.0024278399160949, -9.188101187500093303 ) ) ;
#83551=CARTESIAN_POINT ( 'NONE',  ( 196.3519702320103590, 290.5554067223432639, 17.39042812051341969 ) ) ;
#83555=CARTESIAN_POINT ( 'NONE',  ( 55.14129374593650113, 193.4548013555410080, -4.594050593750042211 ) ) ;
#83558=CARTESIAN_POINT ( 'NONE',  ( 199.1867231605587278, 285.6454706231928071, -17.41989184023605475 ) ) ;
#83559=CARTESIAN_POINT ( 'NONE',  ( 196.7823306783968746, 289.8100005636337073, -17.85370042640856170 ) ) ;
#83562=CARTESIAN_POINT ( 'NONE',  ( 159.4072785079408732, 255.6537108709859183, -16.22214289272363175 ) ) ;
#83563=CARTESIAN_POINT ( 'NONE',  ( 175.5651479323515787, 291.1351013291215395, 2.181378784527221448 ) ) ;
#83567=CARTESIAN_POINT ( 'NONE',  ( 153.0305350670531936, 277.3750776671890890, 8.290292975357761662 ) ) ;
#83568=CARTESIAN_POINT ( 'NONE',  ( 163.3837300346235395, 255.8040548010872612, -14.83920063947459056 ) ) ;
#83571=CARTESIAN_POINT ( 'NONE',  ( 97.88299554183124940, 213.9865022471901455, 1.119607411625061291E-15 ) ) ;
#83572=CARTESIAN_POINT ( 'NONE',  ( 161.1990332043106946, 251.4420796895884394, 14.26998817770995487 ) ) ;
#83573=CARTESIAN_POINT ( 'NONE',  ( 164.8753104327445271, 270.4778681372466735, -17.27537531252914249 ) ) ;
#83575=CARTESIAN_POINT ( 'NONE',  ( 64.58612298413676456, 208.0958772461660544, -9.188101187500095079 ) ) ;
#83577=CARTESIAN_POINT ( 'NONE',  ( 178.5460542442402527, 263.4982612806743987, 15.38449660858491441 ) ) ;
#83578=CARTESIAN_POINT ( 'NONE',  ( 161.5959287003499583, 251.1472748658742944, 12.79373419553940749 ) ) ;
#83579=DIRECTION ( 'NONE',  ( 0.4999999999999998890, -0.8660254037844385966, 0.000000000000000000 ) ) ;
#83580=ORIENTED_EDGE ( 'NONE', *, *, #66203, .T. ) ;
#83585=CARTESIAN_POINT ( 'NONE',  ( 204.7462429809936282, 276.0160998285135179, 13.10238900943261342 ) ) ;
#83590=CARTESIAN_POINT ( 'NONE',  ( 201.1893450866852504, 280.1768276987904756, -16.82388990131531870 ) ) ;
#83592=CARTESIAN_POINT ( 'NONE',  ( 180.8586690819065552, 283.2892246925316044, 14.99098275897606314 ) ) ;
#83593=CARTESIAN_POINT ( 'NONE',  ( 159.5050723400634638, 254.3761059724978679, -15.34938048045353298 ) ) ;
#83594=ORIENTED_EDGE ( 'NONE', *, *, #62756, .T. ) ;
#83598=CARTESIAN_POINT ( 'NONE',  ( 207.5959034698703078, 271.0803430774575418, -1.830000129038042544 ) ) ;
#83599=CARTESIAN_POINT ( 'NONE',  ( 163.8990931530087494, 246.7654386749614162, 5.873176884778091633 ) ) ;
#83600=CARTESIAN_POINT ( 'NONE',  ( 198.6562788533279615, 286.5642271139020636, 17.47134757795404525 ) ) ;
#83602=CARTESIAN_POINT ( 'NONE',  ( 177.8194257969418288, 292.8449071177858514, 6.006967295066290013 ) ) ;
#83604=CARTESIAN_POINT ( 'NONE',  ( 127.2647115830355347, 244.2833772461660544, -9.188101187500095079 ) ) ;
#83605=DIRECTION ( 'NONE',  ( -0.8660254037844359321, -0.5000000000000051070, -0.000000000000000000 ) ) ;
#83606=CARTESIAN_POINT ( 'NONE',  ( 73.95019621043853419, 207.3768266524160140, 9.188101187500098632 ) ) ;
#83608=CARTESIAN_POINT ( 'NONE',  ( 170.2399125551612258, 264.0282869839934961, 16.04968556189760776 ) ) ;
#83615=VERTEX_POINT ( 'NONE', #82163 ) ;
#83618=CARTESIAN_POINT ( 'NONE',  ( 197.4340835798049625, 286.5481627907838060, 16.91565206045372705 ) ) ;
#83619=CARTESIAN_POINT ( 'NONE',  ( 147.1731211915891322, 275.7356719181125868, 0.5879280619134324981 ) ) ;
#83622=CARTESIAN_POINT ( 'NONE',  ( 194.5051734451974426, 293.7541525883582381, 14.61790433731063921 ) ) ;
#83627=EDGE_LOOP ( 'NONE', ( #85781, #16425, #33246, #43834 ) ) ;
#83630=CARTESIAN_POINT ( 'NONE',  ( 162.0336139374437323, 249.9965434567837974, -13.69905126395175365 ) ) ;
#83636=CARTESIAN_POINT ( 'NONE',  ( 147.4298066744680398, 275.2910796202013444, -3.046391898894023953 ) ) ;
#83637=CARTESIAN_POINT ( 'NONE',  ( 173.4505375608857491, 284.9503170016366198, -13.05978560202663452 ) ) ;
#83638=AXIS2_PLACEMENT_3D ( 'NONE', #55329, #93385, #92880 ) ;
#83639=CARTESIAN_POINT ( 'NONE',  ( 196.3432621239062712, 279.8021363881798038, 16.39655255723854665 ) ) ;
#83641=CARTESIAN_POINT ( 'NONE',  ( 141.2025682470151366, 243.1423013555409796, -4.594050593750043987 ) ) ;
#83647=VECTOR ( 'NONE', #22889, 1000.000000000000000 ) ;
#83650=ORIENTED_EDGE ( 'NONE', *, *, #77163, .T. ) ;
#83651=CARTESIAN_POINT ( 'NONE',  ( 199.5713953663193934, 266.2439827736556026, 4.749567076163869750 ) ) ;
#83653=CARTESIAN_POINT ( 'NONE',  ( 181.5127903015804236, 292.0923642003480154, 10.55878241066769441 ) ) ;
#83656=CARTESIAN_POINT ( 'NONE',  ( 198.7494054154245191, 266.3724082695370043, 0.8279625511378244651 ) ) ;
#83657=CARTESIAN_POINT ( 'NONE',  ( 198.5172889092661990, 266.1891015951424606, 0.5731995804530348737 ) ) ;
#83658=CARTESIAN_POINT ( 'NONE',  ( 190.9586609929293104, 299.8968923453624598, -4.970176667899034229 ) ) ;
#83659=CARTESIAN_POINT ( 'NONE',  ( 186.5691198594528259, 282.5508937948688981, 16.19376103776746945 ) ) ;
#83660=B_SPLINE_CURVE_WITH_KNOTS ( 'NONE', 3,
 ( #371, #60646, #91114, #91602, #5974, #100192 ),
 .UNSPECIFIED., .F., .F.,
 ( 4, 2, 4 ),
 ( 0.02174174018087433186, 0.02633378460584469630, 0.03092582903081506074 ),
 .UNSPECIFIED. ) ;
#83661=CARTESIAN_POINT ( 'NONE',  ( 158.1587942607527850, 261.9516103332310308, -17.82285333032626795 ) ) ;
#83662=CARTESIAN_POINT ( 'NONE',  ( 168.9677593865781944, 262.6396129170871632, -17.12250179939312389 ) ) ;
#83665=CARTESIAN_POINT ( 'NONE',  ( 205.0150392401225758, 274.4627107821886511, 11.80085037109421719 ) ) ;
#83667=CARTESIAN_POINT ( 'NONE',  ( 198.3523905153085423, 287.0905771551796306, 18.52598547438866206 ) ) ;
#83669=CARTESIAN_POINT ( 'NONE',  ( 141.4548986661878303, 259.1427522451419350, 10.00000000000009237 ) ) ;
#83670=CARTESIAN_POINT ( 'NONE',  ( 182.3178896938217122, 278.5243308997074791, 17.63982057706049389 ) ) ;
#83674=CARTESIAN_POINT ( 'NONE',  ( 202.4863134139235967, 273.9910293909178449, -13.09725697524322996 ) ) ;
#83675=CARTESIAN_POINT ( 'NONE',  ( 199.1526122334580862, 285.7045524820243259, -17.32174362185583050 ) ) ;
#83676=CARTESIAN_POINT ( 'NONE',  ( 8.727484440040480962, 175.8458772461660828, 9.188101187500095079 ) ) ;
#83678=ADVANCED_FACE ( 'NONE', ( #43087 ), #4618, .T. ) ;
#83681=CARTESIAN_POINT ( 'NONE',  ( 170.1129511229850948, 270.7127029815443393, -17.04003866544655921 ) ) ;
#83684=CYLINDRICAL_SURFACE ( 'NONE', #15117, 17.82106496071139645 ) ;
#83686=CARTESIAN_POINT ( 'NONE',  ( 198.6455782124543248, 286.5827611675690605, 17.19551065434971093 ) ) ;
#83688=CARTESIAN_POINT ( 'NONE',  ( 49.38557292990258674, 205.9865022471902876, 10.00000000000009237 ) ) ;
#83689=CARTESIAN_POINT ( 'NONE',  ( -22.42236680055709641, 157.8615022471902591, 0.000000000000000000 ) ) ;
#83690=CARTESIAN_POINT ( 'NONE',  ( 190.6084209867335915, 300.5035258309363826, -0.5505750481748228342 ) ) ;
#83691=CARTESIAN_POINT ( 'NONE',  ( 15.76359375002403596, 192.1589784336661637, -6.496448406907675876E-16 ) ) ;
#83696=CARTESIAN_POINT ( 'NONE',  ( 136.2587462434812267, 256.1427522451419350, 10.00000000000009415 ) ) ;
#83698=CARTESIAN_POINT ( 'NONE',  ( 189.1862045837368385, 268.2028127389427254, 13.82493371562940432 ) ) ;
#83699=CYLINDRICAL_SURFACE ( 'NONE', #8914, 10.00000000000010658 ) ;
#83700=CARTESIAN_POINT ( 'NONE',  ( 164.1989670955858571, 281.5052563180250900, 9.464287345521309902 ) ) ;
#83702=CARTESIAN_POINT ( 'NONE',  ( 148.3280470635002928, 273.7352816289870248, 9.058704604771318003 ) ) ;
#83704=CARTESIAN_POINT ( 'NONE',  ( 187.0083344850037008, 268.0836409071914090, -15.22627500120235133 ) ) ;
#83705=VERTEX_POINT ( 'NONE', #53200 ) ;
#83706=CIRCLE ( 'NONE', #57768, 17.82106496071138935 ) ;
#83711=ORIENTED_EDGE ( 'NONE', *, *, #90057, .F. ) ;
#83713=CARTESIAN_POINT ( 'NONE',  ( -17.42236680055705023, 149.2012482093457777, 0.000000000000000000 ) ) ;
#83715=CARTESIAN_POINT ( 'NONE',  ( 154.9903553346911735, 262.1958252075976361, -18.39016733948542637 ) ) ;
#83718=AXIS2_PLACEMENT_3D ( 'NONE', #22596, #69186, #60079 ) ;
#83719=CARTESIAN_POINT ( 'NONE',  ( 190.6688270659779221, 284.0946164064107506, -17.60360843008351495 ) ) ;
#83721=ORIENTED_EDGE ( 'NONE', *, *, #94341, .F. ) ;
#83722=CARTESIAN_POINT ( 'NONE',  ( 153.2513309553138470, 265.2079037882803618, -16.24091495603130397 ) ) ;
#83725=CARTESIAN_POINT ( 'NONE',  ( 47.05812965368398437, 204.6427522451419350, -10.00000000000009592 ) ) ;
#83727=FACE_OUTER_BOUND ( 'NONE', #55353, .T. ) ;
#83728=ORIENTED_EDGE ( 'NONE', *, *, #74265, .T. ) ;
#83729=CARTESIAN_POINT ( 'NONE',  ( 165.0538309624641613, 244.7653741195639157, 2.311334310144196547 ) ) ;
#83733=CARTESIAN_POINT ( 'NONE',  ( 190.4841013044967042, 300.7188538369516095, 4.682298117523464143 ) ) ;
#83735=ORIENTED_EDGE ( 'NONE', *, *, #52335, .F. ) ;
#83737=CARTESIAN_POINT ( 'NONE',  ( 25.50001727096127979, 173.9824982072973967, 3.021315404115420679E-15 ) ) ;
#83741=VERTEX_POINT ( 'NONE', #76990 ) ;
#83742=CARTESIAN_POINT ( 'NONE',  ( 155.5487322651507043, 265.9491453245429398, -16.30937882781046611 ) ) ;
#83743=CARTESIAN_POINT ( 'NONE',  ( 147.3984236761635884, 275.3454365677582700, 5.108566646342994844 ) ) ;
#83744=CARTESIAN_POINT ( 'NONE',  ( 190.3049670482083684, 301.0291234702190764, 0.2225066852051815758 ) ) ;
#83745=CARTESIAN_POINT ( 'NONE',  ( 190.0707697440390689, 301.4347651000360884, 4.271360729158901748 ) ) ;
#83746=CARTESIAN_POINT ( 'NONE',  ( 192.6797324865049745, 296.9159090750308110, 12.42053959885222625 ) ) ;
#83748=FACE_OUTER_BOUND ( 'NONE', #11116, .T. ) ;
#83754=CARTESIAN_POINT ( 'NONE',  ( 85.81045474425822306, 231.8967562850347122, -4.648177544792955347E-16 ) ) ;
#83759=ORIENTED_EDGE ( 'NONE', *, *, #66712, .T. ) ;
#83762=CARTESIAN_POINT ( 'NONE',  ( 149.4596969528118393, 273.7752065243203106, 10.43958276706939614 ) ) ;
#83764=CARTESIAN_POINT ( 'NONE',  ( 192.0122163493551284, 297.6569496777016752, -9.909203487807042521 ) ) ;
#83766=CARTESIAN_POINT ( 'NONE',  ( 169.3013571053814132, 285.1638214189113114, -7.896588100169458890 ) ) ;
#83768=CARTESIAN_POINT ( 'NONE',  ( 170.0174658539383188, 255.2014620101463720, -11.63331499112131873 ) ) ;
#83770=CARTESIAN_POINT ( 'NONE',  ( 159.2536436069973718, 254.8115933126508992, -15.76697951715411250 ) ) ;
#83772=CARTESIAN_POINT ( 'NONE',  ( 39.26390101962404344, 200.1427522451419350, -10.00000000000009415 ) ) ;
#83773=CARTESIAN_POINT ( 'NONE',  ( 110.0524566828198232, 234.3458772461660544, 9.188101187500095079 ) ) ;
#83776=CARTESIAN_POINT ( 'NONE',  ( 195.8449251089225811, 291.4336346372613775, 16.14492769602857081 ) ) ;
#83777=CARTESIAN_POINT ( 'NONE',  ( 175.4589951177797218, 253.5542521767871165, -4.185393656649594618 ) ) ;
#83778=CARTESIAN_POINT ( 'NONE',  ( 34.70824655357364463, 190.8458772461660544, 9.188101187500095079 ) ) ;
#83782=CARTESIAN_POINT ( 'NONE',  ( 191.1855593189403635, 298.9439214236015232, 7.483141010870764553 ) ) ;
#83783=CARTESIAN_POINT ( 'NONE',  ( 181.3202242451768598, 267.7749618620028969, 14.98405922250201705 ) ) ;
#83788=CARTESIAN_POINT ( 'NONE',  ( 182.2306686641913132, 262.8049073495537300, 12.70932774860379411 ) ) ;
#83790=CARTESIAN_POINT ( 'NONE',  ( 98.22579726061456995, 237.5177522451419350, 5.000000000000046185 ) ) ;
#83792=CARTESIAN_POINT ( 'NONE',  ( 198.5886434392601529, 267.8836247115091851, -8.069141051336366388 ) ) ;
#83793=B_SPLINE_CURVE_WITH_KNOTS ( 'NONE', 3,
 ( #90586, #59605, #99637, #45892, #75346, #83967, #43916, #14027, #6434, #53509, #21151, #76815, #67729, #29237, #74855, #5437, #44908, #30219, #75849, #82970, #38302, #37312, #82492, #76342, #84463, #68712, #68212, #60103, #5927, #13544, #36318, #22122, #91069, #99137, #6916, #29724, #53014, #69211, #21632, #37803, #52514, #14531, #83463, #45410 ),
 .UNSPECIFIED., .F., .F.,
 ( 4, 2, 2, 2, 2, 2, 2, 2, 2, 2, 2, 2, 2, 2, 2, 2, 2, 2, 2, 2, 2, 4 ),
 ( 0.002160350574709204823, 0.002597591355362379503, 0.002816211745688940171, 0.003034832136015500406, 0.003144142331178779223, 0.003253452526342058039, 0.003362762721505337289, 0.003472072916668616106, 0.003909313697321794255, 0.004783795258628099380, 0.005658276819934403637, 0.006532758381240707894, 0.006969999161893860457, 0.007407239942547013019, 0.007516550137710215941, 0.007571205235291765361, 0.007625860332873313913, 0.007735170528036391935, 0.007844480723199469957, 0.008281721503852156746, 0.008718962284504843535, 0.009156203065157532059 ),
 .UNSPECIFIED. ) ;
#83794=CARTESIAN_POINT ( 'NONE',  ( 156.8729383767137904, 280.5345233313491349, -1.585272415347215080 ) ) ;
#83795=CARTESIAN_POINT ( 'NONE',  ( 154.7326666781059714, 263.9299083186784287, 17.15468183873104735 ) ) ;
#83797=CARTESIAN_POINT ( 'NONE',  ( 16.84647260051960060, 180.5333772461660544, 9.188101187500095079 ) ) ;
#83799=CARTESIAN_POINT ( 'NONE',  ( 196.1666432693615718, 273.5625105224574440, 15.08246463373486002 ) ) ;
#83802=CARTESIAN_POINT ( 'NONE',  ( 174.5805834809822557, 286.5546214993515832, 10.25926391534427751 ) ) ;
#83803=CARTESIAN_POINT ( 'NONE',  ( 63.96340690334295687, 216.9244531367911293, -4.594050593750046652 ) ) ;
#83804=EDGE_CURVE ( 'NONE', #45170, #86137, #74176, .T. ) ;
#83805=CARTESIAN_POINT ( 'NONE',  ( 208.1876422586379647, 270.0554214305024630, 3.377638779759113863 ) ) ;
#83810=CARTESIAN_POINT ( 'NONE',  ( 19.21902136474470524, 175.2365022471902023, 10.00000000000009592 ) ) ;
#83811=CARTESIAN_POINT ( 'NONE',  ( 163.8455942243524248, 246.8581015375447691, -7.178103170949780676 ) ) ;
#83812=CARTESIAN_POINT ( 'NONE',  ( 139.7141738582018604, 239.2202760586659736, -5.415160957724236172E-17 ) ) ;
#83814=CARTESIAN_POINT ( 'NONE',  ( 207.0452084649157314, 272.0341748055130324, -8.323635130805319804 ) ) ;
#83819=CARTESIAN_POINT ( 'NONE',  ( 167.0546803224166297, 282.1702852132879684, 12.27869116404093752 ) ) ;
#83824=CARTESIAN_POINT ( 'NONE',  ( 180.9536487871291968, 287.8037316094353741, 14.06327251346537288 ) ) ;
#83825=CARTESIAN_POINT ( 'NONE',  ( 156.6568488211063936, 280.3666888851813610, -5.413563403562074328 ) ) ;
#83826=CARTESIAN_POINT ( 'NONE',  ( 197.0727265385168607, 273.0519042339707312, -13.37462020030573484 ) ) ;
#83827=VERTEX_POINT ( 'NONE', #10105 ) ;
#83828=CARTESIAN_POINT ( 'NONE',  ( 160.1202562673349803, 253.3105761544636039, 14.69629115143539266 ) ) ;
#83829=VECTOR ( 'NONE', #87998, 1000.000000000000000 ) ;
#83830=CARTESIAN_POINT ( 'NONE',  ( 170.7822565925250160, 283.8216418346244723, -11.11151730791865511 ) ) ;
#83831=B_SPLINE_SURFACE_WITH_KNOTS ( 'NONE', 3, 1, ( 
 ( #1133, #41105 ),
 ( #17320, #16324 ),
 ( #25419, #47217 ),
 ( #9227, #62920 ),
 ( #2644, #25943 ),
 ( #2139, #48225 ),
 ( #71046, #32532 ),
 ( #87308, #63426 ),
 ( #56818, #24919 ),
 ( #55793, #33022 ),
 ( #40611, #56312 ),
 ( #63920, #17841 ),
 ( #48742, #79674 ),
 ( #87801, #97347 ),
 ( #27913, #57316 ),
 ( #73535, #65422 ),
 ( #97838, #66909 ),
 ( #59287, #41611 ),
 ( #82169, #96365 ),
 ( #12744, #36004 ),
 ( #88286, #96868 ),
 ( #95879, #80676 ),
 ( #28407, #18840 ),
 ( #49720, #50218 ),
 ( #81172, #11737 ),
 ( #11252, #42115 ),
 ( #26931, #42601 ),
 ( #35011, #65911 ),
 ( #58310, #73049 ),
 ( #3642, #89764 ),
 ( #81660, #26437 ),
 ( #4116, #80170 ),
 ( #34523, #57810 ),
 ( #88789, #49236 ) ),
 .UNSPECIFIED., .T., .F., .F.,
 ( 4, 2, 2, 2, 2, 2, 2, 2, 2, 2, 2, 2, 2, 2, 2, 2, 4 ),
 ( 2, 2 ),
 ( 0.000000000000000000, 0.06250000000000000000, 0.1250000000000000000, 0.1875000000000000000, 0.2500000000000000000, 0.3125000000000000000, 0.3750000000000000000, 0.4375000000000000000, 0.5000000000000000000, 0.5625000000000000000, 0.6250000000000000000, 0.6875000000000000000, 0.7500000000000000000, 0.8125000000000000000, 0.8750000000000000000, 0.9375000000000000000, 1.000000000000000000 ),
 ( 0.000000000000000000, 1.000000000000000000 ),
 .UNSPECIFIED. ) ;
#83833=CARTESIAN_POINT ( 'NONE',  ( 200.6945232828033738, 282.6247322300178553, -16.66035973746479826 ) ) ;
#83834=FACE_OUTER_BOUND ( 'NONE', #23765, .T. ) ;
#83835=CARTESIAN_POINT ( 'NONE',  ( 32.33569778934854355, 196.1427522451419065, 10.00000000000009415 ) ) ;
#83836=CARTESIAN_POINT ( 'NONE',  ( 208.2874212803407090, 269.8825990953837390, -1.143705256421198690 ) ) ;
#83837=CARTESIAN_POINT ( 'NONE',  ( 201.4617167010348737, 281.7050662241970826, -17.43131506460443703 ) ) ;
#83839=ORIENTED_EDGE ( 'NONE', *, *, #59767, .F. ) ;
#83844=CARTESIAN_POINT ( 'NONE',  ( 148.9275518150011806, 272.6969089400084272, 12.34519124974546500 ) ) ;
#83846=CARTESIAN_POINT ( 'NONE',  ( 189.0627537881084379, 297.0799250450181148, 8.091751816178462064 ) ) ;
#83847=EDGE_LOOP ( 'NONE', ( #7670, #36738, #1198, #43161 ) ) ;
#83851=CARTESIAN_POINT ( 'NONE',  ( 164.1224127655298730, 246.3786377597482158, 7.356982420601481998 ) ) ;
#83854=CARTESIAN_POINT ( 'NONE',  ( 97.65764163903753570, 221.0643266524160424, 9.188101187500095079 ) ) ;
#83855=CARTESIAN_POINT ( 'NONE',  ( 203.1289230791707325, 278.8173800705629901, 16.48573034889792766 ) ) ;
#83856=CARTESIAN_POINT ( 'NONE',  ( 170.7953178271928039, 255.2457615276028093, -12.92277808742838374 ) ) ;
#83857=CARTESIAN_POINT ( 'NONE',  ( 180.9057600473689149, 270.9297146850697686, -15.98331193678458106 ) ) ;
#83869=ADVANCED_FACE ( 'NONE', ( #24788 ), #32398, .T. ) ;
#83870=CARTESIAN_POINT ( 'NONE',  ( 164.4578252119609090, 245.7976863610386999, -6.211333091911165560 ) ) ;
#83872=CARTESIAN_POINT ( 'NONE',  ( 170.6484802770005729, 282.9697387111801845, 11.87827476712554997 ) ) ;
#83873=CARTESIAN_POINT ( 'NONE',  ( 142.4134467818605572, 241.4824982072973967, 3.021315404115420679E-15 ) ) ;
#83879=CARTESIAN_POINT ( 'NONE',  ( 164.4771589409865555, 281.7954605369791921, 8.842136975255975528 ) ) ;
#83884=CARTESIAN_POINT ( 'NONE',  ( 53.17212233558426959, 213.0530062829863311, -4.648177544792955347E-16 ) ) ;
#83885=CARTESIAN_POINT ( 'NONE',  ( 185.1676822857243963, 258.5668278037668983, 2.933763201912603424 ) ) ;
#83886=CARTESIAN_POINT ( 'NONE',  ( 160.6907952011062264, 281.0816080609710639, -6.606445984059675425 ) ) ;
#83887=CARTESIAN_POINT ( 'NONE',  ( 165.8568044060308182, 246.3531759204054481, -2.743205800353976542 ) ) ;
#83888=CARTESIAN_POINT ( 'NONE',  ( 192.7705046643033313, 292.1170781437433561, -14.65601932715136435 ) ) ;
#83889=CARTESIAN_POINT ( 'NONE',  ( 171.3768758103641972, 255.5877274061340643, 11.19587476605279441 ) ) ;
#83890=CARTESIAN_POINT ( 'NONE',  ( 193.5872375690405534, 263.2763237561280221, -0.7636422199292929314 ) ) ;
#83892=CARTESIAN_POINT ( 'NONE',  ( 155.7133958608191620, 260.9434822804128657, -18.28034026974484405 ) ) ;
#83895=CARTESIAN_POINT ( 'NONE',  ( 6.860117161356369841, 164.7677522451418213, -5.000000000000041744 ) ) ;
#83897=CARTESIAN_POINT ( 'NONE',  ( 173.7861983198416453, 280.7065551239853107, -14.21705231541378467 ) ) ;
#83898=CARTESIAN_POINT ( 'NONE',  ( 163.9733507041129883, 246.6368208236034718, -8.809407376596537276 ) ) ;
#83902=CARTESIAN_POINT ( 'NONE',  ( -2.963858511049441979, 169.0958772461660544, -9.188101187500095079 ) ) ;
#83903=CARTESIAN_POINT ( 'NONE',  ( -6.583630525541995127, 178.5530062829863027, -4.648177544792955347E-16 ) ) ;
#83904=CARTESIAN_POINT ( 'NONE',  ( 185.0534184758703873, 295.4269076067080846, 8.465056994707534699 ) ) ;
#83907=ORIENTED_EDGE ( 'NONE', *, *, #62585, .T. ) ;
#83908=CARTESIAN_POINT ( 'NONE',  ( -27.42236680055714260, 166.5217562850347406, 1.224646799147364892E-15 ) ) ;
#83912=CARTESIAN_POINT ( 'NONE',  ( 162.4934061880776426, 249.2001599177594073, -11.48506854272206290 ) ) ;
#83915=CARTESIAN_POINT ( 'NONE',  ( 153.3856580278162198, 278.7073591447287413, 3.760990798762666731 ) ) ;
#83916=CARTESIAN_POINT ( 'NONE',  ( 17.63104780087548562, 190.1744531367911293, 4.594050593750047540 ) ) ;
#83917=CARTESIAN_POINT ( 'NONE',  ( 127.4544149619371609, 235.2048013555409796, 4.594050593750051981 ) ) ;
#83924=CARTESIAN_POINT ( 'NONE',  ( 190.7982574810033611, 262.8194055429554510, 8.405793748174573921 ) ) ;
#83925=CARTESIAN_POINT ( 'NONE',  ( 207.8984236726843164, 270.5563627158673512, -6.084369154771423815 ) ) ;
#83927=CARTESIAN_POINT ( 'NONE',  ( 167.8450657302246896, 278.1957396450247302, 14.42841292292709809 ) ) ;
#83928=CARTESIAN_POINT ( 'NONE',  ( -1.387478102835363769, 181.5530062829863596, 2.649461200531984646E-14 ) ) ;
#83930=CARTESIAN_POINT ( 'NONE',  ( 184.2244543100441376, 268.3421717558753699, -15.77288757490104665 ) ) ;
#83933=CARTESIAN_POINT ( 'NONE',  ( 184.8899540568645534, 269.3660042897924427, 16.00930444126497321 ) ) ;
#83934=CARTESIAN_POINT ( 'NONE',  ( 86.23641098298274699, 232.8464784336661353, 1.353441290958777327E-15 ) ) ;
#83941=CARTESIAN_POINT ( 'NONE',  ( 196.4184597338679339, 290.4402435269564080, 17.72466505881568821 ) ) ;
#83942=CARTESIAN_POINT ( 'NONE',  ( 173.9076247008792393, 277.9417859016587045, -16.84130823774900776 ) ) ;
#83943=FACE_OUTER_BOUND ( 'NONE', #28885, .T. ) ;
#83946=CARTESIAN_POINT ( 'NONE',  ( 127.6706609892855369, 244.5177522451418497, -10.00000000000009592 ) ) ;
#83951=CARTESIAN_POINT ( 'NONE',  ( 146.9370072200009645, 276.1446333132804511, -3.799807221059707363 ) ) ;
#83953=( BOUNDED_CURVE ( )  B_SPLINE_CURVE ( 2, ( #43652, #75077, #27957, #29458, #76087, #44143, #89805, #20884, #74084 ),
 .UNSPECIFIED., .F., .F. ) 
 B_SPLINE_CURVE_WITH_KNOTS ( ( 3, 2, 2, 2, 3 ),
 ( 0.8266129032258064946, 0.8279569892473118697, 0.8306451612903226200, 0.8333333333333333703, 0.8346774193548387455 ),
 .UNSPECIFIED. ) 
 CURVE ( )  GEOMETRIC_REPRESENTATION_ITEM ( )  RATIONAL_B_SPLINE_CURVE ( ( 0.9330127018922194093, 0.9330127018922194093, 1.000000000000000000, 0.8660254037844387076, 1.000000000000000000, 0.8660254037844387076, 1.000000000000000000, 0.9330127018922194093, 0.9330127018922194093 ) ) 
 REPRESENTATION_ITEM ( '' )  );
#83954=EDGE_CURVE ( 'NONE', #55638, #47161, #61508, .T. ) ;
#83956=CARTESIAN_POINT ( 'NONE',  ( 159.9880386575927957, 253.5395837721924863, 15.85893018594752846 ) ) ;
#83957=CARTESIAN_POINT ( 'NONE',  ( 179.8857559909177155, 262.7895619565915695, -12.79994536760057855 ) ) ;
#83958=CARTESIAN_POINT ( 'NONE',  ( 173.2449941322521170, 253.6062056627853565, -9.189074487664372626 ) ) ;
#83959=CARTESIAN_POINT ( 'NONE',  ( 152.6945189806187955, 266.1723304187151484, 16.62409282110771613 ) ) ;
#83960=B_SPLINE_CURVE_WITH_KNOTS ( 'NONE', 3,
 ( #78943, #56607, #49021, #34311, #11031, #79954, #17618, #2433, #33835, #19139, #48523, #3435, #79459, #18628, #3914, #71330, #96652, #50013, #64722, #40391, #42392, #88577, #1922, #95671, #26219, #10024, #71835, #40886, #57095, #49505, #41908, #65210, #72843, #11532, #73325, #34795, #65698, #43394, #59075, #43893, #42878, #98120, #89087, #50496, #67705, #99118, #36793, #75824, #29700, #98632, #19636, #20618, #35302, #52491 ),
 .UNSPECIFIED., .F., .F.,
 ( 4, 2, 2, 2, 2, 2, 2, 2, 2, 2, 2, 2, 2, 2, 2, 2, 2, 2, 2, 2, 2, 2, 2, 2, 2, 2, 4 ),
 ( 0.0005556845649962375948, 0.001563194025267928330, 0.001815071390335872264, 0.002066948755403816632, 0.002192887437937828497, 0.002318826120471841230, 0.002444764803005853530, 0.002570703485539865829, 0.002822580850607883055, 0.003074458215675900715, 0.003578212945811939504, 0.004585722406084010577, 0.005593231866356081217, 0.006096986596492074903, 0.006348863961560030980, 0.006600741326627985323, 0.006663710667895039394, 0.006726680009162093465, 0.006789649350429147537, 0.006852618691696201608, 0.006978557374230344446, 0.007104496056764487283, 0.007356373421832811121, 0.007608250786901134960, 0.007860128151969458798, 0.008112005517037782637, 0.008615760247174428579 ),
 .UNSPECIFIED. ) ;
#83961=( BOUNDED_CURVE ( )  B_SPLINE_CURVE ( 2, ( #22362, #69458, #37064, #99876, #6671, #23849, #565, #73, #60839 ),
 .UNSPECIFIED., .F., .T. ) 
 B_SPLINE_CURVE_WITH_KNOTS ( ( 3, 2, 2, 2, 3 ),
 ( 0.07661290322580645296, 0.07795698924731182811, 0.08064516129032257841, 0.08333333333333332871, 0.08467741935483871774 ),
 .UNSPECIFIED. ) 
 CURVE ( )  GEOMETRIC_REPRESENTATION_ITEM ( )  RATIONAL_B_SPLINE_CURVE ( ( 0.9330127018922194093, 0.9330127018922194093, 1.000000000000000000, 0.8660254037844387076, 1.000000000000000000, 0.8660254037844387076, 1.000000000000000000, 0.9330127018922189652, 0.9330127018922192983 ) ) 
 REPRESENTATION_ITEM ( '' )  );
#83967=CARTESIAN_POINT ( 'NONE',  ( 181.4778897503024098, 291.1215230031817214, -11.26139115722615536 ) ) ;
#83970=CARTESIAN_POINT ( 'NONE',  ( 50.34412104557527812, 188.3262482093458061, 3.021315404115420679E-15 ) ) ;
#83973=CARTESIAN_POINT ( 'NONE',  ( 153.4914073915022072, 264.7920792031019914, -16.65426974031797158 ) ) ;
#83974=CARTESIAN_POINT ( 'NONE',  ( 152.9273493951901628, 265.7690563111299298, -17.70273273795505631 ) ) ;
#83983=ORIENTED_EDGE ( 'NONE', *, *, #10391, .T. ) ;
#83985=CARTESIAN_POINT ( 'NONE',  ( 169.5454513700565258, 269.1796743676548544, 17.00868598083421546 ) ) ;
#83990=CARTESIAN_POINT ( 'NONE',  ( 204.1411873440477223, 275.2830067746622262, 13.39149321096075163 ) ) ;
#83991=CARTESIAN_POINT ( 'NONE',  ( 197.9681508493796116, 273.5361572027358079, -13.40667566358036211 ) ) ;
#83992=CARTESIAN_POINT ( 'NONE',  ( 153.1198285439165545, 279.2890930352092482, 3.903594709581249322 ) ) ;
#83994=CARTESIAN_POINT ( 'NONE',  ( 170.6068698651901627, 287.4926448325904857, -4.619150203187834869 ) ) ;
#83995=CARTESIAN_POINT ( 'NONE',  ( 165.8826895886576835, 265.9047080510878800, 16.87347945222768786 ) ) ;
#83996=ADVANCED_FACE ( 'NONE', ( #25818 ), #33921, .T. ) ;
#83997=B_SPLINE_CURVE_WITH_KNOTS ( 'NONE', 3,
 ( #27629, #89468, #51914, #82854 ),
 .UNSPECIFIED., .F., .F.,
 ( 4, 4 ),
 ( 0.009100633809674477104, 0.01512941253790484920 ),
 .UNSPECIFIED. ) ;
#83998=CARTESIAN_POINT ( 'NONE',  ( 186.7337682150368323, 287.1024196110707862, -15.92981707682468873 ) ) ;
#84000=CARTESIAN_POINT ( 'NONE',  ( 105.6408794604690797, 240.9869531367911293, 4.594050593750046652 ) ) ;
#84001=EDGE_LOOP ( 'NONE', ( #79802, #78850, #65548, #19086 ) ) ;
#84004=DIRECTION ( 'NONE',  ( -0.4999999999999987788, 0.8660254037844392627, 0.000000000000000000 ) ) ;
#84009=EDGE_CURVE ( 'NONE', #42330, #97214, #52798, .T. ) ;
#84016=CARTESIAN_POINT ( 'NONE',  ( 148.6475519825707465, 273.1818828758886752, 9.184624051690363444 ) ) ;
#84017=ORIENTED_EDGE ( 'NONE', *, *, #28193, .T. ) ;
#84021=CARTESIAN_POINT ( 'NONE',  ( 192.7166103851607772, 263.3315064552393778, 4.497380725185501582 ) ) ;
#84022=CARTESIAN_POINT ( 'NONE',  ( 156.6228368065803522, 262.3197220910723217, 17.02064833273061240 ) ) ;
#84023=CARTESIAN_POINT ( 'NONE',  ( 15.22373782933244790, 168.0494855054051868, -2.679491924311274254 ) ) ;
#84024=CARTESIAN_POINT ( 'NONE',  ( 151.8414195360447252, 269.4506305376710884, 14.13415052990332121 ) ) ;
#84026=DIRECTION ( 'NONE',  ( 0.4999999999999998890, -0.8660254037844385966, 0.000000000000000000 ) ) ;
#84027=EDGE_LOOP ( 'NONE', ( #42684, #30264, #78108, #18834 ) ) ;
#84028=CARTESIAN_POINT ( 'NONE',  ( 146.9324727656309335, 276.1524872186338371, 3.813717745456558728 ) ) ;
#84030=CARTESIAN_POINT ( 'NONE',  ( 189.1629689208399157, 263.9982617371560423, -9.142174876481732326 ) ) ;
#84031=CARTESIAN_POINT ( 'NONE',  ( 173.3007741876858177, 251.6123024758747420, -0.5682592644679328453 ) ) ;
#84032=CARTESIAN_POINT ( 'NONE',  ( 192.2191777777270261, 271.1093369735001488, -15.19916813630121410 ) ) ;
#84036=CARTESIAN_POINT ( 'NONE',  ( 155.5204415533959548, 261.2776889444089647, 17.19127227448963424 ) ) ;
#84037=CARTESIAN_POINT ( 'NONE',  ( 191.4150545428761916, 282.8117087430050560, -17.65512190867960740 ) ) ;
#84040=CARTESIAN_POINT ( 'NONE',  ( 79.14634863314516622, 210.3768266524160140, 9.188101187500098632 ) ) ;
#84041=CARTESIAN_POINT ( 'NONE',  ( 206.4640281786353171, 273.0408085897082060, -10.81921452789957883 ) ) ;
#84042=CARTESIAN_POINT ( 'NONE',  ( 147.1125781744767949, 275.8405354997948962, -5.216646253929903665 ) ) ;
#84047=CARTESIAN_POINT ( 'NONE',  ( 161.1061647010182583, 251.6029326557136585, -13.56144933775657613 ) ) ;
#84050=CARTESIAN_POINT ( 'NONE',  ( 159.1344352748853055, 279.7114264697810313, -10.00621538743078354 ) ) ;
#84051=CARTESIAN_POINT ( 'NONE',  ( 196.2953682204578456, 263.5854184417236752, 0.8810977108677261471 ) ) ;
#84053=FACE_OUTER_BOUND ( 'NONE', #71873, .T. ) ;
#84055=B_SPLINE_CURVE_WITH_KNOTS ( 'NONE', 3,
 ( #84051, #37878, #61187, #92155 ),
 .UNSPECIFIED., .F., .F.,
 ( 4, 4 ),
 ( 0.01278664256632899843, 0.02134844601914220180 ),
 .UNSPECIFIED. ) ;
#84058=CARTESIAN_POINT ( 'NONE',  ( 35.79112540406921283, 179.2202760586659736, -5.415160957724236172E-17 ) ) ;
#84059=CARTESIAN_POINT ( 'NONE',  ( 45.15450443884093090, 203.0024278399160949, 9.188101187500095079 ) ) ;
#84060=CARTESIAN_POINT ( 'NONE',  ( 196.1613785401733878, 290.8855212161054737, 15.98157687694135021 ) ) ;
#84061=B_SPLINE_CURVE_WITH_KNOTS ( 'NONE', 3,
 ( #34342, #18657, #80490, #20645, #51533, #66242, #82495, #11061, #41938, #65237, #19169, #76346, #15007, #91557, #82974, #99141, #75856, #98153, #29241, #36825, #90590, #6920, #29728, #60602, #14032, #67734, #60107, #22126, #6438, #53019, #44421, #14536, #45414, #61107, #37807, #98657, #23106, #91073, #30729, #52519, #59610, #21636, #21155, #75351, #68717, #99641, #92080, #30223, #83467, #53997 ),
 .UNSPECIFIED., .F., .F.,
 ( 4, 2, 2, 2, 2, 2, 2, 2, 2, 2, 2, 2, 2, 2, 2, 2, 2, 2, 2, 2, 2, 2, 2, 2, 4 ),
 ( 0.0007347544931350308631, 0.0009412576793029640626, 0.001147760865470897262, 0.001251012458554859579, 0.001354264051638821896, 0.001560767237806692971, 0.001973773610142371369, 0.002386779982478049334, 0.003212792727149403529, 0.004038805471820757290, 0.004864818216492110617, 0.005277824588827823710, 0.005484327774995722757, 0.005587579368079672280, 0.005639205164621694313, 0.005690830961163716346, 0.005742456757705738379, 0.005794082554247760412, 0.005897334147331918103, 0.006103837333500335832, 0.006310340519668754429, 0.006516843705837173026, 0.006723346892005590755, 0.006929850078174008485, 0.007342856450510823127 ),
 .UNSPECIFIED. ) ;
#84062=CARTESIAN_POINT ( 'NONE',  ( 199.4217651877295054, 277.6593044302092039, 15.26469614663150764 ) ) ;
#84065=CARTESIAN_POINT ( 'NONE',  ( 141.2293712190596011, 252.3458772461660260, 9.188101187500095079 ) ) ;
#84066=CARTESIAN_POINT ( 'NONE',  ( 54.70828104404427705, 193.2048013555409796, 4.594050593750051981 ) ) ;
#84069=CARTESIAN_POINT ( 'NONE',  ( 199.2299651681423143, 285.5705732690366858, -17.65328173313980642 ) ) ;
#84070=CARTESIAN_POINT ( 'NONE',  ( 196.4808189786114951, 290.3322341467384717, -17.84817245450773271 ) ) ;
#84074=CARTESIAN_POINT ( 'NONE',  ( 175.7016899852434335, 291.0303512684756697, 2.528121706571572425 ) ) ;
#84075=CARTESIAN_POINT ( 'NONE',  ( 198.2819808855875863, 287.2125302111982705, 18.53535247371401695 ) ) ;
#84076=CARTESIAN_POINT ( 'NONE',  ( 182.3130817044836931, 280.8266231767971703, -16.24680219230945966 ) ) ;
#84077=CARTESIAN_POINT ( 'NONE',  ( 153.3114877943481815, 276.8159031518617326, 7.198048095202238983 ) ) ;
#84078=ADVANCED_FACE ( 'NONE', ( #72930 ), #97231, .T. ) ;
#84081=CARTESIAN_POINT ( 'NONE',  ( 95.42925689777531773, 219.2365022471902023, -10.00000000000009059 ) ) ;
#84082=CARTESIAN_POINT ( 'NONE',  ( 200.4775477985258760, 283.4096967665721536, 16.80647240730505487 ) ) ;
#84083=B_SPLINE_CURVE_WITH_KNOTS ( 'NONE', 3,
 ( #95397, #41113, #73539, #57322 ),
 .UNSPECIFIED., .F., .F.,
 ( 4, 4 ),
 ( 0.009352860264968503035, 0.01452566192536472109 ),
 .UNSPECIFIED. ) ;
#84084=CARTESIAN_POINT ( 'NONE',  ( 194.3231775528952312, 285.3053704592781514, -17.11556690190039376 ) ) ;
#84085=ORIENTED_EDGE ( 'NONE', *, *, #36896, .T. ) ;
#84086=CARTESIAN_POINT ( 'NONE',  ( 61.47358386746269332, 215.4869531367911009, 4.594050593750046652 ) ) ;
#84087=VERTEX_POINT ( 'NONE', #11616 ) ;
#84088=CARTESIAN_POINT ( 'NONE',  ( 165.5617726036975625, 265.0396632758227611, 16.58379757636856056 ) ) ;
#84089=CARTESIAN_POINT ( 'NONE',  ( 190.3453568493779358, 278.9120622883270926, -16.55271846494312626 ) ) ;
#84094=CARTESIAN_POINT ( 'NONE',  ( 148.1974503712686158, 273.9614817352322120, -7.884397846570731616 ) ) ;
#84096=CARTESIAN_POINT ( 'NONE',  ( -22.42236680055709641, 157.8615022471902591, 0.000000000000000000 ) ) ;
#84097=CARTESIAN_POINT ( 'NONE',  ( 204.9604304439480416, 275.6451162603322587, 13.28912526856024279 ) ) ;
#84101=CARTESIAN_POINT ( 'NONE',  ( 173.7423250686665881, 275.4393285809401846, 17.42598933989775389 ) ) ;
#84102=ORIENTED_EDGE ( 'NONE', *, *, #22539, .T. ) ;
#84103=CARTESIAN_POINT ( 'NONE',  ( 202.9899429726835649, 270.3564826351193915, -9.180241878456698146 ) ) ;
#84104=CARTESIAN_POINT ( 'NONE',  ( 159.2394649670193303, 254.8361514374751664, -16.43133403737800791 ) ) ;
#84107=ORIENTED_EDGE ( 'NONE', *, *, #8336, .T. ) ;
#84108=CARTESIAN_POINT ( 'NONE',  ( 173.8526494319628739, 285.7800503636065059, 10.50335656709346033 ) ) ;
#84109=EDGE_CURVE ( 'NONE', #76921, #81902, #19149, .T. ) ;
#84112=CARTESIAN_POINT ( 'NONE',  ( 163.0424334805279045, 248.2492167524936804, -9.671494865076915914 ) ) ;
#84113=CARTESIAN_POINT ( 'NONE',  ( 204.4325665793906524, 276.5594032932251594, 13.33817701435311598 ) ) ;
#84114=CARTESIAN_POINT ( 'NONE',  ( 159.7953104873542145, 253.8733987550956783, 15.41928249285404107 ) ) ;
#84115=CARTESIAN_POINT ( 'NONE',  ( 164.0826012759681305, 264.7739101429210109, -16.65441687119937342 ) ) ;
#84116=CARTESIAN_POINT ( 'NONE',  ( 138.1714793337695824, 241.3923013555409796, 4.594050593750050204 ) ) ;
#84118=CARTESIAN_POINT ( 'NONE',  ( 177.6697782944580979, 268.6434933572430737, 17.08943839160881595 ) ) ;
#84119=CARTESIAN_POINT ( 'NONE',  ( 195.7990362237038369, 290.8591192847630964, -16.03867274897940831 ) ) ;
#84120=CARTESIAN_POINT ( 'NONE',  ( 79.14634863314516622, 210.3768266524160140, 9.188101187500098632 ) ) ;
#84132=CARTESIAN_POINT ( 'NONE',  ( 197.8158846759225469, 287.0879278553931613, 16.95854422743263967 ) ) ;
#84135=CARTESIAN_POINT ( 'NONE',  ( 154.8989000222956349, 262.3542304552891551, 17.41779271305265908 ) ) ;
#84138=AXIS2_PLACEMENT_3D ( 'NONE', #64580, #56955, #87941 ) ;
#84139=B_SPLINE_SURFACE_WITH_KNOTS ( 'NONE', 3, 1, ( 
 ( #15990, #785 ),
 ( #8397, #79837 ),
 ( #86455, #31671 ),
 ( #54463, #46890 ),
 ( #71720, #78308 ),
 ( #1301, #79343 ),
 ( #9910, #48901 ),
 ( #62069, #2312 ),
 ( #32185, #62567 ),
 ( #40271, #93531 ),
 ( #94529, #24087 ),
 ( #16979, #94033 ),
 ( #10403, #41273 ),
 ( #54983, #8889 ),
 ( #93017, #64092 ),
 ( #25081, #55962 ),
 ( #95037, #39758 ),
 ( #72215, #24583 ),
 ( #25601, #56487 ),
 ( #55469, #23571 ),
 ( #47871, #86956 ),
 ( #2819, #51376 ),
 ( #11422, #20503 ),
 ( #81828, #35688 ),
 ( #11910, #27103 ),
 ( #12912, #3803 ),
 ( #57475, #56976 ),
 ( #88969, #49392 ),
 ( #33709, #57988 ),
 ( #80338, #26102 ),
 ( #10906, #43270 ),
 ( #73698, #66588 ),
 ( #95556, #34199 ),
 ( #72728, #64601 ) ),
 .UNSPECIFIED., .T., .F., .F.,
 ( 4, 2, 2, 2, 2, 2, 2, 2, 2, 2, 2, 2, 2, 2, 2, 2, 4 ),
 ( 2, 2 ),
 ( 0.000000000000000000, 0.06250000000000000000, 0.1250000000000000000, 0.1875000000000000000, 0.2500000000000000000, 0.3125000000000000000, 0.3750000000000000000, 0.4375000000000000000, 0.5000000000000000000, 0.5625000000000000000, 0.6250000000000000000, 0.6875000000000000000, 0.7500000000000000000, 0.8125000000000000000, 0.8750000000000000000, 0.9375000000000000000, 1.000000000000000000 ),
 ( 0.000000000000000000, 1.000000000000000000 ),
 .UNSPECIFIED. ) ;
#84141=ORIENTED_EDGE ( 'NONE', *, *, #44819, .F. ) ;
#84143=CARTESIAN_POINT ( 'NONE',  ( 183.9506971135539004, 275.2367033331265702, 16.38750030320872852 ) ) ;
#84146=CARTESIAN_POINT ( 'NONE',  ( 195.5051761698225619, 279.3379179581851304, 16.32977475709600768 ) ) ;
#84148=CARTESIAN_POINT ( 'NONE',  ( 130.0249940097159254, 252.0024278399160949, -9.188101187500093303 ) ) ;
#84149=ORIENTED_EDGE ( 'NONE', *, *, #6143, .T. ) ;
#84151=CARTESIAN_POINT ( 'NONE',  ( 182.0908725605739278, 257.5538491103775414, 6.656128696890800889 ) ) ;
#84153=CARTESIAN_POINT ( 'NONE',  ( 153.4613150239306094, 264.8442007126561748, -16.86932470306368259 ) ) ;
#84157=CARTESIAN_POINT ( 'NONE',  ( 199.3492571032118974, 266.8521786015153907, 4.572492606930079084 ) ) ;
#84158=CARTESIAN_POINT ( 'NONE',  ( 148.3881289992426105, 276.3505094388546581, -3.863952534650588522 ) ) ;
#84161=CARTESIAN_POINT ( 'NONE',  ( 198.5847843579792311, 266.2858474173958143, 0.8381617387219465476 ) ) ;
#84162=CARTESIAN_POINT ( 'NONE',  ( 198.9327437650594845, 265.4802594572302041, 0.07579901079707679346 ) ) ;
#84165=CARTESIAN_POINT ( 'NONE',  ( 186.8895883408185910, 282.0686240457306440, 16.84332228780022689 ) ) ;
#84166=CARTESIAN_POINT ( 'NONE',  ( 164.9335952247126045, 244.9736285262353306, -1.661461410667423255 ) ) ;
#84167=CARTESIAN_POINT ( 'NONE',  ( 177.3308938375265598, 264.6334632213029181, -15.29145188940869282 ) ) ;
#84168=CARTESIAN_POINT ( 'NONE',  ( 196.8833167150979477, 269.7409658301617128, 12.25108723014616352 ) ) ;
#84171=CARTESIAN_POINT ( 'NONE',  ( 166.5995791397127448, 286.3618139744101541, -3.233326376697027715 ) ) ;
#84173=CARTESIAN_POINT ( 'NONE',  ( 159.5573297132660002, 254.2855935470410031, 16.91607698584599007 ) ) ;
#84174=CARTESIAN_POINT ( 'NONE',  ( 145.9293632524074553, 248.3927522451417929, -10.00000000000009059 ) ) ;
#84177=AXIS2_PLACEMENT_3D ( 'NONE', #54020, #341, #15522 ) ;
#84180=CARTESIAN_POINT ( 'NONE',  ( 179.3071757824324095, 289.7729440391376556, 11.79011794106743949 ) ) ;
#84181=CARTESIAN_POINT ( 'NONE',  ( 11.32556065139379875, 177.3458772461660544, 9.188101187500095079 ) ) ;
#84182=CARTESIAN_POINT ( 'NONE',  ( 181.8071258313758278, 275.6022297491251720, -16.43063624076323137 ) ) ;
#84185=CARTESIAN_POINT ( 'NONE',  ( 170.1804300311658551, 270.7854574292069287, -17.38281393466202829 ) ) ;
#84188=CARTESIAN_POINT ( 'NONE',  ( 175.5081009096628577, 253.5491181420100304, -3.811933576842129856 ) ) ;
#84189=CARTESIAN_POINT ( 'NONE',  ( 190.6671659678193862, 261.9269538368635608, -0.7676713603561022836 ) ) ;
#84190=EDGE_CURVE ( 'NONE', #25608, #32094, #19245, .T. ) ;
#84193=CARTESIAN_POINT ( 'NONE',  ( 56.31377616017810084, 209.9865022471902876, -10.00000000000009415 ) ) ;
#84194=DIRECTION ( 'NONE',  ( -0.8660254037844387076, -0.4999999999999998890, -0.000000000000000000 ) ) ;
#84195=CARTESIAN_POINT ( 'NONE',  ( 148.2159754900428936, 273.9293952882992471, 9.267836332806297150 ) ) ;
#84196=ADVANCED_FACE ( 'NONE', ( #3762 ), #71676, .T. ) ;
#84197=CARTESIAN_POINT ( 'NONE',  ( 18.33521408509785644, 172.2048013555409796, 4.594050593750051981 ) ) ;
#84203=CARTESIAN_POINT ( 'NONE',  ( 207.1059763530604698, 271.9289217357780899, 6.370907250589925575 ) ) ;
#84205=CARTESIAN_POINT ( 'NONE',  ( 162.8927609601937263, 281.1658276129857086, -10.34727072843073614 ) ) ;
#84206=CARTESIAN_POINT ( 'NONE',  ( 179.9016459768426728, 262.6902523525472475, -14.18888862508328685 ) ) ;
#84210=CARTESIAN_POINT ( 'NONE',  ( 155.0303156110108489, 262.1266119787277944, 17.11986653161320859 ) ) ;
#84220=CARTESIAN_POINT ( 'NONE',  ( 203.5555343017997529, 278.0784677578903370, -15.71723084798551362 ) ) ;
#84221=B_SPLINE_CURVE_WITH_KNOTS ( 'NONE', 3,
 ( #52651, #30364, #92697, #66496, #54136, #66000, #29864, #14669, #27518, #84601, #30865, #46037, #60735, #14172, #21762, #27991 ),
 .UNSPECIFIED., .F., .F.,
 ( 4, 2, 2, 2, 2, 2, 2, 4 ),
 ( 0.0007292608245178773888, 0.001016117201828066604, 0.001302973579138255820, 0.001589829956448444818, 0.001876686333758634034, 0.002163542711068823250, 0.002450399088379012248, 0.003024111842999491727 ),
 .UNSPECIFIED. ) ;
#84223=ORIENTED_EDGE ( 'NONE', *, *, #54135, .T. ) ;
#84225=CARTESIAN_POINT ( 'NONE',  ( 204.2799274532736433, 276.8237820148827950, 13.55359442435934803 ) ) ;
#84227=CARTESIAN_POINT ( 'NONE',  ( 153.0927037754837556, 265.4826541232073964, -16.15085267704102634 ) ) ;
#84230=CARTESIAN_POINT ( 'NONE',  ( 49.72837464868604940, 199.5177522451418781, -10.00000000000009592 ) ) ;
#84232=CARTESIAN_POINT ( 'NONE',  ( 190.5969391768923913, 300.5234129089444650, -0.7564693504096553500 ) ) ;
#84234=CARTESIAN_POINT ( 'NONE',  ( 205.9642072045669465, 273.9065239114831911, 10.22128930895731536 ) ) ;
#84235=CARTESIAN_POINT ( 'NONE',  ( 158.1669649540034186, 265.2021071281276363, 17.58525919077285593 ) ) ;
#84236=VERTEX_POINT ( 'NONE', #11383 ) ;
#84237=CARTESIAN_POINT ( 'NONE',  ( 190.8138402884741254, 300.1477291634665789, 4.037153726988762514 ) ) ;
#84238=CARTESIAN_POINT ( 'NONE',  ( 189.5599828453989346, 263.0657735508838186, -9.804501003715218488 ) ) ;
#84245=ORIENTED_EDGE ( 'NONE', *, *, #6405, .F. ) ;
#84246=( BOUNDED_CURVE ( )  B_SPLINE_CURVE ( 2, ( #82796, #13362, #22437, #53330, #68533, #97962, #29060, #76641, #82305 ),
 .UNSPECIFIED., .F., .T. ) 
 B_SPLINE_CURVE_WITH_KNOTS ( ( 3, 2, 2, 2, 3 ),
 ( 0.1008064516129032334, 0.1021505376344086086, 0.1048387096774193589, 0.1075268817204301092, 0.1088709677419354843 ),
 .UNSPECIFIED. ) 
 CURVE ( )  GEOMETRIC_REPRESENTATION_ITEM ( )  RATIONAL_B_SPLINE_CURVE ( ( 0.9330127018922192983, 0.9330127018922196314, 1.000000000000000000, 0.8660254037844387076, 1.000000000000000000, 0.8660254037844387076, 1.000000000000000000, 0.9330127018922194093, 0.9330127018922194093 ) ) 
 REPRESENTATION_ITEM ( '' )  );
#84248=CARTESIAN_POINT ( 'NONE',  ( 146.8058449195592061, 276.3718130816831149, 4.181814292810413392 ) ) ;
#84250=CARTESIAN_POINT ( 'NONE',  ( 149.7128599965862463, 271.3367152699035501, 12.33532264622322394 ) ) ;
#84252=CARTESIAN_POINT ( 'NONE',  ( 191.8453175503442196, 298.3611581390557035, 9.038225159363836525 ) ) ;
#84253=CARTESIAN_POINT ( 'NONE',  ( 191.5324528500417216, 298.9030556958743432, -8.286652526617016790 ) ) ;
#84254=CARTESIAN_POINT ( 'NONE',  ( 190.0274641710971082, 301.5097725526222803, 3.738976720635653450 ) ) ;
#84259=CARTESIAN_POINT ( 'NONE',  ( 167.5421813246326792, 287.5986610761024167, 3.969292590682533373 ) ) ;
#84262=CARTESIAN_POINT ( 'NONE',  ( 190.8204521987322835, 300.1362769989643198, -4.254506460977580673 ) ) ;
#84264=CARTESIAN_POINT ( 'NONE',  ( 148.8636819117637629, 274.0699646975406836, 8.926834414297511344 ) ) ;
#84266=CARTESIAN_POINT ( 'NONE',  ( 179.7520283141993787, 283.0547433888561386, -15.89619356914058201 ) ) ;
#84267=CARTESIAN_POINT ( 'NONE',  ( 189.9181943850632308, 301.6990333737651326, -1.201434020889846632 ) ) ;
#84269=CARTESIAN_POINT ( 'NONE',  ( 168.7885031894148256, 286.1153816027461403, -7.680432405603670354 ) ) ;
#84270=ORIENTED_EDGE ( 'NONE', *, *, #44370, .F. ) ;
#84271=CARTESIAN_POINT ( 'NONE',  ( 163.4084407101100851, 247.6152736349200438, -10.68829614238923931 ) ) ;
#84272=CYLINDRICAL_SURFACE ( 'NONE', #27389, 17.82106496071139645 ) ;
#84275=CARTESIAN_POINT ( 'NONE',  ( 39.40823858692142778, 206.8927522451419350, 2.944929066748280225E-16 ) ) ;
#84276=CARTESIAN_POINT ( 'NONE',  ( 117.5758788303146076, 244.8149278399160949, 9.188101187500093303 ) ) ;
#84277=CARTESIAN_POINT ( 'NONE',  ( 180.6753976046032051, 294.2641805748295951, -3.313934977364610734 ) ) ;
#84279=CARTESIAN_POINT ( 'NONE',  ( 157.5042325173297684, 257.8416622032797818, 16.70595240278738203 ) ) ;
#84280=CARTESIAN_POINT ( 'NONE',  ( 172.2717404889760928, 250.6514006074399674, -4.087445548495970193 ) ) ;
#84281=CARTESIAN_POINT ( 'NONE',  ( 24.66750420662404508, 194.2369531367911293, -4.594050593750048428 ) ) ;
#84285=CARTESIAN_POINT ( 'NONE',  ( 191.3698991030772731, 298.7983559512333613, 7.726696955929065247 ) ) ;
#84286=CARTESIAN_POINT ( 'NONE',  ( 181.3932036981916269, 267.7384658855342536, 14.96073790625240996 ) ) ;
#84288=CARTESIAN_POINT ( 'NONE',  ( 147.3023124603499809, 275.5119060767245287, 5.196938859334171212 ) ) ;
#84292=CARTESIAN_POINT ( 'NONE',  ( 106.8138825148102740, 239.1427522451419065, -10.00000000000009415 ) ) ;
#84295=B_SPLINE_CURVE_WITH_KNOTS ( 'NONE', 3,
 ( #28388, #50201, #27414, #74018, #75014, #4603, #35495, #51711, #97326, #69755, #46961, #24163, #55048, #8464 ),
 .UNSPECIFIED., .F., .F.,
 ( 4, 2, 2, 2, 2, 2, 4 ),
 ( 3.469446951953614189E-18, 0.0004440166800142984912, 0.0008880333600285935129, 0.001110041700035716223, 0.001332050040042838824, 0.001554058380049961642, 0.001776066720057084243 ),
 .UNSPECIFIED. ) ;
#84296=CARTESIAN_POINT ( 'NONE',  ( 158.2918428669640605, 281.5729122900692118, -1.602796375854172339 ) ) ;
#84297=DIRECTION ( 'NONE',  ( -0.8660254037844387076, -0.4999999999999998890, -0.000000000000000000 ) ) ;
#84298=CARTESIAN_POINT ( 'NONE',  ( 7.753205860782987457, 175.2833772461660544, -9.188101187500095079 ) ) ;
#84301=CARTESIAN_POINT ( 'NONE',  ( 192.5076277540105423, 297.2140032159341558, -13.10094381206144298 ) ) ;
#84303=CARTESIAN_POINT ( 'NONE',  ( 174.3777206541172404, 286.9002377562176207, 10.20102932312108557 ) ) ;
#84304=CARTESIAN_POINT ( 'NONE',  ( 65.45180129215621889, 220.8464784336661637, 1.353441290958777327E-15 ) ) ;
#84305=CARTESIAN_POINT ( 'NONE',  ( 200.4775477985258760, 283.4096967665721536, 16.80647240730505487 ) ) ;
#84307=CARTESIAN_POINT ( 'NONE',  ( 47.92415505746842541, 205.1427522451419065, 10.00000000000009415 ) ) ;
#84310=CARTESIAN_POINT ( 'NONE',  ( 162.5320791996320224, 267.5315774354641576, 16.48036321604684673 ) ) ;
#84311=CARTESIAN_POINT ( 'NONE',  ( 10.91961124514375925, 187.1115022471903160, -5.000000000000047962 ) ) ;
#84312=CARTESIAN_POINT ( 'NONE',  ( 164.1146561143383167, 246.3920726737087534, -7.362905700427413436 ) ) ;
#84313=CARTESIAN_POINT ( 'NONE',  ( 128.2929432021470859, 251.0024278399160949, 9.188101187500095079 ) ) ;
#84315=CARTESIAN_POINT ( 'NONE',  ( 164.7063722853443437, 260.9203034178046323, -16.15040340005176844 ) ) ;
#84320=CARTESIAN_POINT ( 'NONE',  ( 172.2313928256145630, 289.6871463590026679, -5.851927625370571207 ) ) ;
#84326=CARTESIAN_POINT ( 'NONE',  ( 156.0554005950856151, 280.4150375230931331, -5.525834068163355539 ) ) ;
#84329=CARTESIAN_POINT ( 'NONE',  ( 206.6259318078842284, 272.7603832779192885, 8.129480779612674013 ) ) ;
#84330=CARTESIAN_POINT ( 'NONE',  ( 167.9430779612994797, 282.0224708860221767, -12.05993733932491452 ) ) ;
#84331=CARTESIAN_POINT ( 'NONE',  ( -22.42236680055709641, 157.8615022471902591, 0.000000000000000000 ) ) ;
#84332=DIRECTION ( 'NONE',  ( 0.4999999999999998890, -0.8660254037844385966, 0.000000000000000000 ) ) ;
#84336=CARTESIAN_POINT ( 'NONE',  ( 152.7375212135632125, 266.0978483664162582, -16.47968945089317572 ) ) ;
#84337=B_SPLINE_CURVE_WITH_KNOTS ( 'NONE', 3,
 ( #1960, #72883, #32846, #26261 ),
 .UNSPECIFIED., .F., .F.,
 ( 4, 4 ),
 ( 0.03823235658919261343, 0.04678228248050523425 ),
 .UNSPECIFIED. ) ;
#84340=EDGE_LOOP ( 'NONE', ( #9167, #91596, #66030, #16893 ) ) ;
#84341=CARTESIAN_POINT ( 'NONE',  ( 190.6023073677431512, 300.5141149296460981, 3.174888932019753973 ) ) ;
#84342=CARTESIAN_POINT ( 'NONE',  ( 199.0230529003142692, 272.6643487552923375, 13.78389951960891047 ) ) ;
#84343=CARTESIAN_POINT ( 'NONE',  ( 189.5301620294561360, 297.3496777562929196, 8.148958219677171044 ) ) ;
#84345=CARTESIAN_POINT ( 'NONE',  ( 191.0862225170008628, 299.6759493045793192, -9.402218231374108726 ) ) ;
#84347=CARTESIAN_POINT ( 'NONE',  ( 196.8104339078508076, 289.7613243423628546, -16.40335862274955403 ) ) ;
#84350=CARTESIAN_POINT ( 'NONE',  ( 100.7694865641816051, 238.1744531367911293, 4.594050593750047540 ) ) ;
#84351=CARTESIAN_POINT ( 'NONE',  ( 161.2313178023453588, 251.3861611254901618, 13.12937145726518473 ) ) ;
#84352=CARTESIAN_POINT ( 'NONE',  ( 181.1985647863735664, 271.1040133950066888, -15.97949505363916956 ) ) ;
#84354=B_SPLINE_CURVE_WITH_KNOTS ( 'NONE', 3,
 ( #27850, #34940, #12161, #51137 ),
 .UNSPECIFIED., .F., .F.,
 ( 4, 4 ),
 ( 0.01377033617237334931, 0.02241479314274836751 ),
 .UNSPECIFIED. ) ;
#84358=EDGE_LOOP ( 'NONE', ( #32883, #92190, #57767, #95694 ) ) ;
#84359=CARTESIAN_POINT ( 'NONE',  ( -17.42236680055705023, 149.2012482093457777, 0.000000000000000000 ) ) ;
#84360=VERTEX_POINT ( 'NONE', #79797 ) ;
#84361=CARTESIAN_POINT ( 'NONE',  ( 207.8060684685902686, 270.7163266217015689, 2.015725026008670540 ) ) ;
#84363=CARTESIAN_POINT ( 'NONE',  ( 165.2793717279795942, 271.1751283101625063, 17.08238418428851091 ) ) ;
#84364=B_SPLINE_CURVE_WITH_KNOTS ( 'NONE', 3,
 ( #4242, #73175, #65547, #72687 ),
 .UNSPECIFIED., .F., .F.,
 ( 4, 4 ),
 ( 0.009023986987182482794, 0.01512749127632531665 ),
 .UNSPECIFIED. ) ;
#84366=CARTESIAN_POINT ( 'NONE',  ( 19.16720650933548953, 170.3262482093457777, 3.021315404115420679E-15 ) ) ;
#84367=CARTESIAN_POINT ( 'NONE',  ( 200.4473000517033086, 270.8492857102374387, -11.53500569907702022 ) ) ;
#84370=CARTESIAN_POINT ( 'NONE',  ( 198.5691746959190311, 277.5136763456665676, -15.35557735086660003 ) ) ;
#84372=CARTESIAN_POINT ( 'NONE',  ( 14.65434579541627969, 179.2677522451418497, 10.00000000000009592 ) ) ;
#84374=CARTESIAN_POINT ( 'NONE',  ( 202.4900219881211854, 279.9239892212719383, 15.63116161057562259 ) ) ;
#84375=CARTESIAN_POINT ( 'NONE',  ( 188.8449905984804218, 259.7290283989091222, 2.370086273675485522 ) ) ;
#84378=CARTESIAN_POINT ( 'NONE',  ( 169.1186385402264420, 254.0988134251273038, 11.40381662627904014 ) ) ;
#84379=CARTESIAN_POINT ( 'NONE',  ( 161.1720804342144788, 283.2912763611720379, 2.125355488856659036 ) ) ;
#84381=CARTESIAN_POINT ( 'NONE',  ( 194.4048639213451679, 293.9278937801532834, -15.59881047903446927 ) ) ;
#84383=CARTESIAN_POINT ( 'NONE',  ( 54.07885559584777013, 190.4824982072973967, 3.021315404115420679E-15 ) ) ;
#84384=ADVANCED_FACE ( 'NONE', ( #51331 ), #90892, .T. ) ;
#84385=CARTESIAN_POINT ( 'NONE',  ( 1.230952036757517520, 161.5177522451418213, 5.000000000000051514 ) ) ;
#84386=CARTESIAN_POINT ( 'NONE',  ( 196.0942742968314860, 269.6800398832626229, -11.21024681009520840 ) ) ;
#84387=CARTESIAN_POINT ( 'NONE',  ( 171.3390933369627191, 279.6671480371463758, -14.77428946034695834 ) ) ;
#84388=CARTESIAN_POINT ( 'NONE',  ( 203.4842972674048269, 278.2018539208430639, -15.39142462160632263 ) ) ;
#84391=CARTESIAN_POINT ( 'NONE',  ( -1.394013918807642360, 163.8768266524159856, 9.188101187500098632 ) ) ;
#84392=CARTESIAN_POINT ( 'NONE',  ( 188.1412547211656943, 273.5593357346770063, 17.08033167198486879 ) ) ;
#84402=CARTESIAN_POINT ( 'NONE',  ( 163.1248382027621062, 248.1064875868004549, -11.52679925016660079 ) ) ;
#84404=CARTESIAN_POINT ( 'NONE',  ( 153.5650287317978950, 279.2224830237896640, 3.840963988500594617 ) ) ;
#84405=CARTESIAN_POINT ( 'NONE',  ( 11.37951369124782453, 183.5024278399160949, 9.188101187500095079 ) ) ;
#84406=CARTESIAN_POINT ( 'NONE',  ( 107.8059429699301575, 242.2369531367911009, -4.594050593750048428 ) ) ;
#84407=CARTESIAN_POINT ( 'NONE',  ( 181.8184041672141120, 294.6703142210058104, -6.550043312232509685 ) ) ;
#84411=CARTESIAN_POINT ( 'NONE',  ( 190.6088168084232279, 299.9436237569324248, -4.377057509834942906 ) ) ;
#84413=CARTESIAN_POINT ( 'NONE',  ( 155.5888570658010508, 261.1591898008976500, 17.34682632352454945 ) ) ;
#84414=CARTESIAN_POINT ( 'NONE',  ( 161.2488013048736377, 251.3558788108169040, -13.10044423494716170 ) ) ;
#84415=CARTESIAN_POINT ( 'NONE',  ( 188.5288891056994203, 283.7822663309162294, 16.35679746564665749 ) ) ;
#84417=EDGE_CURVE ( 'NONE', #70733, #48184, #36061, .T. ) ;
#84418=EDGE_CURVE ( 'NONE', #67601, #14882, #29471, .T. ) ;
#84419=CARTESIAN_POINT ( 'NONE',  ( 192.6383675332188830, 265.0412903862384724, 7.554505506666291836 ) ) ;
#84420=CARTESIAN_POINT ( 'NONE',  ( 165.0478369365887374, 249.7899772327647270, -10.67719793920586469 ) ) ;
#84421=CARTESIAN_POINT ( 'NONE',  ( 175.5041665230661465, 256.4755977299537335, -10.91805166175802633 ) ) ;
#84422=FACE_OUTER_BOUND ( 'NONE', #63522, .T. ) ;
#84423=FACE_OUTER_BOUND ( 'NONE', #57331, .T. ) ;
#84424=CARTESIAN_POINT ( 'NONE',  ( -22.42236680055709641, 157.8615022471902591, 0.000000000000000000 ) ) ;
#84426=CARTESIAN_POINT ( 'NONE',  ( 161.6021384458605326, 281.4729049090978492, -9.576418522834517333 ) ) ;
#84427=ADVANCED_FACE ( 'NONE', ( #6740 ), #21526, .F. ) ;
#84429=CARTESIAN_POINT ( 'NONE',  ( 104.8295012880686699, 222.1423013555409796, -4.594050593750043987 ) ) ;
#84434=CARTESIAN_POINT ( 'NONE',  ( 136.1945356951059125, 260.9860189848785694, -2.679491924311252493 ) ) ;
#84435=CARTESIAN_POINT ( 'NONE',  ( 112.9482291249501174, 226.0177522451418213, 5.000000000000051514 ) ) ;
#84436=CARTESIAN_POINT ( 'NONE',  ( 159.9924463476198753, 283.3850188831759169, -3.371971149216307140 ) ) ;
#84437=CARTESIAN_POINT ( 'NONE',  ( 151.0801312611820890, 268.9685319718947198, -15.83903210480701240 ) ) ;
#84442=VERTEX_POINT ( 'NONE', #54818 ) ;
#84444=CARTESIAN_POINT ( 'NONE',  ( 179.0323333429434172, 280.8471605631614239, 16.29919625892006962 ) ) ;
#84445=LINE ( 'NONE', #46379, #10239 ) ;
#84446=CARTESIAN_POINT ( 'NONE',  ( 149.0598351764325002, 272.4677874370131576, -11.59078276432863674 ) ) ;
#84447=EDGE_CURVE ( 'NONE', #49368, #85448, #26395, .T. ) ;
#84450=B_SPLINE_SURFACE_WITH_KNOTS ( 'NONE', 3, 1, ( 
 ( #2127, #62908 ),
 ( #1121, #62390 ),
 ( #33009, #31498 ),
 ( #15803, #9741 ),
 ( #71035, #25409 ),
 ( #79662, #92846 ),
 ( #16809, #85257 ),
 ( #77634, #47204 ),
 ( #8716, #56301 ),
 ( #93347, #1637 ),
 ( #47696, #78128 ),
 ( #16311, #40597 ),
 ( #55783, #8218 ),
 ( #71535, #23903 ),
 ( #10225, #70001 ),
 ( #23397, #54805 ),
 ( #32521, #78633 ),
 ( #63414, #94848 ),
 ( #63910, #94353 ),
 ( #31006, #61895 ),
 ( #54287, #24907 ),
 ( #86775, #85782 ),
 ( #17310, #48215 ),
 ( #17828, #89755 ),
 ( #81161, #95380 ),
 ( #80663, #27903 ),
 ( #26424, #96353 ),
 ( #3631, #88778 ),
 ( #35000, #73523 ),
 ( #49226, #35505 ),
 ( #97334, #89276 ),
 ( #25932, #73038 ),
 ( #12222, #34034 ),
 ( #51191, #34509 ) ),
 .UNSPECIFIED., .T., .F., .F.,
 ( 4, 2, 2, 2, 2, 2, 2, 2, 2, 2, 2, 2, 2, 2, 2, 2, 4 ),
 ( 2, 2 ),
 ( 0.000000000000000000, 0.06250000000000000000, 0.1250000000000000000, 0.1875000000000000000, 0.2500000000000000000, 0.3125000000000000000, 0.3750000000000000000, 0.4375000000000000000, 0.5000000000000000000, 0.5625000000000000000, 0.6250000000000000000, 0.6875000000000000000, 0.7500000000000000000, 0.8125000000000000000, 0.8750000000000000000, 0.9375000000000000000, 1.000000000000000000 ),
 ( 0.000000000000000000, 1.000000000000000000 ),
 .UNSPECIFIED. ) ;
#84452=CARTESIAN_POINT ( 'NONE',  ( 159.8655504377736918, 253.7517395922482706, 15.51368179719542262 ) ) ;
#84453=CARTESIAN_POINT ( 'NONE',  ( 179.9084428208875579, 262.7189347004215847, -12.75842409700454283 ) ) ;
#84454=CARTESIAN_POINT ( 'NONE',  ( 169.3569635281594117, 252.0144808050329175, -8.621157649714792370 ) ) ;
#84456=CARTESIAN_POINT ( 'NONE',  ( 149.1228319324105200, 250.2365022471901739, 10.00000000000009592 ) ) ;
#84462=CARTESIAN_POINT ( 'NONE',  ( 168.0266106847527681, 249.2181159516572393, 6.488127101935972973 ) ) ;
#84463=CARTESIAN_POINT ( 'NONE',  ( 184.6854688042101600, 292.1945499485699997, -10.69498008038247505 ) ) ;
#84468=CARTESIAN_POINT ( 'NONE',  ( 153.7173656711216267, 264.4007079824105517, -16.52087364244192358 ) ) ;
#84469=CARTESIAN_POINT ( 'NONE',  ( 169.3571508527084291, 283.0956279022483955, 12.63651818596384935 ) ) ;
#84473=ORIENTED_EDGE ( 'NONE', *, *, #32916, .F. ) ;
#84477=CARTESIAN_POINT ( 'NONE',  ( 197.9827105953623061, 286.8556216960815846, 16.93946419794055558 ) ) ;
#84478=CARTESIAN_POINT ( 'NONE',  ( 169.8667279133726424, 269.3604332311463168, 16.84841970499969932 ) ) ;
#84479=CARTESIAN_POINT ( 'NONE',  ( 204.9432097630379417, 275.6749433546094679, 13.74700047688257776 ) ) ;
#84481=DIRECTION ( 'NONE',  ( 0.4999999999999992784, -0.8660254037844390407, 0.000000000000000000 ) ) ;
#84482=CARTESIAN_POINT ( 'NONE',  ( 197.8821111871073981, 272.3286829384299494, -13.44603622953895261 ) ) ;
#84483=CARTESIAN_POINT ( 'NONE',  ( 203.5517807763935991, 276.4131063546051337, 14.32831804246049678 ) ) ;
#84485=CARTESIAN_POINT ( 'NONE',  ( 171.6200503532151629, 250.8586239335233756, -5.669471818614393754 ) ) ;
#84487=CARTESIAN_POINT ( 'NONE',  ( 188.7267243920021542, 295.1910411013678299, 11.79826141631466463 ) ) ;
#84488=CARTESIAN_POINT ( 'NONE',  ( 116.5476472112030990, 238.0958772461660544, -9.188101187500095079 ) ) ;
#84489=CARTESIAN_POINT ( 'NONE',  ( 187.1412927779018673, 261.9835105880691231, -10.20549468610707322 ) ) ;
#84492=CARTESIAN_POINT ( 'NONE',  ( 190.0654284128779068, 274.4660007832150086, 15.78607938090247487 ) ) ;
#84493=ORIENTED_EDGE ( 'NONE', *, *, #10202, .F. ) ;
#84494=EDGE_CURVE ( 'NONE', #23594, #86318, #47023, .T. ) ;
#84495=CARTESIAN_POINT ( 'NONE',  ( 162.8503517516483328, 249.0322973948848642, -10.17031201914153549 ) ) ;
#84499=CARTESIAN_POINT ( 'NONE',  ( 157.3025066944120454, 258.1910615777721887, 18.21299529665260053 ) ) ;
#84500=CARTESIAN_POINT ( 'NONE',  ( 206.3423291502491566, 273.2515974901050413, -10.76717883871977577 ) ) ;
#84502=ORIENTED_EDGE ( 'NONE', *, *, #26079, .T. ) ;
#84508=CARTESIAN_POINT ( 'NONE',  ( 191.5637510654044036, 267.2623274562577080, -12.69923334320934849 ) ) ;
#84510=CARTESIAN_POINT ( 'NONE',  ( 191.8436243461450488, 298.3640908547560571, -10.97913512923284785 ) ) ;
#84511=CARTESIAN_POINT ( 'NONE',  ( 158.4114053851006361, 263.3981549859118445, 17.73981754447373049 ) ) ;
#84513=CARTESIAN_POINT ( 'NONE',  ( 184.3547604609693735, 288.6018926698813516, -13.48914676681425817 ) ) ;
#84516=CARTESIAN_POINT ( 'NONE',  ( 153.2906404175950854, 265.1398178023911782, -17.60231834963988007 ) ) ;
#84518=CARTESIAN_POINT ( 'NONE',  ( 147.5848197185516142, 275.0225891520124151, 4.420251097676741736 ) ) ;
#84519=CARTESIAN_POINT ( 'NONE',  ( 190.6531941089592976, 264.1496977764022631, -9.546754457768564350 ) ) ;
#84521=CARTESIAN_POINT ( 'NONE',  ( 190.3419708194589930, 270.7651379722268530, -14.14445603664571038 ) ) ;
#84522=EDGE_CURVE ( 'NONE', #54608, #98801, #83300, .T. ) ;
#84526=CARTESIAN_POINT ( 'NONE',  ( 172.0630936339023265, 254.4764114392720273, 11.54978638049990103 ) ) ;
#84527=CARTESIAN_POINT ( 'NONE',  ( 155.6559071247401960, 261.0430556921643870, 17.79853447468815375 ) ) ;
#84528=CARTESIAN_POINT ( 'NONE',  ( 192.0172256599937555, 283.9084474676165541, -16.63802761579473710 ) ) ;
#84530=CARTESIAN_POINT ( 'NONE',  ( 76.54827242179186442, 208.8768266524160140, 9.188101187500098632 ) ) ;
#84531=CARTESIAN_POINT ( 'NONE',  ( 159.3995226465659982, 254.5589234043588078, -16.81133486613867234 ) ) ;
#84533=CARTESIAN_POINT ( 'NONE',  ( 163.4084407101100851, 247.6152736349200438, -10.68829614238923931 ) ) ;
#84535=CARTESIAN_POINT ( 'NONE',  ( 207.7296438747196134, 270.8486979012336633, -6.692930657757584001 ) ) ;
#84537=CYLINDRICAL_SURFACE ( 'NONE', #33830, 17.82106496071139645 ) ;
#84539=CARTESIAN_POINT ( 'NONE',  ( 120.0388121219831277, 230.1115022471901739, -5.000000000000041744 ) ) ;
#84542=B_SPLINE_CURVE_WITH_KNOTS ( 'NONE', 3,
 ( #97193, #20170, #97677, #88618 ),
 .UNSPECIFIED., .F., .F.,
 ( 4, 4 ),
 ( 0.000000000000000000, 0.006463808766467814271 ),
 .UNSPECIFIED. ) ;
#84543=CARTESIAN_POINT ( 'NONE',  ( 205.2387912373514212, 275.1629812233222765, -12.22529801408222383 ) ) ;
#84544=( BOUNDED_CURVE ( )  B_SPLINE_CURVE ( 2, ( #67020, #27555, #80796, #65532, #28520, #43716, #74660, #58902, #20447 ),
 .UNSPECIFIED., .F., .T. ) 
 B_SPLINE_CURVE_WITH_KNOTS ( ( 3, 2, 2, 2, 3 ),
 ( 0.6814516129032257563, 0.6827956989247311315, 0.6854838709677418818, 0.6881720430107527431, 0.6895161290322581182 ),
 .UNSPECIFIED. ) 
 CURVE ( )  GEOMETRIC_REPRESENTATION_ITEM ( )  RATIONAL_B_SPLINE_CURVE ( ( 0.9330127018922194093, 0.9330127018922194093, 1.000000000000000000, 0.8660254037844387076, 1.000000000000000000, 0.8660254037844387076, 1.000000000000000000, 0.9330127018922194093, 0.9330127018922194093 ) ) 
 REPRESENTATION_ITEM ( '' )  );
#84545=CARTESIAN_POINT ( 'NONE',  ( 157.3412122618683497, 258.1240215684019290, 16.75554199904894048 ) ) ;
#84547=EDGE_CURVE ( 'NONE', #81988, #49930, #10796, .T. ) ;
#84548=CARTESIAN_POINT ( 'NONE',  ( 28.02335264628875677, 196.1744531367911293, 4.594050593750047540 ) ) ;
#84549=B_SPLINE_CURVE_WITH_KNOTS ( 'NONE', 3,
 ( #2580, #72986, #2074, #94300 ),
 .UNSPECIFIED., .F., .F.,
 ( 4, 4 ),
 ( 0.008171735663598354502, 0.009370377214594900056 ),
 .UNSPECIFIED. ) ;
#84550=CARTESIAN_POINT ( 'NONE',  ( 57.63111678181675757, 194.8923013555409796, 4.594050593750050204 ) ) ;
#84554=CARTESIAN_POINT ( 'NONE',  ( 165.5131940759252700, 248.9191784882033005, -9.449485365452053642 ) ) ;
#84555=CARTESIAN_POINT ( 'NONE',  ( 152.3797953885492973, 246.5327760586659451, 1.948934522072303157E-15 ) ) ;
#84558=CARTESIAN_POINT ( 'NONE',  ( -6.761740748788464650, 160.2365022471902023, 10.00000000000009948 ) ) ;
#84559=FACE_OUTER_BOUND ( 'NONE', #98592, .T. ) ;
#84561=CARTESIAN_POINT ( 'NONE',  ( 64.42391676880970408, 201.8768266524159856, -9.188101187500093303 ) ) ;
#84562=CARTESIAN_POINT ( 'NONE',  ( 177.9552638626009298, 260.7378092407702184, -13.94576028113082877 ) ) ;
#84563=CARTESIAN_POINT ( 'NONE',  ( 176.2149847824938433, 291.3419163123382987, 2.559328105002660614 ) ) ;
#84565=CARTESIAN_POINT ( 'NONE',  ( 198.3523905153085423, 287.0905771551796306, 18.52598547438866206 ) ) ;
#84567=CARTESIAN_POINT ( 'NONE',  ( 150.2766721647888062, 275.5052458213636442, 7.345517456364930808 ) ) ;
#84569=CARTESIAN_POINT ( 'NONE',  ( 112.7497649734640817, 229.2365022471902023, 10.00000000000009592 ) ) ;
#84570=CARTESIAN_POINT ( 'NONE',  ( 161.4726291907278721, 250.9681975403669867, 14.52346149734912117 ) ) ;
#84571=CARTESIAN_POINT ( 'NONE',  ( 164.8869957832017690, 270.4589526275615867, -17.34276065877123330 ) ) ;
#84575=CARTESIAN_POINT ( 'NONE',  ( 159.9788992190088948, 253.5554137441726255, -15.81862932303382330 ) ) ;
#84576=CARTESIAN_POINT ( 'NONE',  ( 194.1186324107294752, 293.4280613340856689, 14.71475514768843951 ) ) ;
#84577=CARTESIAN_POINT ( 'NONE',  ( 173.2412943989675398, 277.7050541934257240, 16.79641741871846250 ) ) ;
#84578=ORIENTED_EDGE ( 'NONE', *, *, #5267, .F. ) ;
#84579=CARTESIAN_POINT ( 'NONE',  ( 68.58246938045769525, 203.7365022471902307, 10.00000000000009948 ) ) ;
#84581=CARTESIAN_POINT ( 'NONE',  ( 147.6508870500795467, 274.9081571770856272, -8.950912509993816712 ) ) ;
#84589=EDGE_LOOP ( 'NONE', ( #43505, #66091, #75241, #2892 ) ) ;
#84590=CARTESIAN_POINT ( 'NONE',  ( 132.5240116932087062, 253.9865022471903160, 10.00000000000009415 ) ) ;
#84591=DIRECTION ( 'NONE',  ( 0.4999999999999992784, -0.8660254037844390407, 0.000000000000000000 ) ) ;
#84593=CARTESIAN_POINT ( 'NONE',  ( 174.7910919356739328, 286.1561555264053709, 10.71420828047212659 ) ) ;
#84594=CARTESIAN_POINT ( 'NONE',  ( 163.2724435917976678, 283.7496115282986011, -3.044820943940299784 ) ) ;
#84597=CARTESIAN_POINT ( 'NONE',  ( 204.1793240545508752, 276.9980322128846524, 14.17550310845996187 ) ) ;
#84598=CARTESIAN_POINT ( 'NONE',  ( 159.4889735931715222, 254.4039898200529706, 16.88104032092801887 ) ) ;
#84599=CARTESIAN_POINT ( 'NONE',  ( 161.0576509603776003, 262.9785022463822202, -17.65625271138400976 ) ) ;
#84600=CARTESIAN_POINT ( 'NONE',  ( 164.6290063521823868, 245.5011919288776028, 5.622032409704942779 ) ) ;
#84601=CARTESIAN_POINT ( 'NONE',  ( 159.5585398265464221, 254.8728140044053134, -15.62969674525248642 ) ) ;
#84603=CARTESIAN_POINT ( 'NONE',  ( 181.8843194246268808, 260.3488174177143719, 9.482408816024305409 ) ) ;
#84604=CARTESIAN_POINT ( 'NONE',  ( 70.72975101405640430, 202.4548013555409796, -4.594050593750042211 ) ) ;
#84606=CARTESIAN_POINT ( 'NONE',  ( 173.9522839582943163, 265.4328302768140588, 16.77064627941505748 ) ) ;
#84607=CARTESIAN_POINT ( 'NONE',  ( -22.42236680055709641, 157.8615022471902591, 0.000000000000000000 ) ) ;
#84609=ORIENTED_EDGE ( 'NONE', *, *, #80886, .T. ) ;
#84610=CARTESIAN_POINT ( 'NONE',  ( 160.8697417715285951, 254.0124291816641176, 15.72951850990217437 ) ) ;
#84612=EDGE_LOOP ( 'NONE', ( #59724, #76963, #10798, #86806 ) ) ;
#84617=CARTESIAN_POINT ( 'NONE',  ( 194.2764122224708103, 294.1503786489221284, 15.46903869661980835 ) ) ;
#84618=CARTESIAN_POINT ( 'NONE',  ( 72.70404828370719486, 224.3297689869269789, -2.679491924311252493 ) ) ;
#84619=CARTESIAN_POINT ( 'NONE',  ( 75.30318735596920021, 214.2833772461660544, -9.188101187500095079 ) ) ;
#84621=CARTESIAN_POINT ( 'NONE',  ( 201.0579808891486380, 282.4043571632192311, -17.91925047041473107 ) ) ;
#84623=CARTESIAN_POINT ( 'NONE',  ( 93.04999876614748189, 212.9824982072973683, 3.021315404115420679E-15 ) ) ;
#84624=EDGE_CURVE ( 'NONE', #24993, #92061, #59015, .T. ) ;
#84625=CARTESIAN_POINT ( 'NONE',  ( 183.9161760165103772, 275.2808736645490626, 16.40347525101666193 ) ) ;
#84626=CARTESIAN_POINT ( 'NONE',  ( 165.0565241268390366, 244.7607094220335568, 2.191926263411719589 ) ) ;
#84627=CARTESIAN_POINT ( 'NONE',  ( 162.5349543250319471, 283.9950716909000903, 0.5116008960414863971 ) ) ;
#84628=CARTESIAN_POINT ( 'NONE',  ( 195.1300253905141631, 279.2719974992415359, 16.35492678998735983 ) ) ;
#84629=CARTESIAN_POINT ( 'NONE',  ( 160.4812992605921238, 260.2430605036401516, 16.67286839615865546 ) ) ;
#84631=CARTESIAN_POINT ( 'NONE',  ( 192.1520400720565078, 296.4596862432644571, 11.25539976459215374 ) ) ;
#84632=CARTESIAN_POINT ( 'NONE',  ( 185.4907235204558447, 259.9682112630936786, 5.899277730949330945 ) ) ;
#84634=CARTESIAN_POINT ( 'NONE',  ( 201.1755594471486859, 282.2007051268825535, -18.15567516623250910 ) ) ;
#84637=EDGE_CURVE ( 'NONE', #13195, #71254, #5938, .T. ) ;
#84639=ORIENTED_EDGE ( 'NONE', *, *, #15644, .T. ) ;
#84640=CARTESIAN_POINT ( 'NONE',  ( 195.7061616849477730, 265.3944924174461448, 4.819710038644158701 ) ) ;
#84641=CARTESIAN_POINT ( 'NONE',  ( 201.4430264223318261, 273.1213752465389462, 13.07311719109280546 ) ) ;
#84643=CARTESIAN_POINT ( 'NONE',  ( 184.6976757848609623, 263.8739595640468565, -12.18454262072885541 ) ) ;
#84645=CARTESIAN_POINT ( 'NONE',  ( 195.8374195215319560, 264.5068004645912652, 0.8301787805199302150 ) ) ;
#84647=CARTESIAN_POINT ( 'NONE',  ( 147.4963928429778264, 275.1757489932608109, 4.929816573182678852 ) ) ;
#84648=CARTESIAN_POINT ( 'NONE',  ( 186.5996133936216097, 282.5293965020246674, 16.20464955667571871 ) ) ;
#84651=CARTESIAN_POINT ( 'NONE',  ( 167.5815824773973191, 259.8598515869122707, -16.53346283481762313 ) ) ;
#84654=CARTESIAN_POINT ( 'NONE',  ( 148.9517569034208009, 272.6549844970639924, 12.50737104496728236 ) ) ;
#84655=CARTESIAN_POINT ( 'NONE',  ( 166.1327689491646709, 286.5586531720609855, -3.311317316613562767 ) ) ;
#84659=CARTESIAN_POINT ( 'NONE',  ( 144.0529748775411463, 260.6427522451418781, 10.00000000000009237 ) ) ;
#84666=DIRECTION ( 'NONE',  ( 0.4999999999999998890, -0.8660254037844385966, 0.000000000000000000 ) ) ;
#84667=CARTESIAN_POINT ( 'NONE',  ( 7.969365115964080815, 187.6589784336661637, -6.496448406907676862E-16 ) ) ;
#84668=CARTESIAN_POINT ( 'NONE',  ( 176.1757538807019330, 265.5509619629168583, -16.23131976009116784 ) ) ;
#84669=CARTESIAN_POINT ( 'NONE',  ( 171.9467656383669123, 290.1344116725977642, 2.734564134658529877 ) ) ;
#84670=CARTESIAN_POINT ( 'NONE',  ( 179.5568545132203440, 274.2926861780458125, -16.60646468900087314 ) ) ;
#84672=CARTESIAN_POINT ( 'NONE',  ( 181.0304098800548331, 294.4207640661956020, 6.547035950180724484 ) ) ;
#84673=CARTESIAN_POINT ( 'NONE',  ( 173.0199565421851560, 272.3281153120731233, -16.37689176781418610 ) ) ;
#84674=CARTESIAN_POINT ( 'NONE',  ( 156.5950988087852238, 281.5581451644223421, -2.717916794402165603 ) ) ;
#84675=B_SPLINE_SURFACE_WITH_KNOTS ( 'NONE', 3, 1, ( 
 ( #76434, #43513 ),
 ( #60191, #6525 ),
 ( #91152, #22215 ),
 ( #99230, #28311 ),
 ( #59189, #60690 ),
 ( #5523, #14622 ),
 ( #97258, #90165 ),
 ( #82577, #36910 ),
 ( #74452, #90674 ),
 ( #29816, #21717 ),
 ( #84069, #98239 ),
 ( #83558, #45501 ),
 ( #36407, #7009 ),
 ( #52109, #89675 ),
 ( #20738, #83056 ),
 ( #13629, #86573 ),
 ( #62193, #23201 ),
 ( #24219, #92171 ),
 ( #93654, #55099 ),
 ( #77929, #39389 ),
 ( #39886, #17106 ),
 ( #62697, #919 ),
 ( #53600, #47506 ),
 ( #48002, #45988 ),
 ( #1430, #8520 ),
 ( #78946, #37894 ),
 ( #76905, #22721 ),
 ( #86086, #30819 ),
 ( #69313, #93144 ),
 ( #24707, #9014 ),
 ( #16610, #70306 ),
 ( #77431, #54092 ),
 ( #78433, #94154 ),
 ( #55590, #7503 ) ),
 .UNSPECIFIED., .T., .F., .F.,
 ( 4, 2, 2, 2, 2, 2, 2, 2, 2, 2, 2, 2, 2, 2, 2, 2, 4 ),
 ( 2, 2 ),
 ( 0.000000000000000000, 0.06250000000000000000, 0.1250000000000000000, 0.1875000000000000000, 0.2500000000000000000, 0.3125000000000000000, 0.3750000000000000000, 0.4375000000000000000, 0.5000000000000000000, 0.5625000000000000000, 0.6250000000000000000, 0.6875000000000000000, 0.7500000000000000000, 0.8125000000000000000, 0.8750000000000000000, 0.9375000000000000000, 1.000000000000000000 ),
 ( 0.000000000000000000, 1.000000000000000000 ),
 .UNSPECIFIED. ) ;
#84678=CARTESIAN_POINT ( 'NONE',  ( 191.4137818629626508, 260.8670317507109644, -1.392421146808482169 ) ) ;
#84679=CARTESIAN_POINT ( 'NONE',  ( 183.1080230832341726, 295.7359842595169539, 1.141048727436130727 ) ) ;
#84680=CARTESIAN_POINT ( 'NONE',  ( 76.37669801451764329, 208.2365022471902023, 10.00000000000009592 ) ) ;
#84682=CARTESIAN_POINT ( 'NONE',  ( 147.6947327179224487, 274.8322142526899370, 9.090449717876689206 ) ) ;
#84683=CARTESIAN_POINT ( 'NONE',  ( 22.06942799527072907, 192.7369531367911293, -4.594050593750048428 ) ) ;
#84687=CARTESIAN_POINT ( 'NONE',  ( 199.2205425252482200, 285.5868937652708155, -18.05012564782189344 ) ) ;
#84688=CARTESIAN_POINT ( 'NONE',  ( 164.8329445879545290, 245.1479605429143760, -2.955380775890217304 ) ) ;
#84689=CARTESIAN_POINT ( 'NONE',  ( 198.2505066714982149, 285.2670451491296149, 0.000000000000000000 ) ) ;
#84690=CARTESIAN_POINT ( 'NONE',  ( 163.1799518951598600, 280.9192836996226674, -10.08564493774514403 ) ) ;
#84691=CARTESIAN_POINT ( 'NONE',  ( 179.7565560748202813, 262.9145626453345130, -12.95070181807916043 ) ) ;
#84694=CARTESIAN_POINT ( 'NONE',  ( 189.8147415777049218, 301.8782188922952514, -0.5019643756309712934 ) ) ;
#84696=CARTESIAN_POINT ( 'NONE',  ( 194.2669918475045279, 294.1666952169902629, 14.00965265288584050 ) ) ;
#84705=B_SPLINE_CURVE_WITH_KNOTS ( 'NONE', 3,
 ( #83704, #6162, #16753, #78069, #23342, #17250, #16253, #94296, #85719, #62845, #8656, #71476, #40035, #70976, #32460, #79097, #25352, #47641, #40542, #48154, #56244, #86216, #1577, #9159, #38545, #61840, #55725, #46648, #87237, #54230, #31940, #9681, #78575, #30951, #46133, #94792, #63357, #85197, #68, #7654, #24851, #92787, #63854, #77046, #86713, #54736, #15740, #31442, #77573, #2069, #32949, #8162 ),
 .UNSPECIFIED., .F., .F.,
 ( 4, 2, 2, 2, 2, 2, 2, 2, 2, 2, 2, 2, 2, 2, 2, 2, 2, 2, 2, 2, 2, 2, 2, 2, 2, 4 ),
 ( 0.0008616133506683544942, 0.001349225619325013920, 0.001836837887981673453, 0.002080644022310002787, 0.002324450156638332987, 0.002446353223802498738, 0.002568256290966664922, 0.002690159358130831107, 0.002812062425294997291, 0.003055868559623329660, 0.003299674693951661596, 0.003787286962608326334, 0.004762511499921721729, 0.005737736037235116257, 0.006225348305891820894, 0.006469154440220215713, 0.006712960574548609664, 0.006773912108130736992, 0.006834863641712863452, 0.006895815175294989913, 0.006956766708877116373, 0.007200572843205529407, 0.007688185111862339861, 0.008175797380519149449, 0.008419603514847556411, 0.008663409649175963373 ),
 .UNSPECIFIED. ) ;
#84708=EDGE_CURVE ( 'NONE', #68859, #8907, #53475, .T. ) ;
#84712=ORIENTED_EDGE ( 'NONE', *, *, #31466, .F. ) ;
#84713=CARTESIAN_POINT ( 'NONE',  ( 151.3560786774222322, 268.4905770267490652, 15.54402364351346932 ) ) ;
#84716=CARTESIAN_POINT ( 'NONE',  ( 45.26186829773988052, 208.4860189848785410, -2.679491924311252493 ) ) ;
#84717=EDGE_CURVE ( 'NONE', #2713, #5430, #92981, .T. ) ;
#84719=CARTESIAN_POINT ( 'NONE',  ( 189.8136646974935786, 301.8800841035353528, -0.6430783927310335102 ) ) ;
#84720=CARTESIAN_POINT ( 'NONE',  ( 149.2765980486851731, 272.0923431290771646, -11.40617906909507973 ) ) ;
#84721=CARTESIAN_POINT ( 'NONE',  ( 174.6653058907003526, 271.2610659076526076, 17.81995586319052549 ) ) ;
#84723=CARTESIAN_POINT ( 'NONE',  ( 157.0848929289108469, 258.5679796760466047, 17.57466231005294688 ) ) ;
#84724=CARTESIAN_POINT ( 'NONE',  ( 158.3850792441787689, 265.2446733984589287, 17.11029620794053940 ) ) ;
#84738=CARTESIAN_POINT ( 'NONE',  ( 175.1013262022588037, 291.4808567457044433, 5.510497698069581674 ) ) ;
#84739=CARTESIAN_POINT ( 'NONE',  ( 148.2980785574368952, 273.7871886041155562, 9.134436720559454770 ) ) ;
#84740=CARTESIAN_POINT ( 'NONE',  ( 149.3883679478359454, 271.8987519849911223, 12.99187507659642371 ) ) ;
#84741=CARTESIAN_POINT ( 'NONE',  ( 141.2767884429413243, 240.8262482093457777, 3.021315404115420679E-15 ) ) ;
#84743=CARTESIAN_POINT ( 'NONE',  ( 147.1259762202154207, 275.8173294038533641, -0.6716460511724978710 ) ) ;
#84744=CARTESIAN_POINT ( 'NONE',  ( -22.42236680055709641, 157.8615022471902591, 0.000000000000000000 ) ) ;
#84750=VERTEX_POINT ( 'NONE', #93989 ) ;
#84751=CARTESIAN_POINT ( 'NONE',  ( 190.4076394944172250, 300.8512895768478188, -4.816292592624366264 ) ) ;
#84752=B_SPLINE_CURVE_WITH_KNOTS ( 'NONE', 3,
 ( #14401, #687, #22491, #46788 ),
 .UNSPECIFIED., .F., .F.,
 ( 4, 4 ),
 ( 0.01075463767794331005, 0.01639907954706086926 ),
 .UNSPECIFIED. ) ;
#84760=CARTESIAN_POINT ( 'NONE',  ( 169.2719858167531584, 285.1210977770464865, -7.931911058023441541 ) ) ;
#84762=CARTESIAN_POINT ( 'NONE',  ( 162.6262389125959373, 248.9700868899859074, -10.50380342094597808 ) ) ;
#84763=ADVANCED_FACE ( 'NONE', ( #39221 ), #741, .T. ) ;
#84766=CARTESIAN_POINT ( 'NONE',  ( 46.26427303354824261, 207.5177522451419065, 5.000000000000046185 ) ) ;
#84767=CARTESIAN_POINT ( 'NONE',  ( 123.0428377395863890, 241.8458772461660544, 9.188101187500095079 ) ) ;
#84768=CARTESIAN_POINT ( 'NONE',  ( 198.8533049117289977, 286.2229679703367538, -18.60939981449148561 ) ) ;
#84770=CARTESIAN_POINT ( 'NONE',  ( 196.1613785401733878, 290.8855212161054737, 15.98157687694135021 ) ) ;
#84771=CARTESIAN_POINT ( 'NONE',  ( 174.8240844530040761, 253.1383486689193774, -3.879012981929475856 ) ) ;
#84772=CARTESIAN_POINT ( 'NONE',  ( 49.15987193134396449, 205.3149278399160949, -9.188101187500095079 ) ) ;
#84773=CARTESIAN_POINT ( 'NONE',  ( 175.3149167492775860, 290.9749816300547991, -6.569057798006298299 ) ) ;
#84777=CARTESIAN_POINT ( 'NONE',  ( 181.0877019475456962, 267.6761920141779569, 14.99829969603863944 ) ) ;
#84779=CARTESIAN_POINT ( 'NONE',  ( 190.2648877593310317, 301.0985428348857340, -4.426259207433023590 ) ) ;
#84781=CARTESIAN_POINT ( 'NONE',  ( 156.0916382163451601, 277.5285333452508212, -10.52960063827285886 ) ) ;
#84782=CARTESIAN_POINT ( 'NONE',  ( 164.1065032853484240, 250.1265725945117140, 10.86380703882780452 ) ) ;
#84784=CARTESIAN_POINT ( 'NONE',  ( 99.88567928453477407, 235.1427522451419350, 10.00000000000009237 ) ) ;
#84787=CARTESIAN_POINT ( 'NONE',  ( 162.9796882977680639, 248.3578945969637743, 9.683801903336119565 ) ) ;
#84788=CARTESIAN_POINT ( 'NONE',  ( 208.3699316049496133, 269.7396870210121733, -1.898463622294385811 ) ) ;
#84789=CARTESIAN_POINT ( 'NONE',  ( 21.28450569914983248, 195.3464784336661637, 1.353441290958777327E-15 ) ) ;
#84791=CARTESIAN_POINT ( 'NONE',  ( 192.3278524167367891, 272.0202382274233628, 14.20356147229779964 ) ) ;
#84794=CARTESIAN_POINT ( 'NONE',  ( 198.2817570091511925, 277.3855417112700934, -15.35505783437617566 ) ) ;
#84795=CARTESIAN_POINT ( 'NONE',  ( 68.80799682758592439, 210.5333772461660544, 9.188101187500095079 ) ) ;
#84796=CARTESIAN_POINT ( 'NONE',  ( 161.1089126327036354, 251.5981730984191529, 13.95161017039218976 ) ) ;
#84798=CARTESIAN_POINT ( 'NONE',  ( 45.49391910530875549, 208.6199935810940929, 2.679491924311251605 ) ) ;
#84802=CARTESIAN_POINT ( 'NONE',  ( 3.125382611083808104, 182.6115022471903160, -5.000000000000047962 ) ) ;
#84803=CARTESIAN_POINT ( 'NONE',  ( 208.1757572214753793, 270.0760069187178374, 2.172546422564154867 ) ) ;
#84804=CARTESIAN_POINT ( 'NONE',  ( -8.674473839076844328, 174.9869531367911293, 4.594050593750046652 ) ) ;
#84806=CARTESIAN_POINT ( 'NONE',  ( 166.6645348857815350, 262.0116583737346900, -16.28251305985784114 ) ) ;
#84807=CARTESIAN_POINT ( 'NONE',  ( 189.0517344710061138, 261.8661741762242059, 6.550959291050514999 ) ) ;
#84808=CARTESIAN_POINT ( 'NONE',  ( 206.0041637419966776, 273.8373171585603814, 11.66586596407113596 ) ) ;
#84811=CARTESIAN_POINT ( 'NONE',  ( 185.3943831185000874, 277.6506735163841313, -17.55462980397184580 ) ) ;
#84815=CARTESIAN_POINT ( 'NONE',  ( 208.3303207624000777, 269.8082950128387552, -0.5527213369959232958 ) ) ;
#84816=EDGE_CURVE ( 'NONE', #17862, #18980, #42170, .T. ) ;
#84817=CARTESIAN_POINT ( 'NONE',  ( 177.9378665411170743, 286.3192117283503535, 13.07754552029243733 ) ) ;
#84818=DIRECTION ( 'NONE',  ( -0.8660254037844387076, -0.4999999999999998890, -0.000000000000000000 ) ) ;
#84821=CARTESIAN_POINT ( 'NONE',  ( 206.6055738272482927, 272.7956443347203503, 9.336287257528914196 ) ) ;
#84822=CARTESIAN_POINT ( 'NONE',  ( -6.563276597302431625, 157.0177522451417929, 5.000000000000051514 ) ) ;
#84824=DIRECTION ( 'NONE',  ( -0.8660254037844387076, -0.4999999999999998890, -0.000000000000000000 ) ) ;
#84825=CARTESIAN_POINT ( 'NONE',  ( 191.1092559216791074, 295.6699157252775194, 12.62328014874510274 ) ) ;
#84827=CARTESIAN_POINT ( 'NONE',  ( 162.7070706717508699, 248.8300821762643693, -9.986337079333621247 ) ) ;
#84828=CARTESIAN_POINT ( 'NONE',  ( 153.2513309553138470, 265.2079037882803618, -16.24091495603130397 ) ) ;
#84829=( BOUNDED_CURVE ( )  B_SPLINE_CURVE ( 2, ( #65078, #96028, #49878, #47857, #11408, #71200, #42261, #73196, #34671 ),
 .UNSPECIFIED., .F., .T. ) 
 B_SPLINE_CURVE_WITH_KNOTS ( ( 3, 2, 2, 2, 3 ),
 ( 0.5362903225806451291, 0.5376344086021505042, 0.5403225806451612545, 0.5430107526881720048, 0.5443548387096773800 ),
 .UNSPECIFIED. ) 
 CURVE ( )  GEOMETRIC_REPRESENTATION_ITEM ( )  RATIONAL_B_SPLINE_CURVE ( ( 0.9330127018922194093, 0.9330127018922194093, 1.000000000000000000, 0.8660254037844387076, 1.000000000000000000, 0.8660254037844387076, 1.000000000000000000, 0.9330127018922194093, 0.9330127018922194093 ) ) 
 REPRESENTATION_ITEM ( '' )  );
#84830=ORIENTED_EDGE ( 'NONE', *, *, #62519, .T. ) ;
#84831=CARTESIAN_POINT ( 'NONE',  ( 190.8753273331982427, 280.9408420453412987, 16.64646941022040849 ) ) ;
#84832=CARTESIAN_POINT ( 'NONE',  ( 190.0656191383575333, 292.0158714553608661, 14.79701615165662254 ) ) ;
#84834=CARTESIAN_POINT ( 'NONE',  ( 148.9230895364621574, 272.7046378331555161, 12.20434325797056019 ) ) ;
#84836=CARTESIAN_POINT ( 'NONE',  ( 190.2248117571934642, 297.8128940847054196, 8.178623448509318550 ) ) ;
#84838=CARTESIAN_POINT ( 'NONE',  ( 146.5865263025993954, 276.7516840693029962, 0.4918294119671828835 ) ) ;
#84840=CARTESIAN_POINT ( 'NONE',  ( 197.0184425104562820, 289.4010428742387262, -16.90752553128928426 ) ) ;
#84843=ORIENTED_EDGE ( 'NONE', *, *, #26826, .F. ) ;
#84844=CARTESIAN_POINT ( 'NONE',  ( 107.7791399978856930, 233.0333772461660828, 9.188101187500095079 ) ) ;
#84846=CARTESIAN_POINT ( 'NONE',  ( 190.7851866479434761, 300.1973587246873194, 7.931162401707728016 ) ) ;
#84850=ORIENTED_EDGE ( 'NONE', *, *, #34910, .T. ) ;
#84852=EDGE_LOOP ( 'NONE', ( #60459, #6744, #38449, #32329 ) ) ;
#84854=ORIENTED_EDGE ( 'NONE', *, *, #79545, .F. ) ;
#84855=CARTESIAN_POINT ( 'NONE',  ( 207.6590484093196096, 270.9709728340903894, 3.402057849327809524 ) ) ;
#84857=CARTESIAN_POINT ( 'NONE',  ( 165.8975677354378035, 271.5909624305264174, 17.28637137770206067 ) ) ;
#84858=CARTESIAN_POINT ( 'NONE',  ( 168.1505686650465350, 281.2677474040732477, 11.64546357986301750 ) ) ;
#84859=CARTESIAN_POINT ( 'NONE',  ( 148.3874010092782498, 273.6324775792697892, -8.328854486678444857 ) ) ;
#84862=VERTEX_POINT ( 'NONE', #36685 ) ;
#84863=CARTESIAN_POINT ( 'NONE',  ( 166.9825626143087050, 247.0767275159285816, 1.933851161157992271 ) ) ;
#84865=CARTESIAN_POINT ( 'NONE',  ( 201.9679975669502312, 279.1647446829476280, -15.96203686199545579 ) ) ;
#84867=CARTESIAN_POINT ( 'NONE',  ( 115.9793180381955580, 247.7677522451419065, -5.000000000000047962 ) ) ;
#84869=CARTESIAN_POINT ( 'NONE',  ( 202.6070187115982719, 279.7213449518906145, 15.56322169823762280 ) ) ;
#84870=CARTESIAN_POINT ( 'NONE',  ( 206.1408608592916494, 273.6005508061571732, -10.42739367433323494 ) ) ;
#84875=CARTESIAN_POINT ( 'NONE',  ( 161.3227470381586102, 251.2278010437646856, 14.45097375514160731 ) ) ;
#84877=CARTESIAN_POINT ( 'NONE',  ( 194.1200050480437653, 262.3566822754066834, -0.8120440885529029984 ) ) ;
#84878=ORIENTED_EDGE ( 'NONE', *, *, #79291, .F. ) ;
#84879=CARTESIAN_POINT ( 'NONE',  ( 155.0719444836497871, 262.0545086562551091, -18.28771400695536187 ) ) ;
#84881=CARTESIAN_POINT ( 'NONE',  ( 174.8696466734779449, 292.3029143586743430, -1.153856708368909967 ) ) ;
#84882=ADVANCED_FACE ( 'NONE', ( #4822 ), #42293, .T. ) ;
#84883=CARTESIAN_POINT ( 'NONE',  ( 11.62325688217078223, 167.5177522451418213, 5.000000000000051514 ) ) ;
#84884=CARTESIAN_POINT ( 'NONE',  ( 192.7752508616301839, 267.0407549221993690, -11.17594988838974501 ) ) ;
#84886=CARTESIAN_POINT ( 'NONE',  ( 169.9163657913202314, 280.6881826668949316, -14.21246854472871490 ) ) ;
#84888=CARTESIAN_POINT ( 'NONE',  ( 6.913983429043053519, 183.9869531367911009, 4.594050593750046652 ) ) ;
#84889=CARTESIAN_POINT ( 'NONE',  ( 114.8426596992765099, 227.1115022471901739, -5.000000000000041744 ) ) ;
#84893=CARTESIAN_POINT ( 'NONE',  ( 128.2864073861747727, 233.3262482093457493, 3.021315404115420679E-15 ) ) ;
#84894=B_SPLINE_CURVE_WITH_KNOTS ( 'NONE', 3,
 ( #770, #62553, #31163, #47368, #61064, #31656, #7889, #76304, #69670, #30176, #276, #38766, #14491, #92033, #83927, #91515, #37278, #85945, #7370, #45854, #16473, #62052, #76777, #99102, #45371, #29686, #22082, #54448, #6876, #85425, #46874, #38255, #23061, #84913, #30685, #61565, #92513, #53956, #15456, #9381, #25070, #24569, #55948, #39742, #49378, #17995, #86944, #40756, #78291, #26589 ),
 .UNSPECIFIED., .F., .F.,
 ( 4, 2, 2, 2, 2, 2, 2, 2, 2, 2, 2, 2, 2, 2, 2, 2, 2, 2, 2, 2, 2, 2, 2, 2, 4 ),
 ( 0.0001377106324937234195, 0.001145886038797477424, 0.001397929890373450328, 0.001649973741949423232, 0.001775995667737409684, 0.001902017593525396136, 0.002028039519313382371, 0.002154061445101369040, 0.002406105296677414802, 0.002658149148253460565, 0.003162236851405497012, 0.004170412257709569907, 0.005178587664013642802, 0.005682675367165642387, 0.005934719218741604449, 0.006060741144529589383, 0.006186763070317573450, 0.006249774033211555509, 0.006312784996105537567, 0.006438806921893589288, 0.006690850773469821100, 0.007194938476622280386, 0.007699026179774738805, 0.007951070031351023526, 0.008203113882927307379 ),
 .UNSPECIFIED. ) ;
#84897=CARTESIAN_POINT ( 'NONE',  ( 201.9545259124544145, 280.8514956315805193, -16.42775064268253615 ) ) ;
#84899=CARTESIAN_POINT ( 'NONE',  ( 149.8380350131166949, 277.0589241956989781, 3.095230065015505350 ) ) ;
#84900=CARTESIAN_POINT ( 'NONE',  ( 16.57566611395445477, 186.5024278399160949, 9.188101187500095079 ) ) ;
#84901=CARTESIAN_POINT ( 'NONE',  ( 117.0621101165238542, 229.2048013555409796, 4.594050593750051981 ) ) ;
#84902=CARTESIAN_POINT ( 'NONE',  ( 178.9043521614821941, 291.7907940003793783, -6.168293200034719703 ) ) ;
#84903=CARTESIAN_POINT ( 'NONE',  ( 195.8788359694280814, 275.2028430888133812, 15.68988939746534328 ) ) ;
#84904=CARTESIAN_POINT ( 'NONE',  ( 34.75566377745538205, 179.3262482093457493, 3.021315404115420679E-15 ) ) ;
#84905=CARTESIAN_POINT ( 'NONE',  ( 177.8872019327756959, 273.7990604926155811, -17.82423047383818471 ) ) ;
#84906=CARTESIAN_POINT ( 'NONE',  ( -7.835251407336910390, 166.2833772461660828, -9.188101187500095079 ) ) ;
#84908=CARTESIAN_POINT ( 'NONE',  ( 155.6126298223767890, 261.1180141786725244, 18.15400560664037855 ) ) ;
#84909=CARTESIAN_POINT ( 'NONE',  ( 161.8935665241663457, 250.2391126920490194, -13.69501063978231770 ) ) ;
#84913=CARTESIAN_POINT ( 'NONE',  ( 171.4787937661881756, 279.8757557646238183, 13.90305814568919018 ) ) ;
#84914=CARTESIAN_POINT ( 'NONE',  ( 174.5508403973756515, 260.3590064504865040, -14.93617697178709314 ) ) ;
#84916=CARTESIAN_POINT ( 'NONE',  ( 147.8465295590381743, 274.5692944114487091, 9.322947948439978205 ) ) ;
#84917=CARTESIAN_POINT ( 'NONE',  ( 181.4235159426282564, 267.2807182867468327, -14.77487836696800194 ) ) ;
#84921=CARTESIAN_POINT ( 'NONE',  ( 94.51795245455393513, 231.5024278399160949, 9.188101187500095079 ) ) ;
#84923=CARTESIAN_POINT ( 'NONE',  ( 151.3560786774222322, 268.4905770267490652, 15.54402364351346932 ) ) ;
#84926=CARTESIAN_POINT ( 'NONE',  ( 195.1427698080798336, 279.1118193537853927, 16.30781815010357860 ) ) ;
#84927=CARTESIAN_POINT ( 'NONE',  ( 201.1614673384707714, 270.3972314152816807, -10.08402632729127646 ) ) ;
#84928=CYLINDRICAL_SURFACE ( 'NONE', #48734, 10.00000000000010658 ) ;
#84929=CARTESIAN_POINT ( 'NONE',  ( 149.7819113862974802, 271.9648479771055918, -11.46454315534134238 ) ) ;
#84930=EDGE_CURVE ( 'NONE', #28329, #96454, #20487, .T. ) ;
#84937=CARTESIAN_POINT ( 'NONE',  ( 196.5898038174904343, 267.5261605945568135, 9.655523290058249941 ) ) ;
#84938=CARTESIAN_POINT ( 'NONE',  ( 149.6191398986701415, 271.4990432411842676, -11.66821883946526839 ) ) ;
#84943=CARTESIAN_POINT ( 'NONE',  ( 182.3700640764176342, 263.2847133751610045, -13.94439451147478337 ) ) ;
#84946=CARTESIAN_POINT ( 'NONE',  ( 152.6757560589063303, 266.2048287524194166, 16.73757896668104195 ) ) ;
#84948=CARTESIAN_POINT ( 'NONE',  ( 187.5265405544104453, 278.9627198005699711, 16.98281552316259280 ) ) ;
#84950=ORIENTED_EDGE ( 'NONE', *, *, #96210, .T. ) ;
#84951=CARTESIAN_POINT ( 'NONE',  ( 167.5733308811266227, 249.8690179723528217, 6.942995308039366265 ) ) ;
#84957=CARTESIAN_POINT ( 'NONE',  ( 158.7690100866489900, 256.4985079616176336, 16.45054074394984056 ) ) ;
#84959=CARTESIAN_POINT ( 'NONE',  ( 192.8895823079093077, 296.5524385223993136, -11.97278429023368496 ) ) ;
#84960=CARTESIAN_POINT ( 'NONE',  ( 179.9209375999747351, 276.5811748711908535, 17.74520275588677265 ) ) ;
#84965=CARTESIAN_POINT ( 'NONE',  ( 196.1370092075112268, 290.1209220278959720, 16.40156295354631411 ) ) ;
#84968=CARTESIAN_POINT ( 'NONE',  ( 169.4056471164851132, 269.1093820582442504, 17.36518709487519629 ) ) ;
#84970=CARTESIAN_POINT ( 'NONE',  ( 164.4679336850620075, 246.2674076979392339, 2.485468002151889344 ) ) ;
#84971=CARTESIAN_POINT ( 'NONE',  ( 205.9252530167937323, 273.9739945438741984, -10.37964514155334328 ) ) ;
#84972=CARTESIAN_POINT ( 'NONE',  ( 199.7100744728227539, 274.3991700604664175, -13.57366607680039294 ) ) ;
#84973=DIRECTION ( 'NONE',  ( -0.4999999999999987788, 0.8660254037844392627, 0.000000000000000000 ) ) ;
#84974=CARTESIAN_POINT ( 'NONE',  ( 192.6247335881259630, 297.0111699613833594, -13.30158778996737290 ) ) ;
#84975=CARTESIAN_POINT ( 'NONE',  ( 171.5508816557387206, 250.5181571520007537, -5.758755346447887113 ) ) ;
#84977=CARTESIAN_POINT ( 'NONE',  ( 186.7062459033451489, 286.9011594067970350, -15.58169422348589350 ) ) ;
#84978=CARTESIAN_POINT ( 'NONE',  ( 117.8466853168797428, 238.8458772461660544, 9.188101187500095079 ) ) ;
#84981=CARTESIAN_POINT ( 'NONE',  ( 179.1400961457673304, 290.0475676899061455, -9.404149003805263973 ) ) ;
#84985=EDGE_CURVE ( 'NONE', #55984, #83319, #68723, .T. ) ;
#84988=CARTESIAN_POINT ( 'NONE',  ( 146.7445232850756156, 276.4780252682116384, 2.895314788918020632 ) ) ;
#84990=CARTESIAN_POINT ( 'NONE',  ( 153.3506059258413643, 265.0359544954067132, -16.39100908615009899 ) ) ;
#84992=VERTEX_POINT ( 'NONE', #21993 ) ;
#84993=CARTESIAN_POINT ( 'NONE',  ( 147.9909379325378609, 274.3191717715091045, 10.08496620488601181 ) ) ;
#84995=CARTESIAN_POINT ( 'NONE',  ( 148.0826818691893152, 274.1602666119424043, -9.371267383421741926 ) ) ;
#84998=CARTESIAN_POINT ( 'NONE',  ( 188.0217698280969501, 266.1369699381889973, -11.79292520403407885 ) ) ;
#85001=CARTESIAN_POINT ( 'NONE',  ( 159.0065368070590353, 277.8476692937898065, 10.29608560019760155 ) ) ;
#85002=CARTESIAN_POINT ( 'NONE',  ( 196.1341231099717959, 264.6386869773598960, 3.834808299373879237 ) ) ;
#85003=CARTESIAN_POINT ( 'NONE',  ( 158.3858271822887218, 263.3851922276277833, 17.76837769191611116 ) ) ;
#85007=CARTESIAN_POINT ( 'NONE',  ( 152.8651171364917900, 265.8768457450651113, -16.25664868183201861 ) ) ;
#85009=CARTESIAN_POINT ( 'NONE',  ( 190.7403173041394950, 300.2750747078583800, -4.254144485856557800 ) ) ;
#85010=FACE_OUTER_BOUND ( 'NONE', #40091, .T. ) ;
#85011=CARTESIAN_POINT ( 'NONE',  ( 186.7460619612521953, 262.7540144476575961, -8.976403499855448942 ) ) ;
#85014=CARTESIAN_POINT ( 'NONE',  ( 189.0314999406332959, 269.9387407235815886, -14.02374420418258794 ) ) ;
#85015=CARTESIAN_POINT ( 'NONE',  ( 188.5113832660517232, 298.5244903283103781, -4.265124716804361782 ) ) ;
#85021=CARTESIAN_POINT ( 'NONE',  ( 79.63366147065640632, 204.5327760586659451, 1.948934522072303157E-15 ) ) ;
#85024=CARTESIAN_POINT ( 'NONE',  ( 49.55341318909624704, 210.9637435831424739, 2.679491924311251605 ) ) ;
#85025=CARTESIAN_POINT ( 'NONE',  ( 203.1526193585190470, 278.7763369107815379, -16.67658907091021447 ) ) ;
#85026=CARTESIAN_POINT ( 'NONE',  ( 207.8984236726843164, 270.5563627158673512, -6.084369154771423815 ) ) ;
#85028=CARTESIAN_POINT ( 'NONE',  ( 40.12992642340848448, 200.6427522451419065, 10.00000000000009415 ) ) ;
#85031=DIRECTION ( 'NONE',  ( -0.8660254037844392627, -0.4999999999999987232, 0.000000000000000000 ) ) ;
#85032=CARTESIAN_POINT ( 'NONE',  ( 169.1058430229814462, 251.9997932694548126, -8.779696520905575952 ) ) ;
#85033=CARTESIAN_POINT ( 'NONE',  ( 163.9708803696611028, 246.6410995683858118, -5.146160866179791071 ) ) ;
#85034=CARTESIAN_POINT ( 'NONE',  ( 157.2168982216852555, 258.3393398020932636, 18.09635675623264106 ) ) ;
#85035=CARTESIAN_POINT ( 'NONE',  ( 190.2244606332360490, 298.9447751924984118, -8.130533059491476422 ) ) ;
#85036=CARTESIAN_POINT ( 'NONE',  ( 161.6923300915171922, 250.5876644177310482, -14.43081872899884566 ) ) ;
#85037=CARTESIAN_POINT ( 'NONE',  ( 19.79611131033658111, 191.4244531367911293, -4.594050593750046652 ) ) ;
#85038=CARTESIAN_POINT ( 'NONE',  ( 52.86797706100236383, 192.1423013555410080, -4.594050593750043987 ) ) ;
#85039=CARTESIAN_POINT ( 'NONE',  ( 164.1964637989676987, 247.2500284144306022, -6.878198590015258240 ) ) ;
#85042=CARTESIAN_POINT ( 'NONE',  ( -4.163664537435148638, 161.7365022471902023, 10.00000000000009592 ) ) ;
#85044=CARTESIAN_POINT ( 'NONE',  ( 23.01796646339240837, 172.5494855054051868, -2.679491924311248496 ) ) ;
#85048=CARTESIAN_POINT ( 'NONE',  ( 197.0121621852902933, 287.4119207165142029, 17.64812647472269092 ) ) ;
#85051=CARTESIAN_POINT ( 'NONE',  ( 57.82012596918833935, 210.3149278399160949, 9.188101187500093303 ) ) ;
#85053=FACE_OUTER_BOUND ( 'NONE', #60023, .T. ) ;
#85054=CARTESIAN_POINT ( 'NONE',  ( 159.4285914931787431, 254.5085746851079023, 15.41072477910873673 ) ) ;
#85056=CARTESIAN_POINT ( 'NONE',  ( 149.2964064632859049, 275.3583832525684443, 7.516923408081652269 ) ) ;
#85057=EDGE_CURVE ( 'NONE', #68820, #44309, #47050, .T. ) ;
#85060=CARTESIAN_POINT ( 'NONE',  ( 116.0695290213044757, 224.4865022471901455, 1.119607411625061291E-15 ) ) ;
#85062=CARTESIAN_POINT ( 'NONE',  ( 164.8329445879545290, 245.1479605429143760, -2.955380775890217304 ) ) ;
#85065=FACE_OUTER_BOUND ( 'NONE', #28014, .T. ) ;
#85066=ORIENTED_EDGE ( 'NONE', *, *, #49498, .T. ) ;
#85067=CARTESIAN_POINT ( 'NONE',  ( 159.5050723400634638, 254.3761059724978679, -15.34938048045353298 ) ) ;
#85068=CARTESIAN_POINT ( 'NONE',  ( 187.1296147083845085, 276.7229790764539530, -17.49940255933115196 ) ) ;
#85072=CARTESIAN_POINT ( 'NONE',  ( 173.3065076608714605, 251.6304707193385752, 8.836706110889046588E-05 ) ) ;
#85073=ORIENTED_EDGE ( 'NONE', *, *, #52812, .T. ) ;
#85075=CARTESIAN_POINT ( 'NONE',  ( 194.3442947553755005, 294.0328026529847421, -15.97648891113594871 ) ) ;
#85077=EDGE_LOOP ( 'NONE', ( #60304, #37470, #32726, #21646, #77339, #23798, #6559, #7375, #27148, #21137, #4105, #48637, #95223, #4889, #46655, #88612, #71924, #35223, #37233, #98255, #52067 ) ) ;
#85080=CARTESIAN_POINT ( 'NONE',  ( 38.49039832772786696, 181.4824982072973683, 3.021315404115420679E-15 ) ) ;
#85083=ORIENTED_EDGE ( 'NONE', *, *, #49408, .T. ) ;
#85085=EDGE_CURVE ( 'NONE', #58437, #91328, #3407, .T. ) ;
#85087=CARTESIAN_POINT ( 'NONE',  ( 197.0121621852902933, 287.4119207165142029, 17.64812647472269092 ) ) ;
#85094=CARTESIAN_POINT ( 'NONE',  ( 204.3574891606595827, 276.6894411969685166, 13.41627538812899978 ) ) ;
#85095=CARTESIAN_POINT ( 'NONE',  ( 187.5420919156053401, 294.0784138002250643, -10.86800630351413588 ) ) ;
#85096=CARTESIAN_POINT ( 'NONE',  ( 157.8719920515997046, 257.2046840049564480, -17.69857783492101433 ) ) ;
#85097=CARTESIAN_POINT ( 'NONE',  ( 141.2833242589136375, 258.5024278399160380, 9.188101187500095079 ) ) ;
#85098=CARTESIAN_POINT ( 'NONE',  ( 177.1123716022877943, 269.3477771532123484, 16.09281802875675993 ) ) ;
#85099=CARTESIAN_POINT ( 'NONE',  ( 195.7956752809994327, 291.0480278656929158, -15.87661460891315279 ) ) ;
#85100=CARTESIAN_POINT ( 'NONE',  ( 77.41429782557628414, 209.3768266524159571, -9.188101187500091527 ) ) ;
#85102=CARTESIAN_POINT ( 'NONE',  ( 151.4159295687746294, 268.3869122420484814, 14.78076517566594106 ) ) ;
#85103=DIRECTION ( 'NONE',  ( -0.8660254037844387076, -0.4999999999999998890, -0.000000000000000000 ) ) ;
#85105=CARTESIAN_POINT ( 'NONE',  ( 195.9058436374999701, 291.3281206506429726, -17.17388571147666809 ) ) ;
#85110=CARTESIAN_POINT ( 'NONE',  ( 196.5475680726518988, 286.0355519910975772, 16.91030377461561685 ) ) ;
#85111=CARTESIAN_POINT ( 'NONE',  ( 191.8000917695741805, 298.4394914891611847, -9.452573400474340914 ) ) ;
#85115=CARTESIAN_POINT ( 'NONE',  ( 79.47110815956433783, 210.5643266524160424, 9.188101187500095079 ) ) ;
#85118=VERTEX_POINT ( 'NONE', #80238 ) ;
#85119=CARTESIAN_POINT ( 'NONE',  ( 200.7808116640040055, 282.8844283434642648, -16.74230052443130390 ) ) ;
#85122=EDGE_CURVE ( 'NONE', #30031, #36428, #81303, .T. ) ;
#85124=CARTESIAN_POINT ( 'NONE',  ( 183.9930990868905099, 275.1979307975402094, 16.37542179091846606 ) ) ;
#85125=CARTESIAN_POINT ( 'NONE',  ( 205.9642072045669465, 273.9065239114831911, 10.22128930895731536 ) ) ;
#85129=CARTESIAN_POINT ( 'NONE',  ( 207.2804460909495674, 270.7025114183682035, -2.311883053335581195 ) ) ;
#85130=CARTESIAN_POINT ( 'NONE',  ( 159.8059924763540494, 259.8542309688582463, 16.66854085587838696 ) ) ;
#85131=ORIENTED_EDGE ( 'NONE', *, *, #81003, .F. ) ;
#85132=CARTESIAN_POINT ( 'NONE',  ( 192.4020620555409380, 296.6120898282274538, 11.26082810598535922 ) ) ;
#85133=EDGE_CURVE ( 'NONE', #95124, #17862, #33777, .T. ) ;
#85134=CARTESIAN_POINT ( 'NONE',  ( 185.2191931831976603, 260.2532633546392162, 6.303467285011207011 ) ) ;
#85135=ADVANCED_FACE ( 'NONE', ( #26503 ), #58856, .T. ) ;
#85136=CARTESIAN_POINT ( 'NONE',  ( 147.7724539486783044, 275.5393038904080640, -3.815232554072548687 ) ) ;
#85137=CARTESIAN_POINT ( 'NONE',  ( 152.7729059155601021, 266.0365602647466972, -17.50667083025758686 ) ) ;
#85144=CARTESIAN_POINT ( 'NONE',  ( 148.3187134315808748, 276.1718878684489482, -3.836830238838571550 ) ) ;
#85146=CARTESIAN_POINT ( 'NONE',  ( 168.0624319142297054, 250.1787547974163033, 6.948285211281213236 ) ) ;
#85148=CARTESIAN_POINT ( 'NONE',  ( 152.9231525498888118, 270.9783143214066854, 14.00607015262799671 ) ) ;
#85150=CARTESIAN_POINT ( 'NONE',  ( 163.0683798854284703, 248.2042762609320903, 11.26611642476872710 ) ) ;
#85153=CARTESIAN_POINT ( 'NONE',  ( 155.4812142336614329, 261.3456326552338282, 18.45193178807985745 ) ) ;
#85155=CARTESIAN_POINT ( 'NONE',  ( 176.1346035850542933, 285.3745144875404662, -12.06757559795553192 ) ) ;
#85157=CARTESIAN_POINT ( 'NONE',  ( 170.3771428974362436, 273.8123333415551315, 16.01817606700219088 ) ) ;
#85158=CARTESIAN_POINT ( 'NONE',  ( 166.5066175986279120, 286.1322789562391335, -3.204271455219934062 ) ) ;
#85162=CARTESIAN_POINT ( 'NONE',  ( 192.2608584806236252, 262.0927522878173477, 3.022526856766069692 ) ) ;
#85163=CARTESIAN_POINT ( 'NONE',  ( -7.835251407336910390, 166.2833772461660828, -9.188101187500095079 ) ) ;
#85166=CARTESIAN_POINT ( 'NONE',  ( 177.0173213845591249, 256.3747443458416910, 8.281083027831190435 ) ) ;
#85169=CARTESIAN_POINT ( 'NONE',  ( 202.5511068033279685, 273.9590694375769999, -13.16333768474205357 ) ) ;
#85170=CARTESIAN_POINT ( 'NONE',  ( 99.93749413994396491, 240.0530062829862743, -4.648177544792955347E-16 ) ) ;
#85171=CARTESIAN_POINT ( 'NONE',  ( 30.64892602121659593, 182.3768266524160140, -9.188101187500093303 ) ) ;
#85173=CARTESIAN_POINT ( 'NONE',  ( 181.9416707481567812, 275.7034555988952889, -16.43191976972476809 ) ) ;
#85176=CARTESIAN_POINT ( 'NONE',  ( 170.0877722087189170, 270.7013820935941339, -17.07221500441185214 ) ) ;
#85179=CARTESIAN_POINT ( 'NONE',  ( 168.2820353728258738, 287.7095463320123940, -5.019694092131335772 ) ) ;
#85180=CARTESIAN_POINT ( 'NONE',  ( 79.69646206235805153, 203.4865022471901455, 1.119607411625061291E-15 ) ) ;
#85182=FACE_OUTER_BOUND ( 'NONE', #91457, .T. ) ;
#85183=CARTESIAN_POINT ( 'NONE',  ( 32.86828966629671811, 177.5327760586659736, 1.948934522072303157E-15 ) ) ;
#85186=CARTESIAN_POINT ( 'NONE',  ( 151.2567985338353935, 268.6625352796243646, -15.71756535662528798 ) ) ;
#85189=CARTESIAN_POINT ( 'NONE',  ( -2.575951297163730835, 175.9865022471903160, 10.00000000000009415 ) ) ;
#85190=CARTESIAN_POINT ( 'NONE',  ( 159.8838727533587587, 278.4444054329620712, -9.946836423640300850 ) ) ;
#85194=CARTESIAN_POINT ( 'NONE',  ( 147.9710862514405960, 274.3535558917855042, 7.785500222159708272 ) ) ;
#85197=CARTESIAN_POINT ( 'NONE',  ( 188.9038075421769918, 270.0326964921503645, -14.10267558245943320 ) ) ;
#85198=ORIENTED_EDGE ( 'NONE', *, *, #69952, .T. ) ;
#85203=EDGE_CURVE ( 'NONE', #42320, #89828, #17774, .T. ) ;
#85205=CARTESIAN_POINT ( 'NONE',  ( 16.68302997285341149, 191.9860189848785410, -2.679491924311252493 ) ) ;
#85207=VECTOR ( 'NONE', #44334, 1000.000000000000227 ) ;
#85211=ORIENTED_EDGE ( 'NONE', *, *, #26966, .T. ) ;
#85213=CARTESIAN_POINT ( 'NONE',  ( 202.4421998307519743, 279.5209983176915216, 15.52974020151914480 ) ) ;
#85216=CARTESIAN_POINT ( 'NONE',  ( 153.4361244163197000, 264.8878321249116539, -17.23169627811277493 ) ) ;
#85220=ORIENTED_EDGE ( 'NONE', *, *, #31776, .F. ) ;
#85221=CARTESIAN_POINT ( 'NONE',  ( 190.6071113721798156, 300.5057941498820924, -0.4754021072632813594 ) ) ;
#85226=CARTESIAN_POINT ( 'NONE',  ( 161.3793624665346158, 266.8670659500822921, 16.51829894754524730 ) ) ;
#85229=CARTESIAN_POINT ( 'NONE',  ( 190.7516742497373059, 300.2554039010641418, 4.342609251298632067 ) ) ;
#85233=CARTESIAN_POINT ( 'NONE',  ( 159.5111797645456306, 254.9608776620166850, 15.67735860260454928 ) ) ;
#85237=VERTEX_POINT ( 'NONE', #50776 ) ;
#85240=DIRECTION ( 'NONE',  ( 0.4999999999999998890, -0.8660254037844385966, 0.000000000000000000 ) ) ;
#85242=CARTESIAN_POINT ( 'NONE',  ( 190.3144310910409445, 301.0127312671879167, -1.334877248546042949 ) ) ;
#85243=ORIENTED_EDGE ( 'NONE', *, *, #99719, .F. ) ;
#85245=CARTESIAN_POINT ( 'NONE',  ( 170.9861191376329259, 275.4057932803170274, -16.08545443273202125 ) ) ;
#85246=CARTESIAN_POINT ( 'NONE',  ( 207.8844858873204657, 270.5805036682629066, -6.251308616122969397 ) ) ;
#85247=CARTESIAN_POINT ( 'NONE',  ( 192.7705129102570822, 296.7586727687594816, -13.39629674907774692 ) ) ;
#85255=CARTESIAN_POINT ( 'NONE',  ( 114.7887934315897382, 227.8923013555410080, 4.594050593750050204 ) ) ;
#85257=CARTESIAN_POINT ( 'NONE',  ( 146.9456733906991417, 276.1296230653242105, -0.7988785540157754550 ) ) ;
#85262=CARTESIAN_POINT ( 'NONE',  ( 191.3471005483181102, 298.1160726331887645, -9.452014560043723534 ) ) ;
#85264=CARTESIAN_POINT ( 'NONE',  ( 165.9607527239562614, 283.6245786231995112, -8.165966701861027133 ) ) ;
#85265=ORIENTED_EDGE ( 'NONE', *, *, #10768, .F. ) ;
#85268=CARTESIAN_POINT ( 'NONE',  ( 47.92415505746842541, 205.1427522451419065, 10.00000000000009237 ) ) ;
#85269=CARTESIAN_POINT ( 'NONE',  ( 120.7963240266967375, 249.7369531367911293, -4.594050593750048428 ) ) ;
#85270=CARTESIAN_POINT ( 'NONE',  ( 189.8390163498603158, 294.5874093566309284, -12.44163422039437528 ) ) ;
#85272=CARTESIAN_POINT ( 'NONE',  ( 196.0727848089514964, 291.0389700598140621, 17.56388901715066808 ) ) ;
#85274=CARTESIAN_POINT ( 'NONE',  ( 51.59574192737019160, 200.5958772461660544, -9.188101187500095079 ) ) ;
#85277=CARTESIAN_POINT ( 'NONE',  ( 188.0333306978322128, 299.5241197090491028, 3.603443727378835781 ) ) ;
#85278=ORIENTED_EDGE ( 'NONE', *, *, #50979, .F. ) ;
#85281=B_SPLINE_SURFACE_WITH_KNOTS ( 'NONE', 3, 1, ( 
 ( #18203, #49097 ),
 ( #27298, #57175 ),
 ( #97224, #88155 ),
 ( #96230, #10099 ),
 ( #56171, #58181 ),
 ( #25812, #18703 ),
 ( #41987, #19220 ),
 ( #72422, #56686 ),
 ( #66292, #35380 ),
 ( #80032, #41473 ),
 ( #11610, #3025 ),
 ( #17700, #64802 ),
 ( #88655, #11117 ),
 ( #50577, #49584 ),
 ( #3514, #81527 ),
 ( #4487, #42469 ),
 ( #40963, #72923 ),
 ( #42957, #2509 ),
 ( #34391, #65290 ),
 ( #50091, #81047 ),
 ( #73403, #48602 ),
 ( #3989, #34875 ),
 ( #65776, #96733 ),
 ( #89165, #19711 ),
 ( #79541, #73898 ),
 ( #58666, #74903 ),
 ( #36370, #6488 ),
 ( #28275, #98708 ),
 ( #51070, #66782 ),
 ( #28784, #43965 ),
 ( #29779, #52565 ),
 ( #14587, #83022 ),
 ( #67783, #37366 ),
 ( #60652, #21199 ) ),
 .UNSPECIFIED., .T., .F., .F.,
 ( 4, 2, 2, 2, 2, 2, 2, 2, 2, 2, 2, 2, 2, 2, 2, 2, 4 ),
 ( 2, 2 ),
 ( 0.000000000000000000, 0.06250000000000000000, 0.1250000000000000000, 0.1875000000000000000, 0.2500000000000000000, 0.3125000000000000000, 0.3750000000000000000, 0.4375000000000000000, 0.5000000000000000000, 0.5625000000000000000, 0.6250000000000000000, 0.6875000000000000000, 0.7500000000000000000, 0.8125000000000000000, 0.8750000000000000000, 0.9375000000000000000, 1.000000000000000000 ),
 ( 0.000000000000000000, 1.000000000000000000 ),
 .UNSPECIFIED. ) ;
#85282=CARTESIAN_POINT ( 'NONE',  ( 24.41517378745132660, 178.2365022471902307, 10.00000000000009948 ) ) ;
#85284=CARTESIAN_POINT ( 'NONE',  ( 177.6444986370304946, 293.6980009803469329, 2.770296639708824227 ) ) ;
#85286=CARTESIAN_POINT ( 'NONE',  ( 179.1341793956848676, 261.5303873598331847, 12.21931224842648511 ) ) ;
#85287=CARTESIAN_POINT ( 'NONE',  ( 96.56591523669439425, 239.8927522451419350, 2.944929066748280225E-16 ) ) ;
#85290=ORIENTED_EDGE ( 'NONE', *, *, #91287, .F. ) ;
#85292=CARTESIAN_POINT ( 'NONE',  ( 189.8136646974935786, 301.8800841035353528, -0.6430783927310335102 ) ) ;
#85294=AXIS2_PLACEMENT_3D ( 'NONE', #41238, #24548, #40738 ) ;
#85295=CARTESIAN_POINT ( 'NONE',  ( 22.39418752168989712, 192.9244531367911293, -4.594050593750046652 ) ) ;
#85301=CARTESIAN_POINT ( 'NONE',  ( 196.9509217096318423, 276.5932595302290906, -15.33546036893861420 ) ) ;
#85302=CARTESIAN_POINT ( 'NONE',  ( 69.59257202794182717, 220.1744531367911293, 4.594050593750047540 ) ) ;
#85303=CARTESIAN_POINT ( 'NONE',  ( 200.1444820856229967, 283.9865835035790269, 17.93386694781497326 ) ) ;
#85305=CARTESIAN_POINT ( 'NONE',  ( 56.56090640341663800, 191.9155109091896350, 2.679491924311254714 ) ) ;
#85308=CARTESIAN_POINT ( 'NONE',  ( 165.2390926464214260, 269.1549683505341477, 16.83750853429537031 ) ) ;
#85309=CARTESIAN_POINT ( 'NONE',  ( 25.20903040758703284, 185.3615022471902591, -10.00000000000009592 ) ) ;
#85310=CARTESIAN_POINT ( 'NONE',  ( 164.2090401137261892, 246.2285947913476889, -5.787448100099915393 ) ) ;
#85311=CARTESIAN_POINT ( 'NONE',  ( 148.0493212738620628, 256.2833772461660828, -9.188101187500095079 ) ) ;
#85313=CARTESIAN_POINT ( 'NONE',  ( 164.0862216042829402, 260.4305047126978252, -16.14355404909294123 ) ) ;
#85314=CARTESIAN_POINT ( 'NONE',  ( 189.2475850683314889, 261.5409228790725251, 6.709830765752542447 ) ) ;
#85315=CARTESIAN_POINT ( 'NONE',  ( 164.2813349609167517, 246.1033764428878214, 1.949810150281061638 ) ) ;
#85320=CARTESIAN_POINT ( 'NONE',  ( 191.1489696025915919, 299.5672681643093256, 8.892130899335590755 ) ) ;
#85321=DIRECTION ( 'NONE',  ( -0.8660254037844387076, -0.4999999999999998890, -0.000000000000000000 ) ) ;
#85322=CARTESIAN_POINT ( 'NONE',  ( 177.8663784656789062, 286.4429601165666099, 13.25884385786000230 ) ) ;
#85323=CARTESIAN_POINT ( 'NONE',  ( 196.1245817477023650, 288.9492551302209336, 17.30641872853625074 ) ) ;
#85325=ORIENTED_EDGE ( 'NONE', *, *, #48498, .T. ) ;
#85326=CARTESIAN_POINT ( 'NONE',  ( -22.42236680055709641, 157.8615022471902591, 0.000000000000000000 ) ) ;
#85331=FACE_OUTER_BOUND ( 'NONE', #77786, .T. ) ;
#85334=CARTESIAN_POINT ( 'NONE',  ( 201.0468719883840265, 282.4235983437597497, -16.59631526626950659 ) ) ;
#85337=CARTESIAN_POINT ( 'NONE',  ( 190.5217943342473745, 281.4870030958396683, 17.81127109971334121 ) ) ;
#85338=CARTESIAN_POINT ( 'NONE',  ( 164.0651280066704771, 248.4778578725967861, 9.975266483072225299 ) ) ;
#85340=CARTESIAN_POINT ( 'NONE',  ( -17.42236680055705023, 149.2012482093457777, 0.000000000000000000 ) ) ;
#85346=CIRCLE ( 'NONE', #9304, 17.82106496071138224 ) ;
#85349=CARTESIAN_POINT ( 'NONE',  ( 155.4218027583364687, 261.4485363490496184, 18.59640492044406557 ) ) ;
#85351=CARTESIAN_POINT ( 'NONE',  ( 191.5694344253287511, 298.8390017285333897, 8.250976118904059575 ) ) ;
#85354=EDGE_LOOP ( 'NONE', ( #74130, #93437, #31474, #1089 ) ) ;
#85361=CARTESIAN_POINT ( 'NONE',  ( 208.2555382576270233, 269.9378221106229034, 3.215405476967123199 ) ) ;
#85363=ADVANCED_FACE ( 'NONE', ( #52757 ), #61853, .T. ) ;
#85365=CARTESIAN_POINT ( 'NONE',  ( 165.7697680452210989, 271.5089577923188813, 17.25749984557730343 ) ) ;
#85366=B_SPLINE_CURVE_WITH_KNOTS ( 'NONE', 3,
 ( #33832, #65208, #48521, #25203, #80965, #1424, #40884, #24703, #55585, #56087, #10022, #87591 ),
 .UNSPECIFIED., .F., .F.,
 ( 4, 2, 2, 2, 2, 4 ),
 ( 7.835778008535133478E-15, 0.0004471628226844677760, 0.0008943256453610996977, 0.001341488468037731674, 0.001565069879376075092, 0.001788651290714418510 ),
 .UNSPECIFIED. ) ;
#85368=CARTESIAN_POINT ( 'NONE',  ( 194.1852025340051284, 294.3083584634874796, -15.46421316575964688 ) ) ;
#85370=CARTESIAN_POINT ( 'NONE',  ( 197.6411165541630339, 288.3225397939841628, -17.98373575462852614 ) ) ;
#85371=B_SPLINE_CURVE_WITH_KNOTS ( 'NONE', 3,
 ( #3391, #18076, #50454, #96108 ),
 .UNSPECIFIED., .F., .F.,
 ( 4, 4 ),
 ( 0.04580664796786450277, 0.04887120950165272509 ),
 .UNSPECIFIED. ) ;
#85372=CARTESIAN_POINT ( 'NONE',  ( 165.3992151465029110, 246.6496888978224433, 1.887000115222200458 ) ) ;
#85373=B_SPLINE_CURVE_WITH_KNOTS ( 'NONE', 3,
 ( #2839, #26119, #39776, #9414 ),
 .UNSPECIFIED., .F., .F.,
 ( 4, 4 ),
 ( 0.006146573736721493500, 0.01114496846602976675 ),
 .UNSPECIFIED. ) ;
#85375=CARTESIAN_POINT ( 'NONE',  ( 198.8358800211527750, 276.4754353779146641, -15.71425324584650340 ) ) ;
#85380=CARTESIAN_POINT ( 'NONE',  ( 55.71838369152838766, 209.6427522451419350, 10.00000000000009415 ) ) ;
#85381=CARTESIAN_POINT ( 'NONE',  ( 159.9531724557437826, 253.5999738052623229, -15.71074128491364874 ) ) ;
#85382=FACE_OUTER_BOUND ( 'NONE', #45645, .T. ) ;
#85384=FACE_OUTER_BOUND ( 'NONE', #25138, .T. ) ;
#85385=CARTESIAN_POINT ( 'NONE',  ( 161.3206464153366824, 283.6027336028535615, 2.150076420610042671 ) ) ;
#85387=CARTESIAN_POINT ( 'NONE',  ( 155.3185753361098591, 261.6273314890805750, -17.01637887179724373 ) ) ;
#85389=CARTESIAN_POINT ( 'NONE',  ( 126.8046355855010603, 254.0177522451418781, 5.000000000000046185 ) ) ;
#85391=CARTESIAN_POINT ( 'NONE',  ( 1.663964738649697406, 171.7677522451418781, 10.00000000000009592 ) ) ;
#85392=CARTESIAN_POINT ( 'NONE',  ( 90.40467888234286420, 216.8768266524159571, -9.188101187500093303 ) ) ;
#85393=CARTESIAN_POINT ( 'NONE',  ( 193.6044853607075140, 267.0230459576156932, -11.54443625195158063 ) ) ;
#85395=CARTESIAN_POINT ( 'NONE',  ( 170.3121876137535651, 280.6933715238725426, -13.94289214494337159 ) ) ;
#85396=ADVANCED_FACE ( 'NONE', ( #37556 ), #54240, .T. ) ;
#85397=CARTESIAN_POINT ( 'NONE',  ( 8.321535033790526725, 165.6115022471902023, -5.000000000000041744 ) ) ;
#85398=CARTESIAN_POINT ( 'NONE',  ( 1.717831006336420607, 180.9869531367911293, 4.594050593750046652 ) ) ;
#85400=CARTESIAN_POINT ( 'NONE',  ( 200.9111546617170916, 282.6586676490145464, 17.66063511622358106 ) ) ;
#85402=VERTEX_POINT ( 'NONE', #7672 ) ;
#85404=CARTESIAN_POINT ( 'NONE',  ( 197.5495010542000216, 265.0987281629911081, -2.962445677173857206 ) ) ;
#85405=CARTESIAN_POINT ( 'NONE',  ( 148.1316126177475496, 276.0755160693871630, 5.020219949272568094 ) ) ;
#85407=CARTESIAN_POINT ( 'NONE',  ( 185.8122761056181105, 286.6146716806434256, 15.85193406119726056 ) ) ;
#85409=CARTESIAN_POINT ( 'NONE',  ( 37.90188877791127453, 186.5643266524160424, 9.188101187500095079 ) ) ;
#85410=CARTESIAN_POINT ( 'NONE',  ( 121.9060058492368483, 247.3149278399160949, -9.188101187500095079 ) ) ;
#85412=CARTESIAN_POINT ( 'NONE',  ( 199.4572827948314284, 277.5277167264244440, 15.18863414768032349 ) ) ;
#85414=CARTESIAN_POINT ( 'NONE',  ( 152.0058074760499665, 272.8430352715865865, -11.69865300651101592 ) ) ;
#85419=AXIS2_PLACEMENT_3D ( 'NONE', #53992, #46397, #38301 ) ;
#85420=CARTESIAN_POINT ( 'NONE',  ( 155.0929244053699847, 262.0181703658971628, 18.51426604808664678 ) ) ;
#85421=CARTESIAN_POINT ( 'NONE',  ( 58.11799575139567509, 214.3615022471903160, 5.000000000000046185 ) ) ;
#85422=CARTESIAN_POINT ( 'NONE',  ( 189.5680078729632214, 284.4452857818997131, 16.60658711706803103 ) ) ;
#85423=FACE_OUTER_BOUND ( 'NONE', #31373, .T. ) ;
#85425=CARTESIAN_POINT ( 'NONE',  ( 171.2717486985798701, 279.7763900546701166, 13.89510435958859524 ) ) ;
#85428=CARTESIAN_POINT ( 'NONE',  ( 189.8136646974935786, 301.8800841035353528, -0.6430783927310335102 ) ) ;
#85430=ORIENTED_EDGE ( 'NONE', *, *, #68774, .T. ) ;
#85431=CARTESIAN_POINT ( 'NONE',  ( 183.8836432619000050, 293.1766604090298074, 10.99787141183991501 ) ) ;
#85433=( BOUNDED_CURVE ( )  B_SPLINE_CURVE ( 2, ( #39245, #55942, #85421, #765, #85941, #70667, #16467, #47363, #78286 ),
 .UNSPECIFIED., .F., .T. ) 
 B_SPLINE_CURVE_WITH_KNOTS ( ( 3, 2, 2, 2, 3 ),
 ( 0.4717741935483871218, 0.4731182795698924970, 0.4758064516129032473, 0.4784946236559139976, 0.4798387096774193727 ),
 .UNSPECIFIED. ) 
 CURVE ( )  GEOMETRIC_REPRESENTATION_ITEM ( )  RATIONAL_B_SPLINE_CURVE ( ( 0.9330127018922194093, 0.9330127018922194093, 1.000000000000000000, 0.8660254037844387076, 1.000000000000000000, 0.8660254037844387076, 1.000000000000000000, 0.9330127018922194093, 0.9330127018922194093 ) ) 
 REPRESENTATION_ITEM ( '' )  );
#85435=CARTESIAN_POINT ( 'NONE',  ( 119.3082767336485404, 233.5643266524159856, -9.188101187500093303 ) ) ;
#85437=CARTESIAN_POINT ( 'NONE',  ( 151.2648146047323507, 268.6486510375538614, 15.71323890031163550 ) ) ;
#85441=CARTESIAN_POINT ( 'NONE',  ( 192.5936405006954431, 277.6276709648686847, 16.42609391667364704 ) ) ;
#85442=CARTESIAN_POINT ( 'NONE',  ( 204.6717125599631686, 272.9637062319359870, -9.753211108311461430 ) ) ;
#85443=CARTESIAN_POINT ( 'NONE',  ( 151.1126408083691501, 268.9122237844355254, -15.82705194100464396 ) ) ;
#85444=DIRECTION ( 'NONE',  ( 0.4999999999999998890, -0.8660254037844385966, 0.000000000000000000 ) ) ;
#85448=VERTEX_POINT ( 'NONE', #83719 ) ;
#85449=DIRECTION ( 'NONE',  ( -0.8660254037844387076, -0.4999999999999998890, -0.000000000000000000 ) ) ;
#85452=CARTESIAN_POINT ( 'NONE',  ( 199.2928477948540547, 269.7932124880637161, 9.247559850577539819 ) ) ;
#85453=CARTESIAN_POINT ( 'NONE',  ( 149.4965729687386045, 271.7113353911534546, -11.48413836595348059 ) ) ;
#85455=EDGE_CURVE ( 'NONE', #10482, #30385, #52931, .T. ) ;
#85459=CARTESIAN_POINT ( 'NONE',  ( 189.3832291599495079, 300.6256203239445313, 1.753828516883770838 ) ) ;
#85460=DIRECTION ( 'NONE',  ( -0.8660254037844387076, -0.4999999999999998890, -0.000000000000000000 ) ) ;
#85463=CARTESIAN_POINT ( 'NONE',  ( 190.1875296108910334, 280.4995553090359408, 16.63324803487314796 ) ) ;
#85466=VERTEX_POINT ( 'NONE', #6680 ) ;
#85467=CARTESIAN_POINT ( 'NONE',  ( 167.6493030671569500, 249.8575448609487921, 6.851470149181726477 ) ) ;
#85468=EDGE_CURVE ( 'NONE', #36195, #92664, #98888, .T. ) ;
#85469=DIRECTION ( 'NONE',  ( 0.4999999999999992784, -0.8660254037844390407, 0.000000000000000000 ) ) ;
#85472=CARTESIAN_POINT ( 'NONE',  ( 147.8527080755910958, 276.5585929068648170, -2.411454450074328903 ) ) ;
#85473=FACE_OUTER_BOUND ( 'NONE', #15904, .T. ) ;
#85479=CARTESIAN_POINT ( 'NONE',  ( 201.3363518313238956, 277.3271591401824026, -15.70882811787338618 ) ) ;
#85480=ORIENTED_EDGE ( 'NONE', *, *, #4454, .F. ) ;
#85482=ORIENTED_EDGE ( 'NONE', *, *, #47166, .F. ) ;
#85483=CARTESIAN_POINT ( 'NONE',  ( 169.7343602353587926, 269.2857159740701150, 16.89834073576611573 ) ) ;
#85484=ORIENTED_EDGE ( 'NONE', *, *, #13656, .F. ) ;
#85485=CARTESIAN_POINT ( 'NONE',  ( 165.4473470637335879, 246.0837842385732301, 3.196113342258863899 ) ) ;
#85487=FACE_OUTER_BOUND ( 'NONE', #80616, .T. ) ;
#85491=CARTESIAN_POINT ( 'NONE',  ( 168.0790033696603416, 248.3996430977109355, -4.949810391468747461 ) ) ;
#85493=CARTESIAN_POINT ( 'NONE',  ( 178.0988699194678588, 255.3435402841193707, 5.564670213749401739 ) ) ;
#85494=CARTESIAN_POINT ( 'NONE',  ( 123.3136442261515526, 235.8768266524159856, 9.188101187500098632 ) ) ;
#85496=CARTESIAN_POINT ( 'NONE',  ( 160.7670569121125084, 283.7960714782474270, 2.206094026959618315 ) ) ;
#85497=CARTESIAN_POINT ( 'NONE',  ( 177.9903043249979930, 289.2672226302933041, -9.336760805543203645 ) ) ;
#85499=EDGE_LOOP ( 'NONE', ( #74969, #28782, #94698, #2177 ) ) ;
#85500=CONICAL_SURFACE ( 'NONE', #6189, 16.82106496071143908, 0.7853981633974241872 ) ;
#85502=CARTESIAN_POINT ( 'NONE',  ( 200.2184649266326915, 273.7011556189854105, 13.93284857238957741 ) ) ;
#85504=CARTESIAN_POINT ( 'NONE',  ( 177.7357342257776907, 253.3636629150184945, 1.391642827436562424 ) ) ;
#85505=CARTESIAN_POINT ( 'NONE',  ( 171.0816347564833961, 287.7379295750013739, -5.004374939593263960 ) ) ;
#85506=CARTESIAN_POINT ( 'NONE',  ( 196.1573359623355088, 290.8925231663144473, 17.55680092534192482 ) ) ;
#85508=CARTESIAN_POINT ( 'NONE',  ( 201.1679199471075492, 282.2139371290980989, -16.62385308864941535 ) ) ;
#85509=CARTESIAN_POINT ( 'NONE',  ( 173.4619051054469878, 287.5670256320814246, -9.876641005795255168 ) ) ;
#85510=VERTEX_POINT ( 'NONE', #24865 ) ;
#85511=CARTESIAN_POINT ( 'NONE',  ( 194.8191165606777702, 293.2103871616598099, 16.46019522012304037 ) ) ;
#85512=CARTESIAN_POINT ( 'NONE',  ( 176.1919805722776005, 255.3928090292563695, -7.299666310701137917 ) ) ;
#85514=ORIENTED_EDGE ( 'NONE', *, *, #41856, .T. ) ;
#85515=CARTESIAN_POINT ( 'NONE',  ( 194.7900911235093133, 293.2606606935473792, -14.66228443412922999 ) ) ;
#85518=CARTESIAN_POINT ( 'NONE',  ( 188.5361412926528430, 265.1671748825110626, -11.87835921727136146 ) ) ;
#85520=CARTESIAN_POINT ( 'NONE',  ( 190.7968079096152110, 283.1981913049548325, -16.56890853126571983 ) ) ;
#85521=CARTESIAN_POINT ( 'NONE',  ( 192.7845724167702031, 262.6087076098646094, 4.680582376611854833 ) ) ;
#85522=CARTESIAN_POINT ( 'NONE',  ( 190.4249800432324662, 300.8212548652687133, 3.085047376053959400 ) ) ;
#85525=CARTESIAN_POINT ( 'NONE',  ( 162.1138636377163493, 281.8676824225443625, -6.599314908080229358 ) ) ;
#85526=CARTESIAN_POINT ( 'NONE',  ( 154.8543500088721885, 277.6552608316904980, -8.992244201135354942 ) ) ;
#85527=CARTESIAN_POINT ( 'NONE',  ( 200.6985908945154335, 283.0268388936558495, -17.74173253065502820 ) ) ;
#85529=CARTESIAN_POINT ( 'NONE',  ( 190.1693911629507738, 301.2639477917662703, -5.112716700269980485 ) ) ;
#85530=B_SPLINE_SURFACE_WITH_KNOTS ( 'NONE', 3, 1, ( 
 ( #2701, #72611 ),
 ( #51257, #4168 ),
 ( #95932, #26492 ),
 ( #18901, #96419 ),
 ( #4681, #26986 ),
 ( #88848, #19413 ),
 ( #50270, #81223 ),
 ( #58362, #11799 ),
 ( #74602, #13763 ),
 ( #83199, #84210 ),
 ( #68450, #92304 ),
 ( #97887, #61345 ),
 ( #53255, #22853 ),
 ( #75085, #99378 ),
 ( #82721, #45638 ),
 ( #53737, #37544 ),
 ( #84696, #90319 ),
 ( #59340, #68945 ),
 ( #5665, #91794 ),
 ( #37058, #91296 ),
 ( #29957, #7147 ),
 ( #76566, #13290 ),
 ( #15236, #28979 ),
 ( #76093, #44150 ),
 ( #36554, #60834 ),
 ( #60338, #14756 ),
 ( #59855, #38034 ),
 ( #99870, #98883 ),
 ( #22358, #44642 ),
 ( #51781, #30456 ),
 ( #5176, #36056 ),
 ( #67460, #52258 ),
 ( #98388, #66958 ),
 ( #14263, #6667 ) ),
 .UNSPECIFIED., .T., .F., .F.,
 ( 4, 2, 2, 2, 2, 2, 2, 2, 2, 2, 2, 2, 2, 2, 2, 2, 4 ),
 ( 2, 2 ),
 ( 0.000000000000000000, 0.06250000000000000000, 0.1250000000000000000, 0.1875000000000000000, 0.2500000000000000000, 0.3125000000000000000, 0.3750000000000000000, 0.4375000000000000000, 0.5000000000000000000, 0.5625000000000000000, 0.6250000000000000000, 0.6875000000000000000, 0.7500000000000000000, 0.8125000000000000000, 0.8750000000000000000, 0.9375000000000000000, 1.000000000000000000 ),
 ( 0.000000000000000000, 1.000000000000000000 ),
 .UNSPECIFIED. ) ;
#85532=CARTESIAN_POINT ( 'NONE',  ( 187.3763199732122189, 261.5962347827016288, -9.077379491631687003 ) ) ;
#85533=CARTESIAN_POINT ( 'NONE',  ( 118.2400530232016251, 250.6199935810940929, 2.679491924311251605 ) ) ;
#85534=FACE_OUTER_BOUND ( 'NONE', #58591, .T. ) ;
#85535=CARTESIAN_POINT ( 'NONE',  ( 188.2004726365935880, 299.2930532709519866, -3.673125411237516680 ) ) ;
#85536=CARTESIAN_POINT ( 'NONE',  ( 204.3518858691784885, 276.1737321026752170, 13.13371718507185015 ) ) ;
#85542=CARTESIAN_POINT ( 'NONE',  ( 97.33288211261837830, 220.8768266524160140, 9.188101187500098632 ) ) ;
#85543=LINE ( 'NONE', #87054, #37883 ) ;
#85544=CARTESIAN_POINT ( 'NONE',  ( 193.1028332910263998, 296.1830769848763225, -12.04975758233223893 ) ) ;
#85546=ADVANCED_FACE ( 'NONE', ( #47159 ), #54751, .T. ) ;
#85547=CARTESIAN_POINT ( 'NONE',  ( 155.0304386007204016, 262.1263989543018056, -17.12961552904782181 ) ) ;
#85551=CARTESIAN_POINT ( 'NONE',  ( 37.69969047124883588, 204.1199935810940644, 2.679491924311303119 ) ) ;
#85555=CARTESIAN_POINT ( 'NONE',  ( -4.831225789733595732, 168.0177522451418781, -10.00000000000009592 ) ) ;
#85556=CARTESIAN_POINT ( 'NONE',  ( 164.3918206888665168, 245.9120095485675392, -4.218277793461358449 ) ) ;
#85557=CARTESIAN_POINT ( 'NONE',  ( 157.1135969804030310, 258.5182628004787944, 17.19660297500358226 ) ) ;
#85559=CARTESIAN_POINT ( 'NONE',  ( 38.93012039702277605, 193.2833772461660544, -9.188101187500095079 ) ) ;
#85560=AXIS2_PLACEMENT_3D ( 'NONE', #49477, #11006, #22566 ) ;
#85561=CARTESIAN_POINT ( 'NONE',  ( 74.00414925029257063, 213.5333772461660544, 9.188101187500095079 ) ) ;
#85562=CARTESIAN_POINT ( 'NONE',  ( 164.4567835344609534, 247.2182797030277754, -7.041210626572695475 ) ) ;
#85564=AXIS2_PLACEMENT_3D ( 'NONE', #61435, #38119, #15834 ) ;
#85566=CARTESIAN_POINT ( 'NONE',  ( 149.2944063396847412, 250.8768266524159856, 9.188101187500098632 ) ) ;
#85568=B_SPLINE_CURVE_WITH_KNOTS ( 'NONE', 3,
 ( #17374, #55356, #79723, #87364 ),
 .UNSPECIFIED., .F., .F.,
 ( 4, 4 ),
 ( 0.01386548592622738850, 0.02021667511850969504 ),
 .UNSPECIFIED. ) ;
#85570=CARTESIAN_POINT ( 'NONE',  ( 196.3099158349245670, 269.5646035672020844, -10.80014497079675451 ) ) ;
#85573=CARTESIAN_POINT ( 'NONE',  ( 149.1429535397850827, 272.3238222086447990, -12.91457852089092384 ) ) ;
#85575=CARTESIAN_POINT ( 'NONE',  ( 65.61435460324828739, 214.8149278399160664, 9.188101187500093303 ) ) ;
#85577=CARTESIAN_POINT ( 'NONE',  ( 203.3041373168503299, 278.5139001086923827, -16.61929732091214973 ) ) ;
#85579=CARTESIAN_POINT ( 'NONE',  ( 159.3169041484411537, 254.7020228407560580, 16.67170756419672628 ) ) ;
#85581=CARTESIAN_POINT ( 'NONE',  ( 201.4223166756717660, 281.7733090699454692, 16.49648508032364091 ) ) ;
#85585=CARTESIAN_POINT ( 'NONE',  ( 107.5536125507574354, 226.2365022471902307, 10.00000000000009592 ) ) ;
#85586=CARTESIAN_POINT ( 'NONE',  ( 183.8714358366006820, 278.0135913153196725, -17.80700656249756619 ) ) ;
#85587=CARTESIAN_POINT ( 'NONE',  ( 164.9971748156432056, 244.8635054444190757, -1.825016704039769788 ) ) ;
#85592=CARTESIAN_POINT ( 'NONE',  ( 159.3237119419271437, 254.6902313965507858, -15.56765445935501191 ) ) ;
#85593=CARTESIAN_POINT ( 'NONE',  ( 190.0854368897034874, 279.3748410864815241, -17.22451792153772132 ) ) ;
#85596=ORIENTED_EDGE ( 'NONE', *, *, #12408, .F. ) ;
#85597=CARTESIAN_POINT ( 'NONE',  ( 173.4062743000620515, 251.7440124803043204, -0.2412133965101034005 ) ) ;
#85598=EDGE_LOOP ( 'NONE', ( #34390, #9708, #28341, #20832 ) ) ;
#85600=CARTESIAN_POINT ( 'NONE',  ( 148.3625667886952044, 273.6754917110858401, -8.960758510948144462 ) ) ;
#85608=CARTESIAN_POINT ( 'NONE',  ( 138.7305270869972560, 244.2365022471902307, 10.00000000000009948 ) ) ;
#85609=CARTESIAN_POINT ( 'NONE',  ( 159.8946522441011382, 253.7013337850969492, -16.68230890105693121 ) ) ;
#85611=CARTESIAN_POINT ( 'NONE',  ( 174.4457123674840489, 286.1056755372895850, 10.49813771419831987 ) ) ;
#85614=CARTESIAN_POINT ( 'NONE',  ( 204.8762144138505903, 275.7909827032724479, 14.60855957933206817 ) ) ;
#85616=CARTESIAN_POINT ( 'NONE',  ( 205.2937235227012707, 275.0678357141204629, -12.80017165135291535 ) ) ;
#85617=CARTESIAN_POINT ( 'NONE',  ( 136.3579783227721691, 249.5333772461660544, 9.188101187500095079 ) ) ;
#85618=CARTESIAN_POINT ( 'NONE',  ( 206.4254562207697461, 270.5990383981129526, 2.448344251486097356 ) ) ;
#85619=CARTESIAN_POINT ( 'NONE',  ( 195.7512027426080294, 291.1991186218746748, -15.77572119551195939 ) ) ;
#85620=CARTESIAN_POINT ( 'NONE',  ( 72.92127039979699532, 225.1589784336661637, -6.496448406907675876E-16 ) ) ;
#85621=ORIENTED_EDGE ( 'NONE', *, *, #94713, .T. ) ;
#85622=CARTESIAN_POINT ( 'NONE',  ( 190.7851866479434761, 300.1973587246873194, 7.931162401707728016 ) ) ;
#85623=CARTESIAN_POINT ( 'NONE',  ( 191.2649737798357705, 297.3663430354321235, 11.06343876070684296 ) ) ;
#85624=VERTEX_POINT ( 'NONE', #70989 ) ;
#85625=CARTESIAN_POINT ( 'NONE',  ( 196.1152085310149573, 290.9654900177533818, -16.34875648285824568 ) ) ;
#85626=ORIENTED_EDGE ( 'NONE', *, *, #42615, .F. ) ;
#85629=B_SPLINE_CURVE_WITH_KNOTS ( 'NONE', 3,
 ( #95599, #26643, #88006, #41828, #80387, #10957, #81385, #57526, #42811, #88502, #73252, #41644, #25455, #18371, #72587, #25977, #16851, #17352, #47251, #62953, #9266, #56847, #95421, #93903, #70551, #34076, #64967, #3193, #56343, #1678 ),
 .UNSPECIFIED., .F., .F.,
 ( 4, 2, 2, 2, 2, 2, 2, 2, 2, 2, 2, 2, 2, 2, 4 ),
 ( 0.0005501412985831557892, 0.001170896183476429191, 0.001791651068369702702, 0.003033160838156182502, 0.003653915723049342822, 0.003964293165495931873, 0.004041887526107601145, 0.004080684706413485220, 0.004119481886719368428, 0.004197076247331136579, 0.004274670607942904731, 0.004585048050390315606, 0.004895425492837726482, 0.005205802935285142562, 0.005516180377732559509 ),
 .UNSPECIFIED. ) ;
#85632=CARTESIAN_POINT ( 'NONE',  ( 54.99669585504140912, 195.8927522451417929, -10.00000000000009237 ) ) ;
#85633=CARTESIAN_POINT ( 'NONE',  ( 158.9281150132903520, 281.5174227188211944, 6.950568428669476440 ) ) ;
#85634=CARTESIAN_POINT ( 'NONE',  ( 78.44218234892278474, 228.3464784336661353, 1.353441290958777327E-15 ) ) ;
#85636=ORIENTED_EDGE ( 'NONE', *, *, #31894, .T. ) ;
#85637=CARTESIAN_POINT ( 'NONE',  ( 161.6469353826265660, 250.6662903599244316, -14.26861606608829902 ) ) ;
#85640=B_SPLINE_CURVE_WITH_KNOTS ( 'NONE', 3,
 ( #97222, #81525, #80535, #73895 ),
 .UNSPECIFIED., .F., .F.,
 ( 4, 4 ),
 ( 0.008124507445708663983, 0.01396828671364515329 ),
 .UNSPECIFIED. ) ;
#85645=CARTESIAN_POINT ( 'NONE',  ( 205.8379285891498682, 274.1252448892948905, 10.44730901608240181 ) ) ;
#85649=CARTESIAN_POINT ( 'NONE',  ( 159.5818694439545311, 259.7229583450298378, 16.67297602109374566 ) ) ;
#85651=EDGE_LOOP ( 'NONE', ( #95992, #36081, #61903, #97811 ) ) ;
#85652=CARTESIAN_POINT ( 'NONE',  ( 158.0398765280698683, 259.7347367507720151, 17.70793151717339597 ) ) ;
#85653=B_SPLINE_CURVE_WITH_KNOTS ( 'NONE', 3,
 ( #71765, #57029, #838, #79393 ),
 .UNSPECIFIED., .F., .F.,
 ( 4, 4 ),
 ( 0.04619905480260320940, 0.04887120950165262795 ),
 .UNSPECIFIED. ) ;
#85655=ADVANCED_FACE ( 'NONE', ( #9695 ), #6139, .F. ) ;
#85656=CARTESIAN_POINT ( 'NONE',  ( 147.7401540708734728, 275.1386901812263659, -4.214051892962178414 ) ) ;
#85657=CARTESIAN_POINT ( 'NONE',  ( 152.9273493951901628, 265.7690563111299298, -17.70273273795505631 ) ) ;
#85658=CARTESIAN_POINT ( 'NONE',  ( 102.5355703512972809, 241.5530062829863027, -4.648177544792955347E-16 ) ) ;
#85663=CARTESIAN_POINT ( 'NONE',  ( 181.8770762757046668, 291.4574127364229525, 9.786853623632657317 ) ) ;
#85665=CARTESIAN_POINT ( 'NONE',  ( 171.6338951559981183, 251.5524196502057634, 7.220225173970846733 ) ) ;
#85666=CARTESIAN_POINT ( 'NONE',  ( 198.5095128836955212, 266.2414960645399447, 0.9413577709342229038 ) ) ;
#85668=CARTESIAN_POINT ( 'NONE',  ( 156.5497824763685912, 272.6770023486104719, 14.78669166138748814 ) ) ;
#85669=ORIENTED_EDGE ( 'NONE', *, *, #29555, .T. ) ;
#85670=FACE_OUTER_BOUND ( 'NONE', #95825, .T. ) ;
#85671=CARTESIAN_POINT ( 'NONE',  ( 162.8037981520209314, 248.6625452659484381, 9.809699077002424161 ) ) ;
#85672=VECTOR ( 'NONE', #36167, 1000.000000000000000 ) ;
#85673=CARTESIAN_POINT ( 'NONE',  ( 164.7243055739305078, 245.3361288348881999, -1.445094907380085170 ) ) ;
#85674=CARTESIAN_POINT ( 'NONE',  ( 178.2593621835967497, 264.8045418315043094, -15.94341754528856292 ) ) ;
#85676=CARTESIAN_POINT ( 'NONE',  ( 175.8611927472028640, 285.7234504611549255, -13.40660829471084980 ) ) ;
#85679=CARTESIAN_POINT ( 'NONE',  ( 169.1077096135931015, 273.0669116561859937, 15.96758563191977665 ) ) ;
#85680=CARTESIAN_POINT ( 'NONE',  ( 166.4590851264997582, 286.5435392614748480, -3.277556783383077654 ) ) ;
#85682=CARTESIAN_POINT ( 'NONE',  ( 188.3874671557833551, 260.9085831127977144, 2.874786128283515207 ) ) ;
#85683=CARTESIAN_POINT ( 'NONE',  ( 207.8996209429610360, 270.5542889829179103, -5.987818313449536411 ) ) ;
#85684=CARTESIAN_POINT ( 'NONE',  ( -7.673045192009834814, 172.5024278399160664, -9.188101187500093303 ) ) ;
#85685=CARTESIAN_POINT ( 'NONE',  ( 148.4047294057049271, 273.6024639162449716, 1.815056976409021644E-15 ) ) ;
#85686=ORIENTED_EDGE ( 'NONE', *, *, #3118, .F. ) ;
#85687=CARTESIAN_POINT ( 'NONE',  ( 160.8493410219326165, 253.1035779242602928, -14.73755040960339002 ) ) ;
#85690=CARTESIAN_POINT ( 'NONE',  ( 151.0801312611820890, 268.9685319718947198, -15.83903210480701240 ) ) ;
#85691=CARTESIAN_POINT ( 'NONE',  ( 21.71786549680706102, 183.3458772461660544, 9.188101187500095079 ) ) ;
#85692=CARTESIAN_POINT ( 'NONE',  ( 62.31174343829394502, 218.3297689869269220, -2.679491924311252493 ) ) ;
#85694=CARTESIAN_POINT ( 'NONE',  ( 193.8848781386269309, 267.1185884883711879, -11.59377028749509364 ) ) ;
#85695=CARTESIAN_POINT ( 'NONE',  ( 191.8232488616404225, 298.3993822291468518, -9.342381338555176384 ) ) ;
#85699=DIRECTION ( 'NONE',  ( -0.4999999999999987788, 0.8660254037844392627, 0.000000000000000000 ) ) ;
#85700=CARTESIAN_POINT ( 'NONE',  ( 190.0214546701687652, 261.5450160817866845, -0.7541398968587580409 ) ) ;
#85701=EDGE_CURVE ( 'NONE', #34750, #2250, #23846, .T. ) ;
#85702=CARTESIAN_POINT ( 'NONE',  ( 70.67536410627003818, 221.6115022471903160, -5.000000000000047962 ) ) ;
#85703=CARTESIAN_POINT ( 'NONE',  ( 164.5351584576669381, 246.1509890714488336, 1.273074117816153983 ) ) ;
#85704=CARTESIAN_POINT ( 'NONE',  ( 203.3628419156056282, 270.1034488468966970, 6.158600121215549450 ) ) ;
#85705=CARTESIAN_POINT ( 'NONE',  ( 27.69859311986958872, 195.9869531367911293, 4.594050593750046652 ) ) ;
#85706=CARTESIAN_POINT ( 'NONE',  ( 169.2145527580371152, 252.8177965952870920, -11.54809748734068720 ) ) ;
#85707=EDGE_CURVE ( 'NONE', #82473, #40420, #60090, .T. ) ;
#85708=CARTESIAN_POINT ( 'NONE',  ( 202.9918396203695465, 270.0308483619746198, -6.392315799726350889 ) ) ;
#85709=CARTESIAN_POINT ( 'NONE',  ( 198.8194531333411419, 286.2816009704309863, -17.01510935557533344 ) ) ;
#85713=CARTESIAN_POINT ( 'NONE',  ( -5.006187249323398092, 179.4637435831425023, 2.679491924311264039 ) ) ;
#85714=CARTESIAN_POINT ( 'NONE',  ( 202.7544846896944080, 279.0752537093788419, -15.21816053415730963 ) ) ;
#85717=CARTESIAN_POINT ( 'NONE',  ( 202.8499463704053198, 279.3005819042728604, 17.04674939340617001 ) ) ;
#85718=CARTESIAN_POINT ( 'NONE',  ( 148.9194629746633893, 272.7109192224475009, -12.27648025871169679 ) ) ;
#85719=CARTESIAN_POINT ( 'NONE',  ( 185.7622240277081289, 267.5937315954845417, -14.89893092516080841 ) ) ;
#85721=VECTOR ( 'NONE', #41015, 1000.000000000000000 ) ;
#85722=CARTESIAN_POINT ( 'NONE',  ( 185.2961235551778714, 291.2460235572835927, 13.48139818756336616 ) ) ;
#85724=ADVANCED_FACE ( 'NONE', ( #74382 ), #44970, .F. ) ;
#85725=DIRECTION ( 'NONE',  ( 0.4999999999999992784, -0.8660254037844390407, 0.000000000000000000 ) ) ;
#85731=CARTESIAN_POINT ( 'NONE',  ( 177.4877928417686803, 293.5951873982637608, -2.837372163671336267 ) ) ;
#85733=CARTESIAN_POINT ( 'NONE',  ( 150.7254409736883645, 269.5828735707850683, 14.54962197351449049 ) ) ;
#85735=( BOUNDED_CURVE ( )  B_SPLINE_CURVE ( 2, ( #92486, #21091, #84889, #52953, #15429, #67660, #99568, #76278, #46327 ),
 .UNSPECIFIED., .F., .T. ) 
 B_SPLINE_CURVE_WITH_KNOTS ( ( 3, 2, 2, 2, 3 ),
 ( 0.7701612903225806273, 0.7715053763440860024, 0.7741935483870967527, 0.7768817204301075030, 0.7782258064516128782 ),
 .UNSPECIFIED. ) 
 CURVE ( )  GEOMETRIC_REPRESENTATION_ITEM ( )  RATIONAL_B_SPLINE_CURVE ( ( 0.9330127018922194093, 0.9330127018922194093, 1.000000000000000000, 0.8660254037844387076, 1.000000000000000000, 0.8660254037844387076, 1.000000000000000000, 0.9330127018922194093, 0.9330127018922194093 ) ) 
 REPRESENTATION_ITEM ( '' )  );
#85736=ORIENTED_EDGE ( 'NONE', *, *, #47408, .F. ) ;
#85741=CARTESIAN_POINT ( 'NONE',  ( 153.3939648708017387, 264.9608545997728015, -16.49556533540763681 ) ) ;
#85745=CARTESIAN_POINT ( 'NONE',  ( 190.4744901378711290, 300.7355008658671522, 0.04566709859947504224 ) ) ;
#85747=CARTESIAN_POINT ( 'NONE',  ( 180.3656040069006110, 287.1229193970689835, -13.78812687696878037 ) ) ;
#85748=ORIENTED_EDGE ( 'NONE', *, *, #81679, .F. ) ;
#85749=CARTESIAN_POINT ( 'NONE',  ( 195.9359860111818250, 291.2759125279654882, 17.49638312768267312 ) ) ;
#85753=CARTESIAN_POINT ( 'NONE',  ( 159.3767386493506137, 254.5983864451355032, 15.47015898230477760 ) ) ;
#85755=CARTESIAN_POINT ( 'NONE',  ( 61.79834339388186493, 215.6744531367911293, 4.594050593750047540 ) ) ;
#85756=ORIENTED_EDGE ( 'NONE', *, *, #32439, .F. ) ;
#85760=CARTESIAN_POINT ( 'NONE',  ( 87.06313848696181878, 232.6199935810941213, 2.679491924311251605 ) ) ;
#85762=VERTEX_POINT ( 'NONE', #22643 ) ;
#85764=CARTESIAN_POINT ( 'NONE',  ( 190.2114739955665073, 299.5471927289356699, 6.539000334076677134 ) ) ;
#85765=LINE ( 'NONE', #54271, #83647 ) ;
#85767=CARTESIAN_POINT ( 'NONE',  ( 190.5893431400089923, 300.5365696307625853, -0.3099240395267599535 ) ) ;
#85768=VERTEX_POINT ( 'NONE', #68731 ) ;
#85769=CARTESIAN_POINT ( 'NONE',  ( 149.0359194785865498, 272.5092106407810206, 12.76357969772040590 ) ) ;
#85771=CARTESIAN_POINT ( 'NONE',  ( 207.8984236726843164, 270.5563627158673512, -6.084369154771423815 ) ) ;
#85772=CARTESIAN_POINT ( 'NONE',  ( 192.5076277540105423, 297.2140032159341558, -13.10094381206144298 ) ) ;
#85773=CARTESIAN_POINT ( 'NONE',  ( 160.5559693517773781, 255.9979613941079037, 15.97241449062581076 ) ) ;
#85775=EDGE_CURVE ( 'NONE', #35245, #11947, #68231, .T. ) ;
#85776=CARTESIAN_POINT ( 'NONE',  ( 206.4537138826727301, 273.0586734743599209, 11.45643784582899016 ) ) ;
#85778=CARTESIAN_POINT ( 'NONE',  ( 103.9969882237314351, 242.3967562850347122, -4.648177544792955347E-16 ) ) ;
#85780=CARTESIAN_POINT ( 'NONE',  ( 114.1121243109418799, 230.5643266524159856, -9.188101187500093303 ) ) ;
#85781=ORIENTED_EDGE ( 'NONE', *, *, #29723, .F. ) ;
#85782=CARTESIAN_POINT ( 'NONE',  ( 146.9235493515124062, 276.1679430252639804, 0.7994986043261682607 ) ) ;
#85785=CARTESIAN_POINT ( 'NONE',  ( 203.5258219653775313, 278.1299310341851765, -16.21052911601769608 ) ) ;
#85786=CARTESIAN_POINT ( 'NONE',  ( 204.8284483594339065, 275.8737159363993214, 14.69997973035875383 ) ) ;
#85787=CARTESIAN_POINT ( 'NONE',  ( -12.62545442379354554, 163.5177522451418781, -10.00000000000009592 ) ) ;
#85788=CARTESIAN_POINT ( 'NONE',  ( 168.5060701671863796, 284.6850982760621491, -7.967140632246684895 ) ) ;
#85790=CARTESIAN_POINT ( 'NONE',  ( 162.7007457333762090, 248.8410372908842021, -10.94671474643812914 ) ) ;
#85792=CARTESIAN_POINT ( 'NONE',  ( 206.3712092866207968, 272.8206792488882115, 8.318967530036161406 ) ) ;
#85793=CARTESIAN_POINT ( 'NONE',  ( 125.9117204375048544, 237.3768266524159856, 9.188101187500096856 ) ) ;
#85795=CARTESIAN_POINT ( 'NONE',  ( 190.0654709403812319, 294.6198108877256345, -12.35559205623138723 ) ) ;
#85796=AXIS2_PLACEMENT_3D ( 'NONE', #82149, #36481, #12208 ) ;
#85797=CARTESIAN_POINT ( 'NONE',  ( 185.8803129279731365, 296.7512827758666276, 4.593912753767370738 ) ) ;
#85798=CARTESIAN_POINT ( 'NONE',  ( 196.3720681610792553, 290.5205960880691691, 16.18360420724715354 ) ) ;
#85800=CARTESIAN_POINT ( 'NONE',  ( 51.05482314576993730, 188.0327760586659451, 1.948934522072303157E-15 ) ) ;
#85801=B_SPLINE_CURVE_WITH_KNOTS ( 'NONE', 3,
 ( #42800, #5332, #73735, #12951 ),
 .UNSPECIFIED., .F., .F.,
 ( 4, 4 ),
 ( 0.006434672157312129256, 0.01144118791506597635 ),
 .UNSPECIFIED. ) ;
#85803=ORIENTED_EDGE ( 'NONE', *, *, #98843, .F. ) ;
#85809=CARTESIAN_POINT ( 'NONE',  ( 171.5340268345807146, 259.8473005894099970, 15.39510975745485233 ) ) ;
#85811=CARTESIAN_POINT ( 'NONE',  ( 154.8833801513861772, 262.3811116602312268, -17.49275566389638215 ) ) ;
#85812=AXIS2_PLACEMENT_3D ( 'NONE', #22063, #68158, #83405 ) ;
#85813=CARTESIAN_POINT ( 'NONE',  ( 155.2509783050690544, 269.7933175191985811, -14.93214736645873586 ) ) ;
#85814=CARTESIAN_POINT ( 'NONE',  ( 109.5562962934609459, 247.3927522451419634, 2.944929066748280225E-16 ) ) ;
#85816=CARTESIAN_POINT ( 'NONE',  ( 194.4565572889705152, 292.7111445759336448, -15.25152910787323357 ) ) ;
#85818=CARTESIAN_POINT ( 'NONE',  ( 202.9216520459657147, 279.1763840310111391, 15.75371595331685803 ) ) ;
#85820=CARTESIAN_POINT ( 'NONE',  ( 27.50958393249801404, 180.5643266524160424, 9.188101187500095079 ) ) ;
#85825=CARTESIAN_POINT ( 'NONE',  ( 198.0795109501767115, 277.7783264603462499, -16.13655660432609906 ) ) ;
#85826=CARTESIAN_POINT ( 'NONE',  ( 68.02342162723002161, 200.8923013555409796, 4.594050593750050204 ) ) ;
#85827=CARTESIAN_POINT ( 'NONE',  ( 164.4963285489318991, 245.7309966251440301, -6.672251175510283794 ) ) ;
#85828=CARTESIAN_POINT ( 'NONE',  ( 119.4694200880668831, 251.3297689869269504, -2.679491924311252493 ) ) ;
#85829=CARTESIAN_POINT ( 'NONE',  ( 180.8078237589699029, 256.2600327853984936, 1.558727462200503400 ) ) ;
#85832=ORIENTED_EDGE ( 'NONE', *, *, #89920, .F. ) ;
#85833=EDGE_CURVE ( 'NONE', #61735, #47657, #10601, .T. ) ;
#85834=CARTESIAN_POINT ( 'NONE',  ( 37.40555484421791022, 185.7365022471902023, 10.00000000000009592 ) ) ;
#85836=DIRECTION ( 'NONE',  ( -0.4999999999999987788, 0.8660254037844392627, 0.000000000000000000 ) ) ;
#85837=CARTESIAN_POINT ( 'NONE',  ( -16.46870247313679059, 170.4869531367911293, 4.594050593750046652 ) ) ;
#85839=CARTESIAN_POINT ( 'NONE',  ( 167.7942285755875957, 262.4949493498345987, -16.83134817174553532 ) ) ;
#85840=CARTESIAN_POINT ( 'NONE',  ( 199.9809106644752035, 283.6121499399518484, 16.99530978087883071 ) ) ;
#85841=CARTESIAN_POINT ( 'NONE',  ( 189.2732718030835599, 261.7774826209242178, 6.629783814786226692 ) ) ;
#85842=EDGE_CURVE ( 'NONE', #5449, #38097, #78725, .T. ) ;
#85843=CARTESIAN_POINT ( 'NONE',  ( 206.2456893945931142, 273.4189824569319285, 10.13882547285618152 ) ) ;
#85845=EDGE_CURVE ( 'NONE', #85624, #4581, #55236, .T. ) ;
#85848=CARTESIAN_POINT ( 'NONE',  ( 150.4638999619119204, 271.8026217546109251, -12.79869408032183742 ) ) ;
#85849=CARTESIAN_POINT ( 'NONE',  ( 181.0855840883816938, 287.1795278100775590, 13.27675118985169433 ) ) ;
#85852=CARTESIAN_POINT ( 'NONE',  ( 160.4207999851416560, 252.7900191653268394, 16.17069880550225847 ) ) ;
#85854=CARTESIAN_POINT ( 'NONE',  ( 204.8878784573704195, 275.7707799872745795, -14.13380496213581594 ) ) ;
#85855=ADVANCED_FACE ( 'NONE', ( #25000 ), #17926, .T. ) ;
#85856=CARTESIAN_POINT ( 'NONE',  ( 115.2960263294082068, 225.8262482093458061, 3.021315404115420679E-15 ) ) ;
#85858=CARTESIAN_POINT ( 'NONE',  ( 191.3441257904396764, 298.1785231045369642, 9.312382026386032408 ) ) ;
#85859=CARTESIAN_POINT ( 'NONE',  ( 163.2000388741132895, 247.9762362032568035, -11.19676374274550312 ) ) ;
#85860=CARTESIAN_POINT ( 'NONE',  ( 152.9273493951901628, 265.7690563111299298, -17.70273273795505631 ) ) ;
#85862=ORIENTED_EDGE ( 'NONE', *, *, #9625, .F. ) ;
#85863=CARTESIAN_POINT ( 'NONE',  ( 155.8157825667570080, 277.1861924174589262, -10.41322603298928051 ) ) ;
#85864=CARTESIAN_POINT ( 'NONE',  ( 188.7930588916510999, 290.9633865388665299, 14.97457979531618832 ) ) ;
#85867=CARTESIAN_POINT ( 'NONE',  ( 155.5207183646172950, 261.6826666266933898, -16.99780945766855922 ) ) ;
#85872=CARTESIAN_POINT ( 'NONE',  ( 164.3330377059402849, 246.0138246616164110, 7.208046019122525294 ) ) ;
#85875=CARTESIAN_POINT ( 'NONE',  ( 161.2799361541916028, 251.3019516699124836, 14.40628917569557110 ) ) ;
#85876=CARTESIAN_POINT ( 'NONE',  ( 166.1070111784138703, 253.4115428555481344, -13.60050710122670559 ) ) ;
#85886=ORIENTED_EDGE ( 'NONE', *, *, #40551, .T. ) ;
#85887=CARTESIAN_POINT ( 'NONE',  ( 164.4698008747318738, 245.7769439046653019, -6.272955660526681854 ) ) ;
#85889=CARTESIAN_POINT ( 'NONE',  ( 165.1033008171500001, 270.9562025061328541, 16.67780619943411580 ) ) ;
#85890=CARTESIAN_POINT ( 'NONE',  ( 167.6723227085472558, 281.1242618559421089, 11.55074042278067559 ) ) ;
#85891=EDGE_CURVE ( 'NONE', #91334, #94724, #33563, .T. ) ;
#85892=CARTESIAN_POINT ( 'NONE',  ( 194.9385458806846430, 293.0035295114944347, -15.70518692812489192 ) ) ;
#85894=CARTESIAN_POINT ( 'NONE',  ( 159.0424690102808256, 255.1773584434317570, -17.34001589335112925 ) ) ;
#85895=CARTESIAN_POINT ( 'NONE',  ( 200.8532844524641803, 271.0267732368380962, -11.47671578755057986 ) ) ;
#85898=CARTESIAN_POINT ( 'NONE',  ( 191.6400076255916076, 298.3370758160374976, -8.690192626989791336 ) ) ;
#85899=CARTESIAN_POINT ( 'NONE',  ( 206.7921793621094650, 271.5292813338429596, 6.134403222006724832 ) ) ;
#85900=ORIENTED_EDGE ( 'NONE', *, *, #18526, .F. ) ;
#85901=CARTESIAN_POINT ( 'NONE',  ( 190.8738732131464246, 300.0437490878071003, 5.255515203389859558 ) ) ;
#85903=CARTESIAN_POINT ( 'NONE',  ( 159.3451320108506764, 254.6531307488737355, -16.72997986213134425 ) ) ;
#85906=CARTESIAN_POINT ( 'NONE',  ( 200.3765029811139584, 283.5847115241710981, 16.85207472104531590 ) ) ;
#85907=CARTESIAN_POINT ( 'NONE',  ( 191.1252388389400778, 261.3801678008247791, -0.002822319849339915022 ) ) ;
#85908=ORIENTED_EDGE ( 'NONE', *, *, #41095, .F. ) ;
#85909=CARTESIAN_POINT ( 'NONE',  ( 194.3387753395540472, 294.0423625616157892, -15.64827765940100868 ) ) ;
#85912=CARTESIAN_POINT ( 'NONE',  ( 18.62362889609489969, 194.8927522451419634, 2.944929066748280225E-16 ) ) ;
#85913=CARTESIAN_POINT ( 'NONE',  ( 85.37073267496330686, 220.0958772461660544, -9.188101187500095079 ) ) ;
#85915=CARTESIAN_POINT ( 'NONE',  ( 196.3918367485927376, 269.1678964851112141, -12.08347791044659303 ) ) ;
#85917=CARTESIAN_POINT ( 'NONE',  ( 169.0459840413011534, 279.5632588650593107, -13.46217358039099921 ) ) ;
#85918=CARTESIAN_POINT ( 'NONE',  ( 3.260525530768699998, 178.8149278399161233, 9.188101187500093303 ) ) ;
#85920=CARTESIAN_POINT ( 'NONE',  ( 161.4844649541891499, 250.9476973967054789, 12.93553496455142415 ) ) ;
#85921=ORIENTED_EDGE ( 'NONE', *, *, #14221, .T. ) ;
#85925=CARTESIAN_POINT ( 'NONE',  ( 201.2505344690289064, 267.2087450970302029, -3.778420330458906573 ) ) ;
#85928=EDGE_CURVE ( 'NONE', #71782, #69624, #73404, .T. ) ;
#85930=CARTESIAN_POINT ( 'NONE',  ( 161.8926315922002743, 250.2407320417157166, -13.77020595223768495 ) ) ;
#85931=CARTESIAN_POINT ( 'NONE',  ( 105.1336465626505969, 243.0530062829863027, -4.648177544792955347E-16 ) ) ;
#85933=CARTESIAN_POINT ( 'NONE',  ( 37.27951979288245354, 183.1423013555409796, -4.594050593750043987 ) ) ;
#85934=CARTESIAN_POINT ( 'NONE',  ( 199.5106878072222685, 277.4853542194088618, 15.16379332014005321 ) ) ;
#85935=ORIENTED_EDGE ( 'NONE', *, *, #76851, .T. ) ;
#85936=CARTESIAN_POINT ( 'NONE',  ( 153.4303388563101862, 273.9525667856884183, -11.93370399901073853 ) ) ;
#85937=CARTESIAN_POINT ( 'NONE',  ( 182.3263212693539685, 260.8467281569974716, -10.61505835826066502 ) ) ;
#85938=CARTESIAN_POINT ( 'NONE',  ( -4.215479392844351914, 156.8262482093458061, -4.415768667553308270E-15 ) ) ;
#85939=DIRECTION ( 'NONE',  ( 0.4999999999999992784, -0.8660254037844390407, 0.000000000000000000 ) ) ;
#85940=CARTESIAN_POINT ( 'NONE',  ( 155.1376601545389917, 261.9406857754215707, 18.55063430030667959 ) ) ;
#85941=CARTESIAN_POINT ( 'NONE',  ( 62.88113547221012567, 207.1115022471902307, 10.00000000000009592 ) ) ;
#85943=CARTESIAN_POINT ( 'NONE',  ( 147.8819534105757043, 274.5079385007862811, -9.338341377131436971 ) ) ;
#85944=CARTESIAN_POINT ( 'NONE',  ( 189.8033664021961613, 262.5080370049500971, 8.283948267418471900 ) ) ;
#85945=CARTESIAN_POINT ( 'NONE',  ( 168.1784323372465906, 278.2753528722733449, 14.27304841468856722 ) ) ;
#85946=CARTESIAN_POINT ( 'NONE',  ( 22.61095419623372038, 183.8615022471902591, -10.00000000000009592 ) ) ;
#85948=CARTESIAN_POINT ( 'NONE',  ( 147.8503508990560533, 274.5626756563852950, 7.845851077393495743 ) ) ;
#85949=CARTESIAN_POINT ( 'NONE',  ( 181.2456060316003743, 265.9490061796501550, -15.17417357770760944 ) ) ;
#85952=AXIS2_PLACEMENT_3D ( 'NONE', #31625, #62524, #20022 ) ;
#85953=ADVANCED_FACE ( 'NONE', ( #65502 ), #58074, .F. ) ;
#85954=CARTESIAN_POINT ( 'NONE',  ( 161.5753992217405823, 251.8338521006345161, -13.71391156857418281 ) ) ;
#85955=CARTESIAN_POINT ( 'NONE',  ( 104.0442318961827652, 237.0024278399160949, -9.188101187500093303 ) ) ;
#85957=B_SPLINE_CURVE_WITH_KNOTS ( 'NONE', 3,
 ( #38226, #7858, #38737, #8354 ),
 .UNSPECIFIED., .F., .F.,
 ( 4, 4 ),
 ( 0.01442566870911189854, 0.02312499380068684662 ),
 .UNSPECIFIED. ) ;
#85958=CARTESIAN_POINT ( 'NONE',  ( 150.7226148805041817, 269.5877685077668957, 15.52819754351937576 ) ) ;
#85959=CARTESIAN_POINT ( 'NONE',  ( -22.42236680055709641, 157.8615022471902591, 0.000000000000000000 ) ) ;
#85960=CARTESIAN_POINT ( 'NONE',  ( 205.4925884257800988, 274.0740247280971857, 10.80283695292349222 ) ) ;
#85961=CARTESIAN_POINT ( 'NONE',  ( 191.6210545128721776, 276.9003016344976800, 17.04950522666647217 ) ) ;
#85963=CARTESIAN_POINT ( 'NONE',  ( 192.8725807964287924, 263.8132596570546298, -4.373067053639174695 ) ) ;
#85964=CARTESIAN_POINT ( 'NONE',  ( 149.9052967174216917, 271.6272115183317624, -11.69003756284735829 ) ) ;
#85966=CARTESIAN_POINT ( 'NONE',  ( 189.9879251633717558, 299.5782561228834879, -6.671532329245590809 ) ) ;
#85969=CARTESIAN_POINT ( 'NONE',  ( 192.7355331156994964, 267.2041169143933530, 11.12292375133700517 ) ) ;
#85973=ORIENTED_EDGE ( 'NONE', *, *, #74099, .T. ) ;
#85974=FACE_OUTER_BOUND ( 'NONE', #83847, .T. ) ;
#85975=CARTESIAN_POINT ( 'NONE',  ( 196.1749740761792111, 288.8619730569873809, -17.33086882175758703 ) ) ;
#85977=CARTESIAN_POINT ( 'NONE',  ( 142.9163165386219703, 259.9865022471903444, 10.00000000000009237 ) ) ;
#85978=VERTEX_POINT ( 'NONE', #61377 ) ;
#85981=EDGE_LOOP ( 'NONE', ( #81913, #95079, #56448, #56791, #46413, #94490, #62005, #78245, #81235, #79965, #73734, #81866, #51854, #44957, #56300, #72378, #62422, #30585, #39048, #87630 ) ) ;
#85985=EDGE_LOOP ( 'NONE', ( #64115, #40962, #77481, #23220 ) ) ;
#85988=CARTESIAN_POINT ( 'NONE',  ( 163.9704062730716032, 246.6419207277664327, 7.317582738093436845 ) ) ;
#85991=CARTESIAN_POINT ( 'NONE',  ( 170.5924673348125964, 258.8840003614211582, 15.37362746749550624 ) ) ;
#85993=CARTESIAN_POINT ( 'NONE',  ( 33.34606076043043998, 183.3927522451418497, 10.00000000000009948 ) ) ;
#85996=CARTESIAN_POINT ( 'NONE',  ( 162.8386403195304410, 249.0994062285972461, 10.29435687412694911 ) ) ;
#85999=EDGE_CURVE ( 'NONE', #86029, #79763, #15411, .T. ) ;
#86004=CARTESIAN_POINT ( 'NONE',  ( 190.4750788177879883, 300.1286839245400415, -3.520404030213226676 ) ) ;
#86005=CARTESIAN_POINT ( 'NONE',  ( 164.4306612431381325, 245.8447357351751066, -2.314684942147286595 ) ) ;
#86006=CARTESIAN_POINT ( 'NONE',  ( 147.4018083154577994, 275.3395742005352531, -7.372329269489205750 ) ) ;
#86007=CARTESIAN_POINT ( 'NONE',  ( 196.1019265324206629, 284.4571118909283314, -17.79305111687722274 ) ) ;
#86009=CARTESIAN_POINT ( 'NONE',  ( 171.5849702451724852, 250.5752846868085726, -5.747692145100161021 ) ) ;
#86012=CARTESIAN_POINT ( 'NONE',  ( 157.6776325807875878, 281.5257696872717474, 2.944928808717816704 ) ) ;
#86013=CARTESIAN_POINT ( 'NONE',  ( 129.3758220526426044, 239.3768266524160140, -9.188101187500091527 ) ) ;
#86014=CARTESIAN_POINT ( 'NONE',  ( 183.6008598791219129, 260.5699149889866248, -9.267803207057191628 ) ) ;
#86016=VERTEX_POINT ( 'NONE', #64389 ) ;
#86019=CARTESIAN_POINT ( 'NONE',  ( 200.1188775601148109, 273.7126575094745817, 13.85740573495379557 ) ) ;
#86020=CARTESIAN_POINT ( 'NONE',  ( 178.2114048607894858, 253.3878526894902166, 1.409026425838265872 ) ) ;
#86022=CARTESIAN_POINT ( 'NONE',  ( 147.1444677838046573, 275.7853010762056556, 2.585175795350988626 ) ) ;
#86024=CARTESIAN_POINT ( 'NONE',  ( 201.1060504099706350, 282.3210983108598384, -18.18000168485860257 ) ) ;
#86026=CARTESIAN_POINT ( 'NONE',  ( 174.8987400875574281, 282.4155400008056631, 14.62834699329571286 ) ) ;
#86027=AXIS2_PLACEMENT_3D ( 'NONE', #88376, #54012, #18931 ) ;
#86029=VERTEX_POINT ( 'NONE', #23874 ) ;
#86030=CARTESIAN_POINT ( 'NONE',  ( 194.3708539535661259, 293.9868007723104029, -16.01585187499628304 ) ) ;
#86033=B_SPLINE_CURVE_WITH_KNOTS ( 'NONE', 3,
 ( #51742, #70416, #63817, #33421, #16219, #16716, #24811, #23809, #71435, #86676, #85162, #15706, #31410, #2025, #25314, #32910, #62297, #54698, #23306, #55688, #94257, #8129, #47610, #69908, #92752, #46606, #87197, #56201, #1025, #94752, #17730, #10125, #93254, #85682, #70933, #9644, #86182, #77538, #93765, #31904, #63316, #523, #39003, #48633, #47111, #79566, #40991, #71934, #78031, #8623, #1539, #40503 ),
 .UNSPECIFIED., .F., .F.,
 ( 4, 2, 2, 2, 2, 2, 2, 2, 2, 2, 2, 2, 2, 2, 2, 2, 2, 2, 2, 2, 2, 2, 2, 2, 2, 4 ),
 ( 0.0001164149332258714178, 0.0006113509262942967790, 0.001106286919362722181, 0.001353754915896962637, 0.001601222912431203094, 0.001724956910698308794, 0.001848690908965414711, 0.001972424907232520411, 0.002096158905499626111, 0.002343626902033844016, 0.002591094898568061054, 0.003086030891636534160, 0.004075902877773479940, 0.005065774863910425287, 0.005560710856978898393, 0.005808178853513132345, 0.005931912851780252356, 0.006055646850047372368, 0.006117513849180932807, 0.006179380848314493246, 0.006303114846581607186, 0.006550582843115837668, 0.007045518836184282152, 0.007292986832718569012, 0.007540454829252855005, 0.008035390822321386226 ),
 .UNSPECIFIED. ) ;
#86034=CARTESIAN_POINT ( 'NONE',  ( 191.3399829603070827, 267.7330644374129065, -12.16091939637846231 ) ) ;
#86035=CARTESIAN_POINT ( 'NONE',  ( 190.2972692340288177, 282.9090305667509142, -16.56549508821761663 ) ) ;
#86036=CARTESIAN_POINT ( 'NONE',  ( 151.7124930133047371, 267.8732492884548719, -16.17794402247774244 ) ) ;
#86037=CARTESIAN_POINT ( 'NONE',  ( 190.0259678364800493, 301.5123642802043946, 4.004183174499006626 ) ) ;
#86039=CARTESIAN_POINT ( 'NONE',  ( 161.9065591971467768, 281.7447826133235367, -6.599482603196943131 ) ) ;
#86040=CARTESIAN_POINT ( 'NONE',  ( 160.4448519566613243, 282.3920345168493782, 6.649608260177227059 ) ) ;
#86043=CARTESIAN_POINT ( 'NONE',  ( 146.8000281410530192, 276.3818880375922049, 4.652863924796177386 ) ) ;
#86047=ADVANCED_FACE ( 'NONE', ( #31972 ), #62877, .T. ) ;
#86049=CARTESIAN_POINT ( 'NONE',  ( 185.5568049818104726, 266.1438378612298834, 14.60334785453874140 ) ) ;
#86055=CARTESIAN_POINT ( 'NONE',  ( -0.5819415548772214342, 158.2202760586659451, -5.415160957724236172E-17 ) ) ;
#86056=ADVANCED_FACE ( 'NONE', ( #1609 ), #90522, .F. ) ;
#86057=CARTESIAN_POINT ( 'NONE',  ( 94.46399941469991290, 225.3458772461660544, 9.188101187500095079 ) ) ;
#86058=CARTESIAN_POINT ( 'NONE',  ( 26.94108121515588294, 196.3615022471903160, 5.000000000000046185 ) ) ;
#86059=CARTESIAN_POINT ( 'NONE',  ( 192.6789561813392595, 296.9172536750198219, -11.84591848451790952 ) ) ;
#86064=CARTESIAN_POINT ( 'NONE',  ( 174.0424481033923314, 287.4814580433055653, 10.99910921803667208 ) ) ;
#86067=CARTESIAN_POINT ( 'NONE',  ( 179.7416253924201897, 290.4642672521716236, 9.368538271801467587 ) ) ;
#86068=CARTESIAN_POINT ( 'NONE',  ( 169.2145703546568427, 252.0716163555370883, -8.781996148431376881 ) ) ;
#86069=CARTESIAN_POINT ( 'NONE',  ( 164.7496056545292049, 245.2923078098555436, -4.800585399662008257 ) ) ;
#86070=CARTESIAN_POINT ( 'NONE',  ( 168.3038276672707809, 273.7088255811268596, 16.50406143123535685 ) ) ;
#86071=CARTESIAN_POINT ( 'NONE',  ( 196.1613785401733878, 290.8855212161054737, 15.98157687694135021 ) ) ;
#86072=B_SPLINE_CURVE_WITH_KNOTS ( 'NONE', 3,
 ( #21275, #68848, #21758, #52152, #15136, #99769, #30360, #83101, #61245, #7550, #100275, #30861, #92694, #23245, #44544, #54132, #85095, #15641, #48565, #47056, #48050, #55633, #86618, #9063, #47549, #56137, #77970, #77475, #17152, #31352, #462, #1475, #39432, #24752, #54636, #71878, #8565, #32356, #78992, #87638, #9578, #40442, #39930, #63760, #2477, #64258, #25778, #32851, #24261, #18166, #56653, #62742 ),
 .UNSPECIFIED., .F., .F.,
 ( 4, 2, 2, 2, 2, 2, 2, 2, 2, 2, 2, 2, 2, 2, 2, 2, 2, 2, 2, 2, 2, 2, 2, 2, 2, 4 ),
 ( 0.0008473748616542479744, 0.001046208493274463670, 0.001145625309084543492, 0.001245042124894623313, 0.001443875756514765392, 0.001642709388134907687, 0.002040376651375070197, 0.002438043914615233357, 0.003233378441095451257, 0.004028712967575669157, 0.004824047494055886190, 0.005221714757295984298, 0.005420548388916032918, 0.005519965204726057229, 0.005569673612631022112, 0.005619382020535987864, 0.005669090428440952747, 0.005718798836345917631, 0.005818215652155869951, 0.006017049283775706935, 0.006215882915395543919, 0.006414716547015380903, 0.006613550178635217887, 0.006812383810255055738, 0.007011217441874892722, 0.007210051073494728839 ),
 .UNSPECIFIED. ) ;
#86075=CARTESIAN_POINT ( 'NONE',  ( 39.87759600423577666, 184.6423013555410080, -4.594050593750043987 ) ) ;
#86076=CARTESIAN_POINT ( 'NONE',  ( 65.07308872588301085, 214.5024278399160949, -9.188101187500093303 ) ) ;
#86079=B_SPLINE_CURVE_WITH_KNOTS ( 'NONE', 3,
 ( #16717, #23810, #55199, #54699 ),
 .UNSPECIFIED., .F., .F.,
 ( 4, 4 ),
 ( 0.004402801596837424558, 0.009103939997633007583 ),
 .UNSPECIFIED. ) ;
#86080=CARTESIAN_POINT ( 'NONE',  ( 97.08913892169542237, 236.8615022471903160, 5.000000000000046185 ) ) ;
#86081=CARTESIAN_POINT ( 'NONE',  ( 146.4255236417662616, 255.3458772461660260, 9.188101187500095079 ) ) ;
#86084=CARTESIAN_POINT ( 'NONE',  ( 196.2549797335509538, 269.5255532092754720, -10.78968121037139305 ) ) ;
#86086=CARTESIAN_POINT ( 'NONE',  ( 198.4860348845112981, 286.8590983175747056, -18.20461732983060088 ) ) ;
#86089=CARTESIAN_POINT ( 'NONE',  ( 72.89481452351749624, 203.7048013555409796, 4.594050593750051981 ) ) ;
#86091=CARTESIAN_POINT ( 'NONE',  ( 154.8786460229866577, 262.3893114111486398, -18.06164891362396929 ) ) ;
#86092=CARTESIAN_POINT ( 'NONE',  ( 198.6742831389107096, 286.5330427765190393, 17.60232614297041565 ) ) ;
#86094=CARTESIAN_POINT ( 'NONE',  ( 198.9746108066164254, 281.0633597085003998, 17.36576938231656442 ) ) ;
#86096=CARTESIAN_POINT ( 'NONE',  ( 101.3470971569689283, 235.9865022471903160, 10.00000000000009237 ) ) ;
#86100=CARTESIAN_POINT ( 'NONE',  ( 185.1165591157377150, 271.2723187119548811, 16.65506677990856943 ) ) ;
#86101=ORIENTED_EDGE ( 'NONE', *, *, #84930, .T. ) ;
#86102=CARTESIAN_POINT ( 'NONE',  ( 159.9647205790309101, 253.5799718689968927, -16.48298384325780219 ) ) ;
#86103=CARTESIAN_POINT ( 'NONE',  ( 190.3444704496978659, 278.7135669931259940, -16.51019796646277271 ) ) ;
#86105=CARTESIAN_POINT ( 'NONE',  ( 174.0867956421258498, 252.1420213558926946, -0.2508409156989133693 ) ) ;
#86106=VERTEX_POINT ( 'NONE', #68369 ) ;
#86108=CARTESIAN_POINT ( 'NONE',  ( 194.6943296385021824, 293.4265244509877562, -16.10917128197217352 ) ) ;
#86109=CARTESIAN_POINT ( 'NONE',  ( 206.7325995683429767, 270.5756292972641859, -5.459556455514786855 ) ) ;
#86110=EDGE_CURVE ( 'NONE', #14295, #69000, #56074, .T. ) ;
#86117=CYLINDRICAL_SURFACE ( 'NONE', #93367, 10.00000000000010658 ) ;
#86118=VERTEX_POINT ( 'NONE', #7067 ) ;
#86122=CARTESIAN_POINT ( 'NONE',  ( 168.7621418133986424, 265.8582162196448166, -17.70435637355228664 ) ) ;
#86123=CARTESIAN_POINT ( 'NONE',  ( 154.9226727788713731, 262.3130548330639726, 18.22497199616848818 ) ) ;
#86125=CARTESIAN_POINT ( 'NONE',  ( 157.1458804504438831, 258.4623461901232417, -17.08829597948888335 ) ) ;
#86127=CARTESIAN_POINT ( 'NONE',  ( 137.8192226437758450, 256.5024278399160380, -9.188101187500093303 ) ) ;
#86128=CARTESIAN_POINT ( 'NONE',  ( 203.1890483204367115, 268.4214926066569546, 2.485490542415017767 ) ) ;
#86130=CARTESIAN_POINT ( 'NONE',  ( 97.82019495012963262, 215.0327760586659451, 1.948934522072303157E-15 ) ) ;
#86132=CARTESIAN_POINT ( 'NONE',  ( 151.4361976351029000, 268.3518069213970421, 15.15218985681980612 ) ) ;
#86133=CARTESIAN_POINT ( 'NONE',  ( 192.1779685593947420, 266.1842805242176269, 11.64530923862864142 ) ) ;
#86134=VERTEX_POINT ( 'NONE', #69370 ) ;
#86136=CARTESIAN_POINT ( 'NONE',  ( 195.5954130450106732, 291.8658022090583017, -15.71558652822518987 ) ) ;
#86137=VERTEX_POINT ( 'NONE', #21290 ) ;
#86141=B_SPLINE_SURFACE_WITH_KNOTS ( 'NONE', 3, 1, ( 
 ( #31484, #92342 ),
 ( #99914, #22401 ),
 ( #62376, #29996 ),
 ( #45193, #39073 ),
 ( #108, #54788 ),
 ( #29505, #60878 ),
 ( #22891, #14797 ),
 ( #23383, #46694 ),
 ( #92832, #16295 ),
 ( #54273, #38076 ),
 ( #85242, #45679 ),
 ( #68989, #8204 ),
 ( #15786, #14307 ),
 ( #600, #61388 ),
 ( #39569, #6707 ),
 ( #52787, #37585 ),
 ( #77619, #53776 ),
 ( #38589, #23886 ),
 ( #93333, #69986 ),
 ( #85767, #47190 ),
 ( #78111, #84739 ),
 ( #8701, #7697 ),
 ( #98927, #60382 ),
 ( #91338, #21898 ),
 ( #83744, #69495 ),
 ( #15280, #46175 ),
 ( #99419, #77095 ),
 ( #71521, #41076 ),
 ( #94833, #40075 ),
 ( #40580, #1107 ),
 ( #78616, #70492 ),
 ( #80645, #25396 ),
 ( #95365, #41586 ),
 ( #25918, #11223 ) ),
 .UNSPECIFIED., .T., .F., .F.,
 ( 4, 2, 2, 2, 2, 2, 2, 2, 2, 2, 2, 2, 2, 2, 2, 2, 4 ),
 ( 2, 2 ),
 ( 0.000000000000000000, 0.06250000000000000000, 0.1250000000000000000, 0.1875000000000000000, 0.2500000000000000000, 0.3125000000000000000, 0.3750000000000000000, 0.4375000000000000000, 0.5000000000000000000, 0.5625000000000000000, 0.6250000000000000000, 0.6875000000000000000, 0.7500000000000000000, 0.8125000000000000000, 0.8750000000000000000, 0.9375000000000000000, 1.000000000000000000 ),
 ( 0.000000000000000000, 1.000000000000000000 ),
 .UNSPECIFIED. ) ;
#86143=CARTESIAN_POINT ( 'NONE',  ( -22.42236680055709641, 157.8615022471902591, 0.000000000000000000 ) ) ;
#86144=CARTESIAN_POINT ( 'NONE',  ( 162.6684717218148251, 248.8969375186720754, 11.76041465758671833 ) ) ;
#86145=CARTESIAN_POINT ( 'NONE',  ( 79.55186417146283873, 225.9244531367911293, -4.594050593750046652 ) ) ;
#86148=CARTESIAN_POINT ( 'NONE',  ( 121.6806519464431773, 234.3927522451418213, 10.00000000000009948 ) ) ;
#86150=CARTESIAN_POINT ( 'NONE',  ( 163.1096928939807924, 248.1327200311062882, -9.690381021358412283 ) ) ;
#86155=CARTESIAN_POINT ( 'NONE',  ( -24.92236680055712839, 162.1916292661124999, 6.123233995736853057E-16 ) ) ;
#86158=CARTESIAN_POINT ( 'NONE',  ( 185.7058167950441145, 259.5999620644902848, 5.848445963200036957 ) ) ;
#86159=CARTESIAN_POINT ( 'NONE',  ( 206.1798448551755598, 273.5330285446045195, -10.53862763475382813 ) ) ;
#86160=CARTESIAN_POINT ( 'NONE',  ( 147.8652489956357101, 275.2099377555215369, -4.764731639000758356 ) ) ;
#86161=CARTESIAN_POINT ( 'NONE',  ( -17.42236680055705023, 149.2012482093457777, 0.000000000000000000 ) ) ;
#86162=CARTESIAN_POINT ( 'NONE',  ( 198.9145269359414669, 284.9342556184034265, -17.40143518274985723 ) ) ;
#86165=CARTESIAN_POINT ( 'NONE',  ( 196.2335616883709122, 265.6660282062799183, 4.428010252653890255 ) ) ;
#86166=CARTESIAN_POINT ( 'NONE',  ( 200.6129772034685175, 283.1751261563724142, 18.36811917402039640 ) ) ;
#86168=CARTESIAN_POINT ( 'NONE',  ( 187.8291388526744186, 266.0904899704142963, -11.84232036284073253 ) ) ;
#86169=CARTESIAN_POINT ( 'NONE',  ( 198.5095674088818782, 266.2393955469675575, 0.9580096654556583546 ) ) ;
#86170=CARTESIAN_POINT ( 'NONE',  ( 153.0105784145868881, 270.8266541147344810, 13.92684810197993350 ) ) ;
#86172=VERTEX_POINT ( 'NONE', #90557 ) ;
#86173=CARTESIAN_POINT ( 'NONE',  ( 162.6264071486809542, 248.9697954965390920, 10.36322805486644683 ) ) ;
#86174=CARTESIAN_POINT ( 'NONE',  ( 207.3502731283117555, 271.5057873089173768, 6.280625384230454245 ) ) ;
#86177=CARTESIAN_POINT ( 'NONE',  ( 186.8123841630082040, 258.3999256946553942, 3.104652050626591553 ) ) ;
#86179=CARTESIAN_POINT ( 'NONE',  ( 171.4574563581475388, 274.7666223272099160, 17.16070901681419514 ) ) ;
#86180=CARTESIAN_POINT ( 'NONE',  ( 164.2119285677552796, 284.2824924003866158, -3.118288404568473560 ) ) ;
#86181=CARTESIAN_POINT ( 'NONE',  ( 124.7815979145579632, 254.3967562850346553, -4.648177544792955347E-16 ) ) ;
#86182=CARTESIAN_POINT ( 'NONE',  ( 188.2791287928231156, 260.8518096374758102, 2.898815310248603172 ) ) ;
#86184=CARTESIAN_POINT ( 'NONE',  ( 3.504529045289348055, 163.6423013555410080, -4.594050593750043987 ) ) ;
#86186=CARTESIAN_POINT ( 'NONE',  ( 174.8738442610398067, 255.2983538659211433, 8.879037836851004784 ) ) ;
#86187=CARTESIAN_POINT ( 'NONE',  ( 180.7942833579522812, 266.7097690628117448, -16.23795806611159520 ) ) ;
#86188=CARTESIAN_POINT ( 'NONE',  ( 189.4308808934198680, 289.8491723414206831, 15.72891001903047048 ) ) ;
#86190=CARTESIAN_POINT ( 'NONE',  ( 24.31594170816038059, 184.8458772461660544, 9.188101187500095079 ) ) ;
#86195=CARTESIAN_POINT ( 'NONE',  ( 147.0660117096331874, 275.9211909828330249, -0.7354350123930680772 ) ) ;
#86199=CARTESIAN_POINT ( 'NONE',  ( 70.67536410627006660, 211.6115022471902591, 10.00000000000009592 ) ) ;
#86200=CARTESIAN_POINT ( 'NONE',  ( 165.4315485841760278, 245.8874648686309854, 0.7284626796912114788 ) ) ;
#86201=CARTESIAN_POINT ( 'NONE',  ( 203.3725525628211699, 270.0917528869257467, 6.095119953602265106 ) ) ;
#86202=CARTESIAN_POINT ( 'NONE',  ( 37.30632276492696064, 192.3458772461660544, 9.188101187500095079 ) ) ;
#86205=CARTESIAN_POINT ( 'NONE',  ( 206.3592393881182545, 269.7258222359968158, -3.299573838669981551 ) ) ;
#86206=B_SPLINE_CURVE_WITH_KNOTS ( 'NONE', 3,
 ( #91562, #52524, #14038, #16024 ),
 .UNSPECIFIED., .F., .F.,
 ( 4, 4 ),
 ( 0.001920166038260726462, 0.003922728456736315761 ),
 .UNSPECIFIED. ) ;
#86210=CARTESIAN_POINT ( 'NONE',  ( 202.0661878422603763, 279.1895584290143120, -16.02388874507808225 ) ) ;
#86211=CARTESIAN_POINT ( 'NONE',  ( 205.8195061805951696, 269.6042235147296537, -1.323967559255036175 ) ) ;
#86213=CARTESIAN_POINT ( 'NONE',  ( 202.5245888501533216, 279.8641176599742266, 15.60152447840272494 ) ) ;
#86214=CARTESIAN_POINT ( 'NONE',  ( 149.4965729687386045, 271.7113353911534546, -11.48413836595348059 ) ) ;
#86215=ADVANCED_FACE ( 'NONE', ( #19138 ), #66176, .F. ) ;
#86216=CARTESIAN_POINT ( 'NONE',  ( 186.0519134971170843, 268.1729366909127066, -14.31315269452955441 ) ) ;
#86228=EDGE_LOOP ( 'NONE', ( #7971, #12309, #68246, #2880 ) ) ;
#86236=EDGE_CURVE ( 'NONE', #947, #46582, #5741, .T. ) ;
#86237=CARTESIAN_POINT ( 'NONE',  ( 189.8480911035503880, 301.8204558191226283, -0.8992086515915015399 ) ) ;
#86238=CARTESIAN_POINT ( 'NONE',  ( 184.1636269873439460, 288.8002302501334952, -13.16066999487799372 ) ) ;
#86240=CARTESIAN_POINT ( 'NONE',  ( 172.9438399295877957, 262.8668947608421718, -16.49499919880818766 ) ) ;
#86241=CARTESIAN_POINT ( 'NONE',  ( 162.1853085131137675, 266.5774002991370821, 17.48035941305625940 ) ) ;
#86244=CARTESIAN_POINT ( 'NONE',  ( 159.3169041484411537, 254.7020228407560580, 16.67170756419672628 ) ) ;
#86246=CARTESIAN_POINT ( 'NONE',  ( 55.54680928425421627, 209.0024278399160949, 9.188101187500095079 ) ) ;
#86249=CARTESIAN_POINT ( 'NONE',  ( 150.3470217762446737, 270.2383148473169854, 15.04338213197856078 ) ) ;
#86250=CARTESIAN_POINT ( 'NONE',  ( 173.1064412035568409, 271.2423724309499562, 16.42374108768880347 ) ) ;
#86251=EDGE_LOOP ( 'NONE', ( #2251, #88515, #26641, #51815, #89751, #33983, #24436, #57465, #92453, #47792, #4535, #76235, #86101, #61952, #3017, #45189, #36347, #34815, #39909, #4724, #54231 ) ) ;
#86256=ORIENTED_EDGE ( 'NONE', *, *, #24228, .F. ) ;
#86257=CARTESIAN_POINT ( 'NONE',  ( 172.1481527822565454, 258.6007877254482423, -14.00111594278938298 ) ) ;
#86258=CARTESIAN_POINT ( 'NONE',  ( 157.0906402174166487, 259.4234253662278888, -17.15993715312605516 ) ) ;
#86259=CARTESIAN_POINT ( 'NONE',  ( 161.6127771116929921, 250.7254542206800352, -12.96229604595372464 ) ) ;
#86260=CARTESIAN_POINT ( 'NONE',  ( 192.5551423381268989, 297.1317055421444024, -13.20528585388119858 ) ) ;
#86261=B_SPLINE_CURVE_WITH_KNOTS ( 'NONE', 3,
 ( #82521, #13083, #43943, #31237, #18437, #65513, #34613, #17938, #93071, #23625, #41709, #10829, #54519, #16046, #87892, #96462, #64526, #57406, #46948, #49327, #95483, #56413, #54026, #39322, #84981, #73140, #34131, #85497, #65024, #80266, #79769, #10334, #77865, #26035, #62123, #46428, #15527, #87408, #56906, #72653, #41200, #3248, #77353, #8451, #49818, #7960, #11349, #95970, #70238, #38834, #72138, #80777 ),
 .UNSPECIFIED., .F., .F.,
 ( 4, 2, 2, 2, 2, 2, 2, 2, 2, 2, 2, 2, 2, 2, 2, 2, 2, 2, 2, 2, 2, 2, 2, 2, 2, 4 ),
 ( 0.0003287865336021304915, 0.0007948713104775596231, 0.001027913698915235022, 0.001260956087352910204, 0.001377477281571752024, 0.001493998475790593626, 0.001610519670009435663, 0.001727040864228277482, 0.001960083252665935968, 0.002193125641103594453, 0.002659210417979031987, 0.003125295194854469955, 0.004057464748605345457, 0.004989634302356220526, 0.005455719079231613824, 0.005688761467669310040, 0.005805282661888203251, 0.005863543258997684117, 0.005921803856107164983, 0.005980064453216645849, 0.006038325050326125848, 0.006154846244545025130, 0.006387888632982837572, 0.006853973409858459855, 0.007320058186734081269, 0.007786142963609704419 ),
 .UNSPECIFIED. ) ;
#86262=CARTESIAN_POINT ( 'NONE',  ( 149.5593209768671841, 271.6026526530012575, 11.55487339793564949 ) ) ;
#86263=AXIS2_PLACEMENT_3D ( 'NONE', #63838, #69066, #70958 ) ;
#86264=CARTESIAN_POINT ( 'NONE',  ( 40.00363105557123333, 187.2365022471902023, 10.00000000000009948 ) ) ;
#86265=CARTESIAN_POINT ( 'NONE',  ( 164.2572333502590709, 246.1451216570909253, 2.155809084027023204 ) ) ;
#86267=DIRECTION ( 'NONE',  ( 0.5000000000000048850, -0.8660254037844358210, 0.000000000000000000 ) ) ;
#86269=CARTESIAN_POINT ( 'NONE',  ( 112.6237299221286321, 226.6423013555409796, -4.594050593750043987 ) ) ;
#86270=ORIENTED_EDGE ( 'NONE', *, *, #3737, .T. ) ;
#86271=FACE_OUTER_BOUND ( 'NONE', #11482, .T. ) ;
#86272=ADVANCED_FACE ( 'NONE', ( #7386 ), #84928, .T. ) ;
#86275=CARTESIAN_POINT ( 'NONE',  ( 155.1865148098964937, 261.8560670301561686, -16.99758927948949605 ) ) ;
#86276=CARTESIAN_POINT ( 'NONE',  ( 204.3371846825755824, 276.7246095846310823, 14.72513001683937262 ) ) ;
#86278=CARTESIAN_POINT ( 'NONE',  ( 174.9266790960579954, 252.5411525110792184, 5.174313525909879807 ) ) ;
#86280=CARTESIAN_POINT ( 'NONE',  ( 207.6875671281972870, 270.9215769640275653, -2.211577121115235300 ) ) ;
#86284=CARTESIAN_POINT ( 'NONE',  ( 132.1361044793229951, 247.0958772461660544, -9.188101187500095079 ) ) ;
#86285=CARTESIAN_POINT ( 'NONE',  ( 198.9225589249066957, 286.1030165008847916, -17.03502353404871883 ) ) ;
#86288=CARTESIAN_POINT ( 'NONE',  ( 186.7776399068530395, 297.3129196693114977, 4.679761716601873012 ) ) ;
#86289=CARTESIAN_POINT ( 'NONE',  ( 196.0355168007595523, 291.1035201434990540, 17.55377893960077884 ) ) ;
#86291=CARTESIAN_POINT ( 'NONE',  ( 52.62397354648171444, 207.3149278399161233, 9.188101187500093303 ) ) ;
#86293=ORIENTED_EDGE ( 'NONE', *, *, #37502, .F. ) ;
#86298=CARTESIAN_POINT ( 'NONE',  ( 171.2278541772891742, 259.7605199901955189, 15.25628007220308469 ) ) ;
#86299=CARTESIAN_POINT ( 'NONE',  ( 151.2863714812464764, 278.3609153730897674, -1.671033152792061438 ) ) ;
#86300=CARTESIAN_POINT ( 'NONE',  ( 155.6535436963908694, 261.0471492701456668, -17.87366571046205976 ) ) ;
#86301=CARTESIAN_POINT ( 'NONE',  ( 153.9942695716630965, 269.2746656473301528, -15.26336082132222138 ) ) ;
#86302=CARTESIAN_POINT ( 'NONE',  ( 116.4123307400877820, 248.0177522451419065, 5.000000000000046185 ) ) ;
#86304=VERTEX_POINT ( 'NONE', #38275 ) ;
#86305=CARTESIAN_POINT ( 'NONE',  ( 202.4900219881211854, 279.9239892212719383, 15.63116161057562259 ) ) ;
#86307=CARTESIAN_POINT ( 'NONE',  ( 23.34166312890287998, 184.2833772461660544, -9.188101187500095079 ) ) ;
#86309=CARTESIAN_POINT ( 'NONE',  ( 188.9122134955663910, 290.7695941481946988, -15.11888497690123678 ) ) ;
#86313=CARTESIAN_POINT ( 'NONE',  ( 56.72874666261028409, 196.8927522451418213, 10.00000000000009592 ) ) ;
#86315=CARTESIAN_POINT ( 'NONE',  ( 182.1229068143135237, 256.9979893241743412, 1.317208241454887796 ) ) ;
#86316=CARTESIAN_POINT ( 'NONE',  ( 157.0877926458200307, 258.5629572190321710, -17.40668770468195703 ) ) ;
#86317=CARTESIAN_POINT ( 'NONE',  ( 162.2339947987030087, 251.8158834976649700, -12.96272347646762668 ) ) ;
#86318=VERTEX_POINT ( 'NONE', #68684 ) ;
#86319=( BOUNDED_CURVE ( )  B_SPLINE_CURVE ( 2, ( #99058, #29640, #61012, #7325, #44822, #91469, #84867, #54401, #60513 ),
 .UNSPECIFIED., .F., .T. ) 
 B_SPLINE_CURVE_WITH_KNOTS ( ( 3, 2, 2, 2, 3 ),
 ( 0.8185483870967742437, 0.8198924731182796188, 0.8225806451612903691, 0.8252688172043011194, 0.8266129032258064946 ),
 .UNSPECIFIED. ) 
 CURVE ( )  GEOMETRIC_REPRESENTATION_ITEM ( )  RATIONAL_B_SPLINE_CURVE ( ( 0.9330127018922194093, 0.9330127018922194093, 1.000000000000000000, 0.8660254037844387076, 1.000000000000000000, 0.8660254037844387076, 1.000000000000000000, 0.9330127018922194093, 0.9330127018922194093 ) ) 
 REPRESENTATION_ITEM ( '' )  );
#86320=CARTESIAN_POINT ( 'NONE',  ( 19.14685258109593136, 191.8615022471903160, 5.000000000000046185 ) ) ;
#86322=CARTESIAN_POINT ( 'NONE',  ( 208.3152833949211526, 269.8343404973242059, 2.763633873278860342 ) ) ;
#86323=CARTESIAN_POINT ( 'NONE',  ( -18.01139699756907930, 172.6589784336661637, -6.496448406907675876E-16 ) ) ;
#86325=CARTESIAN_POINT ( 'NONE',  ( 164.4515396538533309, 259.7753611418699506, -16.47110986934525556 ) ) ;
#86326=CARTESIAN_POINT ( 'NONE',  ( 200.0499229738525457, 283.5835379334554887, 16.94138476260983239 ) ) ;
#86327=CARTESIAN_POINT ( 'NONE',  ( 185.7051452101306381, 260.5437674537701014, 6.335629955934896529 ) ) ;
#86328=CARTESIAN_POINT ( 'NONE',  ( 198.2505066714982149, 285.2670451491296149, 0.000000000000000000 ) ) ;
#86329=CARTESIAN_POINT ( 'NONE',  ( 187.1546226255335625, 259.1615550454087042, -2.418851663009157882 ) ) ;
#86332=CARTESIAN_POINT ( 'NONE',  ( 140.8234218128096131, 252.1115022471902591, 10.00000000000009592 ) ) ;
#86333=SHAPE_REPRESENTATION_RELATIONSHIP ( 'NONE' , 'NONE' ,  #88422, #80385 ) ;
#86334=CARTESIAN_POINT ( 'NONE',  ( 180.9635706913343824, 287.0861331774580094, 13.25109203236105060 ) ) ;
#86335=CIRCLE ( 'NONE', #31239, 17.82106496071138935 ) ;
#86336=CARTESIAN_POINT ( 'NONE',  ( 153.2920657472729715, 277.6580568772731112, -5.533179900162121356 ) ) ;
#86338=CARTESIAN_POINT ( 'NONE',  ( 69.30415721694468800, 217.4865022471902876, -10.00000000000009592 ) ) ;
#86340=CARTESIAN_POINT ( 'NONE',  ( 159.9894443651313338, 253.5371490153152081, -16.36035038356864391 ) ) ;
#86342=LINE ( 'NONE', #96424, #35003 ) ;
#86343=EDGE_CURVE ( 'NONE', #96192, #51310, #89250, .T. ) ;
#86344=( BOUNDED_CURVE ( )  B_SPLINE_CURVE ( 2, ( #21702, #52587, #6509, #14606, #46478, #68291, #76419, #6991, #22706 ),
 .UNSPECIFIED., .F., .T. ) 
 B_SPLINE_CURVE_WITH_KNOTS ( ( 3, 2, 2, 2, 3 ),
 ( 0.7217741935483871218, 0.7231182795698924970, 0.7258064516129032473, 0.7284946236559139976, 0.7298387096774193727 ),
 .UNSPECIFIED. ) 
 CURVE ( )  GEOMETRIC_REPRESENTATION_ITEM ( )  RATIONAL_B_SPLINE_CURVE ( ( 0.9330127018922194093, 0.9330127018922194093, 1.000000000000000000, 0.8660254037844387076, 1.000000000000000000, 0.8660254037844387076, 1.000000000000000000, 0.9330127018922194093, 0.9330127018922194093 ) ) 
 REPRESENTATION_ITEM ( '' )  );
#86345=FACE_OUTER_BOUND ( 'NONE', #44550, .T. ) ;
#86348=CARTESIAN_POINT ( 'NONE',  ( 163.4084407101100851, 247.6152736349200438, -10.68829614238923931 ) ) ;
#86349=FACE_OUTER_BOUND ( 'NONE', #11911, .T. ) ;
#86350=ORIENTED_EDGE ( 'NONE', *, *, #42979, .F. ) ;
#86352=CARTESIAN_POINT ( 'NONE',  ( 157.2692844204907203, 277.2926557658657316, -9.947913950199314570 ) ) ;
#86358=VERTEX_POINT ( 'NONE', #83942 ) ;
#86359=EDGE_CURVE ( 'NONE', #56647, #44553, #97643, .T. ) ;
#86360=CARTESIAN_POINT ( 'NONE',  ( -22.42236680055709641, 157.8615022471902591, 0.000000000000000000 ) ) ;
#86364=VERTEX_POINT ( 'NONE', #26104 ) ;
#86365=CARTESIAN_POINT ( 'NONE',  ( 203.6224643629829529, 277.9625414913675172, 16.18209619002064414 ) ) ;
#86366=CARTESIAN_POINT ( 'NONE',  ( 151.4281781455628675, 268.3656970847310390, 15.24742929158552585 ) ) ;
#86367=CARTESIAN_POINT ( 'NONE',  ( 179.5196496019146650, 266.1175816663657656, 16.29367087753972498 ) ) ;
#86368=B_SPLINE_SURFACE_WITH_KNOTS ( 'NONE', 3, 1, ( 
 ( #27721, #91046 ),
 ( #91535, #89562 ),
 ( #44886, #52007 ),
 ( #22099, #29702 ),
 ( #50996, #35304 ),
 ( #67707, #74339 ),
 ( #12525, #5415 ),
 ( #68191, #52493 ),
 ( #36795, #82950 ),
 ( #81452, #20620 ),
 ( #6413, #90048 ),
 ( #99120, #81947 ),
 ( #4408, #60579 ),
 ( #60083, #12024 ),
 ( #43396, #58589 ),
 ( #4928, #35807 ),
 ( #66701, #43895 ),
 ( #44391, #98634 ),
 ( #97636, #28201 ),
 ( #37294, #21130 ),
 ( #13523, #59077 ),
 ( #21613, #51504 ),
 ( #83441, #82471 ),
 ( #59585, #13033 ),
 ( #14008, #42880 ),
 ( #73816, #74835 ),
 ( #36298, #67201 ),
 ( #98123, #90561 ),
 ( #62573, #78312 ),
 ( #76796, #45872 ),
 ( #30704, #54987 ),
 ( #93021, #63091 ),
 ( #14985, #23577 ),
 ( #8400, #1306 ) ),
 .UNSPECIFIED., .T., .F., .F.,
 ( 4, 2, 2, 2, 2, 2, 2, 2, 2, 2, 2, 2, 2, 2, 2, 2, 4 ),
 ( 2, 2 ),
 ( 0.000000000000000000, 0.06250000000000000000, 0.1250000000000000000, 0.1875000000000000000, 0.2500000000000000000, 0.3125000000000000000, 0.3750000000000000000, 0.4375000000000000000, 0.5000000000000000000, 0.5625000000000000000, 0.6250000000000000000, 0.6875000000000000000, 0.7500000000000000000, 0.8125000000000000000, 0.8750000000000000000, 0.9375000000000000000, 1.000000000000000000 ),
 ( 0.000000000000000000, 1.000000000000000000 ),
 .UNSPECIFIED. ) ;
#86372=ORIENTED_EDGE ( 'NONE', *, *, #64947, .F. ) ;
#86373=ADVANCED_FACE ( 'NONE', ( #94530 ), #55963, .T. ) ;
#86381=CARTESIAN_POINT ( 'NONE',  ( 194.9455394410084921, 292.9914163096879065, -15.01116663483170655 ) ) ;
#86383=CYLINDRICAL_SURFACE ( 'NONE', #2998, 17.82106496071139645 ) ;
#86386=CARTESIAN_POINT ( 'NONE',  ( 206.3505875407052486, 273.2372935382459787, 11.62318091048137880 ) ) ;
#86387=FACE_OUTER_BOUND ( 'NONE', #80892, .T. ) ;
#86388=CARTESIAN_POINT ( 'NONE',  ( 197.9002057575219453, 287.8737841300738296, 18.01270164875645818 ) ) ;
#86390=CARTESIAN_POINT ( 'NONE',  ( 146.7742226592052361, 276.4265844432662220, -3.920976060369687932 ) ) ;
#86391=EDGE_CURVE ( 'NONE', #77284, #53616, #11793, .T. ) ;
#86392=DIRECTION ( 'NONE',  ( 0.8660254037844395958, 0.4999999999999985567, 0.000000000000000000 ) ) ;
#86393=CARTESIAN_POINT ( 'NONE',  ( 159.2394649670193303, 254.8361514374751664, -16.43133403737800791 ) ) ;
#86396=CARTESIAN_POINT ( 'NONE',  ( 137.2172943591538967, 238.4824982072973967, 3.021315404115420679E-15 ) ) ;
#86397=CARTESIAN_POINT ( 'NONE',  ( 191.9661401536347114, 262.6107830541747035, -0.7521427156081436083 ) ) ;
#86398=CARTESIAN_POINT ( 'NONE',  ( 193.8979767073725498, 294.8058481884610273, -15.36728096558731593 ) ) ;
#86399=EDGE_CURVE ( 'NONE', #12659, #31705, #16606, .T. ) ;
#86400=CYLINDRICAL_SURFACE ( 'NONE', #46301, 17.82106496071139645 ) ;
#86401=CARTESIAN_POINT ( 'NONE',  ( 164.9586510554008782, 244.9302305544571823, -1.717556444319656039 ) ) ;
#86402=CARTESIAN_POINT ( 'NONE',  ( 10.68506269473756909, 183.6427522451419634, -10.00000000000009415 ) ) ;
#86403=CARTESIAN_POINT ( 'NONE',  ( 82.25819355828922141, 227.4869531367911293, 4.594050593750046652 ) ) ;
#86404=B_SPLINE_CURVE_WITH_KNOTS ( 'NONE', 3,
 ( #7813, #38698, #61981, #92935 ),
 .UNSPECIFIED., .F., .F.,
 ( 4, 4 ),
 ( 0.01353903641422806066, 0.01992619949220648598 ),
 .UNSPECIFIED. ) ;
#86406=ADVANCED_FACE ( 'NONE', ( #96043 ), #66986, .F. ) ;
#86408=CARTESIAN_POINT ( 'NONE',  ( 167.0544376998900589, 277.9796431053840138, -13.80256916416768931 ) ) ;
#86409=CARTESIAN_POINT ( 'NONE',  ( 6.887527552763561545, 162.5327760586659736, 1.948934522072303157E-15 ) ) ;
#86413=CARTESIAN_POINT ( 'NONE',  ( 161.3193951073452581, 251.2336067582368742, 13.01220207292984377 ) ) ;
#86416=EDGE_CURVE ( 'NONE', #22170, #24654, #93991, .T. ) ;
#86418=CARTESIAN_POINT ( 'NONE',  ( 188.7890919132309762, 261.5044042730166893, -5.996600600795340519 ) ) ;
#86425=CARTESIAN_POINT ( 'NONE',  ( 31.65035466828360100, 179.8923013555409796, 4.594050593750050204 ) ) ;
#86426=CARTESIAN_POINT ( 'NONE',  ( 74.41009865654250177, 223.7677522451419350, -5.000000000000047962 ) ) ;
#86427=CARTESIAN_POINT ( 'NONE',  ( 199.5527968932103704, 277.4168076600803374, 15.13942517218949213 ) ) ;
#86429=CARTESIAN_POINT ( 'NONE',  ( 26.50806851326365532, 196.1115022471903160, -5.000000000000047962 ) ) ;
#86431=DIRECTION ( 'NONE',  ( -0.8660254037844359321, -0.5000000000000051070, -0.000000000000000000 ) ) ;
#86432=CARTESIAN_POINT ( 'NONE',  ( -16.14394294671762253, 170.6744531367911293, 4.594050593750047540 ) ) ;
#86433=CARTESIAN_POINT ( 'NONE',  ( 195.7291850945597957, 291.6341022226063160, 17.08310330964873813 ) ) ;
#86434=CARTESIAN_POINT ( 'NONE',  ( 155.5770330754656072, 261.1796695529068302, 18.26969263326161297 ) ) ;
#86435=CARTESIAN_POINT ( 'NONE',  ( 179.4037581149374034, 257.9870511612666064, -10.76565914641300736 ) ) ;
#86437=CARTESIAN_POINT ( 'NONE',  ( 147.9311236323648870, 274.4227731784279172, -7.799459659034405412 ) ) ;
#86438=CARTESIAN_POINT ( 'NONE',  ( 189.4875514829830081, 262.4673988887644214, 8.218528321876050313 ) ) ;
#86439=CARTESIAN_POINT ( 'NONE',  ( 204.7235752877335244, 276.0553614249301972, 14.82397698933823271 ) ) ;
#86440=CARTESIAN_POINT ( 'NONE',  ( 192.5184197856564765, 265.2800136393148591, 8.105435529764278613 ) ) ;
#86441=CARTESIAN_POINT ( 'NONE',  ( 146.5310397537613483, 276.8477895910274356, -0.2793038414862049068 ) ) ;
#86442=CARTESIAN_POINT ( 'NONE',  ( 190.5674408456512765, 300.5745055173924811, -0.9151048603553563199 ) ) ;
#86444=B_SPLINE_CURVE_WITH_KNOTS ( 'NONE', 3,
 ( #8480, #873, #7468, #31752 ),
 .UNSPECIFIED., .F., .F.,
 ( 4, 4 ),
 ( 0.01090216205137726352, 0.01663243029966742295 ),
 .UNSPECIFIED. ) ;
#86446=CARTESIAN_POINT ( 'NONE',  ( 208.2175703429120688, 270.0035844679667889, 2.257951022351344150 ) ) ;
#86447=CARTESIAN_POINT ( 'NONE',  ( 143.9908900580791169, 242.3932355074535394, -2.679491924311248496 ) ) ;
#86448=CARTESIAN_POINT ( 'NONE',  ( 114.1121243109418799, 230.5643266524159856, -9.188101187500093303 ) ) ;
#86450=CARTESIAN_POINT ( 'NONE',  ( -15.63054290230554955, 173.3297689869269504, -2.679491924311249385 ) ) ;
#86452=CARTESIAN_POINT ( 'NONE',  ( 176.9880447955025602, 255.7295297668954959, 9.707864002611934495 ) ) ;
#86453=CARTESIAN_POINT ( 'NONE',  ( 191.7796050947615925, 276.9574050642111160, 17.17898019043861169 ) ) ;
#86454=B_SPLINE_CURVE_WITH_KNOTS ( 'NONE', 3,
 ( #13583, #5971, #45454, #22675 ),
 .UNSPECIFIED., .F., .F.,
 ( 4, 4 ),
 ( 0.006529893551346395777, 0.01223971033066661822 ),
 .UNSPECIFIED. ) ;
#86455=CARTESIAN_POINT ( 'NONE',  ( 190.9361477708944506, 299.9358863897686547, -8.027914178803371215 ) ) ;
#86456=CARTESIAN_POINT ( 'NONE',  ( 189.6941666366152219, 261.1016796491359742, -4.547171728000958701 ) ) ;
#86457=CARTESIAN_POINT ( 'NONE',  ( 149.2593905435863348, 272.1221474021800759, -12.98626158366800176 ) ) ;
#86458=CARTESIAN_POINT ( 'NONE',  ( 91.02696109520442747, 213.3615022471902023, 5.000000000000051514 ) ) ;
#86459=CARTESIAN_POINT ( 'NONE',  ( 175.3706562369355595, 291.2152232206044573, -1.076157994416038877 ) ) ;
#86462=CARTESIAN_POINT ( 'NONE',  ( 131.5677753063154682, 256.7677522451419350, -5.000000000000047962 ) ) ;
#86464=CARTESIAN_POINT ( 'NONE',  ( 200.5678471034125891, 269.1112160442550021, 9.133758541397122954 ) ) ;
#86470=CARTESIAN_POINT ( 'NONE',  ( 153.4477557824949940, 264.8676860077344486, 17.16010094972647693 ) ) ;
#86472=CARTESIAN_POINT ( 'NONE',  ( 191.1408708152463873, 280.4011667686116311, 16.85908246009275402 ) ) ;
#86476=CARTESIAN_POINT ( 'NONE',  ( 166.4682810119589362, 280.3365465379465604, 11.69032492195255202 ) ) ;
#86483=CARTESIAN_POINT ( 'NONE',  ( 204.8523313866422484, 275.8323493198358847, 14.65426965484541100 ) ) ;
#86486=CARTESIAN_POINT ( 'NONE',  ( 24.70930941448223450, 196.6199935810941213, 2.679491924311251605 ) ) ;
#86489=ORIENTED_EDGE ( 'NONE', *, *, #43812, .F. ) ;
#86490=CARTESIAN_POINT ( 'NONE',  ( 162.7457592588995396, 249.1791651530724039, 10.37923698128102856 ) ) ;
#86495=DIRECTION ( 'NONE',  ( -0.8660254037844387076, -0.4999999999999998890, -0.000000000000000000 ) ) ;
#86497=ORIENTED_EDGE ( 'NONE', *, *, #72885, .T. ) ;
#86498=CARTESIAN_POINT ( 'NONE',  ( 186.1746999497612762, 282.5091972200996224, -17.01259697921864245 ) ) ;
#86499=CARTESIAN_POINT ( 'NONE',  ( 206.7156906810202770, 272.6049163492177740, -10.59685249612386571 ) ) ;
#86500=CARTESIAN_POINT ( 'NONE',  ( 147.8139399455021135, 274.6257412778925300, -6.037782032743958638 ) ) ;
#86501=CARTESIAN_POINT ( 'NONE',  ( 196.0478384692391671, 284.4236576599464001, -17.70377088038400615 ) ) ;
#86503=CARTESIAN_POINT ( 'NONE',  ( 167.6519984660217517, 249.1525439965649298, -5.333742874422932267 ) ) ;
#86506=CARTESIAN_POINT ( 'NONE',  ( 157.9092491340927893, 281.1234455293418364, 2.649512146863262974 ) ) ;
#86507=CARTESIAN_POINT ( 'NONE',  ( 128.5905526607566856, 254.2369531367911293, -4.594050593750048428 ) ) ;
#86508=CARTESIAN_POINT ( 'NONE',  ( 186.6466061793297513, 262.7878478665138005, -9.097244108367178228 ) ) ;
#86511=ORIENTED_EDGE ( 'NONE', *, *, #21292, .T. ) ;
#86512=CARTESIAN_POINT ( 'NONE',  ( 200.6029011850095003, 274.3471715891406006, 13.46761961965223264 ) ) ;
#86514=CARTESIAN_POINT ( 'NONE',  ( 174.3091936542869291, 290.3603755278153358, -4.810639208511179099 ) ) ;
#86515=CARTESIAN_POINT ( 'NONE',  ( 147.0544566641476933, 275.9412049086974434, 4.176647824200751202 ) ) ;
#86519=CARTESIAN_POINT ( 'NONE',  ( 174.9674570703506049, 282.3531941054687309, 14.48823916692557923 ) ) ;
#86522=CARTESIAN_POINT ( 'NONE',  ( 194.3541845315608612, 294.0156730581561533, -14.67567721756631016 ) ) ;
#86524=CARTESIAN_POINT ( 'NONE',  ( 151.8899205101083965, 272.8516340236540145, 11.76015270370216470 ) ) ;
#86525=VERTEX_POINT ( 'NONE', #31063 ) ;
#86526=CARTESIAN_POINT ( 'NONE',  ( 188.4443801593399144, 265.3218929820331482, -11.72523327534011806 ) ) ;
#86527=EDGE_CURVE ( 'NONE', #7170, #57805, #75858, .T. ) ;
#86528=CARTESIAN_POINT ( 'NONE',  ( 160.1932291396877588, 279.1613061217781819, 10.72099505396529473 ) ) ;
#86529=CARTESIAN_POINT ( 'NONE',  ( 191.7401253710455364, 298.5433563381600948, -10.97067107967070143 ) ) ;
#86532=CARTESIAN_POINT ( 'NONE',  ( 161.4380241112732222, 281.4543506753062729, -6.652507061251734299 ) ) ;
#86533=CARTESIAN_POINT ( 'NONE',  ( 153.2619048262327794, 276.0433244632241667, -8.635578536908909086 ) ) ;
#86534=CARTESIAN_POINT ( 'NONE',  ( 200.2419102918539693, 267.3236120580114630, 6.328608526495528075 ) ) ;
#86535=ORIENTED_EDGE ( 'NONE', *, *, #98017, .T. ) ;
#86536=CARTESIAN_POINT ( 'NONE',  ( 204.8980137558721708, 272.5951782074533298, -9.440052061925650051 ) ) ;
#86537=CARTESIAN_POINT ( 'NONE',  ( 186.8629439719893810, 262.8562446410389271, -9.020214349775766749 ) ) ;
#86538=EDGE_CURVE ( 'NONE', #26620, #69871, #32721, .T. ) ;
#86539=CARTESIAN_POINT ( 'NONE',  ( 190.4156752604778262, 274.6247770965693462, -15.68896343351512002 ) ) ;
#86540=DIRECTION ( 'NONE',  ( -0.8660254037844359321, -0.5000000000000051070, -0.000000000000000000 ) ) ;
#86541=CARTESIAN_POINT ( 'NONE',  ( 188.3939850883347162, 298.9566551310053342, -3.737861235791795522 ) ) ;
#86542=CARTESIAN_POINT ( 'NONE',  ( 152.7618747630824885, 266.0556667813044101, 16.41480086888796919 ) ) ;
#86543=CARTESIAN_POINT ( 'NONE',  ( -17.42236680055705023, 149.2012482093457777, 0.000000000000000000 ) ) ;
#86546=CARTESIAN_POINT ( 'NONE',  ( -11.38080322590321281, 173.4244531367911293, -4.594050593750046652 ) ) ;
#86547=CARTESIAN_POINT ( 'NONE',  ( 85.37073267496330686, 220.0958772461660544, -9.188101187500095079 ) ) ;
#86548=CARTESIAN_POINT ( 'NONE',  ( 155.5066938333533528, 261.3015006940112244, -18.40036130547566273 ) ) ;
#86550=CARTESIAN_POINT ( 'NONE',  ( 147.7312888952508843, 275.3791301261515514, 3.813061375158469435 ) ) ;
#86551=CARTESIAN_POINT ( 'NONE',  ( 202.9881971861223917, 279.0611244672630278, -15.16231470264511927 ) ) ;
#86552=DIRECTION ( 'NONE',  ( 0.4999999999999992784, -0.8660254037844390407, 0.000000000000000000 ) ) ;
#86555=CARTESIAN_POINT ( 'NONE',  ( 190.3036138866188196, 300.4162036267649682, -1.111846361930479254 ) ) ;
#86557=CARTESIAN_POINT ( 'NONE',  ( 162.0307665587793338, 250.0014752612991913, 13.21085648779418698 ) ) ;
#86558=CARTESIAN_POINT ( 'NONE',  ( 169.3360775606673485, 252.0299813709655439, -9.733642257039461398 ) ) ;
#86559=CARTESIAN_POINT ( 'NONE',  ( 157.6286460899086137, 257.6261715744221306, 18.25526781158026779 ) ) ;
#86562=CARTESIAN_POINT ( 'NONE',  ( 161.5083988044524119, 250.9062427520286178, -14.53522982831775856 ) ) ;
#86563=CARTESIAN_POINT ( 'NONE',  ( 36.49425040099653472, 198.0024278399160949, -9.188101187500093303 ) ) ;
#86564=EDGE_CURVE ( 'NONE', #74259, #57797, #66144, .T. ) ;
#86565=CARTESIAN_POINT ( 'NONE',  ( 62.47501251452968773, 213.0024278399160949, -9.188101187500093303 ) ) ;
#86569=CARTESIAN_POINT ( 'NONE',  ( 182.0338464029501040, 278.3680066549227945, 17.69288446120480174 ) ) ;
#86570=FACE_OUTER_BOUND ( 'NONE', #51464, .T. ) ;
#86571=CARTESIAN_POINT ( 'NONE',  ( 196.2376815664581500, 269.5000789340413689, -10.77412858023367370 ) ) ;
#86573=CARTESIAN_POINT ( 'NONE',  ( 151.0388915836658725, 269.0399611886400635, -14.24896787280406585 ) ) ;
#86576=CARTESIAN_POINT ( 'NONE',  ( 66.15596757637857195, 202.8768266524160140, 9.188101187500096856 ) ) ;
#86579=CARTESIAN_POINT ( 'NONE',  ( 197.9002057575219453, 287.8737841300738296, 18.01270164875645818 ) ) ;
#86581=CARTESIAN_POINT ( 'NONE',  ( 154.0911303478728769, 263.7533285722025767, 17.04017818173372945 ) ) ;
#86582=B_SPLINE_CURVE_WITH_KNOTS ( 'NONE', 3,
 ( #32153, #63060, #94003, #92987, #47838, #54432, #63558, #94497, #85407, #2283, #18988, #95528, #19499, #11879, #96504, #49858, #66060, #97010, #48876, #17982, #64065, #81308, #26073, #10874, #40742, #79811, #65062, #10375, #87449, #50848, #88428, #87935, #49364, #4253, #27578, #34170, #88939, #42735, #50353, #80824, #96012, #80308, #41752, #41245, #11393, #71687, #65556, #73672 ),
 .UNSPECIFIED., .F., .F.,
 ( 4, 2, 2, 2, 2, 2, 2, 2, 2, 2, 2, 2, 2, 2, 2, 2, 2, 2, 2, 2, 2, 2, 2, 4 ),
 ( 0.0004679476576457052245, 0.0009134075131973231568, 0.001136137440973158334, 0.001247502404861099016, 0.001358867368749039697, 0.001470232332636980379, 0.001581597296524921061, 0.001804327224300763394, 0.002249787079852291066, 0.003140706790955346411, 0.004031626502058401756, 0.004922546213161457102, 0.005368006068713020336, 0.005590735996488724324, 0.005702100960376499557, 0.005757783442320386739, 0.005813465924264273922, 0.005869148406208161972, 0.005924830888152049155, 0.006036195852039825255, 0.006258925779815422558, 0.006704385635366572060, 0.007149845490917722431, 0.007595305346468871933 ),
 .UNSPECIFIED. ) ;
#86583=CARTESIAN_POINT ( 'NONE',  ( 193.7599675174199660, 288.1895609423694964, 16.30602659942787369 ) ) ;
#86585=CARTESIAN_POINT ( 'NONE',  ( 109.6465072765698210, 234.1115022471902307, 10.00000000000009592 ) ) ;
#86587=CARTESIAN_POINT ( 'NONE',  ( 207.2824254892180704, 271.6233028670009162, 6.274396967990798046 ) ) ;
#86590=CARTESIAN_POINT ( 'NONE',  ( 184.6787335681921718, 271.1592666014827842, 16.29185237002324982 ) ) ;
#86591=ORIENTED_EDGE ( 'NONE', *, *, #40211, .T. ) ;
#86592=CARTESIAN_POINT ( 'NONE',  ( 206.8313602288537538, 272.4045708154811791, -9.607337080360906612 ) ) ;
#86595=EDGE_LOOP ( 'NONE', ( #49358, #26917, #91607, #52891 ) ) ;
#86596=CARTESIAN_POINT ( 'NONE',  ( 176.9944672240674777, 253.3095680353166870, -0.2591140802082422812 ) ) ;
#86600=CARTESIAN_POINT ( 'NONE',  ( 51.48077938449444702, 188.9824982072973967, 3.021315404115420679E-15 ) ) ;
#86601=CARTESIAN_POINT ( 'NONE',  ( 206.8532690132467451, 270.9563895460929643, -5.334349829856665615 ) ) ;
#86610=CARTESIAN_POINT ( 'NONE',  ( 206.3423291502491566, 273.2515974901050413, -10.76717883871977577 ) ) ;
#86611=ADVANCED_FACE ( 'NONE', ( #2694 ), #71097, .T. ) ;
#86612=ORIENTED_EDGE ( 'NONE', *, *, #54579, .T. ) ;
#86613=CARTESIAN_POINT ( 'NONE',  ( 183.7135354246354666, 296.1227231308993169, 1.015274712648644106 ) ) ;
#86614=CARTESIAN_POINT ( 'NONE',  ( 162.6361072964105006, 284.9137001060370835, -2.721021406022150479 ) ) ;
#86615=CARTESIAN_POINT ( 'NONE',  ( 194.4826705584825390, 293.7931287314651740, -16.11258321617245315 ) ) ;
#86616=CARTESIAN_POINT ( 'NONE',  ( 170.6178593158246315, 266.5408558992322696, -17.65857870869936974 ) ) ;
#86617=CARTESIAN_POINT ( 'NONE',  ( 155.3738696901333469, 261.5315588585399951, 17.02116401938635804 ) ) ;
#86618=CARTESIAN_POINT ( 'NONE',  ( 185.8238740079479214, 292.8821648394323915, -10.72204040993758234 ) ) ;
#86619=CARTESIAN_POINT ( 'NONE',  ( 205.3943609285979051, 274.8935266139653777, -13.14270440534009943 ) ) ;
#86620=CARTESIAN_POINT ( 'NONE',  ( 144.0260350180681712, 257.5444598644534153, -9.188101187500093303 ) ) ;
#86623=CARTESIAN_POINT ( 'NONE',  ( 82.77265646360999085, 218.5958772461660544, -9.188101187500095079 ) ) ;
#86624=ORIENTED_EDGE ( 'NONE', *, *, #38296, .F. ) ;
#86625=CARTESIAN_POINT ( 'NONE',  ( 150.8888667059421209, 269.2998118992572927, 15.79021133717968617 ) ) ;
#86628=CARTESIAN_POINT ( 'NONE',  ( 157.4810658944377906, 257.8817879711681940, -17.75031495925077962 ) ) ;
#86629=ORIENTED_EDGE ( 'NONE', *, *, #44612, .T. ) ;
#86630=FACE_OUTER_BOUND ( 'NONE', #39815, .T. ) ;
#86631=CARTESIAN_POINT ( 'NONE',  ( 84.11911179316838627, 207.8262482093457777, 3.021315404115420679E-15 ) ) ;
#86632=CARTESIAN_POINT ( 'NONE',  ( 146.5689048584090699, 276.7822053059436485, -0.4306668706573002492 ) ) ;
#86635=CARTESIAN_POINT ( 'NONE',  ( 162.7896496350696225, 248.6870512161599436, 11.81710663537990946 ) ) ;
#86636=CARTESIAN_POINT ( 'NONE',  ( 82.06918437091763963, 212.0643266524160140, 9.188101187500095079 ) ) ;
#86641=CARTESIAN_POINT ( 'NONE',  ( 124.2269133023873025, 230.9824982072973683, 3.021315404115420679E-15 ) ) ;
#86643=CARTESIAN_POINT ( 'NONE',  ( 163.4139553296302267, 247.6057220337265505, -10.31482883765270842 ) ) ;
#86644=ORIENTED_EDGE ( 'NONE', *, *, #73514, .F. ) ;
#86647=CARTESIAN_POINT ( 'NONE',  ( 164.3400821678858392, 284.7095078879949028, 0.5037811400987294297 ) ) ;
#86652=CARTESIAN_POINT ( 'NONE',  ( 186.0084645542806072, 259.0743807822461804, 6.274839502105399980 ) ) ;
#86653=CARTESIAN_POINT ( 'NONE',  ( 159.2289198208967775, 254.8544161663325838, -15.88961297684315888 ) ) ;
#86654=CARTESIAN_POINT ( 'NONE',  ( 147.7917198021585534, 275.6304213403500398, -3.790807063116589770 ) ) ;
#86656=CARTESIAN_POINT ( 'NONE',  ( 198.8472775862647666, 285.8620616674365920, -17.00592469681938823 ) ) ;
#86658=VERTEX_POINT ( 'NONE', #2194 ) ;
#86659=CARTESIAN_POINT ( 'NONE',  ( 203.4594108534527095, 277.8640620765348785, -14.42658014575316550 ) ) ;
#86660=CARTESIAN_POINT ( 'NONE',  ( 200.4592688079413847, 283.4413569069752725, 18.39277739746426832 ) ) ;
#86662=CARTESIAN_POINT ( 'NONE',  ( 187.8939482297251686, 266.1432077329668573, -11.85658473688042136 ) ) ;
#86664=CARTESIAN_POINT ( 'NONE',  ( 175.6661633239287994, 291.2999147521263126, -6.611607887066273115 ) ) ;
#86665=CARTESIAN_POINT ( 'NONE',  ( 156.6090548319399431, 272.6926376298130208, 14.76279018684578759 ) ) ;
#86666=ORIENTED_EDGE ( 'NONE', *, *, #65844, .T. ) ;
#86669=CARTESIAN_POINT ( 'NONE',  ( 180.5624607037953808, 267.1083404837390276, -14.97454804253810146 ) ) ;
#86671=CARTESIAN_POINT ( 'NONE',  ( 176.1878285045740711, 285.1602639758941677, -12.77100825351733349 ) ) ;
#86672=B_SPLINE_CURVE_WITH_KNOTS ( 'NONE', 3,
 ( #8722, #68518, #60401, #99440, #31504, #45702, #31012, #39593, #45215, #92363, #61902, #54811, #7718, #62399, #76154, #47212, #92852, #23405, #85264, #91865, #6729, #91357, #15809, #7212, #21921, #85788, #46714, #77642, #16320, #22910, #38096, #76626, #53797, #14815, #84760, #8226, #83766, #39095, #37606, #52809, #38610, #30017, #70008, #22422, #53313, #84269, #77113, #69007, #99937, #15297, #46197, #72549 ),
 .UNSPECIFIED., .F., .F.,
 ( 4, 2, 2, 2, 2, 2, 2, 2, 2, 2, 2, 2, 2, 2, 2, 2, 2, 2, 2, 2, 2, 2, 2, 2, 2, 4 ),
 ( 0.0001379551026079702870, 0.001154483995626299489, 0.001408616218880838055, 0.001662748442135376838, 0.001789814553762667480, 0.001916880665389957689, 0.002043946777017248331, 0.002171012888644538973, 0.002425145111899041327, 0.002679277335153543247, 0.003187541781662507623, 0.004204070674680569081, 0.005220599567698630539, 0.005728864014207661268, 0.005982996237462099437, 0.006110062349089359288, 0.006237128460716620006, 0.006300661516530249931, 0.006364194572343878989, 0.006491260683971138840, 0.006745392907225655939, 0.007253657353734690137, 0.007507789576989207236, 0.007761921800243724336, 0.008016054023498243170, 0.008270186246752759401 ),
 .UNSPECIFIED. ) ;
#86675=CARTESIAN_POINT ( 'NONE',  ( 179.7803990077309777, 275.4327082817983978, -17.81061729480618183 ) ) ;
#86676=CARTESIAN_POINT ( 'NONE',  ( 192.2502979002084658, 262.0516754426723764, 3.027840789192269177 ) ) ;
#86678=B_SPLINE_CURVE_WITH_KNOTS ( 'NONE', 3,
 ( #9659, #40518, #71453, #41523 ),
 .UNSPECIFIED., .F., .F.,
 ( 4, 4 ),
 ( 0.01371562546018176634, 0.02009222533191522969 ),
 .UNSPECIFIED. ) ;
#86679=CARTESIAN_POINT ( 'NONE',  ( -2.098180203030011182, 181.8464784336661353, 1.353441290958777327E-15 ) ) ;
#86681=ORIENTED_EDGE ( 'NONE', *, *, #12845, .F. ) ;
#86682=CARTESIAN_POINT ( 'NONE',  ( 175.7615011029471646, 255.7341681394030957, 8.240769549146955697 ) ) ;
#86685=CARTESIAN_POINT ( 'NONE',  ( 22.50244069716294959, 192.9869531367911293, 4.594050593750046652 ) ) ;
#86688=CARTESIAN_POINT ( 'NONE',  ( 178.3194579432817193, 291.9759310783170463, 5.627940545170020847 ) ) ;
#86692=CARTESIAN_POINT ( 'NONE',  ( 174.3697573357644899, 277.1653490889620457, -17.12727634137145571 ) ) ;
#86693=CARTESIAN_POINT ( 'NONE',  ( 188.5128844555716796, 297.0448699536724462, -7.768193810651193409 ) ) ;
#86694=CARTESIAN_POINT ( 'NONE',  ( 90.23310447506868570, 216.2365022471901739, -10.00000000000009237 ) ) ;
#86696=CARTESIAN_POINT ( 'NONE',  ( 66.77824978924009258, 209.3615022471902591, -10.00000000000009592 ) ) ;
#86698=CARTESIAN_POINT ( 'NONE',  ( 185.6563202890208970, 277.8056579403244086, -17.21583835310515553 ) ) ;
#86699=CARTESIAN_POINT ( 'NONE',  ( 203.3753004216920885, 270.0891535218205490, 6.082445786454247383 ) ) ;
#86700=CARTESIAN_POINT ( 'NONE',  ( 33.40920844789697952, 190.0958772461660544, -9.188101187500095079 ) ) ;
#86701=CARTESIAN_POINT ( 'NONE',  ( 191.7788397968654408, 282.6077912147245570, 17.79992444728804202 ) ) ;
#86703=CARTESIAN_POINT ( 'NONE',  ( 151.1126408083691501, 268.9122237844355254, -15.82705194100464396 ) ) ;
#86705=VERTEX_POINT ( 'NONE', #48792 ) ;
#86706=CARTESIAN_POINT ( 'NONE',  ( -4.235833321083918079, 178.3615022471903160, 5.000000000000046185 ) ) ;
#86711=CARTESIAN_POINT ( 'NONE',  ( 163.2442700311756596, 247.8996255919473697, 11.14021925110252020 ) ) ;
#86712=CARTESIAN_POINT ( 'NONE',  ( 196.8435556370661459, 289.7039558245273838, -16.43899056939217118 ) ) ;
#86713=CARTESIAN_POINT ( 'NONE',  ( 188.7651867339601210, 270.3529595027822552, -14.65709028123318802 ) ) ;
#86716=B_SPLINE_CURVE_WITH_KNOTS ( 'NONE', 3,
 ( #55556, #87047, #77898, #48487, #23168, #16077 ),
 .UNSPECIFIED., .F., .F.,
 ( 4, 2, 4 ),
 ( 0.02242907851741109126, 0.02703286848893578578, 0.03163665846046048030 ),
 .UNSPECIFIED. ) ;
#86717=CARTESIAN_POINT ( 'NONE',  ( 189.4969062498522305, 299.9520335943911391, 5.037320497423551480 ) ) ;
#86720=ORIENTED_EDGE ( 'NONE', *, *, #63555, .T. ) ;
#86723=EDGE_CURVE ( 'NONE', #10695, #56036, #34737, .T. ) ;
#86726=FACE_OUTER_BOUND ( 'NONE', #13930, .T. ) ;
#86728=ORIENTED_EDGE ( 'NONE', *, *, #18526, .T. ) ;
#86730=CARTESIAN_POINT ( 'NONE',  ( 189.6824569201680788, 274.2416051070018739, -15.66895928228713863 ) ) ;
#86733=CARTESIAN_POINT ( 'NONE',  ( 200.8251833487811666, 282.8075743310126882, -16.74393672780000131 ) ) ;
#86734=EDGE_CURVE ( 'NONE', #22875, #94946, #85568, .T. ) ;
#86735=CARTESIAN_POINT ( 'NONE',  ( 168.0462690533684338, 251.4142709888886884, 10.74789308012043954 ) ) ;
#86738=CARTESIAN_POINT ( 'NONE',  ( 165.1533192291969954, 284.0593027945823792, 8.797467712081603608 ) ) ;
#86740=CARTESIAN_POINT ( 'NONE',  ( 102.8537940617441819, 224.0643266524160140, 9.188101187500095079 ) ) ;
#86741=CARTESIAN_POINT ( 'NONE',  ( 149.0203866098534888, 272.5361143586139860, -12.73049804737905255 ) ) ;
#86742=CARTESIAN_POINT ( 'NONE',  ( 183.5196873229465950, 288.4008142763526621, -13.17049365496744784 ) ) ;
#86745=CARTESIAN_POINT ( 'NONE',  ( 180.2261984326610218, 279.1782745765357276, -17.42438828499370729 ) ) ;
#86746=ORIENTED_EDGE ( 'NONE', *, *, #87810, .F. ) ;
#86748=CARTESIAN_POINT ( 'NONE',  ( 157.4313451293784851, 259.5368293376414499, 17.50557870161096830 ) ) ;
#86750=CARTESIAN_POINT ( 'NONE',  ( 57.27886009182306282, 210.0024278399160949, -9.188101187500093303 ) ) ;
#86753=CARTESIAN_POINT ( 'NONE',  ( 198.0827002274358222, 287.5576944360828975, 17.17879237213074006 ) ) ;
#86755=CARTESIAN_POINT ( 'NONE',  ( 176.5315280144691599, 273.2242205654873146, 17.34008498547847665 ) ) ;
#86759=CARTESIAN_POINT ( 'NONE',  ( 176.5752601597114335, 288.5842064133888130, 11.38490813771325350 ) ) ;
#86760=CARTESIAN_POINT ( 'NONE',  ( 153.6596595523362794, 266.9882342533689439, 16.60685250298524807 ) ) ;
#86762=CARTESIAN_POINT ( 'NONE',  ( 101.8522786425098445, 239.6115022471902876, -5.000000000000047962 ) ) ;
#86764=CARTESIAN_POINT ( 'NONE',  ( 161.2977680094314223, 251.2710659906439616, -13.03191437619249982 ) ) ;
#86765=CARTESIAN_POINT ( 'NONE',  ( 192.8607783413999073, 296.6023284558532396, -11.80574095728561446 ) ) ;
#86766=CARTESIAN_POINT ( 'NONE',  ( 149.7166446726674565, 271.3301600186404698, 12.26048591517335495 ) ) ;
#86767=CARTESIAN_POINT ( 'NONE',  ( 136.3105610988903607, 261.0530062829863027, -4.648177544792955347E-16 ) ) ;
#86768=CARTESIAN_POINT ( 'NONE',  ( 206.2520115784021471, 273.4080321133600933, 11.69992874350409018 ) ) ;
#86770=CARTESIAN_POINT ( 'NONE',  ( 154.2604299929738545, 264.1059117911821659, -16.74693418942497303 ) ) ;
#86772=CARTESIAN_POINT ( 'NONE',  ( 105.9656389868882513, 241.1744531367911577, 4.594050593750047540 ) ) ;
#86774=AXIS2_PLACEMENT_3D ( 'NONE', #76397, #5979, #84026 ) ;
#86775=CARTESIAN_POINT ( 'NONE',  ( 191.5893301551938350, 298.8045413135534432, -8.323356515452589477 ) ) ;
#86777=CARTESIAN_POINT ( 'NONE',  ( 155.5211745099813356, 261.2764194263634749, -17.18163098020766810 ) ) ;
#86778=CONICAL_SURFACE ( 'NONE', #83506, 17.82106496071138935, 0.7853981633974672638 ) ;
#86779=CARTESIAN_POINT ( 'NONE',  ( 163.7010375032499212, 247.1084811230698506, 6.649922295230481950 ) ) ;
#86781=CARTESIAN_POINT ( 'NONE',  ( 175.1529877741452026, 252.5256279684296885, 5.213479008607312615 ) ) ;
#86782=VERTEX_POINT ( 'NONE', #48281 ) ;
#86784=CARTESIAN_POINT ( 'NONE',  ( 154.6935981650651684, 273.3457612743501386, -13.11742276744757696 ) ) ;
#86785=CARTESIAN_POINT ( 'NONE',  ( 182.0160447414319549, 260.4886594560794038, 9.565111796795191523 ) ) ;
#86786=CARTESIAN_POINT ( 'NONE',  ( 206.1585898378126274, 271.5698433145930721, 8.212139725584252758 ) ) ;
#86787=CARTESIAN_POINT ( 'NONE',  ( 124.3418758452630613, 242.5958772461660544, -9.188101187500095079 ) ) ;
#86788=CARTESIAN_POINT ( 'NONE',  ( 151.0426280674448378, 269.0334894088936153, -15.84467774422408581 ) ) ;
#86790=CARTESIAN_POINT ( 'NONE',  ( 190.3443929803903814, 298.9608357525441420, -8.219721500574586059 ) ) ;
#86792=CARTESIAN_POINT ( 'NONE',  ( 57.30635725539759306, 194.7048013555409796, 4.594050593750051981 ) ) ;
#86795=CARTESIAN_POINT ( 'NONE',  ( 192.5672132233574700, 296.7161803602032819, 11.26440590052197521 ) ) ;
#86797=CARTESIAN_POINT ( 'NONE',  ( 171.3265457834860399, 259.7800479426538800, 15.31382021385433490 ) ) ;
#86799=CARTESIAN_POINT ( 'NONE',  ( 178.8786905444916897, 291.7200172712762765, -6.473733745693225572 ) ) ;
#86801=CARTESIAN_POINT ( 'NONE',  ( 155.6066474290145720, 261.1283759879266881, -18.16552045242181279 ) ) ;
#86802=CARTESIAN_POINT ( 'NONE',  ( 153.6642320881653632, 269.2038616895226255, -15.45545102632714851 ) ) ;
#86803=CARTESIAN_POINT ( 'NONE',  ( 119.8764323552255604, 240.0177522451418497, -10.00000000000009592 ) ) ;
#86804=B_SPLINE_CURVE_WITH_KNOTS ( 'NONE', 3,
 ( #57992, #79841, #18510, #64096, #26604, #10911, #87479, #41786, #10407, #66094, #27610, #58476, #57479, #18014, #11426, #49896, #34688, #65589 ),
 .UNSPECIFIED., .F., .F.,
 ( 4, 2, 2, 2, 2, 2, 2, 2, 4 ),
 ( 0.000000000000000000, 0.0003050680724331772137, 0.0006101361448663544275, 0.0009152042172995316412, 0.001220272289732708855, 0.001525340362165886069, 0.001830408434599063282, 0.002135476507032240713, 0.002440544579465417710 ),
 .UNSPECIFIED. ) ;
#86806=ORIENTED_EDGE ( 'NONE', *, *, #56222, .T. ) ;
#86807=EDGE_CURVE ( 'NONE', #80416, #96457, #14682, .T. ) ;
#86808=CARTESIAN_POINT ( 'NONE',  ( 202.9093905060991005, 279.1976216410395182, 16.97070083370504179 ) ) ;
#86811=CARTESIAN_POINT ( 'NONE',  ( 25.93973934025619599, 185.7833772461660544, -9.188101187500095079 ) ) ;
#86814=AXIS2_PLACEMENT_3D ( 'NONE', #88401, #72156, #35124 ) ;
#86817=CARTESIAN_POINT ( 'NONE',  ( 198.2595496549591587, 277.4556135032432849, -15.39564098667653980 ) ) ;
#86818=CARTESIAN_POINT ( 'NONE',  ( 54.92452707139267432, 202.5177522451418497, -10.00000000000009592 ) ) ;
#86819=CARTESIAN_POINT ( 'NONE',  ( 174.5901894622132033, 289.1458820068615978, 7.757015802472061239 ) ) ;
#86820=CARTESIAN_POINT ( 'NONE',  ( 181.3084254370976396, 256.5650938848051510, 1.317599750949192350 ) ) ;
#86821=CARTESIAN_POINT ( 'NONE',  ( 205.2937235227012707, 275.0678357141204629, -12.80017165135291535 ) ) ;
#86825=CARTESIAN_POINT ( 'NONE',  ( 20.80673460501611771, 189.4865022471903160, 10.00000000000009237 ) ) ;
#86827=FACE_OUTER_BOUND ( 'NONE', #19787, .T. ) ;
#86828=CARTESIAN_POINT ( 'NONE',  ( -7.212535326543083158, 157.4548013555409796, -4.594050593750042211 ) ) ;
#86830=B_SPLINE_CURVE_WITH_KNOTS ( 'NONE', 3,
 ( #22232, #53621, #98765, #29837 ),
 .UNSPECIFIED., .F., .F.,
 ( 4, 4 ),
 ( 2.797157557069881010E-17, 0.0005907011376378154327 ),
 .UNSPECIFIED. ) ;
#86832=CARTESIAN_POINT ( 'NONE',  ( 200.1775782763787390, 283.4917191864510073, 16.85546934141439124 ) ) ;
#86833=CARTESIAN_POINT ( 'NONE',  ( 152.6845319923753834, 266.1896283897672220, 17.20844521882669653 ) ) ;
#86835=CARTESIAN_POINT ( 'NONE',  ( 164.3754245770190039, 245.9404084473339083, 1.667926061651832992 ) ) ;
#86836=CARTESIAN_POINT ( 'NONE',  ( 184.7859038014685211, 258.6509473366765519, -2.313205586835159089 ) ) ;
#86840=CARTESIAN_POINT ( 'NONE',  ( 178.4072416225018287, 285.5359605631720683, 12.96076950543191408 ) ) ;
#86841=CARTESIAN_POINT ( 'NONE',  ( 153.2956058496949936, 277.6605163919303436, -5.395659764655544421 ) ) ;
#86843=CARTESIAN_POINT ( 'NONE',  ( 207.2758169296838560, 271.6347492278792402, 8.876423122295557633 ) ) ;
#86846=CARTESIAN_POINT ( 'NONE',  ( 159.3451320108506764, 254.6531307488737355, -16.72997986213134425 ) ) ;
#86848=CARTESIAN_POINT ( 'NONE',  ( 153.1164404339926080, 265.4415410246681972, 16.15325778160653414 ) ) ;
#86849=CARTESIAN_POINT ( 'NONE',  ( 207.1601050488701503, 271.8351680844880889, 6.320235450527015075 ) ) ;
#86851=CARTESIAN_POINT ( 'NONE',  ( 96.15094473426229627, 232.9865022471903160, 10.00000000000009415 ) ) ;
#86853=CARTESIAN_POINT ( 'NONE',  ( 155.4917600441137324, 261.3273667757233056, 17.14261720787171939 ) ) ;
#86854=ORIENTED_EDGE ( 'NONE', *, *, #11288, .F. ) ;
#86855=VERTEX_POINT ( 'NONE', #43142 ) ;
#86859=CARTESIAN_POINT ( 'NONE',  ( 186.1370921618058674, 283.3846817430978149, 17.26256540491417368 ) ) ;
#86860=EDGE_CURVE ( 'NONE', #88596, #64801, #20379, .T. ) ;
#86863=DIRECTION ( 'NONE',  ( -0.8660254037844387076, -0.4999999999999998890, -0.000000000000000000 ) ) ;
#86868=CARTESIAN_POINT ( 'NONE',  ( 174.8305575680244317, 267.7453695487130858, 17.43311389002270673 ) ) ;
#86870=CARTESIAN_POINT ( 'NONE',  ( 191.3638605175971747, 299.1950661814348678, 7.382965314423603154 ) ) ;
#86871=CARTESIAN_POINT ( 'NONE',  ( 151.4052515638881573, 274.9757893504045683, -8.619473620707406525 ) ) ;
#86873=CARTESIAN_POINT ( 'NONE',  ( 171.2890091316600092, 255.9655340354736666, -11.60100004170818977 ) ) ;
#86874=CARTESIAN_POINT ( 'NONE',  ( 163.1008115941903895, 248.1481028935802442, 11.25332017433677834 ) ) ;
#86876=B_SPLINE_CURVE_WITH_KNOTS ( 'NONE', 3,
 ( #19044, #75223, #13426, #82367, #73232, #49917, #26623, #12937, #58012, #42788, #96561, #58496, #66112, #21033, #5318, #90464, #58978, #4828, #74243, #34221, #73723, #51916, #59482, #4305, #88993, #65116, #27632, #89470, #35710, #28600, #80873, #43796, #44295, #19546, #12427, #36194, #42299, #97536, #66609, #89948, #28105, #3824, #67100, #20028 ),
 .UNSPECIFIED., .F., .F.,
 ( 4, 2, 2, 2, 2, 2, 2, 2, 2, 2, 2, 2, 2, 2, 2, 2, 2, 2, 2, 2, 2, 4 ),
 ( 0.003413446297188858260, 0.003592890090865467987, 0.003682611987703821206, 0.003772333884542174425, 0.003862055781380527644, 0.003951777678218881297, 0.004131221471895593807, 0.004490109059249017959, 0.004848996646602442978, 0.005566771821309291282, 0.006284546996016138719, 0.007720097345429752060, 0.008078984932783212641, 0.008123845881202462760, 0.008168706829621709409, 0.008213567778040957792, 0.008258428726460206176, 0.008437872520137456450, 0.008617316313814708459, 0.008796760107491960468, 0.008976203901169210742, 0.009155647694846462750 ),
 .UNSPECIFIED. ) ;
#86879=ORIENTED_EDGE ( 'NONE', *, *, #51234, .T. ) ;
#86880=CARTESIAN_POINT ( 'NONE',  ( 161.1242728399023747, 271.1573432374348727, 16.29312882630539150 ) ) ;
#86881=ORIENTED_EDGE ( 'NONE', *, *, #34742, .T. ) ;
#86884=CARTESIAN_POINT ( 'NONE',  ( 194.3011251241114508, 294.1075746476782342, -14.76047579547631905 ) ) ;
#86891=CARTESIAN_POINT ( 'NONE',  ( 205.8918578537579833, 274.0318366629789466, 11.52627491423194250 ) ) ;
#86892=CARTESIAN_POINT ( 'NONE',  ( 205.8452707775803390, 274.1125278458945900, 11.42742867493066328 ) ) ;
#86893=CARTESIAN_POINT ( 'NONE',  ( 206.9721564454444263, 271.1168479221515213, 4.971250805306120846 ) ) ;
#86894=ORIENTED_EDGE ( 'NONE', *, *, #87563, .F. ) ;
#86896=CARTESIAN_POINT ( 'NONE',  ( 147.0973304052008928, 275.8669454108827495, -4.174482164748090085 ) ) ;
#86897=CARTESIAN_POINT ( 'NONE',  ( 168.6951985533295044, 257.0048723434895805, -14.90311372616637264 ) ) ;
#86898=CARTESIAN_POINT ( 'NONE',  ( 206.1405152101578437, 273.6011494880188479, -9.618815605734603480 ) ) ;
#86901=CARTESIAN_POINT ( 'NONE',  ( 161.1027382213887336, 251.6088674925233022, 13.55451100897754557 ) ) ;
#86902=CARTESIAN_POINT ( 'NONE',  ( 191.4231707742389688, 260.8644426583601330, -0.1720874273815105604 ) ) ;
#86904=CARTESIAN_POINT ( 'NONE',  ( -22.42236680055709641, 157.8615022471902591, 0.000000000000000000 ) ) ;
#86908=CARTESIAN_POINT ( 'NONE',  ( 8.086986483384254853, 182.1427522451419350, -10.00000000000009415 ) ) ;
#86909=CARTESIAN_POINT ( 'NONE',  ( 81.47361835793333285, 217.8458772461660544, 9.188101187500095079 ) ) ;
#86911=CARTESIAN_POINT ( 'NONE',  ( 98.29796604426334738, 220.8927522451418213, 10.00000000000009948 ) ) ;
#86912=CARTESIAN_POINT ( 'NONE',  ( 208.1303038335461224, 270.1547344959873840, 3.060743731163897863 ) ) ;
#86913=CARTESIAN_POINT ( 'NONE',  ( 13.57207436428344316, 169.4548013555409796, -4.594050593750042211 ) ) ;
#86916=FACE_OUTER_BOUND ( 'NONE', #27023, .T. ) ;
#86922=CARTESIAN_POINT ( 'NONE',  ( 200.8891374359296833, 267.7797059101260970, -2.891206998117599625 ) ) ;
#86927=CARTESIAN_POINT ( 'NONE',  ( 207.8792014703394671, 270.5896565469619759, -5.780233892547864905 ) ) ;
#86928=( BOUNDED_CURVE ( )  B_SPLINE_CURVE ( 2, ( #55364, #1706, #47277, #86851, #56378, #48802, #9812, #71107, #56875 ),
 .UNSPECIFIED., .F., .T. ) 
 B_SPLINE_CURVE_WITH_KNOTS ( ( 3, 2, 2, 2, 3 ),
 ( 0.6975806451612903691, 0.6989247311827957443, 0.7016129032258064946, 0.7043010752688172449, 0.7056451612903226200 ),
 .UNSPECIFIED. ) 
 CURVE ( )  GEOMETRIC_REPRESENTATION_ITEM ( )  RATIONAL_B_SPLINE_CURVE ( ( 0.9330127018922194093, 0.9330127018922194093, 1.000000000000000000, 0.8660254037844387076, 1.000000000000000000, 0.8660254037844387076, 1.000000000000000000, 0.9330127018922194093, 0.9330127018922194093 ) ) 
 REPRESENTATION_ITEM ( '' )  );
#86931=CARTESIAN_POINT ( 'NONE',  ( 27.59033994439653270, 195.9244531367911293, -4.594050593750046652 ) ) ;
#86932=CARTESIAN_POINT ( 'NONE',  ( 75.78130554586785195, 227.8927522451419350, 2.944929066748280225E-16 ) ) ;
#86933=CARTESIAN_POINT ( 'NONE',  ( 199.3290434049739304, 277.4687221132098784, 15.18886269640733389 ) ) ;
#86934=ORIENTED_EDGE ( 'NONE', *, *, #82321, .F. ) ;
#86935=EDGE_CURVE ( 'NONE', #84442, #80986, #90414, .T. ) ;
#86937=CARTESIAN_POINT ( 'NONE',  ( 175.1939347090631145, 281.3215438300238134, -14.28959980792798667 ) ) ;
#86938=CARTESIAN_POINT ( 'NONE',  ( -6.265406815095104776, 161.0643266524160140, 9.188101187500095079 ) ) ;
#86940=CARTESIAN_POINT ( 'NONE',  ( 161.1093323826042933, 251.5974460702646809, -13.93502574894237078 ) ) ;
#86941=LINE ( 'NONE', #49375, #88923 ) ;
#86942=CARTESIAN_POINT ( 'NONE',  ( 194.5298665426430489, 293.7113828889860656, -16.13302716640051315 ) ) ;
#86943=CARTESIAN_POINT ( 'NONE',  ( 183.8544464940034402, 258.0811408654732872, -7.110849303899298590 ) ) ;
#86944=CARTESIAN_POINT ( 'NONE',  ( 171.5331681153915895, 279.9685107613297532, 15.23806245437180351 ) ) ;
#86945=CARTESIAN_POINT ( 'NONE',  ( 146.5502055023624735, 276.8145935406849389, 0.3770461397900869427 ) ) ;
#86946=CARTESIAN_POINT ( 'NONE',  ( 190.4744901378711290, 300.7355008658671522, 0.04566709859947504224 ) ) ;
#86948=ORIENTED_EDGE ( 'NONE', *, *, #17631, .F. ) ;
#86949=CARTESIAN_POINT ( 'NONE',  ( 164.1821508476733698, 246.2751683663292397, -7.347745041495428175 ) ) ;
#86950=CARTESIAN_POINT ( 'NONE',  ( 112.7044859340271472, 242.0024278399160949, 9.188101187500095079 ) ) ;
#86954=CARTESIAN_POINT ( 'NONE',  ( 157.2333142128019858, 258.3109064714224132, 16.87956768598436597 ) ) ;
#86955=CARTESIAN_POINT ( 'NONE',  ( 185.5841049239575398, 288.2424334149885112, 15.16588072270419651 ) ) ;
#86956=CARTESIAN_POINT ( 'NONE',  ( 150.6684462061087686, 269.6815914039983682, -13.71741525148136098 ) ) ;
#86957=CARTESIAN_POINT ( 'NONE',  ( 192.6126025028360402, 263.6580856887314894, -4.343318140713091857 ) ) ;
#86958=CARTESIAN_POINT ( 'NONE',  ( 148.9504735598738137, 272.6572073132907690, -11.88406006066344744 ) ) ;
#86961=CARTESIAN_POINT ( 'NONE',  ( 172.7262077320602316, 290.4534188193310911, -1.897623738731976983 ) ) ;
#86964=CARTESIAN_POINT ( 'NONE',  ( 139.8153705705071843, 239.9824982072973967, 3.021315404115420679E-15 ) ) ;
#86965=DIRECTION ( 'NONE',  ( 0.4999999999999998890, -0.8660254037844385966, 0.000000000000000000 ) ) ;
#86969=ORIENTED_EDGE ( 'NONE', *, *, #41935, .T. ) ;
#86970=B_SPLINE_SURFACE_WITH_KNOTS ( 'NONE', 3, 1, ( 
 ( #86166, #33402 ),
 ( #64303, #70396 ),
 ( #56182, #95254 ),
 ( #86660, #47592 ),
 ( #10107, #16700 ),
 ( #24792, #57185 ),
 ( #88164, #9626 ),
 ( #31886, #2007 ),
 ( #48094, #95758 ),
 ( #62791, #25822 ),
 ( #78520, #25296 ),
 ( #80043, #1521 ),
 ( #56698, #94734 ),
 ( #94240, #87679 ),
 ( #17192, #93748 ),
 ( #40972, #18214 ),
 ( #40487, #26310 ),
 ( #63800, #48613 ),
 ( #10610, #32401 ),
 ( #87176, #18712 ),
 ( #72431, #63298 ),
 ( #3034, #33925 ),
 ( #24307, #64810 ),
 ( #55673, #71918 ),
 ( #39978, #55183 ),
 ( #49594, #80548 ),
 ( #9105, #11125 ),
 ( #1008, #79035 ),
 ( #71417, #79552 ),
 ( #32893, #17712 ),
 ( #42967, #11618 ),
 ( #34401, #73909 ),
 ( #34885, #43973 ),
 ( #3522, #81055 ) ),
 .UNSPECIFIED., .T., .F., .F.,
 ( 4, 2, 2, 2, 2, 2, 2, 2, 2, 2, 2, 2, 2, 2, 2, 2, 4 ),
 ( 2, 2 ),
 ( 0.000000000000000000, 0.06250000000000000000, 0.1250000000000000000, 0.1875000000000000000, 0.2500000000000000000, 0.3125000000000000000, 0.3750000000000000000, 0.4375000000000000000, 0.5000000000000000000, 0.5625000000000000000, 0.6250000000000000000, 0.6875000000000000000, 0.7500000000000000000, 0.8125000000000000000, 0.8750000000000000000, 0.9375000000000000000, 1.000000000000000000 ),
 ( 0.000000000000000000, 1.000000000000000000 ),
 .UNSPECIFIED. ) ;
#86971=CARTESIAN_POINT ( 'NONE',  ( 147.6095992045671323, 244.4824982072973967, 3.021315404115420679E-15 ) ) ;
#86972=CARTESIAN_POINT ( 'NONE',  ( 180.2375854341549655, 256.9867171265678394, -8.836682230493849488 ) ) ;
#86974=CARTESIAN_POINT ( 'NONE',  ( 192.8132846206021611, 296.6845899933152850, 11.53748932578252351 ) ) ;
#86975=EDGE_CURVE ( 'NONE', #82867, #93959, #25043, .T. ) ;
#86978=CARTESIAN_POINT ( 'NONE',  ( 191.2386481741904163, 280.2331539523593733, 17.67023438497365362 ) ) ;
#86980=CARTESIAN_POINT ( 'NONE',  ( 192.8969106881193909, 288.6213907137100705, -15.93263679494918605 ) ) ;
#86982=CARTESIAN_POINT ( 'NONE',  ( 167.6835809486661049, 280.9580889920492268, 11.68121032124829384 ) ) ;
#86983=CARTESIAN_POINT ( 'NONE',  ( 164.3625597711517230, 265.6729452914248668, -17.82104740451561753 ) ) ;
#86984=CARTESIAN_POINT ( 'NONE',  ( -11.26211276271270378, 158.5313752282679900, 0.000000000000000000 ) ) ;
#86988=CARTESIAN_POINT ( 'NONE',  ( 188.8196614944561418, 293.5935099053481281, 12.74832926005498912 ) ) ;
#86992=CARTESIAN_POINT ( 'NONE',  ( 203.3041373168503299, 278.5139001086923827, -16.61929732091214973 ) ) ;
#86994=ORIENTED_EDGE ( 'NONE', *, *, #85455, .F. ) ;
#87004=CARTESIAN_POINT ( 'NONE',  ( 185.7869666842954075, 282.3491821533310713, -17.27175951461987324 ) ) ;
#87006=CARTESIAN_POINT ( 'NONE',  ( 205.9580306612148490, 273.9172219983844911, -10.82161348643986720 ) ) ;
#87007=CARTESIAN_POINT ( 'NONE',  ( 147.4361307740465179, 275.2801259584190916, -5.848038935779946712 ) ) ;
#87009=CARTESIAN_POINT ( 'NONE',  ( 146.7944005049231180, 276.3916353892955726, -4.243051111306586520 ) ) ;
#87010=CARTESIAN_POINT ( 'NONE',  ( 153.3939648708017387, 264.9608545997728015, -16.49556533540763681 ) ) ;
#87011=CARTESIAN_POINT ( 'NONE',  ( 46.78749671854927783, 204.4865022471903444, 10.00000000000009415 ) ) ;
#87012=CARTESIAN_POINT ( 'NONE',  ( 157.8247281260298109, 280.9212376166452145, 2.089162359923931955 ) ) ;
#87013=CARTESIAN_POINT ( 'NONE',  ( 127.9681836757279001, 250.8149278399160949, 9.188101187500093303 ) ) ;
#87015=DIRECTION ( 'NONE',  ( -0.8660254037844359321, -0.5000000000000051070, -0.000000000000000000 ) ) ;
#87017=ORIENTED_EDGE ( 'NONE', *, *, #87263, .T. ) ;
#87020=CARTESIAN_POINT ( 'NONE',  ( 203.6239051785863410, 276.2879242122419328, 13.38875856211884319 ) ) ;
#87021=CARTESIAN_POINT ( 'NONE',  ( 178.3662840243317760, 253.4271165972424171, 1.412557629060920750 ) ) ;
#87022=CARTESIAN_POINT ( 'NONE',  ( 171.7394409073507120, 288.1570534852701257, -4.630247488080818208 ) ) ;
#87025=CARTESIAN_POINT ( 'NONE',  ( 201.0732166862245549, 282.3779679885897167, -18.18766936363638820 ) ) ;
#87026=CARTESIAN_POINT ( 'NONE',  ( 175.9763040572248656, 288.1059871890528825, -9.332626666196993881 ) ) ;
#87027=CARTESIAN_POINT ( 'NONE',  ( 193.8885253154310249, 293.1561265193603845, -14.44353267613299785 ) ) ;
#87028=CARTESIAN_POINT ( 'NONE',  ( 194.9962653018843071, 291.7955338748228087, 15.77605307729832518 ) ) ;
#87030=CARTESIAN_POINT ( 'NONE',  ( 194.8067605455144076, 293.2317884077015151, -16.00245909155922774 ) ) ;
#87031=CARTESIAN_POINT ( 'NONE',  ( 152.8472162863966730, 273.6966317651701956, 11.99970075400534775 ) ) ;
#87034=CARTESIAN_POINT ( 'NONE',  ( 160.2440860423037350, 278.9300554605163143, 10.54469911904840451 ) ) ;
#87035=CARTESIAN_POINT ( 'NONE',  ( 152.3899997637754211, 266.6997731741686835, -15.63510712473265052 ) ) ;
#87037=CARTESIAN_POINT ( 'NONE',  ( 163.4260108471723640, 247.5848412648317662, 10.45113099391573108 ) ) ;
#87038=CARTESIAN_POINT ( 'NONE',  ( 163.9578236787243100, 284.1347344607588070, -7.051233874980773919 ) ) ;
#87039=CARTESIAN_POINT ( 'NONE',  ( 153.9180730477606573, 276.4901683324925443, -8.670461530457965083 ) ) ;
#87040=CARTESIAN_POINT ( 'NONE',  ( 162.5076833207704965, 285.2105136841905164, -0.5237628275906566211 ) ) ;
#87041=VERTEX_POINT ( 'NONE', #39030 ) ;
#87043=CARTESIAN_POINT ( 'NONE',  ( 167.9126157730074169, 281.9481797483980472, -10.88728177065660851 ) ) ;
#87044=CARTESIAN_POINT ( 'NONE',  ( 187.9582674523677213, 263.4472869081138242, -9.058670945028287846 ) ) ;
#87046=CARTESIAN_POINT ( 'NONE',  ( 82.70950877614343710, 211.8927522451418213, 10.00000000000009948 ) ) ;
#87047=CARTESIAN_POINT ( 'NONE',  ( 169.0357847594885357, 288.9123690687650878, -1.452882998383906221 ) ) ;
#87048=CARTESIAN_POINT ( 'NONE',  ( 152.6992418905140028, 266.1641500988167763, 17.27767170937316621 ) ) ;
#87052=CARTESIAN_POINT ( 'NONE',  ( -15.08856125979659346, 174.3464784336661637, 1.353441290958777525E-15 ) ) ;
#87053=CARTESIAN_POINT ( 'NONE',  ( 79.66011734693590540, 225.9869531367911293, 4.594050593750046652 ) ) ;
#87054=CARTESIAN_POINT ( 'NONE',  ( -29.83289928091279464, 170.6969210143057580, 1.815056976409021644E-15 ) ) ;
#87055=CARTESIAN_POINT ( 'NONE',  ( 146.8574506849497538, 276.2824292740633041, -4.888313306692038118 ) ) ;
#87056=CARTESIAN_POINT ( 'NONE',  ( 182.7920823588448513, 294.2517127691644987, -7.995619123199669609 ) ) ;
#87057=EDGE_CURVE ( 'NONE', #16332, #26607, #55355, .T. ) ;
#87062=B_SPLINE_CURVE_WITH_KNOTS ( 'NONE', 3,
 ( #71368, #47541, #92687, #70344 ),
 .UNSPECIFIED., .F., .F.,
 ( 4, 4 ),
 ( 0.009416156603928334604, 0.01493877551972221454 ),
 .UNSPECIFIED. ) ;
#87065=CARTESIAN_POINT ( 'NONE',  ( 207.9610911165470100, 270.4478195191170471, 5.492635222805117401 ) ) ;
#87066=EDGE_CURVE ( 'NONE', #67601, #25811, #70971, .T. ) ;
#87067=CARTESIAN_POINT ( 'NONE',  ( 169.1328200606558312, 252.0173167888393664, -8.779758093320142009 ) ) ;
#87074=CARTESIAN_POINT ( 'NONE',  ( 41.36599039304901737, 188.5643266524159571, -9.188101187500093303 ) ) ;
#87077=CARTESIAN_POINT ( 'NONE',  ( 66.48072710279772934, 203.0643266524160424, 9.188101187500095079 ) ) ;
#87078=CARTESIAN_POINT ( 'NONE',  ( 64.25234236153551137, 201.2365022471902023, -10.00000000000009237 ) ) ;
#87081=DIRECTION ( 'NONE',  ( 0.4999999999999998890, -0.8660254037844385966, 0.000000000000000000 ) ) ;
#87082=CARTESIAN_POINT ( 'NONE',  ( 151.9298993999875904, 267.4966903808301026, 16.91367899156788468 ) ) ;
#87083=CARTESIAN_POINT ( 'NONE',  ( 20.35567970366385993, 175.8927522451418497, 10.00000000000009948 ) ) ;
#87086=CARTESIAN_POINT ( 'NONE',  ( 196.2878005184348353, 290.6665519265632724, -16.69183432842427806 ) ) ;
#87089=CARTESIAN_POINT ( 'NONE',  ( 76.54827242179185021, 208.8768266524160140, 9.188101187500096856 ) ) ;
#87091=CARTESIAN_POINT ( 'NONE',  ( 172.6820923522780049, 290.5181543830415762, -0.3406277123404243268 ) ) ;
#87093=CARTESIAN_POINT ( 'NONE',  ( 202.0722854591110718, 280.6475301136950407, 16.68111299382005086 ) ) ;
#87095=CARTESIAN_POINT ( 'NONE',  ( 193.6371173231629541, 288.3972668369637518, 16.12142398166468382 ) ) ;
#87097=CARTESIAN_POINT ( 'NONE',  ( 126.4618338667176261, 250.4865022471902876, -10.00000000000009415 ) ) ;
#87098=CARTESIAN_POINT ( 'NONE',  ( 19.85049821812295079, 172.2677522451417929, -5.000000000000041744 ) ) ;
#87100=CARTESIAN_POINT ( 'NONE',  ( 164.7694554770609159, 245.2579269087094076, -3.003635650077957742 ) ) ;
#87103=CARTESIAN_POINT ( 'NONE',  ( 188.5427288919736100, 272.8462714947278300, 15.72219057270026532 ) ) ;
#87105=CARTESIAN_POINT ( 'NONE',  ( 203.0337691736598629, 278.9821914694464340, 16.08167820133810011 ) ) ;
#87107=FACE_OUTER_BOUND ( 'NONE', #57622, .T. ) ;
#87108=EDGE_LOOP ( 'NONE', ( #18770, #43317, #76782, #5200, #50796 ) ) ;
#87109=CARTESIAN_POINT ( 'NONE',  ( 176.1203811719671535, 253.1057001499724208, -0.2550088935518543543 ) ) ;
#87111=VERTEX_POINT ( 'NONE', #24846 ) ;
#87113=EDGE_CURVE ( 'NONE', #63065, #43398, #97568, .T. ) ;
#87114=CARTESIAN_POINT ( 'NONE',  ( 170.6552073324595256, 250.4298647395600881, 3.342757437244376018 ) ) ;
#87115=CARTESIAN_POINT ( 'NONE',  ( 148.4944702278734781, 274.4665431084056308, 7.703859803813626783 ) ) ;
#87117=ORIENTED_EDGE ( 'NONE', *, *, #69452, .T. ) ;
#87124=EDGE_CURVE ( 'NONE', #36064, #14175, #61276, .T. ) ;
#87125=CARTESIAN_POINT ( 'NONE',  ( 160.6526974584403149, 271.0904541309827778, -16.59201714530360050 ) ) ;
#87126=FACE_OUTER_BOUND ( 'NONE', #64561, .T. ) ;
#87129=CARTESIAN_POINT ( 'NONE',  ( 186.0715527847238207, 298.7753624933060337, 1.084710433360843940 ) ) ;
#87130=AXIS2_PLACEMENT_3D ( 'NONE', #72943, #2020, #63814 ) ;
#87132=CARTESIAN_POINT ( 'NONE',  ( 147.8819534105757043, 274.5079385007862811, -9.338341377131436971 ) ) ;
#87134=FACE_OUTER_BOUND ( 'NONE', #49431, .T. ) ;
#87136=CARTESIAN_POINT ( 'NONE',  ( 157.8043799545718286, 257.3217915922150496, -17.97575562758749257 ) ) ;
#87137=CARTESIAN_POINT ( 'NONE',  ( 207.5882819593617796, 271.0935439208888624, -5.111091721253596454 ) ) ;
#87141=CARTESIAN_POINT ( 'NONE',  ( 76.62902843369037953, 224.2369531367911293, -4.594050593750048428 ) ) ;
#87143=CARTESIAN_POINT ( 'NONE',  ( 191.4685399627163633, 299.0137560639802814, 7.545791216288330716 ) ) ;
#87144=CARTESIAN_POINT ( 'NONE',  ( 177.7634369230092091, 252.8608366103077856, -4.270187854574569275E-12 ) ) ;
#87146=CARTESIAN_POINT ( 'NONE',  ( 196.0264968210332768, 291.1191432066681841, -16.98183272759323614 ) ) ;
#87147=VERTEX_POINT ( 'NONE', #54225 ) ;
#87150=CARTESIAN_POINT ( 'NONE',  ( 146.5913834600193582, 276.7432712258716947, -0.4909717733184599253 ) ) ;
#87153=CARTESIAN_POINT ( 'NONE',  ( 163.0959165854295065, 248.1565812974573930, 11.58894702640622754 ) ) ;
#87154=CARTESIAN_POINT ( 'NONE',  ( 97.38683515247240052, 227.0333772461660544, 9.188101187500095079 ) ) ;
#87157=ORIENTED_EDGE ( 'NONE', *, *, #40780, .T. ) ;
#87158=CARTESIAN_POINT ( 'NONE',  ( 113.0439006004949931, 247.6199935810940929, 2.679491924311251605 ) ) ;
#87159=CARTESIAN_POINT ( 'NONE',  ( 201.0579808891486380, 282.4043571632192311, -17.91925047041473107 ) ) ;
#87164=CARTESIAN_POINT ( 'NONE',  ( -8.295327404871391863, 176.0177522451419350, 5.000000000000046185 ) ) ;
#87168=CARTESIAN_POINT ( 'NONE',  ( 156.8153509015677400, 274.0293242336268236, 13.38325589097203228 ) ) ;
#87169=CARTESIAN_POINT ( 'NONE',  ( 206.0946696452135427, 273.6805563358039421, -10.19627505985792837 ) ) ;
#87170=CARTESIAN_POINT ( 'NONE',  ( 147.7528226544125687, 275.1182078777800939, -4.309999617748870193 ) ) ;
#87174=ORIENTED_EDGE ( 'NONE', *, *, #29293, .T. ) ;
#87176=CARTESIAN_POINT ( 'NONE',  ( 200.5621507313343557, 283.2631601884785368, 16.81037192529623425 ) ) ;
#87179=CARTESIAN_POINT ( 'NONE',  ( 171.6425804079232194, 251.4895661525248727, 7.246871942246497333 ) ) ;
#87181=CARTESIAN_POINT ( 'NONE',  ( 175.0511171704688707, 290.6789393214584152, -6.519569310547577601 ) ) ;
#87182=CARTESIAN_POINT ( 'NONE',  ( 153.5047258249362869, 270.3281759409417759, 14.02017829003231597 ) ) ;
#87184=EDGE_CURVE ( 'NONE', #6168, #43553, #63198, .T. ) ;
#87186=AXIS2_PLACEMENT_3D ( 'NONE', #29606, #66608, #21998 ) ;
#87188=CARTESIAN_POINT ( 'NONE',  ( 58.36827475829091583, 216.0530062829863311, -4.648177544792955347E-16 ) ) ;
#87193=CARTESIAN_POINT ( 'NONE',  ( 98.02733310912860532, 220.7365022471901739, -10.00000000000009237 ) ) ;
#87194=CARTESIAN_POINT ( 'NONE',  ( 172.2199326777433441, 275.1102788966048820, 16.82814706134498905 ) ) ;
#87197=CARTESIAN_POINT ( 'NONE',  ( 189.4870307839178452, 261.4823983659626379, 2.871469372538022924 ) ) ;
#87199=CARTESIAN_POINT ( 'NONE',  ( 207.5462191418491500, 271.1663988579299485, -5.239401497773396699 ) ) ;
#87201=CARTESIAN_POINT ( 'NONE',  ( 7.590999645455913658, 169.0643266524160140, -9.188101187500093303 ) ) ;
#87204=CARTESIAN_POINT ( 'NONE',  ( 160.3464284523794561, 253.3627658000544045, -14.66853605427253271 ) ) ;
#87207=CARTESIAN_POINT ( 'NONE',  ( 29.78290061743215134, 181.8768266524160424, 9.188101187500096856 ) ) ;
#87210=CARTESIAN_POINT ( 'NONE',  ( 181.4654272287283447, 294.5040635489617102, 6.489362936760144862 ) ) ;
#87211=CARTESIAN_POINT ( 'NONE',  ( 191.8210230231139803, 298.4032374945642232, -8.800268167321144475 ) ) ;
#87212=CARTESIAN_POINT ( 'NONE',  ( 197.0721673821830962, 289.3079886667778737, 16.89290144598883003 ) ) ;
#87216=CARTESIAN_POINT ( 'NONE',  ( 188.9137685052497773, 297.3500637095433490, -7.801865818255394380 ) ) ;
#87218=CARTESIAN_POINT ( 'NONE',  ( 83.16056367749570200, 225.4865022471902876, 10.00000000000009237 ) ) ;
#87220=EDGE_CURVE ( 'NONE', #78035, #4325, #3376, .T. ) ;
#87222=CARTESIAN_POINT ( 'NONE',  ( 41.04123086662985997, 188.3768266524159856, -9.188101187500091527 ) ) ;
#87227=CARTESIAN_POINT ( 'NONE',  ( 198.5954523381739989, 286.6695817285962562, -18.45134152028667174 ) ) ;
#87229=VERTEX_POINT ( 'NONE', #44903 ) ;
#87230=CARTESIAN_POINT ( 'NONE',  ( 86.76900285993092155, 214.2365022471902023, 10.00000000000009948 ) ) ;
#87235=CARTESIAN_POINT ( 'NONE',  ( 202.6551236945213361, 279.6380246773706517, 15.55476940527561425 ) ) ;
#87236=CARTESIAN_POINT ( 'NONE',  ( 196.4808189786114951, 290.3322341467384717, -17.84817245450773271 ) ) ;
#87237=CARTESIAN_POINT ( 'NONE',  ( 188.2366137343229866, 269.6014790893902955, -14.07889599767974431 ) ) ;
#87238=VERTEX_POINT ( 'NONE', #36313 ) ;
#87241=CARTESIAN_POINT ( 'NONE',  ( 156.6812872898450735, 261.2670451491295012, 0.000000000000000000 ) ) ;
#87243=ORIENTED_EDGE ( 'NONE', *, *, #54652, .F. ) ;
#87245=CARTESIAN_POINT ( 'NONE',  ( 179.7389585068036979, 283.2694176073634935, 16.15404047216739514 ) ) ;
#87246=CARTESIAN_POINT ( 'NONE',  ( 150.6571681785161445, 269.7011255207979730, 15.24894850018880454 ) ) ;
#87247=CARTESIAN_POINT ( 'NONE',  ( 177.3670312401388571, 255.9174922417764435, -7.030267280083029924 ) ) ;
#87248=CARTESIAN_POINT ( 'NONE',  ( 164.7396270603856294, 269.0037874151494179, 17.61975801440670608 ) ) ;
#87250=ORIENTED_EDGE ( 'NONE', *, *, #22716, .T. ) ;
#87251=CARTESIAN_POINT ( 'NONE',  ( 186.6626062937425843, 272.3587087772825726, -15.95341871095174291 ) ) ;
#87252=CARTESIAN_POINT ( 'NONE',  ( 168.8785100482814698, 272.6966330010931756, 17.41127854651366391 ) ) ;
#87253=ORIENTED_EDGE ( 'NONE', *, *, #58301, .T. ) ;
#87254=CARTESIAN_POINT ( 'NONE',  ( 152.6692142062575499, 266.2161595735824449, -16.77985299603479419 ) ) ;
#87259=CARTESIAN_POINT ( 'NONE',  ( 157.1850763439666139, 258.3944569110938687, -16.98181238659443437 ) ) ;
#87260=CARTESIAN_POINT ( 'NONE',  ( 103.3675627755349353, 239.6744531367911577, 4.594050593750047540 ) ) ;
#87263=EDGE_CURVE ( 'NONE', #41237, #42896, #32410, .T. ) ;
#87264=CARTESIAN_POINT ( 'NONE',  ( 87.40047971330916710, 211.2677522451417929, -5.000000000000041744 ) ) ;
#87267=CARTESIAN_POINT ( 'NONE',  ( 161.7691914441718382, 267.0751698082785310, 16.49970973976455113 ) ) ;
#87272=CARTESIAN_POINT ( 'NONE',  ( 49.86334402403631572, 211.8464784336661637, 1.353441290958777525E-15 ) ) ;
#87275=CARTESIAN_POINT ( 'NONE',  ( 150.7254409736883645, 269.5828735707850683, 14.54962197351449049 ) ) ;
#87277=CARTESIAN_POINT ( 'NONE',  ( 172.9863964892439867, 271.2482479143764635, 16.42685820048345491 ) ) ;
#87281=CARTESIAN_POINT ( 'NONE',  ( 178.0447788114544210, 288.9018666865521823, 11.00351160062661826 ) ) ;
#87284=CARTESIAN_POINT ( 'NONE',  ( 171.8690269922494451, 259.0866485604661307, -13.74017874718136056 ) ) ;
#87285=CARTESIAN_POINT ( 'NONE',  ( 174.2854763267832254, 277.2339634087840068, -15.62137160143660175 ) ) ;
#87286=CARTESIAN_POINT ( 'NONE',  ( 207.1285138014047504, 271.8898857301724661, -5.752177443817618752 ) ) ;
#87287=CARTESIAN_POINT ( 'NONE',  ( 193.0761489135300906, 296.2292956824684893, -11.99675185248219655 ) ) ;
#87288=CARTESIAN_POINT ( 'NONE',  ( 50.69007152801540883, 211.6199935810940929, 2.679491924311251605 ) ) ;
#87289=CARTESIAN_POINT ( 'NONE',  ( 177.3316242072715170, 269.5189898217483346, 16.09928397702987368 ) ) ;
#87291=CARTESIAN_POINT ( 'NONE',  ( 206.4943150373521803, 272.9883502116088039, 11.34100825923693101 ) ) ;
#87293=CARTESIAN_POINT ( 'NONE',  ( 167.5840822128345167, 256.4747449104621069, 13.66287527167402693 ) ) ;
#87294=CARTESIAN_POINT ( 'NONE',  ( 131.1144086761837571, 258.0530062829863027, -4.648177544792955347E-16 ) ) ;
#87295=CARTESIAN_POINT ( 'NONE',  ( 117.8198823448352499, 229.6423013555409796, -4.594050593750043987 ) ) ;
#87296=ORIENTED_EDGE ( 'NONE', *, *, #88443, .T. ) ;
#87297=CARTESIAN_POINT ( 'NONE',  ( 148.9673139787263381, 272.6280388522173439, -12.20954562941818722 ) ) ;
#87298=CARTESIAN_POINT ( 'NONE',  ( 92.16361943412358926, 214.0177522451417929, 5.000000000000051514 ) ) ;
#87300=CARTESIAN_POINT ( 'NONE',  ( 191.8986733338516331, 296.2687432111309249, 12.49828825629462337 ) ) ;
#87305=CARTESIAN_POINT ( 'NONE',  ( 156.6472780479514029, 274.0223492104835827, -12.66898415510409137 ) ) ;
#87307=CARTESIAN_POINT ( 'NONE',  ( 184.6885808911535207, 260.6528513612950064, 10.31057805081157852 ) ) ;
#87308=CARTESIAN_POINT ( 'NONE',  ( 206.3528985702396596, 273.2332907176744925, -9.687807306503337657 ) ) ;
#87309=CARTESIAN_POINT ( 'NONE',  ( 146.6963301283313967, 249.3768266524160424, 9.188101187500096856 ) ) ;
#87310=CARTESIAN_POINT ( 'NONE',  ( 189.7009002764073102, 294.6524816643598115, -12.56900444601840938 ) ) ;
#87313=CARTESIAN_POINT ( 'NONE',  ( 70.29673831216418023, 202.2048013555409796, 4.594050593750051981 ) ) ;
#87315=CARTESIAN_POINT ( 'NONE',  ( 157.8719920515997046, 257.2046840049564480, -17.69857783492101433 ) ) ;
#87319=CARTESIAN_POINT ( 'NONE',  ( 171.0837707628333817, 259.8106783156040933, 15.05102682647995849 ) ) ;
#87323=EDGE_CURVE ( 'NONE', #33698, #49174, #68644, .T. ) ;
#87324=CARTESIAN_POINT ( 'NONE',  ( 194.1322773954189813, 288.8521459192547809, 16.09912479026312937 ) ) ;
#87325=CARTESIAN_POINT ( 'NONE',  ( 123.7735466722555628, 242.2677522451418497, 10.00000000000009592 ) ) ;
#87328=ORIENTED_EDGE ( 'NONE', *, *, #29720, .T. ) ;
#87329=EDGE_CURVE ( 'NONE', #54166, #94303, #67197, .T. ) ;
#87331=CARTESIAN_POINT ( 'NONE',  ( 190.3049670482083684, 301.0291234702190764, 0.2225066852051815758 ) ) ;
#87333=CARTESIAN_POINT ( 'NONE',  ( 45.69611741197122257, 191.0643266524160140, 9.188101187500095079 ) ) ;
#87334=CIRCLE ( 'NONE', #43569, 17.82106496071138224 ) ;
#87338=CARTESIAN_POINT ( 'NONE',  ( 147.3154503175461514, 275.4891506405583073, 3.671329888160011823 ) ) ;
#87340=CARTESIAN_POINT ( 'NONE',  ( 198.0840284456224651, 277.7725242502040146, -15.93544264248174969 ) ) ;
#87341=CARTESIAN_POINT ( 'NONE',  ( 49.65620586503731460, 206.1427522451419350, -10.00000000000009415 ) ) ;
#87342=CARTESIAN_POINT ( 'NONE',  ( 123.9359264390130591, 242.3615022471902591, -10.00000000000009592 ) ) ;
#87343=CARTESIAN_POINT ( 'NONE',  ( 181.2352160778011410, 256.5241942803364736, 1.318112620201692398 ) ) ;
#87344=CARTESIAN_POINT ( 'NONE',  ( 205.3465787480556344, 274.9762877783610406, -13.79319041940166279 ) ) ;
#87346=ORIENTED_EDGE ( 'NONE', *, *, #19358, .T. ) ;
#87349=CARTESIAN_POINT ( 'NONE',  ( 179.5139751590971287, 294.9444787810163007, 1.083326342264184117 ) ) ;
#87350=CARTESIAN_POINT ( 'NONE',  ( 38.19941146435361645, 192.8615022471902591, -10.00000000000009592 ) ) ;
#87351=CARTESIAN_POINT ( 'NONE',  ( 40.63510790894947888, 184.2677522451417929, -5.000000000000041744 ) ) ;
#87352=CARTESIAN_POINT ( 'NONE',  ( 162.9796882977680639, 248.3578945969637743, 9.683801903336119565 ) ) ;
#87353=CARTESIAN_POINT ( 'NONE',  ( 7.942909239684589728, 166.2048013555410080, 4.594050593750051981 ) ) ;
#87355=CARTESIAN_POINT ( 'NONE',  ( 164.2304771159539314, 252.5565421600307729, 13.36745210293446107 ) ) ;
#87357=CARTESIAN_POINT ( 'NONE',  ( 152.6656396574222754, 266.2223508737794759, 17.04346597795114349 ) ) ;
#87359=CARTESIAN_POINT ( 'NONE',  ( 155.9941297720162368, 261.2689480174557843, -17.22357958794880517 ) ) ;
#87364=CARTESIAN_POINT ( 'NONE',  ( 183.6215648671697522, 257.5753772875778509, -6.308267261209747012 ) ) ;
#87367=CARTESIAN_POINT ( 'NONE',  ( 168.6548331014163011, 287.6097714008884623, 0.5119831642859076215 ) ) ;
#87372=CARTESIAN_POINT ( 'NONE',  ( 206.8659638600981623, 272.3446355680395641, -10.26115277030573125 ) ) ;
#87373=ORIENTED_EDGE ( 'NONE', *, *, #30664, .F. ) ;
#87375=CARTESIAN_POINT ( 'NONE',  ( 206.8986117509267899, 272.2880877623646825, 6.975890063856878598 ) ) ;
#87378=CARTESIAN_POINT ( 'NONE',  ( 155.5204415533959548, 261.2776889444089647, 17.19127227448963424 ) ) ;
#87381=CARTESIAN_POINT ( 'NONE',  ( 155.9945892501227434, 277.4300987863958312, -10.50269384731501709 ) ) ;
#87388=CYLINDRICAL_SURFACE ( 'NONE', #76677, 17.82106496071139645 ) ;
#87389=EDGE_CURVE ( 'NONE', #33095, #15038, #46745, .T. ) ;
#87390=CARTESIAN_POINT ( 'NONE',  ( 174.5814835802148650, 266.1494510194049781, 17.18910567408474677 ) ) ;
#87391=ORIENTED_EDGE ( 'NONE', *, *, #13889, .T. ) ;
#87392=CARTESIAN_POINT ( 'NONE',  ( 174.1881985213240682, 267.4147193431427354, 17.25901729942388485 ) ) ;
#87393=CARTESIAN_POINT ( 'NONE',  ( 169.3620869378731300, 276.4508859477064675, -16.02936318750594324 ) ) ;
#87394=CARTESIAN_POINT ( 'NONE',  ( 150.8888667059421209, 269.2998118992572927, 15.79021133717968617 ) ) ;
#87395=CARTESIAN_POINT ( 'NONE',  ( 173.7623083844477208, 263.9770854346508600, 16.71843220567729915 ) ) ;
#87396=ORIENTED_EDGE ( 'NONE', *, *, #38002, .T. ) ;
#87397=CARTESIAN_POINT ( 'NONE',  ( 171.2113793187262729, 254.5338664307851957, -11.68439913917253392 ) ) ;
#87400=ORIENTED_EDGE ( 'NONE', *, *, #61020, .T. ) ;
#87401=DIRECTION ( 'NONE',  ( 0.8660254037844395958, 0.4999999999999985567, 0.000000000000000000 ) ) ;
#87406=CARTESIAN_POINT ( 'NONE',  ( 168.7111818900347373, 272.8077130806378818, 15.97973317249935121 ) ) ;
#87407=CARTESIAN_POINT ( 'NONE',  ( 193.9335844648177272, 294.7441737434225502, 14.74820358206551596 ) ) ;
#87408=CARTESIAN_POINT ( 'NONE',  ( 177.3385562594880298, 288.8319590472722780, -9.367248622587959872 ) ) ;
#87410=EDGE_CURVE ( 'NONE', #29964, #62095, #85373, .T. ) ;
#87411=CARTESIAN_POINT ( 'NONE',  ( 200.4906113350036776, 281.3870700576555919, -17.24871243658977704 ) ) ;
#87414=DIRECTION ( 'NONE',  ( 0.4999999999999998890, -0.8660254037844385966, 0.000000000000000000 ) ) ;
#87416=CARTESIAN_POINT ( 'NONE',  ( 172.2831709724378868, 290.7678881282855059, 1.703707976439254201 ) ) ;
#87418=CARTESIAN_POINT ( 'NONE',  ( 164.6241018286200699, 245.5096868128744632, 3.031483545445131433 ) ) ;
#87419=CARTESIAN_POINT ( 'NONE',  ( 206.3907062969896060, 273.1678058140250300, 11.56942460516550675 ) ) ;
#87420=CARTESIAN_POINT ( 'NONE',  ( 159.3528137482544196, 254.6398255893999476, 16.73628156321660398 ) ) ;
#87421=ORIENTED_EDGE ( 'NONE', *, *, #97788, .T. ) ;
#87423=CARTESIAN_POINT ( 'NONE',  ( 190.3865446062718547, 300.8878269948957040, 5.596937249297124772 ) ) ;
#87427=CARTESIAN_POINT ( 'NONE',  ( 200.9110265982630779, 282.6588894614233141, 17.52479721249226685 ) ) ;
#87430=CARTESIAN_POINT ( 'NONE',  ( 192.6361035247282985, 294.0892689374524593, 14.43747539422717630 ) ) ;
#87432=CARTESIAN_POINT ( 'NONE',  ( -8.638129123654803010, 172.4865022471903160, -10.00000000000009592 ) ) ;
#87433=CARTESIAN_POINT ( 'NONE',  ( 8.231324050681633864, 188.8927522451419634, 2.944929066748280225E-16 ) ) ;
#87434=B_SPLINE_CURVE_WITH_KNOTS ( 'NONE', 3,
 ( #8100, #70384, #69879, #99803, #493, #30389, #39962, #62775, #31380, #62265, #61280, #17178, #47578, #93220, #24293, #63284, #78506, #53673, #1505, #84627, #46068, #94227, #76981, #55660, #86647, #48079, #79020, #9609, #15168, #7584, #38475, #5, #69388, #42463, #41980, #80027, #87664, #26788, #65769, #40959, #1994, #56681, #32880, #96224, #10595, #56166 ),
 .UNSPECIFIED., .F., .F.,
 ( 4, 2, 2, 2, 2, 2, 2, 2, 2, 2, 2, 2, 2, 2, 2, 2, 2, 2, 2, 2, 2, 2, 4 ),
 ( 0.0001899055419981224681, 0.0006750962773007901071, 0.001160287012603457638, 0.001402882380254854341, 0.001645477747906250610, 0.001766775431732028976, 0.001888073115557807342, 0.002009370799383585707, 0.002130668483209364073, 0.002615859218512393836, 0.003101049953815423598, 0.004071431424421405494, 0.005041812895027385222, 0.005527003630330376387, 0.005769598997981835106, 0.006012194365633293826, 0.006072843207546120559, 0.006133492049458947291, 0.006254789733284562593, 0.006497385100935834830, 0.006982575836238381038, 0.007467766571540925512, 0.007952957306843470853 ),
 .UNSPECIFIED. ) ;
#87435=CARTESIAN_POINT ( 'NONE',  ( 97.06207562605321471, 226.8458772461660544, 9.188101187500095079 ) ) ;
#87437=DIRECTION ( 'NONE',  ( -0.8660254037844387076, -0.4999999999999998890, -0.000000000000000000 ) ) ;
#87438=CARTESIAN_POINT ( 'NONE',  ( 166.8010608816141769, 278.4144572394360466, -14.76014027413921070 ) ) ;
#87439=CARTESIAN_POINT ( 'NONE',  ( 22.85469738715664434, 177.8768266524160140, -9.188101187500091527 ) ) ;
#87441=CARTESIAN_POINT ( 'NONE',  ( 161.6673510627899191, 250.6309293646106653, 13.01175935005004192 ) ) ;
#87443=EDGE_LOOP ( 'NONE', ( #59788, #75971, #85886, #28001 ) ) ;
#87444=CARTESIAN_POINT ( 'NONE',  ( 197.7156036016341147, 265.5775033884078766, -2.905260353570674248 ) ) ;
#87447=CARTESIAN_POINT ( 'NONE',  ( 193.1380270375380803, 263.9472543795415049, -4.333440441786139630 ) ) ;
#87448=CARTESIAN_POINT ( 'NONE',  ( 207.8984236726843164, 270.5563627158673512, -6.084369154771423815 ) ) ;
#87449=CARTESIAN_POINT ( 'NONE',  ( 182.5715074166515990, 284.2755724526985546, 14.95694440675247527 ) ) ;
#87451=CARTESIAN_POINT ( 'NONE',  ( 40.49996498926459054, 188.0643266524160140, 9.188101187500095079 ) ) ;
#87452=CARTESIAN_POINT ( 'NONE',  ( 86.17361039128121547, 213.8927522451417929, -10.00000000000009059 ) ) ;
#87456=CARTESIAN_POINT ( 'NONE',  ( 179.4037581149374034, 257.9870511612666064, -10.76565914641300736 ) ) ;
#87457=CARTESIAN_POINT ( 'NONE',  ( -1.691623377417284635, 160.6423013555410080, -4.594050593750043987 ) ) ;
#87459=CARTESIAN_POINT ( 'NONE',  ( 207.3874697692679945, 271.4413608369101780, -6.809237722377445401 ) ) ;
#87460=CARTESIAN_POINT ( 'NONE',  ( -22.42236680055709641, 157.8615022471902591, 0.000000000000000000 ) ) ;
#87461=CARTESIAN_POINT ( 'NONE',  ( 147.1603453755519695, 275.7578002805973370, -5.230822882238410187 ) ) ;
#87462=CARTESIAN_POINT ( 'NONE',  ( 185.6713631041849055, 258.9584525764907426, -6.747383155299178092 ) ) ;
#87463=CARTESIAN_POINT ( 'NONE',  ( 164.1259971043086239, 246.3724295028720519, 5.761669507629934905 ) ) ;
#87464=CARTESIAN_POINT ( 'NONE',  ( 147.2180753513904961, 275.6578090293250511, 0.4909717733184589261 ) ) ;
#87465=CARTESIAN_POINT ( 'NONE',  ( 189.8533352240220893, 301.8113727360248504, -0.2033756396389863053 ) ) ;
#87467=CARTESIAN_POINT ( 'NONE',  ( 181.4283053378885597, 267.7238133557910373, 16.48022347432943135 ) ) ;
#87468=CARTESIAN_POINT ( 'NONE',  ( 106.6423081075360813, 238.5024278399160949, -9.188101187500093303 ) ) ;
#87472=CARTESIAN_POINT ( 'NONE',  ( 35.10161425989549855, 202.6199935810940929, 2.679491924311251605 ) ) ;
#87473=CARTESIAN_POINT ( 'NONE',  ( 195.8627871995700502, 291.4026965887302936, 17.41145040657729481 ) ) ;
#87474=CARTESIAN_POINT ( 'NONE',  ( 185.5154138499543990, 288.0851626838443735, 14.99196749104353366 ) ) ;
#87475=CARTESIAN_POINT ( 'NONE',  ( 204.5925719030185803, 272.9227966449359997, -9.752334820156695727 ) ) ;
#87476=VERTEX_POINT ( 'NONE', #18525 ) ;
#87477=CARTESIAN_POINT ( 'NONE',  ( 189.6299445318082348, 261.2437137164477008, -4.504590422874706235 ) ) ;
#87478=CARTESIAN_POINT ( 'NONE',  ( 196.9728329903666122, 289.4800408803428695, -17.53478045286815856 ) ) ;
#87479=CARTESIAN_POINT ( 'NONE',  ( 190.3641678128861656, 300.0032373684350659, 4.431439196076422782 ) ) ;
#87480=CARTESIAN_POINT ( 'NONE',  ( 175.9678860382099685, 292.6092798174653353, -1.135237467879147699 ) ) ;
#87482=ORIENTED_EDGE ( 'NONE', *, *, #80161, .T. ) ;
#87484=CARTESIAN_POINT ( 'NONE',  ( 181.0697057238064644, 271.7990502603447567, 17.55876967510761233 ) ) ;
#87487=CARTESIAN_POINT ( 'NONE',  ( 155.5311623832600958, 261.6886619413561448, 17.00987194985870943 ) ) ;
#87490=CARTESIAN_POINT ( 'NONE',  ( 179.5358833587677907, 289.0109454785418848, 12.61662917182883525 ) ) ;
#87495=CARTESIAN_POINT ( 'NONE',  ( 191.9702732701751984, 288.0542607666495201, -15.86116857044228290 ) ) ;
#87498=CARTESIAN_POINT ( 'NONE',  ( 147.7785919239399846, 274.6869658471848652, -7.924750738206837397 ) ) ;
#87502=DIRECTION ( 'NONE',  ( -0.8660254037844387076, -0.4999999999999998890, -0.000000000000000000 ) ) ;
#87503=CARTESIAN_POINT ( 'NONE',  ( 151.3284628043366524, 268.5384091220288383, 14.49047510809488237 ) ) ;
#87504=EDGE_CURVE ( 'NONE', #104, #45744, #90221, .T. ) ;
#87507=CARTESIAN_POINT ( 'NONE',  ( 189.4688130559096635, 300.2814762872015422, 3.283936888853890679 ) ) ;
#87509=ORIENTED_EDGE ( 'NONE', *, *, #10193, .T. ) ;
#87510=ORIENTED_EDGE ( 'NONE', *, *, #25376, .F. ) ;
#87511=CARTESIAN_POINT ( 'NONE',  ( 178.3793764524178016, 261.0518008416202633, 12.17990814227386842 ) ) ;
#87512=ORIENTED_EDGE ( 'NONE', *, *, #4575, .T. ) ;
#87514=EDGE_LOOP ( 'NONE', ( #9694, #78617, #45939, #99887 ) ) ;
#87517=ORIENTED_EDGE ( 'NONE', *, *, #32054, .F. ) ;
#87518=CARTESIAN_POINT ( 'NONE',  ( 186.1994311542131868, 282.5051706948743799, -16.93927830648238597 ) ) ;
#87521=CARTESIAN_POINT ( 'NONE',  ( 147.8970867440366419, 274.4817267983439137, -7.002141163459742579 ) ) ;
#87522=CARTESIAN_POINT ( 'NONE',  ( 194.8244254126244357, 266.5110688616923653, 10.33380443192758591 ) ) ;
#87524=CARTESIAN_POINT ( 'NONE',  ( 201.0468719883840265, 282.4235983437597497, -16.59631526626950659 ) ) ;
#87527=CARTESIAN_POINT ( 'NONE',  ( 153.8473343600284977, 279.7776813690406925, 2.204527152494932807 ) ) ;
#87528=CARTESIAN_POINT ( 'NONE',  ( 117.0885659928033817, 250.6589784336661637, -6.496448406907675876E-16 ) ) ;
#87533=CARTESIAN_POINT ( 'NONE',  ( 203.5754129385376530, 276.1909035769679690, 13.33079715167354884 ) ) ;
#87534=CARTESIAN_POINT ( 'NONE',  ( 179.3580451049573981, 255.3422994520020950, 1.318133649256687745 ) ) ;
#87536=CARTESIAN_POINT ( 'NONE',  ( 147.1854439606469498, 275.7143282560145963, 4.140517173074471202 ) ) ;
#87537=CARTESIAN_POINT ( 'NONE',  ( 157.3877702592915568, 280.2823303078274648, -7.027478506402013103 ) ) ;
#87542=( BOUNDED_CURVE ( )  B_SPLINE_CURVE ( 2, ( #42383, #10507, #65688, #27209, #64200, #79944, #41387, #65202, #72330 ),
 .UNSPECIFIED., .F., .T. ) 
 B_SPLINE_CURVE_WITH_KNOTS ( ( 3, 2, 2, 2, 3 ),
 ( 0.6088709677419354982, 0.6102150537634408733, 0.6129032258064516236, 0.6155913978494623739, 0.6169354838709677491 ),
 .UNSPECIFIED. ) 
 CURVE ( )  GEOMETRIC_REPRESENTATION_ITEM ( )  RATIONAL_B_SPLINE_CURVE ( ( 0.9330127018922194093, 0.9330127018922194093, 1.000000000000000000, 0.8660254037844387076, 1.000000000000000000, 0.8660254037844387076, 1.000000000000000000, 0.9330127018922194093, 0.9330127018922194093 ) ) 
 REPRESENTATION_ITEM ( '' )  );
#87544=CARTESIAN_POINT ( 'NONE',  ( 184.2680897726975786, 272.7852115255601007, -16.27692906205965073 ) ) ;
#87548=CARTESIAN_POINT ( 'NONE',  ( 201.0208763613437952, 267.8406677295997156, -2.841550210549272037 ) ) ;
#87549=CARTESIAN_POINT ( 'NONE',  ( 151.7688039545068364, 267.7757158772707839, -15.79694986370314069 ) ) ;
#87551=CARTESIAN_POINT ( 'NONE',  ( 163.1691520398773321, 248.0297337694385931, 11.21816141384514331 ) ) ;
#87552=CARTESIAN_POINT ( 'NONE',  ( 153.3178590226085589, 270.2078922168774398, 14.03864727403227874 ) ) ;
#87553=CARTESIAN_POINT ( 'NONE',  ( 151.5065022431975876, 275.0122692438795866, -8.642473134862484585 ) ) ;
#87554=CYLINDRICAL_SURFACE ( 'NONE', #25239, 17.82106496071139645 ) ;
#87556=ADVANCED_FACE ( 'NONE', ( #9927 ), #40788, .T. ) ;
#87559=EDGE_CURVE ( 'NONE', #49074, #6076, #16453, .T. ) ;
#87561=CARTESIAN_POINT ( 'NONE',  ( 152.8107382695299918, 265.9710327055011589, 16.32045346488711246 ) ) ;
#87563=EDGE_CURVE ( 'NONE', #74702, #72615, #32215, .T. ) ;
#87566=CARTESIAN_POINT ( 'NONE',  ( -12.49048504844327390, 175.8464784336661637, 1.353441290958777525E-15 ) ) ;
#87567=CARTESIAN_POINT ( 'NONE',  ( 95.60083130504949622, 219.8768266524159856, -9.188101187500091527 ) ) ;
#87568=CARTESIAN_POINT ( 'NONE',  ( 155.6328838216860220, 261.0829332228125850, -17.51014940606912518 ) ) ;
#87570=CARTESIAN_POINT ( 'NONE',  ( 147.7588084490480185, 275.1283837748432575, 4.327974371148282984 ) ) ;
#87575=CARTESIAN_POINT ( 'NONE',  ( 164.1453682657562752, 284.0231398948004085, 5.767891135377496425 ) ) ;
#87576=CARTESIAN_POINT ( 'NONE',  ( -22.42236680055709641, 157.8615022471902591, 0.000000000000000000 ) ) ;
#87579=CARTESIAN_POINT ( 'NONE',  ( 207.8744451524485441, 270.5978947312061678, 6.164818021356627042 ) ) ;
#87582=CARTESIAN_POINT ( 'NONE',  ( 190.0534303668326288, 269.9073674132432643, 15.26070177760127322 ) ) ;
#87585=CARTESIAN_POINT ( 'NONE',  ( 44.66719160132967659, 208.8464784336661353, 1.353441290958777327E-15 ) ) ;
#87586=CARTESIAN_POINT ( 'NONE',  ( 175.9190705534530252, 265.3157217463270285, -16.43460560943317361 ) ) ;
#87587=CARTESIAN_POINT ( 'NONE',  ( 71.40607303893924040, 212.0333772461660544, 9.188101187500095079 ) ) ;
#87588=CARTESIAN_POINT ( 'NONE',  ( 207.2167723318516153, 271.7370174712370954, -6.606038862010207957 ) ) ;
#87591=CARTESIAN_POINT ( 'NONE',  ( 198.7408816115379864, 285.9624092822338071, -17.04496721243561197 ) ) ;
#87593=CARTESIAN_POINT ( 'NONE',  ( 22.01556172758404628, 173.5177522451417929, 5.000000000000051514 ) ) ;
#87596=CARTESIAN_POINT ( 'NONE',  ( -3.099174982164758951, 179.0177522451419350, 5.000000000000046185 ) ) ;
#87599=CARTESIAN_POINT ( 'NONE',  ( 83.72013207082297015, 209.9548013555409796, -4.594050593750042211 ) ) ;
#87603=CARTESIAN_POINT ( 'NONE',  ( 201.9081421151641962, 280.9318347251351611, 16.34854216200801247 ) ) ;
#87606=CARTESIAN_POINT ( 'NONE',  ( 124.7815979145579632, 254.3967562850346553, -4.648177544792955347E-16 ) ) ;
#87607=CARTESIAN_POINT ( 'NONE',  ( 124.0080952226617086, 255.7365022471903444, 2.944929066748280225E-16 ) ) ;
#87608=CARTESIAN_POINT ( 'NONE',  ( 204.6470611188870521, 276.1878878528713130, -13.02652554726987866 ) ) ;
#87613=CARTESIAN_POINT ( 'NONE',  ( 202.4323889586180201, 280.0238125565655878, 15.69595176008160919 ) ) ;
#87614=CARTESIAN_POINT ( 'NONE',  ( 150.5438776023515004, 278.3016033182416322, -9.804454847755098641E-05 ) ) ;
#87616=ORIENTED_EDGE ( 'NONE', *, *, #71819, .T. ) ;
#87619=CARTESIAN_POINT ( 'NONE',  ( 189.3598067383799730, 290.0015115173640083, 14.41535925276077812 ) ) ;
#87620=CARTESIAN_POINT ( 'NONE',  ( 167.4563744213245684, 247.8076185277009529, 3.554669314528694724 ) ) ;
#87622=VERTEX_POINT ( 'NONE', #8149 ) ;
#87627=EDGE_CURVE ( 'NONE', #28084, #47657, #57510, .T. ) ;
#87630=ORIENTED_EDGE ( 'NONE', *, *, #98347, .F. ) ;
#87633=CARTESIAN_POINT ( 'NONE',  ( 183.1481327660158342, 295.7621509781383793, 0.9827986306915983405 ) ) ;
#87634=CARTESIAN_POINT ( 'NONE',  ( 164.2712161151136172, 246.1209027979328710, 7.276091357954241445 ) ) ;
#87637=CARTESIAN_POINT ( 'NONE',  ( 154.9683083969241011, 262.2340116239618055, 18.33261662430134109 ) ) ;
#87638=CARTESIAN_POINT ( 'NONE',  ( 185.4446033158241960, 292.4306437117321025, -11.14656972876700003 ) ) ;
#87640=CARTESIAN_POINT ( 'NONE',  ( 164.1706088557112935, 246.2951596828278298, 5.725034427997321984 ) ) ;
#87642=CARTESIAN_POINT ( 'NONE',  ( 203.8566748796650359, 269.0194278887698260, 2.458571758291232978 ) ) ;
#87644=CARTESIAN_POINT ( 'NONE',  ( 90.56688509766992468, 223.0958772461660260, -9.188101187500095079 ) ) ;
#87645=ORIENTED_EDGE ( 'NONE', *, *, #54776, .F. ) ;
#87648=ORIENTED_EDGE ( 'NONE', *, *, #50620, .F. ) ;
#87649=CARTESIAN_POINT ( 'NONE',  ( 195.9058436374999701, 291.3281206506429726, -17.17388571147666809 ) ) ;
#87653=CARTESIAN_POINT ( 'NONE',  ( 191.0933613939813540, 299.6635844069401173, -8.689828987424775164 ) ) ;
#87654=DIRECTION ( 'NONE',  ( -0.8660254037844359321, -0.5000000000000051070, -0.000000000000000000 ) ) ;
#87655=CARTESIAN_POINT ( 'NONE',  ( 206.3018347371251195, 273.3217358710584790, -9.309724106897926177 ) ) ;
#87656=CARTESIAN_POINT ( 'NONE',  ( 162.4777017143181581, 249.2273608642169904, 10.60452504456504919 ) ) ;
#87658=CARTESIAN_POINT ( 'NONE',  ( 88.45577462806285496, 228.0024278399160664, -9.188101187500093303 ) ) ;
#87659=ORIENTED_EDGE ( 'NONE', *, *, #99968, .T. ) ;
#87661=CARTESIAN_POINT ( 'NONE',  ( 163.2256942281324541, 247.9317998266098471, -9.780520296312531059 ) ) ;
#87662=VERTEX_POINT ( 'NONE', #56739 ) ;
#87664=CARTESIAN_POINT ( 'NONE',  ( 165.5828704949435064, 285.3748741401371376, 0.6646079123997954419 ) ) ;
#87665=CARTESIAN_POINT ( 'NONE',  ( 186.0348036264326481, 259.0250182415348945, 6.435743254585703177 ) ) ;
#87666=CARTESIAN_POINT ( 'NONE',  ( 147.4771206202524354, 275.6046823160672830, -0.001107820683494442279 ) ) ;
#87670=CARTESIAN_POINT ( 'NONE',  ( 157.0019680973974801, 274.0489577305648368, 13.29051776178687838 ) ) ;
#87674=CARTESIAN_POINT ( 'NONE',  ( 174.9037822226496814, 284.1633774455944490, 13.90002592669620185 ) ) ;
#87677=CARTESIAN_POINT ( 'NONE',  ( 149.0769653949221549, 274.3756200000332797, 9.020936583412852983 ) ) ;
#87678=EDGE_CURVE ( 'NONE', #96454, #36629, #35803, .T. ) ;
#87679=CARTESIAN_POINT ( 'NONE',  ( 161.3193951073452581, 251.2336067582368742, 13.01220207292984377 ) ) ;
#87681=CARTESIAN_POINT ( 'NONE',  ( 167.6497685817575700, 249.8759886161104475, 7.693690790770736143 ) ) ;
#87684=CARTESIAN_POINT ( 'NONE',  ( 202.7344253759264916, 279.5006701360513830, -16.45903677349620864 ) ) ;
#87690=CARTESIAN_POINT ( 'NONE',  ( 207.5338226493333025, 271.1878702128032614, 6.432541580693135863 ) ) ;
#87691=CARTESIAN_POINT ( 'NONE',  ( 183.0285049134369899, 264.2983816328642774, 14.23074442033831488 ) ) ;
#87694=CARTESIAN_POINT ( 'NONE',  ( 91.00660716696484087, 234.8967562850347122, -4.648177544792955347E-16 ) ) ;
#87695=CARTESIAN_POINT ( 'NONE',  ( 180.7904606653500821, 273.2281357677318852, 16.74012675949395756 ) ) ;
#87696=CARTESIAN_POINT ( 'NONE',  ( 161.0980924722764769, 273.3945384687940532, -15.29422357739410110 ) ) ;
#87698=CARTESIAN_POINT ( 'NONE',  ( 186.1577919818338387, 274.1963684029099682, -17.47416603093387621 ) ) ;
#87699=CARTESIAN_POINT ( 'NONE',  ( 9.323050453024791295, 170.0643266524160140, 9.188101187500095079 ) ) ;
#87704=CARTESIAN_POINT ( 'NONE',  ( 204.1986089961618234, 275.4461207950287189, -12.65196423004078419 ) ) ;
#87706=CARTESIAN_POINT ( 'NONE',  ( 28.75397480679061601, 199.6589784336661353, -6.496448406907676862E-16 ) ) ;
#87707=DIRECTION ( 'NONE',  ( 0.4999999999999992784, -0.8660254037844390407, 0.000000000000000000 ) ) ;
#87710=CARTESIAN_POINT ( 'NONE',  ( 199.7952696689775109, 267.3031272996356620, -6.755464101794886211 ) ) ;
#87711=CARTESIAN_POINT ( 'NONE',  ( 107.6178230991326927, 221.3932355074535678, -2.679491924311248496 ) ) ;
#87712=CARTESIAN_POINT ( 'NONE',  ( 149.7104618599964851, 271.3408689643206344, 11.89409965450183293 ) ) ;
#87713=CARTESIAN_POINT ( 'NONE',  ( 182.5845504737252725, 280.2578898108608882, -16.09494218299740353 ) ) ;
#87716=CARTESIAN_POINT ( 'NONE',  ( 84.89261448506458407, 226.4865022471902876, -10.00000000000009592 ) ) ;
#87717=CARTESIAN_POINT ( 'NONE',  ( 83.66574516303663245, 229.1115022471903160, -5.000000000000047962 ) ) ;
#87720=CARTESIAN_POINT ( 'NONE',  ( 45.88512659934279014, 206.4869531367911009, 4.594050593750046652 ) ) ;
#87724=CARTESIAN_POINT ( 'NONE',  ( 190.9498149295421570, 299.9122141765958531, -5.138500224925297566 ) ) ;
#87727=CARTESIAN_POINT ( 'NONE',  ( 167.3994242795659488, 285.0697971307098442, 7.791926321083453288 ) ) ;
#87728=CARTESIAN_POINT ( 'NONE',  ( -5.676897265278508797, 155.9824982072973683, -6.972266317189433020E-16 ) ) ;
#87729=CARTESIAN_POINT ( 'NONE',  ( 193.2871234453870386, 295.8638770741889061, 14.00693169951743755 ) ) ;
#87732=CARTESIAN_POINT ( 'NONE',  ( 163.3706531435203146, 247.6807236201477735, 10.06957846017757241 ) ) ;
#87733=CARTESIAN_POINT ( 'NONE',  ( 196.7491951525289835, 289.8673929779723721, -16.35352603081977207 ) ) ;
#87735=ORIENTED_EDGE ( 'NONE', *, *, #21436, .T. ) ;
#87737=CARTESIAN_POINT ( 'NONE',  ( 15.54637163393425148, 191.3297689869269504, -2.679491924311252493 ) ) ;
#87740=CARTESIAN_POINT ( 'NONE',  ( 178.6316378771798554, 282.3279298503816221, 15.59256888213965198 ) ) ;
#87746=CARTESIAN_POINT ( 'NONE',  ( 187.0452942487604275, 272.6200080864273332, -15.85002353977101386 ) ) ;
#87747=CARTESIAN_POINT ( 'NONE',  ( 151.1448005994188577, 269.3082076351089995, -13.99603974239249737 ) ) ;
#87749=EDGE_LOOP ( 'NONE', ( #35473, #16638, #36688, #52755 ) ) ;
#87754=CARTESIAN_POINT ( 'NONE',  ( 204.7242223814549504, 276.0542406257275161, -13.93608974681376189 ) ) ;
#87755=CARTESIAN_POINT ( 'NONE',  ( 108.1307024963493149, 242.4244531367911293, -4.594050593750046652 ) ) ;
#87756=ADVANCED_FACE ( 'NONE', ( #43405 ), #55222, .T. ) ;
#87757=CARTESIAN_POINT ( 'NONE',  ( 196.2630260332681189, 290.7094625936034049, -17.43112004684450866 ) ) ;
#87758=CARTESIAN_POINT ( 'NONE',  ( 184.1488128701229812, 288.7864932478067885, -13.16340755393728834 ) ) ;
#87760=CARTESIAN_POINT ( 'NONE',  ( 208.2939409893161553, 269.8713066281881083, 2.523744790997269227 ) ) ;
#87763=CARTESIAN_POINT ( 'NONE',  ( 197.8977219949227049, 287.8780861330898801, 17.48564646125164046 ) ) ;
#87764=CARTESIAN_POINT ( 'NONE',  ( 204.6748560047368244, 275.6941871888094511, -12.57733492443129464 ) ) ;
#87765=CARTESIAN_POINT ( 'NONE',  ( 60.66220569506229765, 196.6423013555410080, -4.594050593750043987 ) ) ;
#87766=ADVANCED_FACE ( 'NONE', ( #47631 ), #5531, .F. ) ;
#87769=CARTESIAN_POINT ( 'NONE',  ( 98.24615118885414233, 215.9824982072973683, 3.021315404115420679E-15 ) ) ;
#87770=CARTESIAN_POINT ( 'NONE',  ( 172.9450931783573537, 271.2952670478148320, 16.43454517436645546 ) ) ;
#87772=VERTEX_POINT ( 'NONE', #6425 ) ;
#87775=CARTESIAN_POINT ( 'NONE',  ( 176.8722193823187183, 288.7079821761982430, 11.35092617276139393 ) ) ;
#87776=CARTESIAN_POINT ( 'NONE',  ( 184.5457051153594534, 294.3635293766698169, 10.03055039675435367 ) ) ;
#87778=CARTESIAN_POINT ( 'NONE',  ( 171.9484922859593041, 258.9508083473583042, -13.76153770011480937 ) ) ;
#87780=CARTESIAN_POINT ( 'NONE',  ( 160.4646087359858484, 258.1587684244410070, -17.17204240885691746 ) ) ;
#87781=CARTESIAN_POINT ( 'NONE',  ( 206.5103405372297232, 270.6423507306794249, 2.445296693522686748 ) ) ;
#87782=CARTESIAN_POINT ( 'NONE',  ( 149.3833831332874240, 271.9073859370555510, 11.40518020539810173 ) ) ;
#87783=CARTESIAN_POINT ( 'NONE',  ( 33.79711566178269777, 196.9865022471903444, 10.00000000000009415 ) ) ;
#87784=CARTESIAN_POINT ( 'NONE',  ( 164.2545401858843945, 246.1497863546213978, 2.275217130759496609 ) ) ;
#87786=CARTESIAN_POINT ( 'NONE',  ( 168.1601509168907569, 255.5064425537701993, 14.08313907349351446 ) ) ;
#87787=CARTESIAN_POINT ( 'NONE',  ( 164.4578252119609090, 245.7976863610386999, -6.211333091911165560 ) ) ;
#87788=CARTESIAN_POINT ( 'NONE',  ( 122.0685591603289026, 241.2833772461660544, -9.188101187500095079 ) ) ;
#87789=EDGE_LOOP ( 'NONE', ( #95700, #31091, #27646, #95028 ) ) ;
#87795=CARTESIAN_POINT ( 'NONE',  ( 174.9640303183041112, 252.5332431885451854, 5.182172288090916012 ) ) ;
#87799=CARTESIAN_POINT ( 'NONE',  ( 158.5026241661040558, 275.0849458030947972, -12.46164233742350902 ) ) ;
#87801=CARTESIAN_POINT ( 'NONE',  ( 205.9334673742153257, 273.9597668594684023, -10.28447216160094158 ) ) ;
#87806=CARTESIAN_POINT ( 'NONE',  ( 54.73473692032377613, 214.6589784336661637, -6.496448406907675876E-16 ) ) ;
#87809=CARTESIAN_POINT ( 'NONE',  ( 173.6395413452840728, 251.9775273180457873, 3.447188466571927457 ) ) ;
#87810=EDGE_CURVE ( 'NONE', #27127, #81475, #15328, .T. ) ;
#87811=B_SPLINE_SURFACE_WITH_KNOTS ( 'NONE', 3, 1, ( 
 ( #86483, #35083 ),
 ( #96436, #27000 ),
 ( #19428, #9424 ),
 ( #57884, #50284 ),
 ( #81237, #40299 ),
 ( #81727, #85988 ),
 ( #11811, #4182 ),
 ( #71241, #35588 ),
 ( #50777, #1834 ),
 ( #65987, #19905 ),
 ( #58376, #55010 ),
 ( #89352, #74104 ),
 ( #16516, #47411 ),
 ( #70717, #1332 ),
 ( #32214, #97410 ),
 ( #29972, #98898 ),
 ( #84225, #74617 ),
 ( #75101, #58857 ),
 ( #36072, #89826 ),
 ( #82237, #59356 ),
 ( #43675, #21872 ),
 ( #5679, #90834 ),
 ( #13778, #44656 ),
 ( #37074, #97900 ),
 ( #36568, #60849 ),
 ( #60353, #7163 ),
 ( #29480, #5190 ),
 ( #22372, #90332 ),
 ( #44165, #13306 ),
 ( #67475, #91312 ),
 ( #37557, #12813 ),
 ( #52758, #20402 ),
 ( #66973, #51271 ),
 ( #28475, #20909 ) ),
 .UNSPECIFIED., .T., .F., .F.,
 ( 4, 2, 2, 2, 2, 2, 2, 2, 2, 2, 2, 2, 2, 2, 2, 2, 4 ),
 ( 2, 2 ),
 ( 0.000000000000000000, 0.06250000000000000000, 0.1250000000000000000, 0.1875000000000000000, 0.2500000000000000000, 0.3125000000000000000, 0.3750000000000000000, 0.4375000000000000000, 0.5000000000000000000, 0.5625000000000000000, 0.6250000000000000000, 0.6875000000000000000, 0.7500000000000000000, 0.8125000000000000000, 0.8750000000000000000, 0.9375000000000000000, 1.000000000000000000 ),
 ( 0.000000000000000000, 1.000000000000000000 ),
 .UNSPECIFIED. ) ;
#87812=CARTESIAN_POINT ( 'NONE',  ( 172.0338011489890278, 260.6545490261862597, 14.59499001995644640 ) ) ;
#87813=CARTESIAN_POINT ( 'NONE',  ( 155.4155621527535800, 279.6985967190125848, -1.505547091306592478 ) ) ;
#87814=CARTESIAN_POINT ( 'NONE',  ( 170.8463542321686077, 287.4393069310528972, -8.645854640182026429 ) ) ;
#87815=CARTESIAN_POINT ( 'NONE',  ( 202.9881971861223917, 279.0611244672630278, -15.16231470264511927 ) ) ;
#87816=CARTESIAN_POINT ( 'NONE',  ( 157.5084939801577093, 271.0392582902702543, -14.68761352887457861 ) ) ;
#87817=CARTESIAN_POINT ( 'NONE',  ( 127.6706609892855369, 244.5177522451418497, -10.00000000000009592 ) ) ;
#87820=CARTESIAN_POINT ( 'NONE',  ( 160.4170979800060479, 258.1363065642061088, -17.22270422867546102 ) ) ;
#87821=CARTESIAN_POINT ( 'NONE',  ( -7.212535326543083158, 157.4548013555409796, -4.594050593750042211 ) ) ;
#87822=CARTESIAN_POINT ( 'NONE',  ( 42.06911538997637479, 207.3464784336661353, 1.353441290958777327E-15 ) ) ;
#87826=CARTESIAN_POINT ( 'NONE',  ( 189.9211050898329347, 290.8589279105092942, -14.43444364813599634 ) ) ;
#87827=CARTESIAN_POINT ( 'NONE',  ( 147.1249913145849177, 275.8190353104462815, 3.637773609013635223 ) ) ;
#87829=CARTESIAN_POINT ( 'NONE',  ( 50.52223126882174853, 206.6427522451419065, 10.00000000000009237 ) ) ;
#87830=CARTESIAN_POINT ( 'NONE',  ( 172.8951663193395234, 288.9549776225803157, 8.104654168245465584 ) ) ;
#87831=CARTESIAN_POINT ( 'NONE',  ( 180.9259186355868394, 256.3478317398164563, 1.329846375023655547 ) ) ;
#87835=ADVANCED_FACE ( 'NONE', ( #85974 ), #55976, .T. ) ;
#87836=CARTESIAN_POINT ( 'NONE',  ( 37.33338606056913989, 202.3615022471903160, 5.000000000000046185 ) ) ;
#87837=CARTESIAN_POINT ( 'NONE',  ( 185.0922654080720235, 294.3675542256470408, 9.847061582960922266 ) ) ;
#87839=CARTESIAN_POINT ( 'NONE',  ( -6.509410329615746171, 176.2369531367911293, -4.594050593750048428 ) ) ;
#87841=EDGE_CURVE ( 'NONE', #85448, #80622, #74594, .T. ) ;
#87842=CARTESIAN_POINT ( 'NONE',  ( 152.6615646578087819, 266.2294089801508221, 16.94722993326405813 ) ) ;
#87844=CARTESIAN_POINT ( 'NONE',  ( 206.5479446040613141, 272.8954610772809133, 10.74757481123993230 ) ) ;
#87847=CARTESIAN_POINT ( 'NONE',  ( 148.9322735291567597, 272.6887306911919495, -12.40988026045598858 ) ) ;
#87848=CARTESIAN_POINT ( 'NONE',  ( 177.8071669554300058, 260.6696581013277410, -13.92674055003218747 ) ) ;
#87850=CARTESIAN_POINT ( 'NONE',  ( 167.9901924881250181, 286.9604587259559594, 0.5049872151095315953 ) ) ;
#87852=CARTESIAN_POINT ( 'NONE',  ( 207.1328285129854976, 271.8824124304944689, 9.368303624280315489 ) ) ;
#87853=CARTESIAN_POINT ( 'NONE',  ( 152.8910811562359413, 278.3431035384439269, -4.654733895217889383 ) ) ;
#87856=ORIENTED_EDGE ( 'NONE', *, *, #71324, .T. ) ;
#87857=CARTESIAN_POINT ( 'NONE',  ( 152.5564169041443847, 266.8265214178677525, 15.57863003859133499 ) ) ;
#87858=CARTESIAN_POINT ( 'NONE',  ( 164.9971748156432056, 244.8635054444190757, -1.825016704039769788 ) ) ;
#87861=CARTESIAN_POINT ( 'NONE',  ( 155.4186054393023255, 261.4540742680644598, 17.05753227160644769 ) ) ;
#87862=ORIENTED_EDGE ( 'NONE', *, *, #25590, .T. ) ;
#87863=VERTEX_POINT ( 'NONE', #86971 ) ;
#87864=CARTESIAN_POINT ( 'NONE',  ( 138.7947376353724849, 239.3932355074535963, -2.679491924311248496 ) ) ;
#87871=DIRECTION ( 'NONE',  ( 0.4999999999999998890, -0.8660254037844385966, 0.000000000000000000 ) ) ;
#87873=AXIS2_PLACEMENT_3D ( 'NONE', #48133, #1043, #85699 ) ;
#87874=ORIENTED_EDGE ( 'NONE', *, *, #38388, .F. ) ;
#87875=CARTESIAN_POINT ( 'NONE',  ( 173.6846226408814573, 267.2224573121649769, 16.82899224521884207 ) ) ;
#87876=CARTESIAN_POINT ( 'NONE',  ( 169.1248369069356841, 276.0452466230211712, -15.48103994540444717 ) ) ;
#87877=CARTESIAN_POINT ( 'NONE',  ( 151.3635996277190827, 275.1454279078836862, -8.423308477353403489 ) ) ;
#87879=CARTESIAN_POINT ( 'NONE',  ( 170.7362026651413203, 255.3656839902395177, -11.44183947388228084 ) ) ;
#87883=EDGE_LOOP ( 'NONE', ( #79530, #27286, #25864, #92011 ) ) ;
#87884=CARTESIAN_POINT ( 'NONE',  ( 157.0081533241564102, 266.1116096007127112, -16.83218197677382122 ) ) ;
#87887=CARTESIAN_POINT ( 'NONE',  ( 162.1151829103941964, 273.8406652419924967, -15.84115298045961673 ) ) ;
#87889=CARTESIAN_POINT ( 'NONE',  ( 78.01622611019826081, 227.3967562850346837, -4.648177544792955347E-16 ) ) ;
#87891=CARTESIAN_POINT ( 'NONE',  ( 147.3528235038055811, 275.4244183831162900, 5.914741335832481184 ) ) ;
#87892=CARTESIAN_POINT ( 'NONE',  ( 180.5791919176537874, 291.4317077338294553, -9.732688088917043956 ) ) ;
#87894=CARTESIAN_POINT ( 'NONE',  ( 152.8107382695299918, 265.9710327055011589, 16.32045346488711246 ) ) ;
#87896=FACE_OUTER_BOUND ( 'NONE', #37978, .T. ) ;
#87901=CARTESIAN_POINT ( 'NONE',  ( 164.8616299252405213, 245.0982760813026857, 1.544363874765093625 ) ) ;
#87902=B_SPLINE_CURVE_WITH_KNOTS ( 'NONE', 3,
 ( #83437, #14504, #44387, #91042 ),
 .UNSPECIFIED., .F., .F.,
 ( 4, 4 ),
 ( 7.881068500304280180E-17, 0.004334768247277024505 ),
 .UNSPECIFIED. ) ;
#87908=CARTESIAN_POINT ( 'NONE',  ( 186.6673878995319455, 276.5074556901925007, 17.73048906045012529 ) ) ;
#87909=CARTESIAN_POINT ( 'NONE',  ( 171.4605843149748523, 259.7787113614812142, -14.34284248236907722 ) ) ;
#87911=CARTESIAN_POINT ( 'NONE',  ( 179.0976092565113902, 278.1804918307850585, -17.48872506936735505 ) ) ;
#87912=B_SPLINE_CURVE_WITH_KNOTS ( 'NONE', 3,
 ( #14318, #56297, #71532, #63411 ),
 .UNSPECIFIED., .F., .F.,
 ( 4, 4 ),
 ( 0.008452089677209189203, 0.01483908248598288238 ),
 .UNSPECIFIED. ) ;
#87913=CARTESIAN_POINT ( 'NONE',  ( 160.5146108177758890, 252.6275340369041942, -16.06237538655383545 ) ) ;
#87914=CARTESIAN_POINT ( 'NONE',  ( 190.7994525848730234, 261.9583232506778927, -0.5433290425362596876 ) ) ;
#87915=ORIENTED_EDGE ( 'NONE', *, *, #82821, .T. ) ;
#87916=CARTESIAN_POINT ( 'NONE',  ( 177.6785493476784552, 271.3070803369324153, -17.73189896442177016 ) ) ;
#87917=EDGE_CURVE ( 'NONE', #16332, #19447, #818, .T. ) ;
#87918=CARTESIAN_POINT ( 'NONE',  ( 164.3274319858398087, 246.0235340536434592, -1.770631424362269168 ) ) ;
#87919=CARTESIAN_POINT ( 'NONE',  ( 19.85049821812290816, 182.2677522451418497, 10.00000000000009592 ) ) ;
#87920=CARTESIAN_POINT ( 'NONE',  ( 105.6144235841895664, 219.5327760586659451, 1.948934522072302763E-15 ) ) ;
#87922=B_SPLINE_CURVE_WITH_KNOTS ( 'NONE', 3,
 ( #48346, #94986, #87916, #10355, #3269, #80798 ),
 .UNSPECIFIED., .F., .F.,
 ( 4, 2, 4 ),
 ( 0.02063947560780285406, 0.02520718459488528046, 0.02977489358196770339 ),
 .UNSPECIFIED. ) ;
#87923=CARTESIAN_POINT ( 'NONE',  ( 100.7282019964230244, 217.4155109091896065, 2.679491924311254714 ) ) ;
#87924=CARTESIAN_POINT ( 'NONE',  ( 207.8616498235123231, 270.6200568910230118, 3.132900500943239130 ) ) ;
#87926=CARTESIAN_POINT ( 'NONE',  ( 22.06942799527072907, 192.7369531367911293, -4.594050593750048428 ) ) ;
#87927=CARTESIAN_POINT ( 'NONE',  ( -27.42236680055714260, 166.5217562850347406, 1.224646799147364892E-15 ) ) ;
#87931=CARTESIAN_POINT ( 'NONE',  ( 179.0484917649878298, 259.9789987921100192, 12.89662402083353854 ) ) ;
#87933=CYLINDRICAL_SURFACE ( 'NONE', #53084, 10.00000000000010658 ) ;
#87934=CARTESIAN_POINT ( 'NONE',  ( 207.8570869662935365, 270.6279599915536664, -5.669188455878507504 ) ) ;
#87935=CARTESIAN_POINT ( 'NONE',  ( 182.4691726830119194, 284.2328283816569865, 14.94772914765149530 ) ) ;
#87937=CARTESIAN_POINT ( 'NONE',  ( 46.18343024948246978, 185.2202760586659451, -5.415160957724236172E-17 ) ) ;
#87938=CARTESIAN_POINT ( 'NONE',  ( 81.69914580506156199, 224.6427522451419065, 10.00000000000009237 ) ) ;
#87939=VERTEX_POINT ( 'NONE', #44775 ) ;
#87941=DIRECTION ( 'NONE',  ( 0.4999999999999992784, -0.8660254037844390407, 0.000000000000000000 ) ) ;
#87942=EDGE_CURVE ( 'NONE', #46058, #32613, #92722, .T. ) ;
#87943=CARTESIAN_POINT ( 'NONE',  ( -2.098180203030011182, 181.8464784336661353, 1.353441290958777327E-15 ) ) ;
#87945=CARTESIAN_POINT ( 'NONE',  ( 151.4188942279983223, 268.3817773016460251, -14.77302265413830895 ) ) ;
#87946=CARTESIAN_POINT ( 'NONE',  ( 186.4826759020093334, 282.7967963076828823, 16.16522040270928784 ) ) ;
#87947=CARTESIAN_POINT ( 'NONE',  ( 192.8301672656986341, 296.6553483942417415, -13.40355799340913556 ) ) ;
#87948=DIRECTION ( 'NONE',  ( 0.8660254037844395958, 0.4999999999999985567, 0.000000000000000000 ) ) ;
#87949=CARTESIAN_POINT ( 'NONE',  ( 163.8040269124969939, 246.9300982336122559, 6.025552750865228013 ) ) ;
#87950=CARTESIAN_POINT ( 'NONE',  ( 146.5046981847821428, 276.8934145268504494, 0.02269072295920678689 ) ) ;
#87951=CARTESIAN_POINT ( 'NONE',  ( 207.6477529416552557, 270.9905371579805546, 7.447146952410988341 ) ) ;
#87953=CARTESIAN_POINT ( 'NONE',  ( -8.638129123654804786, 172.4865022471903160, -10.00000000000009415 ) ) ;
#87954=CARTESIAN_POINT ( 'NONE',  ( 16.68515570176661811, 168.8932355074535678, -2.679491924311248496 ) ) ;
#87955=CARTESIAN_POINT ( 'NONE',  ( 119.4704829489755724, 239.7833772461660544, -9.188101187500095079 ) ) ;
#87960=CARTESIAN_POINT ( 'NONE',  ( 157.0848929289108469, 258.5679796760466047, 17.57466231005294688 ) ) ;
#87961=CARTESIAN_POINT ( 'NONE',  ( 185.7606924044570462, 288.4259988650926516, 15.28553487407920386 ) ) ;
#87964=CARTESIAN_POINT ( 'NONE',  ( 189.9217467546592104, 261.7193677635744962, -4.432260095178574666 ) ) ;
#87965=CARTESIAN_POINT ( 'NONE',  ( 149.5390997184345281, 271.6376768999995761, -11.52989534384373016 ) ) ;
#87967=CARTESIAN_POINT ( 'NONE',  ( 176.0908325915940793, 292.6123105786978726, -1.131283208944192431 ) ) ;
#87970=CARTESIAN_POINT ( 'NONE',  ( 189.1378126190901980, 265.5228191422445434, 11.86773559132568323 ) ) ;
#87971=CARTESIAN_POINT ( 'NONE',  ( 175.6080711066265110, 278.5854651567873930, 15.44675607434413855 ) ) ;
#87972=CARTESIAN_POINT ( 'NONE',  ( 168.7748138323674709, 271.7814369042428098, -16.73069365461695668 ) ) ;
#87973=CARTESIAN_POINT ( 'NONE',  ( 196.8684470336377501, 271.1649120511164028, 12.04039631205532679 ) ) ;
#87976=CARTESIAN_POINT ( 'NONE',  ( 192.2943420783192323, 297.5834248427583475, 12.53393473147773562 ) ) ;
#87980=CARTESIAN_POINT ( 'NONE',  ( 174.0334219321320575, 272.1732822737818083, -16.75381009008792788 ) ) ;
#87982=CARTESIAN_POINT ( 'NONE',  ( 163.8309440367553975, 279.3941924811222179, 12.19413334027601081 ) ) ;
#87983=CARTESIAN_POINT ( 'NONE',  ( 148.2352135776142177, 273.8960739431854563, -9.245976304249309052 ) ) ;
#87988=CARTESIAN_POINT ( 'NONE',  ( 191.0816511748900268, 299.6838671013740623, 7.311127128005925790 ) ) ;
#87991=CARTESIAN_POINT ( 'NONE',  ( 189.6420494643790278, 300.2261056104030104, 3.258464925664200429 ) ) ;
#87992=CARTESIAN_POINT ( 'NONE',  ( 203.5477091018662748, 278.0920214017542662, -16.09930363698006062 ) ) ;
#87995=EDGE_CURVE ( 'NONE', #43017, #19180, #36560, .T. ) ;
#87996=CARTESIAN_POINT ( 'NONE',  ( -22.42236680055709641, 157.8615022471902591, 0.000000000000000000 ) ) ;
#87998=DIRECTION ( 'NONE',  ( -0.5000000000000006661, 0.8660254037844382635, -1.877843081442121204E-16 ) ) ;
#87999=ORIENTED_EDGE ( 'NONE', *, *, #93507, .T. ) ;
#88002=CARTESIAN_POINT ( 'NONE',  ( 202.9881971861223917, 279.0611244672630278, -15.16231470264511927 ) ) ;
#88003=ORIENTED_EDGE ( 'NONE', *, *, #14715, .F. ) ;
#88004=CARTESIAN_POINT ( 'NONE',  ( 186.1755760447797456, 282.4646021076670195, -16.83160945059842462 ) ) ;
#88006=CARTESIAN_POINT ( 'NONE',  ( 160.5948787015109360, 254.3126484189558880, -15.26349502958301585 ) ) ;
#88007=CARTESIAN_POINT ( 'NONE',  ( 158.6960675524883584, 274.7800521535589269, -12.92120065756460079 ) ) ;
#88008=CARTESIAN_POINT ( 'NONE',  ( 192.9633865298379476, 296.4246058602058156, -11.85717392250713864 ) ) ;
#88012=CARTESIAN_POINT ( 'NONE',  ( 154.3430704429289619, 279.5595050419421455, 2.149449913245343069 ) ) ;
#88013=CARTESIAN_POINT ( 'NONE',  ( 140.0925393287100178, 257.8149278399160949, -9.188101187500095079 ) ) ;
#88016=ORIENTED_EDGE ( 'NONE', *, *, #34513, .T. ) ;
#88020=FACE_OUTER_BOUND ( 'NONE', #55249, .T. ) ;
#88021=CARTESIAN_POINT ( 'NONE',  ( 186.8123841630082040, 258.3999256946553942, 3.104652050626591553 ) ) ;
#88022=CARTESIAN_POINT ( 'NONE',  ( 192.1545761101252481, 297.8255066008389349, 12.36758039018573108 ) ) ;
#88023=CARTESIAN_POINT ( 'NONE',  ( 153.0319512166365712, 277.3779982626183482, 6.711626137538481807 ) ) ;
#88025=CARTESIAN_POINT ( 'NONE',  ( 176.9795757823318638, 289.3634148552241641, -8.962721485982672931 ) ) ;
#88026=CARTESIAN_POINT ( 'NONE',  ( 171.3220061097250948, 280.3562742204175038, 13.76436716405364891 ) ) ;
#88028=CARTESIAN_POINT ( 'NONE',  ( 176.6970911207717165, 255.7224310037160535, -7.285259763286168422 ) ) ;
#88029=ORIENTED_EDGE ( 'NONE', *, *, #73314, .F. ) ;
#88030=CARTESIAN_POINT ( 'NONE',  ( 194.2154056360670040, 294.2560451561701029, -15.66696967429384557 ) ) ;
#88034=CARTESIAN_POINT ( 'NONE',  ( 163.9104742396420704, 278.2281419285811239, 13.48933418416708996 ) ) ;
#88036=CARTESIAN_POINT ( 'NONE',  ( 200.9679874475659460, 267.7110922426995785, -2.589691348594355791 ) ) ;
#88037=CARTESIAN_POINT ( 'NONE',  ( 192.0613504677270384, 297.9869781500409545, -10.79912279808309350 ) ) ;
#88039=CARTESIAN_POINT ( 'NONE',  ( 162.9466247808429102, 248.4151622881552441, 11.25765811906727443 ) ) ;
#88043=ORIENTED_EDGE ( 'NONE', *, *, #35208, .F. ) ;
#88044=B_SPLINE_SURFACE_WITH_KNOTS ( 'NONE', 3, 1, ( 
 ( #64512, #81741 ),
 ( #33615, #95470 ),
 ( #26023, #97423 ),
 ( #29982, #13315 ),
 ( #89841, #52282 ),
 ( #14783, #44176 ),
 ( #82747, #20414 ),
 ( #90846, #6691 ),
 ( #75113, #51282 ),
 ( #60861, #27992 ),
 ( #36082, #74119 ),
 ( #45179, #58871 ),
 ( #68475, #21398 ),
 ( #37084, #13789 ),
 ( #82251, #44665 ),
 ( #12824, #5689 ),
 ( #4713, #67485 ),
 ( #75601, #99404 ),
 ( #91824, #83223 ),
 ( #67988, #6188 ),
 ( #84234, #98908 ),
 ( #29489, #36579 ),
 ( #60364, #28485 ),
 ( #29007, #59367 ),
 ( #22384, #91323 ),
 ( #5201, #35599 ),
 ( #21883, #66984 ),
 ( #52769, #43686 ),
 ( #74627, #83729 ),
 ( #76118, #98415 ),
 ( #53282, #97911 ),
 ( #66497, #90343 ),
 ( #20922, #14292 ),
 ( #37568, #51805 ) ),
 .UNSPECIFIED., .T., .F., .F.,
 ( 4, 2, 2, 2, 2, 2, 2, 2, 2, 2, 2, 2, 2, 2, 2, 2, 4 ),
 ( 2, 2 ),
 ( 0.000000000000000000, 0.06250000000000000000, 0.1250000000000000000, 0.1875000000000000000, 0.2500000000000000000, 0.3125000000000000000, 0.3750000000000000000, 0.4375000000000000000, 0.5000000000000000000, 0.5625000000000000000, 0.6250000000000000000, 0.6875000000000000000, 0.7500000000000000000, 0.8125000000000000000, 0.8750000000000000000, 0.9375000000000000000, 1.000000000000000000 ),
 ( 0.000000000000000000, 1.000000000000000000 ),
 .UNSPECIFIED. ) ;
#88051=CARTESIAN_POINT ( 'NONE',  ( 202.3421728196210552, 280.1800714929709670, 16.85915999540957344 ) ) ;
#88052=CARTESIAN_POINT ( 'NONE',  ( -13.97887943725652882, 171.9244531367911293, -4.594050593750046652 ) ) ;
#88053=CARTESIAN_POINT ( 'NONE',  ( 102.6097905472235539, 239.2369531367911009, -4.594050593750048428 ) ) ;
#88056=CARTESIAN_POINT ( 'NONE',  ( 183.3634088509504352, 284.6525016221286251, -16.42631288611494256 ) ) ;
#88057=EDGE_CURVE ( 'NONE', #69571, #14857, #96319, .T. ) ;
#88059=CARTESIAN_POINT ( 'NONE',  ( 164.1651990362067011, 284.0577512603656487, 5.775159962432079297 ) ) ;
#88062=CARTESIAN_POINT ( 'NONE',  ( 161.7554271570718356, 250.4783770943820969, 12.69314527299759909 ) ) ;
#88069=CARTESIAN_POINT ( 'NONE',  ( 47.75258065019424691, 204.5024278399160949, 9.188101187500095079 ) ) ;
#88070=B_SPLINE_CURVE_WITH_KNOTS ( 'NONE', 3,
 ( #29584, #44276, #83824, #91926, #74221, #35692, #5783, #36671, #39148, #15355, #32063, #679, #47268, #99998, #70061, #7780, #16377, #85849, #86334, #55845, #40158, #16872, #38153, #31560, #46776, #62451, #77699, #47757, #94415, #63478, #92907, #93418, #46251, #78696, #71099, #62974, #86840, #23969, #78190, #70569, #9283, #23459, #53854, #8778, #84817, #54349, #85322, #1187, #92417, #77175 ),
 .UNSPECIFIED., .F., .F.,
 ( 4, 2, 2, 2, 2, 2, 2, 2, 2, 2, 2, 2, 2, 2, 2, 2, 2, 2, 2, 2, 2, 2, 2, 2, 4 ),
 ( 0.0002857323352533271284, 0.0007593487685542560112, 0.001232965201855184840, 0.001469773418505610114, 0.001588177526830845520, 0.001706581635156080492, 0.001943389851806547400, 0.002180198068457014308, 0.002653814501757891312, 0.003127430935058769183, 0.004074663801660423877, 0.005021896668262079873, 0.005495513101562916544, 0.005732321318213334446, 0.005850725426538501764, 0.005909927480701086290, 0.005969129534863669949, 0.006028331589026254475, 0.006087533643188839001, 0.006205937751514171118, 0.006442745968164699175, 0.006916362401465711920, 0.007153170618116217426, 0.007389978834766722064, 0.007863595268067727004 ),
 .UNSPECIFIED. ) ;
#88073=CARTESIAN_POINT ( 'NONE',  ( 86.64296780859545777, 211.6423013555409796, -4.594050593750043987 ) ) ;
#88074=CARTESIAN_POINT ( 'NONE',  ( 161.7767236248226084, 250.4414905302161287, -13.15904643207033153 ) ) ;
#88081=VERTEX_POINT ( 'NONE', #52884 ) ;
#88083=CARTESIAN_POINT ( 'NONE',  ( 75.51934661115031133, 226.6589784336661637, -6.496448406907676862E-16 ) ) ;
#88085=B_SPLINE_CURVE_WITH_KNOTS ( 'NONE', 3,
 ( #72874, #64755, #19170, #18658, #4956, #43427, #35835, #3943, #26251, #50528 ),
 .UNSPECIFIED., .F., .F.,
 ( 4, 2, 2, 2, 4 ),
 ( 2.752498918913566419E-15, 0.0004302583884043699046, 0.0008605167768059872367, 0.001290775165207604623, 0.001721033553609222118 ),
 .UNSPECIFIED. ) ;
#88088=CARTESIAN_POINT ( 'NONE',  ( 201.7463482373744910, 281.2120699418204595, 16.24774024092229396 ) ) ;
#88093=CARTESIAN_POINT ( 'NONE',  ( 127.8330407560430757, 234.6115022471901739, -5.000000000000041744 ) ) ;
#88094=CARTESIAN_POINT ( 'NONE',  ( 157.2104826425669728, 258.3504519110855995, -16.92635148710569482 ) ) ;
#88096=ORIENTED_EDGE ( 'NONE', *, *, #23354, .T. ) ;
#88098=ORIENTED_EDGE ( 'NONE', *, *, #38040, .T. ) ;
#88099=CARTESIAN_POINT ( 'NONE',  ( 202.6070187115982719, 279.7213449518906145, 15.56322169823762280 ) ) ;
#88100=CARTESIAN_POINT ( 'NONE',  ( 207.4437983686434848, 270.9555910830893026, -0.9151573623704182259 ) ) ;
#88106=CARTESIAN_POINT ( 'NONE',  ( 169.7479376959777824, 249.8559926079458933, 3.422520443736486673 ) ) ;
#88108=CARTESIAN_POINT ( 'NONE',  ( 153.4495116231415750, 264.8646448025247082, -16.73555355292144498 ) ) ;
#88113=CARTESIAN_POINT ( 'NONE',  ( -27.42236680055714260, 166.5217562850347406, 1.224646799147364892E-15 ) ) ;
#88117=CARTESIAN_POINT ( 'NONE',  ( 184.3226795282388650, 274.5458599865910969, 17.66928848808302988 ) ) ;
#88118=( BOUNDED_CURVE ( )  B_SPLINE_CURVE ( 2, ( #58404, #66512, #96463, #4211, #57913, #50310, #35108, #89377, #20939 ),
 .UNSPECIFIED., .F., .T. ) 
 B_SPLINE_CURVE_WITH_KNOTS ( ( 3, 2, 2, 2, 3 ),
 ( 0.9395161290322581182, 0.9408602150537634934, 0.9435483870967742437, 0.9462365591397849940, 0.9475806451612903691 ),
 .UNSPECIFIED. ) 
 CURVE ( )  GEOMETRIC_REPRESENTATION_ITEM ( )  RATIONAL_B_SPLINE_CURVE ( ( 0.9330127018922194093, 0.9330127018922194093, 1.000000000000000000, 0.8660254037844387076, 1.000000000000000000, 0.8660254037844387076, 1.000000000000000000, 0.9330127018922194093, 0.9330127018922194093 ) ) 
 REPRESENTATION_ITEM ( '' )  );
#88119=CARTESIAN_POINT ( 'NONE',  ( 204.1780753366177237, 277.0001950557890495, 14.05599973203924158 ) ) ;
#88120=CARTESIAN_POINT ( 'NONE',  ( 194.5298665426430489, 293.7113828889860656, -16.13302716640051315 ) ) ;
#88122=CARTESIAN_POINT ( 'NONE',  ( 154.8838596469624349, 262.3802811495310152, 18.07457254681616021 ) ) ;
#88124=CARTESIAN_POINT ( 'NONE',  ( 187.4334564798314489, 291.4426959843206077, -14.06091351875603479 ) ) ;
#88125=ADVANCED_FACE ( 'NONE', ( #83834 ), #36183, .T. ) ;
#88126=CARTESIAN_POINT ( 'NONE',  ( 208.1496619281015512, 270.1212052926800880, -4.495150198885598414 ) ) ;
#88130=CARTESIAN_POINT ( 'NONE',  ( 97.33288211261837830, 220.8768266524160140, 9.188101187500098632 ) ) ;
#88131=ORIENTED_EDGE ( 'NONE', *, *, #4972, .T. ) ;
#88133=CARTESIAN_POINT ( 'NONE',  ( 163.1014196328097512, 276.5356776938393750, -13.94729885495409860 ) ) ;
#88139=CARTESIAN_POINT ( 'NONE',  ( 206.8791291248445532, 272.3218326606039454, -10.16823074922856840 ) ) ;
#88140=CARTESIAN_POINT ( 'NONE',  ( 207.1811052634604380, 270.9586164604430678, -3.621044357883208775 ) ) ;
#88141=CARTESIAN_POINT ( 'NONE',  ( 89.59260651841245249, 222.5333772461660544, 9.188101187500095079 ) ) ;
#88142=ORIENTED_EDGE ( 'NONE', *, *, #75275, .F. ) ;
#88143=ORIENTED_EDGE ( 'NONE', *, *, #28918, .F. ) ;
#88146=ORIENTED_EDGE ( 'NONE', *, *, #30909, .T. ) ;
#88147=CARTESIAN_POINT ( 'NONE',  ( 185.9608592076092464, 288.5956984647530703, 15.36535719480430018 ) ) ;
#88148=CARTESIAN_POINT ( 'NONE',  ( 21.81709757609801770, 176.7365022471902307, 10.00000000000009948 ) ) ;
#88150=CARTESIAN_POINT ( 'NONE',  ( 138.2797325092426490, 241.4548013555409796, -4.594050593750042211 ) ) ;
#88152=CARTESIAN_POINT ( 'NONE',  ( -0.9341114727035790821, 160.2677522451418213, -5.000000000000041744 ) ) ;
#88155=CARTESIAN_POINT ( 'NONE',  ( 157.0482715255472215, 258.6314098073167997, 18.43444315619183271 ) ) ;
#88156=CARTESIAN_POINT ( 'NONE',  ( 160.6010507955586490, 275.6504566167214989, 12.84439325828979861 ) ) ;
#88158=CARTESIAN_POINT ( 'NONE',  ( 188.9774666975129662, 269.5299829227286068, 14.91052322670039132 ) ) ;
#88159=CARTESIAN_POINT ( 'NONE',  ( 175.1187049791955701, 283.7737228748806615, 13.32334552399349548 ) ) ;
#88162=CARTESIAN_POINT ( 'NONE',  ( 198.8382651030371449, 282.3441860183548329, -16.97453155116460977 ) ) ;
#88164=CARTESIAN_POINT ( 'NONE',  ( 200.2631011806900005, 283.7811292041749311, 18.23377125296567058 ) ) ;
#88166=CARTESIAN_POINT ( 'NONE',  ( 167.6693233113157646, 249.9456431551184039, 6.971576484633508208 ) ) ;
#88168=CARTESIAN_POINT ( 'NONE',  ( 177.9794308749766856, 291.2700001626445214, -6.136377113293979058 ) ) ;
#88170=CARTESIAN_POINT ( 'NONE',  ( 198.3697893717576051, 274.2502983357130120, 15.02126222074246797 ) ) ;
#88176=EDGE_CURVE ( 'NONE', #18677, #69383, #42474, .T. ) ;
#88179=CARTESIAN_POINT ( 'NONE',  ( 183.1223740192843081, 274.6153891519672356, 16.37435194274504369 ) ) ;
#88182=CARTESIAN_POINT ( 'NONE',  ( 20.58138070222249638, 176.5643266524160140, -9.188101187500093303 ) ) ;
#88184=ORIENTED_EDGE ( 'NONE', *, *, #87995, .T. ) ;
#88185=ADVANCED_FACE ( 'NONE', ( #62459 ), #24978, .T. ) ;
#88188=CARTESIAN_POINT ( 'NONE',  ( 38.06444208900335013, 180.5327760586659736, 1.948934522072302763E-15 ) ) ;
#88190=CARTESIAN_POINT ( 'NONE',  ( 147.4963928429778264, 275.1757489932608109, 4.929816573182678852 ) ) ;
#88192=CARTESIAN_POINT ( 'NONE',  ( 199.6026874660839781, 267.3423861812402720, -6.701379308517451783 ) ) ;
#88193=CARTESIAN_POINT ( 'NONE',  ( 146.7434471017767521, 276.4798892723637209, 0.7354350123930684102 ) ) ;
#88194=CARTESIAN_POINT ( 'NONE',  ( 149.0223506047763635, 272.5327126196219183, 12.70178612879041502 ) ) ;
#88195=CARTESIAN_POINT ( 'NONE',  ( 182.5027709831066431, 280.4898292648059055, -16.09026386679935783 ) ) ;
#88196=CARTESIAN_POINT ( 'NONE',  ( 169.9836960595253572, 273.3332435997890570, -17.42200768236145336 ) ) ;
#88201=CARTESIAN_POINT ( 'NONE',  ( 82.43887584100865240, 231.7365022471903160, 2.944929066748280225E-16 ) ) ;
#88204=CARTESIAN_POINT ( 'NONE',  ( 39.90439897628026955, 193.8458772461660544, 9.188101187500095079 ) ) ;
#88205=CARTESIAN_POINT ( 'NONE',  ( 198.2114954873088948, 287.3346145022089786, 18.52864136173620935 ) ) ;
#88208=CARTESIAN_POINT ( 'NONE',  ( 190.5653282632609091, 300.5781646174276602, -5.775635208185608604 ) ) ;
#88209=DIRECTION ( 'NONE',  ( -0.8660254037844387076, -0.4999999999999998890, -0.000000000000000000 ) ) ;
#88210=EDGE_LOOP ( 'NONE', ( #90968, #78269, #87296, #28227 ) ) ;
#88211=CARTESIAN_POINT ( 'NONE',  ( 171.3427733889341482, 286.5388357190055331, 7.606204075628364869 ) ) ;
#88212=CARTESIAN_POINT ( 'NONE',  ( 206.9878665138179770, 272.1334939782196329, 6.566295309274049252 ) ) ;
#88213=CARTESIAN_POINT ( 'NONE',  ( 147.1448590109090162, 275.7846234509833607, 6.573501232734778377 ) ) ;
#88215=CARTESIAN_POINT ( 'NONE',  ( 188.3608790720148534, 265.1764494128112233, 10.74626820104000302 ) ) ;
#88217=CARTESIAN_POINT ( 'NONE',  ( 171.4196486961773189, 255.6818549069291748, 11.25747882315595305 ) ) ;
#88218=EDGE_LOOP ( 'NONE', ( #25801, #88258, #29121 ) ) ;
#88224=CARTESIAN_POINT ( 'NONE',  ( 175.8939073520130592, 252.7054158260212375, 5.280091837693253964 ) ) ;
#88225=CARTESIAN_POINT ( 'NONE',  ( 166.8902351030177726, 261.4103272712569606, 16.60908148647677862 ) ) ;
#88226=CARTESIAN_POINT ( 'NONE',  ( 177.4659907304532851, 255.7405978883358557, -6.896888922040105285 ) ) ;
#88232=CARTESIAN_POINT ( 'NONE',  ( 161.1061647010182583, 251.6029326557136585, -13.56144933775657613 ) ) ;
#88233=CYLINDRICAL_SURFACE ( 'NONE', #58853, 17.82106496071139645 ) ;
#88237=CARTESIAN_POINT ( 'NONE',  ( 175.4039180538638050, 286.4985578832265105, -12.71199677751706503 ) ) ;
#88240=CARTESIAN_POINT ( 'NONE',  ( 157.8696211474012330, 257.2087905314882619, -17.27527248276125604 ) ) ;
#88242=CARTESIAN_POINT ( 'NONE',  ( 113.7334117446687287, 224.2202760586659167, -5.415160957724236172E-17 ) ) ;
#88246=CARTESIAN_POINT ( 'NONE',  ( 207.6172352878830907, 271.0433952848413810, 3.316653249540578496 ) ) ;
#88247=ORIENTED_EDGE ( 'NONE', *, *, #73082, .T. ) ;
#88248=EDGE_CURVE ( 'NONE', #73611, #28264, #40632, .T. ) ;
#88253=CARTESIAN_POINT ( 'NONE',  ( 74.00414925029257063, 213.5333772461660544, 9.188101187500095079 ) ) ;
#88255=CARTESIAN_POINT ( 'NONE',  ( 151.2057546125658973, 268.7509459446807227, 15.78031848731319187 ) ) ;
#88256=CARTESIAN_POINT ( 'NONE',  ( 198.3452313965520375, 287.1029771126029573, 18.55943827821351988 ) ) ;
#88258=ORIENTED_EDGE ( 'NONE', *, *, #1692, .T. ) ;
#88261=ORIENTED_EDGE ( 'NONE', *, *, #69967, .T. ) ;
#88262=CARTESIAN_POINT ( 'NONE',  ( 153.6323727466833873, 269.3172676078306154, -15.66543061290010641 ) ) ;
#88263=CARTESIAN_POINT ( 'NONE',  ( 174.2197551875393629, 277.1311307515431395, -15.63619229037431069 ) ) ;
#88264=CARTESIAN_POINT ( 'NONE',  ( 207.2167723318516153, 271.7370174712370954, -6.606038862010207957 ) ) ;
#88266=CARTESIAN_POINT ( 'NONE',  ( 180.4366689915419784, 271.0272158672133855, 17.24581807274774548 ) ) ;
#88271=ORIENTED_EDGE ( 'NONE', *, *, #35650, .F. ) ;
#88272=CARTESIAN_POINT ( 'NONE',  ( 163.8947349411736525, 246.7729873192901664, -5.868803394723933309 ) ) ;
#88273=CARTESIAN_POINT ( 'NONE',  ( 123.0160347675418677, 232.6423013555409796, -4.594050593750043987 ) ) ;
#88276=CARTESIAN_POINT ( 'NONE',  ( 165.4781454232152953, 246.0304399151612245, -2.837517270351797016 ) ) ;
#88277=CARTESIAN_POINT ( 'NONE',  ( 166.2786698706664765, 279.3007919285489606, -14.16120680810289301 ) ) ;
#88278=CARTESIAN_POINT ( 'NONE',  ( 164.2851776226980860, 246.0967207574460929, 5.847738044744511754 ) ) ;
#88279=CARTESIAN_POINT ( 'NONE',  ( 0.9806730298622799991, 159.8262482093458061, 3.021315404115420679E-15 ) ) ;
#88280=CARTESIAN_POINT ( 'NONE',  ( 178.0312528307557898, 255.3900881702813024, 4.808504629698181709 ) ) ;
#88283=CARTESIAN_POINT ( 'NONE',  ( 158.2340186899420189, 275.5716318946143701, -12.34771995126616417 ) ) ;
#88284=CYLINDRICAL_SURFACE ( 'NONE', #71069, 10.00000000000010658 ) ;
#88286=CARTESIAN_POINT ( 'NONE',  ( 206.0316325540811704, 273.7897397804065918, -11.04223638802967322 ) ) ;
#88287=B_SPLINE_CURVE_WITH_KNOTS ( 'NONE', 3,
 ( #61806, #47115, #78034, #1029 ),
 .UNSPECIFIED., .F., .F.,
 ( 4, 4 ),
 ( 2.129127682876557597E-15, 0.004546946768845585782 ),
 .UNSPECIFIED. ) ;
#88288=CARTESIAN_POINT ( 'NONE',  ( 144.5855667544892924, 242.0327760586659451, 1.948934522072302763E-15 ) ) ;
#88290=CARTESIAN_POINT ( 'NONE',  ( -22.42236680055709641, 157.8615022471902591, 0.000000000000000000 ) ) ;
#88292=CARTESIAN_POINT ( 'NONE',  ( 73.32782722540972031, 203.9548013555409796, -4.594050593750042211 ) ) ;
#88293=CARTESIAN_POINT ( 'NONE',  ( 205.2937235227012707, 275.0678357141204629, -12.80017165135291535 ) ) ;
#88294=CARTESIAN_POINT ( 'NONE',  ( 181.4632975752175525, 255.1188003790442167, 1.936479460681336695 ) ) ;
#88296=CARTESIAN_POINT ( 'NONE',  ( 190.8138402884741254, 300.1477291634665789, 4.037153726988762514 ) ) ;
#88297=CARTESIAN_POINT ( 'NONE',  ( 155.4093994093388176, 279.7353005465348019, -1.380077325180699921 ) ) ;
#88298=CARTESIAN_POINT ( 'NONE',  ( 172.6200275220975300, 287.6579637919017500, -8.258093202231311381 ) ) ;
#88300=CARTESIAN_POINT ( 'NONE',  ( 202.7602807045765019, 279.4558873931827065, -15.90558713185497020 ) ) ;
#88301=CARTESIAN_POINT ( 'NONE',  ( 193.5548866660658121, 288.5596665684437312, 16.05153972607462975 ) ) ;
#88302=CARTESIAN_POINT ( 'NONE',  ( 143.1869494737568118, 240.1427522451417644, 1.119607411625061291E-15 ) ) ;
#88304=VERTEX_POINT ( 'NONE', #54358 ) ;
#88306=ADVANCED_FACE ( 'NONE', ( #15875 ), #34602, .F. ) ;
#88308=CARTESIAN_POINT ( 'NONE',  ( 160.5099781893591455, 258.1706592185460067, -17.21824937912870013 ) ) ;
#88309=CARTESIAN_POINT ( 'NONE',  ( -13.19395714113563045, 169.3149278399160949, -9.188101187500095079 ) ) ;
#88310=CARTESIAN_POINT ( 'NONE',  ( 32.78649236710315762, 198.9244531367911293, -4.594050593750046652 ) ) ;
#88311=CARTESIAN_POINT ( 'NONE',  ( 178.6233049832252107, 259.3218917414808971, -11.04666618235884279 ) ) ;
#88313=CARTESIAN_POINT ( 'NONE',  ( 38.03703169759612734, 192.7677522451418781, 10.00000000000009592 ) ) ;
#88314=CARTESIAN_POINT ( 'NONE',  ( 157.2104826425669728, 258.3504519110855995, -16.92635148710569482 ) ) ;
#88315=CARTESIAN_POINT ( 'NONE',  ( 192.0881900057259486, 293.2991038262234156, -14.57190693698760775 ) ) ;
#88316=CARTESIAN_POINT ( 'NONE',  ( 190.2648877593310317, 301.0985428348857340, -4.426259207433023590 ) ) ;
#88318=CARTESIAN_POINT ( 'NONE',  ( 66.16250339235085676, 220.5530062829863027, -4.648177544792955347E-16 ) ) ;
#88319=CARTESIAN_POINT ( 'NONE',  ( 62.71875570545262946, 207.0177522451418497, -10.00000000000009592 ) ) ;
#88320=CARTESIAN_POINT ( 'NONE',  ( 180.8696061126360348, 256.1446004347802159, 1.863214197090637958 ) ) ;
#88321=EDGE_CURVE ( 'NONE', #64907, #89705, #25026, .T. ) ;
#88322=CARTESIAN_POINT ( 'NONE',  ( 204.6713671561005299, 276.1457885614869951, -12.94307097876490431 ) ) ;
#88324=B_SPLINE_CURVE_WITH_KNOTS ( 'NONE', 3,
 ( #39066, #18307, #48706, #78104 ),
 .UNSPECIFIED., .F., .F.,
 ( 4, 4 ),
 ( 0.005060962031092128451, 0.01063827492794387417 ),
 .UNSPECIFIED. ) ;
#88325=EDGE_CURVE ( 'NONE', #28883, #42203, #28428, .T. ) ;
#88326=CARTESIAN_POINT ( 'NONE',  ( 33.79711566178269777, 196.9865022471903160, 10.00000000000009237 ) ) ;
#88327=FACE_OUTER_BOUND ( 'NONE', #3342, .T. ) ;
#88328=CARTESIAN_POINT ( 'NONE',  ( 149.8050492866161392, 271.5723974896224604, -11.69608657949948061 ) ) ;
#88329=CARTESIAN_POINT ( 'NONE',  ( -1.664820405372784862, 169.8458772461660544, 9.188101187500095079 ) ) ;
#88331=CARTESIAN_POINT ( 'NONE',  ( 162.5088600558392500, 251.8859699354127883, 13.03670156802715674 ) ) ;
#88332=CARTESIAN_POINT ( 'NONE',  ( 192.6470966816805230, 296.9724359471326807, 11.11268290051284424 ) ) ;
#88335=CARTESIAN_POINT ( 'NONE',  ( 207.4826643481121664, 271.2764789897469768, 7.783310782367018454 ) ) ;
#88336=CARTESIAN_POINT ( 'NONE',  ( 152.7043854946215049, 268.1552411151685078, 15.94764448997051964 ) ) ;
#88337=CARTESIAN_POINT ( 'NONE',  ( 176.9081908142109398, 260.3210854900437425, -13.74092692686856587 ) ) ;
#88338=( LENGTH_UNIT ( ) NAMED_UNIT ( * ) SI_UNIT ( .MILLI., .METRE. ) );
#88340=CARTESIAN_POINT ( 'NONE',  ( 153.2681147270651252, 277.6995928556744389, -5.735428835157149408 ) ) ;
#88342=CARTESIAN_POINT ( 'NONE',  ( 157.9207213236967675, 258.7415897385611743, 16.78933168291549194 ) ) ;
#88344=CARTESIAN_POINT ( 'NONE',  ( 153.1373638848023120, 277.6226180988243755, -5.202466352909343783 ) ) ;
#88345=CARTESIAN_POINT ( 'NONE',  ( 161.5515493166768977, 252.8315038724842623, 14.92355679770252053 ) ) ;
#88346=CARTESIAN_POINT ( 'NONE',  ( 206.2313482792274328, 273.4438219973828268, -9.403385562213845361 ) ) ;
#88348=CARTESIAN_POINT ( 'NONE',  ( 192.3401793061076717, 297.5040324353506094, 12.56432540404525611 ) ) ;
#88349=CARTESIAN_POINT ( 'NONE',  ( 207.4826643481121664, 271.2764789897469768, 7.783310782367018454 ) ) ;
#88354=ORIENTED_EDGE ( 'NONE', *, *, #91521, .T. ) ;
#88361=CARTESIAN_POINT ( 'NONE',  ( 174.6066048939933921, 262.0940252294753918, 15.79829227059981278 ) ) ;
#88369=CARTESIAN_POINT ( 'NONE',  ( 174.4001821373126404, 267.7328157961984516, 16.40384357689936934 ) ) ;
#88370=CARTESIAN_POINT ( 'NONE',  ( 166.2445671850063889, 273.7634225484549688, -16.23583275697997053 ) ) ;
#88371=VECTOR ( 'NONE', #50838, 1000.000000000000000 ) ;
#88372=CARTESIAN_POINT ( 'NONE',  ( -22.42236680055709641, 157.8615022471902591, 0.000000000000000000 ) ) ;
#88373=B_SPLINE_CURVE_WITH_KNOTS ( 'NONE', 3,
 ( #43947, #13086, #50554, #72903 ),
 .UNSPECIFIED., .F., .F.,
 ( 4, 4 ),
 ( 0.04183888476990187816, 0.04887120950165264183 ),
 .UNSPECIFIED. ) ;
#88375=EDGE_CURVE ( 'NONE', #48247, #68558, #82231, .T. ) ;
#88376=CARTESIAN_POINT ( 'NONE',  ( -22.42236680055709641, 157.8615022471902591, 0.000000000000000000 ) ) ;
#88377=CARTESIAN_POINT ( 'NONE',  ( 163.3706531435203146, 247.6807236201477735, 10.06957846017757241 ) ) ;
#88380=CARTESIAN_POINT ( 'NONE',  ( 157.0111464366968619, 266.1057930065318260, -17.09359609089053222 ) ) ;
#88383=CARTESIAN_POINT ( 'NONE',  ( 158.2450265141656018, 269.1956154815484297, 15.62383266220220968 ) ) ;
#88385=CARTESIAN_POINT ( 'NONE',  ( 168.7684621475002302, 272.8101242616207855, 15.98675317345763958 ) ) ;
#88386=CARTESIAN_POINT ( 'NONE',  ( 147.9364826856482864, 274.4134910258607079, 6.769466817982260132 ) ) ;
#88387=CARTESIAN_POINT ( 'NONE',  ( -22.42236680055709641, 157.8615022471902591, 0.000000000000000000 ) ) ;
#88388=CARTESIAN_POINT ( 'NONE',  ( -22.42236680055709641, 157.8615022471902591, 0.000000000000000000 ) ) ;
#88389=CARTESIAN_POINT ( 'NONE',  ( 150.5287101026835330, 271.9236214347867531, -12.89083132144543775 ) ) ;
#88390=CARTESIAN_POINT ( 'NONE',  ( 178.5528122206513046, 291.5498836112694221, 6.349106513625528692 ) ) ;
#88391=CARTESIAN_POINT ( 'NONE',  ( 196.9892929991941912, 289.4515313087606501, -17.86022972575499068 ) ) ;
#88392=ORIENTED_EDGE ( 'NONE', *, *, #29594, .T. ) ;
#88393=CARTESIAN_POINT ( 'NONE',  ( 92.14326550588401687, 235.5530062829863027, -4.648177544792955347E-16 ) ) ;
#88395=CARTESIAN_POINT ( 'NONE',  ( 164.7297297678022403, 245.3267338555121455, 3.020078936458732599 ) ) ;
#88398=ORIENTED_EDGE ( 'NONE', *, *, #21839, .F. ) ;
#88399=CARTESIAN_POINT ( 'NONE',  ( 190.4665781587570734, 300.7492048156811393, 6.617184385853465578 ) ) ;
#88401=CARTESIAN_POINT ( 'NONE',  ( -22.42236680055709641, 157.8615022471902591, 0.000000000000000000 ) ) ;
#88402=CARTESIAN_POINT ( 'NONE',  ( 122.4745085665788906, 241.5177522451418497, -10.00000000000009592 ) ) ;
#88404=CARTESIAN_POINT ( 'NONE',  ( 199.2279464128285724, 285.5740698558083182, -17.12749070589345024 ) ) ;
#88405=CARTESIAN_POINT ( 'NONE',  ( 190.4340612255839460, 300.8055257960429003, -1.331319038338205196 ) ) ;
#88406=ORIENTED_EDGE ( 'NONE', *, *, #20350, .T. ) ;
#88407=DIRECTION ( 'NONE',  ( 0.4999999999999998890, -0.8660254037844385966, 0.000000000000000000 ) ) ;
#88411=CARTESIAN_POINT ( 'NONE',  ( 25.04665064082949755, 195.2677522451419350, -5.000000000000047962 ) ) ;
#88412=CARTESIAN_POINT ( 'NONE',  ( 106.1553423657898492, 232.0958772461660260, -9.188101187500095079 ) ) ;
#88413=CARTESIAN_POINT ( 'NONE',  ( 172.0728039219370658, 285.9831811572526021, 11.38650458882361427 ) ) ;
#88415=CARTESIAN_POINT ( 'NONE',  ( 162.4777017143181581, 249.2273608642169904, 10.60452504456504919 ) ) ;
#88416=CARTESIAN_POINT ( 'NONE',  ( 30.27021345494340565, 176.0327760586659736, 1.948934522072303157E-15 ) ) ;
#88418=CARTESIAN_POINT ( 'NONE',  ( 161.4726291907278721, 250.9681975403669867, 14.52346149734912117 ) ) ;
#88420=ORIENTED_EDGE ( 'NONE', *, *, #51502, .T. ) ;
#88421=CARTESIAN_POINT ( 'NONE',  ( 186.4151829245328429, 260.6633168624404675, -5.822087422882750829 ) ) ;
#88422=SHAPE_REPRESENTATION ( 'Lead Screw Acme Drive Shaft', ( #68784 ), #59069 ) ;
#88427=CARTESIAN_POINT ( 'NONE',  ( 207.5785076975260779, 271.1104734389944042, -6.824813054587777650 ) ) ;
#88428=CARTESIAN_POINT ( 'NONE',  ( 182.5044606565503784, 284.2441587155593652, 14.95203780250641046 ) ) ;
#88429=CARTESIAN_POINT ( 'NONE',  ( 166.6595125297302502, 251.3695113782756323, 10.25274148534845864 ) ) ;
#88430=CARTESIAN_POINT ( 'NONE',  ( 39.47103917862304456, 205.8464784336661637, 1.353441290958777525E-15 ) ) ;
#88431=CARTESIAN_POINT ( 'NONE',  ( 86.10144160763246646, 220.5177522451418497, -10.00000000000009592 ) ) ;
#88432=ORIENTED_EDGE ( 'NONE', *, *, #4915, .T. ) ;
#88434=EDGE_CURVE ( 'NONE', #1543, #43165, #23853, .T. ) ;
#88437=CARTESIAN_POINT ( 'NONE',  ( 151.3999564459286375, 268.4145785023736153, -15.40574304386609050 ) ) ;
#88438=AXIS2_PLACEMENT_3D ( 'NONE', #90874, #41342, #2887 ) ;
#88440=CARTESIAN_POINT ( 'NONE',  ( 193.2140586456748679, 295.9904290195353269, -12.67640480829088823 ) ) ;
#88442=CARTESIAN_POINT ( 'NONE',  ( 204.7986527064648214, 275.9253235211867263, 14.74587861556245905 ) ) ;
#88443=EDGE_CURVE ( 'NONE', #18151, #10695, #17492, .T. ) ;
#88444=CARTESIAN_POINT ( 'NONE',  ( 191.7247331938518187, 298.5700163710982338, -9.650650827884682315 ) ) ;
#88445=CARTESIAN_POINT ( 'NONE',  ( 207.6727254509676186, 270.9472835030587703, 7.315149605389819953 ) ) ;
#88449=CARTESIAN_POINT ( 'NONE',  ( 207.8060684685902686, 270.7163266217015689, 2.015725026008670540 ) ) ;
#88450=CARTESIAN_POINT ( 'NONE',  ( -3.297639133650789756, 182.2365022471903444, 2.944929066748280225E-16 ) ) ;
#88452=CARTESIAN_POINT ( 'NONE',  ( 121.9063529450018137, 235.0643266524159856, -9.188101187500093303 ) ) ;
#88455=CARTESIAN_POINT ( 'NONE',  ( 46.16860155800336685, 185.9155109091895781, 2.679491924311254714 ) ) ;
#88457=CARTESIAN_POINT ( 'NONE',  ( 185.6554113515731217, 288.0628275752804370, 14.84040072038121139 ) ) ;
#88459=ORIENTED_EDGE ( 'NONE', *, *, #48506, .T. ) ;
#88460=CARTESIAN_POINT ( 'NONE',  ( 190.9061255863007318, 299.9878863388391892, 7.497146773253707153 ) ) ;
#88461=CARTESIAN_POINT ( 'NONE',  ( 149.4171629335945681, 271.8488776066536730, -11.42564036194071520 ) ) ;
#88462=CARTESIAN_POINT ( 'NONE',  ( 183.7496303464618279, 290.0633936972313904, 13.69834534244574442 ) ) ;
#88463=CARTESIAN_POINT ( 'NONE',  ( 176.3202518409931656, 292.2088383860199770, -1.100976535451413385 ) ) ;
#88465=VERTEX_POINT ( 'NONE', #40549 ) ;
#88467=FACE_OUTER_BOUND ( 'NONE', #88218, .T. ) ;
#88471=CARTESIAN_POINT ( 'NONE',  ( 179.4408063581041688, 277.4340371255875652, 17.62723233342114071 ) ) ;
#88473=CARTESIAN_POINT ( 'NONE',  ( 192.2185419806677942, 297.7147144631093170, 12.45868041609393728 ) ) ;
#88475=ADVANCED_FACE ( 'NONE', ( #2079 ), #41043, .T. ) ;
#88476=CARTESIAN_POINT ( 'NONE',  ( 190.9415060515185587, 280.7361723716825850, 16.66172594339581181 ) ) ;
#88478=CARTESIAN_POINT ( 'NONE',  ( 174.0797739608361780, 272.0896664596502887, -17.07181625714556361 ) ) ;
#88480=CARTESIAN_POINT ( 'NONE',  ( 163.9610465543719329, 279.7500988940785192, 12.43876487773592920 ) ) ;
#88481=CARTESIAN_POINT ( 'NONE',  ( 147.7467138384290308, 274.7421803109381813, -9.190172068879620682 ) ) ;
#88485=CARTESIAN_POINT ( 'NONE',  ( 185.4400636248849139, 291.0517812546900700, 12.13220115290137358 ) ) ;
#88490=CARTESIAN_POINT ( 'NONE',  ( 183.5502601116926940, 258.9811193475696314, -5.834672144206265010 ) ) ;
#88493=CARTESIAN_POINT ( 'NONE',  ( 176.9703162662242164, 260.2192451074442374, 12.27184398422452993 ) ) ;
#88498=CARTESIAN_POINT ( 'NONE',  ( 202.7602807045765019, 279.4558873931827065, -15.90558713185497020 ) ) ;
#88500=CARTESIAN_POINT ( 'NONE',  ( 182.8485886489254426, 280.3539150357451604, -16.11020329633530679 ) ) ;
#88502=CARTESIAN_POINT ( 'NONE',  ( 162.9152754634673101, 255.8478433609669480, -14.94487196607794566 ) ) ;
#88503=DIRECTION ( 'NONE',  ( 0.4999999999999998890, -0.8660254037844385966, 0.000000000000000000 ) ) ;
#88504=CARTESIAN_POINT ( 'NONE',  ( 193.1569697810063531, 296.0893098336876506, -13.02398914535779539 ) ) ;
#88505=CARTESIAN_POINT ( 'NONE',  ( 152.6692142062575499, 266.2161595735824449, -16.77985299603479419 ) ) ;
#88508=CARTESIAN_POINT ( 'NONE',  ( 139.4158702080621879, 260.4869531367911009, 4.594050593750046652 ) ) ;
#88512=ORIENTED_EDGE ( 'NONE', *, *, #42459, .F. ) ;
#88514=CARTESIAN_POINT ( 'NONE',  ( 199.9111308183154279, 270.2641321296042065, 9.500731247801665447 ) ) ;
#88515=ORIENTED_EDGE ( 'NONE', *, *, #41602, .T. ) ;
#88518=CARTESIAN_POINT ( 'NONE',  ( -8.295327404871391863, 176.0177522451419350, 5.000000000000046185 ) ) ;
#88519=DIRECTION ( 'NONE',  ( 0.5000000000000048850, -0.8660254037844358210, 0.000000000000000000 ) ) ;
#88520=CARTESIAN_POINT ( 'NONE',  ( 157.3938364985311011, 279.9930687026446776, -6.917094818336486206 ) ) ;
#88527=CARTESIAN_POINT ( 'NONE',  ( 185.1132493422790617, 273.1213101841942148, -16.83739034747381069 ) ) ;
#88529=VERTEX_POINT ( 'NONE', #88224 ) ;
#88530=CARTESIAN_POINT ( 'NONE',  ( 163.7274143833883784, 277.7048757494857227, 13.04941950082464430 ) ) ;
#88531=CARTESIAN_POINT ( 'NONE',  ( 201.3079779175387500, 267.1163987143520444, -2.193808737881617787 ) ) ;
#88532=CARTESIAN_POINT ( 'NONE',  ( 204.2538229384546469, 276.8689963608560447, -15.05174826659082221 ) ) ;
#88533=CARTESIAN_POINT ( 'NONE',  ( 190.6094661480870798, 300.5017155583701083, 4.598210453186021951 ) ) ;
#88534=CARTESIAN_POINT ( 'NONE',  ( 203.0507839702407580, 278.9527209772879814, 16.21318481136342626 ) ) ;
#88537=CARTESIAN_POINT ( 'NONE',  ( 167.1864846243946658, 248.1417588236094787, 6.437963532893948404 ) ) ;
#88546=CARTESIAN_POINT ( 'NONE',  ( 5.696048431029936410, 186.3464784336661637, 1.353441290958777525E-15 ) ) ;
#88547=CARTESIAN_POINT ( 'NONE',  ( 105.9931361504627603, 225.8768266524159856, -9.188101187500091527 ) ) ;
#88548=CARTESIAN_POINT ( 'NONE',  ( 154.8579861482817535, 262.4250953638155011, -17.69813260923097786 ) ) ;
#88550=CARTESIAN_POINT ( 'NONE',  ( 182.6933049510233218, 257.5106189887609958, -2.311194929639305951 ) ) ;
#88554=AXIS2_PLACEMENT_3D ( 'NONE', #31133, #54422, #85 ) ;
#88556=CARTESIAN_POINT ( 'NONE',  ( 148.2670916631250861, 273.8408594794321971, -7.980554973576580835 ) ) ;
#88557=CARTESIAN_POINT ( 'NONE',  ( 181.6650930950966085, 291.4988380269174968, 9.336250461819773250 ) ) ;
#88558=B_SPLINE_CURVE_WITH_KNOTS ( 'NONE', 3,
 ( #57809, #11251, #96364, #3641 ),
 .UNSPECIFIED., .F., .F.,
 ( 4, 4 ),
 ( 1.014933693205114626E-16, 0.0002129429434441837334 ),
 .UNSPECIFIED. ) ;
#88560=CARTESIAN_POINT ( 'NONE',  ( 164.2092127378751059, 246.2282957975508282, -5.762401283578112654 ) ) ;
#88561=CARTESIAN_POINT ( 'NONE',  ( 0.2927578493243047641, 177.6427522451419350, -10.00000000000009592 ) ) ;
#88565=EDGE_CURVE ( 'NONE', #734, #62639, #99683, .T. ) ;
#88570=CARTESIAN_POINT ( 'NONE',  ( 82.93520977470207356, 212.5643266524159856, -9.188101187500093303 ) ) ;
#88571=CARTESIAN_POINT ( 'NONE',  ( 207.2337123599961899, 271.7076764818092443, -5.443417788256701861 ) ) ;
#88573=FACE_OUTER_BOUND ( 'NONE', #21745, .T. ) ;
#88575=CARTESIAN_POINT ( 'NONE',  ( 199.7269368322551202, 284.7097930968712376, 17.25965714184168931 ) ) ;
#88577=CARTESIAN_POINT ( 'NONE',  ( 175.5673309417393568, 269.5851035110758289, -16.45774993793282448 ) ) ;
#88583=CARTESIAN_POINT ( 'NONE',  ( 69.94448162217048548, 217.3149278399160664, -9.188101187500095079 ) ) ;
#88585=CARTESIAN_POINT ( 'NONE',  ( 169.2047444088227053, 288.5477631478519243, -1.125125296904627925 ) ) ;
#88587=CARTESIAN_POINT ( 'NONE',  ( 191.6956933185365131, 288.0999053561845926, -15.81058546843402191 ) ) ;
#88589=CARTESIAN_POINT ( 'NONE',  ( 193.4121261747727942, 288.4174338016593424, 16.05890728405906032 ) ) ;
#88590=CARTESIAN_POINT ( 'NONE',  ( 175.4967466201937611, 291.2628096033125189, 6.560984766252938805 ) ) ;
#88591=CARTESIAN_POINT ( 'NONE',  ( 131.6579862894243433, 233.4865022471901455, 1.119607411625061291E-15 ) ) ;
#88592=CARTESIAN_POINT ( 'NONE',  ( 204.8385597977314490, 275.8562024115307167, -12.64672659107585240 ) ) ;
#88596=VERTEX_POINT ( 'NONE', #43031 ) ;
#88597=CARTESIAN_POINT ( 'NONE',  ( 202.8211298556536804, 279.3504935719197988, 17.07914446815911447 ) ) ;
#88600=ORIENTED_EDGE ( 'NONE', *, *, #75168, .T. ) ;
#88602=ORIENTED_EDGE ( 'NONE', *, *, #61502, .F. ) ;
#88603=CARTESIAN_POINT ( 'NONE',  ( 192.1581366030953859, 291.7909651536984370, 14.80011484029171953 ) ) ;
#88604=CARTESIAN_POINT ( 'NONE',  ( 167.5369157106011073, 247.4367840998064310, 3.630136079718237152 ) ) ;
#88605=CARTESIAN_POINT ( 'NONE',  ( 152.7045549149684405, 246.7202760586659736, -5.415160957724236172E-17 ) ) ;
#88606=CARTESIAN_POINT ( 'NONE',  ( 153.2283961777204695, 265.2476279883323400, -17.66880461074566000 ) ) ;
#88607=ORIENTED_EDGE ( 'NONE', *, *, #25559, .T. ) ;
#88610=CARTESIAN_POINT ( 'NONE',  ( 164.5588179998277383, 274.5918845762219576, 14.68862726419591169 ) ) ;
#88611=DIRECTION ( 'NONE',  ( 0.4999999999999992784, -0.8660254037844390407, 0.000000000000000000 ) ) ;
#88612=ORIENTED_EDGE ( 'NONE', *, *, #82386, .T. ) ;
#88613=ORIENTED_EDGE ( 'NONE', *, *, #95791, .T. ) ;
#88615=CARTESIAN_POINT ( 'NONE',  ( 164.1259971043086239, 246.3724295028720519, 5.761669507629934905 ) ) ;
#88616=CARTESIAN_POINT ( 'NONE',  ( 148.3253847707240141, 273.7398928553401447, -9.074433450356286457 ) ) ;
#88618=CARTESIAN_POINT ( 'NONE',  ( 169.9469112398214747, 250.9785751410766750, -8.718312767540300712 ) ) ;
#88621=CARTESIAN_POINT ( 'NONE',  ( 207.4789536975254691, 271.2829060250925295, -4.960982614616589181 ) ) ;
#88622=CARTESIAN_POINT ( 'NONE',  ( 166.5034556664195691, 265.5931899439500512, 16.54637507192525447 ) ) ;
#88623=CARTESIAN_POINT ( 'NONE',  ( 180.9962514683335257, 255.6518059654043782, 5.281628127585873855 ) ) ;
#88624=CARTESIAN_POINT ( 'NONE',  ( 99.30858933894288043, 218.9548013555409511, -4.594050593750042211 ) ) ;
#88628=CARTESIAN_POINT ( 'NONE',  ( 119.1467862834650902, 228.0494855054051584, -2.679491924311248496 ) ) ;
#88630=EDGE_LOOP ( 'NONE', ( #22886, #79760, #86879, #70476, #19159, #16898, #98045, #58245, #54669, #78970, #61605, #25784, #86591, #74635, #1710, #86881, #33224, #53405, #7809, #41825, #75192, #63741 ) ) ;
#88635=CARTESIAN_POINT ( 'NONE',  ( 177.3755417603144338, 293.4917590415172413, -2.831906106862874584 ) ) ;
#88639=CARTESIAN_POINT ( 'NONE',  ( 207.1917959879256728, 271.3993813902129659, -4.219514555173214276 ) ) ;
#88640=CARTESIAN_POINT ( 'NONE',  ( 95.54687826519547400, 213.7202760586659167, -5.415160957724236172E-17 ) ) ;
#88641=ORIENTED_EDGE ( 'NONE', *, *, #14398, .T. ) ;
#88647=CARTESIAN_POINT ( 'NONE',  ( 193.4694029979582979, 265.6208689502353764, -7.753311972763973436 ) ) ;
#88649=CARTESIAN_POINT ( 'NONE',  ( 123.8274129399422918, 251.4869531367911577, 4.594050593750046652 ) ) ;
#88651=CARTESIAN_POINT ( 'NONE',  ( -2.160980794731546695, 162.8927522451418213, -10.00000000000009059 ) ) ;
#88652=CARTESIAN_POINT ( 'NONE',  ( 172.9698904924519240, 250.6642211707864476, -4.168778760986519671 ) ) ;
#88653=ORIENTED_EDGE ( 'NONE', *, *, #27895, .F. ) ;
#88655=CARTESIAN_POINT ( 'NONE',  ( 204.4814917997891541, 276.4746623257233296, 13.21872368206963877 ) ) ;
#88656=CARTESIAN_POINT ( 'NONE',  ( 157.3881051607127119, 274.1628151507284201, 13.17500510233437261 ) ) ;
#88659=CARTESIAN_POINT ( 'NONE',  ( 114.3892930691446850, 248.3967562850347122, -4.648177544792955347E-16 ) ) ;
#88661=CARTESIAN_POINT ( 'NONE',  ( 199.0763421850443251, 281.8631602056879615, -16.59742191502687092 ) ) ;
#88663=CARTESIAN_POINT ( 'NONE',  ( 153.5960728533304405, 266.9358381153638788, 16.61214075660420519 ) ) ;
#88666=CARTESIAN_POINT ( 'NONE',  ( 159.9788992190088948, 253.5554137441726255, -15.81862932303382330 ) ) ;
#88668=CARTESIAN_POINT ( 'NONE',  ( 208.3790849386676598, 269.7238329819538762, -1.525282248498321946 ) ) ;
#88671=CARTESIAN_POINT ( 'NONE',  ( 182.1706919099075037, 264.0156754124984673, 13.98243676683973824 ) ) ;
#88673=ADVANCED_FACE ( 'NONE', ( #28347 ), #90201, .T. ) ;
#88677=CARTESIAN_POINT ( 'NONE',  ( 157.6561448699392827, 271.0329277901845444, -14.72207385342193220 ) ) ;
#88679=CARTESIAN_POINT ( 'NONE',  ( 19.17374232530777078, 188.0024278399161233, 9.188101187500095079 ) ) ;
#88682=AXIS2_PLACEMENT_3D ( 'NONE', #57089, #25197, #18620 ) ;
#88686=CARTESIAN_POINT ( 'NONE',  ( 208.1415148974628266, 270.1353163636768500, 3.453641150550738725 ) ) ;
#88688=CARTESIAN_POINT ( 'NONE',  ( 35.05980905203730913, 200.2369531367911293, -4.594050593750048428 ) ) ;
#88691=CARTESIAN_POINT ( 'NONE',  ( 147.5177358149801421, 275.1387818813681179, 4.867883209065928085 ) ) ;
#88693=CARTESIAN_POINT ( 'NONE',  ( 178.4130537636820009, 291.8182790410380676, 5.746090763460109940 ) ) ;
#88694=CARTESIAN_POINT ( 'NONE',  ( 191.7741832257749195, 298.4843664033717801, -8.615487418695501276 ) ) ;
#88696=CARTESIAN_POINT ( 'NONE',  ( 116.4844995237365453, 231.3927522451418497, 10.00000000000009948 ) ) ;
#88700=CARTESIAN_POINT ( 'NONE',  ( 81.57285043722427531, 211.2365022471902023, 10.00000000000009592 ) ) ;
#88703=CARTESIAN_POINT ( 'NONE',  ( 175.1378461883211912, 279.3152656845848583, 16.63146252814350134 ) ) ;
#88704=CARTESIAN_POINT ( 'NONE',  ( 46.39958950466356669, 197.5958772461660544, -9.188101187500095079 ) ) ;
#88707=CARTESIAN_POINT ( 'NONE',  ( 198.6363782946250183, 286.5986958926748116, -18.50260615857378355 ) ) ;
#88709=ORIENTED_EDGE ( 'NONE', *, *, #61906, .F. ) ;
#88711=CARTESIAN_POINT ( 'NONE',  ( 167.4364575273616822, 285.0497252248627547, 7.773533576968246983 ) ) ;
#88712=CARTESIAN_POINT ( 'NONE',  ( 207.6477529416552557, 270.9905371579805546, 7.447146952410988341 ) ) ;
#88715=CARTESIAN_POINT ( 'NONE',  ( 187.5114625740205270, 264.6447095084205330, 10.77906233194030250 ) ) ;
#88716=CARTESIAN_POINT ( 'NONE',  ( 190.9474291326297930, 266.7645650087163745, -12.82661358031884546 ) ) ;
#88717=CARTESIAN_POINT ( 'NONE',  ( 171.5429889697022645, 255.3861488387996701, 12.49561417135016406 ) ) ;
#88721=CARTESIAN_POINT ( 'NONE',  ( 173.1828068919900829, 254.0980817964978371, 8.310286840905920513 ) ) ;
#88722=CARTESIAN_POINT ( 'NONE',  ( 10.91961124514380366, 177.1115022471902307, 10.00000000000009592 ) ) ;
#88724=CARTESIAN_POINT ( 'NONE',  ( 178.6961944256588879, 282.3096576696289048, 15.48889775239164024 ) ) ;
#88725=CARTESIAN_POINT ( 'NONE',  ( 167.1103609241472157, 261.4346035182707055, 16.90549041653298445 ) ) ;
#88726=CARTESIAN_POINT ( 'NONE',  ( 32.38751264475774860, 201.0530062829863027, -4.648177544792955347E-16 ) ) ;
#88730=CIRCLE ( 'NONE', #32027, 16.82106496071145685 ) ;
#88731=CARTESIAN_POINT ( 'NONE',  ( 161.6755750489535046, 250.6166850027345276, -13.01404233079112061 ) ) ;
#88732=FACE_OUTER_BOUND ( 'NONE', #61104, .T. ) ;
#88733=CARTESIAN_POINT ( 'NONE',  ( 149.1429535397850827, 272.3238222086447990, -12.91457852089092384 ) ) ;
#88735=CARTESIAN_POINT ( 'NONE',  ( 206.7893622945242385, 272.4773133715531230, -10.52881283832460291 ) ) ;
#88736=CARTESIAN_POINT ( 'NONE',  ( 159.2511875226268216, 254.8158473755685520, 15.75855490706745599 ) ) ;
#88739=CARTESIAN_POINT ( 'NONE',  ( 205.2414727015710412, 275.1583367910551488, -12.71338796362297963 ) ) ;
#88740=CARTESIAN_POINT ( 'NONE',  ( 123.0160347675418677, 232.6423013555409796, -4.594050593750043987 ) ) ;
#88741=CARTESIAN_POINT ( 'NONE',  ( 106.7110898388691851, 243.9637435831425307, 2.679491924311251605 ) ) ;
#88743=ORIENTED_EDGE ( 'NONE', *, *, #40629, .T. ) ;
#88744=CARTESIAN_POINT ( 'NONE',  ( 208.3152833949211526, 269.8343404973242059, 2.763633873278860342 ) ) ;
#88747=CARTESIAN_POINT ( 'NONE',  ( 159.6978881494930249, 254.0421391940632532, 15.34888828951022610 ) ) ;
#88750=CARTESIAN_POINT ( 'NONE',  ( 75.30318735596920021, 214.2833772461660544, -9.188101187500095079 ) ) ;
#88753=CARTESIAN_POINT ( 'NONE',  ( 191.2729698983822288, 299.3524933518466469, 8.871011392605806734 ) ) ;
#88754=CARTESIAN_POINT ( 'NONE',  ( 193.9204722154232741, 294.7668848255750049, 15.43855698596013859 ) ) ;
#88755=CARTESIAN_POINT ( 'NONE',  ( 171.8605515403996833, 276.6437741024603838, 16.15068646528671437 ) ) ;
#88756=VERTEX_POINT ( 'NONE', #60721 ) ;
#88761=CARTESIAN_POINT ( 'NONE',  ( 148.0169957629716464, 274.2740382852624634, 9.106122941397371662 ) ) ;
#88763=EDGE_CURVE ( 'NONE', #82127, #73330, #36869, .T. ) ;
#88764=CARTESIAN_POINT ( 'NONE',  ( 207.3874697692679945, 271.4413608369101780, -6.809237722377445401 ) ) ;
#88766=VECTOR ( 'NONE', #57846, 1000.000000000000000 ) ;
#88769=CARTESIAN_POINT ( 'NONE',  ( 164.2813349609167517, 246.1033764428878214, 1.949810150281061638 ) ) ;
#88770=CARTESIAN_POINT ( 'NONE',  ( 206.1215120922853146, 273.6340638536760821, 10.12238414215620885 ) ) ;
#88771=DIRECTION ( 'NONE',  ( 0.4999999999999998890, -0.8660254037844385966, 0.000000000000000000 ) ) ;
#88772=CARTESIAN_POINT ( 'NONE',  ( 164.1998033881670551, 254.1351517766089501, 14.29502161760787438 ) ) ;
#88774=CARTESIAN_POINT ( 'NONE',  ( 208.3132655666949233, 269.8378354783333180, 2.688523655043302707 ) ) ;
#88776=CARTESIAN_POINT ( 'NONE',  ( 120.7695210546522446, 240.5333772461660544, 9.188101187500095079 ) ) ;
#88778=CARTESIAN_POINT ( 'NONE',  ( 146.5095091551180815, 276.8850816817948726, 0.1418322875769769398 ) ) ;
#88779=CARTESIAN_POINT ( 'NONE',  ( 87.40047971330913867, 221.2677522451418497, 10.00000000000009592 ) ) ;
#88788=CARTESIAN_POINT ( 'NONE',  ( -22.42236680055709641, 157.8615022471902591, 0.000000000000000000 ) ) ;
#88789=CARTESIAN_POINT ( 'NONE',  ( 206.7044739906782809, 272.6243442267827959, -10.28926534613781030 ) ) ;
#88792=DIRECTION ( 'NONE',  ( -0.8660254037844387076, -0.4999999999999998890, -0.000000000000000000 ) ) ;
#88793=CARTESIAN_POINT ( 'NONE',  ( 152.7980788416505220, 279.6030702425718459, 0.5086631364502993691 ) ) ;
#88794=B_SPLINE_CURVE_WITH_KNOTS ( 'NONE', 3,
 ( #89298, #3172, #34058, #4637, #64948, #87324, #65926, #95892, #96882, #81185, #73060, #3655, #26453, #4130, #57328, #88301, #18856, #79689, #34535, #57826, #19852, #88804, #50720, #81674, #17856, #50231, #43106, #2657, #10250, #41121 ),
 .UNSPECIFIED., .F., .F.,
 ( 4, 2, 2, 2, 2, 2, 2, 2, 2, 2, 2, 2, 2, 2, 4 ),
 ( 0.0004150180397800705846, 0.001518865485007307205, 0.002622712930234544042, 0.003174636652848163328, 0.003312617583501567715, 0.003381608048828311543, 0.003416103281491683456, 0.003450598514155055370, 0.003519588979481798330, 0.003588579444808541290, 0.003726560375461841594, 0.004002522236768397967, 0.004278484098074954341, 0.004554445959381510714, 0.004830407820688066220 ),
 .UNSPECIFIED. ) ;
#88795=B_SPLINE_CURVE_WITH_KNOTS ( 'NONE', 3,
 ( #75942, #98739, #29318, #60185 ),
 .UNSPECIFIED., .F., .F.,
 ( 4, 4 ),
 ( 0.01394906585337539820, 0.02027515528328900640 ),
 .UNSPECIFIED. ) ;
#88796=CARTESIAN_POINT ( 'NONE',  ( 157.8043799545718286, 257.3217915922150496, -17.97575562758749257 ) ) ;
#88797=CARTESIAN_POINT ( 'NONE',  ( 174.6137999045392064, 252.0957045990745939, 3.527324166098372515 ) ) ;
#88800=CARTESIAN_POINT ( 'NONE',  ( 148.9228818358559749, 272.7049975811580680, 12.13823097167056275 ) ) ;
#88802=CARTESIAN_POINT ( 'NONE',  ( 169.5047115304352872, 285.2286671053543614, -7.972866365725085558 ) ) ;
#88803=CARTESIAN_POINT ( 'NONE',  ( 154.8786460229866577, 262.3893114111486398, -18.06164891362396929 ) ) ;
#88804=CARTESIAN_POINT ( 'NONE',  ( 193.3797031396337047, 288.8503464183884262, 16.03552877166950452 ) ) ;
#88806=CARTESIAN_POINT ( 'NONE',  ( 145.0633378486230072, 247.8927522451418213, 10.00000000000009592 ) ) ;
#88809=EDGE_CURVE ( 'NONE', #36428, #40233, #28891, .T. ) ;
#88810=CARTESIAN_POINT ( 'NONE',  ( 157.4656258344471098, 257.9085309395441641, 18.30485740784190796 ) ) ;
#88811=CARTESIAN_POINT ( 'NONE',  ( 190.6071113721798156, 300.5057941498820924, -0.4754021072632813594 ) ) ;
#88812=CARTESIAN_POINT ( 'NONE',  ( -6.590166341514275494, 160.8768266524160140, 9.188101187500096856 ) ) ;
#88814=CARTESIAN_POINT ( 'NONE',  ( 40.58072100116311276, 203.4244531367911293, -4.594050593750046652 ) ) ;
#88815=CARTESIAN_POINT ( 'NONE',  ( 178.9896671260052301, 258.6863495541695670, -11.59027018806768794 ) ) ;
#88817=CARTESIAN_POINT ( 'NONE',  ( 34.93377400070185956, 197.6427522451419065, 10.00000000000009415 ) ) ;
#88818=CARTESIAN_POINT ( 'NONE',  ( 157.4805323096970255, 257.8827121670497036, -16.70238855805511591 ) ) ;
#88820=CARTESIAN_POINT ( 'NONE',  ( 190.5541309856500050, 300.5975588711562523, -4.167177996129430184 ) ) ;
#88823=CARTESIAN_POINT ( 'NONE',  ( 172.6714394711437706, 279.8122014979473988, -15.90111829678659028 ) ) ;
#88824=CARTESIAN_POINT ( 'NONE',  ( 65.24466313315720356, 215.1427522451419065, -10.00000000000009415 ) ) ;
#88827=CARTESIAN_POINT ( 'NONE',  ( 171.1295603993285965, 249.6517061031812545, 4.344809613321301889 ) ) ;
#88829=CARTESIAN_POINT ( 'NONE',  ( 35.52916646935157274, 197.9865022471903160, -10.00000000000009415 ) ) ;
#88830=CARTESIAN_POINT ( 'NONE',  ( 182.7818713244062678, 292.2108625818275982, 9.360646295977867126 ) ) ;
#88831=CARTESIAN_POINT ( 'NONE',  ( 149.7178657912151607, 271.8703460001313488, -11.47881117598261369 ) ) ;
#88833=CARTESIAN_POINT ( 'NONE',  ( -0.3657822996961275219, 170.5958772461660544, -9.188101187500095079 ) ) ;
#88836=CARTESIAN_POINT ( 'NONE',  ( 152.7153488183568300, 266.1362520814392951, 17.33540622643059237 ) ) ;
#88838=CARTESIAN_POINT ( 'NONE',  ( 75.41814989884494480, 225.8967562850346837, -4.648177544792955347E-16 ) ) ;
#88839=AXIS2_PLACEMENT_3D ( 'NONE', #20759, #6546, #7030 ) ;
#88840=CARTESIAN_POINT ( 'NONE',  ( 179.4126076325937902, 277.4822272090366369, 16.59173480958843072 ) ) ;
#88841=CARTESIAN_POINT ( 'NONE',  ( 196.4170778717353585, 290.4426369823788718, -17.78762421190030452 ) ) ;
#88843=AXIS2_PLACEMENT_3D ( 'NONE', #13468, #74289, #59526 ) ;
#88847=CARTESIAN_POINT ( 'NONE',  ( 159.1258744071607225, 259.4344880999452130, 16.68999608692717018 ) ) ;
#88848=CARTESIAN_POINT ( 'NONE',  ( 193.7261517370125432, 295.1034577671335342, 14.97744313279139661 ) ) ;
#88849=VERTEX_POINT ( 'NONE', #23236 ) ;
#88851=CARTESIAN_POINT ( 'NONE',  ( 156.8438492009701974, 276.4973248573016349, 10.30341974258334936 ) ) ;
#88854=EDGE_LOOP ( 'NONE', ( #47769, #74767, #39915, #31264 ) ) ;
#88855=CARTESIAN_POINT ( 'NONE',  ( 192.1640094933931096, 297.8091675017319062, 12.36911124822534447 ) ) ;
#88856=CARTESIAN_POINT ( 'NONE',  ( 207.2383675728608239, 271.6996134166075763, 7.873592648726489784 ) ) ;
#88862=CARTESIAN_POINT ( 'NONE',  ( 159.7486141406463673, 278.6331531155009884, -9.641193493407582693 ) ) ;
#88864=CARTESIAN_POINT ( 'NONE',  ( 152.9920137376499838, 265.6570543845515431, 16.15798175643282164 ) ) ;
#88867=CARTESIAN_POINT ( 'NONE',  ( 174.6563431587044590, 262.3393413554219933, 14.36283845981329144 ) ) ;
#88870=CARTESIAN_POINT ( 'NONE',  ( 80.90528918492583443, 217.5177522451418497, -10.00000000000009592 ) ) ;
#88871=B_SPLINE_CURVE_WITH_KNOTS ( 'NONE', 3,
 ( #31204, #24111, #100136, #77833, #37802, #91552, #77322, #8416, #55004, #69708, #7408, #39780, #68710, #39288, #93550, #316, #93039, #84951, #23595, #70198, #69210, #62595, #85467, #53013, #16012, #76341, #6914, #92073, #99636, #22623, #84462, #76814, #30218, #61101 ),
 .UNSPECIFIED., .F., .F.,
 ( 4, 2, 2, 2, 2, 2, 2, 2, 2, 2, 2, 2, 2, 2, 2, 2, 4 ),
 ( 0.001328748612904130048, 0.001671321452974920511, 0.002013894293045710542, 0.002699039973187349582, 0.004069331333470678838, 0.004754477013612343900, 0.005097049853683153012, 0.005268336273718570578, 0.005353979483736278494, 0.005396801088745134187, 0.005439622693753988145, 0.005525265903771676979, 0.005610909113789364078, 0.005782195533824741746, 0.006124768373895498816, 0.006467341213966254151, 0.006809914054037011222 ),
 .UNSPECIFIED. ) ;
#88872=CARTESIAN_POINT ( 'NONE',  ( 196.6800254274587019, 289.9871984561398222, -17.90749311895638129 ) ) ;
#88874=CARTESIAN_POINT ( 'NONE',  ( 39.33606980327277824, 193.5177522451418781, -10.00000000000009592 ) ) ;
#88875=EDGE_CURVE ( 'NONE', #24654, #96030, #65936, .T. ) ;
#88877=CARTESIAN_POINT ( 'NONE',  ( 161.6256441450323678, 250.7031678651938762, 14.48526717260977037 ) ) ;
#88882=CARTESIAN_POINT ( 'NONE',  ( 148.9228818358559749, 272.7049975811580680, 12.13823097167056275 ) ) ;
#88885=CARTESIAN_POINT ( 'NONE',  ( 160.3232326710177063, 268.8205896071553980, -16.66338050398602277 ) ) ;
#88886=EDGE_LOOP ( 'NONE', ( #93082, #57374, #35580, #54885, #73146 ) ) ;
#88887=CARTESIAN_POINT ( 'NONE',  ( 158.7190333866803655, 269.4707014042647302, 15.62828681828240107 ) ) ;
#88888=VERTEX_POINT ( 'NONE', #14656 ) ;
#88889=CARTESIAN_POINT ( 'NONE',  ( 158.8065584601817477, 260.0459917420977263, 17.43621632757881557 ) ) ;
#88890=CARTESIAN_POINT ( 'NONE',  ( 193.7606469113726462, 295.0437103725260499, 14.91128319924638745 ) ) ;
#88893=CARTESIAN_POINT ( 'NONE',  ( 193.7173197858508900, 294.7288552955487830, 13.42109144984733682 ) ) ;
#88894=EDGE_CURVE ( 'NONE', #82087, #73983, #70796, .T. ) ;
#88895=CARTESIAN_POINT ( 'NONE',  ( 178.3444744936179518, 291.9204168475665711, 7.080535521235421292 ) ) ;
#88896=CARTESIAN_POINT ( 'NONE',  ( 197.0367503649972036, 289.3693327399964801, -16.94195272704401845 ) ) ;
#88900=CARTESIAN_POINT ( 'NONE',  ( 87.85384634344086408, 209.9824982072973967, 3.021315404115420679E-15 ) ) ;
#88902=CARTESIAN_POINT ( 'NONE',  ( 164.7462163020046262, 245.2981783406326599, 1.451255823150352064 ) ) ;
#88903=CARTESIAN_POINT ( 'NONE',  ( 198.4772197948566372, 286.8743665007300478, 18.43646439804394532 ) ) ;
#88905=CARTESIAN_POINT ( 'NONE',  ( 190.3865446062718547, 300.8878269948957040, 5.596937249297124772 ) ) ;
#88906=CARTESIAN_POINT ( 'NONE',  ( 171.4730959963652595, 259.7561518679366372, -14.77276439450797696 ) ) ;
#88907=DIRECTION ( 'NONE',  ( -0.8660254037844387076, -0.4999999999999998890, -0.000000000000000000 ) ) ;
#88908=EDGE_CURVE ( 'NONE', #83705, #23987, #88998, .T. ) ;
#88912=CARTESIAN_POINT ( 'NONE',  ( 160.1913727725009835, 253.1873987542595614, -16.21806651737331251 ) ) ;
#88913=CARTESIAN_POINT ( 'NONE',  ( 190.4876730617585849, 300.7126673719016594, -1.247921881438171621 ) ) ;
#88914=ORIENTED_EDGE ( 'NONE', *, *, #52522, .F. ) ;
#88915=CARTESIAN_POINT ( 'NONE',  ( 167.3930310403720796, 252.8207621138501224, -12.36123731186929930 ) ) ;
#88916=CARTESIAN_POINT ( 'NONE',  ( -22.42236680055709641, 157.8615022471902591, 0.000000000000000000 ) ) ;
#88917=CARTESIAN_POINT ( 'NONE',  ( 201.1060504099706350, 282.3210983108598384, -18.18000168485860257 ) ) ;
#88919=CARTESIAN_POINT ( 'NONE',  ( 207.1059763530604698, 271.9289217357780899, 6.370907250589925575 ) ) ;
#88920=CARTESIAN_POINT ( 'NONE',  ( 38.03703169759616287, 182.7677522451417929, -5.000000000000041744 ) ) ;
#88921=CARTESIAN_POINT ( 'NONE',  ( 109.2678814824639204, 224.7048013555410080, 4.594050593750051981 ) ) ;
#88922=CARTESIAN_POINT ( 'NONE',  ( 183.9211145108844221, 296.5969538952800235, -2.738914410665766130 ) ) ;
#88923=VECTOR ( 'NONE', #17992, 1000.000000000000000 ) ;
#88924=CARTESIAN_POINT ( 'NONE',  ( 164.0550791845173535, 280.3860225496770795, -11.45558117589946612 ) ) ;
#88926=CARTESIAN_POINT ( 'NONE',  ( 208.2018443082727970, 270.0308227589636090, 1.727811837614598556 ) ) ;
#88927=CARTESIAN_POINT ( 'NONE',  ( 10.56744132731740216, 189.1589784336661637, -6.496448406907675876E-16 ) ) ;
#88933=CARTESIAN_POINT ( 'NONE',  ( 185.1797296270955542, 259.8357583151453696, -5.558726417257365604 ) ) ;
#88934=FACE_OUTER_BOUND ( 'NONE', #43329, .T. ) ;
#88936=CARTESIAN_POINT ( 'NONE',  ( 193.0398521437286377, 263.8906099786534583, -4.323427293014181494 ) ) ;
#88939=CARTESIAN_POINT ( 'NONE',  ( 182.3656953904154534, 284.2887812106879437, 14.91155821018728034 ) ) ;
#88942=CARTESIAN_POINT ( 'NONE',  ( 42.06911538997637479, 207.3464784336661637, 1.353441290958777525E-15 ) ) ;
#88943=CARTESIAN_POINT ( 'NONE',  ( 102.5559242795368391, 220.0177522451417929, 5.000000000000051514 ) ) ;
#88945=CARTESIAN_POINT ( 'NONE',  ( 150.0670708984111457, 271.4758772266419555, -12.06937736578899312 ) ) ;
#88949=CARTESIAN_POINT ( 'NONE',  ( 2.719259653403430121, 178.5024278399160949, -9.188101187500093303 ) ) ;
#88952=CARTESIAN_POINT ( 'NONE',  ( 150.6386650955079176, 269.7331738006648720, -15.06054658539322766 ) ) ;
#88954=CARTESIAN_POINT ( 'NONE',  ( 193.0142717932987182, 296.3364699985351081, -13.30037542329744937 ) ) ;
#88955=CARTESIAN_POINT ( 'NONE',  ( 182.0312531846501258, 257.2221692175513112, -7.485986072910417732 ) ) ;
#88956=CARTESIAN_POINT ( 'NONE',  ( 203.6760479211504276, 276.2018596621056190, 13.30539550760933132 ) ) ;
#88958=CARTESIAN_POINT ( 'NONE',  ( 206.9059968923335475, 272.2752963222270068, 6.902135944297345560 ) ) ;
#88960=CARTESIAN_POINT ( 'NONE',  ( 1.754175721758462370, 178.4865022471903728, -10.00000000000009415 ) ) ;
#88961=B_SPLINE_CURVE_WITH_KNOTS ( 'NONE', 3,
 ( #46333, #77257, #7865, #71683, #93998, #48365, #40237, #751, #54428, #85404, #8853, #71178, #23535, #64058, #39722, #87444, #31634, #16946, #56452, #8364, #33156, #62535, #95002, #25563, #17455, #72177, #47833, #1775, #55926, #2275, #24053, #86922, #79805, #93494, #79312, #9881, #32654, #17977, #10369, #48871, #54948, #85925, #15952, #78270 ),
 .UNSPECIFIED., .F., .F.,
 ( 4, 2, 2, 2, 2, 2, 2, 2, 2, 2, 2, 2, 2, 2, 2, 2, 2, 2, 2, 2, 2, 4 ),
 ( 0.002346744725963096061, 0.002773758852798046456, 0.002987265916215522087, 0.003094019447924267058, 0.003200772979633012896, 0.003307526511341757867, 0.003414280043050503272, 0.003627787106467994516, 0.004054801233303112311, 0.004908829486973232542, 0.005762857740643351906, 0.006616885994313471270, 0.007043900121148489318, 0.007470914247983505632, 0.007577667779692260144, 0.007631044545546630462, 0.007684421311401002513, 0.007791174843109744882, 0.007897928374818488986, 0.008324942501653435911, 0.008751956628488386306, 0.009178970755323333230 ),
 .UNSPECIFIED. ) ;
#88963=CARTESIAN_POINT ( 'NONE',  ( 124.6666353716822186, 242.7833772461660544, -9.188101187500095079 ) ) ;
#88969=CARTESIAN_POINT ( 'NONE',  ( 190.5994576334820181, 300.5190508141740793, -7.527957223721390534 ) ) ;
#88971=CARTESIAN_POINT ( 'NONE',  ( 151.4025156491502742, 268.4101458323662541, 14.71049357081981235 ) ) ;
#88972=CARTESIAN_POINT ( 'NONE',  ( 207.6314056968649595, 271.0188514165208744, -1.280821594136880126 ) ) ;
#88974=CARTESIAN_POINT ( 'NONE',  ( 169.5601139872289309, 266.0306789591197116, -17.01818431075402671 ) ) ;
#88976=ORIENTED_EDGE ( 'NONE', *, *, #56222, .F. ) ;
#88978=CARTESIAN_POINT ( 'NONE',  ( 168.4739816692278396, 271.7343923863479063, -17.32961767935828590 ) ) ;
#88982=B_SPLINE_CURVE_WITH_KNOTS ( 'NONE', 3,
 ( #47323, #24025, #46831, #54924 ),
 .UNSPECIFIED., .F., .F.,
 ( 4, 4 ),
 ( 0.01057495740738979666, 0.01616209098191098009 ),
 .UNSPECIFIED. ) ;
#88983=CARTESIAN_POINT ( 'NONE',  ( 185.5205021638500114, 297.3465265719306103, 5.673669933437759383 ) ) ;
#88985=CARTESIAN_POINT ( 'NONE',  ( 149.1326317111226558, 276.5594127424867565, -0.0002112342455116459836 ) ) ;
#88986=CARTESIAN_POINT ( 'NONE',  ( 194.1909060474912110, 282.8098373099740570, 17.20683189011229430 ) ) ;
#88988=CARTESIAN_POINT ( 'NONE',  ( 173.8490933012782307, 272.4998881216204154, -16.42193024097150200 ) ) ;
#88990=CYLINDRICAL_SURFACE ( 'NONE', #78978, 17.82106496071139645 ) ;
#88991=EDGE_CURVE ( 'NONE', #9838, #21251, #91268, .T. ) ;
#88992=CARTESIAN_POINT ( 'NONE',  ( 197.7196744852244876, 271.6120449130532393, 13.56729386884406630 ) ) ;
#88993=CARTESIAN_POINT ( 'NONE',  ( 156.2033007795417348, 262.0734030644348991, -16.95518515663351877 ) ) ;
#88994=VERTEX_POINT ( 'NONE', #10058 ) ;
#88998=B_SPLINE_CURVE_WITH_KNOTS ( 'NONE', 3,
 ( #76940, #24253, #29852, #45533 ),
 .UNSPECIFIED., .F., .F.,
 ( 4, 4 ),
 ( 0.02742407849190809863, 0.03663494907973673109 ),
 .UNSPECIFIED. ) ;
#89002=CARTESIAN_POINT ( 'NONE',  ( 91.40610752940987993, 214.3923013555409796, 4.594050593750050204 ) ) ;
#89005=CYLINDRICAL_SURFACE ( 'NONE', #16495, 10.00000000000010658 ) ;
#89006=CARTESIAN_POINT ( 'NONE',  ( 185.2750378117470689, 259.6499128198802282, -6.774890732820249895 ) ) ;
#89015=CARTESIAN_POINT ( 'NONE',  ( 155.0304386007204016, 262.1263989543018056, -17.12961552904782181 ) ) ;
#89017=CARTESIAN_POINT ( 'NONE',  ( 182.8048260423933584, 279.9985300298516790, -16.23004993202965807 ) ) ;
#89019=CARTESIAN_POINT ( 'NONE',  ( 161.3257284758417143, 277.4216702933620695, -13.36329991415315455 ) ) ;
#89023=CARTESIAN_POINT ( 'NONE',  ( 5.723458822437168081, 174.1115022471902591, 10.00000000000009592 ) ) ;
#89024=CARTESIAN_POINT ( 'NONE',  ( 148.2390246527636748, 247.2048013555409511, 4.594050593750051981 ) ) ;
#89025=ORIENTED_EDGE ( 'NONE', *, *, #51197, .T. ) ;
#89028=EDGE_LOOP ( 'NONE', ( #92950, #52556, #95676, #89846 ) ) ;
#89030=CARTESIAN_POINT ( 'NONE',  ( 200.4530980307013124, 270.4255315980906289, 9.273059835868647127 ) ) ;
#89031=ORIENTED_EDGE ( 'NONE', *, *, #6687, .T. ) ;
#89034=CARTESIAN_POINT ( 'NONE',  ( 127.7428297729342717, 237.8927522451417929, -10.00000000000009237 ) ) ;
#89036=EDGE_CURVE ( 'NONE', #10368, #100061, #25769, .T. ) ;
#89038=( BOUNDED_CURVE ( )  B_SPLINE_CURVE ( 2, ( #47676, #85760, #24395, #39563, #72007, #95358, #23879, #16289, #87769 ),
 .UNSPECIFIED., .F., .T. ) 
 B_SPLINE_CURVE_WITH_KNOTS ( ( 3, 2, 2, 2, 3 ),
 ( 0.6491935483870967527, 0.6505376344086021279, 0.6532258064516128782, 0.6559139784946236285, 0.6572580645161290036 ),
 .UNSPECIFIED. ) 
 CURVE ( )  GEOMETRIC_REPRESENTATION_ITEM ( )  RATIONAL_B_SPLINE_CURVE ( ( 0.9330127018922194093, 0.9330127018922194093, 1.000000000000000000, 0.8660254037844387076, 1.000000000000000000, 0.8660254037844387076, 1.000000000000000000, 0.9330127018922194093, 0.9330127018922194093 ) ) 
 REPRESENTATION_ITEM ( '' )  );
#89039=CARTESIAN_POINT ( 'NONE',  ( 174.7756533518544302, 282.0975554114792203, 14.28861982422490762 ) ) ;
#89044=CARTESIAN_POINT ( 'NONE',  ( 184.1103630465501624, 272.4158174899661731, -17.30342150099949450 ) ) ;
#89047=CARTESIAN_POINT ( 'NONE',  ( 194.2102773769292128, 293.8493148023329127, -14.16464662972703614 ) ) ;
#89048=CARTESIAN_POINT ( 'NONE',  ( 200.9384910137331417, 267.7722853946023065, -2.751277086281960216 ) ) ;
#89051=CARTESIAN_POINT ( 'NONE',  ( 164.0982892389591825, 274.1344140775349842, 14.77298282198140456 ) ) ;
#89052=CARTESIAN_POINT ( 'NONE',  ( -13.35616335646270691, 163.0958772461660544, -9.188101187500095079 ) ) ;
#89054=CARTESIAN_POINT ( 'NONE',  ( 202.2072345662346038, 269.4162813440198647, 6.010783582451708185 ) ) ;
#89057=CARTESIAN_POINT ( 'NONE',  ( 189.8573735225914731, 274.2923351804632830, -15.65845412275707105 ) ) ;
#89061=DIRECTION ( 'NONE',  ( -0.8660254037844387076, -0.4999999999999998890, -0.000000000000000000 ) ) ;
#89063=CARTESIAN_POINT ( 'NONE',  ( 15.38522827951586081, 173.5643266524160140, -9.188101187500093303 ) ) ;
#89064=CARTESIAN_POINT ( 'NONE',  ( 103.5572661544365332, 230.5958772461660260, -9.188101187500095079 ) ) ;
#89065=CARTESIAN_POINT ( 'NONE',  ( 202.8549823380854491, 279.2918593523859272, -16.39745931995414807 ) ) ;
#89067=CARTESIAN_POINT ( 'NONE',  ( 180.1480783116751923, 255.5411283896334567, -2.368270940572544614 ) ) ;
#89070=B_SPLINE_CURVE_WITH_KNOTS ( 'NONE', 3,
 ( #71351, #95696, #3456, #64746, #88100, #80988, #56631, #34335, #94671, #48024, #26243, #65231, #42413, #18649 ),
 .UNSPECIFIED., .F., .F.,
 ( 4, 2, 2, 2, 2, 2, 4 ),
 ( 0.001093769620356032464, 0.001335766207658145837, 0.001577762794960259427, 0.002061755969564524772, 0.002303752556866657444, 0.002545749144168790116, 0.003029742318773055460 ),
 .UNSPECIFIED. ) ;
#89072=CARTESIAN_POINT ( 'NONE',  ( 157.8501323257721083, 280.8042112442767007, -7.123878780571343050 ) ) ;
#89073=CARTESIAN_POINT ( 'NONE',  ( 148.0346525705264469, 274.2434557974783615, -9.381294579651672905 ) ) ;
#89078=AXIS2_PLACEMENT_3D ( 'NONE', #54708, #8631, #46105 ) ;
#89079=CARTESIAN_POINT ( 'NONE',  ( 172.9743055469626825, 262.8123507573143343, -16.34602756528129319 ) ) ;
#89080=CARTESIAN_POINT ( 'NONE',  ( 85.15457341978220995, 207.7202760586659167, -5.415160957724236172E-17 ) ) ;
#89081=CARTESIAN_POINT ( 'NONE',  ( 161.6755750489535046, 250.6166850027345276, -13.01404233079112061 ) ) ;
#89082=CARTESIAN_POINT ( 'NONE',  ( 163.2257943664163236, 247.9316263820140307, 0.000000000000000000 ) ) ;
#89084=CARTESIAN_POINT ( 'NONE',  ( 196.4351339088274813, 290.4113630087520050, 17.20526457544535504 ) ) ;
#89085=CARTESIAN_POINT ( 'NONE',  ( 199.7543762271261301, 284.6622666708254314, 18.24097302174371293 ) ) ;
#89086=CARTESIAN_POINT ( 'NONE',  ( 151.1126408083691501, 268.9122237844355254, -15.82705194100464396 ) ) ;
#89087=CARTESIAN_POINT ( 'NONE',  ( 173.2921293650385337, 267.8776318488850734, -16.33130809225368552 ) ) ;
#89093=CARTESIAN_POINT ( 'NONE',  ( 173.1211852740584334, 289.6938670388238393, -0.9942850523788112627 ) ) ;
#89095=CARTESIAN_POINT ( 'NONE',  ( 191.7482382276744772, 287.9955150116063010, -15.83237412442799830 ) ) ;
#89097=CARTESIAN_POINT ( 'NONE',  ( 157.7355870688748496, 268.4989845473052696, 15.89826748515501009 ) ) ;
#89100=CARTESIAN_POINT ( 'NONE',  ( 128.2660534579352145, 254.8615022471902876, 5.000000000000046185 ) ) ;
#89101=CARTESIAN_POINT ( 'NONE',  ( 204.7519188734507622, 276.0062688943993408, -12.76027478560537531 ) ) ;
#89103=ORIENTED_EDGE ( 'NONE', *, *, #81639, .F. ) ;
#89104=CARTESIAN_POINT ( 'NONE',  ( 169.5934039790062684, 248.5513711909993901, -1.936694667797326685 ) ) ;
#89106=CARTESIAN_POINT ( 'NONE',  ( 162.6626107288841467, 248.9070890562113902, 10.12509462564867313 ) ) ;
#89108=EDGE_CURVE ( 'NONE', #85978, #98021, #50150, .T. ) ;
#89111=VERTEX_POINT ( 'NONE', #58621 ) ;
#89114=CARTESIAN_POINT ( 'NONE',  ( 137.5794118583994532, 267.3524639162450285, 1.815056976409021644E-15 ) ) ;
#89119=CARTESIAN_POINT ( 'NONE',  ( 164.1807942228835770, 275.2290214034088081, 14.89732332872395304 ) ) ;
#89120=FACE_OUTER_BOUND ( 'NONE', #50372, .T. ) ;
#89121=EDGE_LOOP ( 'NONE', ( #52026, #58881, #32044, #93160 ) ) ;
#89123=CARTESIAN_POINT ( 'NONE',  ( 182.6850850546973106, 296.4922765959772164, 0.2764116486899246827 ) ) ;
#89125=CARTESIAN_POINT ( 'NONE',  ( 165.9392095978298869, 274.2621017338486809, -15.13082047531800178 ) ) ;
#89127=CARTESIAN_POINT ( 'NONE',  ( 201.2981219894440414, 274.9036200554554625, -14.05226934314597464 ) ) ;
#89129=CARTESIAN_POINT ( 'NONE',  ( -27.42236680055714260, 166.5217562850347406, 1.224646799147364892E-15 ) ) ;
#89130=CARTESIAN_POINT ( 'NONE',  ( 207.7579944447645346, 270.7995932734924054, -3.579072180489195620 ) ) ;
#89132=CARTESIAN_POINT ( 'NONE',  ( 169.4258527407971826, 267.1907338905178904, 17.61138475887533517 ) ) ;
#89134=CARTESIAN_POINT ( 'NONE',  ( 103.0163473728362504, 218.0327760586659451, 1.948934522072303157E-15 ) ) ;
#89138=CARTESIAN_POINT ( 'NONE',  ( 166.7207440965885326, 278.5315519395303454, -13.22152219497125358 ) ) ;
#89140=ORIENTED_EDGE ( 'NONE', *, *, #61460, .F. ) ;
#89141=CARTESIAN_POINT ( 'NONE',  ( 183.1426684129219780, 267.5694331394444703, -16.03671021927237206 ) ) ;
#89142=CARTESIAN_POINT ( 'NONE',  ( 177.5820306303727136, 292.5357431145801002, -2.681843810317637189 ) ) ;
#89143=CARTESIAN_POINT ( 'NONE',  ( 164.7647380297938184, 248.9862001899016946, 10.10785415616959071 ) ) ;
#89144=CARTESIAN_POINT ( 'NONE',  ( 159.9635946688021022, 268.7707599091479551, -17.14635356962945778 ) ) ;
#89147=CARTESIAN_POINT ( 'NONE',  ( 99.98491136382573075, 228.5333772461660828, 9.188101187500095079 ) ) ;
#89148=ORIENTED_EDGE ( 'NONE', *, *, #10623, .F. ) ;
#89151=ORIENTED_EDGE ( 'NONE', *, *, #61391, .T. ) ;
#89156=EDGE_CURVE ( 'NONE', #60494, #39924, #42949, .T. ) ;
#89157=CARTESIAN_POINT ( 'NONE',  ( 194.6929193942598317, 266.3728879037764159, -7.804718999318556172 ) ) ;
#89160=CARTESIAN_POINT ( 'NONE',  ( 132.1361044793229951, 247.0958772461660544, -9.188101187500095079 ) ) ;
#89162=CARTESIAN_POINT ( 'NONE',  ( -5.625082409869304634, 160.8927522451418213, 10.00000000000009592 ) ) ;
#89165=CARTESIAN_POINT ( 'NONE',  ( 205.0957184426459321, 275.4107905729332515, 13.78964280781899632 ) ) ;
#89166=CARTESIAN_POINT ( 'NONE',  ( 160.6678256987136706, 275.6111059978462663, 12.91046967929992384 ) ) ;
#89169=CARTESIAN_POINT ( 'NONE',  ( 177.9371141619689070, 285.1367043548689821, 13.03223046609528879 ) ) ;
#89174=CARTESIAN_POINT ( 'NONE',  ( 206.6148326247335092, 272.1004287451723371, 7.183687323914591971 ) ) ;
#89175=CARTESIAN_POINT ( 'NONE',  ( 167.7724828596593341, 250.0038861993971295, 6.958639209991310359 ) ) ;
#89177=CARTESIAN_POINT ( 'NONE',  ( 207.6555576926778883, 270.9770189326688410, -1.235081510489080436 ) ) ;
#89180=CARTESIAN_POINT ( 'NONE',  ( 185.3369900536077068, 266.4498558932299375, 13.14662191727306073 ) ) ;
#89187=CARTESIAN_POINT ( 'NONE',  ( 207.1158949475991164, 271.9117422260973740, -5.823035679195911918 ) ) ;
#89188=CARTESIAN_POINT ( 'NONE',  ( 11.92112666437810908, 171.5643266524160140, 9.188101187500095079 ) ) ;
#89192=CARTESIAN_POINT ( 'NONE',  ( 30.33301404664494427, 194.9865022471903160, -10.00000000000009592 ) ) ;
#89194=CARTESIAN_POINT ( 'NONE',  ( 32.11017034222032862, 189.3458772461660544, 9.188101187500095079 ) ) ;
#89195=ADVANCED_FACE ( 'NONE', ( #51029 ), #36833, .T. ) ;
#89196=CARTESIAN_POINT ( 'NONE',  ( 200.8551880497955437, 282.7556046643899776, 18.00894873733387058 ) ) ;
#89197=CARTESIAN_POINT ( 'NONE',  ( 147.4811722709131914, 275.2021117973970377, 3.890385073228495916 ) ) ;
#89199=CARTESIAN_POINT ( 'NONE',  ( 201.8398744800204838, 269.4056535102417342, -6.425511374294321953 ) ) ;
#89200=CARTESIAN_POINT ( 'NONE',  ( 147.2180753513904961, 275.6578090293250511, 0.4909717733184589261 ) ) ;
#89201=CARTESIAN_POINT ( 'NONE',  ( 179.0376912146908523, 278.3007504662035103, -16.65281315354532410 ) ) ;
#89207=CARTESIAN_POINT ( 'NONE',  ( 79.69646206235795205, 223.4865022471902591, -10.00000000000009415 ) ) ;
#89211=CARTESIAN_POINT ( 'NONE',  ( 40.25596147474394826, 203.2369531367911293, -4.594050593750048428 ) ) ;
#89212=ORIENTED_EDGE ( 'NONE', *, *, #28920, .T. ) ;
#89214=CARTESIAN_POINT ( 'NONE',  ( 190.3286155001717930, 300.9881631498979004, -5.624828231725103045 ) ) ;
#89217=CARTESIAN_POINT ( 'NONE',  ( 171.0937289546497766, 286.9986480494256966, 8.572633432616918014 ) ) ;
#89218=FACE_OUTER_BOUND ( 'NONE', #70222, .T. ) ;
#89221=CARTESIAN_POINT ( 'NONE',  ( 186.9609134277102669, 264.2677986880410685, 10.82359653245352682 ) ) ;
#89222=CARTESIAN_POINT ( 'NONE',  ( 196.4501996009505831, 290.3852684645433442, -17.82325615854289680 ) ) ;
#89223=CARTESIAN_POINT ( 'NONE',  ( 172.6087892508253390, 256.3355526837004845, 11.23066983786553941 ) ) ;
#89227=CARTESIAN_POINT ( 'NONE',  ( 172.5056581661058033, 253.5720814276482997, 8.377529669797983303 ) ) ;
#89228=CARTESIAN_POINT ( 'NONE',  ( 16.45310489419773958, 168.7592609112379876, 2.679491924311254714 ) ) ;
#89229=ORIENTED_EDGE ( 'NONE', *, *, #15084, .F. ) ;
#89230=CARTESIAN_POINT ( 'NONE',  ( 181.9138868423064821, 283.8759538834763134, 14.95563825545625747 ) ) ;
#89231=FACE_OUTER_BOUND ( 'NONE', #90958, .T. ) ;
#89234=VERTEX_POINT ( 'NONE', #19668 ) ;
#89235=CARTESIAN_POINT ( 'NONE',  ( 161.8668411317136986, 250.2854024296290447, -13.43522912998426655 ) ) ;
#89243=CARTESIAN_POINT ( 'NONE',  ( 197.9771301758180186, 286.8468337050553600, 16.93947910494098608 ) ) ;
#89244=CARTESIAN_POINT ( 'NONE',  ( 123.6384037525706958, 236.0643266524160140, 9.188101187500095079 ) ) ;
#89246=DIRECTION ( 'NONE',  ( 0.4999999999999992784, -0.8660254037844390407, 0.000000000000000000 ) ) ;
#89247=CARTESIAN_POINT ( 'NONE',  ( 74.97949069045873216, 202.5494855054051584, -2.679491924311248496 ) ) ;
#89248=CARTESIAN_POINT ( 'NONE',  ( 163.7595992360150490, 247.0070492265414828, -6.976205010573520049 ) ) ;
#89250=B_SPLINE_CURVE_WITH_KNOTS ( 'NONE', 3,
 ( #14505, #38781, #76318, #53485 ),
 .UNSPECIFIED., .F., .F.,
 ( 4, 4 ),
 ( 0.005435284012089665502, 0.01347523137567103318 ),
 .UNSPECIFIED. ) ;
#89252=CARTESIAN_POINT ( 'NONE',  ( 159.6419305724666344, 254.1390605605417079, 16.92015248457581933 ) ) ;
#89253=DIRECTION ( 'NONE',  ( -0.8660254037844387076, -0.4999999999999998890, -0.000000000000000000 ) ) ;
#89254=CARTESIAN_POINT ( 'NONE',  ( 75.46539357129627490, 220.5024278399160949, -9.188101187500093303 ) ) ;
#89255=CARTESIAN_POINT ( 'NONE',  ( 176.4104406952913848, 285.9470522879340137, 13.60907346279267927 ) ) ;
#89256=CARTESIAN_POINT ( 'NONE',  ( 151.4025156491502742, 268.4101458323662541, 14.71049357081981235 ) ) ;
#89257=CARTESIAN_POINT ( 'NONE',  ( 154.9455285025717615, 262.2734675583710100, 18.28470720339922551 ) ) ;
#89258=CARTESIAN_POINT ( 'NONE',  ( 175.5536407316448333, 278.4519599138486114, 15.47712664167736030 ) ) ;
#89260=EDGE_CURVE ( 'NONE', #69600, #90508, #78919, .T. ) ;
#89262=FACE_OUTER_BOUND ( 'NONE', #40850, .T. ) ;
#89263=ORIENTED_EDGE ( 'NONE', *, *, #75314, .F. ) ;
#89264=CARTESIAN_POINT ( 'NONE',  ( 194.7327554194830554, 293.3599690460087572, 15.69670373610146363 ) ) ;
#89265=CARTESIAN_POINT ( 'NONE',  ( -16.97593537095525917, 172.5530062829863027, 9.296355089585912665E-16 ) ) ;
#89266=CARTESIAN_POINT ( 'NONE',  ( 160.5379721355672586, 258.2968622624442787, -16.86137763422037494 ) ) ;
#89268=CARTESIAN_POINT ( 'NONE',  ( 206.7036107519802783, 270.2074794926728032, 1.825126258972860516 ) ) ;
#89270=CARTESIAN_POINT ( 'NONE',  ( 150.3616303100281471, 275.4795733169851815, 8.855240024576275459 ) ) ;
#89271=CARTESIAN_POINT ( 'NONE',  ( 164.4573439719129340, 245.7985198932525748, 1.541132361166968501 ) ) ;
#89274=CARTESIAN_POINT ( 'NONE',  ( 125.6141109788952122, 234.1423013555409796, -4.594050593750043987 ) ) ;
#89275=ORIENTED_EDGE ( 'NONE', *, *, #11020, .T. ) ;
#89276=CARTESIAN_POINT ( 'NONE',  ( 146.5310397537613483, 276.8477895910274356, -0.2793038414862049068 ) ) ;
#89278=CARTESIAN_POINT ( 'NONE',  ( 205.6477917841175156, 273.8035238412935541, -10.40835627202817903 ) ) ;
#89279=CARTESIAN_POINT ( 'NONE',  ( 164.4272222519600746, 245.8506922426221593, 7.021336339662529902 ) ) ;
#89285=CARTESIAN_POINT ( 'NONE',  ( 167.5883605658670490, 249.2390751195395353, -5.691470653330944707 ) ) ;
#89288=CARTESIAN_POINT ( 'NONE',  ( 142.6123662252853421, 259.5780487066560340, -7.305945665944390655 ) ) ;
#89289=CARTESIAN_POINT ( 'NONE',  ( 195.4818567523729200, 263.4360957373327778, 0.8675948490323511786 ) ) ;
#89291=CARTESIAN_POINT ( 'NONE',  ( 180.2260403442535051, 295.0423342771414923, -3.480517403894910711 ) ) ;
#89292=CARTESIAN_POINT ( 'NONE',  ( 192.2429491947952158, 297.0140665128034243, 10.97773268720420248 ) ) ;
#89294=CARTESIAN_POINT ( 'NONE',  ( 149.3833831332874240, 271.9073859370555510, 11.40518020539810173 ) ) ;
#89296=CARTESIAN_POINT ( 'NONE',  ( 169.4074305931134461, 285.1542170432204557, -8.003578837916338173 ) ) ;
#89297=CARTESIAN_POINT ( 'NONE',  ( 198.1300353965528984, 287.4757075181870505, 18.48278456664528946 ) ) ;
#89298=CARTESIAN_POINT ( 'NONE',  ( 196.1370092075112268, 290.1209220278959720, 16.40156295354631411 ) ) ;
#89299=( BOUNDED_CURVE ( )  B_SPLINE_CURVE ( 2, ( #87606, #54726, #7135, #16243, #60820, #47134, #78058, #8646, #18133 ),
 .UNSPECIFIED., .F., .T. ) 
 B_SPLINE_CURVE_WITH_KNOTS ( ( 3, 2, 2, 2, 3 ),
 ( 0.8911290322580645018, 0.8924731182795698770, 0.8951612903225806273, 0.8978494623655913776, 0.8991935483870967527 ),
 .UNSPECIFIED. ) 
 CURVE ( )  GEOMETRIC_REPRESENTATION_ITEM ( )  RATIONAL_B_SPLINE_CURVE ( ( 0.9330127018922194093, 0.9330127018922194093, 1.000000000000000000, 0.8660254037844387076, 1.000000000000000000, 0.8660254037844387076, 1.000000000000000000, 0.9330127018922194093, 0.9330127018922194093 ) ) 
 REPRESENTATION_ITEM ( '' )  );
#89300=CARTESIAN_POINT ( 'NONE',  ( 146.7232198725432113, 245.5177522451417644, 5.000000000000051514 ) ) ;
#89301=CARTESIAN_POINT ( 'NONE',  ( 183.1489178096782950, 278.9636052248775400, 17.34984484178414377 ) ) ;
#89302=ORIENTED_EDGE ( 'NONE', *, *, #28193, .F. ) ;
#89303=CARTESIAN_POINT ( 'NONE',  ( 157.7529601300917363, 257.4108533407307959, 16.91445305439664892 ) ) ;
#89304=CARTESIAN_POINT ( 'NONE',  ( 189.8533352240220893, 301.8113727360248504, -0.2033756396389863053 ) ) ;
#89305=CARTESIAN_POINT ( 'NONE',  ( 1.204062292545672319, 165.3768266524160140, 9.188101187500096856 ) ) ;
#89307=CARTESIAN_POINT ( 'NONE',  ( 51.37958267218910891, 188.2202760586659451, -5.415160957724236172E-17 ) ) ;
#89308=CARTESIAN_POINT ( 'NONE',  ( 178.4286190058349746, 259.0350523900441431, -10.32048496258370918 ) ) ;
#89311=CARTESIAN_POINT ( 'NONE',  ( 164.2257943664163236, 246.1995755744451060, 2.059986336238496279E-15 ) ) ;
#89315=CARTESIAN_POINT ( 'NONE',  ( 167.6657660674999022, 256.6202425009460626, 13.71097750828161743 ) ) ;
#89318=LINE ( 'NONE', #9782, #88766 ) ;
#89320=CARTESIAN_POINT ( 'NONE',  ( 45.92147131476491495, 183.9865022471901455, 1.119607411625061291E-15 ) ) ;
#89321=CARTESIAN_POINT ( 'NONE',  ( 182.0785557626968796, 291.7619114360715002, 9.330709163805311235 ) ) ;
#89322=CARTESIAN_POINT ( 'NONE',  ( 149.7165891736972014, 271.9666657501144869, -11.45573312492119022 ) ) ;
#89323=CARTESIAN_POINT ( 'NONE',  ( 2.070087696330116689, 165.8768266524159856, -9.188101187500091527 ) ) ;
#89324=CARTESIAN_POINT ( 'NONE',  ( 164.3014958605646143, 285.1311274651320673, 4.328674906941893497 ) ) ;
#89326=EDGE_CURVE ( 'NONE', #19809, #18420, #97368, .T. ) ;
#89330=CARTESIAN_POINT ( 'NONE',  ( 179.3397263455709663, 277.6061668572808117, 16.87921206249952633 ) ) ;
#89331=CARTESIAN_POINT ( 'NONE',  ( 154.9344967692067598, 262.2925750810547356, 17.30210568643136781 ) ) ;
#89332=CARTESIAN_POINT ( 'NONE',  ( 196.4808189786114951, 290.3322341467384717, -17.84817245450773271 ) ) ;
#89336=CARTESIAN_POINT ( 'NONE',  ( 118.0722127640079577, 245.6427522451419350, 10.00000000000009415 ) ) ;
#89338=CARTESIAN_POINT ( 'NONE',  ( 159.2638637293276531, 259.2554630532692954, 16.67674092906833394 ) ) ;
#89339=CARTESIAN_POINT ( 'NONE',  ( 153.2048789493636605, 277.6616380186837318, -5.192392496551228476 ) ) ;
#89341=CARTESIAN_POINT ( 'NONE',  ( 103.8809628199470012, 242.3297689869269504, -2.679491924311252493 ) ) ;
#89345=CARTESIAN_POINT ( 'NONE',  ( 153.1390349443021535, 266.6901594501808290, 16.22385130400761710 ) ) ;
#89352=CARTESIAN_POINT ( 'NONE',  ( 204.1793240545508752, 276.9980322128846524, 14.17550310845996187 ) ) ;
#89353=CARTESIAN_POINT ( 'NONE',  ( 152.7618747630824885, 266.0556667813044101, 16.41480086888796919 ) ) ;
#89356=CARTESIAN_POINT ( 'NONE',  ( 177.6567394906847710, 263.3673336801520577, 15.42114140403424649 ) ) ;
#89357=ORIENTED_EDGE ( 'NONE', *, *, #1692, .F. ) ;
#89361=CARTESIAN_POINT ( 'NONE',  ( 202.9779954277112495, 268.0318619332833805, 2.519114201778603679 ) ) ;
#89362=CARTESIAN_POINT ( 'NONE',  ( 168.4437225316406170, 276.0757796713103289, -16.34630765130609120 ) ) ;
#89364=VERTEX_POINT ( 'NONE', #61614 ) ;
#89367=CARTESIAN_POINT ( 'NONE',  ( 177.7711228786548077, 279.3620349116163197, -16.19571528524508963 ) ) ;
#89368=CARTESIAN_POINT ( 'NONE',  ( 169.3408527021580881, 261.4620406432418349, -16.56737040952816642 ) ) ;
#89369=ORIENTED_EDGE ( 'NONE', *, *, #44983, .T. ) ;
#89370=CARTESIAN_POINT ( 'NONE',  ( 156.9003456755540924, 266.6926263611233026, -16.21475809265606571 ) ) ;
#89371=ORIENTED_EDGE ( 'NONE', *, *, #13353, .F. ) ;
#89376=CARTESIAN_POINT ( 'NONE',  ( 188.6399219150083297, 298.6042682482373607, -4.272446188806214629 ) ) ;
#89377=CARTESIAN_POINT ( 'NONE',  ( 143.7588392505102206, 242.2592609112379876, 2.679491924311254714 ) ) ;
#89378=CARTESIAN_POINT ( 'NONE',  ( 152.6615646578087819, 266.2294089801508221, 16.94722993326405813 ) ) ;
#89380=CARTESIAN_POINT ( 'NONE',  ( 178.3915236234910537, 291.5165576824842901, 6.088472439993570795 ) ) ;
#89382=CARTESIAN_POINT ( 'NONE',  ( 158.8815770798748588, 255.4560314414227662, -16.10048816751885425 ) ) ;
#89388=CARTESIAN_POINT ( 'NONE',  ( 180.6066648745947134, 283.7006809008031496, -16.18202752516933174 ) ) ;
#89389=CARTESIAN_POINT ( 'NONE',  ( 198.6587626159274294, 286.5599251108861267, 17.99840276545888784 ) ) ;
#89391=ORIENTED_EDGE ( 'NONE', *, *, #10962, .T. ) ;
#89392=CARTESIAN_POINT ( 'NONE',  ( 187.5500012533888423, 277.1004024971114745, 17.01394763479494898 ) ) ;
#89395=CARTESIAN_POINT ( 'NONE',  ( 175.6925083280133322, 275.2066185980531259, -17.63772206380936680 ) ) ;
#89396=CARTESIAN_POINT ( 'NONE',  ( 198.6433817073464922, 286.5865656260148171, -17.57789766230896689 ) ) ;
#89397=CARTESIAN_POINT ( 'NONE',  ( 148.2514616260410776, 273.8679314977858894, -10.42361479059151996 ) ) ;
#89398=ORIENTED_EDGE ( 'NONE', *, *, #1901, .F. ) ;
#89399=CARTESIAN_POINT ( 'NONE',  ( 170.4959927957777097, 255.7634325838962184, -12.27116094425178616 ) ) ;
#89403=CARTESIAN_POINT ( 'NONE',  ( 28.07773955407504118, 197.0177522451419350, 5.000000000000046185 ) ) ;
#89404=CARTESIAN_POINT ( 'NONE',  ( 106.3175485811169239, 238.3149278399160949, -9.188101187500095079 ) ) ;
#89405=CARTESIAN_POINT ( 'NONE',  ( 183.9039741337527403, 297.0480174192951495, -2.803343177518471396 ) ) ;
#89406=CARTESIAN_POINT ( 'NONE',  ( 167.7101951474509463, 282.4104349734390098, -10.63977280035835449 ) ) ;
#89408=DIRECTION ( 'NONE',  ( -0.8660254037844387076, -0.4999999999999998890, -0.000000000000000000 ) ) ;
#89409=CARTESIAN_POINT ( 'NONE',  ( 24.04513522159523475, 190.8149278399161233, 9.188101187500093303 ) ) ;
#89410=CARTESIAN_POINT ( 'NONE',  ( 161.7587802986029999, 250.4725692828850754, 14.33336164792646450 ) ) ;
#89413=DIRECTION ( 'NONE',  ( -0.8660254037844387076, -0.4999999999999998890, -0.000000000000000000 ) ) ;
#89417=CARTESIAN_POINT ( 'NONE',  ( 161.0965315767822972, 251.6196177163260188, -13.76772246540905442 ) ) ;
#89419=CARTESIAN_POINT ( 'NONE',  ( 55.03304057046344866, 193.3923013555409796, 4.594050593750050204 ) ) ;
#89420=CARTESIAN_POINT ( 'NONE',  ( 84.80240350195578003, 229.7677522451419350, -5.000000000000047962 ) ) ;
#89423=CARTESIAN_POINT ( 'NONE',  ( 194.7831888682312638, 266.3050563660650027, -7.630817898648720288 ) ) ;
#89424=CARTESIAN_POINT ( 'NONE',  ( 178.7614077125761298, 259.1314107520656194, -10.22190746354665514 ) ) ;
#89426=CARTESIAN_POINT ( 'NONE',  ( 1.258015332399702757, 171.5333772461660828, 9.188101187500095079 ) ) ;
#89427=CARTESIAN_POINT ( 'NONE',  ( 198.4860348845112981, 286.8590983175747056, -18.20461732983060088 ) ) ;
#89429=CARTESIAN_POINT ( 'NONE',  ( 147.5749398328735822, 275.0397016159798227, -4.620786157167191099 ) ) ;
#89430=EDGE_CURVE ( 'NONE', #94451, #43534, #68262, .T. ) ;
#89431=CARTESIAN_POINT ( 'NONE',  ( 208.0045976720423084, 270.3724639545367836, 2.002128742561712471 ) ) ;
#89434=CARTESIAN_POINT ( 'NONE',  ( 207.2383675728608239, 271.6996134166075763, 7.873592648726489784 ) ) ;
#89435=ORIENTED_EDGE ( 'NONE', *, *, #2397, .T. ) ;
#89436=CARTESIAN_POINT ( 'NONE',  ( -5.967884128652756637, 167.3615022471902591, -10.00000000000009592 ) ) ;
#89438=CARTESIAN_POINT ( 'NONE',  ( 126.7237928014352804, 231.7202760586659736, -5.415160957724236172E-17 ) ) ;
#89442=CARTESIAN_POINT ( 'NONE',  ( 179.9400117196032340, 293.3606267625540340, -7.512348598490236284 ) ) ;
#89443=CARTESIAN_POINT ( 'NONE',  ( 157.8562613713738472, 257.2319303423452652, 17.81420683562559404 ) ) ;
#89446=ORIENTED_EDGE ( 'NONE', *, *, #86391, .T. ) ;
#89447=CARTESIAN_POINT ( 'NONE',  ( 191.5694344253287511, 298.8390017285333897, 8.250976118904059575 ) ) ;
#89448=CARTESIAN_POINT ( 'NONE',  ( 207.9188266366356572, 270.5210237456789173, -1.812149220496467317 ) ) ;
#89449=CARTESIAN_POINT ( 'NONE',  ( 168.7096392155106344, 280.2107777274362093, -14.47775774749160682 ) ) ;
#89450=CARTESIAN_POINT ( 'NONE',  ( 172.7932728846461998, 268.7208518688015602, -16.72593362587508992 ) ) ;
#89460=CARTESIAN_POINT ( 'NONE',  ( 197.2265362901041499, 271.3495626856545755, 12.05940019673365882 ) ) ;
#89461=CARTESIAN_POINT ( 'NONE',  ( 182.0535125315628875, 295.0180786344971011, 4.789782204045892833 ) ) ;
#89462=CARTESIAN_POINT ( 'NONE',  ( 183.6422324172568210, 264.5785696717482551, 14.31652553825990104 ) ) ;
#89463=CARTESIAN_POINT ( 'NONE',  ( 150.7717849006677397, 278.2227778944624674, -0.0001987781867447356013 ) ) ;
#89464=ORIENTED_EDGE ( 'NONE', *, *, #91884, .F. ) ;
#89468=CARTESIAN_POINT ( 'NONE',  ( 169.8382097412835492, 278.9609387177634403, 15.53294725421295475 ) ) ;
#89469=CARTESIAN_POINT ( 'NONE',  ( 147.6054094044680198, 274.9869267698931594, -8.596541856229405809 ) ) ;
#89470=CARTESIAN_POINT ( 'NONE',  ( 156.0496192001932911, 261.9777799244599805, -16.96333935241061397 ) ) ;
#89477=CARTESIAN_POINT ( 'NONE',  ( 80.66154599400290692, 223.5024278399160949, -9.188101187500093303 ) ) ;
#89478=CARTESIAN_POINT ( 'NONE',  ( 155.0032822503481498, 262.1734351328947241, 17.58937370742663830 ) ) ;
#89480=CARTESIAN_POINT ( 'NONE',  ( 184.8337230598654628, 259.8048592364006595, -5.814933208005341747 ) ) ;
#89482=EDGE_CURVE ( 'NONE', #82234, #66081, #70594, .T. ) ;
#89484=DIRECTION ( 'NONE',  ( 0.5000000000000048850, -0.8660254037844358210, 0.000000000000000000 ) ) ;
#89485=ORIENTED_EDGE ( 'NONE', *, *, #69149, .F. ) ;
#89486=CARTESIAN_POINT ( 'NONE',  ( 192.6310446484023089, 294.0709696340792902, 14.41910184865714584 ) ) ;
#89491=ADVANCED_FACE ( 'NONE', ( #11823 ), #88044, .F. ) ;
#89492=CARTESIAN_POINT ( 'NONE',  ( 182.8998698049672100, 279.8255271273169456, -17.32748555055102813 ) ) ;
#89494=CARTESIAN_POINT ( 'NONE',  ( 147.1444650661958065, 275.7853057832419381, -6.658585314799819521 ) ) ;
#89498=EDGE_CURVE ( 'NONE', #31479, #83705, #25949, .T. ) ;
#89499=CARTESIAN_POINT ( 'NONE',  ( 134.8963869060034142, 254.8149278399161233, -9.188101187500095079 ) ) ;
#89500=CARTESIAN_POINT ( 'NONE',  ( 195.7590296971629300, 291.5824098545663219, -17.26820314939903156 ) ) ;
#89505=CARTESIAN_POINT ( 'NONE',  ( 197.9901163037401943, 272.1418500761980681, -13.83221381771805625 ) ) ;
#89506=CARTESIAN_POINT ( 'NONE',  ( 203.0372054888979392, 271.5441584837204800, 9.486415998612690359 ) ) ;
#89507=EDGE_LOOP ( 'NONE', ( #63658, #13234, #60031, #58626 ) ) ;
#89510=CARTESIAN_POINT ( 'NONE',  ( -0.4289299871626708338, 163.8927522451418213, 10.00000000000009948 ) ) ;
#89512=CARTESIAN_POINT ( 'NONE',  ( 156.7314430005651786, 279.2576428315608723, 7.355496758818486747 ) ) ;
#89517=VERTEX_POINT ( 'NONE', #93315 ) ;
#89518=CARTESIAN_POINT ( 'NONE',  ( 147.6508870500795467, 274.9081571770856272, -8.950912509993816712 ) ) ;
#89520=CARTESIAN_POINT ( 'NONE',  ( 160.4603375272029382, 276.0096574431570389, 12.65041034736400505 ) ) ;
#89523=CARTESIAN_POINT ( 'NONE',  ( 149.5633513747893346, 271.5956717990251832, 12.83777201928511325 ) ) ;
#89524=CARTESIAN_POINT ( 'NONE',  ( 160.7925456682749257, 272.6590809960079014, 15.51096013201097534 ) ) ;
#89528=CARTESIAN_POINT ( 'NONE',  ( 158.8270733235451075, 260.0119502166541565, 17.68969926203419618 ) ) ;
#89532=CARTESIAN_POINT ( 'NONE',  ( 117.1033946842824633, 249.9637435831424739, 2.679491924311251605 ) ) ;
#89536=CARTESIAN_POINT ( 'NONE',  ( 152.8522706834672533, 265.8990964544007056, 17.63080661522264947 ) ) ;
#89538=CARTESIAN_POINT ( 'NONE',  ( 202.7282074973916792, 277.5114398175890642, -15.40750263959311184 ) ) ;
#89539=CARTESIAN_POINT ( 'NONE',  ( -0.5554856785977280165, 179.6744531367911577, 4.594050593750047540 ) ) ;
#89540=CARTESIAN_POINT ( 'NONE',  ( 95.24857461505581568, 234.9869531367911293, 4.594050593750046652 ) ) ;
#89541=CARTESIAN_POINT ( 'NONE',  ( 154.9048824156581361, 262.3438686460345366, -17.40627786727128168 ) ) ;
#89542=CARTESIAN_POINT ( 'NONE',  ( 48.99872857692556494, 187.5494855054051868, -2.679491924311248496 ) ) ;
#89543=CARTESIAN_POINT ( 'NONE',  ( 180.5275139809070595, 254.9285515434814329, -2.470345461842613499 ) ) ;
#89548=CARTESIAN_POINT ( 'NONE',  ( 194.1972774922283236, 294.2874440223457100, -15.09915398317898649 ) ) ;
#89552=CARTESIAN_POINT ( 'NONE',  ( 172.9031624820008233, 263.9926013823168205, -15.45005316810910578 ) ) ;
#89553=CARTESIAN_POINT ( 'NONE',  ( 80.66154599400290692, 223.5024278399160949, -9.188101187500093303 ) ) ;
#89554=CARTESIAN_POINT ( 'NONE',  ( 207.8718670335145475, 270.6023601641878713, -6.322166851501095586 ) ) ;
#89558=CARTESIAN_POINT ( 'NONE',  ( 190.5217943342473745, 281.4870030958396683, 17.81127109971334121 ) ) ;
#89559=CARTESIAN_POINT ( 'NONE',  ( 152.3267809444392071, 266.8092713812532679, 15.53817502085608204 ) ) ;
#89560=CARTESIAN_POINT ( 'NONE',  ( 151.3999564459286375, 268.4145785023736153, -15.40574304386609050 ) ) ;
#89562=CARTESIAN_POINT ( 'NONE',  ( 146.9978162861947908, 276.0393089210717790, -5.134868500856280882 ) ) ;
#89568=CARTESIAN_POINT ( 'NONE',  ( 55.51991954004235907, 212.8615022471903160, 5.000000000000046185 ) ) ;
#89573=CARTESIAN_POINT ( 'NONE',  ( 153.6515342823389290, 266.9718399987636417, 16.58081301308793698 ) ) ;
#89574=CARTESIAN_POINT ( 'NONE',  ( 186.2855123196275713, 281.1790728086402282, -17.65699997733639037 ) ) ;
#89575=CARTESIAN_POINT ( 'NONE',  ( 135.6272693901029243, 259.1115022471903444, -5.000000000000047962 ) ) ;
#89576=( BOUNDED_CURVE ( )  B_SPLINE_CURVE ( 2, ( #43608, #50707, #58795, #74545, #18342, #12234, #43094, #74036, #35517 ),
 .UNSPECIFIED., .F., .T. ) 
 B_SPLINE_CURVE_WITH_KNOTS ( ( 3, 2, 2, 2, 3 ),
 ( 0.2862903225806451846, 0.2876344086021505597, 0.2903225806451613100, 0.2930107526881720603, 0.2943548387096774355 ),
 .UNSPECIFIED. ) 
 CURVE ( )  GEOMETRIC_REPRESENTATION_ITEM ( )  RATIONAL_B_SPLINE_CURVE ( ( 0.9330127018922194093, 0.9330127018922194093, 1.000000000000000000, 0.8660254037844387076, 1.000000000000000000, 0.8660254037844387076, 1.000000000000000000, 0.9330127018922194093, 0.9330127018922194093 ) ) 
 REPRESENTATION_ITEM ( '' )  );
#89581=CARTESIAN_POINT ( 'NONE',  ( 168.7200283246967274, 248.5543435357514568, -1.887890150557830271 ) ) ;
#89588=CARTESIAN_POINT ( 'NONE',  ( 192.7874605187217014, 292.5376213369709149, 15.36506066506490598 ) ) ;
#89589=CARTESIAN_POINT ( 'NONE',  ( 158.3666238253319705, 256.3479566418141076, 17.18714134412729777 ) ) ;
#89590=CARTESIAN_POINT ( 'NONE',  ( 157.7201504851624918, 257.9064828177920958, -16.69192179801337161 ) ) ;
#89591=CARTESIAN_POINT ( 'NONE',  ( 204.1512742367690976, 273.0118811181309866, 11.00484496069812224 ) ) ;
#89597=( BOUNDED_CURVE ( )  B_SPLINE_CURVE ( 2, ( #36664, #98504, #83315, #13877, #75691, #37172, #68070, #16371, #55350 ),
 .UNSPECIFIED., .F., .T. ) 
 B_SPLINE_CURVE_WITH_KNOTS ( ( 3, 2, 2, 2, 3 ),
 ( 0.5040322580645161255, 0.5053763440860215006, 0.5080645161290322509, 0.5107526881720430012, 0.5120967741935483764 ),
 .UNSPECIFIED. ) 
 CURVE ( )  GEOMETRIC_REPRESENTATION_ITEM ( )  RATIONAL_B_SPLINE_CURVE ( ( 0.9330127018922194093, 0.9330127018922194093, 1.000000000000000000, 0.8660254037844387076, 1.000000000000000000, 0.8660254037844387076, 1.000000000000000000, 0.9330127018922194093, 0.9330127018922194093 ) ) 
 REPRESENTATION_ITEM ( '' )  );
#89598=CARTESIAN_POINT ( 'NONE',  ( 190.1058098001619499, 300.4953350946266823, 0.1248780210120518375 ) ) ;
#89599=ORIENTED_EDGE ( 'NONE', *, *, #46124, .T. ) ;
#89602=ADVANCED_FACE ( 'NONE', ( #92814 ), #59716, .F. ) ;
#89603=CARTESIAN_POINT ( 'NONE',  ( 163.7010375032499212, 247.1084811230698506, 6.649922295230481950 ) ) ;
#89606=DIRECTION ( 'NONE',  ( 0.8660254037844395958, 0.4999999999999985567, 0.000000000000000000 ) ) ;
#89611=CARTESIAN_POINT ( 'NONE',  ( 161.5780152162786294, 275.6215250102659979, -14.77109549141536604 ) ) ;
#89613=CARTESIAN_POINT ( 'NONE',  ( 182.0331739629101833, 256.8600016389484608, 5.117587312389543008 ) ) ;
#89615=CARTESIAN_POINT ( 'NONE',  ( 94.19319292813476352, 231.3149278399160664, 9.188101187500093303 ) ) ;
#89618=CARTESIAN_POINT ( 'NONE',  ( 163.2872205587920007, 276.9580280363520046, -14.32771847714696989 ) ) ;
#89619=ORIENTED_EDGE ( 'NONE', *, *, #64577, .F. ) ;
#89623=CARTESIAN_POINT ( 'NONE',  ( 176.7665383743514838, 292.6345017810178888, -2.761319672360143862 ) ) ;
#89624=CARTESIAN_POINT ( 'NONE',  ( 157.1135969804030310, 258.5182628004787944, 17.19660297500358226 ) ) ;
#89625=CARTESIAN_POINT ( 'NONE',  ( 206.3454060440500086, 273.2462681537123785, -9.268083217908118954 ) ) ;
#89626=CARTESIAN_POINT ( 'NONE',  ( 207.1975773162273811, 271.0654058925244954, -3.690837417035307766 ) ) ;
#89628=ORIENTED_EDGE ( 'NONE', *, *, #59084, .T. ) ;
#89631=CARTESIAN_POINT ( 'NONE',  ( 194.7008455304638233, 266.4113774656392479, -8.389308597226909470 ) ) ;
#89632=CARTESIAN_POINT ( 'NONE',  ( 153.2303786119591678, 265.7391886871019437, 16.12463036271180883 ) ) ;
#89634=CARTESIAN_POINT ( 'NONE',  ( 131.9738982639959488, 240.8768266524160140, -9.188101187500091527 ) ) ;
#89636=CARTESIAN_POINT ( 'NONE',  ( 156.9694903541507074, 266.1758412851487492, -17.34135443527054576 ) ) ;
#89638=CARTESIAN_POINT ( 'NONE',  ( 146.8516045228164160, 276.2925551239072774, 3.995954059407343273 ) ) ;
#89640=CARTESIAN_POINT ( 'NONE',  ( 159.7692415128758228, 253.9185515433934768, -16.85856106119654285 ) ) ;
#89641=CARTESIAN_POINT ( 'NONE',  ( 170.4855375986076638, 248.6613294790634541, -0.2716024841417116753 ) ) ;
#89642=CARTESIAN_POINT ( 'NONE',  ( 178.5227689348290028, 285.2834003422560727, 13.20235085433959732 ) ) ;
#89643=B_SPLINE_CURVE_WITH_KNOTS ( 'NONE', 3,
 ( #64769, #20171, #65742, #10569 ),
 .UNSPECIFIED., .F., .F.,
 ( 4, 4 ),
 ( 0.03159426384393204668, 0.04060813801016246311 ),
 .UNSPECIFIED. ) ;
#89645=CARTESIAN_POINT ( 'NONE',  ( 196.6627808473781158, 280.4533039363431044, -16.65813739920714909 ) ) ;
#89646=CARTESIAN_POINT ( 'NONE',  ( 130.4311169673963775, 236.1115022471901739, -5.000000000000041744 ) ) ;
#89649=CARTESIAN_POINT ( 'NONE',  ( 159.9770824720811220, 253.5585604421560788, -16.42166711341322483 ) ) ;
#89651=CARTESIAN_POINT ( 'NONE',  ( 207.6163508138795635, 271.0449272387537576, -1.385071889578343152 ) ) ;
#89653=CARTESIAN_POINT ( 'NONE',  ( -22.42236680055709641, 157.8615022471902591, 0.000000000000000000 ) ) ;
#89654=AXIS2_PLACEMENT_3D ( 'NONE', #84689, #36545, #28969 ) ;
#89656=CARTESIAN_POINT ( 'NONE',  ( 173.4026771546767804, 273.2456497557084845, -17.70700034978624515 ) ) ;
#89660=CARTESIAN_POINT ( 'NONE',  ( 149.7259699431006652, 272.1435073784675751, -11.43438802284230249 ) ) ;
#89661=CARTESIAN_POINT ( 'NONE',  ( 203.1044072055706806, 278.8598428092302584, -16.67109798570195878 ) ) ;
#89664=CARTESIAN_POINT ( 'NONE',  ( 12.00188267627663308, 186.9244531367911293, -4.594050593750046652 ) ) ;
#89666=CARTESIAN_POINT ( 'NONE',  ( 43.32339510341152788, 202.4865022471903160, -10.00000000000009592 ) ) ;
#89670=EDGE_CURVE ( 'NONE', #53889, #86525, #29513, .T. ) ;
#89673=CARTESIAN_POINT ( 'NONE',  ( 29.24128764430186322, 193.8149278399160664, 9.188101187500093303 ) ) ;
#89675=CARTESIAN_POINT ( 'NONE',  ( 151.1699610800269511, 268.8129421616204695, -14.28929860221299286 ) ) ;
#89676=CARTESIAN_POINT ( 'NONE',  ( 190.9335643195044838, 299.9403610588350944, -4.692880224846124548 ) ) ;
#89678=CARTESIAN_POINT ( 'NONE',  ( 203.2115566785326450, 269.6228474973083280, -7.486280564945728244 ) ) ;
#89679=CARTESIAN_POINT ( 'NONE',  ( 178.7545946287733898, 293.8895248776133258, 2.709369586333742586 ) ) ;
#89680=CARTESIAN_POINT ( 'NONE',  ( 179.7878600106018894, 276.7683181353822874, 16.31861665154247376 ) ) ;
#89681=CARTESIAN_POINT ( 'NONE',  ( 181.0417453565561914, 279.3340925255673710, -16.14945566808648891 ) ) ;
#89685=EDGE_CURVE ( 'NONE', #66081, #79277, #88795, .T. ) ;
#89688=CARTESIAN_POINT ( 'NONE',  ( 96.22311351791105949, 216.3615022471902023, 5.000000000000051514 ) ) ;
#89689=CARTESIAN_POINT ( 'NONE',  ( 7.984193807443177526, 186.9637435831424739, 2.679491924311251605 ) ) ;
#89691=ORIENTED_EDGE ( 'NONE', *, *, #99932, .T. ) ;
#89692=CARTESIAN_POINT ( 'NONE',  ( 59.22776434610305785, 198.8768266524159856, -9.188101187500091527 ) ) ;
#89693=ORIENTED_EDGE ( 'NONE', *, *, #37903, .T. ) ;
#89696=LINE ( 'NONE', #43533, #22381 ) ;
#89699=CARTESIAN_POINT ( 'NONE',  ( 207.4285356523023154, 271.3702326410368642, 7.833982582429932506 ) ) ;
#89702=CARTESIAN_POINT ( 'NONE',  ( 185.8599028000333817, 262.9727172135272326, 11.31732244974326207 ) ) ;
#89704=CARTESIAN_POINT ( 'NONE',  ( 156.7423333928520890, 259.1613101971172455, 17.21575223094429319 ) ) ;
#89705=VERTEX_POINT ( 'NONE', #63205 ) ;
#89710=EDGE_LOOP ( 'NONE', ( #71692, #82007, #8359 ) ) ;
#89712=CARTESIAN_POINT ( 'NONE',  ( 191.5766842709549280, 298.8264446275616137, 8.039910086100929831 ) ) ;
#89716=CARTESIAN_POINT ( 'NONE',  ( 207.5785076975260779, 271.1104734389944042, -6.824813054587777650 ) ) ;
#89718=CARTESIAN_POINT ( 'NONE',  ( 196.4501996009505831, 290.3852684645433442, -17.82325615854289680 ) ) ;
#89724=CARTESIAN_POINT ( 'NONE',  ( 121.0403275412173656, 234.5643266524160140, 9.188101187500095079 ) ) ;
#89725=CARTESIAN_POINT ( 'NONE',  ( 111.9072422615758313, 246.9637435831425023, 2.679491924311251605 ) ) ;
#89726=CARTESIAN_POINT ( 'NONE',  ( 85.81045474425822306, 231.8967562850347122, -4.648177544792955347E-16 ) ) ;
#89728=CARTESIAN_POINT ( 'NONE',  ( 164.4698008747318738, 245.7769439046653019, -6.272955660526681854 ) ) ;
#89730=EDGE_LOOP ( 'NONE', ( #20911, #98311, #16557, #48610 ) ) ;
#89731=CARTESIAN_POINT ( 'NONE',  ( 198.5558597050348908, 286.7381581807989051, 17.16554469393394200 ) ) ;
#89733=CARTESIAN_POINT ( 'NONE',  ( 71.05451054047556170, 202.6423013555409796, -4.594050593750043987 ) ) ;
#89734=CARTESIAN_POINT ( 'NONE',  ( 14.31700456906896868, 190.6199935810940929, 2.679491924311251605 ) ) ;
#89736=CARTESIAN_POINT ( 'NONE',  ( 198.0355408163131585, 287.6393769322024241, 18.20720360189982756 ) ) ;
#89737=CARTESIAN_POINT ( 'NONE',  ( -18.22861911365886201, 171.8297689869269504, -2.679491924311252049 ) ) ;
#89741=CARTESIAN_POINT ( 'NONE',  ( 201.4617167010348737, 281.7050662241970826, -17.43131506460443703 ) ) ;
#89742=CARTESIAN_POINT ( 'NONE',  ( 203.3205561747472814, 278.4854618126124706, -15.14439614831292147 ) ) ;
#89743=EDGE_LOOP ( 'NONE', ( #95865, #51419, #47068, #24243 ) ) ;
#89745=CARTESIAN_POINT ( 'NONE',  ( 160.4627341472859428, 258.2288165694186546, -16.94036994928822182 ) ) ;
#89746=CARTESIAN_POINT ( 'NONE',  ( 164.2540650184052708, 246.7815632513715514, 5.192739529124178688 ) ) ;
#89747=AXIS2_PLACEMENT_3D ( 'NONE', #34609, #42690, #65509 ) ;
#89751=ORIENTED_EDGE ( 'NONE', *, *, #42911, .F. ) ;
#89752=CARTESIAN_POINT ( 'NONE',  ( 163.7012083107868534, 247.1081852757374975, -6.544933039329257518 ) ) ;
#89753=CARTESIAN_POINT ( 'NONE',  ( 121.5540962550081190, 250.1744531367911009, 4.594050593750047540 ) ) ;
#89755=CARTESIAN_POINT ( 'NONE',  ( 146.7434471017767521, 276.4798892723637209, 0.7354350123930684102 ) ) ;
#89758=CARTESIAN_POINT ( 'NONE',  ( 204.4781092559247782, 276.4805210635553863, 13.30606382016679490 ) ) ;
#89760=ORIENTED_EDGE ( 'NONE', *, *, #26633, .T. ) ;
#89762=CARTESIAN_POINT ( 'NONE',  ( 183.4890902768438536, 276.5613345365970304, -16.51246737540926546 ) ) ;
#89763=CARTESIAN_POINT ( 'NONE',  ( 166.7438987807396416, 248.6309438778351364, -5.495826098545110838 ) ) ;
#89764=CARTESIAN_POINT ( 'NONE',  ( 165.0260329286864760, 244.8135217264176049, -2.114260670082726890 ) ) ;
#89765=CARTESIAN_POINT ( 'NONE',  ( 200.2169152151696210, 267.0719894846549778, 0.8300188801736234634 ) ) ;
#89766=CARTESIAN_POINT ( 'NONE',  ( 172.6012549852709412, 290.2025030293380610, -5.021894074213228087 ) ) ;
#89767=CARTESIAN_POINT ( 'NONE',  ( 196.2134504588463244, 270.7881804218938555, 11.99659543724280830 ) ) ;
#89769=CARTESIAN_POINT ( 'NONE',  ( 149.7119746935222793, 271.3382486597900538, 12.05352563709836922 ) ) ;
#89770=CARTESIAN_POINT ( 'NONE',  ( 169.1470411999185046, 285.5095826478136587, -9.079696797922760965 ) ) ;
#89771=CARTESIAN_POINT ( 'NONE',  ( 202.7676489560256528, 279.4431252073101746, -16.04062356091568020 ) ) ;
#89772=CARTESIAN_POINT ( 'NONE',  ( 161.2700728932001368, 251.3190353390782263, 13.72566802940053421 ) ) ;
#89773=CARTESIAN_POINT ( 'NONE',  ( 134.6710330032098000, 241.8927522451418213, 10.00000000000009592 ) ) ;
#89774=CARTESIAN_POINT ( 'NONE',  ( 183.0161482713612031, 278.8971254581520611, 17.42167469373847055 ) ) ;
#89776=CARTESIAN_POINT ( 'NONE',  ( 157.7861133721078772, 257.3534302411229646, 18.03837896619386783 ) ) ;
#89777=CARTESIAN_POINT ( 'NONE',  ( 151.4188942279983223, 268.3817773016460251, -14.77302265413830895 ) ) ;
#89778=CARTESIAN_POINT ( 'NONE',  ( -1.935626891937929139, 175.8149278399161233, 9.188101187500093303 ) ) ;
#89779=CARTESIAN_POINT ( 'NONE',  ( 55.03304057046344866, 193.3923013555409796, 4.594050593750050204 ) ) ;
#89783=CARTESIAN_POINT ( 'NONE',  ( 204.8385597977314490, 275.8562024115307167, -12.64672659107585240 ) ) ;
#89786=CARTESIAN_POINT ( 'NONE',  ( 170.4061711814250941, 277.8873091166869358, -16.16315208799353442 ) ) ;
#89787=CARTESIAN_POINT ( 'NONE',  ( 179.4666841005951312, 254.9493157538499304, -4.056432808702910009 ) ) ;
#89788=CARTESIAN_POINT ( 'NONE',  ( 198.7520972810255842, 286.3982647288286785, 17.58825518441947722 ) ) ;
#89791=EDGE_CURVE ( 'NONE', #58170, #42330, #1722, .T. ) ;
#89792=CARTESIAN_POINT ( 'NONE',  ( 59.85004655896462111, 195.3615022471901739, 5.000000000000051514 ) ) ;
#89793=CARTESIAN_POINT ( 'NONE',  ( 181.2925019527557993, 292.4819523310474096, 9.067989712515277745 ) ) ;
#89794=CARTESIAN_POINT ( 'NONE',  ( 163.1953264782998758, 283.8895661455310915, -7.125257539458086598 ) ) ;
#89795=EDGE_CURVE ( 'NONE', #34942, #23533, #56041, .T. ) ;
#89796=CARTESIAN_POINT ( 'NONE',  ( 20.58103360645747770, 188.8149278399161233, -9.188101187500095079 ) ) ;
#89797=CARTESIAN_POINT ( 'NONE',  ( 167.4367084379770461, 285.8522310990644542, 4.088904900943554743 ) ) ;
#89801=CARTESIAN_POINT ( 'NONE',  ( 161.3261849411383650, 273.2032229615781489, 15.91718547624222957 ) ) ;
#89803=CARTESIAN_POINT ( 'NONE',  ( 183.2210599555355088, 278.9435890925142303, 16.90865785365091156 ) ) ;
#89805=CARTESIAN_POINT ( 'NONE',  ( 124.8019518427975356, 232.8615022471901739, 5.000000000000051514 ) ) ;
#89806=CARTESIAN_POINT ( 'NONE',  ( 143.9266795097038596, 247.2365022471902023, 10.00000000000009948 ) ) ;
#89813=ORIENTED_EDGE ( 'NONE', *, *, #77485, .T. ) ;
#89814=CARTESIAN_POINT ( 'NONE',  ( 182.1439385020048860, 290.0253507885926183, 13.01467259685074573 ) ) ;
#89818=ORIENTED_EDGE ( 'NONE', *, *, #76246, .T. ) ;
#89819=FACE_OUTER_BOUND ( 'NONE', #4298, .T. ) ;
#89822=CARTESIAN_POINT ( 'NONE',  ( 155.6281496932864457, 261.0911329737299980, -18.07904265579665548 ) ) ;
#89825=CARTESIAN_POINT ( 'NONE',  ( -22.42236680055709641, 157.8615022471902591, 0.000000000000000000 ) ) ;
#89826=CARTESIAN_POINT ( 'NONE',  ( 163.9942050550062049, 246.6007000282974673, 5.791111691696777974 ) ) ;
#89827=CARTESIAN_POINT ( 'NONE',  ( 153.1745822862813498, 265.3408363824576668, 16.18092354043443493 ) ) ;
#89828=VERTEX_POINT ( 'NONE', #8512 ) ;
#89831=CARTESIAN_POINT ( 'NONE',  ( 174.5613027801699104, 262.3032192610774018, 14.37391627158726592 ) ) ;
#89835=B_SPLINE_CURVE_WITH_KNOTS ( 'NONE', 3,
 ( #22774, #14177, #53651, #7062 ),
 .UNSPECIFIED., .F., .F.,
 ( 4, 4 ),
 ( 0.009239321009562585091, 0.01510611881184145515 ),
 .UNSPECIFIED. ) ;
#89836=CARTESIAN_POINT ( 'NONE',  ( 149.4456112649506281, 271.7996036513546869, -12.95648166494593667 ) ) ;
#89840=CARTESIAN_POINT ( 'NONE',  ( 177.2486161470519903, 269.3311939352316813, 16.08193494513130872 ) ) ;
#89841=CARTESIAN_POINT ( 'NONE',  ( 206.3505875407052486, 273.2372935382459787, 11.62318091048137880 ) ) ;
#89844=CARTESIAN_POINT ( 'NONE',  ( 149.0761751337341821, 272.4394858007734683, 11.56094486755886130 ) ) ;
#89845=CARTESIAN_POINT ( 'NONE',  ( 171.7602284589083297, 263.3278815159662827, -15.48272920416244780 ) ) ;
#89846=ORIENTED_EDGE ( 'NONE', *, *, #27823, .T. ) ;
#89849=CARTESIAN_POINT ( 'NONE',  ( 158.9550220667411224, 269.6099541869315317, 15.63534711726525650 ) ) ;
#89850=CARTESIAN_POINT ( 'NONE',  ( 156.2799659027096482, 267.3694502300024851, -16.55794083374155079 ) ) ;
#89851=CARTESIAN_POINT ( 'NONE',  ( 168.9959839960517343, 272.4983489875348823, 17.21357309856028550 ) ) ;
#89853=CARTESIAN_POINT ( 'NONE',  ( 190.0791367161676817, 299.5868483356907177, -4.299622452797303929 ) ) ;
#89854=LINE ( 'NONE', #20429, #1002 ) ;
#89855=CARTESIAN_POINT ( 'NONE',  ( 192.8325075361489382, 296.6512949269187516, 11.74553025762331515 ) ) ;
#89856=CARTESIAN_POINT ( 'NONE',  ( 37.40555484421791732, 185.7365022471902023, 10.00000000000009948 ) ) ;
#89857=CARTESIAN_POINT ( 'NONE',  ( 196.9614093077011034, 289.4998272791294767, -17.73636689563254265 ) ) ;
#89860=EDGE_CURVE ( 'NONE', #52219, #31824, #67641, .T. ) ;
#89861=CARTESIAN_POINT ( 'NONE',  ( 165.0538309624641613, 244.7653741195639157, 2.311334310144196547 ) ) ;
#89864=CARTESIAN_POINT ( 'NONE',  ( 190.5326571414909154, 300.2205002393729956, 2.724935789587299872 ) ) ;
#89868=CARTESIAN_POINT ( 'NONE',  ( 195.3907986064563431, 271.8404647846490434, 14.62512701364267720 ) ) ;
#89869=CARTESIAN_POINT ( 'NONE',  ( 174.5502087336647890, 274.2231652844577070, -17.67598756992128983 ) ) ;
#89871=CARTESIAN_POINT ( 'NONE',  ( 160.0818573676674248, 253.3770849996428467, -14.73248899536566725 ) ) ;
#89872=CARTESIAN_POINT ( 'NONE',  ( 148.5965889108988733, 273.2701535053342354, -9.061290301873665243 ) ) ;
#89874=CARTESIAN_POINT ( 'NONE',  ( 167.4572242298301319, 253.2714284328981762, -12.01198848564598798 ) ) ;
#89875=CARTESIAN_POINT ( 'NONE',  ( 205.6309316812484553, 272.7254639723831815, 10.07723110209571438 ) ) ;
#89876=CARTESIAN_POINT ( 'NONE',  ( 153.1627746953036535, 265.3612877299463548, -17.72069958822647351 ) ) ;
#89877=CARTESIAN_POINT ( 'NONE',  ( 164.2953672501826929, 246.0790718049323687, -2.576662677987826111 ) ) ;
#89879=CARTESIAN_POINT ( 'NONE',  ( 24.54146915528859196, 191.6427522451419350, 10.00000000000009237 ) ) ;
#89880=CARTESIAN_POINT ( 'NONE',  ( 124.1796696299359724, 236.3768266524159856, -9.188101187500093303 ) ) ;
#89882=CARTESIAN_POINT ( 'NONE',  ( 164.9647332961995403, 281.3995515670802092, -11.83162694151289429 ) ) ;
#89883=CARTESIAN_POINT ( 'NONE',  ( 157.1837449796689725, 258.3967629017010381, 16.97243084443542216 ) ) ;
#89884=CARTESIAN_POINT ( 'NONE',  ( 207.6256228060221076, 271.0288676772754002, 1.885008341157026646 ) ) ;
#89885=CARTESIAN_POINT ( 'NONE',  ( 38.60536087060361154, 193.0958772461660544, -9.188101187500095079 ) ) ;
#89886=CARTESIAN_POINT ( 'NONE',  ( 161.5431944097339851, 250.8459749958011287, 14.52339846942414603 ) ) ;
#89894=FACE_OUTER_BOUND ( 'NONE', #33871, .T. ) ;
#89895=CARTESIAN_POINT ( 'NONE',  ( 176.1937425061808256, 285.1457250574052296, -12.61256593275989601 ) ) ;
#89896=DIRECTION ( 'NONE',  ( -0.8660254037844387076, -0.4999999999999998890, -0.000000000000000000 ) ) ;
#89897=CARTESIAN_POINT ( 'NONE',  ( 98.29796604426333317, 220.8927522451418213, 10.00000000000009592 ) ) ;
#89899=CARTESIAN_POINT ( 'NONE',  ( 198.6181852710878104, 267.3834214339108257, -8.306438527148390705 ) ) ;
#89900=CARTESIAN_POINT ( 'NONE',  ( 158.5924551307156491, 281.8915015218287863, -1.614670045172950763 ) ) ;
#89902=CARTESIAN_POINT ( 'NONE',  ( 7.238742955462222461, 184.1744531367911293, 4.594050593750047540 ) ) ;
#89903=CARTESIAN_POINT ( 'NONE',  ( 151.1126408083691501, 268.9122237844355254, -15.82705194100464396 ) ) ;
#89908=CARTESIAN_POINT ( 'NONE',  ( 46.88655524640979166, 204.0024278399160949, -9.188101187500093303 ) ) ;
#89909=CARTESIAN_POINT ( 'NONE',  ( 164.4578252119609090, 245.7976863610386999, -6.211333091911165560 ) ) ;
#89910=CARTESIAN_POINT ( 'NONE',  ( 204.9427641582406636, 275.6757151647582305, 14.40446820030680897 ) ) ;
#89915=CARTESIAN_POINT ( 'NONE',  ( 2.620201125542898080, 178.9865022471903160, 10.00000000000009237 ) ) ;
#89917=CARTESIAN_POINT ( 'NONE',  ( 134.5180214354952284, 236.2202760586659736, -5.415160957724236172E-17 ) ) ;
#89919=CARTESIAN_POINT ( 'NONE',  ( 183.8381394033181095, 262.6696733492485691, 12.83785572541065356 ) ) ;
#89920=EDGE_CURVE ( 'NONE', #89828, #70911, #31822, .T. ) ;
#89921=DIRECTION ( 'NONE',  ( -0.8660254037844387076, -0.4999999999999998890, -0.000000000000000000 ) ) ;
#89923=CARTESIAN_POINT ( 'NONE',  ( 157.4177733328310467, 257.9914139036126812, 18.29188238796808363 ) ) ;
#89924=CARTESIAN_POINT ( 'NONE',  ( 189.3135512084097627, 289.8933911928067459, 14.45002620918027603 ) ) ;
#89926=ORIENTED_EDGE ( 'NONE', *, *, #62303, .T. ) ;
#89927=CARTESIAN_POINT ( 'NONE',  ( 151.2455280670316711, 268.6820563007532314, 14.35914944935941229 ) ) ;
#89928=CARTESIAN_POINT ( 'NONE',  ( 163.4095610489648323, 247.6133331511015570, 7.708395487792730094 ) ) ;
#89930=CARTESIAN_POINT ( 'NONE',  ( 170.0748205669605966, 266.3782777737114884, -16.69754429407689145 ) ) ;
#89931=CARTESIAN_POINT ( 'NONE',  ( 197.3031208747801770, 273.3096235846996933, -13.48493542629869424 ) ) ;
#89934=CARTESIAN_POINT ( 'NONE',  ( 170.3926468640515282, 283.5039894459525271, -11.04026963884475698 ) ) ;
#89937=CARTESIAN_POINT ( 'NONE',  ( 196.1373634161230939, 271.0470652014707298, 12.52493849620521438 ) ) ;
#89940=CARTESIAN_POINT ( 'NONE',  ( 181.8805694890828590, 295.3104365690353461, 4.888136459776745824 ) ) ;
#89942=CARTESIAN_POINT ( 'NONE',  ( 150.4247937244904847, 277.5422073757840735, -0.0002234595357659979081 ) ) ;
#89944=CARTESIAN_POINT ( 'NONE',  ( 191.9824032073976241, 287.6194387751458521, -17.05427143794285882 ) ) ;
#89948=CARTESIAN_POINT ( 'NONE',  ( 156.2927583276759265, 261.4325586500398799, -17.29092458739067339 ) ) ;
#89949=ORIENTED_EDGE ( 'NONE', *, *, #93952, .T. ) ;
#89951=CARTESIAN_POINT ( 'NONE',  ( 185.2906591010065824, 291.2658010436550740, 11.98603346923743196 ) ) ;
#89952=CARTESIAN_POINT ( 'NONE',  ( 164.3961040135806968, 245.9045906125373904, 7.095190383188031191 ) ) ;
#89956=CARTESIAN_POINT ( 'NONE',  ( 85.69549220138247847, 220.2833772461660544, -9.188101187500095079 ) ) ;
#89958=CARTESIAN_POINT ( 'NONE',  ( 189.9427917847951335, 300.2559228831493101, 3.234880823342468403 ) ) ;
#89962=CARTESIAN_POINT ( 'NONE',  ( -3.078821053925192786, 157.4824982072974251, -4.415768667553307481E-15 ) ) ;
#89963=ORIENTED_EDGE ( 'NONE', *, *, #69067, .T. ) ;
#89965=ORIENTED_EDGE ( 'NONE', *, *, #6915, .F. ) ;
#89966=CARTESIAN_POINT ( 'NONE',  ( 159.5402296058379932, 258.6146098258784605, 17.42708900733146393 ) ) ;
#89969=CARTESIAN_POINT ( 'NONE',  ( 86.94711308317737064, 232.5530062829863027, -4.648177544792955347E-16 ) ) ;
#89970=DIRECTION ( 'NONE',  ( -0.8660254037844387076, -0.4999999999999998890, -0.000000000000000000 ) ) ;
#89973=B_SPLINE_CURVE_WITH_KNOTS ( 'NONE', 3,
 ( #66867, #20795, #51687, #13196 ),
 .UNSPECIFIED., .F., .F.,
 ( 4, 4 ),
 ( 2.510712456960930795E-15, 0.0006326563949759604621 ),
 .UNSPECIFIED. ) ;
#89975=CARTESIAN_POINT ( 'NONE',  ( 165.3647683453818900, 265.5104300138660278, -16.61231484167872807 ) ) ;
#89981=ADVANCED_FACE ( 'NONE', ( #58582 ), #44354, .F. ) ;
#89982=CARTESIAN_POINT ( 'NONE',  ( 166.1657757771597232, 246.5300435090155702, 3.345633037118004971 ) ) ;
#89983=CARTESIAN_POINT ( 'NONE',  ( 199.9670970817828959, 270.1972007199732388, 9.297565887923761707 ) ) ;
#89986=CARTESIAN_POINT ( 'NONE',  ( 202.8499463704053198, 279.3005819042728604, 17.04674939340617001 ) ) ;
#89988=DIRECTION ( 'NONE',  ( -0.8660254037844359321, -0.5000000000000051070, -0.000000000000000000 ) ) ;
#89989=CARTESIAN_POINT ( 'NONE',  ( 161.2692160765192000, 281.6605574864539676, -6.284999054169885468 ) ) ;
#89992=CARTESIAN_POINT ( 'NONE',  ( 192.8204393314547929, 292.0303437406023477, -14.99545193480984295 ) ) ;
#89993=CARTESIAN_POINT ( 'NONE',  ( 168.2231244631735763, 252.8766363897699136, 11.96496842206752298 ) ) ;
#89996=CARTESIAN_POINT ( 'NONE',  ( 194.3387753395540472, 294.0423625616157892, -15.64827765940100868 ) ) ;
#89999=CARTESIAN_POINT ( 'NONE',  ( 161.0848266318867843, 275.9577594623067398, 12.81057407668478909 ) ) ;
#90000=EDGE_CURVE ( 'NONE', #51127, #77284, #14957, .T. ) ;
#90001=CARTESIAN_POINT ( 'NONE',  ( 196.2350291401047571, 264.4780031501763347, 5.359379669934941859 ) ) ;
#90002=CARTESIAN_POINT ( 'NONE',  ( 164.1105936565050740, 246.3991090570794427, -8.431210343695774156 ) ) ;
#90004=CARTESIAN_POINT ( 'NONE',  ( 164.4864175853093400, 274.3409801786992830, 14.76212816031865316 ) ) ;
#90007=DIRECTION ( 'NONE',  ( 0.4999999999999998890, -0.8660254037844385966, 0.000000000000000000 ) ) ;
#90015=CARTESIAN_POINT ( 'NONE',  ( 175.6288174815807395, 290.9689912212052718, 2.671585321903346966 ) ) ;
#90017=DIRECTION ( 'NONE',  ( 0.4999999999999992784, -0.8660254037844390407, 0.000000000000000000 ) ) ;
#90020=CARTESIAN_POINT ( 'NONE',  ( 15.00651571324267763, 167.2202760586659736, -5.415160957724236172E-17 ) ) ;
#90021=CARTESIAN_POINT ( 'NONE',  ( 103.7194723697636221, 236.8149278399160949, -9.188101187500095079 ) ) ;
#90022=CARTESIAN_POINT ( 'NONE',  ( 43.46773267070898328, 189.2365022471901739, -10.00000000000009237 ) ) ;
#90023=CARTESIAN_POINT ( 'NONE',  ( 180.2025839467132187, 255.6036467507360896, -2.364551107801861729 ) ) ;
#90025=CYLINDRICAL_SURFACE ( 'NONE', #3787, 10.00000000000010658 ) ;
#90027=CARTESIAN_POINT ( 'NONE',  ( 180.4684049967686121, 272.9861046151806931, 17.22288380119585938 ) ) ;
#90028=CARTESIAN_POINT ( 'NONE',  ( 194.2900850603946310, 294.1266965989547657, -15.88613936555681505 ) ) ;
#90029=EDGE_CURVE ( 'NONE', #31705, #23235, #74218, .T. ) ;
#90031=CARTESIAN_POINT ( 'NONE',  ( 196.5203034526607553, 266.3675359752309078, 8.294030003277784502 ) ) ;
#90033=CARTESIAN_POINT ( 'NONE',  ( 55.88622395072203375, 214.6199935810940929, 2.679491924311251605 ) ) ;
#90034=CARTESIAN_POINT ( 'NONE',  ( 163.4341025207368716, 282.8476932499685859, 9.116081536633066307 ) ) ;
#90036=CARTESIAN_POINT ( 'NONE',  ( 172.7618964688483914, 263.9129700666785538, -15.45032261957535091 ) ) ;
#90037=CARTESIAN_POINT ( 'NONE',  ( 78.06346978264959091, 222.0024278399160949, -9.188101187500093303 ) ) ;
#90038=CARTESIAN_POINT ( 'NONE',  ( 161.8750289368003621, 250.2712207352165592, -13.97436367953006098 ) ) ;
#90039=CARTESIAN_POINT ( 'NONE',  ( 166.7187202459675746, 278.5591580196478958, -14.78021074750266273 ) ) ;
#90042=CARTESIAN_POINT ( 'NONE',  ( 196.2048238403250764, 290.8102717488927169, 17.53926796892840656 ) ) ;
#90043=CARTESIAN_POINT ( 'NONE',  ( 199.8309894386080714, 284.5295686960079706, 18.38040563926018933 ) ) ;
#90048=CARTESIAN_POINT ( 'NONE',  ( 147.5749398328735822, 275.0397016159798227, -4.620786157167191099 ) ) ;
#90049=FACE_OUTER_BOUND ( 'NONE', #91450, .T. ) ;
#90054=CARTESIAN_POINT ( 'NONE',  ( 146.7944005049231180, 276.3916353892955726, -4.243051111306586520 ) ) ;
#90055=CARTESIAN_POINT ( 'NONE',  ( 63.38631695775107033, 200.7365022471902023, 10.00000000000009948 ) ) ;
#90057=EDGE_CURVE ( 'NONE', #65702, #1543, #45720, .T. ) ;
#90058=VERTEX_POINT ( 'NONE', #64039 ) ;
#90062=LINE ( 'NONE', #98136, #65496 ) ;
#90064=CARTESIAN_POINT ( 'NONE',  ( 131.7301550730730071, 246.8615022471902591, -10.00000000000009592 ) ) ;
#90065=CARTESIAN_POINT ( 'NONE',  ( 157.1539462478114615, 258.4483758192793061, -17.96006278656275867 ) ) ;
#90067=CARTESIAN_POINT ( 'NONE',  ( 191.1702014251404762, 299.1495971912260075, -6.870741027620923091 ) ) ;
#90071=ORIENTED_EDGE ( 'NONE', *, *, #97462, .F. ) ;
#90074=CARTESIAN_POINT ( 'NONE',  ( 152.3360070569975449, 270.2436951681156643, -14.78697292633622951 ) ) ;
#90075=CARTESIAN_POINT ( 'NONE',  ( 158.8212741314356151, 255.5604792119658839, 16.06181463215755656 ) ) ;
#90078=CARTESIAN_POINT ( 'NONE',  ( 201.2949053258274148, 281.9939920013367782, -18.04004790210578335 ) ) ;
#90081=AXIS2_PLACEMENT_3D ( 'NONE', #91105, #59651, #99178 ) ;
#90083=CARTESIAN_POINT ( 'NONE',  ( 168.0256816748547521, 276.6459939533307306, 15.18346966318006963 ) ) ;
#90088=CARTESIAN_POINT ( 'NONE',  ( 175.1271263694729328, 272.4273639404348728, 17.81557788710851042 ) ) ;
#90089=CARTESIAN_POINT ( 'NONE',  ( 174.2275517580468716, 256.7939704606039300, -12.33692674397253519 ) ) ;
#90090=CARTESIAN_POINT ( 'NONE',  ( 147.8163551302855296, 274.6215580551378821, -9.286329195885331345 ) ) ;
#90094=CARTESIAN_POINT ( 'NONE',  ( 189.8533352240220893, 301.8113727360248504, -0.2033756396389863053 ) ) ;
#90095=CARTESIAN_POINT ( 'NONE',  ( 167.9989611498101283, 286.3222843798857866, -4.708603968260846706 ) ) ;
#90098=CARTESIAN_POINT ( 'NONE',  ( 99.66015183740654493, 228.3458772461660544, 9.188101187500095079 ) ) ;
#90101=CARTESIAN_POINT ( 'NONE',  ( 163.8835510476618254, 277.4261113242017132, -14.47671527678674330 ) ) ;
#90106=CARTESIAN_POINT ( 'NONE',  ( 195.9713281756800427, 291.2146981034049418, 17.52210387885178022 ) ) ;
#90108=CARTESIAN_POINT ( 'NONE',  ( 207.1185389259403564, 270.6189067899559291, -3.459716224787868111 ) ) ;
#90110=ORIENTED_EDGE ( 'NONE', *, *, #52910, .F. ) ;
#90111=CARTESIAN_POINT ( 'NONE',  ( 163.4178923001155681, 247.5989030008181260, -10.38047187240561442 ) ) ;
#90113=EDGE_CURVE ( 'NONE', #64789, #63141, #1758, .T. ) ;
#90114=CARTESIAN_POINT ( 'NONE',  ( 194.6831946052555224, 266.4359861671931640, -8.033020006878627939 ) ) ;
#90117=CARTESIAN_POINT ( 'NONE',  ( 140.8778087205959650, 242.9548013555409796, -4.594050593750042211 ) ) ;
#90121=VECTOR ( 'NONE', #50649, 1000.000000000000000 ) ;
#90122=CARTESIAN_POINT ( 'NONE',  ( 190.1858949294064871, 301.2353624297489887, -5.249932979468886707 ) ) ;
#90125=CARTESIAN_POINT ( 'NONE',  ( 170.0299321831109580, 248.8356535510476704, -0.2657980000988006131 ) ) ;
#90126=CARTESIAN_POINT ( 'NONE',  ( 171.2966090128296059, 286.2859491661027960, 10.55860849112605848 ) ) ;
#90131=B_SPLINE_CURVE_WITH_KNOTS ( 'NONE', 3,
 ( #99381, #53259, #60838, #15238 ),
 .UNSPECIFIED., .F., .F.,
 ( 4, 4 ),
 ( 0.01398566235667206108, 0.02029681779994522983 ),
 .UNSPECIFIED. ) ;
#90132=CARTESIAN_POINT ( 'NONE',  ( 198.7898295845099881, 282.4313312432652197, -17.48232341387986111 ) ) ;
#90133=CARTESIAN_POINT ( 'NONE',  ( 141.9600801517287607, 252.7677522451418497, 10.00000000000009592 ) ) ;
#90136=CARTESIAN_POINT ( 'NONE',  ( 64.74832919946385346, 214.3149278399160949, -9.188101187500095079 ) ) ;
#90138=CARTESIAN_POINT ( 'NONE',  ( 197.6456421031980994, 287.3858497455466932, 17.15283754821559015 ) ) ;
#90139=CARTESIAN_POINT ( 'NONE',  ( 178.3664302925846812, 292.5873534235060447, -5.659256624530483393 ) ) ;
#90140=CARTESIAN_POINT ( 'NONE',  ( 197.2363158218765307, 288.6427788515542261, -16.66249965469193839 ) ) ;
#90143=AXIS2_PLACEMENT_3D ( 'NONE', #47693, #95377, #48726 ) ;
#90151=( BOUNDED_CURVE ( )  B_SPLINE_CURVE ( 2, ( #54677, #37980, #68891, #99818, #15182, #16202, #39472, #61294, #92257 ),
 .UNSPECIFIED., .F., .T. ) 
 B_SPLINE_CURVE_WITH_KNOTS ( ( 3, 2, 2, 2, 3 ),
 ( 0.5846774193548387455, 0.5860215053763441206, 0.5887096774193548709, 0.5913978494623656212, 0.5927419354838709964 ),
 .UNSPECIFIED. ) 
 CURVE ( )  GEOMETRIC_REPRESENTATION_ITEM ( )  RATIONAL_B_SPLINE_CURVE ( ( 0.9330127018922194093, 0.9330127018922194093, 1.000000000000000000, 0.8660254037844387076, 1.000000000000000000, 0.8660254037844387076, 1.000000000000000000, 0.9330127018922194093, 0.9330127018922194093 ) ) 
 REPRESENTATION_ITEM ( '' )  );
#90152=EDGE_CURVE ( 'NONE', #23266, #46780, #84544, .T. ) ;
#90153=CARTESIAN_POINT ( 'NONE',  ( 9.836819166815537585, 185.6744531367911293, 4.594050593750047540 ) ) ;
#90154=CARTESIAN_POINT ( 'NONE',  ( 49.89075441544358824, 189.6115022471902023, -5.000000000000041744 ) ) ;
#90155=ORIENTED_EDGE ( 'NONE', *, *, #32793, .T. ) ;
#90156=ADVANCED_FACE ( 'NONE', ( #90381 ), #98593, .F. ) ;
#90157=CARTESIAN_POINT ( 'NONE',  ( 181.4044655424706036, 257.2299798609144545, -8.137251057251219777 ) ) ;
#90158=B_SPLINE_CURVE_WITH_KNOTS ( 'NONE', 3,
 ( #92725, #77509, #24294, #63784, #85129, #54164, #15678, #47083, #93734, #78003, #8595, #31381 ),
 .UNSPECIFIED., .F., .F.,
 ( 4, 2, 2, 2, 2, 4 ),
 ( 7.936458345170772500E-15, 0.0004846319482286064900, 0.0009692638964492765116, 0.001453895844669946371, 0.001696211818780285745, 0.001938527792890625120 ),
 .UNSPECIFIED. ) ;
#90159=CARTESIAN_POINT ( 'NONE',  ( 199.4805356068138167, 277.5836055926158110, 15.20881834789949494 ) ) ;
#90160=EDGE_CURVE ( 'NONE', #441, #87238, #95952, .T. ) ;
#90163=CARTESIAN_POINT ( 'NONE',  ( 41.74435586355720318, 207.1589784336661637, -6.496448406907676862E-16 ) ) ;
#90164=CARTESIAN_POINT ( 'NONE',  ( 200.7583183585857967, 282.9233878912788214, 16.96937806979494212 ) ) ;
#90165=CARTESIAN_POINT ( 'NONE',  ( 151.3999564459286375, 268.4145785023736153, -15.40574304386609050 ) ) ;
#90166=CARTESIAN_POINT ( 'NONE',  ( 146.7845206192450007, 276.4087478532630939, 4.443586170796542945 ) ) ;
#90168=CARTESIAN_POINT ( 'NONE',  ( 159.8005360292372075, 255.6865549803747797, -16.53985196810166869 ) ) ;
#90169=CARTESIAN_POINT ( 'NONE',  ( 178.0910872001942664, 292.7183277186941268, 2.601818848788350458 ) ) ;
#90171=CARTESIAN_POINT ( 'NONE',  ( 176.2039003160224411, 274.8852082280174614, 16.86700035928189934 ) ) ;
#90174=CARTESIAN_POINT ( 'NONE',  ( 93.04999876614748189, 212.9824982072973683, 3.021315404115420679E-15 ) ) ;
#90175=CARTESIAN_POINT ( 'NONE',  ( 158.2603635358720453, 279.8418491720760812, 9.156985719881870267 ) ) ;
#90176=CARTESIAN_POINT ( 'NONE',  ( 98.74902094561561228, 234.4865022471902876, 10.00000000000009237 ) ) ;
#90178=CARTESIAN_POINT ( 'NONE',  ( 194.7418280156398396, 285.5977080998097790, -17.49241544463354714 ) ) ;
#90180=CARTESIAN_POINT ( 'NONE',  ( 50.02589733512838421, 205.8149278399161233, 9.188101187500093303 ) ) ;
#90182=CARTESIAN_POINT ( 'NONE',  ( 166.5911685708541086, 264.6661525622017734, 17.39495636922530863 ) ) ;
#90183=CARTESIAN_POINT ( 'NONE',  ( 162.8756881843043516, 250.5380280774768949, 12.81046238701583029 ) ) ;
#90187=CARTESIAN_POINT ( 'NONE',  ( 165.0509870607838252, 244.7702999017660375, -2.356357909806504392 ) ) ;
#90190=CARTESIAN_POINT ( 'NONE',  ( 189.7638670438123540, 264.4198756543991635, 11.07887947409659368 ) ) ;
#90193=CARTESIAN_POINT ( 'NONE',  ( 204.3341445623842674, 276.7298752272635625, 14.23430099947301031 ) ) ;
#90195=AXIS2_PLACEMENT_3D ( 'NONE', #87996, #80888, #18544 ) ;
#90198=CARTESIAN_POINT ( 'NONE',  ( 175.0308087517243507, 255.0036995273806610, 7.960308888445424280 ) ) ;
#90199=CARTESIAN_POINT ( 'NONE',  ( 5.270092192305421364, 185.3967562850347122, -4.648177544792955347E-16 ) ) ;
#90201=CYLINDRICAL_SURFACE ( 'NONE', #51408, 17.82106496071139645 ) ;
#90202=CARTESIAN_POINT ( 'NONE',  ( 167.4230310137581910, 261.5705748858933930, 17.03473681314420674 ) ) ;
#90203=CARTESIAN_POINT ( 'NONE',  ( 206.8775514429320026, 272.3245652858344670, -9.838455694836268250 ) ) ;
#90207=CARTESIAN_POINT ( 'NONE',  ( 161.6127771116929921, 250.7254542206800352, -12.96229604595372464 ) ) ;
#90208=CARTESIAN_POINT ( 'NONE',  ( 53.05609693179983566, 212.9860189848785410, -2.679491924311252493 ) ) ;
#90209=CARTESIAN_POINT ( 'NONE',  ( 148.9504735598738137, 272.6572073132907690, -11.88406006066344744 ) ) ;
#90211=CARTESIAN_POINT ( 'NONE',  ( 159.9770824720811220, 253.5585604421560788, -16.42166711341322483 ) ) ;
#90212=CARTESIAN_POINT ( 'NONE',  ( 159.6610344727618269, 254.1059716346071866, 15.33388637456589620 ) ) ;
#90214=CARTESIAN_POINT ( 'NONE',  ( 180.7318441963247437, 294.8020894299626775, 5.305383234495177902 ) ) ;
#90217=CARTESIAN_POINT ( 'NONE',  ( 123.0967907794404113, 248.0024278399161517, 9.188101187500095079 ) ) ;
#90218=FACE_OUTER_BOUND ( 'NONE', #76619, .T. ) ;
#90219=B_SPLINE_CURVE_WITH_KNOTS ( 'NONE', 3,
 ( #17071, #1890, #47473, #78397 ),
 .UNSPECIFIED., .F., .F.,
 ( 4, 4 ),
 ( 0.002837985946942163905, 0.008232558240303692806 ),
 .UNSPECIFIED. ) ;
#90221=B_SPLINE_CURVE_WITH_KNOTS ( 'NONE', 3,
 ( #71735, #49409, #80356, #79362 ),
 .UNSPECIFIED., .F., .F.,
 ( 4, 4 ),
 ( 0.04736994433111862968, 0.04887120950165270428 ),
 .UNSPECIFIED. ) ;
#90222=CARTESIAN_POINT ( 'NONE',  ( 170.4462059903102045, 263.7743965880969768, 15.83889961394278245 ) ) ;
#90223=CARTESIAN_POINT ( 'NONE',  ( 203.6925490392534925, 269.5270927311577793, 7.084861529579629114 ) ) ;
#90226=CARTESIAN_POINT ( 'NONE',  ( 160.1860556839894230, 253.6250155762421059, 14.83728034098512616 ) ) ;
#90227=ORIENTED_EDGE ( 'NONE', *, *, #81325, .T. ) ;
#90229=CARTESIAN_POINT ( 'NONE',  ( 198.5612432604688991, 286.7288335892616260, 18.30793681285053509 ) ) ;
#90231=CARTESIAN_POINT ( 'NONE',  ( 84.04489159724214176, 210.1423013555409796, -4.594050593750043987 ) ) ;
#90235=CARTESIAN_POINT ( 'NONE',  ( 174.8748641034385969, 278.1051818648194853, 15.47627503780401703 ) ) ;
#90239=CARTESIAN_POINT ( 'NONE',  ( 201.3505934466285510, 281.8975373467312693, -16.83770227898004279 ) ) ;
#90243=CARTESIAN_POINT ( 'NONE',  ( 163.9684994123220179, 260.5718777511302164, -16.18805203446126129 ) ) ;
#90244=CARTESIAN_POINT ( 'NONE',  ( 175.0387250457744983, 253.3993311541219953, -7.863511161993287146 ) ) ;
#90245=EDGE_CURVE ( 'NONE', #96457, #48389, #13346, .T. ) ;
#90247=CARTESIAN_POINT ( 'NONE',  ( 206.3505875407052486, 273.2372935382459787, 11.62318091048137880 ) ) ;
#90248=CARTESIAN_POINT ( 'NONE',  ( 47.74604483422196921, 186.8262482093457777, 3.021315404115420679E-15 ) ) ;
#90250=CARTESIAN_POINT ( 'NONE',  ( 5.561079055679667427, 174.0177522451418781, -10.00000000000009592 ) ) ;
#90251=CARTESIAN_POINT ( 'NONE',  ( 132.6230702210692414, 253.5024278399160949, -9.188101187500093303 ) ) ;
#90253=CARTESIAN_POINT ( 'NONE',  ( -6.040052912301486998, 173.9865022471903160, -10.00000000000009592 ) ) ;
#90254=CARTESIAN_POINT ( 'NONE',  ( 182.5422306857729495, 258.3868535584214214, 6.448336885657590223 ) ) ;
#90255=CARTESIAN_POINT ( 'NONE',  ( 155.8781371459173215, 261.8896788882548208, -16.97225651315609696 ) ) ;
#90257=B_SPLINE_CURVE_WITH_KNOTS ( 'NONE', 3,
 ( #100080, #68655, #99577, #61043 ),
 .UNSPECIFIED., .F., .F.,
 ( 4, 4 ),
 ( 0.007478447391378081031, 0.01563385345884502065 ),
 .UNSPECIFIED. ) ;
#90258=CARTESIAN_POINT ( 'NONE',  ( 163.8670932201372352, 246.8208641845333773, 5.912697114930636211 ) ) ;
#90261=CARTESIAN_POINT ( 'NONE',  ( 178.7600897929267774, 254.1784503161647706, 4.743017227330367014 ) ) ;
#90262=VERTEX_POINT ( 'NONE', #53796 ) ;
#90264=CARTESIAN_POINT ( 'NONE',  ( -13.51183432020139819, 142.4280072687214442, 0.000000000000000000 ) ) ;
#90266=CARTESIAN_POINT ( 'NONE',  ( 202.5213466331059351, 267.6576707457072644, 0.8617883848194879404 ) ) ;
#90267=CARTESIAN_POINT ( 'NONE',  ( 197.2988255893771736, 265.5460696373069709, 0.8212393553507734145 ) ) ;
#90268=CARTESIAN_POINT ( 'NONE',  ( 190.1607982559816890, 301.2788311432216233, -4.972636536415983244 ) ) ;
#90269=CARTESIAN_POINT ( 'NONE',  ( 182.8932037339787939, 280.6271841624986791, 16.75229298683104417 ) ) ;
#90272=CARTESIAN_POINT ( 'NONE',  ( 204.6235849755581455, 276.2285497258825444, -13.59355699282649432 ) ) ;
#90273=CARTESIAN_POINT ( 'NONE',  ( 192.8438934858417895, 268.2918492126220258, 12.53398668708618402 ) ) ;
#90274=B_SPLINE_SURFACE_WITH_KNOTS ( 'NONE', 3, 1, ( 
 ( #54510, #93572 ),
 ( #16037, #46938 ),
 ( #77855, #70229 ),
 ( #834, #24141 ),
 ( #7290, #30600 ),
 ( #1590, #71487 ),
 ( #2082, #38171 ),
 ( #94309, #69589 ),
 ( #100015, #79108 ),
 ( #14886, #25363 ),
 ( #6304, #32472 ),
 ( #44784, #61486 ),
 ( #84341, #75720 ),
 ( #92436, #17263 ),
 ( #14409, #76225 ),
 ( #7800, #45775 ),
 ( #46270, #30100 ),
 ( #13903, #45291 ),
 ( #15372, #48167 ),
 ( #63864, #38685 ),
 ( #37195, #60982 ),
 ( #56254, #32959 ),
 ( #69089, #91947 ),
 ( #9691, #94803 ),
 ( #22498, #22983 ),
 ( #40553, #68593 ),
 ( #53389, #77193 ),
 ( #99019, #68097 ),
 ( #24861, #29605 ),
 ( #60478, #91436 ),
 ( #63369, #21997 ),
 ( #52892, #83844 ),
 ( #55736, #53872 ),
 ( #76697, #84834 ) ),
 .UNSPECIFIED., .T., .F., .F.,
 ( 4, 2, 2, 2, 2, 2, 2, 2, 2, 2, 2, 2, 2, 2, 2, 2, 4 ),
 ( 2, 2 ),
 ( 0.000000000000000000, 0.06250000000000000000, 0.1250000000000000000, 0.1875000000000000000, 0.2500000000000000000, 0.3125000000000000000, 0.3750000000000000000, 0.4375000000000000000, 0.5000000000000000000, 0.5625000000000000000, 0.6250000000000000000, 0.6875000000000000000, 0.7500000000000000000, 0.8125000000000000000, 0.8750000000000000000, 0.9375000000000000000, 1.000000000000000000 ),
 ( 0.000000000000000000, 1.000000000000000000 ),
 .UNSPECIFIED. ) ;
#90276=CARTESIAN_POINT ( 'NONE',  ( 149.0802055316563326, 272.4325049467973940, 12.84384348890831085 ) ) ;
#90279=CARTESIAN_POINT ( 'NONE',  ( 159.2077906806335932, 254.8910129107889588, 16.14624949541834553 ) ) ;
#90280=CARTESIAN_POINT ( 'NONE',  ( 207.2031141856176930, 271.7606740744515719, 5.319265574913023542 ) ) ;
#90283=CARTESIAN_POINT ( 'NONE',  ( 126.3716228836088362, 253.7677522451419065, -5.000000000000047962 ) ) ;
#90284=CARTESIAN_POINT ( 'NONE',  ( 182.1760933249994139, 278.4465760882033578, 17.66821597207981398 ) ) ;
#90285=VERTEX_POINT ( 'NONE', #85787 ) ;
#90288=CARTESIAN_POINT ( 'NONE',  ( 150.7691137448031213, 269.5072301123068428, -15.63821625702598084 ) ) ;
#90289=CARTESIAN_POINT ( 'NONE',  ( 18.33521408509785644, 172.2048013555409796, 4.594050593750051981 ) ) ;
#90290=CARTESIAN_POINT ( 'NONE',  ( 178.6505746094053961, 259.2109398937957963, -10.36763312313177110 ) ) ;
#90294=CARTESIAN_POINT ( 'NONE',  ( 205.3708847852691406, 274.9341884869767227, -13.70973585089674174 ) ) ;
#90297=CARTESIAN_POINT ( 'NONE',  ( 167.5258221105458745, 256.6147765433380528, 14.95940915016304551 ) ) ;
#90298=ADVANCED_FACE ( 'NONE', ( #16318 ), #1127, .T. ) ;
#90300=CARTESIAN_POINT ( 'NONE',  ( 150.9462701294987141, 269.2003862531290110, 13.98983978186602073 ) ) ;
#90301=CARTESIAN_POINT ( 'NONE',  ( 51.11762373747147592, 206.9865022471902876, -10.00000000000009415 ) ) ;
#90302=CARTESIAN_POINT ( 'NONE',  ( 185.0483992081186670, 294.1025820707552043, 9.705500343873069369 ) ) ;
#90304=CARTESIAN_POINT ( 'NONE',  ( 147.8465295590381743, 274.5692944114487091, 9.322947948439978205 ) ) ;
#90305=CARTESIAN_POINT ( 'NONE',  ( 26.56245542105003210, 176.9548013555409796, -4.594050593750042211 ) ) ;
#90307=CARTESIAN_POINT ( 'NONE',  ( 192.2943420783192323, 297.5834248427583475, 12.53393473147773562 ) ) ;
#90310=CARTESIAN_POINT ( 'NONE',  ( 181.8200170576783705, 278.0724415165672099, 16.45581006755550746 ) ) ;
#90311=CARTESIAN_POINT ( 'NONE',  ( 185.5878794376151575, 266.6731272799339649, 13.19771459954216652 ) ) ;
#90313=CARTESIAN_POINT ( 'NONE',  ( 163.4142949803911620, 281.2077642141172760, 8.863657438064944216 ) ) ;
#90316=CARTESIAN_POINT ( 'NONE',  ( 189.4199209167946663, 300.3895034224956930, 3.306026617473488027 ) ) ;
#90318=CARTESIAN_POINT ( 'NONE',  ( 189.2845499996045930, 259.5340837477176024, -0.8149847707460528001 ) ) ;
#90319=CARTESIAN_POINT ( 'NONE',  ( 155.5204415533959548, 261.2776889444089647, 17.19127227448963424 ) ) ;
#90320=ORIENTED_EDGE ( 'NONE', *, *, #2, .F. ) ;
#90321=CARTESIAN_POINT ( 'NONE',  ( 181.5350816980370325, 289.2740427057465809, 12.64428308550723479 ) ) ;
#90322=CARTESIAN_POINT ( 'NONE',  ( 108.3474691708931630, 233.3615022471902591, -10.00000000000009592 ) ) ;
#90324=ORIENTED_EDGE ( 'NONE', *, *, #71424, .T. ) ;
#90325=CARTESIAN_POINT ( 'NONE',  ( 196.0896742213610082, 290.2260983427040060, -16.35227306082677146 ) ) ;
#90328=CARTESIAN_POINT ( 'NONE',  ( 203.4682009197399566, 278.2297336128146412, -15.36039508894693206 ) ) ;
#90332=CARTESIAN_POINT ( 'NONE',  ( 164.4936379324916516, 245.7356569095223051, 6.719479797016231437 ) ) ;
#90333=CARTESIAN_POINT ( 'NONE',  ( 192.8132846206021611, 296.6845899933152850, 11.53748932578252351 ) ) ;
#90335=CARTESIAN_POINT ( 'NONE',  ( 190.8001679306945277, 300.1714103817999444, 7.815449226872675403 ) ) ;
#90338=CARTESIAN_POINT ( 'NONE',  ( 174.5060864132779557, 262.3161859066883039, 14.40012180740343872 ) ) ;
#90341=AXIS2_PLACEMENT_3D ( 'NONE', #24925, #72044, #93364 ) ;
#90342=ORIENTED_EDGE ( 'NONE', *, *, #34513, .F. ) ;
#90343=CARTESIAN_POINT ( 'NONE',  ( 164.9617201910520237, 244.9249146555742414, 2.745022583679548767 ) ) ;
#90346=VERTEX_POINT ( 'NONE', #56811 ) ;
#90348=CARTESIAN_POINT ( 'NONE',  ( 172.3812282607925397, 263.7635464947321111, -15.48109893273863236 ) ) ;
#90350=CARTESIAN_POINT ( 'NONE',  ( 83.32840393668934098, 230.4637435831425023, 2.679491924311251605 ) ) ;
#90351=CARTESIAN_POINT ( 'NONE',  ( 147.1034852426517148, 275.8562849197056153, -3.648177088342072327 ) ) ;
#90353=EDGE_LOOP ( 'NONE', ( #23567, #65849, #7911, #65654 ) ) ;
#90357=CARTESIAN_POINT ( 'NONE',  ( 188.6257896815903621, 298.5631806337704006, -4.505592037249916970 ) ) ;
#90359=CARTESIAN_POINT ( 'NONE',  ( 153.4619471835925708, 264.8431057800031567, 16.95044998314351758 ) ) ;
#90360=CARTESIAN_POINT ( 'NONE',  ( 191.8308278875103099, 298.3862549712684995, 9.280152759256424133 ) ) ;
#90361=CARTESIAN_POINT ( 'NONE',  ( 147.2999496562918296, 275.5159985734018164, -0.1418322875769767455 ) ) ;
#90362=B_SPLINE_CURVE_WITH_KNOTS ( 'NONE', 3,
 ( #32629, #17427, #1750, #723 ),
 .UNSPECIFIED., .F., .F.,
 ( 4, 4 ),
 ( 0.003952496786374898145, 0.009435233971604372813 ),
 .UNSPECIFIED. ) ;
#90366=CARTESIAN_POINT ( 'NONE',  ( 148.9504735598738137, 272.6572073132907690, -11.88406006066344744 ) ) ;
#90367=CARTESIAN_POINT ( 'NONE',  ( 206.5508451493652444, 272.8904371854448527, 11.05407534521577695 ) ) ;
#90370=CARTESIAN_POINT ( 'NONE',  ( 169.0014201196099748, 286.7460675995289989, 4.080809884116825437 ) ) ;
#90371=B_SPLINE_CURVE_WITH_KNOTS ( 'NONE', 3,
 ( #1034, #92760, #62305, #8136 ),
 .UNSPECIFIED., .F., .F.,
 ( 4, 4 ),
 ( 0.009425792323206581835, 0.01476071270588196274 ),
 .UNSPECIFIED. ) ;
#90372=CARTESIAN_POINT ( 'NONE',  ( 176.5750811079351763, 290.0661888821730372, -9.631901365267058424 ) ) ;
#90374=CARTESIAN_POINT ( 'NONE',  ( 149.3583220794619422, 271.9507929555723535, -11.49772206859406332 ) ) ;
#90376=CARTESIAN_POINT ( 'NONE',  ( 202.9752796556865064, 278.6631792541300001, 14.99201349560580532 ) ) ;
#90379=CARTESIAN_POINT ( 'NONE',  ( 198.7177703306137460, 286.4577207510109247, -18.34263739182689790 ) ) ;
#90380=EDGE_CURVE ( 'NONE', #53811, #45557, #94896, .T. ) ;
#90381=FACE_OUTER_BOUND ( 'NONE', #42110, .T. ) ;
#90382=ORIENTED_EDGE ( 'NONE', *, *, #97710, .F. ) ;
#90383=CARTESIAN_POINT ( 'NONE',  ( 170.3022864262811140, 255.3823714536916327, -11.62275972992479645 ) ) ;
#90387=CARTESIAN_POINT ( 'NONE',  ( 207.6727254509676186, 270.9472835030587703, 7.315149605389819953 ) ) ;
#90388=EDGE_CURVE ( 'NONE', #65702, #39606, #66902, .T. ) ;
#90389=CARTESIAN_POINT ( 'NONE',  ( 36.66582480827081980, 178.6427522451417644, 1.119607411625061291E-15 ) ) ;
#90390=CARTESIAN_POINT ( 'NONE',  ( 113.7873647845227083, 230.3768266524159856, -9.188101187500093303 ) ) ;
#90391=CARTESIAN_POINT ( 'NONE',  ( 151.1699610800269511, 268.8129421616204695, -14.28929860221299286 ) ) ;
#90392=CARTESIAN_POINT ( 'NONE',  ( 167.9211909854000169, 281.9652706170933243, -10.87640062917275507 ) ) ;
#90393=CARTESIAN_POINT ( 'NONE',  ( 190.7405042774493324, 298.2747508605859821, 9.591131971744578877 ) ) ;
#90395=CARTESIAN_POINT ( 'NONE',  ( 35.05980905203730913, 200.2369531367911293, -4.594050593750048428 ) ) ;
#90399=DIRECTION ( 'NONE',  ( 0.4999999999999992784, -0.8660254037844390407, 0.000000000000000000 ) ) ;
#90400=CARTESIAN_POINT ( 'NONE',  ( 181.3415465419150792, 267.7713915340963240, 14.97876564237039254 ) ) ;
#90404=CARTESIAN_POINT ( 'NONE',  ( 179.4042561553460757, 287.8475187006056331, -12.55830537432352401 ) ) ;
#90405=CARTESIAN_POINT ( 'NONE',  ( 164.2365267202495431, 249.9047677799958365, 11.29870037847212672 ) ) ;
#90406=CARTESIAN_POINT ( 'NONE',  ( 95.19470834736904408, 235.7677522451419065, -5.000000000000047962 ) ) ;
#90409=B_SPLINE_CURVE_WITH_KNOTS ( 'NONE', 3,
 ( #13379, #44248, #7753, #45249, #75184, #52849, #83799, #14363, #91900, #76185, #22942, #6760, #68549, #53831, #69551, #5758, #36648, #83296, #156, #69045, #61931, #22455, #67554, #53350, #59943, #92883, #98487, #98977, #37638, #61443, #99474, #76657, #51873, #13860, #84791, #7245, #30050, #82811, #44739, #6258, #29561, #37155, #77150, #29078, #91391, #38127, #15332, #93897, #55820, #47245 ),
 .UNSPECIFIED., .F., .F.,
 ( 4, 2, 2, 2, 2, 2, 2, 2, 2, 2, 2, 2, 2, 2, 2, 2, 2, 2, 2, 2, 2, 2, 2, 2, 4 ),
 ( 0.0006309157225252743240, 0.0008450400362799124782, 0.001059164350034550849, 0.001166226506911871011, 0.001273288663789191172, 0.001380350820666511550, 0.001487412977543831711, 0.001701537291298473335, 0.001915661605053114959, 0.002343910232562398423, 0.003200407487580905069, 0.004056904742599411716, 0.004913401997617919230, 0.005341650625127209416, 0.005555774938881930837, 0.005662837095759329711, 0.005716368174197957591, 0.005769899252636586338, 0.005876961409513709392, 0.005984023566390833312, 0.006198147880145075950, 0.006412272193899318587, 0.006626396507653561224, 0.007054645135162053438, 0.007482893762670545651 ),
 .UNSPECIFIED. ) ;
#90410=CARTESIAN_POINT ( 'NONE',  ( 194.9180876943665055, 266.4584948954776564, -7.740551621638591229 ) ) ;
#90412=CARTESIAN_POINT ( 'NONE',  ( 155.5784045870823036, 279.7726721642641792, -1.593457801340965929 ) ) ;
#90414=B_SPLINE_CURVE_WITH_KNOTS ( 'NONE', 3,
 ( #65966, #87848, #50265, #35059, #81218, #18388, #88337, #97390, #12281, #42649, #18894, #10786, #49773, #74085, #4674, #97881, #66465, #42162, #73098, #74595, #27958, #51250, #66952, #82218, #12790, #3208, #36049, #34093, #95926, #80729, #11794, #11304, #3690, #73581, #34569, #4163, #65470, #45633, #84691, #69447, #76561, #7649, #7142, #38029, #67454, #84206, #30450, #14752 ),
 .UNSPECIFIED., .F., .F.,
 ( 4, 2, 2, 2, 2, 2, 2, 2, 2, 2, 2, 2, 2, 2, 2, 2, 2, 2, 2, 2, 2, 2, 2, 4 ),
 ( 0.0001582601720098061036, 0.0006504983501745226302, 0.001142736528339238994, 0.001388855617421661144, 0.001634974706504083077, 0.001758034251045258265, 0.001881093795586433453, 0.002004153340127608641, 0.002127212884668783829, 0.002373331973751017978, 0.002619451062833252561, 0.003111689240997658843, 0.004096165597326570720, 0.005080641953655483031, 0.005572880131819939187, 0.005818999220902246194, 0.006065118309984554069, 0.006126648082255130821, 0.006188177854525706706, 0.006311237399066868016, 0.006557356488149255688, 0.007049594666314037104, 0.007541832844478820255, 0.008034071022643600804 ),
 .UNSPECIFIED. ) ;
#90416=CARTESIAN_POINT ( 'NONE',  ( 22.31343150979137846, 177.5643266524160424, 9.188101187500095079 ) ) ;
#90422=CARTESIAN_POINT ( 'NONE',  ( 57.11665387649598813, 203.7833772461660828, -9.188101187500095079 ) ) ;
#90423=CARTESIAN_POINT ( 'NONE',  ( 198.7134558283731280, 282.8386145195935910, 17.66748989068429054 ) ) ;
#90427=ORIENTED_EDGE ( 'NONE', *, *, #40222, .T. ) ;
#90429=CARTESIAN_POINT ( 'NONE',  ( 12.29081813446910409, 191.2365022471903444, 2.944929066748280225E-16 ) ) ;
#90431=CARTESIAN_POINT ( 'NONE',  ( 140.4172988551291610, 258.0024278399160949, -9.188101187500093303 ) ) ;
#90433=CARTESIAN_POINT ( 'NONE',  ( 207.5610651195029845, 271.1406848703456944, -7.832979109022246256 ) ) ;
#90434=LINE ( 'NONE', #44758, #17719 ) ;
#90438=CARTESIAN_POINT ( 'NONE',  ( 171.7154418923348942, 259.3365693118849435, -15.26938553599716641 ) ) ;
#90439=VERTEX_POINT ( 'NONE', #97831 ) ;
#90440=CARTESIAN_POINT ( 'NONE',  ( 191.5544531425776427, 298.8649500714207647, 8.366689293739112188 ) ) ;
#90443=CARTESIAN_POINT ( 'NONE',  ( 151.3638679738639610, 268.9271637915409769, -14.29068541092436462 ) ) ;
#90444=CARTESIAN_POINT ( 'NONE',  ( 170.0766860910346168, 266.2494559554864395, -17.52215767842801242 ) ) ;
#90445=DIRECTION ( 'NONE',  ( -0.8660254037844387076, -0.4999999999999998890, -0.000000000000000000 ) ) ;
#90447=ORIENTED_EDGE ( 'NONE', *, *, #92662, .T. ) ;
#90449=CARTESIAN_POINT ( 'NONE',  ( 168.4165475187242862, 282.2027335547327311, -10.92266496736840686 ) ) ;
#90452=DIRECTION ( 'NONE',  ( -0.8660254037844387076, -0.4999999999999998890, -0.000000000000000000 ) ) ;
#90453=DIRECTION ( 'NONE',  ( -0.8660254037844387076, -0.4999999999999998890, -0.000000000000000000 ) ) ;
#90455=CARTESIAN_POINT ( 'NONE',  ( 150.8074912838825128, 278.0825890836262602, -0.0002049239830752711748 ) ) ;
#90459=CARTESIAN_POINT ( 'NONE',  ( 147.7840666256145425, 276.6774833857293174, 0.9737628777943441172 ) ) ;
#90461=CARTESIAN_POINT ( 'NONE',  ( 163.3838389430857774, 253.5546336541830783, 14.73126852126472386 ) ) ;
#90462=ADVANCED_FACE ( 'NONE', ( #51724 ), #82667, .T. ) ;
#90464=CARTESIAN_POINT ( 'NONE',  ( 159.1138359885003126, 263.7651727890922757, -17.14152579247067720 ) ) ;
#90465=VERTEX_POINT ( 'NONE', #1744 ) ;
#90466=CARTESIAN_POINT ( 'NONE',  ( 147.2405539530007559, 275.6188749492528132, 0.4306668706573002492 ) ) ;
#90467=CARTESIAN_POINT ( 'NONE',  ( 204.6823371430232896, 272.9704135290961062, -9.754921121218281144 ) ) ;
#90468=CARTESIAN_POINT ( 'NONE',  ( 163.7010375032499212, 247.1084811230698506, 6.649922295230481950 ) ) ;
#90471=CARTESIAN_POINT ( 'NONE',  ( 94.00418374076319594, 215.8923013555410080, 4.594050593750050204 ) ) ;
#90472=CARTESIAN_POINT ( 'NONE',  ( 169.5608527833963421, 251.6396950762901952, -9.960993533446050208 ) ) ;
#90474=CARTESIAN_POINT ( 'NONE',  ( 181.3013930180519253, 271.1797949997417732, -15.98288922033975012 ) ) ;
#90475=CARTESIAN_POINT ( 'NONE',  ( 181.9690984642188312, 257.1582083484186114, -6.131635832278763409 ) ) ;
#90478=CARTESIAN_POINT ( 'NONE',  ( -8.728340106763567974, 165.7677522451418781, 10.00000000000009592 ) ) ;
#90483=ORIENTED_EDGE ( 'NONE', *, *, #57233, .T. ) ;
#90487=CARTESIAN_POINT ( 'NONE',  ( 153.0790963368640689, 265.5062228982576471, -17.74594954892339160 ) ) ;
#90488=FACE_OUTER_BOUND ( 'NONE', #89730, .T. ) ;
#90491=CARTESIAN_POINT ( 'NONE',  ( 168.3064590912703693, 267.1730826594816790, -17.42781320323403804 ) ) ;
#90492=ORIENTED_EDGE ( 'NONE', *, *, #46060, .F. ) ;
#90496=VERTEX_POINT ( 'NONE', #39195 ) ;
#90498=CARTESIAN_POINT ( 'NONE',  ( 199.9393105959312891, 270.2060721569587258, 10.05715988195613164 ) ) ;
#90499=VERTEX_POINT ( 'NONE', #40709 ) ;
#90500=CARTESIAN_POINT ( 'NONE',  ( 163.2437751800324293, 247.9004826992694461, 9.806027032984305336 ) ) ;
#90501=CARTESIAN_POINT ( 'NONE',  ( 188.6938424665491141, 259.9925076287862566, 2.228382896047578665 ) ) ;
#90502=CARTESIAN_POINT ( 'NONE',  ( 149.4444163961335050, 276.2143034153455687, -5.416261063417526778 ) ) ;
#90504=CARTESIAN_POINT ( 'NONE',  ( 192.7288556637334125, 292.1918731402626577, -15.52061534916644447 ) ) ;
#90505=CARTESIAN_POINT ( 'NONE',  ( 170.0343890063719527, 248.3992706227272151, -0.1813713061637557133 ) ) ;
#90506=CARTESIAN_POINT ( 'NONE',  ( 195.1681749095326097, 291.9751310054545570, 15.48020786373133184 ) ) ;
#90508=VERTEX_POINT ( 'NONE', #9850 ) ;
#90509=CARTESIAN_POINT ( 'NONE',  ( 181.5560669682341484, 271.2834731898979044, -15.97545557697810104 ) ) ;
#90511=ORIENTED_EDGE ( 'NONE', *, *, #86527, .T. ) ;
#90512=CARTESIAN_POINT ( 'NONE',  ( 160.5756158696236469, 275.8270879902572688, 12.72679581559236617 ) ) ;
#90514=CARTESIAN_POINT ( 'NONE',  ( 174.3820402454518614, 281.0329706854971619, -14.18843254014566924 ) ) ;
#90515=CARTESIAN_POINT ( 'NONE',  ( 204.2406320560561142, 276.8918436393669822, -14.88456622902110915 ) ) ;
#90516=CARTESIAN_POINT ( 'NONE',  ( 174.4665098196985298, 288.5002641398569949, -10.08633113632384237 ) ) ;
#90517=CARTESIAN_POINT ( 'NONE',  ( 164.8411062115066841, 274.0701676799238840, 15.65099743181538194 ) ) ;
#90518=CARTESIAN_POINT ( 'NONE',  ( -15.79203335248894469, 167.8149278399160949, -9.188101187500095079 ) ) ;
#90520=CARTESIAN_POINT ( 'NONE',  ( 185.1996946330573621, 295.7366452146979441, 8.572466393607147239 ) ) ;
#90521=ORIENTED_EDGE ( 'NONE', *, *, #47274, .F. ) ;
#90522=B_SPLINE_SURFACE_WITH_KNOTS ( 'NONE', 3, 1, ( 
 ( #48186, #24881 ),
 ( #9190, #2100 ),
 ( #10697, #32495 ),
 ( #48700, #41576 ),
 ( #17282, #86244 ),
 ( #9712, #32980 ),
 ( #72517, #54774 ),
 ( #79634, #41064 ),
 ( #25908, #78098 ),
 ( #2606, #56780 ),
 ( #87763, #3126 ),
 ( #78604, #85753 ),
 ( #40065, #16282 ),
 ( #47176, #24389 ),
 ( #93835, #55262 ),
 ( #16781, #47672 ),
 ( #3604, #88747 ),
 ( #74509, #66870 ),
 ( #34972, #73497 ),
 ( #34483, #95842 ),
 ( #97803, #11703 ),
 ( #89731, #82640 ),
 ( #35968, #81137 ),
 ( #66382, #4080 ),
 ( #74997, #27393 ),
 ( #28372, #19320 ),
 ( #36468, #65874 ),
 ( #59250, #35478 ),
 ( #90229, #5576 ),
 ( #26397, #51169 ),
 ( #20798, #89252 ),
 ( #42080, #5088 ),
 ( #51691, #96830 ),
 ( #44057, #65382 ) ),
 .UNSPECIFIED., .T., .F., .F.,
 ( 4, 2, 2, 2, 2, 2, 2, 2, 2, 2, 2, 2, 2, 2, 2, 2, 4 ),
 ( 2, 2 ),
 ( 0.000000000000000000, 0.06250000000000000000, 0.1250000000000000000, 0.1875000000000000000, 0.2500000000000000000, 0.3125000000000000000, 0.3750000000000000000, 0.4375000000000000000, 0.5000000000000000000, 0.5625000000000000000, 0.6250000000000000000, 0.6875000000000000000, 0.7500000000000000000, 0.8125000000000000000, 0.8750000000000000000, 0.9375000000000000000, 1.000000000000000000 ),
 ( 0.000000000000000000, 1.000000000000000000 ),
 .UNSPECIFIED. ) ;
#90530=CARTESIAN_POINT ( 'NONE',  ( 150.0802157573592126, 276.6422289437092559, 3.399058894176778534 ) ) ;
#90531=CARTESIAN_POINT ( 'NONE',  ( 2.719259653403429233, 178.5024278399160949, -9.188101187500093303 ) ) ;
#90532=CARTESIAN_POINT ( 'NONE',  ( 121.7437996339097310, 241.0958772461660544, -9.188101187500095079 ) ) ;
#90534=CARTESIAN_POINT ( 'NONE',  ( 180.8614647981713119, 256.2301897900337053, -2.334466546830306299 ) ) ;
#90536=CARTESIAN_POINT ( 'NONE',  ( 198.4160757083882345, 267.1808215963346242, -8.346050686629251203 ) ) ;
#90537=CARTESIAN_POINT ( 'NONE',  ( 190.6585475213478560, 299.9177820201669533, -4.437337276038273437 ) ) ;
#90540=CARTESIAN_POINT ( 'NONE',  ( 183.8673499631198354, 275.0308414889168489, 16.36260528999715902 ) ) ;
#90541=CARTESIAN_POINT ( 'NONE',  ( 148.3629184514745987, 273.6748826132846375, -8.219814532462343948 ) ) ;
#90544=CARTESIAN_POINT ( 'NONE',  ( 196.0328332463135155, 266.6894456190431697, 8.014243085850971227 ) ) ;
#90545=DIRECTION ( 'NONE',  ( -0.8660254037844387076, -0.4999999999999998890, -0.000000000000000000 ) ) ;
#90546=CARTESIAN_POINT ( 'NONE',  ( 162.5729406961995096, 251.2985046087954402, -12.76312550842038718 ) ) ;
#90548=CARTESIAN_POINT ( 'NONE',  ( 172.9828220029686747, 262.8000787801868228, -16.17504394412311086 ) ) ;
#90549=CARTESIAN_POINT ( 'NONE',  ( 97.38683515247240052, 227.0333772461660544, 9.188101187500095079 ) ) ;
#90551=DIRECTION ( 'NONE',  ( 0.8660254037844395958, 0.4999999999999985567, 0.000000000000000000 ) ) ;
#90554=CARTESIAN_POINT ( 'NONE',  ( 195.9713281756800427, 291.2146981034049418, 17.52210387885178022 ) ) ;
#90556=CARTESIAN_POINT ( 'NONE',  ( 149.0651262117185354, 272.4586230950732784, 12.81403047969042319 ) ) ;
#90557=CARTESIAN_POINT ( 'NONE',  ( 205.2706556652093752, 273.1077904153184477, -10.97544480913108167 ) ) ;
#90558=CARTESIAN_POINT ( 'NONE',  ( 160.9155581428462085, 282.2930683307629920, -7.657675304491033508 ) ) ;
#90561=CARTESIAN_POINT ( 'NONE',  ( 146.7842303614460207, 276.4092505945183689, -4.491116827832889236 ) ) ;
#90563=ORIENTED_EDGE ( 'NONE', *, *, #65419, .T. ) ;
#90566=CARTESIAN_POINT ( 'NONE',  ( 172.4678624035182679, 290.8891845726454903, -0.5858198065817201705 ) ) ;
#90567=CARTESIAN_POINT ( 'NONE',  ( 197.3327212804159103, 267.5970440452412049, 9.861675131224707513 ) ) ;
#90568=CARTESIAN_POINT ( 'NONE',  ( 187.9710278913847219, 285.9884846539495129, -16.45153272977178460 ) ) ;
#90571=CARTESIAN_POINT ( 'NONE',  ( 198.6562788533279615, 286.5642271139020636, 17.47134757795404525 ) ) ;
#90572=CARTESIAN_POINT ( 'NONE',  ( 157.4753914210714356, 268.7471219652609875, 15.64991620571603015 ) ) ;
#90574=LINE ( 'NONE', #36808, #17795 ) ;
#90575=AXIS2_PLACEMENT_3D ( 'NONE', #5566, #60732, #14169 ) ;
#90576=CARTESIAN_POINT ( 'NONE',  ( 134.3282312844263231, 248.3615022471902591, -10.00000000000009592 ) ) ;
#90577=CARTESIAN_POINT ( 'NONE',  ( 157.0877926458200307, 258.5629572190321710, -17.40668770468195703 ) ) ;
#90578=ORIENTED_EDGE ( 'NONE', *, *, #64431, .F. ) ;
#90580=B_SPLINE_SURFACE_WITH_KNOTS ( 'NONE', 3, 1, ( 
 ( #34328, #73341 ),
 ( #3928, #18643 ),
 ( #57613, #34811 ),
 ( #49523, #73832 ),
 ( #97166, #58601 ),
 ( #4421, #65712 ),
 ( #96168, #96667 ),
 ( #35317, #43410 ),
 ( #41924, #72358 ),
 ( #27235, #25745 ),
 ( #95690, #19651 ),
 ( #51011, #26237 ),
 ( #57112, #20139 ),
 ( #74357, #58120 ),
 ( #56625, #12039 ),
 ( #88592, #88094 ),
 ( #80476, #11046 ),
 ( #89101, #65225 ),
 ( #50513, #72860 ),
 ( #81962, #35821 ),
 ( #87608, #90577 ),
 ( #59091, #13537 ),
 ( #70066, #39153 ),
 ( #100005, #90065 ),
 ( #66716, #92912 ),
 ( #98139, #684 ),
 ( #15362, #53860 ),
 ( #85854, #44407 ),
 ( #77181, #46258 ),
 ( #69579, #69078 ),
 ( #7787, #23974 ),
 ( #46784, #31566 ),
 ( #31069, #93423 ),
 ( #74848, #28724 ) ),
 .UNSPECIFIED., .T., .F., .F.,
 ( 4, 2, 2, 2, 2, 2, 2, 2, 2, 2, 2, 2, 2, 2, 2, 2, 4 ),
 ( 2, 2 ),
 ( 0.000000000000000000, 0.06250000000000000000, 0.1250000000000000000, 0.1875000000000000000, 0.2500000000000000000, 0.3125000000000000000, 0.3750000000000000000, 0.4375000000000000000, 0.5000000000000000000, 0.5625000000000000000, 0.6250000000000000000, 0.6875000000000000000, 0.7500000000000000000, 0.8125000000000000000, 0.8750000000000000000, 0.9375000000000000000, 1.000000000000000000 ),
 ( 0.000000000000000000, 1.000000000000000000 ),
 .UNSPECIFIED. ) ;
#90582=CARTESIAN_POINT ( 'NONE',  ( 155.5311623832600958, 261.6886619413561448, 17.00987194985870943 ) ) ;
#90586=CARTESIAN_POINT ( 'NONE',  ( 181.9559929377375056, 291.6402902057536721, -11.43735378946719372 ) ) ;
#90590=CARTESIAN_POINT ( 'NONE',  ( 191.4302501518540396, 279.3169626480661805, -16.56989974033457358 ) ) ;
#90591=CARTESIAN_POINT ( 'NONE',  ( 192.9772420103627724, 296.4006074639731310, -13.54979510632026063 ) ) ;
#90592=CARTESIAN_POINT ( 'NONE',  ( 201.4214977800931763, 281.7747274386935601, -17.04225209925078133 ) ) ;
#90599=VERTEX_POINT ( 'NONE', #25013 ) ;
#90600=CARTESIAN_POINT ( 'NONE',  ( 182.5579995116864325, 296.7134427671203980, 0.3470945606806519201 ) ) ;
#90603=CARTESIAN_POINT ( 'NONE',  ( 181.3346534254663140, 271.3440730695800767, -17.45372068697093226 ) ) ;
#90605=CARTESIAN_POINT ( 'NONE',  ( 147.6947327179224487, 274.8322142526899370, 9.090449717876689206 ) ) ;
#90606=CARTESIAN_POINT ( 'NONE',  ( 167.2132997600114379, 286.2193399160603349, -4.798080686485812762 ) ) ;
#90608=CARTESIAN_POINT ( 'NONE',  ( 181.4694507228112457, 256.9988949691801281, 4.992663963241201763 ) ) ;
#90609=CARTESIAN_POINT ( 'NONE',  ( 104.5854977735480560, 237.3149278399160664, 9.188101187500093303 ) ) ;
#90611=CARTESIAN_POINT ( 'NONE',  ( 148.2404373810095706, 275.8870260502966403, -5.709515531134017330 ) ) ;
#90612=B_SPLINE_CURVE_WITH_KNOTS ( 'NONE', 3,
 ( #82414, #90992, #28150, #12979, #36238, #74288, #50945, #29646, #99064, #43840, #21553, #59525 ),
 .UNSPECIFIED., .F., .F.,
 ( 4, 2, 2, 2, 2, 4 ),
 ( 0.001199298977550974313, 0.001655502193913219351, 0.001883603802094317801, 0.002111705410275416250, 0.002567908626637613149, 0.003024111842999810049 ),
 .UNSPECIFIED. ) ;
#90613=CARTESIAN_POINT ( 'NONE',  ( 188.2363250879724887, 273.5010258966393621, 15.66123827714173089 ) ) ;
#90614=VERTEX_POINT ( 'NONE', #40200 ) ;
#90615=ORIENTED_EDGE ( 'NONE', *, *, #8680, .T. ) ;
#90618=EDGE_CURVE ( 'NONE', #65984, #3452, #48841, .T. ) ;
#90619=CARTESIAN_POINT ( 'NONE',  ( 180.6668490247078864, 294.2638964725952633, -2.198001587704702331 ) ) ;
#90620=CARTESIAN_POINT ( 'NONE',  ( 196.4994169513186364, 290.3000215130921902, 16.82935102260526961 ) ) ;
#90621=CARTESIAN_POINT ( 'NONE',  ( 206.6703863510205679, 272.6833857505801006, -10.72500664779635393 ) ) ;
#90622=CARTESIAN_POINT ( 'NONE',  ( 192.0969986600162827, 271.0201763999182845, -15.22553433325905736 ) ) ;
#90629=CARTESIAN_POINT ( 'NONE',  ( 192.6230444026213036, 263.8685375577596233, -8.332581229518458699 ) ) ;
#90630=CARTESIAN_POINT ( 'NONE',  ( 185.7952724173880483, 257.5178294002433290, 0.9274047933272019373 ) ) ;
#90632=CARTESIAN_POINT ( 'NONE',  ( 187.4684169401624843, 291.1055366833039670, -13.65599679362259167 ) ) ;
#90634=CARTESIAN_POINT ( 'NONE',  ( 153.0927037754837556, 265.4826541232073964, -16.15085267704102634 ) ) ;
#90635=ORIENTED_EDGE ( 'NONE', *, *, #31635, .F. ) ;
#90636=B_SPLINE_CURVE_WITH_KNOTS ( 'NONE', 3,
 ( #41915, #28079, #40893, #74212 ),
 .UNSPECIFIED., .F., .F.,
 ( 4, 4 ),
 ( 0.0008273161503298089633, 0.008754319486608567666 ),
 .UNSPECIFIED. ) ;
#90637=CARTESIAN_POINT ( 'NONE',  ( 190.2510882691990730, 301.1224442529128851, -5.480893437181090455 ) ) ;
#90638=ADVANCED_FACE ( 'NONE', ( #72144 ), #86383, .T. ) ;
#90640=CARTESIAN_POINT ( 'NONE',  ( 190.6103240053217860, 264.3150132381076673, -9.438093754014104775 ) ) ;
#90641=EDGE_CURVE ( 'NONE', #80312, #16011, #59560, .T. ) ;
#90642=CARTESIAN_POINT ( 'NONE',  ( 173.3711701851306941, 251.4955055664892427, -0.7996342223137038463 ) ) ;
#90643=CARTESIAN_POINT ( 'NONE',  ( 118.7397740163064128, 239.3615022471902307, -10.00000000000009592 ) ) ;
#90646=CARTESIAN_POINT ( 'NONE',  ( 137.1969404309142817, 260.0177522451418781, 5.000000000000046185 ) ) ;
#90650=CARTESIAN_POINT ( 'NONE',  ( 56.79189435007682363, 203.5958772461660544, -9.188101187500095079 ) ) ;
#90651=CARTESIAN_POINT ( 'NONE',  ( 159.7692415128758228, 253.9185515433934768, -16.85856106119654285 ) ) ;
#90653=CARTESIAN_POINT ( 'NONE',  ( 208.1303168694798273, 270.1547119170880364, -0.9257663487928086132 ) ) ;
#90655=B_SPLINE_CURVE_WITH_KNOTS ( 'NONE', 3,
 ( #94018, #7890, #39251, #24570, #55455, #34067, #64958, #26461, #84421, #76778, #7371, #69170, #18865, #57834, #42626, #96387, #57337, #97858, #19862, #74569, #66443, #67427, #51751, #11763, #28429, #49747, #43115, #58332, #81684, #89308, #59311, #5633, #75056, #4139, #74059, #26951, #90290, #82693, #43630, #98358, #4648, #27462, #88311, #80700, #35034, #65442, #58818, #88815, #65938, #96892 ),
 .UNSPECIFIED., .F., .F.,
 ( 4, 2, 2, 2, 2, 2, 2, 2, 2, 2, 2, 2, 2, 2, 2, 2, 2, 2, 2, 2, 2, 2, 2, 2, 4 ),
 ( 0.0002689362054544326024, 0.0007455428061392906005, 0.001222149406824148653, 0.001460452707166577570, 0.001579604357337793114, 0.001698756007509008657, 0.001817907657680224200, 0.001937059307851439743, 0.002175362608193776286, 0.002651969208878449807, 0.003128575809563122461, 0.004081789010932469937, 0.005035002212301816979, 0.005511608812986444964, 0.005749912113328714720, 0.005869063763499849165, 0.005988215413670983610, 0.006047791238756500959, 0.006107367063842016573, 0.006226518714013051271, 0.006464822014355107657, 0.006941428615039225633, 0.007418035215723343609, 0.007656338516065450302, 0.007894641816407556995 ),
 .UNSPECIFIED. ) ;
#90657=CARTESIAN_POINT ( 'NONE',  ( 161.8668411317136986, 250.2854024296290447, -13.43522912998426655 ) ) ;
#90658=CARTESIAN_POINT ( 'NONE',  ( 189.6738045434663320, 300.1223289962524063, 4.832295392723879424 ) ) ;
#90659=CARTESIAN_POINT ( 'NONE',  ( 185.9562832929018157, 265.4319297318980375, 13.85577190340941378 ) ) ;
#90662=B_SPLINE_CURVE_WITH_KNOTS ( 'NONE', 3,
 ( #21262, #29359, #14153, #60225 ),
 .UNSPECIFIED., .F., .F.,
 ( 4, 4 ),
 ( 0.03672685766160826981, 0.04538173523955296024 ),
 .UNSPECIFIED. ) ;
#90663=CARTESIAN_POINT ( 'NONE',  ( 149.8532179585512267, 272.8608575990943450, -11.50785342781380116 ) ) ;
#90666=CARTESIAN_POINT ( 'NONE',  ( 32.70573635520464251, 183.5643266524160140, 9.188101187500095079 ) ) ;
#90667=CARTESIAN_POINT ( 'NONE',  ( 157.6673516573649181, 257.5591315650518141, 16.79781451397666103 ) ) ;
#90671=CARTESIAN_POINT ( 'NONE',  ( 55.76366273096530080, 196.8768266524160140, 9.188101187500096856 ) ) ;
#90672=EDGE_CURVE ( 'NONE', #83319, #28762, #98436, .T. ) ;
#90674=CARTESIAN_POINT ( 'NONE',  ( 151.4428545556028780, 268.3402767968688067, -15.03309903163500749 ) ) ;
#90675=CARTESIAN_POINT ( 'NONE',  ( 149.5796913320911870, 271.5673701627850960, -12.80793412251569841 ) ) ;
#90677=CARTESIAN_POINT ( 'NONE',  ( 198.1847055346428590, 286.9842163890704683, 16.95145238430053070 ) ) ;
#90679=CARTESIAN_POINT ( 'NONE',  ( 179.6504827179812480, 276.7753844222579573, 16.30384834125107218 ) ) ;
#90682=CARTESIAN_POINT ( 'NONE',  ( 163.6073896235010636, 255.4122057569755952, -14.91336208084822168 ) ) ;
#90684=DIRECTION ( 'NONE',  ( 0.4999999999999992784, -0.8660254037844390407, 0.000000000000000000 ) ) ;
#90685=CARTESIAN_POINT ( 'NONE',  ( 105.8215617431885818, 225.2365022471902023, -10.00000000000009059 ) ) ;
#90686=FACE_OUTER_BOUND ( 'NONE', #51898, .T. ) ;
#90687=CARTESIAN_POINT ( 'NONE',  ( 170.3290958195750022, 289.6815776661216546, -1.151831906498994140 ) ) ;
#90688=ORIENTED_EDGE ( 'NONE', *, *, #41807, .T. ) ;
#90689=CARTESIAN_POINT ( 'NONE',  ( 52.89478003304684250, 201.3458772461660260, 9.188101187500095079 ) ) ;
#90691=CARTESIAN_POINT ( 'NONE',  ( 166.4514803149947966, 264.9061636045831847, 16.72458767844168648 ) ) ;
#90692=CARTESIAN_POINT ( 'NONE',  ( 147.3023124603499809, 275.5119060767245287, 5.196938859334171212 ) ) ;
#90693=ADVANCED_FACE ( 'NONE', ( #77745 ), #18424, .F. ) ;
#90694=VECTOR ( 'NONE', #43839, 1000.000000000000000 ) ;
#90695=CARTESIAN_POINT ( 'NONE',  ( 171.9208136763257926, 265.2263239767592040, 17.32491798815716422 ) ) ;
#90696=ORIENTED_EDGE ( 'NONE', *, *, #52909, .T. ) ;
#90697=DIRECTION ( 'NONE',  ( -0.8660254037844359321, -0.5000000000000051070, -0.000000000000000000 ) ) ;
#90698=CARTESIAN_POINT ( 'NONE',  ( 207.6826438088389750, 270.9301044032979462, 7.252082088659585146 ) ) ;
#90702=CARTESIAN_POINT ( 'NONE',  ( 157.3880781592554285, 258.0428474529849723, 18.15852591502753555 ) ) ;
#90703=VERTEX_POINT ( 'NONE', #96467 ) ;
#90708=EDGE_CURVE ( 'NONE', #35, #59274, #67007, .T. ) ;
#90711=CARTESIAN_POINT ( 'NONE',  ( 167.9276914116459523, 262.1860323319936015, 16.09630263804044148 ) ) ;
#90712=ADVANCED_FACE ( 'NONE', ( #87896 ), #95297, .F. ) ;
#90713=CARTESIAN_POINT ( 'NONE',  ( 159.2102594322688844, 254.8867369075254885, -16.13039487917589199 ) ) ;
#90717=CYLINDRICAL_SURFACE ( 'NONE', #21645, 10.00000000000010658 ) ;
#90720=CARTESIAN_POINT ( 'NONE',  ( 159.9880386575927957, 253.5395837721924863, 15.85893018594752846 ) ) ;
#90722=CARTESIAN_POINT ( 'NONE',  ( 164.5959123184142356, 265.0909081389784205, -16.62699299347688253 ) ) ;
#90723=CARTESIAN_POINT ( 'NONE',  ( 131.9199452241419124, 234.7202760586659736, -5.415160957724236172E-17 ) ) ;
#90724=CYLINDRICAL_SURFACE ( 'NONE', #66680, 17.82106496071139645 ) ;
#90726=CARTESIAN_POINT ( 'NONE',  ( 170.1494630792247449, 264.1798617481715610, 16.79485409072000834 ) ) ;
#90727=CARTESIAN_POINT ( 'NONE',  ( -22.42236680055709641, 157.8615022471902591, 0.000000000000000000 ) ) ;
#90729=CARTESIAN_POINT ( 'NONE',  ( 160.4401160996124815, 253.2479743581097580, 14.60890098605380949 ) ) ;
#90730=EDGE_LOOP ( 'NONE', ( #71238, #73345, #61509, #66380 ) ) ;
#90731=ORIENTED_EDGE ( 'NONE', *, *, #30205, .F. ) ;
#90733=CARTESIAN_POINT ( 'NONE',  ( 87.90566119885008334, 214.8927522451418497, 10.00000000000009948 ) ) ;
#90734=CARTESIAN_POINT ( 'NONE',  ( 194.7442550381435638, 291.6868277426822260, -16.06123382811687605 ) ) ;
#90735=CARTESIAN_POINT ( 'NONE',  ( -4.903394573382326094, 174.6427522451419350, -10.00000000000009592 ) ) ;
#90736=CARTESIAN_POINT ( 'NONE',  ( 25.38399186717684231, 173.9155109091896350, 2.679491924311254714 ) ) ;
#90738=CARTESIAN_POINT ( 'NONE',  ( 194.0672051292551430, 294.5127359636757660, 15.53337744471869364 ) ) ;
#90741=ADVANCED_FACE ( 'NONE', ( #92837 ), #49144, .F. ) ;
#90742=CARTESIAN_POINT ( 'NONE',  ( 114.6081111488702220, 243.6427522451419065, -10.00000000000009592 ) ) ;
#90743=CARTESIAN_POINT ( 'NONE',  ( 200.7484899876179441, 282.9404111291507888, -16.88964748465601673 ) ) ;
#90750=EDGE_CURVE ( 'NONE', #46359, #64907, #39792, .T. ) ;
#90751=CARTESIAN_POINT ( 'NONE',  ( 205.8918578537579833, 274.0318366629789466, 11.52627491423194250 ) ) ;
#90753=CARTESIAN_POINT ( 'NONE',  ( 196.2630260332681189, 290.7094625936034049, -17.43112004684450866 ) ) ;
#90754=CARTESIAN_POINT ( 'NONE',  ( 194.8811071667591364, 279.6953583877882465, 17.03940305312293901 ) ) ;
#90755=CARTESIAN_POINT ( 'NONE',  ( 207.5570596878370679, 271.1476224814971374, 2.444960520848353358 ) ) ;
#90757=CARTESIAN_POINT ( 'NONE',  ( 131.5133883985292016, 255.9244531367911293, -4.594050593750046652 ) ) ;
#90758=VERTEX_POINT ( 'NONE', #73512 ) ;
#90764=CARTESIAN_POINT ( 'NONE',  ( 178.7427661924620850, 254.2096309538193282, 4.677055477819860307 ) ) ;
#90767=( BOUNDED_CURVE ( )  B_SPLINE_CURVE ( 2, ( #56268, #17796, #87264, #3121, #31966, #18297, #64891, #80129, #71995 ),
 .UNSPECIFIED., .F., .T. ) 
 B_SPLINE_CURVE_WITH_KNOTS ( ( 3, 2, 2, 2, 3 ),
 ( 0.5927419354838709964, 0.5940860215053763715, 0.5967741935483871218, 0.5994623655913978721, 0.6008064516129032473 ),
 .UNSPECIFIED. ) 
 CURVE ( )  GEOMETRIC_REPRESENTATION_ITEM ( )  RATIONAL_B_SPLINE_CURVE ( ( 0.9330127018922194093, 0.9330127018922194093, 1.000000000000000000, 0.8660254037844387076, 1.000000000000000000, 0.8660254037844387076, 1.000000000000000000, 0.9330127018922194093, 0.9330127018922194093 ) ) 
 REPRESENTATION_ITEM ( '' )  );
#90771=CARTESIAN_POINT ( 'NONE',  ( 202.4223208072874343, 267.6828090875848147, 0.8583124146943408306 ) ) ;
#90772=CARTESIAN_POINT ( 'NONE',  ( 190.4240181651484818, 300.8229208869809668, -4.214281362166949485 ) ) ;
#90773=CARTESIAN_POINT ( 'NONE',  ( 183.0325607505932624, 280.7969938308983160, 17.10607354250000967 ) ) ;
#90774=CARTESIAN_POINT ( 'NONE',  ( 157.6500260163024620, 257.5891404556457474, -18.23450497588216379 ) ) ;
#90775=CARTESIAN_POINT ( 'NONE',  ( 192.8720113526765374, 268.2812397856054645, 12.55819112576203977 ) ) ;
#90778=CARTESIAN_POINT ( 'NONE',  ( 71.35865581505748878, 223.5530062829863027, -4.648177544792955347E-16 ) ) ;
#90780=CARTESIAN_POINT ( 'NONE',  ( 159.5284711081640125, 254.3355781173132755, 15.34104435652608522 ) ) ;
#90783=CARTESIAN_POINT ( 'NONE',  ( -0.5819415548772214342, 158.2202760586659736, -5.415160957724236172E-17 ) ) ;
#90784=CARTESIAN_POINT ( 'NONE',  ( 175.1877765885950851, 284.8709350377350233, -12.04777258482997659 ) ) ;
#90785=EDGE_LOOP ( 'NONE', ( #13776, #82404, #19605, #19778 ) ) ;
#90788=CARTESIAN_POINT ( 'NONE',  ( 150.6626254231123880, 269.6916732958875969, -15.32062296289003811 ) ) ;
#90789=CARTESIAN_POINT ( 'NONE',  ( -0.8802452050168975139, 179.4869531367911293, 4.594050593750046652 ) ) ;
#90790=CARTESIAN_POINT ( 'NONE',  ( 181.5896340430631710, 275.4731096103383265, -16.43232654997619235 ) ) ;
#90793=CARTESIAN_POINT ( 'NONE',  ( 157.5487431480040925, 257.7645675294749594, -18.29554785922338311 ) ) ;
#90795=CARTESIAN_POINT ( 'NONE',  ( 149.8677590727400855, 277.0051387818008948, 4.638989373348268330 ) ) ;
#90797=CARTESIAN_POINT ( 'NONE',  ( 73.97708595465037718, 203.5177522451417929, 5.000000000000051514 ) ) ;
#90799=CARTESIAN_POINT ( 'NONE',  ( 198.3791677596651368, 287.0441976074670833, 16.95474403075850134 ) ) ;
#90800=CARTESIAN_POINT ( 'NONE',  ( 65.47921168356349142, 198.6115022471902023, -5.000000000000041744 ) ) ;
#90803=CARTESIAN_POINT ( 'NONE',  ( 12.11013585174968554, 186.9869531367911293, 4.594050593750046652 ) ) ;
#90804=CARTESIAN_POINT ( 'NONE',  ( 168.0810693606937605, 286.6467868267807830, 4.970377858261654680 ) ) ;
#90805=CARTESIAN_POINT ( 'NONE',  ( 13.97105408662886461, 167.3262482093458061, -5.229199737892075682E-14 ) ) ;
#90807=CARTESIAN_POINT ( 'NONE',  ( 172.3741624485570867, 252.4865239976215037, 8.880853820034850798 ) ) ;
#90808=EDGE_CURVE ( 'NONE', #19784, #99484, #1529, .T. ) ;
#90809=CARTESIAN_POINT ( 'NONE',  ( 165.0437781805843258, 244.7827860485373606, -2.050141714668513693 ) ) ;
#90810=CARTESIAN_POINT ( 'NONE',  ( 185.2207215791545707, 266.7315570652577321, 13.46751314241562447 ) ) ;
#90812=CARTESIAN_POINT ( 'NONE',  ( 163.0000163990417548, 280.9966438126449475, 8.877784272329016346 ) ) ;
#90815=CARTESIAN_POINT ( 'NONE',  ( 165.0258157087664870, 286.3787970787498125, -0.1841640296008903166 ) ) ;
#90818=DIRECTION ( 'NONE',  ( -0.8660254037844387076, -0.4999999999999998890, -0.000000000000000000 ) ) ;
#90821=CARTESIAN_POINT ( 'NONE',  ( 173.4877205307014378, 258.6818873298753374, 14.30620870653597976 ) ) ;
#90824=EDGE_LOOP ( 'NONE', ( #59040, #81033, #40341, #61523 ) ) ;
#90825=CARTESIAN_POINT ( 'NONE',  ( 195.3624787578944222, 290.3824063481519602, -16.76522224015156226 ) ) ;
#90826=CARTESIAN_POINT ( 'NONE',  ( 80.63465624979117763, 207.3615022471901739, 5.000000000000051514 ) ) ;
#90827=B_SPLINE_CURVE_WITH_KNOTS ( 'NONE', 3,
 ( #7909, #38784, #62073, #2316, #73213, #63592, #24587, #94533, #26605, #40772 ),
 .UNSPECIFIED., .F., .F.,
 ( 4, 2, 2, 2, 4 ),
 ( 0.001461773093899133673, 0.001796020748610993242, 0.002130268403322852812, 0.002464516058034712381, 0.002798763712746571951 ),
 .UNSPECIFIED. ) ;
#90830=CARTESIAN_POINT ( 'NONE',  ( 203.3349860717029571, 278.4604684979374838, -16.59553970625579566 ) ) ;
#90831=ORIENTED_EDGE ( 'NONE', *, *, #91408, .T. ) ;
#90833=CARTESIAN_POINT ( 'NONE',  ( 187.3286608096677526, 272.3913705820498308, -16.85577171651204154 ) ) ;
#90834=CARTESIAN_POINT ( 'NONE',  ( 164.2297246530060875, 246.1927681183832988, 5.803160395959773510 ) ) ;
#90835=CARTESIAN_POINT ( 'NONE',  ( 192.0712386031329686, 297.9698513971258649, 12.12276320360788873 ) ) ;
#90837=CARTESIAN_POINT ( 'NONE',  ( 190.8264243556038195, 300.1259329198319961, 8.466983560044813117 ) ) ;
#90843=CARTESIAN_POINT ( 'NONE',  ( 196.9728329903666122, 289.4800408803428695, -17.53478045286815856 ) ) ;
#90845=ORIENTED_EDGE ( 'NONE', *, *, #71455, .T. ) ;
#90846=CARTESIAN_POINT ( 'NONE',  ( 206.0691053506789387, 273.7248349927971844, 11.70564474658248422 ) ) ;
#90849=CARTESIAN_POINT ( 'NONE',  ( 174.4171900096681327, 277.1582007793262505, -15.66121359032516658 ) ) ;
#90850=CARTESIAN_POINT ( 'NONE',  ( 172.3180150275962603, 263.6756876961334797, -15.46435045179676671 ) ) ;
#90852=CARTESIAN_POINT ( 'NONE',  ( 158.9933333928889851, 275.2344634518124167, -12.53406194300261767 ) ) ;
#90857=ORIENTED_EDGE ( 'NONE', *, *, #36055, .T. ) ;
#90860=CARTESIAN_POINT ( 'NONE',  ( 190.8545714895799392, 300.0771806536980648, -5.516553996882049837 ) ) ;
#90863=CARTESIAN_POINT ( 'NONE',  ( 153.4242699508872647, 264.9083646613370320, 16.62000820703435267 ) ) ;
#90864=CARTESIAN_POINT ( 'NONE',  ( 191.8082373951299076, 298.4253828518392879, 9.404421445770532628 ) ) ;
#90865=CARTESIAN_POINT ( 'NONE',  ( 147.2229325088103735, 275.6493961858936927, -0.4918294119671829390 ) ) ;
#90866=ORIENTED_EDGE ( 'NONE', *, *, #39194, .T. ) ;
#90867=EDGE_CURVE ( 'NONE', #79855, #57805, #11231, .T. ) ;
#90870=CARTESIAN_POINT ( 'NONE',  ( 197.0313051377892748, 289.3787641501790517, -17.15509075150697882 ) ) ;
#90873=CARTESIAN_POINT ( 'NONE',  ( 167.6323876601624647, 287.4389059340153381, 3.681410875200846089 ) ) ;
#90874=CARTESIAN_POINT ( 'NONE',  ( -22.42236680055709641, 157.8615022471902591, 0.000000000000000000 ) ) ;
#90876=CARTESIAN_POINT ( 'NONE',  ( 205.0859877718122561, 268.9368413191317586, -3.038556538008958974 ) ) ;
#90877=B_SPLINE_CURVE_WITH_KNOTS ( 'NONE', 3,
 ( #84943, #800, #30211, #60590, #61093, #92064, #22613, #309, #70190, #38292, #7399, #39772, #69202, #100128, #23094, #38795, #16003, #54479, #14994, #62086, #6906, #99130, #45403, #29713, #53006, #37795, #53499, #23586, #30714, #46903, #8409, #7921, #78322, #83957, #22113, #15488, #84453, #62584, #39281, #31681, #14521, #24100, #93543, #68699, #54994, #61596 ),
 .UNSPECIFIED., .F., .F.,
 ( 4, 2, 2, 2, 2, 2, 2, 2, 2, 2, 2, 2, 2, 2, 2, 2, 2, 2, 2, 2, 2, 2, 4 ),
 ( 0.0002647527076360194857, 0.001281163540060212573, 0.001789368956272361158, 0.002043471664378435342, 0.002170523018431519055, 0.002297574372484603202, 0.002424625726537686481, 0.002551677080590770627, 0.002805779788696939787, 0.003313985204909353569, 0.004330396037334254856, 0.005346806869759156144, 0.005855012285971683550, 0.006109114994078024448, 0.006363217702184365346, 0.006426743379210956425, 0.006490269056237549239, 0.006553794733264140318, 0.006617320410290732265, 0.006871423118397062754, 0.007379628534609765367, 0.007887833950822469714, 0.008396039367035172327 ),
 .UNSPECIFIED. ) ;
#90880=CARTESIAN_POINT ( 'NONE',  ( 202.6932411237282565, 279.0175140182560085, 15.29984597618553543 ) ) ;
#90882=CARTESIAN_POINT ( 'NONE',  ( 182.6185197117589212, 284.2352000010978941, -15.00009734104487258 ) ) ;
#90885=CARTESIAN_POINT ( 'NONE',  ( 208.3682389855799499, 269.7426187237583690, -1.431169231381201890 ) ) ;
#90886=CARTESIAN_POINT ( 'NONE',  ( 192.3743613796607406, 267.3190593529452030, 12.60351243473677307 ) ) ;
#90887=CARTESIAN_POINT ( 'NONE',  ( 164.4440639631384045, 245.8215215431751233, -2.910115319305802029 ) ) ;
#90888=CARTESIAN_POINT ( 'NONE',  ( 40.63510790894943625, 194.2677522451418781, 10.00000000000009592 ) ) ;
#90889=CARTESIAN_POINT ( 'NONE',  ( 110.4040191812834735, 243.7369531367911009, -4.594050593750048428 ) ) ;
#90890=CARTESIAN_POINT ( 'NONE',  ( 180.2260403442535051, 295.0423342771414923, -3.480517403894910711 ) ) ;
#90891=CYLINDRICAL_SURFACE ( 'NONE', #99845, 17.82106496071139645 ) ;
#90892=CYLINDRICAL_SURFACE ( 'NONE', #66363, 17.82106496071139645 ) ;
#90894=CARTESIAN_POINT ( 'NONE',  ( 37.30632276492696064, 192.3458772461660544, 9.188101187500095079 ) ) ;
#90895=CARTESIAN_POINT ( 'NONE',  ( 147.6628748529174402, 275.3469524600083105, -3.428921689675848317 ) ) ;
#90896=ORIENTED_EDGE ( 'NONE', *, *, #82321, .T. ) ;
#90898=CARTESIAN_POINT ( 'NONE',  ( 181.8441098414710666, 266.9845076301842823, 15.29841396442351709 ) ) ;
#90899=CARTESIAN_POINT ( 'NONE',  ( 25.04665064082954729, 185.2677522451418497, 10.00000000000009592 ) ) ;
#90900=CARTESIAN_POINT ( 'NONE',  ( 190.1635032421960148, 301.2741459696644029, -5.047660290019184259 ) ) ;
#90902=CARTESIAN_POINT ( 'NONE',  ( -22.42236680055709641, 157.8615022471902591, 0.000000000000000000 ) ) ;
#90903=CARTESIAN_POINT ( 'NONE',  ( 179.4099431796017257, 287.9386474004925276, -12.64039063190630685 ) ) ;
#90905=CARTESIAN_POINT ( 'NONE',  ( 103.4941184669699936, 223.8927522451417929, 10.00000000000009592 ) ) ;
#90906=VERTEX_POINT ( 'NONE', #16058 ) ;
#90908=CARTESIAN_POINT ( 'NONE',  ( 198.4160757083882345, 267.1808215963346242, -8.346050686629251203 ) ) ;
#90909=B_SPLINE_CURVE_WITH_KNOTS ( 'NONE', 3,
 ( #22074, #5882, #36769, #98608, #29677, #91021, #83415, #44859, #75800, #99585, #6385, #37269, #60552, #68167, #37757, #99093 ),
 .UNSPECIFIED., .F., .F.,
 ( 4, 2, 2, 2, 2, 2, 2, 4 ),
 ( 6.664589960562511959E-17, 0.0003089471551300475966, 0.0006178943102600286232, 0.0009268414653900095956, 0.001235788620519990460, 0.001544735775649971323, 0.001853682930779952404, 0.002471577241040045538 ),
 .UNSPECIFIED. ) ;
#90910=CARTESIAN_POINT ( 'NONE',  ( 155.4994079124308257, 279.7286834434665366, -1.607709304407256123 ) ) ;
#90911=CARTESIAN_POINT ( 'NONE',  ( 207.9743173328493526, 270.4249110404894054, -2.481515874287090639 ) ) ;
#90912=CARTESIAN_POINT ( 'NONE',  ( 8.294124642383250645, 187.8464784336662206, 1.353441290958777327E-15 ) ) ;
#90917=CARTESIAN_POINT ( 'NONE',  ( 174.1338248144772649, 287.3177669875508400, 10.47848546623640686 ) ) ;
#90918=CARTESIAN_POINT ( 'NONE',  ( 49.86334402403631572, 211.8464784336661637, 1.353441290958777327E-15 ) ) ;
#90919=CARTESIAN_POINT ( 'NONE',  ( 163.9354095869165633, 246.7025367662834014, -7.289870401565430313 ) ) ;
#90920=CARTESIAN_POINT ( 'NONE',  ( 203.7265596842292439, 276.1056548365280605, 13.24074560745231466 ) ) ;
#90922=CARTESIAN_POINT ( 'NONE',  ( 165.0509870607838252, 244.7702999017660375, -2.356357909806504392 ) ) ;
#90925=CARTESIAN_POINT ( 'NONE',  ( 164.4817765375028102, 245.7562014482918755, -6.334578229142199035 ) ) ;
#90926=CARTESIAN_POINT ( 'NONE',  ( 18.71383987920379255, 171.6115022471901739, -5.000000000000041744 ) ) ;
#90927=CARTESIAN_POINT ( 'NONE',  ( 164.4963285489318991, 245.7309966251440301, -6.672251175510283794 ) ) ;
#90928=CARTESIAN_POINT ( 'NONE',  ( 147.0210896547505399, 249.5643266524160140, 9.188101187500095079 ) ) ;
#90930=CARTESIAN_POINT ( 'NONE',  ( 206.8387077773648173, 272.3918444881492746, -7.972442346115986567 ) ) ;
#90932=CARTESIAN_POINT ( 'NONE',  ( 198.8081898473356262, 282.3983615885804284, -17.60554210735202574 ) ) ;
#90936=ORIENTED_EDGE ( 'NONE', *, *, #36446, .F. ) ;
#90938=CARTESIAN_POINT ( 'NONE',  ( 164.0405267935391294, 246.5204684236636581, 7.644396071283796168 ) ) ;
#90940=CARTESIAN_POINT ( 'NONE',  ( 170.3462095380075425, 266.3929324287667555, -17.59993820609288306 ) ) ;
#90945=EDGE_CURVE ( 'NONE', #5430, #64025, #6362, .T. ) ;
#90946=CARTESIAN_POINT ( 'NONE',  ( 148.9346857181035091, 273.2112271305713307, -9.473665380863973695 ) ) ;
#90947=CARTESIAN_POINT ( 'NONE',  ( 23.40481081636943372, 190.9865022471903160, 10.00000000000009415 ) ) ;
#90948=CARTESIAN_POINT ( 'NONE',  ( 185.8885322232007979, 296.6982464125469505, 4.785400323938857170 ) ) ;
#90950=CARTESIAN_POINT ( 'NONE',  ( 149.9706620097691143, 271.4333556379564243, -12.01292532367938293 ) ) ;
#90951=CARTESIAN_POINT ( 'NONE',  ( 190.4940980602978300, 281.5357392997901798, 17.69179316189531903 ) ) ;
#90953=CARTESIAN_POINT ( 'NONE',  ( 192.0403215870056783, 287.5166130765638854, -16.83829816813398139 ) ) ;
#90955=CARTESIAN_POINT ( 'NONE',  ( 167.4011299790239775, 281.5488363183706042, 12.98604958840868662 ) ) ;
#90958=EDGE_LOOP ( 'NONE', ( #96551, #92816, #92925 ) ) ;
#90959=CARTESIAN_POINT ( 'NONE',  ( 146.9235493515124062, 276.1679430252639804, 0.7994986043261682607 ) ) ;
#90961=CARTESIAN_POINT ( 'NONE',  ( 164.2059258710715994, 246.2339888178522926, 7.329631442356459914 ) ) ;
#90962=FACE_OUTER_BOUND ( 'NONE', #46374, .T. ) ;
#90963=ORIENTED_EDGE ( 'NONE', *, *, #78226, .F. ) ;
#90964=CARTESIAN_POINT ( 'NONE',  ( 91.83912023130210400, 214.6423013555409796, -4.594050593750043987 ) ) ;
#90965=CARTESIAN_POINT ( 'NONE',  ( 198.9446342420995109, 283.0329230195785044, 17.26884992386511897 ) ) ;
#90968=ORIENTED_EDGE ( 'NONE', *, *, #46785, .T. ) ;
#90972=ORIENTED_EDGE ( 'NONE', *, *, #93523, .T. ) ;
#90973=CARTESIAN_POINT ( 'NONE',  ( 158.9054571277534649, 258.0742575434156834, 17.39430999040402526 ) ) ;
#90974=VERTEX_POINT ( 'NONE', #25674 ) ;
#90975=CARTESIAN_POINT ( 'NONE',  ( 164.5613517958998955, 245.6183730577221809, 2.459055975528789517 ) ) ;
#90980=CARTESIAN_POINT ( 'NONE',  ( 156.7370215179966237, 259.1705106342505474, -18.04600119725074947 ) ) ;
#90984=ORIENTED_EDGE ( 'NONE', *, *, #9126, .T. ) ;
#90985=CARTESIAN_POINT ( 'NONE',  ( 166.4301960487401004, 284.1355213801691093, 9.513592484950153860 ) ) ;
#90986=CARTESIAN_POINT ( 'NONE',  ( 20.18783944447021383, 170.9155109091896065, 2.679491924311254714 ) ) ;
#90988=CARTESIAN_POINT ( 'NONE',  ( 163.4260108471723640, 247.5848412648317662, 10.45113099391573108 ) ) ;
#90989=CARTESIAN_POINT ( 'NONE',  ( 185.1149126255429849, 258.5007932025994819, 2.939304387390308193 ) ) ;
#90990=CARTESIAN_POINT ( 'NONE',  ( 161.2113459091177674, 281.3599108807870834, -6.589518380948089948 ) ) ;
#90991=CARTESIAN_POINT ( 'NONE',  ( 165.8064460562817430, 246.4435469418012588, -2.717970023973333316 ) ) ;
#90992=CARTESIAN_POINT ( 'NONE',  ( 157.4718321624326620, 258.3312158842189774, 16.78309831726782164 ) ) ;
#90993=CARTESIAN_POINT ( 'NONE',  ( 172.0630936339023265, 254.4764114392720273, 11.54978638049990103 ) ) ;
#90994=CARTESIAN_POINT ( 'NONE',  ( 158.2761760943415652, 281.1697532028657065, 2.074752331550637319 ) ) ;
#90995=ORIENTED_EDGE ( 'NONE', *, *, #16899, .F. ) ;
#90998=CARTESIAN_POINT ( 'NONE',  ( 160.2308819960220490, 276.4003654746809957, 12.70007076641597088 ) ) ;
#90999=CARTESIAN_POINT ( 'NONE',  ( 13.42747647338834760, 171.8927522451418213, -10.00000000000009059 ) ) ;
#91002=CARTESIAN_POINT ( 'NONE',  ( 164.0644709900060718, 246.4789958588364698, -8.616711260302015063 ) ) ;
#91005=CARTESIAN_POINT ( 'NONE',  ( 164.6506446267413253, 274.3553168417332131, 14.79851574671830505 ) ) ;
#91006=CARTESIAN_POINT ( 'NONE',  ( 4.289451341410244645, 161.0327760586659451, 1.948934522072303157E-15 ) ) ;
#91007=CARTESIAN_POINT ( 'NONE',  ( 189.0750166644107821, 297.0310844892443356, 8.177982547853755335 ) ) ;
#91010=CARTESIAN_POINT ( 'NONE',  ( 198.7134558283731280, 282.8386145195935910, 17.66748989068429054 ) ) ;
#91012=CARTESIAN_POINT ( 'NONE',  ( 174.7639949172803995, 290.4895449553895901, 2.562946516734061930 ) ) ;
#91014=DIRECTION ( 'NONE',  ( -0.8660254037844382635, -0.5000000000000006661, 0.000000000000000000 ) ) ;
#91016=CARTESIAN_POINT ( 'NONE',  ( 153.2019974609038115, 278.5196124964878095, 3.744932174532282332 ) ) ;
#91017=CARTESIAN_POINT ( 'NONE',  ( 22.39418752168989712, 192.9244531367911293, -4.594050593750046652 ) ) ;
#91018=CARTESIAN_POINT ( 'NONE',  ( 106.6962611473900893, 244.6589784336661069, -6.496448406907675876E-16 ) ) ;
#91019=CARTESIAN_POINT ( 'NONE',  ( 40.18174127881769664, 205.5530062829863027, -4.648177544792955347E-16 ) ) ;
#91020=CARTESIAN_POINT ( 'NONE',  ( 183.7400870242638860, 256.7387704515565474, -3.095244190633015702 ) ) ;
#91021=CARTESIAN_POINT ( 'NONE',  ( 206.4069886254544031, 272.1500834713139625, -7.842899504808422684 ) ) ;
#91023=AXIS2_PLACEMENT_3D ( 'NONE', #10289, #1190, #56372 ) ;
#91025=CARTESIAN_POINT ( 'NONE',  ( 154.8989000222956349, 262.3542304552891551, 17.41779271305265908 ) ) ;
#91026=CARTESIAN_POINT ( 'NONE',  ( 207.7320178805681508, 270.8445860024863237, -5.379955943374661764 ) ) ;
#91030=CARTESIAN_POINT ( 'NONE',  ( 196.6001939379022758, 266.5684052957021208, 8.222072963770980181 ) ) ;
#91031=CARTESIAN_POINT ( 'NONE',  ( 198.5725620961998459, 266.5936579278944691, -7.138590148556124504 ) ) ;
#91032=CARTESIAN_POINT ( 'NONE',  ( 164.0412359135344786, 252.8541476746656826, -12.95066152372220536 ) ) ;
#91035=CARTESIAN_POINT ( 'NONE',  ( 101.7984123748231298, 220.3923013555410080, 4.594050593750050204 ) ) ;
#91037=CARTESIAN_POINT ( 'NONE',  ( 150.6453220160077251, 269.7216436761371483, 14.94145576020818034 ) ) ;
#91040=CARTESIAN_POINT ( 'NONE',  ( 157.5042325173297684, 257.8416622032797818, 16.70595240278738203 ) ) ;
#91042=CARTESIAN_POINT ( 'NONE',  ( 191.2622316156482043, 288.8574828335728171, -16.55244734589887656 ) ) ;
#91043=CARTESIAN_POINT ( 'NONE',  ( 164.8075539017095252, 280.4672370525465226, 12.63796469268613265 ) ) ;
#91046=CARTESIAN_POINT ( 'NONE',  ( 146.9700173529739970, 276.0874580858064746, -5.099093031535578469 ) ) ;
#91048=EDGE_LOOP ( 'NONE', ( #20686, #38584, #50787, #88914 ) ) ;
#91050=DIRECTION ( 'NONE',  ( 0.4999999999999998890, -0.8660254037844385966, 0.000000000000000000 ) ) ;
#91051=CARTESIAN_POINT ( 'NONE',  ( 147.2567621633200474, 275.5908015054806128, -3.647191014543873955 ) ) ;
#91052=CARTESIAN_POINT ( 'NONE',  ( 149.4171629335945681, 271.8488776066536730, -11.42564036194071520 ) ) ;
#91057=CARTESIAN_POINT ( 'NONE',  ( 198.3075590527773784, 287.1682275260610027, 16.94807365630277118 ) ) ;
#91061=CARTESIAN_POINT ( 'NONE',  ( 133.0291931787496651, 247.6115022471902591, 10.00000000000009592 ) ) ;
#91062=ORIENTED_EDGE ( 'NONE', *, *, #1004, .T. ) ;
#91069=CARTESIAN_POINT ( 'NONE',  ( 185.3093006960060336, 292.6213584219709105, -10.65003670060383101 ) ) ;
#91072=CARTESIAN_POINT ( 'NONE',  ( 205.5340210668974237, 274.6516281586387436, 11.25376706788097714 ) ) ;
#91073=CARTESIAN_POINT ( 'NONE',  ( 190.6012238204759228, 278.5005121819996816, -16.53506780650642582 ) ) ;
#91074=CARTESIAN_POINT ( 'NONE',  ( 154.0631780868778264, 263.8017433084320942, -17.71705682590848951 ) ) ;
#91075=CARTESIAN_POINT ( 'NONE',  ( 152.7375212135632125, 266.0978483664162582, -16.47968945089317572 ) ) ;
#91077=CARTESIAN_POINT ( 'NONE',  ( 194.4572733120733119, 265.4698506025051188, 9.231589761896536572 ) ) ;
#91082=CARTESIAN_POINT ( 'NONE',  ( 198.1186603539670728, 286.9451690787467442, 16.94706959193672446 ) ) ;
#91084=CARTESIAN_POINT ( 'NONE',  ( 174.0349010169910287, 257.2697708657194084, -11.84118670213688240 ) ) ;
#91085=CARTESIAN_POINT ( 'NONE',  ( 162.5812530041002049, 272.3672700969655693, -15.68205036963906807 ) ) ;
#91087=CARTESIAN_POINT ( 'NONE',  ( 197.4226313177773591, 273.1407988583247288, -13.32284819095123751 ) ) ;
#91088=CARTESIAN_POINT ( 'NONE',  ( 156.4445880091442120, 261.3333284696779515, -17.64838406174382612 ) ) ;
#91089=CARTESIAN_POINT ( 'NONE',  ( 190.3691966041315311, 300.9178746160123410, 0.1783449565851275009 ) ) ;
#91090=CARTESIAN_POINT ( 'NONE',  ( 169.7116465267147873, 287.0218441930870199, -4.634240893799990602 ) ) ;
#91092=CARTESIAN_POINT ( 'NONE',  ( 186.3888140740535562, 286.9988348145756163, -16.10978017299487064 ) ) ;
#91093=CARTESIAN_POINT ( 'NONE',  ( 112.2989703957094605, 226.4548013555409796, -4.594050593750042211 ) ) ;
#91096=CARTESIAN_POINT ( 'NONE',  ( 191.9588319567279200, 275.3209462115174233, 16.40384393395227747 ) ) ;
#91098=AXIS2_PLACEMENT_3D ( 'NONE', #70303, #77925, #15095 ) ;
#91102=B_SPLINE_SURFACE_WITH_KNOTS ( 'NONE', 3, 1, ( 
 ( #1634, #56802 ),
 ( #72540, #87787 ),
 ( #11238, #42101 ),
 ( #18326, #18821 ),
 ( #49705, #49223 ),
 ( #10721, #73035 ),
 ( #41597, #3146 ),
 ( #34031, #64918 ),
 ( #95863, #26421 ),
 ( #57300, #88272 ),
 ( #31995, #62905 ),
 ( #93857, #24412 ),
 ( #55288, #78628 ),
 ( #40088, #71032 ),
 ( #12219, #89752 ),
 ( #35990, #42587 ),
 ( #11725, #82659 ),
 ( #66895, #26915 ),
 ( #75019, #4103 ),
 ( #90755, #44079 ),
 ( #5110, #50692 ),
 ( #81158, #44577 ),
 ( #98320, #67395 ),
 ( #13222, #28911 ),
 ( #43078, #21307 ),
 ( #74531, #97331 ),
 ( #81647, #19822 ),
 ( #58779, #73520 ),
 ( #57795, #59786 ),
 ( #74021, #5601 ),
 ( #52184, #4609 ),
 ( #88774, #83133 ),
 ( #65898, #12728 ),
 ( #35502, #20318 ) ),
 .UNSPECIFIED., .T., .F., .F.,
 ( 4, 2, 2, 2, 2, 2, 2, 2, 2, 2, 2, 2, 2, 2, 2, 2, 4 ),
 ( 2, 2 ),
 ( 0.000000000000000000, 0.06250000000000000000, 0.1250000000000000000, 0.1875000000000000000, 0.2500000000000000000, 0.3125000000000000000, 0.3750000000000000000, 0.4375000000000000000, 0.5000000000000000000, 0.5625000000000000000, 0.6250000000000000000, 0.6875000000000000000, 0.7500000000000000000, 0.8125000000000000000, 0.8750000000000000000, 0.9375000000000000000, 1.000000000000000000 ),
 ( 0.000000000000000000, 1.000000000000000000 ),
 .UNSPECIFIED. ) ;
#91103=CARTESIAN_POINT ( 'NONE',  ( 157.1606030646430554, 258.4368458743103361, 17.96998724893680688 ) ) ;
#91105=CARTESIAN_POINT ( 'NONE',  ( -22.42236680055709641, 157.8615022471902591, 0.000000000000000000 ) ) ;
#91107=CARTESIAN_POINT ( 'NONE',  ( 195.3286257065703069, 292.3278914340530719, 16.60614309818382495 ) ) ;
#91108=ORIENTED_EDGE ( 'NONE', *, *, #99405, .T. ) ;
#91111=CARTESIAN_POINT ( 'NONE',  ( 206.5117639185820906, 272.9581278627833285, 11.28485531511759099 ) ) ;
#91112=CIRCLE ( 'NONE', #13500, 10.00000000000011369 ) ;
#91113=CARTESIAN_POINT ( 'NONE',  ( 194.8492499382162180, 264.8919437935018664, 4.416793385568180241 ) ) ;
#91114=CARTESIAN_POINT ( 'NONE',  ( 177.5879455283492234, 272.4518736442240083, -17.80684084945183088 ) ) ;
#91115=EDGE_CURVE ( 'NONE', #94946, #59130, #66812, .T. ) ;
#91119=FACE_OUTER_BOUND ( 'NONE', #81026, .T. ) ;
#91124=CARTESIAN_POINT ( 'NONE',  ( 192.5458920237629457, 271.5594986157455537, 14.05193011733685005 ) ) ;
#91125=CARTESIAN_POINT ( 'NONE',  ( 165.0952264510788154, 281.4963861521250124, -11.84807672454148886 ) ) ;
#91127=EDGE_CURVE ( 'NONE', #63007, #8285, #25760, .T. ) ;
#91132=CARTESIAN_POINT ( 'NONE',  ( 84.34250105585179824, 213.3768266524160140, 9.188101187500098632 ) ) ;
#91133=CARTESIAN_POINT ( 'NONE',  ( 159.2394649670193303, 254.8361514374751664, -16.43133403737800791 ) ) ;
#91138=CARTESIAN_POINT ( 'NONE',  ( 207.1211793645798878, 271.9025893473983047, -6.294110402770905388 ) ) ;
#91141=CARTESIAN_POINT ( 'NONE',  ( 111.6751914540069635, 246.8297689869268936, -2.679491924311252493 ) ) ;
#91146=CARTESIAN_POINT ( 'NONE',  ( 157.5710319558766344, 257.7259621817996162, 18.28704422422941533 ) ) ;
#91147=CARTESIAN_POINT ( 'NONE',  ( 199.4716132138953242, 277.5915922024631755, 15.21463707318425662 ) ) ;
#91150=CARTESIAN_POINT ( 'NONE',  ( 50.29670382169353360, 199.8458772461660260, 9.188101187500095079 ) ) ;
#91152=CARTESIAN_POINT ( 'NONE',  ( 198.8533049117289977, 286.2229679703367538, -18.60939981449148561 ) ) ;
#91155=CARTESIAN_POINT ( 'NONE',  ( 202.3081618345277946, 269.6788042618418331, -6.424812278093250839 ) ) ;
#91159=CARTESIAN_POINT ( 'NONE',  ( 153.0558112840829210, 276.6942330888239212, 7.179448329669019024 ) ) ;
#91161=CARTESIAN_POINT ( 'NONE',  ( 163.7892944603517833, 255.0961238338549322, -15.29376416924185556 ) ) ;
#91164=CARTESIAN_POINT ( 'NONE',  ( 87.49069069641790009, 227.9865022471902876, -10.00000000000009415 ) ) ;
#91165=CARTESIAN_POINT ( 'NONE',  ( 182.9360775077161918, 292.9515156215683760, -10.62356958548592445 ) ) ;
#91169=CARTESIAN_POINT ( 'NONE',  ( 57.33281313167710636, 216.1589784336661921, -6.496448406907675876E-16 ) ) ;
#91172=CARTESIAN_POINT ( 'NONE',  ( 182.7616540338069342, 265.0621685301391040, 14.91793811211548082 ) ) ;
#91173=CARTESIAN_POINT ( 'NONE',  ( 185.3705633484216264, 298.4094130272380880, -0.2897616204090320280 ) ) ;
#91175=EDGE_CURVE ( 'NONE', #2973, #44048, #98237, .T. ) ;
#91178=CARTESIAN_POINT ( 'NONE',  ( 159.9950753608005130, 276.8117990079294373, 13.35014033362692487 ) ) ;
#91182=CARTESIAN_POINT ( 'NONE',  ( 206.8139415932446354, 271.7863864866807262, -6.273988927840268737 ) ) ;
#91183=CARTESIAN_POINT ( 'NONE',  ( 157.1187995864133882, 258.5092516225370218, 18.42986330599266509 ) ) ;
#91190=B_SPLINE_CURVE_WITH_KNOTS ( 'NONE', 3,
 ( #65603, #2330, #55983, #32708 ),
 .UNSPECIFIED., .F., .F.,
 ( 4, 4 ),
 ( 0.01002733877639494162, 0.01522564162345051847 ),
 .UNSPECIFIED. ) ;
#91192=ORIENTED_EDGE ( 'NONE', *, *, #100099, .T. ) ;
#91194=CARTESIAN_POINT ( 'NONE',  ( 168.0160359207364991, 287.1960299647130341, -6.005792533259211474 ) ) ;
#91196=CARTESIAN_POINT ( 'NONE',  ( 163.0056347026689707, 248.3129541054019569, -11.27842346302751508 ) ) ;
#91197=CARTESIAN_POINT ( 'NONE',  ( 164.2297246530060875, 246.1927681183832988, 5.803160395959773510 ) ) ;
#91200=CARTESIAN_POINT ( 'NONE',  ( 164.3713636635203841, 264.9441660766296991, -16.63686112330542599 ) ) ;
#91201=CARTESIAN_POINT ( 'NONE',  ( 126.7502486777147794, 253.1744531367911009, 4.594050593750047540 ) ) ;
#91202=CARTESIAN_POINT ( 'NONE',  ( 84.82981389336303835, 207.5327760586659167, 1.948934522072303157E-15 ) ) ;
#91203=ORIENTED_EDGE ( 'NONE', *, *, #76526, .T. ) ;
#91204=CARTESIAN_POINT ( 'NONE',  ( 174.1591195100927791, 265.6402296398555904, 16.51580490226363906 ) ) ;
#91209=VERTEX_POINT ( 'NONE', #91234 ) ;
#91213=CARTESIAN_POINT ( 'NONE',  ( 191.8329718516215223, 298.3825415164982928, -8.871589506312979267 ) ) ;
#91215=CARTESIAN_POINT ( 'NONE',  ( 155.5204415533959548, 261.2776889444089647, 17.19127227448963424 ) ) ;
#91216=CARTESIAN_POINT ( 'NONE',  ( 81.06766895168337328, 207.6115022471902023, -5.000000000000041744 ) ) ;
#91217=CARTESIAN_POINT ( 'NONE',  ( 182.0915030940412862, 257.1429800395595748, -6.159901684290187696 ) ) ;
#91218=ORIENTED_EDGE ( 'NONE', *, *, #97446, .F. ) ;
#91219=CARTESIAN_POINT ( 'NONE',  ( 161.9258069053378222, 250.1832707138045180, -14.03928993546631254 ) ) ;
#91221=CARTESIAN_POINT ( 'NONE',  ( 163.9634607461725011, 260.5862723289976088, -16.19362549185895261 ) ) ;
#91222=CARTESIAN_POINT ( 'NONE',  ( 164.8962722568797687, 246.6821832418063707, 5.577076257785627433 ) ) ;
#91223=CARTESIAN_POINT ( 'NONE',  ( 187.4299001019809623, 277.0409167645560728, 16.92852667520122267 ) ) ;
#91224=CARTESIAN_POINT ( 'NONE',  ( 206.0627831668701901, 273.7357853363691902, 10.14454147593459687 ) ) ;
#91226=CARTESIAN_POINT ( 'NONE',  ( 149.2223635749290622, 272.1862799931444670, -12.97307652490353647 ) ) ;
#91227=CARTESIAN_POINT ( 'NONE',  ( 198.6773598015395521, 281.0098537826190181, 16.91893506919627654 ) ) ;
#91229=CARTESIAN_POINT ( 'NONE',  ( 146.3987206697217403, 246.1423013555409796, -4.594050593750043987 ) ) ;
#91234=CARTESIAN_POINT ( 'NONE',  ( 167.2900023830132170, 283.1360949131732809, -11.47530909209802275 ) ) ;
#91240=CARTESIAN_POINT ( 'NONE',  ( 182.2006005650631266, 275.4475936646326204, -16.49366260708473320 ) ) ;
#91241=CARTESIAN_POINT ( 'NONE',  ( 172.8951663193395234, 288.9549776225803157, 8.104654168245465584 ) ) ;
#91243=CARTESIAN_POINT ( 'NONE',  ( 185.6631226553351439, 263.8051797751761001, -12.74678442662920652 ) ) ;
#91244=CARTESIAN_POINT ( 'NONE',  ( 202.5128468779458331, 267.1751508879428343, 0.8823122286173835649 ) ) ;
#91246=CARTESIAN_POINT ( 'NONE',  ( 195.1818950096821368, 263.7941917347654908, 0.8445903136804231437 ) ) ;
#91248=CARTESIAN_POINT ( 'NONE',  ( 147.1199024702499969, 275.8278494473859723, 5.224467159276165340 ) ) ;
#91249=CARTESIAN_POINT ( 'NONE',  ( 186.8638380190930377, 282.1138426105056283, 17.22312890734132296 ) ) ;
#91250=CARTESIAN_POINT ( 'NONE',  ( 164.8251969117060298, 245.1613799118173063, -1.508678420156898348 ) ) ;
#91251=CARTESIAN_POINT ( 'NONE',  ( 196.8251380678160274, 269.8453290852096416, 12.06679547565278909 ) ) ;
#91254=EDGE_CURVE ( 'NONE', #17524, #16763, #78868, .T. ) ;
#91255=CARTESIAN_POINT ( 'NONE',  ( 149.0359194785865498, 272.5092106407810206, 12.76357969772040590 ) ) ;
#91256=CARTESIAN_POINT ( 'NONE',  ( 79.60625107924921906, 206.7677522451417929, -5.000000000000041744 ) ) ;
#91259=CARTESIAN_POINT ( 'NONE',  ( 159.9307118030769175, 253.6388767968520881, 16.60600887889890487 ) ) ;
#91260=CARTESIAN_POINT ( 'NONE',  ( 207.2934823643110178, 271.6041517975674537, 5.071655803097819160 ) ) ;
#91261=CARTESIAN_POINT ( 'NONE',  ( 140.7332108297007665, 265.3927522451418781, 2.944929066748280225E-16 ) ) ;
#91266=CARTESIAN_POINT ( 'NONE',  ( 151.0426280674448378, 269.0334894088936153, -15.84467774422408581 ) ) ;
#91267=CARTESIAN_POINT ( 'NONE',  ( 7.266240119036749157, 168.8768266524159856, -9.188101187500093303 ) ) ;
#91268=B_SPLINE_CURVE_WITH_KNOTS ( 'NONE', 3,
 ( #65245, #87125, #72879, #57132 ),
 .UNSPECIFIED., .F., .F.,
 ( 4, 4 ),
 ( 0.03752702852749528750, 0.04612527040108949095 ),
 .UNSPECIFIED. ) ;
#91271=CARTESIAN_POINT ( 'NONE',  ( 170.0577865676564215, 270.6915287872138833, -17.14917795963988212 ) ) ;
#91273=CARTESIAN_POINT ( 'NONE',  ( 150.1280791300635826, 276.5080219999884434, 3.727701050747722178 ) ) ;
#91275=CARTESIAN_POINT ( 'NONE',  ( 175.5054462216997422, 253.5402674413775799, -3.793157809723892271 ) ) ;
#91276=CARTESIAN_POINT ( 'NONE',  ( 150.2678036912315349, 270.3755245954375823, 14.25047800729520375 ) ) ;
#91278=CARTESIAN_POINT ( 'NONE',  ( 53.86003751612224733, 195.2365022471902023, -10.00000000000009059 ) ) ;
#91280=CARTESIAN_POINT ( 'NONE',  ( 148.1672759425158290, 274.0137453789218398, 7.847779094015780110 ) ) ;
#91281=CARTESIAN_POINT ( 'NONE',  ( 21.98867198337220685, 177.3768266524160140, 9.188101187500098632 ) ) ;
#91282=CARTESIAN_POINT ( 'NONE',  ( 164.8765683363924666, 284.8271691914964663, 4.187516861581451977 ) ) ;
#91283=CARTESIAN_POINT ( 'NONE',  ( 152.7531861616124615, 266.0707158804971186, 17.45453282433162556 ) ) ;
#91287=EDGE_CURVE ( 'NONE', #20951, #68688, #22154, .T. ) ;
#91288=CARTESIAN_POINT ( 'NONE',  ( 185.3021252847411802, 266.6084221390160565, 13.26759877312805180 ) ) ;
#91289=CARTESIAN_POINT ( 'NONE',  ( 153.6392919293977002, 266.5359356698173769, -16.75038546547492402 ) ) ;
#91293=CARTESIAN_POINT ( 'NONE',  ( 190.6071113721798156, 300.5057941498820924, -0.4754021072632813594 ) ) ;
#91296=CARTESIAN_POINT ( 'NONE',  ( 155.6276701977099890, 261.0919634844306643, 17.49722577287685255 ) ) ;
#91298=DIRECTION ( 'NONE',  ( 0.4999999999999998890, -0.8660254037844385966, 0.000000000000000000 ) ) ;
#91300=EDGE_CURVE ( 'NONE', #6702, #4197, #45109, .T. ) ;
#91303=EDGE_CURVE ( 'NONE', #8797, #67335, #61953, .T. ) ;
#91306=CARTESIAN_POINT ( 'NONE',  ( 148.2404373810095706, 275.8870260502966403, -5.709515531134017330 ) ) ;
#91308=CARTESIAN_POINT ( 'NONE',  ( 203.5629025532486196, 278.0657055720176913, -15.85226727704602823 ) ) ;
#91310=ORIENTED_EDGE ( 'NONE', *, *, #7613, .T. ) ;
#91312=CARTESIAN_POINT ( 'NONE',  ( 164.4272222519600746, 245.8506922426221593, 7.021336339662529902 ) ) ;
#91314=CARTESIAN_POINT ( 'NONE',  ( 153.1961624462112752, 265.3034584490234806, -16.19494717845262954 ) ) ;
#91321=CARTESIAN_POINT ( 'NONE',  ( 196.9098758191317700, 289.5890858996224324, -16.54412079817003800 ) ) ;
#91322=ORIENTED_EDGE ( 'NONE', *, *, #476, .F. ) ;
#91323=CARTESIAN_POINT ( 'NONE',  ( 164.9171241593586217, 245.0021572482830550, 1.622680932994367220 ) ) ;
#91326=CARTESIAN_POINT ( 'NONE',  ( 190.4163244163388242, 300.8362468508201459, 4.691083071570470331 ) ) ;
#91327=CARTESIAN_POINT ( 'NONE',  ( 195.1474640768281290, 265.6393084148356252, -8.887799905196541062 ) ) ;
#91328=VERTEX_POINT ( 'NONE', #78008 ) ;
#91332=CARTESIAN_POINT ( 'NONE',  ( 103.4423036115607601, 218.9824982072974251, 3.021315404115420679E-15 ) ) ;
#91334=VERTEX_POINT ( 'NONE', #8600 ) ;
#91335=( BOUNDED_CURVE ( )  B_SPLINE_CURVE ( 2, ( #35872, #98195, #66776, #36364, #97701, #28777, #11109, #41979, #34384 ),
 .UNSPECIFIED., .F., .T. ) 
 B_SPLINE_CURVE_WITH_KNOTS ( ( 3, 2, 2, 2, 3 ),
 ( 0.6895161290322581182, 0.6908602150537634934, 0.6935483870967742437, 0.6962365591397849940, 0.6975806451612903691 ),
 .UNSPECIFIED. ) 
 CURVE ( )  GEOMETRIC_REPRESENTATION_ITEM ( )  RATIONAL_B_SPLINE_CURVE ( ( 0.9330127018922194093, 0.9330127018922194093, 1.000000000000000000, 0.8660254037844387076, 1.000000000000000000, 0.8660254037844387076, 1.000000000000000000, 0.9330127018922194093, 0.9330127018922194093 ) ) 
 REPRESENTATION_ITEM ( '' )  );
#91337=CARTESIAN_POINT ( 'NONE',  ( 147.4368675721658519, 275.2788497866417288, 5.050119523016719292 ) ) ;
#91338=CARTESIAN_POINT ( 'NONE',  ( 190.3691966041315311, 300.9178746160123410, 0.1783449565851275009 ) ) ;
#91339=CARTESIAN_POINT ( 'NONE',  ( 190.1751179328237242, 301.2540287353828035, 3.252640783176552475 ) ) ;
#91340=CARTESIAN_POINT ( 'NONE',  ( 192.2943420783192323, 297.5834248427583475, 12.53393473147773562 ) ) ;
#91341=CARTESIAN_POINT ( 'NONE',  ( 147.3005892150715113, 275.5148908251009061, -0.09882562957467407039 ) ) ;
#91342=CARTESIAN_POINT ( 'NONE',  ( 146.5913834600193582, 276.7432712258716947, -0.4909717733184599253 ) ) ;
#91343=B_SPLINE_CURVE_WITH_KNOTS ( 'NONE', 3,
 ( #79718, #19402, #65466, #25470, #87359, #50261, #17888, #48787, #72089, #51246 ),
 .UNSPECIFIED., .F., .F.,
 ( 4, 2, 2, 2, 4 ),
 ( 0.0003596424459949675977, 0.0006587098368031852821, 0.0009577772276114028581, 0.001256844618419620434, 0.001555912009227838119 ),
 .UNSPECIFIED. ) ;
#91348=CARTESIAN_POINT ( 'NONE',  ( 168.2949371938393597, 286.3488455771775421, 4.006590656272537743 ) ) ;
#91350=EDGE_LOOP ( 'NONE', ( #37815, #42706, #87328, #58231 ) ) ;
#91351=CARTESIAN_POINT ( 'NONE',  ( 190.0373668968398988, 301.4926205285023002, -3.919393248615649306 ) ) ;
#91353=CARTESIAN_POINT ( 'NONE',  ( 148.8662434136574291, 273.1977519777474299, 9.320112586661617016 ) ) ;
#91355=CARTESIAN_POINT ( 'NONE',  ( 39.04508293989853485, 204.8967562850347122, -4.648177544792955347E-16 ) ) ;
#91356=CARTESIAN_POINT ( 'NONE',  ( 147.9216321868252066, 274.4392128443400907, -9.725520637227743848 ) ) ;
#91357=CARTESIAN_POINT ( 'NONE',  ( 166.8351002587995140, 283.9006457132830974, -8.055937853886671718 ) ) ;
#91358=EDGE_LOOP ( 'NONE', ( #22602, #85935, #56911, #61133, #4216 ) ) ;
#91359=CARTESIAN_POINT ( 'NONE',  ( 170.5981529699230066, 255.5880127657044625, -12.68729301884834371 ) ) ;
#91362=CARTESIAN_POINT ( 'NONE',  ( 48.93451802855033606, 192.3927522451418213, 10.00000000000009592 ) ) ;
#91363=CARTESIAN_POINT ( 'NONE',  ( 120.7155680147981940, 234.3768266524159856, 9.188101187500096856 ) ) ;
#91364=EDGE_CURVE ( 'NONE', #94561, #45170, #32395, .T. ) ;
#91365=CARTESIAN_POINT ( 'NONE',  ( 151.2964716097791325, 268.5938194963972592, -15.66250187539618111 ) ) ;
#91368=CARTESIAN_POINT ( 'NONE',  ( 172.5941544643821999, 251.3792726610714112, -3.974732898687233895 ) ) ;
#91369=CARTESIAN_POINT ( 'NONE',  ( 30.97333845187074886, 194.8149278399160949, -9.188101187500095079 ) ) ;
#91372=CARTESIAN_POINT ( 'NONE',  ( 190.1774295428112396, 299.2500249094251217, 7.542682482482700124 ) ) ;
#91373=CARTESIAN_POINT ( 'NONE',  ( 15.10771242554802463, 167.9824982072973967, -5.229199737892075682E-14 ) ) ;
#91375=CARTESIAN_POINT ( 'NONE',  ( 18.20865839366279459, 187.9865022471902876, 10.00000000000009415 ) ) ;
#91377=CARTESIAN_POINT ( 'NONE',  ( 146.8000281410530192, 276.3818880375922049, 4.652863924796177386 ) ) ;
#91381=CARTESIAN_POINT ( 'NONE',  ( 176.2784227036720210, 285.4830148766054663, -12.04998877190618067 ) ) ;
#91382=CARTESIAN_POINT ( 'NONE',  ( 164.1276822366001511, 250.0947574105164506, 10.98824708228447733 ) ) ;
#91383=CARTESIAN_POINT ( 'NONE',  ( 107.7520767022434853, 223.0177522451418213, 5.000000000000051514 ) ) ;
#91385=CARTESIAN_POINT ( 'NONE',  ( 195.7767944968437632, 266.9069622423809847, -7.771366023404486789 ) ) ;
#91387=CARTESIAN_POINT ( 'NONE',  ( 158.5437609352171933, 281.8370119815768362, -1.612487481721458948 ) ) ;
#91388=CARTESIAN_POINT ( 'NONE',  ( 163.1369207721744772, 248.0855599626920593, -11.24692769914530110 ) ) ;
#91389=CARTESIAN_POINT ( 'NONE',  ( 12.43489537816885537, 187.1744531367911293, 4.594050593750047540 ) ) ;
#91391=CARTESIAN_POINT ( 'NONE',  ( 192.1258111988436781, 272.3008933654719499, 14.87177412048350966 ) ) ;
#91393=CARTESIAN_POINT ( 'NONE',  ( 157.2948870673828026, 280.9759411348209142, 6.053012778684776940 ) ) ;
#91394=CARTESIAN_POINT ( 'NONE',  ( 174.9881383257676646, 286.4353486899028667, 10.48873152270803466 ) ) ;
#91395=CARTESIAN_POINT ( 'NONE',  ( 63.34103791831414298, 213.5024278399161233, 9.188101187500095079 ) ) ;
#91396=CARTESIAN_POINT ( 'NONE',  ( 208.3057440179679531, 269.8508631828800617, 2.969924427282375046 ) ) ;
#91402=CARTESIAN_POINT ( 'NONE',  ( 9.548404355818409073, 182.9865022471903160, -10.00000000000009415 ) ) ;
#91403=CARTESIAN_POINT ( 'NONE',  ( 207.7655736232174206, 270.7864657513322300, 3.530742899761726949 ) ) ;
#91404=CARTESIAN_POINT ( 'NONE',  ( 132.6230702210692414, 253.5024278399160949, -9.188101187500093303 ) ) ;
#91406=CARTESIAN_POINT ( 'NONE',  ( 189.4381674897702794, 265.0040801212285828, 12.03645615491573828 ) ) ;
#91408=EDGE_CURVE ( 'NONE', #95312, #98060, #17301, .T. ) ;
#91416=CARTESIAN_POINT ( 'NONE',  ( 152.1434865710199063, 268.6225420542635902, -15.29845542693487914 ) ) ;
#91417=CARTESIAN_POINT ( 'NONE',  ( 196.4280118926366185, 289.9318269284742655, 16.33325042109277803 ) ) ;
#91420=CARTESIAN_POINT ( 'NONE',  ( 159.9468613345221684, 253.6109049878705832, 15.91085046606713327 ) ) ;
#91427=CARTESIAN_POINT ( 'NONE',  ( 149.7206294291796667, 272.5596913884758123, 11.32704556092920889 ) ) ;
#91428=CARTESIAN_POINT ( 'NONE',  ( 175.7622132985686392, 274.0430017844784629, -17.75579533532145504 ) ) ;
#91429=CARTESIAN_POINT ( 'NONE',  ( 200.7694952279801157, 282.9040289856181403, -17.94628235092568502 ) ) ;
#91434=CARTESIAN_POINT ( 'NONE',  ( 84.34903687182406884, 231.0530062829863027, -4.648177544792955347E-16 ) ) ;
#91436=CARTESIAN_POINT ( 'NONE',  ( 148.9719199701866899, 272.6200610409887872, 12.59512981512031438 ) ) ;
#91439=ORIENTED_EDGE ( 'NONE', *, *, #9468, .T. ) ;
#91440=CARTESIAN_POINT ( 'NONE',  ( 191.1192699377806719, 299.6187094927299199, -9.526914969203620132 ) ) ;
#91442=CARTESIAN_POINT ( 'NONE',  ( 163.7729086741176161, 246.9839966035275438, 6.099406794390714204 ) ) ;
#91446=CARTESIAN_POINT ( 'NONE',  ( 98.17141035282828909, 236.6744531367911293, 4.594050593750047540 ) ) ;
#91447=CARTESIAN_POINT ( 'NONE',  ( 202.8812894462602401, 279.2462941044264539, 15.70414016608259722 ) ) ;
#91448=CARTESIAN_POINT ( 'NONE',  ( 179.2330864023228685, 269.9232757945108006, -16.11891054009439728 ) ) ;
#91450=EDGE_LOOP ( 'NONE', ( #67203, #10986, #38862, #624 ) ) ;
#91451=ORIENTED_EDGE ( 'NONE', *, *, #30959, .T. ) ;
#91454=AXIS2_PLACEMENT_3D ( 'NONE', #98035, #19556, #35221 ) ;
#91455=ORIENTED_EDGE ( 'NONE', *, *, #7992, .F. ) ;
#91457=EDGE_LOOP ( 'NONE', ( #87735, #85198, #64099, #21392 ) ) ;
#91458=CARTESIAN_POINT ( 'NONE',  ( 163.7085541710205234, 247.0954618725873217, -6.713544974106887331 ) ) ;
#91459=CARTESIAN_POINT ( 'NONE',  ( 200.9521687275011175, 282.5876292032514243, -18.16013154125647944 ) ) ;
#91464=B_SPLINE_CURVE_WITH_KNOTS ( 'NONE', 3,
 ( #64302, #95253, #41484, #25820, #56697, #87677, #18213, #49105, #49593, #80547 ),
 .UNSPECIFIED., .F., .F.,
 ( 4, 2, 2, 2, 4 ),
 ( 0.001136000421166406512, 0.001208387388216028554, 0.001280774355265650597, 0.001425548289364900753, 0.001715096157563401067 ),
 .UNSPECIFIED. ) ;
#91467=CARTESIAN_POINT ( 'NONE',  ( 167.2650757157126407, 283.7916248837542526, 9.058252512891741048 ) ) ;
#91469=CARTESIAN_POINT ( 'NONE',  ( 117.2061873602235238, 245.1427522451419065, -10.00000000000009592 ) ) ;
#91470=VERTEX_POINT ( 'NONE', #58184 ) ;
#91471=CARTESIAN_POINT ( 'NONE',  ( 199.1165320752825494, 285.7670451491295580, 0.000000000000000000 ) ) ;
#91473=CARTESIAN_POINT ( 'NONE',  ( 158.3909187560116436, 280.0920373912738910, -6.736592508546087821 ) ) ;
#91476=CARTESIAN_POINT ( 'NONE',  ( 171.3293103646413726, 255.5786316856422786, 11.21396041803508581 ) ) ;
#91477=CARTESIAN_POINT ( 'NONE',  ( 157.6839078477695182, 281.5272880355949496, 1.407186217441265264 ) ) ;
#91479=CARTESIAN_POINT ( 'NONE',  ( 101.8522786425099156, 219.6115022471901739, -5.000000000000041744 ) ) ;
#91482=CARTESIAN_POINT ( 'NONE',  ( 1.663964738649737374, 161.7677522451418213, -5.000000000000041744 ) ) ;
#91484=CARTESIAN_POINT ( 'NONE',  ( 193.3208433121157839, 266.9444617411745071, -11.48094634684561122 ) ) ;
#91485=CARTESIAN_POINT ( 'NONE',  ( 172.1197128340322422, 279.8946286459532757, -14.44200207385173229 ) ) ;
#91486=CARTESIAN_POINT ( 'NONE',  ( 163.4060470519778505, 247.6194195724207248, -7.715457960547858818 ) ) ;
#91489=CARTESIAN_POINT ( 'NONE',  ( -15.41332078621576329, 174.1589784336661637, -6.496448406907675876E-16 ) ) ;
#91492=CARTESIAN_POINT ( 'NONE',  ( 185.1771979290287220, 295.2786484640562321, 8.360689780431474816 ) ) ;
#91494=EDGE_LOOP ( 'NONE', ( #76513, #57135, #89151, #27284, #70194, #22447 ) ) ;
#91495=CARTESIAN_POINT ( 'NONE',  ( 4.715407580134756138, 161.9824982072973683, 3.021315404115420679E-15 ) ) ;
#91497=EDGE_CURVE ( 'NONE', #51125, #72620, #71696, .T. ) ;
#91498=CARTESIAN_POINT ( 'NONE',  ( 175.0803495703506769, 291.9523537460119655, 3.393087883739125399 ) ) ;
#91501=CARTESIAN_POINT ( 'NONE',  ( 162.5371025824206868, 249.1244755426497477, -11.58906134139951760 ) ) ;
#91505=CARTESIAN_POINT ( 'NONE',  ( 18.30771692152332975, 187.5024278399160949, -9.188101187500093303 ) ) ;
#91506=CARTESIAN_POINT ( 'NONE',  ( 125.9117204375048544, 237.3768266524159856, 9.188101187500098632 ) ) ;
#91507=CARTESIAN_POINT ( 'NONE',  ( 182.0998838648946219, 294.4493588421104846, -6.417080199048857736 ) ) ;
#91508=CARTESIAN_POINT ( 'NONE',  ( 183.6633101453114421, 256.8715506259877088, -3.169286389211312560 ) ) ;
#91510=FACE_OUTER_BOUND ( 'NONE', #87789, .T. ) ;
#91512=CARTESIAN_POINT ( 'NONE',  ( 188.1160556981905358, 261.6047048220251554, 8.946321273836643329 ) ) ;
#91514=CARTESIAN_POINT ( 'NONE',  ( 189.9056560155743796, 284.8180517316223472, 17.31073399879909047 ) ) ;
#91515=CARTESIAN_POINT ( 'NONE',  ( 167.9520823679746684, 278.2100738273422280, 14.36288932855387657 ) ) ;
#91516=CARTESIAN_POINT ( 'NONE',  ( 192.5741980485687463, 265.2346019687918215, 7.836594753621663578 ) ) ;
#91517=CARTESIAN_POINT ( 'NONE',  ( 86.71718800452170228, 209.3262482093457493, 3.021315404115420679E-15 ) ) ;
#91518=CARTESIAN_POINT ( 'NONE',  ( 164.6063343576543048, 274.4739709976624908, 16.17759516952312637 ) ) ;
#91521=EDGE_CURVE ( 'NONE', #983, #11813, #20918, .T. ) ;
#91522=CARTESIAN_POINT ( 'NONE',  ( 183.8277868541691191, 269.1745150400024045, 15.18432627555796799 ) ) ;
#91524=CARTESIAN_POINT ( 'NONE',  ( 103.3411068992554362, 218.2202760586659736, -5.415160957724236172E-17 ) ) ;
#91527=CARTESIAN_POINT ( 'NONE',  ( 151.1926529451685326, 268.7736386982768408, 14.30343427984827365 ) ) ;
#91531=CARTESIAN_POINT ( 'NONE',  ( 201.4530334248365762, 270.8746905162315670, -9.895680216334456603 ) ) ;
#91532=CARTESIAN_POINT ( 'NONE',  ( 198.4344074287054696, 286.9485196940960918, -17.83642855442570152 ) ) ;
#91533=CARTESIAN_POINT ( 'NONE',  ( 149.8302639188106866, 271.5858334631676030, -11.69480209898182110 ) ) ;
#91535=CARTESIAN_POINT ( 'NONE',  ( 192.5284579606305613, 297.1779242397361713, -13.15228012403107272 ) ) ;
#91539=CARTESIAN_POINT ( 'NONE',  ( 157.9225728654248257, 276.1116997103654285, -12.95724163227552239 ) ) ;
#91540=CARTESIAN_POINT ( 'NONE',  ( 147.5851099763508216, 275.0220864107570264, -4.372720440640867956 ) ) ;
#91541=CARTESIAN_POINT ( 'NONE',  ( 149.2923684163597784, 272.0650280510108701, -12.99082738998495756 ) ) ;
#91542=EDGE_LOOP ( 'NONE', ( #2855, #70493, #68380 ) ) ;
#91544=CARTESIAN_POINT ( 'NONE',  ( 198.2414483977475754, 287.2827345394944700, 16.94931984969033678 ) ) ;
#91545=CARTESIAN_POINT ( 'NONE',  ( 176.8917175299031896, 289.5346434493817469, -10.53293604869262978 ) ) ;
#91546=CARTESIAN_POINT ( 'NONE',  ( 172.9204717250658234, 253.1639062637733275, -9.325132519940664722 ) ) ;
#91548=CARTESIAN_POINT ( 'NONE',  ( 152.6615646578087819, 266.2294089801508221, 16.94722993326405813 ) ) ;
#91551=ORIENTED_EDGE ( 'NONE', *, *, #11007, .F. ) ;
#91552=CARTESIAN_POINT ( 'NONE',  ( 165.0109473288163997, 247.9890283962741080, 7.117481719421622444 ) ) ;
#91556=DIRECTION ( 'NONE',  ( -0.8660254037844387076, -0.4999999999999998890, -0.000000000000000000 ) ) ;
#91557=CARTESIAN_POINT ( 'NONE',  ( 193.5421561915196094, 280.4896855936574411, -16.96249572231928937 ) ) ;
#91558=CARTESIAN_POINT ( 'NONE',  ( 193.2629712555779236, 295.9057098940524497, -12.42285136223522635 ) ) ;
#91559=CARTESIAN_POINT ( 'NONE',  ( 200.9812045408918380, 282.5373376992193926, -16.61165062382494284 ) ) ;
#91560=EDGE_CURVE ( 'NONE', #59881, #40710, #50187, .T. ) ;
#91562=CARTESIAN_POINT ( 'NONE',  ( 149.7854447168632817, 277.1467554076948545, 4.663160563959508842 ) ) ;
#91567=ORIENTED_EDGE ( 'NONE', *, *, #74474, .T. ) ;
#91568=CARTESIAN_POINT ( 'NONE',  ( 197.9778315518523755, 286.8276560105644535, 16.94107069242976138 ) ) ;
#91569=CARTESIAN_POINT ( 'NONE',  ( 169.6029602999246606, 269.2276831600792093, 17.52968384675503088 ) ) ;
#91570=CARTESIAN_POINT ( 'NONE',  ( 164.2712161151136172, 246.1209027979328710, 7.276091357954241445 ) ) ;
#91573=CARTESIAN_POINT ( 'NONE',  ( 197.9440596760970834, 272.2187063198555848, -13.59033992601415619 ) ) ;
#91576=CARTESIAN_POINT ( 'NONE',  ( 170.9705878662882412, 287.7050143283094030, -4.597967457045799122 ) ) ;
#91578=CARTESIAN_POINT ( 'NONE',  ( 186.2570902956351233, 286.9438662100191664, -16.14904440706751032 ) ) ;
#91579=CARTESIAN_POINT ( 'NONE',  ( 105.2078667585768557, 240.7369531367911009, -4.594050593750048428 ) ) ;
#91583=CARTESIAN_POINT ( 'NONE',  ( 188.1536819913596048, 273.5597847156771536, 15.70283653734317042 ) ) ;
#91589=CARTESIAN_POINT ( 'NONE',  ( 180.6056823850905744, 294.3695497894205459, -2.098957692436339784 ) ) ;
#91590=CARTESIAN_POINT ( 'NONE',  ( 192.8319655484016835, 296.6522336772339941, 11.62706545001314673 ) ) ;
#91591=CARTESIAN_POINT ( 'NONE',  ( 149.7247407264208618, 272.0633196944937140, -11.44969454563192279 ) ) ;
#91593=VERTEX_POINT ( 'NONE', #46459 ) ;
#91596=ORIENTED_EDGE ( 'NONE', *, *, #50395, .F. ) ;
#91597=CARTESIAN_POINT ( 'NONE',  ( 37.46763966367993248, 203.9860189848785694, -2.679491924311201423 ) ) ;
#91601=FACE_OUTER_BOUND ( 'NONE', #56814, .T. ) ;
#91602=CARTESIAN_POINT ( 'NONE',  ( 175.2682827652102446, 270.4545196086085639, -17.77314019766468078 ) ) ;
#91604=CARTESIAN_POINT ( 'NONE',  ( 198.2102933758524159, 286.2539132522722980, 17.34058952251382735 ) ) ;
#91605=CARTESIAN_POINT ( 'NONE',  ( 159.0114971902875425, 280.6994106969128211, 5.657252936029947499 ) ) ;
#91606=CARTESIAN_POINT ( 'NONE',  ( 200.9812045408918380, 282.5373376992193926, -16.61165062382494284 ) ) ;
#91607=ORIENTED_EDGE ( 'NONE', *, *, #9145, .T. ) ;
#91608=CARTESIAN_POINT ( 'NONE',  ( 58.36827475829091583, 216.0530062829863311, -4.648177544792955347E-16 ) ) ;
#91610=CARTESIAN_POINT ( 'NONE',  ( 190.2591659045147310, 264.3349555848182604, -9.311233699776803263 ) ) ;
#91611=CARTESIAN_POINT ( 'NONE',  ( 192.8229667366133810, 271.0818589901656424, 14.33785869832464499 ) ) ;
#91612=CARTESIAN_POINT ( 'NONE',  ( 189.3508290737234745, 269.3566302321018497, -14.03381184610130994 ) ) ;
#91614=CARTESIAN_POINT ( 'NONE',  ( 151.1237910559533475, 270.8929109891034841, -13.93008610078706688 ) ) ;
#91618=CARTESIAN_POINT ( 'NONE',  ( 191.6801986094837105, 283.7096785499923044, -16.61112168735793659 ) ) ;
#91622=CARTESIAN_POINT ( 'NONE',  ( 65.12704176573704729, 220.6589784336661637, -6.496448406907675876E-16 ) ) ;
#91623=LINE ( 'NONE', #14599, #44336 ) ;
#91624=CARTESIAN_POINT ( 'NONE',  ( 146.9978162861947908, 276.0393089210717790, -5.134868500856280882 ) ) ;
#91626=EDGE_CURVE ( 'NONE', #41192, #86855, #70907, .T. ) ;
#91629=CARTESIAN_POINT ( 'NONE',  ( 207.8718670335145475, 270.6023601641878713, -6.322166851501095586 ) ) ;
#91634=CARTESIAN_POINT ( 'NONE',  ( 192.7686961758011250, 263.9209412561240811, -8.347089341778378468 ) ) ;
#91635=CARTESIAN_POINT ( 'NONE',  ( 163.9801047297222283, 246.6251225080926588, -5.240962994374625872 ) ) ;
#91636=( BOUNDED_CURVE ( )  B_SPLINE_CURVE ( 2, ( #54597, #78440, #47513, #61706, #92658, #62201, #77439, #69813, #93151 ),
 .UNSPECIFIED., .F., .T. ) 
 B_SPLINE_CURVE_WITH_KNOTS ( ( 3, 2, 2, 2, 3 ),
 ( 0.4072580645161290591, 0.4086021505376344343, 0.4112903225806451846, 0.4139784946236559349, 0.4153225806451613100 ),
 .UNSPECIFIED. ) 
 CURVE ( )  GEOMETRIC_REPRESENTATION_ITEM ( )  RATIONAL_B_SPLINE_CURVE ( ( 0.9330127018922194093, 0.9330127018922207416, 1.000000000000000000, 0.8660254037844387076, 1.000000000000000000, 0.8660254037844387076, 1.000000000000000000, 0.9330127018922194093, 0.9330127018922194093 ) ) 
 REPRESENTATION_ITEM ( '' )  );
#91640=CARTESIAN_POINT ( 'NONE',  ( 48.80796233711527776, 208.1744531367911293, 4.594050593750047540 ) ) ;
#91641=CARTESIAN_POINT ( 'NONE',  ( 157.3363371328520088, 258.1324655395517311, 18.24585617226787093 ) ) ;
#91642=CARTESIAN_POINT ( 'NONE',  ( 199.5508424383191368, 277.6004065077516429, 15.20186197903527336 ) ) ;
#91644=CARTESIAN_POINT ( 'NONE',  ( 142.0139464194155039, 261.9869531367911009, 4.594050593750046652 ) ) ;
#91645=CARTESIAN_POINT ( 'NONE',  ( 46.56179571999064137, 203.8149278399160949, -9.188101187500095079 ) ) ;
#91648=CARTESIAN_POINT ( 'NONE',  ( 171.3409795094679566, 286.6460634318879102, 7.397566566911762287 ) ) ;
#91649=CARTESIAN_POINT ( 'NONE',  ( 149.6890529486499872, 271.3779502865075983, -12.51465682618088593 ) ) ;
#91651=CARTESIAN_POINT ( 'NONE',  ( 204.6235849755581455, 276.2285497258825444, -13.59355699282649432 ) ) ;
#91655=CARTESIAN_POINT ( 'NONE',  ( 169.5727729373952002, 284.0798650663272156, -11.84966624384599676 ) ) ;
#91657=CARTESIAN_POINT ( 'NONE',  ( 152.8305949863981255, 276.5798620968483306, 7.183986870886582388 ) ) ;
#91658=AXIS2_PLACEMENT_3D ( 'NONE', #97861, #42139, #58335 ) ;
#91659=DIRECTION ( 'NONE',  ( -0.8660254037844387076, -0.4999999999999998890, -0.000000000000000000 ) ) ;
#91661=CARTESIAN_POINT ( 'NONE',  ( 94.49106271034210636, 235.3615022471903160, 5.000000000000046185 ) ) ;
#91662=CARTESIAN_POINT ( 'NONE',  ( 200.2690241097007799, 283.7708703901988656, 16.96680019208369927 ) ) ;
#91663=CARTESIAN_POINT ( 'NONE',  ( 165.2675333416819683, 269.7192504327577467, -16.28158008568958692 ) ) ;
#91665=CARTESIAN_POINT ( 'NONE',  ( 67.02199298016300588, 203.3768266524159856, -9.188101187500091527 ) ) ;
#91667=CARTESIAN_POINT ( 'NONE',  ( 164.9673962408295722, 264.6939453157682465, 16.63392279346217606 ) ) ;
#91668=CARTESIAN_POINT ( 'NONE',  ( 190.1696443193688708, 301.2635093119881162, -4.804312979389741223 ) ) ;
#91669=CARTESIAN_POINT ( 'NONE',  ( 186.6728043966838868, 269.6571610938119079, 16.06727167421729163 ) ) ;
#91674=CARTESIAN_POINT ( 'NONE',  ( 194.1972774922283236, 294.2874440223457100, -15.09915398317898649 ) ) ;
#91676=CYLINDRICAL_SURFACE ( 'NONE', #62829, 17.82106496071139645 ) ;
#91677=EDGE_CURVE ( 'NONE', #25284, #84360, #57754, .T. ) ;
#91678=CARTESIAN_POINT ( 'NONE',  ( 157.4843645388753544, 257.8760745514064183, 17.70049730742206862 ) ) ;
#91681=CARTESIAN_POINT ( 'NONE',  ( 175.2052744318867497, 254.7077291441659952, 7.835194671154784629 ) ) ;
#91683=VERTEX_POINT ( 'NONE', #23165 ) ;
#91685=CARTESIAN_POINT ( 'NONE',  ( 159.8188415394622268, 253.8326417772889840, -15.43862849427313222 ) ) ;
#91689=CARTESIAN_POINT ( 'NONE',  ( 159.4254556662896221, 282.2729508943065184, -3.240908821865370992 ) ) ;
#91691=CARTESIAN_POINT ( 'NONE',  ( 208.1912724900461740, 270.0491336852600170, -0.9856800448607289100 ) ) ;
#91693=CARTESIAN_POINT ( 'NONE',  ( 159.8655504377736918, 253.7517395922482706, 15.51368179719542262 ) ) ;
#91694=CARTESIAN_POINT ( 'NONE',  ( 164.5141650773065862, 265.0320900047184978, -16.63006306576538762 ) ) ;
#91695=ADVANCED_FACE ( 'NONE', ( #85534 ), #15066, .T. ) ;
#91696=CARTESIAN_POINT ( 'NONE',  ( 127.4269177983626236, 250.5024278399160949, -9.188101187500093303 ) ) ;
#91697=CARTESIAN_POINT ( 'NONE',  ( 203.1072020527783479, 267.8656079271395924, 2.549640738347975333 ) ) ;
#91698=CARTESIAN_POINT ( 'NONE',  ( 178.7125369615259558, 257.8607718938011431, 9.903824436443219525 ) ) ;
#91699=CARTESIAN_POINT ( 'NONE',  ( 71.86588871287597158, 221.4869531367911293, 4.594050593750046652 ) ) ;
#91701=CARTESIAN_POINT ( 'NONE',  ( 173.9684503405311204, 265.6129390675949367, 16.27754927923930950 ) ) ;
#91703=DIRECTION ( 'NONE',  ( 0.8660254037844395958, 0.4999999999999985567, 0.000000000000000000 ) ) ;
#91711=CARTESIAN_POINT ( 'NONE',  ( 197.7287339728600841, 286.7199927125528234, 16.92603034138073426 ) ) ;
#91713=CARTESIAN_POINT ( 'NONE',  ( 191.0862225170008628, 299.6759493045793192, -9.402218231374108726 ) ) ;
#91714=B_SPLINE_SURFACE_WITH_KNOTS ( 'NONE', 3, 1, ( 
 ( #28653, #59535 ),
 ( #51963, #90002 ),
 ( #88532, #34757 ),
 ( #90515, #19093 ),
 ( #12484, #20577 ),
 ( #51457, #82424 ),
 ( #12989, #82904 ),
 ( #21087, #3395 ),
 ( #13476, #65657 ),
 ( #96615, #58066 ),
 ( #27178, #42838 ),
 ( #19599, #99564 ),
 ( #76274, #92974 ),
 ( #7341, #68147 ),
 ( #98586, #13962 ),
 ( #6848, #91486 ),
 ( #77249, #100069 ),
 ( #44841, #60533 ),
 ( #21565, #67655 ),
 ( #6364, #75777 ),
 ( #84388, #22049 ),
 ( #7856, #37248 ),
 ( #30147, #52448 ),
 ( #38224, #61032 ),
 ( #69642, #37734 ),
 ( #29169, #60037 ),
 ( #22552, #52949 ),
 ( #14461, #31130 ),
 ( #99073, #76748 ),
 ( #45343, #83898 ),
 ( #68643, #15942 ),
 ( #61540, #91002 ),
 ( #38736, #29655 ),
 ( #75278, #83393 ) ),
 .UNSPECIFIED., .T., .F., .F.,
 ( 4, 2, 2, 2, 2, 2, 2, 2, 2, 2, 2, 2, 2, 2, 2, 2, 4 ),
 ( 2, 2 ),
 ( 0.000000000000000000, 0.06250000000000000000, 0.1250000000000000000, 0.1875000000000000000, 0.2500000000000000000, 0.3125000000000000000, 0.3750000000000000000, 0.4375000000000000000, 0.5000000000000000000, 0.5625000000000000000, 0.6250000000000000000, 0.6875000000000000000, 0.7500000000000000000, 0.8125000000000000000, 0.8750000000000000000, 0.9375000000000000000, 1.000000000000000000 ),
 ( 0.000000000000000000, 1.000000000000000000 ),
 .UNSPECIFIED. ) ;
#91723=CARTESIAN_POINT ( 'NONE',  ( 183.6471037257901173, 275.7322458396929505, 17.25674916785948909 ) ) ;
#91724=CARTESIAN_POINT ( 'NONE',  ( 206.2456893945931142, 273.4189824569319285, 10.13882547285618152 ) ) ;
#91725=CARTESIAN_POINT ( 'NONE',  ( 148.9194629746633893, 272.7109192224475009, -12.27648025871169679 ) ) ;
#91726=CARTESIAN_POINT ( 'NONE',  ( 42.09652578138359047, 195.1115022471902591, 10.00000000000009592 ) ) ;
#91728=CARTESIAN_POINT ( 'NONE',  ( 134.1114646098825176, 257.4244531367911577, -4.594050593750046652 ) ) ;
#91733=EDGE_CURVE ( 'NONE', #74751, #73620, #61774, .T. ) ;
#91735=CARTESIAN_POINT ( 'NONE',  ( 152.9607371460978129, 265.7112270302071124, -16.17698032818104537 ) ) ;
#91739=CARTESIAN_POINT ( 'NONE',  ( 195.8065633768937914, 265.4443555257707885, 4.436325927742740483 ) ) ;
#91742=CARTESIAN_POINT ( 'NONE',  ( 184.7196529705373393, 263.5678720036872278, -12.47054388087118681 ) ) ;
#91743=CARTESIAN_POINT ( 'NONE',  ( 198.9902718401575044, 266.4967149787970584, 0.8259339281635468266 ) ) ;
#91744=CARTESIAN_POINT ( 'NONE',  ( 198.8214910967091669, 265.6694977507734734, 0.07193098711981385507 ) ) ;
#91745=EDGE_CURVE ( 'NONE', #63141, #90758, #39209, .T. ) ;
#91747=CARTESIAN_POINT ( 'NONE',  ( 190.7403173041394950, 300.2750747078583800, -4.254144485856557800 ) ) ;
#91748=CARTESIAN_POINT ( 'NONE',  ( 183.1289407222409693, 280.7186293386456555, 16.57674227110009113 ) ) ;
#91750=CARTESIAN_POINT ( 'NONE',  ( 177.2629247679169850, 264.4881137859267710, -15.48121825248645500 ) ) ;
#91751=CARTESIAN_POINT ( 'NONE',  ( 192.8158590921061943, 268.4179402270660830, 12.40538664778730826 ) ) ;
#91754=CARTESIAN_POINT ( 'NONE',  ( 78.37938175722123901, 209.3927522451418213, -10.00000000000009237 ) ) ;
#91757=CARTESIAN_POINT ( 'NONE',  ( -11.73236572436687730, 164.0333772461660544, 9.188101187500095079 ) ) ;
#91762=CARTESIAN_POINT ( 'NONE',  ( 151.3999564459286375, 268.4145785023736153, -15.40574304386609050 ) ) ;
#91763=CARTESIAN_POINT ( 'NONE',  ( 0.1751364819041374699, 183.1589784336661353, -6.496448406907676862E-16 ) ) ;
#91765=CARTESIAN_POINT ( 'NONE',  ( 172.1128792045810201, 290.3147750570036010, 2.746125360738576937 ) ) ;
#91766=CARTESIAN_POINT ( 'NONE',  ( 180.4252347176669389, 274.7960680257757531, -16.49030086573319309 ) ) ;
#91769=CARTESIAN_POINT ( 'NONE',  ( 170.3679664779006373, 270.9046122409516215, -17.49121570188935593 ) ) ;
#91772=CARTESIAN_POINT ( 'NONE',  ( 150.1492354317374236, 276.5066157258622752, 3.807244489742962035 ) ) ;
#91773=CARTESIAN_POINT ( 'NONE',  ( 177.8716437711887863, 254.8016637181727617, -3.895127477326730148 ) ) ;
#91774=CARTESIAN_POINT ( 'NONE',  ( 191.0543065984834925, 261.4893840380978531, -1.560471719009105973 ) ) ;
#91775=AXIS2_PLACEMENT_3D ( 'NONE', #92617, #86540, #47961 ) ;
#91776=CARTESIAN_POINT ( 'NONE',  ( 182.9811911498659924, 295.6553585014947316, 1.023933121683335390 ) ) ;
#91777=CARTESIAN_POINT ( 'NONE',  ( 58.91185237153150211, 191.4865022471901455, 1.119607411625061291E-15 ) ) ;
#91779=CARTESIAN_POINT ( 'NONE',  ( 147.9710862514405960, 274.3535558917855042, 7.785500222159708272 ) ) ;
#91780=CARTESIAN_POINT ( 'NONE',  ( 20.41882739113040302, 182.5958772461660544, -9.188101187500095079 ) ) ;
#91785=CARTESIAN_POINT ( 'NONE',  ( 164.9404048476745004, 244.9618339132846074, -2.801285734921658666 ) ) ;
#91786=CARTESIAN_POINT ( 'NONE',  ( 185.2395268517200293, 266.6953418153134407, 13.39566909832231723 ) ) ;
#91788=CARTESIAN_POINT ( 'NONE',  ( 164.0173503523412251, 281.8225298789022872, 9.954678856299715051 ) ) ;
#91791=CARTESIAN_POINT ( 'NONE',  ( 147.6220714307702622, 274.9580672937808572, 8.392894244419288441 ) ) ;
#91793=ADVANCED_FACE ( 'NONE', ( #63677 ), #79427, .T. ) ;
#91794=CARTESIAN_POINT ( 'NONE',  ( 155.5888570658010508, 261.1591898008976500, 17.34682632352454945 ) ) ;
#91796=VECTOR ( 'NONE', #23481, 1000.000000000000000 ) ;
#91797=CARTESIAN_POINT ( 'NONE',  ( 185.4839599128850693, 290.9053401448446152, 12.29227739265569674 ) ) ;
#91803=EDGE_LOOP ( 'NONE', ( #17212, #82598, #87517, #59393 ) ) ;
#91807=CARTESIAN_POINT ( 'NONE',  ( 202.8535267948003593, 279.2943804273081696, -15.36804658072946062 ) ) ;
#91810=CIRCLE ( 'NONE', #67545, 17.82106496071138224 ) ;
#91815=CARTESIAN_POINT ( 'NONE',  ( 153.4542976351440302, 264.8563551865710224, -17.11782692037292009 ) ) ;
#91818=CARTESIAN_POINT ( 'NONE',  ( 159.0906380018002153, 259.2649656523443582, -17.57712761084927067 ) ) ;
#91821=CARTESIAN_POINT ( 'NONE',  ( 190.0515794655415789, 301.4680036374047063, -1.296825456579539626 ) ) ;
#91822=CARTESIAN_POINT ( 'NONE',  ( 149.3801359649374092, 271.9130101976182914, -11.41245530317637424 ) ) ;
#91824=CARTESIAN_POINT ( 'NONE',  ( 205.8610808625997208, 274.0851439753691920, 10.38803237360972531 ) ) ;
#91827=CARTESIAN_POINT ( 'NONE',  ( 190.7222376050763444, 300.3063896652212179, 3.365789908110941475 ) ) ;
#91831=ADVANCED_FACE ( 'NONE', ( #27890 ), #80766, .F. ) ;
#91834=CARTESIAN_POINT ( 'NONE',  ( 185.9406580756425171, 265.4572926502605128, 14.02042132963198817 ) ) ;
#91837=CARTESIAN_POINT ( 'NONE',  ( 156.4389512583130681, 266.4418172495878139, -16.23539328966390727 ) ) ;
#91841=CARTESIAN_POINT ( 'NONE',  ( 149.6676065383367416, 271.4150965588098074, 11.80358707172367261 ) ) ;
#91842=CARTESIAN_POINT ( 'NONE',  ( 170.8444319527499999, 275.3490660935767096, -16.15441094210034478 ) ) ;
#91843=B_SPLINE_CURVE_WITH_KNOTS ( 'NONE', 3,
 ( #38744, #38233, #46332, #1263 ),
 .UNSPECIFIED., .F., .F.,
 ( 4, 4 ),
 ( 0.04153493918636062820, 0.04887066958154935581 ),
 .UNSPECIFIED. ) ;
#91844=CARTESIAN_POINT ( 'NONE',  ( 191.3733179707528791, 299.1786853920590374, 9.861994297794856479 ) ) ;
#91845=CARTESIAN_POINT ( 'NONE',  ( 147.2937583206075942, 275.5267222813735088, 0.1877253132609109920 ) ) ;
#91846=CARTESIAN_POINT ( 'NONE',  ( 163.4180467003458261, 257.8218550979400447, 15.55521868025378218 ) ) ;
#91850=CARTESIAN_POINT ( 'NONE',  ( 149.6564118588553924, 271.4344863124460971, -11.76165597393390172 ) ) ;
#91851=CARTESIAN_POINT ( 'NONE',  ( -13.51183432020139819, 142.4280072687214442, 0.000000000000000000 ) ) ;
#91853=CARTESIAN_POINT ( 'NONE',  ( 168.1067394590192521, 286.6168014624556122, 3.602430751267735598 ) ) ;
#91857=CARTESIAN_POINT ( 'NONE',  ( 190.4558984197548170, 300.7677026662446451, -4.819771570275049655 ) ) ;
#91861=CARTESIAN_POINT ( 'NONE',  ( 203.0126454322200402, 278.3859261051122189, 14.97126004913892139 ) ) ;
#91863=CARTESIAN_POINT ( 'NONE',  ( 191.5873934714740301, 298.0279652477457262, -9.452854836254962478 ) ) ;
#91864=CARTESIAN_POINT ( 'NONE',  ( 189.8449610424057425, 301.8258772440559028, -0.9803210874536477659 ) ) ;
#91865=CARTESIAN_POINT ( 'NONE',  ( 166.2025478939213770, 283.6845846615859159, -8.127517485801055486 ) ) ;
#91867=CARTESIAN_POINT ( 'NONE',  ( 162.7070706717508699, 248.8300821762643693, -9.986337079333621247 ) ) ;
#91872=CARTESIAN_POINT ( 'NONE',  ( 45.83126033165611091, 187.2677522451417929, -5.000000000000041744 ) ) ;
#91873=CARTESIAN_POINT ( 'NONE',  ( 116.0331843058823296, 246.9869531367911293, 4.594050593750046652 ) ) ;
#91874=CARTESIAN_POINT ( 'NONE',  ( 199.2205425252482200, 285.5868937652708155, -18.05012564782189344 ) ) ;
#91878=CARTESIAN_POINT ( 'NONE',  ( 157.8562613713738472, 257.2319303423452652, 17.81420683562559404 ) ) ;
#91879=CARTESIAN_POINT ( 'NONE',  ( 172.8923325490025036, 251.6825938466021455, -3.947792175603512810 ) ) ;
#91880=CARTESIAN_POINT ( 'NONE',  ( 33.40920844789697952, 190.0958772461660544, -9.188101187500095079 ) ) ;
#91881=CARTESIAN_POINT ( 'NONE',  ( 147.8527080755910958, 276.5585929068648170, -2.411454450074328903 ) ) ;
#91883=FACE_OUTER_BOUND ( 'NONE', #49460, .T. ) ;
#91884=EDGE_CURVE ( 'NONE', #9692, #45778, #95764, .T. ) ;
#91888=CARTESIAN_POINT ( 'NONE',  ( 147.5498377207569263, 275.0831797495432056, 4.097967709737811326 ) ) ;
#91890=FACE_OUTER_BOUND ( 'NONE', #69515, .T. ) ;
#91893=CARTESIAN_POINT ( 'NONE',  ( 110.7831656154890254, 224.7677522451417929, -5.000000000000041744 ) ) ;
#91894=CARTESIAN_POINT ( 'NONE',  ( 194.3452430042056847, 293.4673175397701357, -14.50972866970454866 ) ) ;
#91895=ORIENTED_EDGE ( 'NONE', *, *, #21395, .T. ) ;
#91896=FACE_OUTER_BOUND ( 'NONE', #47240, .T. ) ;
#91898=CARTESIAN_POINT ( 'NONE',  ( 15.70964071017000663, 186.0024278399160949, -9.188101187500093303 ) ) ;
#91900=CARTESIAN_POINT ( 'NONE',  ( 196.2097543372840391, 273.6352822109456611, 15.01336023606802783 ) ) ;
#91903=CARTESIAN_POINT ( 'NONE',  ( 175.1643429085319497, 286.5391626044407190, 10.49485163562685663 ) ) ;
#91904=CARTESIAN_POINT ( 'NONE',  ( 72.54290492928882372, 206.5643266524159571, -9.188101187500093303 ) ) ;
#91905=CYLINDRICAL_SURFACE ( 'NONE', #60290, 10.00000000000010658 ) ;
#91910=ORIENTED_EDGE ( 'NONE', *, *, #67686, .T. ) ;
#91911=CARTESIAN_POINT ( 'NONE',  ( 18.28082717731156848, 171.3615022471901739, 5.000000000000051514 ) ) ;
#91912=CARTESIAN_POINT ( 'NONE',  ( 164.4698008747318738, 245.7769439046653019, -6.272955660526681854 ) ) ;
#91914=CARTESIAN_POINT ( 'NONE',  ( 136.0871718362070339, 255.5024278399161233, 9.188101187500095079 ) ) ;
#91916=CARTESIAN_POINT ( 'NONE',  ( 167.7336762235300682, 262.4260227015225269, -16.94079744808321664 ) ) ;
#91918=CARTESIAN_POINT ( 'NONE',  ( 198.4753670019441643, 282.2770161063888281, -17.61508457932132288 ) ) ;
#91923=CARTESIAN_POINT ( 'NONE',  ( 60.12067949409930634, 205.5177522451418497, -10.00000000000009592 ) ) ;
#91924=DIRECTION ( 'NONE',  ( 0.000000000000000000, 0.000000000000000000, 1.000000000000000000 ) ) ;
#91926=CARTESIAN_POINT ( 'NONE',  ( 181.2434141109869756, 287.9121743413131185, 13.99700062213659280 ) ) ;
#91927=CARTESIAN_POINT ( 'NONE',  ( 156.6019793714546893, 280.4068591911544672, -5.433895450329538690 ) ) ;
#91928=CARTESIAN_POINT ( 'NONE',  ( -17.42236680055705023, 149.2012482093457777, 0.000000000000000000 ) ) ;
#91930=CARTESIAN_POINT ( 'NONE',  ( 160.1554125499368411, 253.2496836867922809, 14.66957084865053140 ) ) ;
#91933=CARTESIAN_POINT ( 'NONE',  ( 168.0402147318401944, 281.8818710449446598, -11.04375926519547768 ) ) ;
#91934=B_SPLINE_CURVE_WITH_KNOTS ( 'NONE', 3,
 ( #87908, #60269, #4743, #34144, #3749, #2759, #18451, #56919, #41722, #26547, #34626, #35121, #96475, #89392, #11849, #91223, #27044, #57925, #50324, #66032, #35627, #81276, #73639, #4222, #21791, #19943, #81767, #54162, #38473, #93731, #8097, #47081, #70383, #31871, #24290, #490, #85124, #99309, #84143, #84625, #62773, #22288, #37473, #6599, #46066, #990, #69385, #91723, #92723, #77505, #30888, #55167 ),
 .UNSPECIFIED., .F., .F.,
 ( 4, 2, 2, 2, 2, 2, 2, 2, 2, 2, 2, 2, 2, 2, 2, 2, 2, 2, 2, 2, 2, 2, 2, 2, 2, 4 ),
 ( 0.0002653169772839772465, 0.0007391932915139334034, 0.001213069605743889723, 0.001450007762858867774, 0.001568476841416391711, 0.001686945919973915865, 0.001805414998531439802, 0.001923884077088963739, 0.002160822234204006192, 0.002634698548434018673, 0.003108574862664031588, 0.004056327491123986294, 0.005004080119583941000, 0.005477956433813918787, 0.005714894590928907246, 0.005833363669486404078, 0.005892598208765155096, 0.005951832748043906114, 0.006011067287322656265, 0.006070301826601406416, 0.006188770905158779215, 0.006425709062273484047, 0.006899585376502746260, 0.007136523533617395582, 0.007373461690732044035, 0.007847338004961328800 ),
 .UNSPECIFIED. ) ;
#91938=CARTESIAN_POINT ( 'NONE',  ( 89.99855592466239784, 232.7677522451419065, -5.000000000000047962 ) ) ;
#91939=CARTESIAN_POINT ( 'NONE',  ( 207.9328781051891042, 270.4966858882232259, -0.8820402142964423042 ) ) ;
#91940=CARTESIAN_POINT ( 'NONE',  ( 153.3939648708017387, 264.9608545997728015, -16.49556533540763681 ) ) ;
#91942=( BOUNDED_CURVE ( )  B_SPLINE_CURVE ( 2, ( #65867, #82634, #26888, #19314, #97307, #59243, #96825, #4076, #36463 ),
 .UNSPECIFIED., .F., .T. ) 
 B_SPLINE_CURVE_WITH_KNOTS ( ( 3, 2, 2, 2, 3 ),
 ( 0.2701612903225806273, 0.2715053763440860024, 0.2741935483870967527, 0.2768817204301075030, 0.2782258064516128782 ),
 .UNSPECIFIED. ) 
 CURVE ( )  GEOMETRIC_REPRESENTATION_ITEM ( )  RATIONAL_B_SPLINE_CURVE ( ( 0.9330127018922194093, 0.9330127018922194093, 1.000000000000000000, 0.8660254037844387076, 1.000000000000000000, 0.8660254037844387076, 1.000000000000000000, 0.9330127018922194093, 0.9330127018922194093 ) ) 
 REPRESENTATION_ITEM ( '' )  );
#91947=CARTESIAN_POINT ( 'NONE',  ( 149.5633513747893346, 271.5956717990251832, 12.83777201928511325 ) ) ;
#91951=EDGE_CURVE ( 'NONE', #29135, #22165, #98053, .T. ) ;
#91952=CARTESIAN_POINT ( 'NONE',  ( 147.2180753513904961, 275.6578090293250511, 0.4909717733184589261 ) ) ;
#91955=CARTESIAN_POINT ( 'NONE',  ( 164.4936379324916516, 245.7356569095223051, 6.719479797016231437 ) ) ;
#91958=VERTEX_POINT ( 'NONE', #24649 ) ;
#91959=CARTESIAN_POINT ( 'NONE',  ( 95.14032143958276322, 234.9244531367911009, -4.594050593750046652 ) ) ;
#91960=CARTESIAN_POINT ( 'NONE',  ( 155.7926064421430112, 260.8062855290629045, 17.74927770606829469 ) ) ;
#91966=ORIENTED_EDGE ( 'NONE', *, *, #75286, .F. ) ;
#91967=EDGE_CURVE ( 'NONE', #10047, #8803, #35250, .T. ) ;
#91972=VERTEX_POINT ( 'NONE', #11487 ) ;
#91973=CARTESIAN_POINT ( 'NONE',  ( 164.0179800784044915, 246.5595204798204065, -5.772998092557310557 ) ) ;
#91976=CARTESIAN_POINT ( 'NONE',  ( 192.3926678149021825, 295.4131196713046847, -13.42882169270698256 ) ) ;
#91977=CARTESIAN_POINT ( 'NONE',  ( 17.48697055717582316, 174.2365022471902023, -10.00000000000009237 ) ) ;
#91979=B_SPLINE_CURVE_WITH_KNOTS ( 'NONE', 3,
 ( #56807, #96860, #18334, #65903, #49228, #88277 ),
 .UNSPECIFIED., .F., .F.,
 ( 4, 2, 4 ),
 ( 0.02208471075069790360, 0.02668293858277623332, 0.03128116641485456650 ),
 .UNSPECIFIED. ) ;
#91982=CARTESIAN_POINT ( 'NONE',  ( 163.4341025207368716, 282.8476932499685859, 9.116081536633066307 ) ) ;
#91983=FACE_OUTER_BOUND ( 'NONE', #36312, .T. ) ;
#91986=ADVANCED_FACE ( 'NONE', ( #66649 ), #3386, .T. ) ;
#91987=CARTESIAN_POINT ( 'NONE',  ( 163.4004183463084416, 247.6291687766210146, 10.19167732382099345 ) ) ;
#91988=CARTESIAN_POINT ( 'NONE',  ( 187.5027153640760105, 260.3852002302687083, 2.859512323897527963 ) ) ;
#91991=CARTESIAN_POINT ( 'NONE',  ( 171.7256454430782924, 255.0603003222375378, 10.96627809234114359 ) ) ;
#91992=CARTESIAN_POINT ( 'NONE',  ( 158.8074424692007938, 281.4784585291520784, 2.074645808957411575 ) ) ;
#91995=EDGE_CURVE ( 'NONE', #130, #61735, #36486, .T. ) ;
#91999=CARTESIAN_POINT ( 'NONE',  ( -1.439292958244568821, 176.6427522451419065, 10.00000000000009237 ) ) ;
#92003=CARTESIAN_POINT ( 'NONE',  ( 174.9330555342984610, 281.7317282589606862, -14.07090496212465069 ) ) ;
#92004=CARTESIAN_POINT ( 'NONE',  ( 193.8848781386269309, 267.1185884883711879, -11.59377028749509364 ) ) ;
#92006=CIRCLE ( 'NONE', #90341, 2.471954595299370006 ) ;
#92007=CARTESIAN_POINT ( 'NONE',  ( 162.2842013956643825, 250.7983415291583071, -12.77801933371535448 ) ) ;
#92008=CARTESIAN_POINT ( 'NONE',  ( 0.5816933075168655431, 161.9548013555410080, -4.594050593750042211 ) ) ;
#92010=CARTESIAN_POINT ( 'NONE',  ( 16.79905537663784898, 192.0530062829863311, -4.648177544792955347E-16 ) ) ;
#92011=ORIENTED_EDGE ( 'NONE', *, *, #64033, .F. ) ;
#92016=FACE_OUTER_BOUND ( 'NONE', #8928, .T. ) ;
#92017=CARTESIAN_POINT ( 'NONE',  ( 152.7122812589697958, 277.9324518551267147, 6.933031942251369983 ) ) ;
#92019=CARTESIAN_POINT ( 'NONE',  ( 162.9923277572749214, 248.3360024109179847, -11.73806682979623695 ) ) ;
#92021=CARTESIAN_POINT ( 'NONE',  ( 153.4490520802545177, 279.2845403698434552, 3.866127127660768714 ) ) ;
#92022=CARTESIAN_POINT ( 'NONE',  ( 20.90579313287664220, 189.0024278399160949, -9.188101187500093303 ) ) ;
#92023=CARTESIAN_POINT ( 'NONE',  ( 119.6601863278771845, 230.7048013555409796, 4.594050593750051981 ) ) ;
#92024=CARTESIAN_POINT ( 'NONE',  ( 179.8548388294205438, 292.4099480123907142, -6.160154682680708760 ) ) ;
#92025=CARTESIAN_POINT ( 'NONE',  ( 170.4037115821164434, 284.7129311807937029, 11.70618658742957940 ) ) ;
#92026=CARTESIAN_POINT ( 'NONE',  ( 149.9807464961409664, 271.6463072190915682, -11.70746914540981010 ) ) ;
#92027=CARTESIAN_POINT ( 'NONE',  ( 178.3812519316271903, 283.9015146232569009, -15.02767978356603962 ) ) ;
#92029=FACE_OUTER_BOUND ( 'NONE', #27329, .T. ) ;
#92030=CARTESIAN_POINT ( 'NONE',  ( 154.9455285025717615, 262.2734675583710100, 18.28470720339922551 ) ) ;
#92031=CARTESIAN_POINT ( 'NONE',  ( 184.2649791758939273, 274.6463348420198258, 16.49567768463042583 ) ) ;
#92032=CARTESIAN_POINT ( 'NONE',  ( 190.1045438606958271, 284.8339252823208199, 16.91879847483513188 ) ) ;
#92033=CARTESIAN_POINT ( 'NONE',  ( 167.8099627665611706, 278.1935700092135448, 14.45340646069998947 ) ) ;
#92034=CARTESIAN_POINT ( 'NONE',  ( 196.5944846034172713, 266.5326877703075752, 8.237093742074783620 ) ) ;
#92037=CARTESIAN_POINT ( 'NONE',  ( 162.8014500637598871, 250.9066623883947216, -12.97690139725125746 ) ) ;
#92039=CARTESIAN_POINT ( 'NONE',  ( 164.0771906360838273, 283.2204635009451863, -9.130928687893741014 ) ) ;
#92040=CARTESIAN_POINT ( 'NONE',  ( 207.5195222358739784, 271.2126392554839640, 2.810970398613041432 ) ) ;
#92041=CARTESIAN_POINT ( 'NONE',  ( 181.3746470502182149, 267.9051538131957955, 15.02264890925958696 ) ) ;
#92042=EDGE_CURVE ( 'NONE', #46359, #98253, #4355, .T. ) ;
#92043=CARTESIAN_POINT ( 'NONE',  ( 102.5829875751790468, 230.0333772461660828, 9.188101187500095079 ) ) ;
#92045=B_SPLINE_CURVE_WITH_KNOTS ( 'NONE', 3,
 ( #15056, #69764, #78387, #54541 ),
 .UNSPECIFIED., .F., .F.,
 ( 4, 4 ),
 ( 0.02560006208908528064, 0.03484442351368802898 ),
 .UNSPECIFIED. ) ;
#92046=CARTESIAN_POINT ( 'NONE',  ( 151.0036289208911171, 269.1010379121764799, 14.24595189915657478 ) ) ;
#92048=CARTESIAN_POINT ( 'NONE',  ( 143.3312870410541677, 246.8927522451417929, -10.00000000000009237 ) ) ;
#92049=CARTESIAN_POINT ( 'NONE',  ( 105.0818317072414061, 238.1427522451419065, 10.00000000000009415 ) ) ;
#92050=CARTESIAN_POINT ( 'NONE',  ( 149.3318355652811817, 271.9966689438488743, 13.09533505091524397 ) ) ;
#92051=CARTESIAN_POINT ( 'NONE',  ( 198.5201458116119397, 286.8000164587433005, -18.30276554821096013 ) ) ;
#92055=DIRECTION ( 'NONE',  ( 0.4999999999999998890, -0.8660254037844385966, 0.000000000000000000 ) ) ;
#92056=VERTEX_POINT ( 'NONE', #3862 ) ;
#92059=CARTESIAN_POINT ( 'NONE',  ( 147.2089949622447875, 275.6735367246781720, -3.633014386235353221 ) ) ;
#92060=CARTESIAN_POINT ( 'NONE',  ( 149.1939152435731728, 272.2355539484436235, -11.44223522189843933 ) ) ;
#92061=VERTEX_POINT ( 'NONE', #5357 ) ;
#92064=CARTESIAN_POINT ( 'NONE',  ( 183.5859071331518351, 264.2830035368942276, -13.62284648814853050 ) ) ;
#92065=CARTESIAN_POINT ( 'NONE',  ( 169.3267103143955410, 252.0916492433576934, -8.716375534122970947 ) ) ;
#92067=CARTESIAN_POINT ( 'NONE',  ( 152.9262073036446168, 265.7710344717137900, 16.19159804214501008 ) ) ;
#92069=CARTESIAN_POINT ( 'NONE',  ( 187.1950062442360831, 278.7691670715128112, 17.33431566565705495 ) ) ;
#92072=ORIENTED_EDGE ( 'NONE', *, *, #61818, .F. ) ;
#92073=CARTESIAN_POINT ( 'NONE',  ( 167.8000401002150568, 249.6086421576515306, 6.575756818014385274 ) ) ;
#92074=DIRECTION ( 'NONE',  ( 0.4999999999999992784, -0.8660254037844390407, 0.000000000000000000 ) ) ;
#92075=ORIENTED_EDGE ( 'NONE', *, *, #14721, .F. ) ;
#92076=EDGE_CURVE ( 'NONE', #87476, #93085, #56937, .T. ) ;
#92079=CARTESIAN_POINT ( 'NONE',  ( 206.0571735407143592, 273.7455014938826707, 12.27159782092593332 ) ) ;
#92080=CARTESIAN_POINT ( 'NONE',  ( 190.8789531733649483, 278.0110512791312090, -17.17207137177770448 ) ) ;
#92081=CARTESIAN_POINT ( 'NONE',  ( 153.9709862450691560, 263.9614242624880376, -16.70428749416571890 ) ) ;
#92082=CARTESIAN_POINT ( 'NONE',  ( 201.0356089830534643, 282.4431064412383989, -18.18835788025466371 ) ) ;
#92087=CARTESIAN_POINT ( 'NONE',  ( 152.3360070569975449, 270.2436951681156643, -14.78697292633622951 ) ) ;
#92089=ORIENTED_EDGE ( 'NONE', *, *, #81003, .T. ) ;
#92090=B_SPLINE_CURVE_WITH_KNOTS ( 'NONE', 3,
 ( #54017, #46939, #835, #9444 ),
 .UNSPECIFIED., .F., .F.,
 ( 4, 4 ),
 ( 0.01228877948971598445, 0.01655137231517712568 ),
 .UNSPECIFIED. ) ;
#92091=CARTESIAN_POINT ( 'NONE',  ( 162.7054358649808705, 249.4575268515429798, 10.87536955962176499 ) ) ;
#92093=ORIENTED_EDGE ( 'NONE', *, *, #11543, .T. ) ;
#92096=CARTESIAN_POINT ( 'NONE',  ( 161.5600482970121163, 274.5147329235393840, 15.37191611340452724 ) ) ;
#92098=CARTESIAN_POINT ( 'NONE',  ( 204.8523313866422484, 275.8323493198358847, 14.65426965484541100 ) ) ;
#92100=CARTESIAN_POINT ( 'NONE',  ( 165.0831640657340529, 244.7145676943567878, -1.661138566959525775 ) ) ;
#92101=CARTESIAN_POINT ( 'NONE',  ( 200.3018037382982470, 274.6393581797076990, -13.69157862092785116 ) ) ;
#92103=CARTESIAN_POINT ( 'NONE',  ( 189.8763472015711216, 301.7715148217271803, -0.1184663095182975079 ) ) ;
#92104=CARTESIAN_POINT ( 'NONE',  ( 171.5969307849138659, 250.8838870372819372, -5.657895903504599922 ) ) ;
#92106=CARTESIAN_POINT ( 'NONE',  ( 178.2870251902395466, 255.0132465080435225, 5.857099106615994089 ) ) ;
#92107=CARTESIAN_POINT ( 'NONE',  ( 114.4640339051705666, 227.7048013555410080, 4.594050593750051981 ) ) ;
#92108=EDGE_LOOP ( 'NONE', ( #20638, #79844, #90511 ) ) ;
#92109=CARTESIAN_POINT ( 'NONE',  ( 185.1790142135946837, 260.5378326486920741, -9.806357480331048038 ) ) ;
#92110=CARTESIAN_POINT ( 'NONE',  ( 161.0764005243388226, 283.8056199075659265, 2.187379043674367196 ) ) ;
#92111=CARTESIAN_POINT ( 'NONE',  ( 187.9439182355510809, 273.9003972453228926, 16.19719593720451911 ) ) ;
#92113=CARTESIAN_POINT ( 'NONE',  ( 162.8594194046838197, 248.9559446593948167, -10.02318146003397636 ) ) ;
#92114=CARTESIAN_POINT ( 'NONE',  ( 180.4686966669306969, 294.6099987018001229, -1.982722432560759973 ) ) ;
#92115=CARTESIAN_POINT ( 'NONE',  ( 192.0571890000333042, 297.9941860235205127, 11.61994745305988275 ) ) ;
#92116=CARTESIAN_POINT ( 'NONE',  ( 206.7408728089182546, 272.5612996242556960, -10.63134519248043475 ) ) ;
#92117=CARTESIAN_POINT ( 'NONE',  ( 92.75901190277325270, 224.3615022471902591, -10.00000000000009592 ) ) ;
#92119=CARTESIAN_POINT ( 'NONE',  ( 195.4838507530383254, 292.0590337669632390, 15.61368894501154259 ) ) ;
#92121=CARTESIAN_POINT ( 'NONE',  ( 51.46042545625488174, 210.5177522451419065, 5.000000000000046185 ) ) ;
#92122=ADVANCED_FACE ( 'NONE', ( #85382 ), #44333, .T. ) ;
#92125=CARTESIAN_POINT ( 'NONE',  ( 188.6360227007297112, 264.9932382472330232, -12.30697744625317291 ) ) ;
#92126=CARTESIAN_POINT ( 'NONE',  ( 195.8318599711807053, 265.1596923740410716, 4.002729224306967204 ) ) ;
#92129=CARTESIAN_POINT ( 'NONE',  ( 184.2754218782066289, 288.8003507295421741, -13.20763826220184178 ) ) ;
#92131=CARTESIAN_POINT ( 'NONE',  ( 201.4617167010348737, 281.7050662241970826, -17.43131506460443703 ) ) ;
#92133=CARTESIAN_POINT ( 'NONE',  ( 190.8957779480239765, 300.0058089740729770, -4.541438514207768229 ) ) ;
#92140=CARTESIAN_POINT ( 'NONE',  ( 196.4164021072083983, 270.5621661862001019, 13.33908636140236936 ) ) ;
#92141=CARTESIAN_POINT ( 'NONE',  ( 194.5051734451974426, 293.7541525883582381, 14.61790433731063921 ) ) ;
#92142=CARTESIAN_POINT ( 'NONE',  ( 34.63963837367094811, 179.2592609112380160, 2.679491924311254714 ) ) ;
#92145=CARTESIAN_POINT ( 'NONE',  ( 77.73871025623044773, 221.8149278399160949, -9.188101187500095079 ) ) ;
#92146=CARTESIAN_POINT ( 'NONE',  ( 159.5895502557670795, 254.2297859303815244, -16.92708575547316485 ) ) ;
#92147=CARTESIAN_POINT ( 'NONE',  ( 192.8301672656986341, 296.6553483942417415, -13.40355799340913556 ) ) ;
#92148=CARTESIAN_POINT ( 'NONE',  ( 163.0056347026689707, 248.3129541054019569, -11.27842346302751508 ) ) ;
#92152=CARTESIAN_POINT ( 'NONE',  ( 207.6357208050208101, 271.0113774299547913, -6.790259683043212036 ) ) ;
#92153=CARTESIAN_POINT ( 'NONE',  ( 194.5758046545716411, 288.3945151952651713, 17.23224542525024816 ) ) ;
#92155=CARTESIAN_POINT ( 'NONE',  ( 188.9516232634142909, 259.5449388965931234, 2.625812016075142807 ) ) ;
#92157=CARTESIAN_POINT ( 'NONE',  ( 161.7489939963169263, 252.0668770259760265, 14.13598244775917934 ) ) ;
#92158=CARTESIAN_POINT ( 'NONE',  ( 157.5710319558766344, 257.7259621817996162, 18.28704422422941533 ) ) ;
#92160=EDGE_CURVE ( 'NONE', #62531, #23462, #29645, .T. ) ;
#92161=CARTESIAN_POINT ( 'NONE',  ( 26.48065812185646806, 198.3464784336661637, 1.353441290958777327E-15 ) ) ;
#92163=CARTESIAN_POINT ( 'NONE',  ( 54.51857766514267212, 202.2833772461660828, -9.188101187500095079 ) ) ;
#92164=CARTESIAN_POINT ( 'NONE',  ( 196.2609093297512857, 290.7131288316392670, 16.03897268885959448 ) ) ;
#92167=CARTESIAN_POINT ( 'NONE',  ( 149.7817191771959244, 245.0327760586659451, 1.948934522072303157E-15 ) ) ;
#92168=CARTESIAN_POINT ( 'NONE',  ( 48.45674693441662129, 186.5327760586659451, 1.948934522072302763E-15 ) ) ;
#92171=CARTESIAN_POINT ( 'NONE',  ( 150.9363692955544991, 269.2175350005573478, -14.27857383982596140 ) ) ;
#92172=CARTESIAN_POINT ( 'NONE',  ( 196.9728329903666122, 289.4800408803428695, -17.53478045286815856 ) ) ;
#92177=CARTESIAN_POINT ( 'NONE',  ( 198.0792648159935538, 287.5636447432459022, 17.04758482866669667 ) ) ;
#92178=CARTESIAN_POINT ( 'NONE',  ( 182.1968425487349919, 281.0285068568209113, -17.15452853389480126 ) ) ;
#92179=CARTESIAN_POINT ( 'NONE',  ( 201.3491118187633901, 281.9001036014715282, 16.71671293284840587 ) ) ;
#92181=CARTESIAN_POINT ( 'NONE',  ( 117.9459173961707137, 232.2365022471902307, 10.00000000000009592 ) ) ;
#92182=DIRECTION ( 'NONE',  ( -0.8660254037844387076, -0.4999999999999998890, -0.000000000000000000 ) ) ;
#92183=CARTESIAN_POINT ( 'NONE',  ( 166.7087160314272296, 287.6354326016939353, -0.3369197202164816995 ) ) ;
#92187=CARTESIAN_POINT ( 'NONE',  ( 206.6268150440956504, 272.7588534679261443, -10.76664753678610609 ) ) ;
#92188=CARTESIAN_POINT ( 'NONE',  ( 190.1333673262456330, 279.2923110579273498, -17.65696406450081213 ) ) ;
#92190=ORIENTED_EDGE ( 'NONE', *, *, #43057, .T. ) ;
#92191=CARTESIAN_POINT ( 'NONE',  ( 59.94571803450949687, 216.9637435831425023, 2.679491924311251605 ) ) ;
#92193=CARTESIAN_POINT ( 'NONE',  ( 194.6310785344323904, 293.5360785768717165, -14.54510914272505495 ) ) ;
#92198=CARTESIAN_POINT ( 'NONE',  ( 23.67544375150414737, 191.1427522451419350, -10.00000000000009592 ) ) ;
#92199=DIRECTION ( 'NONE',  ( 0.4999999999999992784, -0.8660254037844390407, 0.000000000000000000 ) ) ;
#92201=CARTESIAN_POINT ( 'NONE',  ( 185.2391986358457530, 295.7873944733689768, 8.585680893828113724 ) ) ;
#92206=CARTESIAN_POINT ( 'NONE',  ( 174.0013662709156108, 285.8605094670047606, 10.49998161009456155 ) ) ;
#92207=CARTESIAN_POINT ( 'NONE',  ( 163.1953264782998758, 283.8895661455310915, -7.125257539458086598 ) ) ;
#92209=CARTESIAN_POINT ( 'NONE',  ( 207.6555576926778883, 270.9770189326688410, -1.235081510489080436 ) ) ;
#92210=CARTESIAN_POINT ( 'NONE',  ( 164.4990934228277411, 245.7262077230798809, 6.470820838822735510 ) ) ;
#92212=CARTESIAN_POINT ( 'NONE',  ( 159.7897726928491409, 253.8829904965402875, 16.83923858130328810 ) ) ;
#92213=CARTESIAN_POINT ( 'NONE',  ( 161.1999634265268924, 263.0548667757333874, -17.77828691421615304 ) ) ;
#92215=CARTESIAN_POINT ( 'NONE',  ( 132.4608640057421667, 247.2833772461660544, -9.188101187500095079 ) ) ;
#92217=CARTESIAN_POINT ( 'NONE',  ( 203.0744322039535632, 268.2681989120735011, 2.496359996990924923 ) ) ;
#92218=CARTESIAN_POINT ( 'NONE',  ( 179.0724974991984766, 257.7164609560927033, 10.12017508776513530 ) ) ;
#92219=CARTESIAN_POINT ( 'NONE',  ( 69.94448162217048548, 217.3149278399160949, -9.188101187500095079 ) ) ;
#92221=CARTESIAN_POINT ( 'NONE',  ( 173.2165366525584602, 265.2663209395350918, 16.02481246879085575 ) ) ;
#92222=CYLINDRICAL_SURFACE ( 'NONE', #30159, 17.82106496071139645 ) ;
#92226=CARTESIAN_POINT ( 'NONE',  ( 163.9961211234992788, 256.9275610305372766, 16.20495027727189807 ) ) ;
#92230=CARTESIAN_POINT ( 'NONE',  ( 194.1605905766382136, 284.7225647929109300, 17.53772805858957184 ) ) ;
#92233=CARTESIAN_POINT ( 'NONE',  ( 155.0898745997320134, 262.0234527842152374, 17.05457557403769542 ) ) ;
#92235=CARTESIAN_POINT ( 'NONE',  ( 78.92949518643405327, 222.5024278399160949, 9.188101187500095079 ) ) ;
#92236=ORIENTED_EDGE ( 'NONE', *, *, #18696, .T. ) ;
#92237=ADVANCED_FACE ( 'NONE', ( #62508 ), #55906, .T. ) ;
#92239=CARTESIAN_POINT ( 'NONE',  ( 200.5016309952337394, 283.3679834462653844, -16.85167051214465772 ) ) ;
#92241=CARTESIAN_POINT ( 'NONE',  ( 163.7196345835096452, 261.0355710201180841, -16.91880463402510060 ) ) ;
#92245=CARTESIAN_POINT ( 'NONE',  ( 197.4614820106550326, 280.4067882521826505, 16.54892308915801991 ) ) ;
#92246=CARTESIAN_POINT ( 'NONE',  ( 161.6101421750211671, 260.8786438988923351, 16.75479683814266707 ) ) ;
#92247=ORIENTED_EDGE ( 'NONE', *, *, #25483, .T. ) ;
#92249=CARTESIAN_POINT ( 'NONE',  ( 156.7582088183394546, 274.2853207512858944, 13.68792815068864854 ) ) ;
#92251=CARTESIAN_POINT ( 'NONE',  ( 201.2535035105529744, 282.0657020489176716, -18.08976065250591958 ) ) ;
#92255=ORIENTED_EDGE ( 'NONE', *, *, #72657, .F. ) ;
#92256=CARTESIAN_POINT ( 'NONE',  ( 195.6998486595285840, 265.4147343413312115, 4.643485329879461609 ) ) ;
#92257=CARTESIAN_POINT ( 'NONE',  ( 87.85384634344086408, 209.9824982072973683, 3.021315404115420679E-15 ) ) ;
#92262=CARTESIAN_POINT ( 'NONE',  ( 147.5634954182374372, 275.0595239235922236, 4.682022975662822439 ) ) ;
#92265=CARTESIAN_POINT ( 'NONE',  ( 207.6007741873543750, 271.0719067473055475, 7.587922723682903658 ) ) ;
#92266=CARTESIAN_POINT ( 'NONE',  ( 155.0929244053699847, 262.0181703658971628, 18.51426604808664678 ) ) ;
#92269=CARTESIAN_POINT ( 'NONE',  ( 19.28110618420672395, 193.4860189848785126, -2.679491924311252493 ) ) ;
#92270=CARTESIAN_POINT ( 'NONE',  ( 163.3652774841088444, 283.7749973649284811, -3.153219606719814827 ) ) ;
#92272=CARTESIAN_POINT ( 'NONE',  ( 159.8416255366773839, 253.7931787365127434, 16.77980437810719394 ) ) ;
#92273=CARTESIAN_POINT ( 'NONE',  ( -15.08856125979659346, 174.3464784336661353, 1.353441290958777327E-15 ) ) ;
#92274=CARTESIAN_POINT ( 'NONE',  ( 82.77371932451866599, 207.0494855054051584, -2.679491924311248496 ) ) ;
#92277=CARTESIAN_POINT ( 'NONE',  ( 178.6997720573820061, 256.4289685822167257, 8.737427515670157518 ) ) ;
#92280=CARTESIAN_POINT ( 'NONE',  ( 15.06046875309669630, 173.3768266524159856, -9.188101187500093303 ) ) ;
#92283=CARTESIAN_POINT ( 'NONE',  ( 64.01779381112923772, 217.7677522451419065, -5.000000000000047962 ) ) ;
#92286=CARTESIAN_POINT ( 'NONE',  ( 190.8432295316381442, 261.8533477349316740, -1.278961237959173491 ) ) ;
#92287=CARTESIAN_POINT ( 'NONE',  ( 75.87151652897675547, 204.6115022471901739, -5.000000000000041744 ) ) ;
#92289=CARTESIAN_POINT ( 'NONE',  ( 147.6088797830324779, 274.9809158978982850, 8.531536684623960198 ) ) ;
#92290=CARTESIAN_POINT ( 'NONE',  ( 34.43744006700849525, 196.8149278399160664, 9.188101187500093303 ) ) ;
#92294=CARTESIAN_POINT ( 'NONE',  ( 151.3681950933278983, 268.4695907787949523, -15.50699599486383917 ) ) ;
#92295=CARTESIAN_POINT ( 'NONE',  ( 206.9059968923335475, 272.2752963222270068, 6.902135944297345560 ) ) ;
#92296=CARTESIAN_POINT ( 'NONE',  ( 188.2139646732387348, 267.9741926252710300, 13.43593211841361779 ) ) ;
#92297=CARTESIAN_POINT ( 'NONE',  ( 162.9658701564373189, 281.1729661104742490, -10.32510856000857125 ) ) ;
#92298=B_SPLINE_CURVE_WITH_KNOTS ( 'NONE', 3,
 ( #81951, #52012, #68195, #20624 ),
 .UNSPECIFIED., .F., .F.,
 ( 4, 4 ),
 ( 0.008917401783766700993, 0.01511162993189288720 ),
 .UNSPECIFIED. ) ;
#92299=CARTESIAN_POINT ( 'NONE',  ( 161.4425099228864440, 280.3143438959959894, 8.996476011744888979 ) ) ;
#92302=CARTESIAN_POINT ( 'NONE',  ( 148.3930300673291640, 273.6227277647267897, 8.375036249079425232 ) ) ;
#92304=CARTESIAN_POINT ( 'NONE',  ( 155.0898745997320134, 262.0234527842152374, 17.05457557403769542 ) ) ;
#92307=CARTESIAN_POINT ( 'NONE',  ( 148.7305541605275607, 275.0381188865328568, -8.045727261058747359 ) ) ;
#92310=CARTESIAN_POINT ( 'NONE',  ( 196.1972786361653789, 290.1674837226785826, -16.31932546841715137 ) ) ;
#92314=CARTESIAN_POINT ( 'NONE',  ( 203.3041373168503299, 278.5139001086923827, -16.61929732091214973 ) ) ;
#92319=CARTESIAN_POINT ( 'NONE',  ( 202.2560213337884250, 279.9099699780790615, 15.68235421671478669 ) ) ;
#92320=ORIENTED_EDGE ( 'NONE', *, *, #38847, .T. ) ;
#92321=CARTESIAN_POINT ( 'NONE',  ( 150.8888667059421209, 269.2998118992572927, 15.79021133717968617 ) ) ;
#92323=CARTESIAN_POINT ( 'NONE',  ( -22.42236680055709641, 157.8615022471902591, 0.000000000000000000 ) ) ;
#92325=ORIENTED_EDGE ( 'NONE', *, *, #34417, .F. ) ;
#92326=CARTESIAN_POINT ( 'NONE',  ( 190.5444288681022442, 300.6143634316900943, -1.000014190476072873 ) ) ;
#92328=ORIENTED_EDGE ( 'NONE', *, *, #90000, .F. ) ;
#92329=CARTESIAN_POINT ( 'NONE',  ( 195.6974783896144174, 291.6890198465123945, 16.70600479393688431 ) ) ;
#92331=ORIENTED_EDGE ( 'NONE', *, *, #27017, .F. ) ;
#92338=EDGE_LOOP ( 'NONE', ( #85621, #52031, #66894, #9421 ) ) ;
#92342=CARTESIAN_POINT ( 'NONE',  ( 147.6220714307702622, 274.9580672937808572, 8.392894244419288441 ) ) ;
#92343=CARTESIAN_POINT ( 'NONE',  ( 149.2511585606875428, 272.1364056148075292, 11.40684181024752242 ) ) ;
#92344=CARTESIAN_POINT ( 'NONE',  ( 171.8663912998340777, 275.8233464154953936, -15.83653131706603112 ) ) ;
#92345=CARTESIAN_POINT ( 'NONE',  ( 147.2650827261924746, 275.5763898678378041, 0.3422986961735832168 ) ) ;
#92346=CARTESIAN_POINT ( 'NONE',  ( 146.5865263025993954, 276.7516840693029962, 0.4918294119671828835 ) ) ;
#92347=CARTESIAN_POINT ( 'NONE',  ( 162.9808515016160300, 257.5771916527201029, 15.58578234508959781 ) ) ;
#92349=CARTESIAN_POINT ( 'NONE',  ( 196.5806080813426888, 290.1593943507663766, -16.31912166233602690 ) ) ;
#92352=CARTESIAN_POINT ( 'NONE',  ( 189.7791324398369852, 300.5155985523547884, 1.795207924923805987 ) ) ;
#92356=CARTESIAN_POINT ( 'NONE',  ( 149.6144381846877991, 271.5071868486843414, -11.67527394954620590 ) ) ;
#92360=CARTESIAN_POINT ( 'NONE',  ( 191.9248140970461804, 297.5186077601156285, -10.25883709677317945 ) ) ;
#92361=CARTESIAN_POINT ( 'NONE',  ( 189.8679201377346999, 301.7861109244506679, -1.065287660593647434 ) ) ;
#92363=CARTESIAN_POINT ( 'NONE',  ( 165.3821918710930845, 283.7844301331062979, -8.403629075564190032 ) ) ;
#92365=CARTESIAN_POINT ( 'NONE',  ( 207.5886452961740076, 271.0929146030698007, -1.661373005306138184 ) ) ;
#92366=CARTESIAN_POINT ( 'NONE',  ( 149.8622666665893632, 273.0779353264732663, 11.47145096717591528 ) ) ;
#92367=CARTESIAN_POINT ( 'NONE',  ( 54.85235828774403899, 189.1427522451417644, 1.119607411625061291E-15 ) ) ;
#92368=CARTESIAN_POINT ( 'NONE',  ( 126.7777458412893168, 237.8768266524159856, -9.188101187500093303 ) ) ;
#92369=CARTESIAN_POINT ( 'NONE',  ( 151.1126408083691501, 268.9122237844355254, -15.82705194100464396 ) ) ;
#92371=CARTESIAN_POINT ( 'NONE',  ( 187.3902638176308244, 281.3068701335633364, -17.14294349842597498 ) ) ;
#92372=CARTESIAN_POINT ( 'NONE',  ( 175.9466766006847536, 252.7179606613870249, -4.818959155576430398 ) ) ;
#92373=CARTESIAN_POINT ( 'NONE',  ( 48.83545950068980090, 192.8768266524159856, -9.188101187500091527 ) ) ;
#92374=ADVANCED_FACE ( 'NONE', ( #25543 ), #78251, .T. ) ;
#92375=CARTESIAN_POINT ( 'NONE',  ( 183.1426684129219780, 267.5694331394444703, -16.03671021927237206 ) ) ;
#92380=CARTESIAN_POINT ( 'NONE',  ( 26.07505581137152006, 175.8615022471901739, 5.000000000000051514 ) ) ;
#92381=CARTESIAN_POINT ( 'NONE',  ( 164.4344613858980608, 251.5011570344067877, -12.86682041478359295 ) ) ;
#92382=FACE_OUTER_BOUND ( 'NONE', #84001, .T. ) ;
#92384=CARTESIAN_POINT ( 'NONE',  ( 154.4765043762321000, 276.8026792959899467, -10.28524050916173138 ) ) ;
#92385=CARTESIAN_POINT ( 'NONE',  ( 182.2623503800200240, 262.6690854021607606, 12.85806171487328875 ) ) ;
#92387=CARTESIAN_POINT ( 'NONE',  ( 114.6802799325189284, 237.0177522451418497, -10.00000000000009592 ) ) ;
#92388=CARTESIAN_POINT ( 'NONE',  ( 192.9518127100452034, 296.0217619941561793, -12.12386602825073645 ) ) ;
#92391=CARTESIAN_POINT ( 'NONE',  ( 163.1008115941903895, 248.1481028935802442, 11.25332017433677834 ) ) ;
#92392=CARTESIAN_POINT ( 'NONE',  ( 163.3409975114459485, 247.7320886816312111, -10.96358124877083640 ) ) ;
#92393=CARTESIAN_POINT ( 'NONE',  ( 25.39882055865593458, 173.2202760586659736, -5.415160957724236172E-17 ) ) ;
#92396=CARTESIAN_POINT ( 'NONE',  ( 31.70422093597028734, 199.1115022471903160, -5.000000000000047962 ) ) ;
#92398=CARTESIAN_POINT ( 'NONE',  ( 174.7354935756264638, 286.3370388987765409, 10.43770612672979503 ) ) ;
#92399=CARTESIAN_POINT ( 'NONE',  ( 60.74296170696083408, 212.0024278399160949, 9.188101187500095079 ) ) ;
#92400=CARTESIAN_POINT ( 'NONE',  ( 164.4989226152910646, 245.7265035704120351, -6.575810094723514965 ) ) ;
#92405=CARTESIAN_POINT ( 'NONE',  ( 20.08504676852914272, 175.7365022471902307, -10.00000000000009059 ) ) ;
#92406=CARTESIAN_POINT ( 'NONE',  ( 208.2777459429579210, 269.8993572713111462, 3.129643751043610589 ) ) ;
#92407=CARTESIAN_POINT ( 'NONE',  ( 142.6909626358283560, 247.0643266524159856, -9.188101187500093303 ) ) ;
#92409=CARTESIAN_POINT ( 'NONE',  ( 164.3421951250510631, 260.7081190328407843, -16.15447616004134446 ) ) ;
#92410=CARTESIAN_POINT ( 'NONE',  ( 21.99520779934447745, 195.0530062829863311, -4.648177544792955347E-16 ) ) ;
#92411=CARTESIAN_POINT ( 'NONE',  ( 194.9528736489464791, 280.9848362485358280, -17.70191856674237840 ) ) ;
#92413=CARTESIAN_POINT ( 'NONE',  ( 185.4588683995272902, 277.6883572167094485, -17.52057745498484920 ) ) ;
#92415=ORIENTED_EDGE ( 'NONE', *, *, #9594, .T. ) ;
#92416=CARTESIAN_POINT ( 'NONE',  ( 150.8359915840788688, 269.3913942967808453, 15.73449616766854575 ) ) ;
#92417=CARTESIAN_POINT ( 'NONE',  ( 177.8086748658496674, 286.5436072803887555, 13.62650167180037641 ) ) ;
#92418=CARTESIAN_POINT ( 'NONE',  ( 156.6086985941140313, 280.0481763786762599, -5.331284326237024196 ) ) ;
#92421=CARTESIAN_POINT ( 'NONE',  ( 160.3024851031978528, 252.9949465521450520, 16.22879458631637561 ) ) ;
#92428=CARTESIAN_POINT ( 'NONE',  ( 149.6779600888696677, 272.0038180561006698, 11.37632069153431580 ) ) ;
#92429=CARTESIAN_POINT ( 'NONE',  ( 162.8223739550644211, 248.6303710312858186, -11.16939803179192658 ) ) ;
#92431=CARTESIAN_POINT ( 'NONE',  ( 200.6583719735737645, 283.0965001081523269, -17.35266956530146132 ) ) ;
#92433=CARTESIAN_POINT ( 'NONE',  ( 192.4947987708966650, 281.8339256886280282, 16.78223888497653604 ) ) ;
#92436=CARTESIAN_POINT ( 'NONE',  ( 190.6893905452545823, 300.3632824417117604, 3.294993852933539191 ) ) ;
#92437=CARTESIAN_POINT ( 'NONE',  ( 16.81940930487741426, 170.5177522451417929, 5.000000000000051514 ) ) ;
#92439=VERTEX_POINT ( 'NONE', #63032 ) ;
#92440=CARTESIAN_POINT ( 'NONE',  ( 146.6138605399200117, 276.7043397814778132, -0.5394499176159462950 ) ) ;
#92443=CARTESIAN_POINT ( 'NONE',  ( 196.6317700900902139, 290.0707791521982131, -17.91116578096951883 ) ) ;
#92446=EDGE_LOOP ( 'NONE', ( #69949, #78349, #58596 ) ) ;
#92447=CARTESIAN_POINT ( 'NONE',  ( 108.5372593219620683, 221.2202760586659167, -5.415160957724236172E-17 ) ) ;
#92448=CARTESIAN_POINT ( 'NONE',  ( 155.7819252383450248, 260.8247859167269667, 17.61512984275023896 ) ) ;
#92449=CARTESIAN_POINT ( 'NONE',  ( 150.6533415055477008, 269.7077535128032082, 14.84621632544246062 ) ) ;
#92451=ORIENTED_EDGE ( 'NONE', *, *, #33282, .T. ) ;
#92453=ORIENTED_EDGE ( 'NONE', *, *, #62772, .F. ) ;
#92455=B_SPLINE_CURVE_WITH_KNOTS ( 'NONE', 3,
 ( #98886, #6165, #13293, #59858 ),
 .UNSPECIFIED., .F., .F.,
 ( 4, 4 ),
 ( 0.009316165907098234583, 0.01506860168139122214 ),
 .UNSPECIFIED. ) ;
#92459=CARTESIAN_POINT ( 'NONE',  ( 207.5290616128274337, 271.1961165699281651, 2.604679844609484984 ) ) ;
#92462=CARTESIAN_POINT ( 'NONE',  ( 194.6310785344323904, 293.5360785768717165, -14.54510914272505495 ) ) ;
#92470=CARTESIAN_POINT ( 'NONE',  ( 163.1484656051875106, 248.0655637253488806, 9.714247672444804138 ) ) ;
#92471=CARTESIAN_POINT ( 'NONE',  ( 206.7893622945242385, 272.4773133715531230, -10.52881283832460291 ) ) ;
#92472=CARTESIAN_POINT ( 'NONE',  ( 165.9091197491159164, 246.2627970730538323, -2.747640711776688338 ) ) ;
#92474=CARTESIAN_POINT ( 'NONE',  ( 171.4611298474229386, 255.5042682504870584, 11.10224729584274428 ) ) ;
#92475=CARTESIAN_POINT ( 'NONE',  ( 158.0103319884112523, 281.0314316241064603, 2.028691772727660769 ) ) ;
#92477=CARTESIAN_POINT ( 'NONE',  ( 194.6195663601007766, 293.5560182477196918, -14.78158780203209233 ) ) ;
#92480=CARTESIAN_POINT ( 'NONE',  ( 2.890834060677703210, 159.1427522451417644, 1.119607411625061291E-15 ) ) ;
#92481=CARTESIAN_POINT ( 'NONE',  ( 196.1299550548953050, 269.6200306317458057, -11.66289591416585480 ) ) ;
#92482=CARTESIAN_POINT ( 'NONE',  ( 144.6270795744234476, 268.7413018095040798, -2.761272660171008000E-15 ) ) ;
#92483=CARTESIAN_POINT ( 'NONE',  ( 169.6888855313890474, 280.6163284094095047, -14.28460871240806540 ) ) ;
#92485=CARTESIAN_POINT ( 'NONE',  ( -0.5279885150232012103, 164.3768266524160140, -9.188101187500091527 ) ) ;
#92486=CARTESIAN_POINT ( 'NONE',  ( 115.2960263294082068, 225.8262482093458061, 3.021315404115420679E-15 ) ) ;
#92488=CARTESIAN_POINT ( 'NONE',  ( 17.68543470866176648, 191.0177522451419065, 5.000000000000046185 ) ) ;
#92490=ORIENTED_EDGE ( 'NONE', *, *, #95250, .F. ) ;
#92496=DIRECTION ( 'NONE',  ( -0.5000000000000006661, 0.8660254037844382635, -1.877843081442120958E-16 ) ) ;
#92498=CARTESIAN_POINT ( 'NONE',  ( 153.1046550690079187, 278.4315285291231135, 3.738693302458024448 ) ) ;
#92499=CARTESIAN_POINT ( 'NONE',  ( 8.294124642383250645, 187.8464784336662206, 1.353441290958777525E-15 ) ) ;
#92500=CARTESIAN_POINT ( 'NONE',  ( 115.2486091055264410, 237.3458772461660544, 9.188101187500095079 ) ) ;
#92501=CARTESIAN_POINT ( 'NONE',  ( 179.1786855675093477, 291.9707536515992956, -6.147306910137406710 ) ) ;
#92502=CARTESIAN_POINT ( 'NONE',  ( 195.9340754144258199, 275.1539484599448997, 15.83571573274672417 ) ) ;
#92503=EDGE_CURVE ( 'NONE', #86106, #9838, #23198, .T. ) ;
#92504=CARTESIAN_POINT ( 'NONE',  ( 150.0488362022254023, 271.5008970094041842, -11.96187989116652162 ) ) ;
#92505=CARTESIAN_POINT ( 'NONE',  ( 178.4764170025789554, 283.7516055304348583, -14.72289439906822217 ) ) ;
#92507=CARTESIAN_POINT ( 'NONE',  ( 195.6986305151803549, 291.6870243064952888, 16.84182339398051909 ) ) ;
#92508=CARTESIAN_POINT ( 'NONE',  ( 194.4459411895494725, 293.8567458645873103, 14.31012567920753042 ) ) ;
#92509=CARTESIAN_POINT ( 'NONE',  ( 207.1572261440131797, 271.8401544939704877, -5.633070628900782140 ) ) ;
#92510=CARTESIAN_POINT ( 'NONE',  ( 190.1357066293690536, 284.8999334207817924, 17.11029449594927243 ) ) ;
#92512=CARTESIAN_POINT ( 'NONE',  ( 189.2284142613084157, 262.6620465936063056, 8.058909338376276210 ) ) ;
#92513=CARTESIAN_POINT ( 'NONE',  ( 171.5551119485164975, 279.8722202788326285, 13.93221665515422991 ) ) ;
#92514=CARTESIAN_POINT ( 'NONE',  ( 192.5337445403046104, 265.2601942734702902, 7.958587396316798568 ) ) ;
#92515=CARTESIAN_POINT ( 'NONE',  ( 191.5521510896938935, 298.8689373439769952, -9.847378829740700112 ) ) ;
#92516=CARTESIAN_POINT ( 'NONE',  ( 189.9925954911225290, 301.5701668779311717, 0.1154287172046158938 ) ) ;
#92517=CARTESIAN_POINT ( 'NONE',  ( 180.7798174273501388, 266.8764815076470995, -14.74666571146830307 ) ) ;
#92520=CARTESIAN_POINT ( 'NONE',  ( 154.0199539993881217, 276.0341879782693582, -10.88229598812187682 ) ) ;
#92521=( BOUNDED_CURVE ( )  B_SPLINE_CURVE ( 2, ( #75045, #13249, #91256, #91754, #50717, #44106, #12754, #43617, #90778 ),
 .UNSPECIFIED., .F., .T. ) 
 B_SPLINE_CURVE_WITH_KNOTS ( ( 3, 2, 2, 2, 3 ),
 ( 0.5443548387096773800, 0.5456989247311827551, 0.5483870967741935054, 0.5510752688172042557, 0.5524193548387096309 ),
 .UNSPECIFIED. ) 
 CURVE ( )  GEOMETRIC_REPRESENTATION_ITEM ( )  RATIONAL_B_SPLINE_CURVE ( ( 0.9330127018922194093, 0.9330127018922194093, 1.000000000000000000, 0.8660254037844387076, 1.000000000000000000, 0.8660254037844387076, 1.000000000000000000, 0.9330127018922194093, 0.9330127018922194093 ) ) 
 REPRESENTATION_ITEM ( '' )  );
#92522=CARTESIAN_POINT ( 'NONE',  ( 163.7587049410067266, 247.0085981909329576, -6.137518685179130351 ) ) ;
#92524=CARTESIAN_POINT ( 'NONE',  ( 98.52366704282199805, 221.5643266524159856, -9.188101187500093303 ) ) ;
#92526=CARTESIAN_POINT ( 'NONE',  ( 191.5766842709549280, 298.8264446275616137, 8.039910086100929831 ) ) ;
#92528=DIRECTION ( 'NONE',  ( 0.4999999999999992784, -0.8660254037844390407, 0.000000000000000000 ) ) ;
#92530=CARTESIAN_POINT ( 'NONE',  ( 149.2285814192496218, 272.1755103708678121, 13.04936292285073485 ) ) ;
#92531=B_SPLINE_CURVE_WITH_KNOTS ( 'NONE', 3,
 ( #52121, #36925, #97756, #20753, #90178, #74952, #52615, #45020, #99245, #60702, #22226, #84084, #14635, #37907, #68817, #99744, #61219, #22736, #77396, #7474, #84528, #91618, #38873, #92622, #75407, #69280, #45475, #21694, #68777, #69778, #387, #62163, #100206, #53573, #67793, #52576, #53083, #31275, #93112, #37376, #15072, #14596, #45961, #76878, #37867, #30793, #38369, #98719, #83530, #84037, #23664, #54556 ),
 .UNSPECIFIED., .F., .F.,
 ( 4, 2, 2, 2, 2, 2, 2, 2, 2, 2, 2, 2, 2, 2, 2, 2, 2, 2, 2, 2, 2, 2, 2, 2, 2, 4 ),
 ( 0.0008597875087230317853, 0.001056026466501868441, 0.001154145945391277283, 0.001252265424280685907, 0.001448504382059393435, 0.001644743339838100745, 0.002037221255395451399, 0.002429699170952801836, 0.003214655002067501408, 0.003999610833182200113, 0.004784566664296898385, 0.005177044579854248388, 0.005373283537632888261, 0.005471403016522252000, 0.005520462755966851036, 0.005569522495411450939, 0.005618582234856050843, 0.005667641974300649879, 0.005765761453189883513, 0.005962000410968388946, 0.006158239368746893511, 0.006354478326525398076, 0.006550717284303903508, 0.006746956242082408073, 0.006943195199860913505, 0.007139434157639417203 ),
 .UNSPECIFIED. ) ;
#92532=CARTESIAN_POINT ( 'NONE',  ( 150.8168331730346949, 269.4245776381016526, -15.71017957295074652 ) ) ;
#92533=CARTESIAN_POINT ( 'NONE',  ( 149.8554569740625197, 271.5993192349010315, -11.69353262999953103 ) ) ;
#92534=CARTESIAN_POINT ( 'NONE',  ( 58.13834967963523326, 192.8262482093458061, 3.021315404115420679E-15 ) ) ;
#92540=CARTESIAN_POINT ( 'NONE',  ( 196.5802072422632421, 267.8039352643175448, 9.492349405241153448 ) ) ;
#92541=CARTESIAN_POINT ( 'NONE',  ( 196.6317700900902139, 290.0707791521982131, -17.91116578096951883 ) ) ;
#92548=CARTESIAN_POINT ( 'NONE',  ( 173.1432744218939774, 253.4296248983395401, -9.251738304191658102 ) ) ;
#92549=CARTESIAN_POINT ( 'NONE',  ( 192.2431834237441706, 297.6720342317289578, 11.07782187406058938 ) ) ;
#92550=EDGE_CURVE ( 'NONE', #5319, #34942, #54586, .T. ) ;
#92551=ORIENTED_EDGE ( 'NONE', *, *, #14832, .F. ) ;
#92552=CARTESIAN_POINT ( 'NONE',  ( 187.5872943901169378, 278.9980123648381891, 16.95840433791729396 ) ) ;
#92560=EDGE_CURVE ( 'NONE', #90346, #63237, #49589, .T. ) ;
#92561=CARTESIAN_POINT ( 'NONE',  ( 206.2925202860113245, 273.3378689736323963, 11.27730907742713384 ) ) ;
#92563=CARTESIAN_POINT ( 'NONE',  ( 154.0425198334700099, 263.8375244529303245, -16.86014285715240035 ) ) ;
#92564=CARTESIAN_POINT ( 'NONE',  ( 201.1679199471075492, 282.2139371290980989, -16.62385308864941535 ) ) ;
#92566=DIRECTION ( 'NONE',  ( 0.4999999999999992784, -0.8660254037844390407, 0.000000000000000000 ) ) ;
#92570=VERTEX_POINT ( 'NONE', #58900 ) ;
#92571=CARTESIAN_POINT ( 'NONE',  ( 176.0924988190274121, 258.7481610597934605, 13.20100988338283088 ) ) ;
#92572=ORIENTED_EDGE ( 'NONE', *, *, #88248, .T. ) ;
#92574=CARTESIAN_POINT ( 'NONE',  ( 172.8345891994052579, 271.0481249001369406, 16.42822092899199049 ) ) ;
#92578=CARTESIAN_POINT ( 'NONE',  ( 164.4200829731848046, 246.2493134173791418, 2.172245655849200485 ) ) ;
#92579=DIRECTION ( 'NONE',  ( 0.4999999999999992784, -0.8660254037844390407, 0.000000000000000000 ) ) ;
#92580=CARTESIAN_POINT ( 'NONE',  ( 200.4204578720470522, 274.6855620619879232, -13.71762816491924220 ) ) ;
#92582=CARTESIAN_POINT ( 'NONE',  ( 147.0314375879888757, 275.9810751181479986, -5.168577011192616588 ) ) ;
#92583=CARTESIAN_POINT ( 'NONE',  ( 171.4353610529350078, 250.3536029180922640, -5.787908394485046237 ) ) ;
#92585=CARTESIAN_POINT ( 'NONE',  ( 178.0362726450289017, 255.4666490453336678, 5.105776653552220878 ) ) ;
#92588=CARTESIAN_POINT ( 'NONE',  ( 188.1412547211656943, 273.5593357346770063, 17.08033167198486879 ) ) ;
#92593=CARTESIAN_POINT ( 'NONE',  ( 192.0519773745460554, 298.0032128236547351, 11.68523422658327249 ) ) ;
#92595=CARTESIAN_POINT ( 'NONE',  ( 201.1755594471486859, 282.2007051268825535, -18.15567516623250910 ) ) ;
#92596=FACE_OUTER_BOUND ( 'NONE', #1617, .T. ) ;
#92597=VERTEX_POINT ( 'NONE', #3752 ) ;
#92598=CARTESIAN_POINT ( 'NONE',  ( 195.0715819075916215, 292.7731043536545030, 16.72244352212509710 ) ) ;
#92600=CARTESIAN_POINT ( 'NONE',  ( 194.8432095198904221, 293.1686569321988145, -14.74101036184996616 ) ) ;
#92603=CARTESIAN_POINT ( 'NONE',  ( 190.3065890357339356, 267.3458242085297911, -11.97292556197838209 ) ) ;
#92604=B_SPLINE_CURVE_WITH_KNOTS ( 'NONE', 3,
 ( #65718, #64232, #34817, #55609 ),
 .UNSPECIFIED., .F., .F.,
 ( 4, 4 ),
 ( 0.02515406699106021923, 0.03440006065807557634 ),
 .UNSPECIFIED. ) ;
#92605=CARTESIAN_POINT ( 'NONE',  ( 190.8715817853789645, 283.7415510105400926, -16.63753925581049486 ) ) ;
#92606=CARTESIAN_POINT ( 'NONE',  ( 192.3743113064165584, 262.7446559956477472, 4.590962410021210971 ) ) ;
#92607=CARTESIAN_POINT ( 'NONE',  ( -10.09954699608895901, 171.6427522451419350, -10.00000000000009592 ) ) ;
#92608=CARTESIAN_POINT ( 'NONE',  ( 204.8008807586744524, 272.7600038595665524, -10.89009281376315741 ) ) ;
#92609=CARTESIAN_POINT ( 'NONE',  ( 184.3834185992925825, 288.5535061363751765, -13.68474095756436881 ) ) ;
#92610=CARTESIAN_POINT ( 'NONE',  ( 160.7842430252816541, 281.5629877887335510, 5.625797120217996827 ) ) ;
#92611=CIRCLE ( 'NONE', #82925, 17.82106496071138935 ) ;
#92612=CARTESIAN_POINT ( 'NONE',  ( 153.3506059258413643, 265.0359544954067132, -16.39100908615009899 ) ) ;
#92616=CARTESIAN_POINT ( 'NONE',  ( 186.9340657304752540, 262.8988569655599576, -9.024534070206733816 ) ) ;
#92617=CARTESIAN_POINT ( 'NONE',  ( 198.2505066714982149, 285.2670451491296149, 0.000000000000000000 ) ) ;
#92618=CARTESIAN_POINT ( 'NONE',  ( 192.6739937146571151, 271.4875022964622531, -15.03443561379086191 ) ) ;
#92619=CARTESIAN_POINT ( 'NONE',  ( 3.924699723655708627, 184.6199935810940929, 2.679491924311251605 ) ) ;
#92622=CARTESIAN_POINT ( 'NONE',  ( 191.3994361718305015, 283.5433174942932624, -16.59339826374022309 ) ) ;
#92624=CARTESIAN_POINT ( 'NONE',  ( 66.23672358827711548, 218.2369531367911293, -4.594050593750048428 ) ) ;
#92626=CARTESIAN_POINT ( 'NONE',  ( 147.4323331177958494, 275.2867036919951147, -5.064030047414062707 ) ) ;
#92627=CARTESIAN_POINT ( 'NONE',  ( 163.1369207721744772, 248.0855599626920593, -11.24692769914530110 ) ) ;
#92629=CARTESIAN_POINT ( 'NONE',  ( 154.9067123643522734, 262.3406990819208886, -18.18534662427576265 ) ) ;
#92630=CARTESIAN_POINT ( 'NONE',  ( 207.7836085030675690, 270.7552284231231852, -5.468305433308493058 ) ) ;
#92631=CARTESIAN_POINT ( 'NONE',  ( 202.8499463704053198, 279.3005819042728604, 17.04674939340617001 ) ) ;
#92632=CARTESIAN_POINT ( 'NONE',  ( 162.8513067182543921, 284.1523628685703216, 6.041541777105626565 ) ) ;
#92635=CARTESIAN_POINT ( 'NONE',  ( 185.7372650184451857, 257.4645284076796656, -2.264991511946413505E-12 ) ) ;
#92637=CARTESIAN_POINT ( 'NONE',  ( 169.2563262549492151, 252.1410605716396560, -8.850704283268973072 ) ) ;
#92638=CARTESIAN_POINT ( 'NONE',  ( 205.1068273514435703, 275.3915493784789419, -12.24197861934597142 ) ) ;
#92639=CARTESIAN_POINT ( 'NONE',  ( 195.7291534503633272, 291.6341570319625021, 16.44925029361851543 ) ) ;
#92642=CARTESIAN_POINT ( 'NONE',  ( 35.30381256655795852, 185.0643266524160140, 9.188101187500095079 ) ) ;
#92643=CARTESIAN_POINT ( 'NONE',  ( 52.46142023538963173, 213.3464784336661637, 1.353441290958777327E-15 ) ) ;
#92644=CARTESIAN_POINT ( 'NONE',  ( 164.1172920531512318, 247.2548588590273368, -6.812855435237894497 ) ) ;
#92647=CARTESIAN_POINT ( 'NONE',  ( 138.9828575061699496, 260.2369531367911009, -4.594050593750048428 ) ) ;
#92649=CARTESIAN_POINT ( 'NONE',  ( 197.9229657308372907, 270.3857085654402113, -10.89782717189174654 ) ) ;
#92651=CARTESIAN_POINT ( 'NONE',  ( -15.39849209473666569, 173.4637435831425307, 2.679491924311255158 ) ) ;
#92654=CARTESIAN_POINT ( 'NONE',  ( 56.27743144475606130, 212.4869531367911009, 4.594050593750046652 ) ) ;
#92655=CARTESIAN_POINT ( 'NONE',  ( 158.8209852333526158, 256.8487328634645337, -16.76518060723513415 ) ) ;
#92657=CARTESIAN_POINT ( 'NONE',  ( 159.4230536986738400, 254.5181664265525683, 16.83068086755798376 ) ) ;
#92658=CARTESIAN_POINT ( 'NONE',  ( 53.62548896571601631, 201.7677522451418781, 10.00000000000009592 ) ) ;
#92659=CARTESIAN_POINT ( 'NONE',  ( 151.4592217034740997, 275.9376209827681237, 7.243053434427960013 ) ) ;
#92660=CARTESIAN_POINT ( 'NONE',  ( 112.2445834879230944, 245.6115022471903160, -5.000000000000047962 ) ) ;
#92661=CARTESIAN_POINT ( 'NONE',  ( 200.3134965941964651, 283.6938417875134064, 18.29802468362849766 ) ) ;
#92662=EDGE_CURVE ( 'NONE', #19580, #71349, #40059, .T. ) ;
#92663=CARTESIAN_POINT ( 'NONE',  ( 165.0437781805843258, 244.7827860485373606, -2.050141714668513693 ) ) ;
#92664=VERTEX_POINT ( 'NONE', #20444 ) ;
#92667=ORIENTED_EDGE ( 'NONE', *, *, #38296, .T. ) ;
#92668=CARTESIAN_POINT ( 'NONE',  ( 160.0081047537594543, 253.5048282741223602, -16.11956848123596941 ) ) ;
#92669=CARTESIAN_POINT ( 'NONE',  ( 193.7981402883559099, 293.2477674331528874, 15.14322874797242768 ) ) ;
#92673=CARTESIAN_POINT ( 'NONE',  ( 165.0437781805843258, 244.7827860485373606, -2.050141714668513693 ) ) ;
#92675=CARTESIAN_POINT ( 'NONE',  ( 147.7467138384290308, 274.7421803109381813, -9.190172068879620682 ) ) ;
#92676=CARTESIAN_POINT ( 'NONE',  ( -22.42236680055709641, 157.8615022471902591, 0.000000000000000000 ) ) ;
#92687=CARTESIAN_POINT ( 'NONE',  ( 172.2853610648057838, 258.8912576570302235, 14.85002519649902908 ) ) ;
#92692=CARTESIAN_POINT ( 'NONE',  ( 207.5920568422024814, 271.0870056320159165, -1.586464549033245186 ) ) ;
#92693=CARTESIAN_POINT ( 'NONE',  ( 163.9587364689194260, 246.6621334214722481, 5.816126667419880825 ) ) ;
#92694=CARTESIAN_POINT ( 'NONE',  ( 188.3275099133877006, 294.7511660258297184, -11.02676022468676287 ) ) ;
#92695=CARTESIAN_POINT ( 'NONE',  ( 205.0716081116550527, 275.4525508911965517, -12.57761053684872188 ) ) ;
#92696=CARTESIAN_POINT ( 'NONE',  ( 140.7695555451228984, 242.8923013555409796, 4.594050593750050204 ) ) ;
#92697=CARTESIAN_POINT ( 'NONE',  ( 160.1046160203818545, 254.1427746626272324, -15.31471876624168793 ) ) ;
#92699=CARTESIAN_POINT ( 'NONE',  ( 180.5113990821174355, 259.4917306361832061, 9.538867622362561249 ) ) ;
#92700=CARTESIAN_POINT ( 'NONE',  ( 72.38035161819672680, 212.5958772461660544, -9.188101187500095079 ) ) ;
#92702=CARTESIAN_POINT ( 'NONE',  ( 150.6533415055477008, 269.7077535128032082, 14.84621632544246062 ) ) ;
#92704=ORIENTED_EDGE ( 'NONE', *, *, #67685, .F. ) ;
#92705=CARTESIAN_POINT ( 'NONE',  ( 157.3026460594630294, 258.1908201904226985, -16.97013930368657242 ) ) ;
#92706=ORIENTED_EDGE ( 'NONE', *, *, #40455, .F. ) ;
#92709=CARTESIAN_POINT ( 'NONE',  ( 194.5843950310221828, 284.9301011135724480, 17.17984868612067118 ) ) ;
#92710=CARTESIAN_POINT ( 'NONE',  ( 147.2229325088103735, 275.6493961858936927, -0.4918294119671829390 ) ) ;
#92712=CARTESIAN_POINT ( 'NONE',  ( 193.7118145980225279, 295.1282904202991517, 14.61271143546694162 ) ) ;
#92714=CARTESIAN_POINT ( 'NONE',  ( 84.04489159724214176, 210.1423013555409796, -4.594050593750043987 ) ) ;
#92718=CARTESIAN_POINT ( 'NONE',  ( 161.4285303944317036, 251.0445788961045537, -12.80520346941578502 ) ) ;
#92722=B_SPLINE_CURVE_WITH_KNOTS ( 'NONE', 3,
 ( #76215, #74229, #30090, #59975 ),
 .UNSPECIFIED., .F., .F.,
 ( 4, 4 ),
 ( 2.823925224926892107E-17, 0.003590681989198405560 ),
 .UNSPECIFIED. ) ;
#92723=CARTESIAN_POINT ( 'NONE',  ( 183.6537928361365175, 275.7188707068767144, 17.33434013053200928 ) ) ;
#92725=CARTESIAN_POINT ( 'NONE',  ( 207.0624025450594843, 270.0043937851150417, -2.644299678167422840 ) ) ;
#92726=CARTESIAN_POINT ( 'NONE',  ( 162.7006039569504594, 261.3497057169571463, 17.57720365097131676 ) ) ;
#92727=ORIENTED_EDGE ( 'NONE', *, *, #35728, .F. ) ;
#92728=CARTESIAN_POINT ( 'NONE',  ( 191.2234062282808509, 295.9205195230730965, 11.25357184734625626 ) ) ;
#92730=CARTESIAN_POINT ( 'NONE',  ( 201.4520623681621316, 281.7217880192456505, -17.56577389517433119 ) ) ;
#92734=CARTESIAN_POINT ( 'NONE',  ( 195.7006838637995827, 265.4149546518947318, 4.607653087064138120 ) ) ;
#92735=CARTESIAN_POINT ( 'NONE',  ( 181.6234035976268615, 291.8979964657406754, 10.50546202400086671 ) ) ;
#92737=CARTESIAN_POINT ( 'NONE',  ( 188.0529924718924519, 265.9906442623397993, -13.09709986203515797 ) ) ;
#92739=DIRECTION ( 'NONE',  ( -0.8660254037844387076, -0.4999999999999998890, -0.000000000000000000 ) ) ;
#92742=CARTESIAN_POINT ( 'NONE',  ( 162.7644741734472120, 248.7306563947940958, 9.865755277559742353 ) ) ;
#92744=CARTESIAN_POINT ( 'NONE',  ( 194.4263876777154394, 293.8906135405502482, 15.23185943445137802 ) ) ;
#92752=CARTESIAN_POINT ( 'NONE',  ( 190.3922147189167902, 261.8887683268970932, 2.888942485245276526 ) ) ;
#92753=ADVANCED_FACE ( 'NONE', ( #10227 ), #3072, .F. ) ;
#92754=CARTESIAN_POINT ( 'NONE',  ( -12.00317221093202136, 170.0024278399160949, 9.188101187500095079 ) ) ;
#92755=CARTESIAN_POINT ( 'NONE',  ( 80.97745796857455503, 210.8927522451417929, -10.00000000000009237 ) ) ;
#92760=CARTESIAN_POINT ( 'NONE',  ( 163.2669474939272902, 273.3144560705613912, 16.33214292347920349 ) ) ;
#92761=CARTESIAN_POINT ( 'NONE',  ( 26.12944271915780448, 176.7048013555409796, 4.594050593750051981 ) ) ;
#92765=CARTESIAN_POINT ( 'NONE',  ( 157.8043799545718286, 257.3217915922150496, -17.97575562758749257 ) ) ;
#92767=B_SPLINE_SURFACE_WITH_KNOTS ( 'NONE', 3, 1, ( 
 ( #32173, #70674 ),
 ( #62556, #54970 ),
 ( #85428, #39745 ),
 ( #31166, #48388 ),
 ( #24572, #8877 ),
 ( #63077, #1289 ),
 ( #24076, #85948 ),
 ( #15976, #78294 ),
 ( #54451, #78796 ),
 ( #94021, #55457 ),
 ( #16476, #8386 ),
 ( #23064, #32677 ),
 ( #39253, #47371 ),
 ( #9900, #47858 ),
 ( #86442, #55950 ),
 ( #15459, #9383 ),
 ( #62055, #773 ),
 ( #16969, #46877 ),
 ( #69673, #279 ),
 ( #77802, #2301 ),
 ( #40261, #71709 ),
 ( #71201, #70164 ),
 ( #86946, #93006 ),
 ( #53959, #17479 ),
 ( #79332, #1794 ),
 ( #63576, #84916 ),
 ( #94520, #61568 ),
 ( #92516, #38769 ),
 ( #46357, #77282 ),
 ( #7892, #81324 ),
 ( #87465, #34672 ),
 ( #73687, #65574 ),
 ( #74203, #81817 ),
 ( #56965, #72717 ) ),
 .UNSPECIFIED., .T., .F., .F.,
 ( 4, 2, 2, 2, 2, 2, 2, 2, 2, 2, 2, 2, 2, 2, 2, 2, 4 ),
 ( 2, 2 ),
 ( 0.000000000000000000, 0.06250000000000000000, 0.1250000000000000000, 0.1875000000000000000, 0.2500000000000000000, 0.3125000000000000000, 0.3750000000000000000, 0.4375000000000000000, 0.5000000000000000000, 0.5625000000000000000, 0.6250000000000000000, 0.6875000000000000000, 0.7500000000000000000, 0.8125000000000000000, 0.8750000000000000000, 0.9375000000000000000, 1.000000000000000000 ),
 ( 0.000000000000000000, 1.000000000000000000 ),
 .UNSPECIFIED. ) ;
#92769=CARTESIAN_POINT ( 'NONE',  ( 190.4498225699937564, 261.8013334372093937, -0.7578904268681307954 ) ) ;
#92770=CARTESIAN_POINT ( 'NONE',  ( 182.8250716288524131, 295.5606410807013162, 1.016483728176388324 ) ) ;
#92771=CARTESIAN_POINT ( 'NONE',  ( 66.85041857288875633, 222.7365022471903160, 2.944929066748280225E-16 ) ) ;
#92773=EDGE_CURVE ( 'NONE', #86172, #23023, #67702, .T. ) ;
#92774=CARTESIAN_POINT ( 'NONE',  ( 203.4957782983326524, 270.1299432202798698, 6.025416085054049908 ) ) ;
#92775=CARTESIAN_POINT ( 'NONE',  ( 40.17520546284541894, 187.8768266524160140, 9.188101187500098632 ) ) ;
#92776=CARTESIAN_POINT ( 'NONE',  ( 167.1385956060480282, 251.2337521017574602, -11.14139130086932639 ) ) ;
#92778=CARTESIAN_POINT ( 'NONE',  ( 65.02584505343169496, 219.8967562850346837, -4.648177544792955347E-16 ) ) ;
#92780=CARTESIAN_POINT ( 'NONE',  ( 164.2723164851102808, 246.1189969011916503, -1.993789335506892302 ) ) ;
#92782=CARTESIAN_POINT ( 'NONE',  ( 161.8432519094067175, 279.7467170949879574, -9.831637663153189877 ) ) ;
#92783=CARTESIAN_POINT ( 'NONE',  ( 158.7942145198741741, 261.8960026634072733, 17.81789268137834625 ) ) ;
#92785=CARTESIAN_POINT ( 'NONE',  ( 189.9462859318020946, 301.6503773875500087, -1.164147598593831656 ) ) ;
#92787=CARTESIAN_POINT ( 'NONE',  ( 188.8678792399009581, 270.1696821249879576, -14.21866136085443877 ) ) ;
#92789=CARTESIAN_POINT ( 'NONE',  ( 185.5458178329047882, 290.8126708647759529, 12.98563741746813349 ) ) ;
#92790=CARTESIAN_POINT ( 'NONE',  ( 178.6782777294722848, 260.6412425082613709, 13.57969907341511551 ) ) ;
#92794=ORIENTED_EDGE ( 'NONE', *, *, #13650, .T. ) ;
#92798=CARTESIAN_POINT ( 'NONE',  ( 181.1390130125879807, 257.6774870082531379, -7.540388427927620540 ) ) ;
#92800=( BOUNDED_CURVE ( )  B_SPLINE_CURVE ( 2, ( #83884, #99549, #22538, #85380, #62007, #54404, #25023, #47812, #9337 ),
 .UNSPECIFIED., .F., .F. ) 
 B_SPLINE_CURVE_WITH_KNOTS ( ( 3, 2, 2, 2, 3 ),
 ( 0.4395161290322580627, 0.4408602150537634379, 0.4435483870967741882, 0.4462365591397849385, 0.4475806451612903136 ),
 .UNSPECIFIED. ) 
 CURVE ( )  GEOMETRIC_REPRESENTATION_ITEM ( )  RATIONAL_B_SPLINE_CURVE ( ( 0.9330127018922194093, 0.9330127018922194093, 1.000000000000000000, 0.8660254037844387076, 1.000000000000000000, 0.8660254037844387076, 1.000000000000000000, 0.9330127018922194093, 0.9330127018922194093 ) ) 
 REPRESENTATION_ITEM ( '' )  );
#92801=ORIENTED_EDGE ( 'NONE', *, *, #75470, .F. ) ;
#92805=CARTESIAN_POINT ( 'NONE',  ( 151.0099717111976076, 269.0900518771037468, 15.84752309685681659 ) ) ;
#92809=ORIENTED_EDGE ( 'NONE', *, *, #18319, .F. ) ;
#92810=CARTESIAN_POINT ( 'NONE',  ( 189.8238368927809745, 301.8624653444729802, -0.3620111495846872751 ) ) ;
#92811=EDGE_CURVE ( 'NONE', #28762, #97214, #64119, .T. ) ;
#92814=FACE_OUTER_BOUND ( 'NONE', #65220, .T. ) ;
#92816=ORIENTED_EDGE ( 'NONE', *, *, #47497, .T. ) ;
#92822=( BOUNDED_CURVE ( )  B_SPLINE_CURVE ( 2, ( #46449, #84023, #32264, #70259, #45947, #23650, #47462, #867, #37853 ),
 .UNSPECIFIED., .F., .T. ) 
 B_SPLINE_CURVE_WITH_KNOTS ( ( 3, 2, 2, 2, 3 ),
 ( 0.1411290322580645296, 0.1424731182795699047, 0.1451612903225806550, 0.1478494623655914053, 0.1491935483870967805 ),
 .UNSPECIFIED. ) 
 CURVE ( )  GEOMETRIC_REPRESENTATION_ITEM ( )  RATIONAL_B_SPLINE_CURVE ( ( 0.9330127018922194093, 0.9330127018922200755, 1.000000000000000000, 0.8660254037844387076, 1.000000000000000000, 0.8660254037844387076, 1.000000000000000000, 0.9330127018922194093, 0.9330127018922194093 ) ) 
 REPRESENTATION_ITEM ( '' )  );
#92823=CARTESIAN_POINT ( 'NONE',  ( 190.7851866479434761, 300.1973587246873194, 7.931162401707728016 ) ) ;
#92828=CARTESIAN_POINT ( 'NONE',  ( -22.42236680055709641, 157.8615022471902591, 0.000000000000000000 ) ) ;
#92831=CARTESIAN_POINT ( 'NONE',  ( 190.1696443193688708, 301.2635093119881162, -4.804312979389741223 ) ) ;
#92832=CARTESIAN_POINT ( 'NONE',  ( 190.1158090214649405, 301.3567547831981983, -1.340987185199551845 ) ) ;
#92834=CARTESIAN_POINT ( 'NONE',  ( 190.8187029736043883, 300.1393067457597681, 3.941064102378585954 ) ) ;
#92835=CARTESIAN_POINT ( 'NONE',  ( 171.6872963709983821, 276.1252452772627635, -16.94555118095737711 ) ) ;
#92837=FACE_OUTER_BOUND ( 'NONE', #71292, .T. ) ;
#92838=CARTESIAN_POINT ( 'NONE',  ( 148.9230895364621574, 272.7046378331555161, 12.20434325797056019 ) ) ;
#92840=CARTESIAN_POINT ( 'NONE',  ( 94.56323149399085537, 218.7365022471901739, 10.00000000000009948 ) ) ;
#92842=CARTESIAN_POINT ( 'NONE',  ( 154.6387566766715054, 264.1588125162423353, -17.13921758461861700 ) ) ;
#92844=CARTESIAN_POINT ( 'NONE',  ( 107.5083335113205578, 239.0024278399160949, 9.188101187500095079 ) ) ;
#92846=CARTESIAN_POINT ( 'NONE',  ( 146.8859094598974480, 276.2331372299326517, -0.7994986043261681496 ) ) ;
#92849=CARTESIAN_POINT ( 'NONE',  ( 202.7602807045765019, 279.4558873931827065, -15.90558713185497020 ) ) ;
#92850=CARTESIAN_POINT ( 'NONE',  ( 182.0697224992034648, 283.9259822107836158, -15.01725063203069865 ) ) ;
#92852=CARTESIAN_POINT ( 'NONE',  ( 165.7172767540421319, 283.5836649089671937, -8.214104100105947381 ) ) ;
#92853=ORIENTED_EDGE ( 'NONE', *, *, #25121, .T. ) ;
#92854=CARTESIAN_POINT ( 'NONE',  ( 208.3764315856425640, 269.7284287242038658, -1.833640725398759441 ) ) ;
#92856=CARTESIAN_POINT ( 'NONE',  ( 49.72837464868604940, 199.5177522451418781, -10.00000000000009592 ) ) ;
#92857=CARTESIAN_POINT ( 'NONE',  ( 131.1078728602114722, 240.3768266524160424, 9.188101187500096856 ) ) ;
#92858=CARTESIAN_POINT ( 'NONE',  ( 150.7133245577828689, 269.6038598187387834, -14.58664962216439598 ) ) ;
#92860=CARTESIAN_POINT ( 'NONE',  ( 196.4982648257524147, 290.3020170531091821, 16.69353242256149628 ) ) ;
#92862=CARTESIAN_POINT ( 'NONE',  ( 46.91405240998433612, 188.7048013555409796, 4.594050593750051981 ) ) ;
#92864=ORIENTED_EDGE ( 'NONE', *, *, #41701, .T. ) ;
#92869=CARTESIAN_POINT ( 'NONE',  ( 190.1693911629507738, 301.2639477917662703, -5.112716700269980485 ) ) ;
#92873=CARTESIAN_POINT ( 'NONE',  ( 178.5272579798314894, 261.1979847487124289, 12.22333219613103239 ) ) ;
#92874=CARTESIAN_POINT ( 'NONE',  ( 106.8860512984590088, 232.5177522451418781, -10.00000000000009592 ) ) ;
#92879=CARTESIAN_POINT ( 'NONE',  ( 189.9052851100924215, 301.7213928939034986, -1.077181946533001256 ) ) ;
#92880=DIRECTION ( 'NONE',  ( 0.4999999999999992784, -0.8660254037844390407, 0.000000000000000000 ) ) ;
#92881=CARTESIAN_POINT ( 'NONE',  ( 20.74358691754956396, 182.7833772461660544, -9.188101187500095079 ) ) ;
#92883=CARTESIAN_POINT ( 'NONE',  ( 192.9465561454275928, 272.3177685425281993, 14.20360320959197686 ) ) ;
#92884=CARTESIAN_POINT ( 'NONE',  ( 160.3733185927383715, 282.5102941377067509, 6.606729549618552078 ) ) ;
#92886=CARTESIAN_POINT ( 'NONE',  ( 197.8951961584970149, 277.1396171073823211, -15.32953000722216430 ) ) ;
#92887=CARTESIAN_POINT ( 'NONE',  ( 69.15955932604958889, 219.9244531367911293, -4.594050593750046652 ) ) ;
#92888=CARTESIAN_POINT ( 'NONE',  ( 208.3152833949211526, 269.8343404973242059, 2.763633873278860342 ) ) ;
#92894=CARTESIAN_POINT ( 'NONE',  ( 25.28119919123569304, 198.7365022471903444, 2.944929066748280225E-16 ) ) ;
#92895=CARTESIAN_POINT ( 'NONE',  ( 207.6471633721571379, 270.9915583223058206, 2.196965492132801678 ) ) ;
#92896=CARTESIAN_POINT ( 'NONE',  ( -15.41332078621576329, 174.1589784336661637, -6.496448406907675876E-16 ) ) ;
#92898=CARTESIAN_POINT ( 'NONE',  ( 167.5778442440516471, 262.4579367844059448, -16.54578138360918160 ) ) ;
#92899=CARTESIAN_POINT ( 'NONE',  ( 186.0023642507784416, 260.7041546637453848, 6.337017704808292962 ) ) ;
#92900=CARTESIAN_POINT ( 'NONE',  ( 206.1215120922853146, 273.6340638536760821, 10.12238414215620885 ) ) ;
#92901=AXIS2_PLACEMENT_3D ( 'NONE', #47410, #87502, #78336 ) ;
#92906=CARTESIAN_POINT ( 'NONE',  ( 164.0943423276914643, 246.4272571842752484, 8.509643519936494371 ) ) ;
#92907=CARTESIAN_POINT ( 'NONE',  ( 178.5527154611763763, 285.5147197797991794, 13.02099474314520400 ) ) ;
#92911=DIRECTION ( 'NONE',  ( -0.8660254037844387076, -0.4999999999999998890, -0.000000000000000000 ) ) ;
#92912=CARTESIAN_POINT ( 'NONE',  ( 157.1965120183049578, 258.3746497421212780, -18.06591467563559306 ) ) ;
#92915=CARTESIAN_POINT ( 'NONE',  ( 41.08847453908118297, 182.9824982072973967, 3.021315404115420679E-15 ) ) ;
#92916=CARTESIAN_POINT ( 'NONE',  ( 163.3939361803663246, 247.6403962173759226, -10.78041711314006790 ) ) ;
#92917=CARTESIAN_POINT ( 'NONE',  ( 200.8147387322574957, 282.8256649374973790, -18.02438097732020239 ) ) ;
#92918=ORIENTED_EDGE ( 'NONE', *, *, #31217, .F. ) ;
#92920=CARTESIAN_POINT ( 'NONE',  ( 190.7147070850360819, 281.1586976679043346, 16.70495451513169272 ) ) ;
#92922=ORIENTED_EDGE ( 'NONE', *, *, #18760, .F. ) ;
#92925=ORIENTED_EDGE ( 'NONE', *, *, #98793, .T. ) ;
#92927=CARTESIAN_POINT ( 'NONE',  ( 186.2798660816079632, 264.0713031700501006, -12.82791401631097550 ) ) ;
#92933=CARTESIAN_POINT ( 'NONE',  ( 200.1385401540174769, 283.9968752310148830, 17.30012534137638625 ) ) ;
#92935=CARTESIAN_POINT ( 'NONE',  ( 172.6505904036989136, 280.8448313155626579, -15.39888677054324440 ) ) ;
#92938=ORIENTED_EDGE ( 'NONE', *, *, #36360, .T. ) ;
#92939=CARTESIAN_POINT ( 'NONE',  ( 160.0767744118185476, 268.8186339879788989, -17.09306701113738569 ) ) ;
#92943=CARTESIAN_POINT ( 'NONE',  ( 163.9354095869165633, 246.7025367662834014, -7.289870401565430313 ) ) ;
#92945=CARTESIAN_POINT ( 'NONE',  ( 167.4568069247567905, 281.4715426663276503, 11.40307132674027457 ) ) ;
#92946=EDGE_CURVE ( 'NONE', #58975, #18309, #91979, .T. ) ;
#92947=CARTESIAN_POINT ( 'NONE',  ( 148.3629184514745987, 273.6748826132846375, -8.219814532462343948 ) ) ;
#92950=ORIENTED_EDGE ( 'NONE', *, *, #95434, .F. ) ;
#92953=DIRECTION ( 'NONE',  ( -0.8660254037844387076, -0.4999999999999998890, -0.000000000000000000 ) ) ;
#92955=CARTESIAN_POINT ( 'NONE',  ( 206.8495915765685140, 270.6470149864544510, 5.005496931752787759 ) ) ;
#92957=CARTESIAN_POINT ( 'NONE',  ( 147.2851682955343620, 275.5416006412388583, -4.045222947525739521 ) ) ;
#92958=CARTESIAN_POINT ( 'NONE',  ( 168.6819343819337575, 257.4928200986727234, -14.24392100367956893 ) ) ;
#92959=CARTESIAN_POINT ( 'NONE',  ( 206.8791291248445532, 272.3218326606039454, -10.16823074922856840 ) ) ;
#92963=AXIS2_PLACEMENT_3D ( 'NONE', #67190, #90551, #74827 ) ;
#92964=CARTESIAN_POINT ( 'NONE',  ( 171.3137948708142062, 255.5715404926284862, 11.21645684402445831 ) ) ;
#92965=CARTESIAN_POINT ( 'NONE',  ( 161.2178929573049402, 283.3531530028743077, 2.129142326282500886 ) ) ;
#92966=VERTEX_POINT ( 'NONE', #49710 ) ;
#92967=CARTESIAN_POINT ( 'NONE',  ( 194.5442727646457399, 293.6864305805324307, -14.41394159254472029 ) ) ;
#92969=CARTESIAN_POINT ( 'NONE',  ( 162.1461328301699609, 255.8963067295628662, -16.22074050756077668 ) ) ;
#92970=CARTESIAN_POINT ( 'NONE',  ( -4.037369169597886831, 175.1427522451419350, 10.00000000000009237 ) ) ;
#92971=CARTESIAN_POINT ( 'NONE',  ( 89.61940949045693117, 231.7369531367911009, -4.594050593750048428 ) ) ;
#92974=CARTESIAN_POINT ( 'NONE',  ( 163.5897630428932246, 247.3012141419924603, -7.420471801261374623 ) ) ;
#92976=CARTESIAN_POINT ( 'NONE',  ( 10.97399815293012892, 167.9548013555409796, -4.594050593750042211 ) ) ;
#92978=CARTESIAN_POINT ( 'NONE',  ( 161.1990332043106946, 251.4420796895884394, 14.26998817770995487 ) ) ;
#92979=ORIENTED_EDGE ( 'NONE', *, *, #88763, .T. ) ;
#92981=B_SPLINE_CURVE_WITH_KNOTS ( 'NONE', 3,
 ( #23029, #78262, #15425, #24041 ),
 .UNSPECIFIED., .F., .F.,
 ( 4, 4 ),
 ( 0.006441154778305856546, 0.01214362524711681476 ),
 .UNSPECIFIED. ) ;
#92982=CARTESIAN_POINT ( 'NONE',  ( 188.9125033604726411, 260.9492661745924238, -6.201642747674654288 ) ) ;
#92985=CARTESIAN_POINT ( 'NONE',  ( 205.1300674467857164, 275.3512963525735131, -12.60245643603069610 ) ) ;
#92986=CARTESIAN_POINT ( 'NONE',  ( 201.9828021040781891, 280.8025198310436394, -16.96692439557026688 ) ) ;
#92987=CARTESIAN_POINT ( 'NONE',  ( 185.5309115041763164, 286.5403957835872006, 16.01510129901755164 ) ) ;
#92989=CARTESIAN_POINT ( 'NONE',  ( 29.56604717072103483, 194.0024278399160949, 9.188101187500095079 ) ) ;
#92990=CARTESIAN_POINT ( 'NONE',  ( 125.6409139509397050, 243.3458772461660544, 9.188101187500095079 ) ) ;
#92991=CARTESIAN_POINT ( 'NONE',  ( 182.8698629865610030, 257.6187957884557136, -2.313844758695299042 ) ) ;
#92993=CARTESIAN_POINT ( 'NONE',  ( 153.4632062653391529, 273.9939398201073004, -11.95209943642215933 ) ) ;
#92994=EDGE_CURVE ( 'NONE', #74626, #51127, #30192, .T. ) ;
#92997=CARTESIAN_POINT ( 'NONE',  ( 197.5443661845914107, 266.8897665035560181, 8.689862809994204795 ) ) ;
#92998=CARTESIAN_POINT ( 'NONE',  ( 154.9910882912764123, 262.1945556895526579, 18.38052604520346023 ) ) ;
#92999=CARTESIAN_POINT ( 'NONE',  ( 161.5757715694810770, 250.7895496999525449, -14.51803553215175135 ) ) ;
#93001=CARTESIAN_POINT ( 'NONE',  ( 148.3025927079438304, 273.7793698660844939, -8.046026357031887954 ) ) ;
#93003=CARTESIAN_POINT ( 'NONE',  ( 164.6664072718354532, 249.8410913454628144, -10.49978785697552119 ) ) ;
#93004=CARTESIAN_POINT ( 'NONE',  ( 192.8633186137653865, 264.6749303248840306, 8.942253059790195024 ) ) ;
#93006=CARTESIAN_POINT ( 'NONE',  ( 148.1634546024981205, 274.0203641339852538, 9.324875965062235039 ) ) ;
#93007=CARTESIAN_POINT ( 'NONE',  ( 149.4596969528118393, 273.7752065243203106, 10.43958276706939614 ) ) ;
#93010=CARTESIAN_POINT ( 'NONE',  ( 182.9346993922109448, 268.7180793606257794, 15.07033917878656837 ) ) ;
#93011=CARTESIAN_POINT ( 'NONE',  ( 111.1353355333153843, 222.7202760586659167, -5.415160957724236172E-17 ) ) ;
#93013=CARTESIAN_POINT ( 'NONE',  ( 190.8623743139412454, 300.0636657654615647, 8.577953960666059530 ) ) ;
#93016=CARTESIAN_POINT ( 'NONE',  ( 195.0461724950329767, 279.0680765902233134, 16.30667399101714921 ) ) ;
#93017=CARTESIAN_POINT ( 'NONE',  ( 191.2176534171005926, 299.4483043079223421, -6.603228034478700437 ) ) ;
#93018=CARTESIAN_POINT ( 'NONE',  ( 191.2557879401978198, 261.3776189723048446, -4.694998167070893125 ) ) ;
#93019=FACE_OUTER_BOUND ( 'NONE', #5750, .T. ) ;
#93021=CARTESIAN_POINT ( 'NONE',  ( 192.4663556654298588, 297.2854885702906245, -12.98646995774174684 ) ) ;
#93023=ORIENTED_EDGE ( 'NONE', *, *, #33309, .T. ) ;
#93024=CARTESIAN_POINT ( 'NONE',  ( 193.0322577453413260, 267.1504813846829620, 11.29149517974427042 ) ) ;
#93026=CARTESIAN_POINT ( 'NONE',  ( 200.5156711751714909, 269.2042492623063481, 9.044317516942950164 ) ) ;
#93027=CARTESIAN_POINT ( 'NONE',  ( 149.7072529793668707, 271.3464269086063041, -11.98883662638834657 ) ) ;
#93028=ORIENTED_EDGE ( 'NONE', *, *, #35761, .F. ) ;
#93035=ORIENTED_EDGE ( 'NONE', *, *, #88325, .F. ) ;
#93039=CARTESIAN_POINT ( 'NONE',  ( 167.5352006701565415, 249.8483303177359858, 6.949831534123834587 ) ) ;
#93048=CARTESIAN_POINT ( 'NONE',  ( 112.8760603413013399, 242.6427522451419350, 10.00000000000009415 ) ) ;
#93053=CARTESIAN_POINT ( 'NONE',  ( 175.0972523130546676, 258.5006466257072475, 12.88669541573133159 ) ) ;
#93054=ORIENTED_EDGE ( 'NONE', *, *, #28525, .F. ) ;
#93057=CARTESIAN_POINT ( 'NONE',  ( 156.5497824763685912, 272.6770023486104719, 14.78669166138748814 ) ) ;
#93058=EDGE_LOOP ( 'NONE', ( #3837, #28620, #85484, #18548, #69199, #48870 ) ) ;
#93059=CARTESIAN_POINT ( 'NONE',  ( 165.5525849530957885, 274.9503981232618912, -15.45021171627992906 ) ) ;
#93061=CARTESIAN_POINT ( 'NONE',  ( 190.6281757562097710, 300.4693095665120381, 3.199750815899911505 ) ) ;
#93063=CARTESIAN_POINT ( 'NONE',  ( 147.1603453755519695, 275.7578002805973370, -5.230822882238410187 ) ) ;
#93064=CARTESIAN_POINT ( 'NONE',  ( 167.7603581743459813, 248.9573463932346158, -5.085697366910332029 ) ) ;
#93065=EDGE_CURVE ( 'NONE', #8119, #51824, #58016, .T. ) ;
#93067=CARTESIAN_POINT ( 'NONE',  ( 183.4229765504979923, 284.5723098315226025, -15.06534290927836572 ) ) ;
#93068=CARTESIAN_POINT ( 'NONE',  ( 119.3079296378835181, 245.8149278399160949, -9.188101187500095079 ) ) ;
#93071=CARTESIAN_POINT ( 'NONE',  ( 180.3975999145519324, 291.6145726629062551, -9.903595297598538849 ) ) ;
#93075=CARTESIAN_POINT ( 'NONE',  ( 180.4159519357722274, 256.0394304848937281, 1.308251353306819187 ) ) ;
#93076=CARTESIAN_POINT ( 'NONE',  ( 171.0865663407766704, 287.7261751874844435, -4.922011468251167088 ) ) ;
#93077=CARTESIAN_POINT ( 'NONE',  ( 146.7826225510319489, 276.4120354038443566, 2.803222021035590927 ) ) ;
#93082=ORIENTED_EDGE ( 'NONE', *, *, #65455, .T. ) ;
#93083=CARTESIAN_POINT ( 'NONE',  ( 148.2681081336820057, 273.8390989007832559, 10.43132051060321963 ) ) ;
#93085=VERTEX_POINT ( 'NONE', #12650 ) ;
#93089=CARTESIAN_POINT ( 'NONE',  ( 188.1067865297412709, 265.9162154355072971, -11.65400840555840567 ) ) ;
#93090=CARTESIAN_POINT ( 'NONE',  ( 156.8527937823772902, 276.5847309089942883, 10.20935908917872581 ) ) ;
#93091=CARTESIAN_POINT ( 'NONE',  ( 192.3892185349728265, 262.7068694540994898, 4.602004816464169146 ) ) ;
#93093=CARTESIAN_POINT ( 'NONE',  ( 204.6659862557271481, 272.9955293577589259, -9.800396827976472380 ) ) ;
#93094=CARTESIAN_POINT ( 'NONE',  ( 164.5092017753200935, 284.2060207574768356, -6.958017126009926834 ) ) ;
#93095=CARTESIAN_POINT ( 'NONE',  ( 157.9099320729108342, 280.2816496675481517, 5.725259973247741385 ) ) ;
#93096=CARTESIAN_POINT ( 'NONE',  ( 201.0732166862245549, 282.3779679885897167, -18.18766936363638820 ) ) ;
#93098=CARTESIAN_POINT ( 'NONE',  ( 204.6905575775918464, 272.9566935833489083, -9.732807054487977894 ) ) ;
#93103=CARTESIAN_POINT ( 'NONE',  ( 143.1652255295228997, 257.3466091724133094, -10.00000000000009770 ) ) ;
#93105=CARTESIAN_POINT ( 'NONE',  ( 188.5830972050926846, 298.6249682447369196, -4.133896775017286807 ) ) ;
#93109=EDGE_CURVE ( 'NONE', #19580, #99795, #4923, .T. ) ;
#93111=CARTESIAN_POINT ( 'NONE',  ( 194.2764122224708103, 294.1503786489221284, 15.46903869661980835 ) ) ;
#93112=CARTESIAN_POINT ( 'NONE',  ( 191.2589732073035975, 283.0812871616826669, -16.69315749097196289 ) ) ;
#93114=CARTESIAN_POINT ( 'NONE',  ( 75.92590343676303632, 205.4548013555409796, -4.594050593750042211 ) ) ;
#93115=CARTESIAN_POINT ( 'NONE',  ( 37.23771458502426412, 180.7592609112380444, 2.679491924311254714 ) ) ;
#93116=CARTESIAN_POINT ( 'NONE',  ( 147.5851099763508216, 275.0220864107570264, -4.372720440640867956 ) ) ;
#93118=EDGE_CURVE ( 'NONE', #86364, #90974, #53165, .T. ) ;
#93123=B_SPLINE_CURVE_WITH_KNOTS ( 'NONE', 3,
 ( #16647, #69349, #55130, #40433 ),
 .UNSPECIFIED., .F., .F.,
 ( 4, 4 ),
 ( 0.01401868009846423541, 0.02031335532182578993 ),
 .UNSPECIFIED. ) ;
#93128=CARTESIAN_POINT ( 'NONE',  ( 193.3641403297651777, 293.0000335917870871, 15.29877003740085861 ) ) ;
#93129=ADVANCED_FACE ( 'NONE', ( #99738 ), #45509, .T. ) ;
#93130=CARTESIAN_POINT ( 'NONE',  ( -0.4807448425718762741, 158.9824982072973683, 3.021315404115420679E-15 ) ) ;
#93131=CARTESIAN_POINT ( 'NONE',  ( 164.0223914878876883, 246.5518796944625421, -5.434886772145694600 ) ) ;
#93132=CARTESIAN_POINT ( 'NONE',  ( 157.4177733328310467, 257.9914139036126812, 18.29188238796808363 ) ) ;
#93133=CARTESIAN_POINT ( 'NONE',  ( 170.8926691088181542, 251.4534695730977774, 8.613095916456943613 ) ) ;
#93134=CARTESIAN_POINT ( 'NONE',  ( 161.8153478334749877, 250.3745914384277285, -14.21120979595050215 ) ) ;
#93135=CARTESIAN_POINT ( 'NONE',  ( 39.44458330234355969, 184.3923013555410080, 4.594050593750050204 ) ) ;
#93136=CARTESIAN_POINT ( 'NONE',  ( 55.54680928425421627, 209.0024278399160949, 9.188101187500095079 ) ) ;
#93140=CARTESIAN_POINT ( 'NONE',  ( -12.46307465703604400, 163.6115022471902591, 10.00000000000009592 ) ) ;
#93141=CARTESIAN_POINT ( 'NONE',  ( 197.4342445231449119, 270.1541731842395961, -10.85943118219619485 ) ) ;
#93144=CARTESIAN_POINT ( 'NONE',  ( 150.8168331730346949, 269.4245776381016526, -15.71017957295074652 ) ) ;
#93147=CARTESIAN_POINT ( 'NONE',  ( 69.62006919151632189, 204.8768266524159856, -9.188101187500093303 ) ) ;
#93150=CARTESIAN_POINT ( 'NONE',  ( 159.2876523829509665, 254.7526883847961017, 15.64395448151312351 ) ) ;
#93151=CARTESIAN_POINT ( 'NONE',  ( 59.27500801855438795, 193.4824982072973683, 3.021315404115420679E-15 ) ) ;
#93152=CARTESIAN_POINT ( 'NONE',  ( 149.1655084001637022, 275.4698895707030601, 7.593777017023739973 ) ) ;
#93157=CARTESIAN_POINT ( 'NONE',  ( 111.7394020023821781, 241.9865022471903160, 10.00000000000009237 ) ) ;
#93159=CARTESIAN_POINT ( 'NONE',  ( 164.4858674010174298, 245.7491158648375347, -2.958464974013825355 ) ) ;
#93160=ORIENTED_EDGE ( 'NONE', *, *, #2012, .T. ) ;
#93162=CARTESIAN_POINT ( 'NONE',  ( 184.6846741228996507, 271.1466850869315977, 16.33319160510210111 ) ) ;
#93163=EDGE_LOOP ( 'NONE', ( #22743, #3964, #79378, #92451, #32099 ) ) ;
#93164=CARTESIAN_POINT ( 'NONE',  ( 159.8597520197352537, 253.7617827468940277, -16.74905990210778839 ) ) ;
#93165=CARTESIAN_POINT ( 'NONE',  ( 190.3814439774240554, 278.7562814661916946, -16.51409031520932302 ) ) ;
#93168=CARTESIAN_POINT ( 'NONE',  ( 176.7695020951789218, 253.2860360199555316, -0.2578646269232350852 ) ) ;
#93169=EDGE_LOOP ( 'NONE', ( #4578, #57932 ) ) ;
#93171=CARTESIAN_POINT ( 'NONE',  ( 194.8598199529639317, 293.1398868181796615, -15.91766051364927570 ) ) ;
#93178=ORIENTED_EDGE ( 'NONE', *, *, #21160, .F. ) ;
#93179=CARTESIAN_POINT ( 'NONE',  ( 156.9440562780969231, 274.4750137900673508, 13.77464823823377316 ) ) ;
#93182=CARTESIAN_POINT ( 'NONE',  ( 174.6666250183130842, 286.3799292530254093, 11.61780681835062445 ) ) ;
#93185=CARTESIAN_POINT ( 'NONE',  ( 163.2000388741132895, 247.9762362032568035, -11.19676374274550312 ) ) ;
#93186=CARTESIAN_POINT ( 'NONE',  ( 204.9608076533459950, 275.6444629144898499, 14.31488288944633069 ) ) ;
#93187=CARTESIAN_POINT ( 'NONE',  ( 162.1260167985288376, 266.6785162637209510, 17.71249957499354366 ) ) ;
#93188=CARTESIAN_POINT ( 'NONE',  ( 204.6075833744878878, 276.2562653119390461, -13.34672481898815910 ) ) ;
#93190=CARTESIAN_POINT ( 'NONE',  ( 179.6160012257981862, 295.0481727651569486, 1.085779272287555663 ) ) ;
#93193=CARTESIAN_POINT ( 'NONE',  ( 195.6684633869053016, 291.3492540482502022, -15.70191374158172160 ) ) ;
#93194=CARTESIAN_POINT ( 'NONE',  ( 74.03095222233704931, 222.7369531367911293, -4.594050593750048428 ) ) ;
#93196=CARTESIAN_POINT ( 'NONE',  ( 151.2648146047323507, 268.6486510375538614, 15.71323890031163550 ) ) ;
#93199=CARTESIAN_POINT ( 'NONE',  ( 157.3433393808201117, 258.1203372903034960, -18.24816514480781393 ) ) ;
#93200=ORIENTED_EDGE ( 'NONE', *, *, #32915, .T. ) ;
#93201=ORIENTED_EDGE ( 'NONE', *, *, #30664, .T. ) ;
#93205=CARTESIAN_POINT ( 'NONE',  ( 147.2937583206075942, 275.5267222813735088, 0.1877253132609109920 ) ) ;
#93210=CARTESIAN_POINT ( 'NONE',  ( 83.09741599002914825, 218.7833772461660544, -9.188101187500095079 ) ) ;
#93215=ORIENTED_EDGE ( 'NONE', *, *, #65624, .F. ) ;
#93218=CARTESIAN_POINT ( 'NONE',  ( 164.5348324038273518, 245.6643059921780718, 1.473102934610569958 ) ) ;
#93220=CARTESIAN_POINT ( 'NONE',  ( 161.6936156625698970, 283.9059814617143047, 0.5218588777158598146 ) ) ;
#93221=CARTESIAN_POINT ( 'NONE',  ( 107.5536125507574354, 226.2365022471902876, 10.00000000000009948 ) ) ;
#93222=CARTESIAN_POINT ( 'NONE',  ( 188.2735287570237688, 299.1710073388255751, -5.251721556916531419 ) ) ;
#93227=CARTESIAN_POINT ( 'NONE',  ( 201.2139346379346705, 282.1342373466909521, -16.65315141107179286 ) ) ;
#93232=DIRECTION ( 'NONE',  ( -0.8660254037844387076, -0.4999999999999998890, -0.000000000000000000 ) ) ;
#93235=CARTESIAN_POINT ( 'NONE',  ( 29.10614472461704949, 177.6115022471902023, -5.000000000000041744 ) ) ;
#93236=CARTESIAN_POINT ( 'NONE',  ( 171.6377315803280794, 251.4568186439958879, 7.258662687126358648 ) ) ;
#93238=CARTESIAN_POINT ( 'NONE',  ( 156.3322239406982703, 272.0717997662977155, 14.16949642306787815 ) ) ;
#93239=EDGE_CURVE ( 'NONE', #50293, #56647, #16916, .T. ) ;
#93245=CARTESIAN_POINT ( 'NONE',  ( 207.6727254509676186, 270.9472835030587703, 7.315149605389819953 ) ) ;
#93246=CARTESIAN_POINT ( 'NONE',  ( 178.8595466249924755, 265.0989930076032124, -16.03772641351113748 ) ) ;
#93248=CARTESIAN_POINT ( 'NONE',  ( 61.50992858288473286, 212.9865022471902876, -10.00000000000009592 ) ) ;
#93251=CARTESIAN_POINT ( 'NONE',  ( 168.5245981071017809, 273.3323447180702033, 16.01708071253985111 ) ) ;
#93252=CARTESIAN_POINT ( 'NONE',  ( 166.4096179326797937, 285.9983886822901127, -3.191241580084798191 ) ) ;
#93254=CARTESIAN_POINT ( 'NONE',  ( 188.4600153102442732, 260.9481083049865902, 2.870696243003649339 ) ) ;
#93255=CARTESIAN_POINT ( 'NONE',  ( 207.3646600298985447, 271.4808684644054324, -5.284084612275558257 ) ) ;
#93256=CARTESIAN_POINT ( 'NONE',  ( 7.753205860782987457, 175.2833772461660544, -9.188101187500095079 ) ) ;
#93257=DIRECTION ( 'NONE',  ( -0.8660254037844387076, -0.4999999999999998890, -0.000000000000000000 ) ) ;
#93259=CARTESIAN_POINT ( 'NONE',  ( 174.8608349436526055, 255.3260918886272179, 8.528007662106622533 ) ) ;
#93262=CARTESIAN_POINT ( 'NONE',  ( 23.55782238408398044, 196.6589784336661353, -6.496448406907676862E-16 ) ) ;
#93266=CARTESIAN_POINT ( 'NONE',  ( 103.1513167481865310, 230.3615022471902591, -10.00000000000009592 ) ) ;
#93267=CARTESIAN_POINT ( 'NONE',  ( 134.1658515176688127, 258.2677522451419350, -5.000000000000047962 ) ) ;
#93269=CARTESIAN_POINT ( 'NONE',  ( 188.3805762680232192, 260.4081077799571631, -0.7596527320232882019 ) ) ;
#93270=CARTESIAN_POINT ( 'NONE',  ( 64.18017357788677657, 207.8615022471902307, -10.00000000000009592 ) ) ;
#93272=CARTESIAN_POINT ( 'NONE',  ( 206.5545904789651388, 271.4197609012314274, 6.179362329135090981 ) ) ;
#93273=CARTESIAN_POINT ( 'NONE',  ( 35.84507844392322085, 185.3768266524159856, -9.188101187500091527 ) ) ;
#93275=EDGE_CURVE ( 'NONE', #23755, #45951, #2143, .T. ) ;
#93277=CARTESIAN_POINT ( 'NONE',  ( 203.9116033662877783, 270.5127528292231318, -6.455590966117181750 ) ) ;
#93279=CARTESIAN_POINT ( 'NONE',  ( 151.1230807375396807, 268.8941412966845519, -14.26613110909109849 ) ) ;
#93282=CARTESIAN_POINT ( 'NONE',  ( 159.9029087581434396, 278.3966458521681488, -10.39982288579484582 ) ) ;
#93285=CARTESIAN_POINT ( 'NONE',  ( 189.9052851100924215, 301.7213928939034986, -1.077181946533001256 ) ) ;
#93288=CARTESIAN_POINT ( 'NONE',  ( 174.7028696250029043, 256.5417377999049222, 12.02695302890117546 ) ) ;
#93291=AXIS2_PLACEMENT_3D ( 'NONE', #59018, #89988, #88519 ) ;
#93295=ORIENTED_EDGE ( 'NONE', *, *, #54975, .T. ) ;
#93299=CARTESIAN_POINT ( 'NONE',  ( 150.6453220160077251, 269.7216436761371483, 14.94145576020818034 ) ) ;
#93300=CARTESIAN_POINT ( 'NONE',  ( 172.5992896740868616, 281.6695515350652954, -14.94842763437895350 ) ) ;
#93302=ORIENTED_EDGE ( 'NONE', *, *, #26826, .T. ) ;
#93303=CARTESIAN_POINT ( 'NONE',  ( 186.5384767560921091, 272.2703538590346852, -15.99658917633080613 ) ) ;
#93305=ORIENTED_EDGE ( 'NONE', *, *, #78804, .T. ) ;
#93306=CARTESIAN_POINT ( 'NONE',  ( 201.4520623681621316, 281.7217880192456505, -17.56577389517433119 ) ) ;
#93310=CARTESIAN_POINT ( 'NONE',  ( 189.8763472015711216, 301.7715148217271803, -0.1184663095182975079 ) ) ;
#93311=EDGE_CURVE ( 'NONE', #75967, #8895, #91636, .T. ) ;
#93312=CARTESIAN_POINT ( 'NONE',  ( 196.4501996009505831, 290.3852684645433442, -17.82325615854289680 ) ) ;
#93315=CARTESIAN_POINT ( 'NONE',  ( 156.5497824763685912, 272.6770023486104719, 14.78669166138748814 ) ) ;
#93317=CARTESIAN_POINT ( 'NONE',  ( 162.0238244467804805, 266.8515061766926237, 16.62455803315057068 ) ) ;
#93320=CARTESIAN_POINT ( 'NONE',  ( 190.3572031550745294, 300.9386478791372497, 3.093832330100951378 ) ) ;
#93326=CARTESIAN_POINT ( 'NONE',  ( 150.3774144590728952, 270.1856731764797814, 13.91914410364283938 ) ) ;
#93331=CARTESIAN_POINT ( 'NONE',  ( 185.5036743169331430, 269.5266205919543268, -16.28606374402843571 ) ) ;
#93332=CARTESIAN_POINT ( 'NONE',  ( 147.3023124603499809, 275.5119060767245287, 5.196938859334171212 ) ) ;
#93333=CARTESIAN_POINT ( 'NONE',  ( 190.6071113721798156, 300.5057941498820924, -0.4754021072632813594 ) ) ;
#93334=ORIENTED_EDGE ( 'NONE', *, *, #92773, .T. ) ;
#93335=CARTESIAN_POINT ( 'NONE',  ( 149.0802055316563326, 272.4325049467973940, 12.84384348890831085 ) ) ;
#93336=CARTESIAN_POINT ( 'NONE',  ( 174.1990609491486737, 253.0008501898304871, 8.022018053261177783 ) ) ;
#93338=CARTESIAN_POINT ( 'NONE',  ( 192.4335622838504207, 297.3422883733380786, -12.83044365323471325 ) ) ;
#93339=CARTESIAN_POINT ( 'NONE',  ( 163.9961211234992788, 256.9275610305372766, 16.20495027727189807 ) ) ;
#93341=CARTESIAN_POINT ( 'NONE',  ( 164.3754245770190039, 245.9404084473339083, 1.667926061651832992 ) ) ;
#93345=CARTESIAN_POINT ( 'NONE',  ( 100.7694865641816051, 238.1744531367911293, 4.594050593750047540 ) ) ;
#93347=CARTESIAN_POINT ( 'NONE',  ( 191.6723191112861855, 298.6608002251342100, -9.737039817265848995 ) ) ;
#93350=CARTESIAN_POINT ( 'NONE',  ( 203.5080190724872011, 278.1607665491929993, -15.47044080916498743 ) ) ;
#93352=CARTESIAN_POINT ( 'NONE',  ( 163.9704062730716032, 246.6419207277664327, 7.317582738093436845 ) ) ;
#93356=CARTESIAN_POINT ( 'NONE',  ( 208.1612901671020381, 270.1010645919285480, -2.401583477149568768 ) ) ;
#93359=CARTESIAN_POINT ( 'NONE',  ( 206.1542244435759983, 272.8725460781796528, 8.903176382340632244 ) ) ;
#93360=CARTESIAN_POINT ( 'NONE',  ( 127.1021582719434662, 250.3149278399160949, -9.188101187500095079 ) ) ;
#93361=CARTESIAN_POINT ( 'NONE',  ( 156.6812872898450735, 261.2670451491295012, 0.000000000000000000 ) ) ;
#93362=CARTESIAN_POINT ( 'NONE',  ( 186.0639839519483019, 296.8412207699221881, 4.661798123928299731 ) ) ;
#93363=CARTESIAN_POINT ( 'NONE',  ( 157.5520850189458884, 257.7587792392113215, 16.71892742266126319 ) ) ;
#93364=DIRECTION ( 'NONE',  ( -0.8660254037844392627, -0.4999999999999987232, 0.000000000000000000 ) ) ;
#93365=CARTESIAN_POINT ( 'NONE',  ( 54.19381813872350762, 202.0958772461660544, -9.188101187500095079 ) ) ;
#93367=AXIS2_PLACEMENT_3D ( 'NONE', #78469, #39424, #84591 ) ;
#93371=B_SPLINE_CURVE_WITH_KNOTS ( 'NONE', 3,
 ( #75152, #96485, #36617, #58908, #4233, #67525, #59918, #13830, #3758, #98455 ),
 .UNSPECIFIED., .F., .F.,
 ( 4, 2, 2, 2, 4 ),
 ( 3.453764301715650149E-15, 0.0004337349686803219548, 0.0008674699373571900752, 0.001301204906034058358, 0.001734939874710926533 ),
 .UNSPECIFIED. ) ;
#93373=EDGE_CURVE ( 'NONE', #99290, #11051, #31256, .T. ) ;
#93374=B_SPLINE_SURFACE_WITH_KNOTS ( 'NONE', 3, 1, ( 
 ( #26052, #64543 ),
 ( #56925, #87913 ),
 ( #47327, #18456 ),
 ( #10852, #72672 ),
 ( #3265, #50329 ),
 ( #81280, #28026 ),
 ( #74659, #49838 ),
 ( #36115, #96480 ),
 ( #75146, #80795 ),
 ( #88404, #11372 ),
 ( #97458, #11854 ),
 ( #96983, #73161 ),
 ( #50823, #67019 ),
 ( #42223, #81773 ),
 ( #57425, #97946 ),
 ( #58901, #43212 ),
 ( #82779, #89871 ),
 ( #51839, #12857 ),
 ( #43715, #20446 ),
 ( #89396, #57930 ),
 ( #3753, #26551 ),
 ( #27554, #12346 ),
 ( #51315, #66532 ),
 ( #34631, #28519 ),
 ( #90379, #82284 ),
 ( #44211, #19947 ),
 ( #65531, #58420 ),
 ( #27048, #59402 ),
 ( #5237, #88912 ),
 ( #19472, #95989 ),
 ( #42711, #73645 ),
 ( #4226, #35126 ),
 ( #66036, #74155 ),
 ( #4747, #20956 ) ),
 .UNSPECIFIED., .T., .F., .F.,
 ( 4, 2, 2, 2, 2, 2, 2, 2, 2, 2, 2, 2, 2, 2, 2, 2, 4 ),
 ( 2, 2 ),
 ( 0.000000000000000000, 0.06250000000000000000, 0.1250000000000000000, 0.1875000000000000000, 0.2500000000000000000, 0.3125000000000000000, 0.3750000000000000000, 0.4375000000000000000, 0.5000000000000000000, 0.5625000000000000000, 0.6250000000000000000, 0.6875000000000000000, 0.7500000000000000000, 0.8125000000000000000, 0.8750000000000000000, 0.9375000000000000000, 1.000000000000000000 ),
 ( 0.000000000000000000, 1.000000000000000000 ),
 .UNSPECIFIED. ) ;
#93376=CARTESIAN_POINT ( 'NONE',  ( 174.6105168250273323, 262.0571681988877799, 14.27631620660720735 ) ) ;
#93378=CARTESIAN_POINT ( 'NONE',  ( 203.4357368910538355, 278.2859629599173559, -16.45855118664066197 ) ) ;
#93379=CARTESIAN_POINT ( 'NONE',  ( 153.6187353439852075, 269.2963960243311021, -15.64461193481829504 ) ) ;
#93381=CARTESIAN_POINT ( 'NONE',  ( 108.1850894041357094, 223.2677522451417929, -5.000000000000041744 ) ) ;
#93382=CARTESIAN_POINT ( 'NONE',  ( 194.2385081474906769, 292.6568478422810244, -15.46372919447845362 ) ) ;
#93383=ORIENTED_EDGE ( 'NONE', *, *, #85122, .F. ) ;
#93384=CARTESIAN_POINT ( 'NONE',  ( 162.8789161433191452, 248.5324370884573568, 9.731756914259689140 ) ) ;
#93385=DIRECTION ( 'NONE',  ( -0.8660254037844387076, -0.4999999999999998890, -0.000000000000000000 ) ) ;
#93387=CARTESIAN_POINT ( 'NONE',  ( 27.99689677000926125, 174.7202760586659736, -5.415160957724236172E-17 ) ) ;
#93393=CARTESIAN_POINT ( 'NONE',  ( 198.2212904662371500, 277.5279118919263510, -15.45398242064391781 ) ) ;
#93394=CARTESIAN_POINT ( 'NONE',  ( 68.53719034102077501, 216.5024278399160664, 9.188101187500095079 ) ) ;
#93395=CARTESIAN_POINT ( 'NONE',  ( 161.3193951073452581, 251.2336067582368742, 13.01220207292984377 ) ) ;
#93396=CARTESIAN_POINT ( 'NONE',  ( 174.5315600938332921, 289.3520206179668435, 7.862896886311159683 ) ) ;
#93399=ORIENTED_EDGE ( 'NONE', *, *, #24354, .T. ) ;
#93400=B_SPLINE_CURVE_WITH_KNOTS ( 'NONE', 3,
 ( #39588, #16313, #26296, #87665 ),
 .UNSPECIFIED., .F., .F.,
 ( 4, 4 ),
 ( 0.01540896664962445803, 0.02418941936981118535 ),
 .UNSPECIFIED. ) ;
#93401=( BOUNDED_CURVE ( )  B_SPLINE_CURVE ( 2, ( #49859, #80309, #2795, #18989, #66556, #80825, #50849, #43240, #3291 ),
 .UNSPECIFIED., .F., .T. ) 
 B_SPLINE_CURVE_WITH_KNOTS ( ( 3, 2, 2, 2, 3 ),
 ( 0.7137096774193548709, 0.7150537634408602461, 0.7177419354838709964, 0.7204301075268817467, 0.7217741935483871218 ),
 .UNSPECIFIED. ) 
 CURVE ( )  GEOMETRIC_REPRESENTATION_ITEM ( )  RATIONAL_B_SPLINE_CURVE ( ( 0.9330127018922194093, 0.9330127018922194093, 1.000000000000000000, 0.8660254037844387076, 1.000000000000000000, 0.8660254037844387076, 1.000000000000000000, 0.9330127018922194093, 0.9330127018922194093 ) ) 
 REPRESENTATION_ITEM ( '' )  );
#93402=CARTESIAN_POINT ( 'NONE',  ( 163.2842962196203302, 267.9677010721593433, 16.49754710497367682 ) ) ;
#93403=CARTESIAN_POINT ( 'NONE',  ( 23.40481081636943017, 190.9865022471903160, 10.00000000000009237 ) ) ;
#93404=CARTESIAN_POINT ( 'NONE',  ( 34.06774859691741142, 197.1427522451419350, -10.00000000000009592 ) ) ;
#93405=VECTOR ( 'NONE', #38251, 1000.000000000000000 ) ;
#93406=CARTESIAN_POINT ( 'NONE',  ( 162.9466247808429102, 248.4151622881552441, 11.25765811906727443 ) ) ;
#93407=CARTESIAN_POINT ( 'NONE',  ( -3.126064726376516667, 162.8768266524159856, -9.188101187500091527 ) ) ;
#93409=CARTESIAN_POINT ( 'NONE',  ( 168.6534459294139481, 262.6503232764572431, 15.96541089746672171 ) ) ;
#93411=CARTESIAN_POINT ( 'NONE',  ( 185.3010781374966882, 260.3148984547196960, 6.941109534206622911 ) ) ;
#93412=CARTESIAN_POINT ( 'NONE',  ( 205.7639495959071212, 274.2533802642843170, 10.79039487422292432 ) ) ;
#93413=CARTESIAN_POINT ( 'NONE',  ( 183.1769575194604158, 257.7542008109865037, -2.146814141465986481 ) ) ;
#93417=CARTESIAN_POINT ( 'NONE',  ( 176.2544971312975974, 263.4220703943961439, 15.96855061784746610 ) ) ;
#93418=CARTESIAN_POINT ( 'NONE',  ( 178.5167212123578224, 285.5003866454536023, 13.01602787300356923 ) ) ;
#93419=CARTESIAN_POINT ( 'NONE',  ( 156.1933712160320908, 280.4387541887718953, -5.510142736702231758 ) ) ;
#93422=CARTESIAN_POINT ( 'NONE',  ( 159.9681198662056545, 253.5740841309004452, 14.91312641984554688 ) ) ;
#93423=CARTESIAN_POINT ( 'NONE',  ( 157.7847820078105201, 257.3557362317297361, -18.02899742403477035 ) ) ;
#93424=FACE_OUTER_BOUND ( 'NONE', #77719, .T. ) ;
#93428=CARTESIAN_POINT ( 'NONE',  ( 207.8136982414359579, 270.7031114674828700, -0.9536989003868096004 ) ) ;
#93429=CARTESIAN_POINT ( 'NONE',  ( 152.6692142062575499, 266.2161595735824449, -16.77985299603479419 ) ) ;
#93437=ORIENTED_EDGE ( 'NONE', *, *, #26945, .F. ) ;
#93440=CARTESIAN_POINT ( 'NONE',  ( 30.69616969366791537, 176.9824982072973967, 3.021315404115420679E-15 ) ) ;
#93443=VERTEX_POINT ( 'NONE', #10033 ) ;
#93444=CARTESIAN_POINT ( 'NONE',  ( 203.3278261089206183, 278.4728699172566735, 16.54899263865330994 ) ) ;
#93446=CARTESIAN_POINT ( 'NONE',  ( 150.6453220160077251, 269.7216436761371483, 14.94145576020818034 ) ) ;
#93449=ORIENTED_EDGE ( 'NONE', *, *, #87184, .T. ) ;
#93451=CARTESIAN_POINT ( 'NONE',  ( 160.2402339746914777, 268.8803885730948195, -16.99231777190169623 ) ) ;
#93452=VERTEX_POINT ( 'NONE', #73822 ) ;
#93455=ORIENTED_EDGE ( 'NONE', *, *, #3560, .F. ) ;
#93456=CARTESIAN_POINT ( 'NONE',  ( 163.8947349411736525, 246.7729873192901664, -5.868803394723933309 ) ) ;
#93459=ADVANCED_FACE ( 'NONE', ( #64220 ), #35428, .F. ) ;
#93460=CARTESIAN_POINT ( 'NONE',  ( 165.3974121193675160, 271.2591920438384818, 17.13699628004796693 ) ) ;
#93463=CARTESIAN_POINT ( 'NONE',  ( 147.9311236323648870, 274.4227731784279172, -7.799459659034405412 ) ) ;
#93464=DIRECTION ( 'NONE',  ( -0.8660254037844387076, -0.4999999999999998890, -0.000000000000000000 ) ) ;
#93465=DIRECTION ( 'NONE',  ( -0.8660254037844387076, -0.4999999999999998890, -0.000000000000000000 ) ) ;
#93466=CARTESIAN_POINT ( 'NONE',  ( 166.3150859005863254, 247.0070523979024983, 1.903668903753348518 ) ) ;
#93468=CARTESIAN_POINT ( 'NONE',  ( 178.0302064638906074, 292.4640037680099454, 7.106335582765731296 ) ) ;
#93470=CARTESIAN_POINT ( 'NONE',  ( 159.2554912534056939, 254.8083930951974878, 16.49944922174842432 ) ) ;
#93472=AXIS2_PLACEMENT_3D ( 'NONE', #16426, #86392, #94469 ) ;
#93473=DIRECTION ( 'NONE',  ( -0.8660254037844387076, -0.4999999999999998890, -0.000000000000000000 ) ) ;
#93474=CARTESIAN_POINT ( 'NONE',  ( 160.0061168334508750, 253.5082714530983026, -16.02306982074888708 ) ) ;
#93477=CARTESIAN_POINT ( 'NONE',  ( 200.7523954295751594, 282.9336467052548869, 18.23634913067694185 ) ) ;
#93478=VERTEX_POINT ( 'NONE', #74840 ) ;
#93479=CARTESIAN_POINT ( 'NONE',  ( 155.1126062595885458, 261.9840803944032359, -18.37531408727430104 ) ) ;
#93480=CARTESIAN_POINT ( 'NONE',  ( 134.1658515176688411, 248.2677522451418497, 10.00000000000009592 ) ) ;
#93481=CARTESIAN_POINT ( 'NONE',  ( 179.9645220515723167, 295.2954571389396392, -0.1274745643057336175 ) ) ;
#93482=CARTESIAN_POINT ( 'NONE',  ( 25.04665064082957926, 175.2677522451417929, -5.000000000000041744 ) ) ;
#93483=CARTESIAN_POINT ( 'NONE',  ( 90.02596631606968458, 210.5327760586659451, 1.948934522072302763E-15 ) ) ;
#93484=CARTESIAN_POINT ( 'NONE',  ( 196.4287751515431921, 269.1031666285815618, -12.09581130873691279 ) ) ;
#93485=CARTESIAN_POINT ( 'NONE',  ( 174.5193869908134445, 282.4549705599221170, -14.99235812395697920 ) ) ;
#93486=CARTESIAN_POINT ( 'NONE',  ( 166.9537089176444624, 278.1996852497881605, -13.41525378165041182 ) ) ;
#93487=CARTESIAN_POINT ( 'NONE',  ( 1.754175721758462148, 178.4865022471903728, -10.00000000000009592 ) ) ;
#93488=CARTESIAN_POINT ( 'NONE',  ( 9.512059640396367755, 185.4869531367911293, 4.594050593750046652 ) ) ;
#93490=CARTESIAN_POINT ( 'NONE',  ( 200.2316334480823912, 283.8356329158505105, 17.02791935830326508 ) ) ;
#93492=ORIENTED_EDGE ( 'NONE', *, *, #60881, .T. ) ;
#93494=CARTESIAN_POINT ( 'NONE',  ( 200.9031254216535842, 267.7938560626140543, -2.960348916509118578 ) ) ;
#93497=CARTESIAN_POINT ( 'NONE',  ( 161.1061647010182583, 251.6029326557136585, -13.56144933775657613 ) ) ;
#93500=CARTESIAN_POINT ( 'NONE',  ( 33.19304919271588972, 177.7202760586659451, -5.415160957724236172E-17 ) ) ;
#93502=CARTESIAN_POINT ( 'NONE',  ( 196.1313296246206619, 275.4698387032307778, 15.47109719661084704 ) ) ;
#93504=CARTESIAN_POINT ( 'NONE',  ( 153.3327503926682596, 274.2549037607562354, -12.22769268488517902 ) ) ;
#93505=CARTESIAN_POINT ( 'NONE',  ( 182.5206069704653089, 260.8428654270882134, -10.69627834319913795 ) ) ;
#93506=AXIS2_PLACEMENT_3D ( 'NONE', #4468, #81027, #97207 ) ;
#93507=EDGE_CURVE ( 'NONE', #53063, #83615, #35029, .T. ) ;
#93508=CARTESIAN_POINT ( 'NONE',  ( -16.57695564860984661, 170.4244531367911293, -4.594050593750046652 ) ) ;
#93509=CARTESIAN_POINT ( 'NONE',  ( 196.0051728737935832, 265.8263463907475170, 8.406970388261065352 ) ) ;
#93511=CARTESIAN_POINT ( 'NONE',  ( 194.2199708651012600, 294.2481379475345875, 15.50834247347371253 ) ) ;
#93512=CARTESIAN_POINT ( 'NONE',  ( 161.2133744761260061, 251.4172398781588811, -14.30368667312104058 ) ) ;
#93513=FACE_OUTER_BOUND ( 'NONE', #65762, .T. ) ;
#93514=CARTESIAN_POINT ( 'NONE',  ( 194.9455394410084921, 292.9914163096879065, -15.01116663483170655 ) ) ;
#93515=CARTESIAN_POINT ( 'NONE',  ( 189.3832291599495079, 300.6256203239445313, 1.753828516883770838 ) ) ;
#93517=CARTESIAN_POINT ( 'NONE',  ( 193.0126352936363503, 264.4189281174865869, 8.906082567666748773 ) ) ;
#93520=CARTESIAN_POINT ( 'NONE',  ( 181.4735074999749145, 292.1586133693310785, 10.55809797880889001 ) ) ;
#93522=CARTESIAN_POINT ( 'NONE',  ( 173.9008529106967558, 272.4049662731551962, -17.79092985220220058 ) ) ;
#93523=EDGE_CURVE ( 'NONE', #86318, #82867, #73810, .T. ) ;
#93524=CARTESIAN_POINT ( 'NONE',  ( 114.2743305262689404, 236.7833772461660544, -9.188101187500095079 ) ) ;
#93526=CARTESIAN_POINT ( 'NONE',  ( 150.8888667059421209, 269.2998118992572927, 15.79021133717968617 ) ) ;
#93531=CARTESIAN_POINT ( 'NONE',  ( 151.0170062819612440, 269.0778676431315830, -14.83004665419763946 ) ) ;
#93532=CARTESIAN_POINT ( 'NONE',  ( 190.8403443996919293, 262.5132785920529273, -4.370171634604190558 ) ) ;
#93538=CARTESIAN_POINT ( 'NONE',  ( 191.8538237116409846, 266.9476526621388643, 10.93440350035595365 ) ) ;
#93540=CARTESIAN_POINT ( 'NONE',  ( 200.4850423784957343, 269.2554961546323398, 9.006584850389378616 ) ) ;
#93541=B_SPLINE_CURVE_WITH_KNOTS ( 'NONE', 3,
 ( #97507, #28078, #58949, #39642, #62966, #15347, #22959, #70055, #85314, #54862, #69567, #70563, #85841, #47262, #23451, #84807, #15860, #7771, #16370, #46767, #77693, #71092, #54343, #53847, #8276, #47751, #92899, #38145, #86327, #39143, #671, #46243, #78184, #55349, #175, #31554, #14863, #77168, #62443, #38664, #61461, #93916, #93411, #31058, #24469, #55838, #61948, #16865, #23960, #8772, #1180, #32055 ),
 .UNSPECIFIED., .F., .F.,
 ( 4, 2, 2, 2, 2, 2, 2, 2, 2, 2, 2, 2, 2, 2, 2, 2, 2, 2, 2, 2, 2, 2, 2, 2, 2, 4 ),
 ( 0.0001062343114664006984, 0.001128839385260167923, 0.001384490653708566167, 0.001640141922156964412, 0.001767967556381141525, 0.001895793190605319072, 0.002023618824829496402, 0.002151444459053673732, 0.002407095727502028826, 0.002662746995950384787, 0.003174049532847176506, 0.004196654606640761245, 0.005219259680434346418, 0.005730562217331175434, 0.005986213485779591677, 0.006114039120003762935, 0.006241864754227933326, 0.006305777571339981659, 0.006369690388452029124, 0.006497516022676135330, 0.006753167291124355549, 0.007008818559572576636, 0.007264469828020798589, 0.007520121096469019675, 0.007775772364917239894, 0.008287074901813495584 ),
 .UNSPECIFIED. ) ;
#93543=CARTESIAN_POINT ( 'NONE',  ( 180.3992865667702574, 261.8415815662849013, -12.99249967246676718 ) ) ;
#93544=CARTESIAN_POINT ( 'NONE',  ( 168.8668831836475590, 259.3240382218725131, -16.04453771237437110 ) ) ;
#93549=ORIENTED_EDGE ( 'NONE', *, *, #51096, .F. ) ;
#93550=CARTESIAN_POINT ( 'NONE',  ( 167.4359517046813437, 249.7873561267534512, 6.955981803495778770 ) ) ;
#93551=CARTESIAN_POINT ( 'NONE',  ( 148.5272680744187141, 275.3902207161408455, -7.185975151065171929 ) ) ;
#93553=ORIENTED_EDGE ( 'NONE', *, *, #16780, .T. ) ;
#93555=CARTESIAN_POINT ( 'NONE',  ( 159.1045919238213457, 255.0697584008655383, 17.12809966849329513 ) ) ;
#93556=DIRECTION ( 'NONE',  ( -0.8660254037844387076, -0.4999999999999998890, -0.000000000000000000 ) ) ;
#93560=ORIENTED_EDGE ( 'NONE', *, *, #88565, .T. ) ;
#93562=CARTESIAN_POINT ( 'NONE',  ( 167.6502826215564994, 287.3877002845107995, 4.891367078714356609 ) ) ;
#93566=CARTESIAN_POINT ( 'NONE',  ( 170.9560043375414864, 269.9813116362016103, 16.58206790160089383 ) ) ;
#93570=CARTESIAN_POINT ( 'NONE',  ( 206.6672608846700427, 272.6887992170966299, -10.88770374553082121 ) ) ;
#93571=CARTESIAN_POINT ( 'NONE',  ( 147.9415534642045884, 274.4047081797672263, -6.588256216760665751 ) ) ;
#93572=CARTESIAN_POINT ( 'NONE',  ( 148.9230895364621574, 272.7046378331555161, 12.20434325797056019 ) ) ;
#93576=EDGE_CURVE ( 'NONE', #64387, #48406, #84445, .T. ) ;
#93578=CARTESIAN_POINT ( 'NONE',  ( 157.9640733854634789, 281.0222844342897588, 2.394995417900620982 ) ) ;
#93579=CARTESIAN_POINT ( 'NONE',  ( 124.5040820605901217, 248.8149278399161233, -9.188101187500095079 ) ) ;
#93583=AXIS2_PLACEMENT_3D ( 'NONE', #40458, #87654, #9596 ) ;
#93586=FACE_OUTER_BOUND ( 'NONE', #71096, .T. ) ;
#93587=CARTESIAN_POINT ( 'NONE',  ( 173.3788830315178870, 289.3113284895608217, -4.680553739743101183 ) ) ;
#93588=CARTESIAN_POINT ( 'NONE',  ( 192.2557068912079501, 297.6503429497950037, 11.10070071572538275 ) ) ;
#93591=CARTESIAN_POINT ( 'NONE',  ( 173.3932497502476906, 287.2264128176810800, -9.697408833419370211 ) ) ;
#93593=CARTESIAN_POINT ( 'NONE',  ( 173.8830265265375772, 282.0958691128189457, 14.99492924356757584 ) ) ;
#93594=CARTESIAN_POINT ( 'NONE',  ( 194.5253693406981483, 291.7191722712467481, 16.18900132190417551 ) ) ;
#93596=ORIENTED_EDGE ( 'NONE', *, *, #8317, .F. ) ;
#93597=CARTESIAN_POINT ( 'NONE',  ( 148.0637215040603394, 274.1931069276759558, -7.795633835291665648 ) ) ;
#93598=CARTESIAN_POINT ( 'NONE',  ( 4.262040950002970341, 183.2677522451419065, -5.000000000000047962 ) ) ;
#93599=VERTEX_POINT ( 'NONE', #78820 ) ;
#93600=CARTESIAN_POINT ( 'NONE',  ( 188.0563983182514960, 266.0109151943670440, -11.70562387175789532 ) ) ;
#93602=CARTESIAN_POINT ( 'NONE',  ( 152.4236611112960986, 266.6414700100113464, -15.70435633784547669 ) ) ;
#93604=CARTESIAN_POINT ( 'NONE',  ( 153.4476745504623239, 270.0653357872154174, 15.15442168775317278 ) ) ;
#93605=CARTESIAN_POINT ( 'NONE',  ( 154.8984264370756136, 277.3990238811145446, -8.847142293553330816 ) ) ;
#93606=CARTESIAN_POINT ( 'NONE',  ( 152.7295469705997277, 266.1116601603806657, -17.40211458100010589 ) ) ;
#93608=CARTESIAN_POINT ( 'NONE',  ( 146.8195026170398023, 276.3481572557323034, 4.765869558735466249 ) ) ;
#93609=B_SPLINE_SURFACE_WITH_KNOTS ( 'NONE', 3, 1, ( 
 ( #702, #23997 ),
 ( #39176, #32090 ),
 ( #77725, #31586 ),
 ( #16894, #54895 ),
 ( #46280, #85875 ),
 ( #63003, #93947 ),
 ( #47294, #24501 ),
 ( #9308, #22994 ),
 ( #47785, #71122 ),
 ( #31092, #38696 ),
 ( #60993, #61979 ),
 ( #92933, #22508 ),
 ( #53402, #84351 ),
 ( #45787, #23485 ),
 ( #38183, #54375 ),
 ( #40688, #96446 ),
 ( #71628, #17921 ),
 ( #72122, #34119 ),
 ( #2223, #10316 ),
 ( #49802, #42193 ),
 ( #65012, #80763 ),
 ( #73128, #27013 ),
 ( #64001, #11822 ),
 ( #63502, #33104 ),
 ( #48819, #95956 ),
 ( #3721, #72635 ),
 ( #94942, #11334 ),
 ( #34599, #10816 ),
 ( #57897, #2727 ),
 ( #25506, #94440 ),
 ( #65498, #88877 ),
 ( #79752, #24994 ),
 ( #41692, #41185 ),
 ( #1726, #50294 ) ),
 .UNSPECIFIED., .T., .F., .F.,
 ( 4, 2, 2, 2, 2, 2, 2, 2, 2, 2, 2, 2, 2, 2, 2, 2, 4 ),
 ( 2, 2 ),
 ( 0.000000000000000000, 0.06250000000000000000, 0.1250000000000000000, 0.1875000000000000000, 0.2500000000000000000, 0.3125000000000000000, 0.3750000000000000000, 0.4375000000000000000, 0.5000000000000000000, 0.5625000000000000000, 0.6250000000000000000, 0.6875000000000000000, 0.7500000000000000000, 0.8125000000000000000, 0.8750000000000000000, 0.9375000000000000000, 1.000000000000000000 ),
 ( 0.000000000000000000, 1.000000000000000000 ),
 .UNSPECIFIED. ) ;
#93612=CARTESIAN_POINT ( 'NONE',  ( 190.7945136500361230, 274.8346541966113818, -15.71499985172781066 ) ) ;
#93614=CARTESIAN_POINT ( 'NONE',  ( 184.6334634352423905, 296.8755821276896540, -4.397454188638743489 ) ) ;
#93615=CARTESIAN_POINT ( 'NONE',  ( 198.1679321590325458, 277.6257778925182720, -16.56331389466651061 ) ) ;
#93617=CARTESIAN_POINT ( 'NONE',  ( 154.9910882912764123, 262.1945556895526579, 18.38052604520346023 ) ) ;
#93620=CARTESIAN_POINT ( 'NONE',  ( -5.751638101304356709, 176.6744531367911293, 4.594050593750047540 ) ) ;
#93621=CARTESIAN_POINT ( 'NONE',  ( 89.61940949045693117, 231.7369531367911009, -4.594050593750048428 ) ) ;
#93622=CARTESIAN_POINT ( 'NONE',  ( 203.3349860717029571, 278.4604684979374838, -16.59553970625579566 ) ) ;
#93623=CARTESIAN_POINT ( 'NONE',  ( 192.7705129102570822, 296.7586727687594816, -13.39629674907774692 ) ) ;
#93624=CARTESIAN_POINT ( 'NONE',  ( 183.0282842160764574, 294.7209337947608674, -8.144370267713933131 ) ) ;
#93629=CARTESIAN_POINT ( 'NONE',  ( 202.0661878422603763, 279.1895584290143120, -16.02388874507808225 ) ) ;
#93633=CARTESIAN_POINT ( 'NONE',  ( 161.5907339951948245, 250.7636340184123469, 12.67682986482127028 ) ) ;
#93634=CARTESIAN_POINT ( 'NONE',  ( 166.0167935002967283, 249.2348392641485191, -9.295598770875054484 ) ) ;
#93635=CARTESIAN_POINT ( 'NONE',  ( 204.8371018956013074, 275.8587275720924481, -12.67884532777024198 ) ) ;
#93636=CARTESIAN_POINT ( 'NONE',  ( 196.0727848089514964, 291.0389700598140621, 17.56388901715066808 ) ) ;
#93639=CARTESIAN_POINT ( 'NONE',  ( 207.6357208050208101, 271.0113774299547913, -6.790259683043212036 ) ) ;
#93640=B_SPLINE_CURVE_WITH_KNOTS ( 'NONE', 3,
 ( #39072, #49211, #80143, #10708 ),
 .UNSPECIFIED., .F., .F.,
 ( 4, 4 ),
 ( 0.008487571838833373600, 0.009484744147854903482 ),
 .UNSPECIFIED. ) ;
#93641=CARTESIAN_POINT ( 'NONE',  ( 31.29809797828990270, 195.0024278399160664, -9.188101187500093303 ) ) ;
#93643=EDGE_CURVE ( 'NONE', #64147, #31573, #45968, .T. ) ;
#93644=CARTESIAN_POINT ( 'NONE',  ( 67.50895872190925218, 209.7833772461660544, -9.188101187500095079 ) ) ;
#93645=CARTESIAN_POINT ( 'NONE',  ( 190.8429499865819707, 278.0757709512191695, -17.64141544901220371 ) ) ;
#93647=CARTESIAN_POINT ( 'NONE',  ( 107.5017976953482446, 221.3262482093458061, 3.021315404115420679E-15 ) ) ;
#93648=CARTESIAN_POINT ( 'NONE',  ( 140.9585647324944659, 258.3149278399160380, 9.188101187500093303 ) ) ;
#93652=CARTESIAN_POINT ( 'NONE',  ( 198.1689325269066444, 270.4971866185222780, -10.92086016236654444 ) ) ;
#93654=CARTESIAN_POINT ( 'NONE',  ( 198.8194531333411419, 286.2816009704309863, -17.01510935557533344 ) ) ;
#93655=CARTESIAN_POINT ( 'NONE',  ( 149.2223635749290622, 272.1862799931444670, -12.97307652490353647 ) ) ;
#93657=CARTESIAN_POINT ( 'NONE',  ( 67.18419919549008057, 209.5958772461660544, -9.188101187500095079 ) ) ;
#93658=CARTESIAN_POINT ( 'NONE',  ( 158.7800074345649648, 256.0125694611146514, -16.06375889119701483 ) ) ;
#93659=CARTESIAN_POINT ( 'NONE',  ( 202.7676489560256528, 279.4431252073101746, -16.04062356091568020 ) ) ;
#93661=CARTESIAN_POINT ( 'NONE',  ( 159.3528137482544196, 254.6398255893999476, 16.73628156321660398 ) ) ;
#93666=CARTESIAN_POINT ( 'NONE',  ( 118.6676052326577633, 225.9865022471901455, 1.119607411625061291E-15 ) ) ;
#93668=CARTESIAN_POINT ( 'NONE',  ( 207.6860335175200589, 270.9242332556395922, 6.913225035677485586 ) ) ;
#93671=CARTESIAN_POINT ( 'NONE',  ( 185.4348243712239821, 271.7623222876268301, 15.85896177974588639 ) ) ;
#93673=CARTESIAN_POINT ( 'NONE',  ( 159.2651917302844993, 254.7915913763855258, -16.53922207549818424 ) ) ;
#93674=CARTESIAN_POINT ( 'NONE',  ( 193.9893413146322132, 294.1401140054277334, 13.97219244730923471 ) ) ;
#93677=CARTESIAN_POINT ( 'NONE',  ( 173.7058431582960054, 250.9251529220507564, 0.5223538383735283341 ) ) ;
#93678=ORIENTED_EDGE ( 'NONE', *, *, #38121, .F. ) ;
#93680=CARTESIAN_POINT ( 'NONE',  ( 148.4083960970861256, 273.5961130204771052, -8.574185186226726429 ) ) ;
#93681=CARTESIAN_POINT ( 'NONE',  ( 148.4820959031164023, 274.3664125831473939, 7.729347682778947792 ) ) ;
#93688=EDGE_CURVE ( 'NONE', #29382, #73834, #82298, .T. ) ;
#93691=CARTESIAN_POINT ( 'NONE',  ( 206.7408728089182546, 272.5612996242556960, -10.63134519248043475 ) ) ;
#93692=ORIENTED_EDGE ( 'NONE', *, *, #14645, .T. ) ;
#93697=CARTESIAN_POINT ( 'NONE',  ( 178.0302064638906074, 292.4640037680099454, 7.106335582765731296 ) ) ;
#93699=CARTESIAN_POINT ( 'NONE',  ( 204.7764732025852084, 275.9637395487929439, -14.02287343454361412 ) ) ;
#93700=CARTESIAN_POINT ( 'NONE',  ( 207.9607810208533749, 270.4483566206134242, -3.700399523436301408 ) ) ;
#93702=CARTESIAN_POINT ( 'NONE',  ( 206.4545408510063567, 270.6145640749817289, 2.451115620848321797 ) ) ;
#93703=CARTESIAN_POINT ( 'NONE',  ( 180.7872516664550915, 259.6763394889495089, 9.523190573527278602 ) ) ;
#93704=CARTESIAN_POINT ( 'NONE',  ( 91.51436070488293240, 214.4548013555409796, -4.594050593750042211 ) ) ;
#93705=ORIENTED_EDGE ( 'NONE', *, *, #23458, .F. ) ;
#93706=CARTESIAN_POINT ( 'NONE',  ( 150.6931560952953646, 269.6387926204777727, 14.65021044537114037 ) ) ;
#93707=CARTESIAN_POINT ( 'NONE',  ( 156.6168467568483891, 276.9391697405689001, 11.51099842983860633 ) ) ;
#93710=CARTESIAN_POINT ( 'NONE',  ( 156.9736299494965408, 258.7606928093932197, -16.87440706565485016 ) ) ;
#93717=CARTESIAN_POINT ( 'NONE',  ( 191.5324528500417216, 298.9030556958743432, -8.286652526617016790 ) ) ;
#93720=CARTESIAN_POINT ( 'NONE',  ( 162.9529104326093716, 248.4042752199367214, 11.77079043123004176 ) ) ;
#93721=CARTESIAN_POINT ( 'NONE',  ( 71.13526655237410523, 218.0024278399160664, 9.188101187500095079 ) ) ;
#93724=( BOUNDED_CURVE ( )  B_SPLINE_CURVE ( 2, ( #59563, #6387, #52471, #14486, #36772, #6870, #76299, #37761, #37273 ),
 .UNSPECIFIED., .F., .T. ) 
 B_SPLINE_CURVE_WITH_KNOTS ( ( 3, 2, 2, 2, 3 ),
 ( 0.4798387096774193727, 0.4811827956989247479, 0.4838709677419354982, 0.4865591397849462485, 0.4879032258064516236 ),
 .UNSPECIFIED. ) 
 CURVE ( )  GEOMETRIC_REPRESENTATION_ITEM ( )  RATIONAL_B_SPLINE_CURVE ( ( 0.9330127018922194093, 0.9330127018922194093, 1.000000000000000000, 0.8660254037844387076, 1.000000000000000000, 0.8660254037844387076, 1.000000000000000000, 0.9330127018922194093, 0.9330127018922194093 ) ) 
 REPRESENTATION_ITEM ( '' )  );
#93725=ORIENTED_EDGE ( 'NONE', *, *, #45931, .T. ) ;
#93726=CARTESIAN_POINT ( 'NONE',  ( 201.0201945934902028, 282.4698049471293757, -18.03844186250218229 ) ) ;
#93728=VERTEX_POINT ( 'NONE', #37184 ) ;
#93731=CARTESIAN_POINT ( 'NONE',  ( 184.2134048493523721, 275.2594305566963726, 16.37148162228643145 ) ) ;
#93732=AXIS2_PLACEMENT_3D ( 'NONE', #1516, #79548, #79030 ) ;
#93734=CARTESIAN_POINT ( 'NONE',  ( 207.4188537709976572, 270.9991043259717571, -1.591865268704130587 ) ) ;
#93736=ORIENTED_EDGE ( 'NONE', *, *, #34950, .F. ) ;
#93739=CARTESIAN_POINT ( 'NONE',  ( 206.1062572280473546, 273.6604860535989587, -9.773577984388410300 ) ) ;
#93740=CARTESIAN_POINT ( 'NONE',  ( 147.7314489675487152, 275.2273187821839429, -4.041098034711884779 ) ) ;
#93741=CARTESIAN_POINT ( 'NONE',  ( 175.6685219133858311, 284.7759717101654928, 14.09206119860363415 ) ) ;
#93743=CARTESIAN_POINT ( 'NONE',  ( 198.9782931523127445, 285.5098555092977222, -17.06882919058305603 ) ) ;
#93748=CARTESIAN_POINT ( 'NONE',  ( 161.3644539559160478, 251.1555625431813894, 12.97746593258196413 ) ) ;
#93750=CARTESIAN_POINT ( 'NONE',  ( 187.0949703139557130, 265.6442697474142278, -11.84038648041589070 ) ) ;
#93757=CARTESIAN_POINT ( 'NONE',  ( 207.6727254509676186, 270.9472835030587703, 7.315149605389819953 ) ) ;
#93760=CARTESIAN_POINT ( 'NONE',  ( 199.3295071964006979, 281.4960670786311425, -16.63318914033289886 ) ) ;
#93763=DIRECTION ( 'NONE',  ( -0.8660254037844387076, -0.4999999999999998890, -0.000000000000000000 ) ) ;
#93764=CARTESIAN_POINT ( 'NONE',  ( 131.8023238567217561, 240.2365022471901739, -10.00000000000009237 ) ) ;
#93765=CARTESIAN_POINT ( 'NONE',  ( 188.2455483746452671, 260.8383077707633220, 2.948178099069697300 ) ) ;
#93767=CARTESIAN_POINT ( 'NONE',  ( -0.2032289886040369309, 164.5643266524160140, -9.188101187500093303 ) ) ;
#93769=ORIENTED_EDGE ( 'NONE', *, *, #44612, .F. ) ;
#93771=CARTESIAN_POINT ( 'NONE',  ( 160.7608406066382258, 253.1279765243780275, -14.70232046160609229 ) ) ;
#93773=DIRECTION ( 'NONE',  ( -0.8660254037844387076, -0.4999999999999998890, -0.000000000000000000 ) ) ;
#93774=CARTESIAN_POINT ( 'NONE',  ( 22.85469738715664434, 177.8768266524159856, -9.188101187500093303 ) ) ;
#93775=CARTESIAN_POINT ( 'NONE',  ( 62.42776884207837895, 218.3967562850346837, -4.648177544792955347E-16 ) ) ;
#93778=CARTESIAN_POINT ( 'NONE',  ( 146.7373254022577100, 276.4904923669593586, -0.7242168585908188572 ) ) ;
#93782=CARTESIAN_POINT ( 'NONE',  ( 187.8880901142922824, 259.9596066364514400, -0.7662718320385906168 ) ) ;
#93784=CARTESIAN_POINT ( 'NONE',  ( 69.30415721694475906, 197.4865022471901455, 1.119607411625061291E-15 ) ) ;
#93786=CARTESIAN_POINT ( 'NONE',  ( 203.6370189927176284, 270.2020975153263862, 6.025740961596683931 ) ) ;
#93787=CARTESIAN_POINT ( 'NONE',  ( 33.24700223256990483, 183.8768266524160140, -9.188101187500091527 ) ) ;
#93790=CARTESIAN_POINT ( 'NONE',  ( 203.0474655300526763, 270.0767168047294149, -6.426262563393472682 ) ) ;
#93791=CARTESIAN_POINT ( 'NONE',  ( 151.3898985249405200, 268.4319993325432847, -14.65018536945715510 ) ) ;
#93794=CARTESIAN_POINT ( 'NONE',  ( 78.90260544222221029, 226.3615022471903160, 5.000000000000046185 ) ) ;
#93795=CARTESIAN_POINT ( 'NONE',  ( 202.3402481470395742, 279.2721451994542576, -15.68818295843871624 ) ) ;
#93796=CARTESIAN_POINT ( 'NONE',  ( 205.7253228364901645, 269.4700910448960940, -1.329327177517085845 ) ) ;
#93798=CARTESIAN_POINT ( 'NONE',  ( 162.6220573360242270, 248.9773295930640131, 10.49878733418918486 ) ) ;
#93799=CARTESIAN_POINT ( 'NONE',  ( 196.9319848161575806, 289.5507919934690335, -17.64330560362266453 ) ) ;
#93800=CARTESIAN_POINT ( 'NONE',  ( 175.2944853640667873, 257.1826618528377253, 11.78886922157304085 ) ) ;
#93801=ORIENTED_EDGE ( 'NONE', *, *, #64750, .F. ) ;
#93802=AXIS2_PLACEMENT_3D ( 'NONE', #99344, #93257, #60797 ) ;
#93809=CARTESIAN_POINT ( 'NONE',  ( 16.79905537663784898, 192.0530062829863311, -4.648177544792955347E-16 ) ) ;
#93811=CARTESIAN_POINT ( 'NONE',  ( 190.8094645593471341, 300.1553081486349015, 8.399847186519689757 ) ) ;
#93812=CARTESIAN_POINT ( 'NONE',  ( 180.1993755460965758, 257.5231556457691795, -7.374963718432667292 ) ) ;
#93815=EDGE_CURVE ( 'NONE', #21, #63881, #32536, .T. ) ;
#93816=CARTESIAN_POINT ( 'NONE',  ( 189.4970640320313748, 274.7204259376300683, -16.57914224039128470 ) ) ;
#93818=ORIENTED_EDGE ( 'NONE', *, *, #98262, .T. ) ;
#93819=CARTESIAN_POINT ( 'NONE',  ( 200.7694952279801157, 282.9040289856181403, -17.94628235092568502 ) ) ;
#93823=CARTESIAN_POINT ( 'NONE',  ( 190.1063449786324213, 301.3731469862293011, 0.2163967485516588019 ) ) ;
#93825=CARTESIAN_POINT ( 'NONE',  ( 196.3286486926436680, 290.5958008134369948, -16.58330917766970458 ) ) ;
#93827=CARTESIAN_POINT ( 'NONE',  ( 183.9298583336507136, 289.3229830586321327, -13.00965999724257749 ) ) ;
#93829=VERTEX_POINT ( 'NONE', #80096 ) ;
#93830=CARTESIAN_POINT ( 'NONE',  ( 157.1606030646430554, 258.4368458743103361, 17.96998724893680688 ) ) ;
#93831=CARTESIAN_POINT ( 'NONE',  ( 161.9337977053698694, 266.9980763431651667, 16.53593164407537941 ) ) ;
#93835=CARTESIAN_POINT ( 'NONE',  ( 198.1230806404959139, 287.4877535090322453, 17.00698319228197164 ) ) ;
#93836=CARTESIAN_POINT ( 'NONE',  ( 154.4986966408730211, 266.8510081643221952, -16.80735267183326087 ) ) ;
#93837=CARTESIAN_POINT ( 'NONE',  ( 57.63111678181675757, 194.8923013555409796, 4.594050593750050204 ) ) ;
#93841=CARTESIAN_POINT ( 'NONE',  ( 160.3857432900783522, 254.1750887689990179, 15.54860199936536702 ) ) ;
#93843=ORIENTED_EDGE ( 'NONE', *, *, #81465, .F. ) ;
#93845=CARTESIAN_POINT ( 'NONE',  ( 190.5541309856500050, 300.5975588711562523, -4.167177996129430184 ) ) ;
#93848=CARTESIAN_POINT ( 'NONE',  ( 172.0550459485834267, 258.7583009836712336, -13.85092418383490731 ) ) ;
#93849=CARTESIAN_POINT ( 'NONE',  ( 170.8756936250306069, 275.5691713738015096, -16.70647311572992066 ) ) ;
#93850=CARTESIAN_POINT ( 'NONE',  ( 146.5281990801392453, 276.8527097820684730, 0.2636021916935416542 ) ) ;
#93851=CARTESIAN_POINT ( 'NONE',  ( 192.9633865298379476, 296.4246058602058156, -11.85717392250713864 ) ) ;
#93852=CARTESIAN_POINT ( 'NONE',  ( 160.7492247939479171, 256.1349200705061548, 15.91803943147225908 ) ) ;
#93853=CARTESIAN_POINT ( 'NONE',  ( 177.9641021733659727, 269.8628481474571572, 16.10824436788937675 ) ) ;
#93854=CARTESIAN_POINT ( 'NONE',  ( 206.0691053506789387, 273.7248349927971844, 11.70564474658248422 ) ) ;
#93857=CARTESIAN_POINT ( 'NONE',  ( 207.6590484093196096, 270.9709728340903894, 3.402057849327809524 ) ) ;
#93858=CARTESIAN_POINT ( 'NONE',  ( 118.4422513298640638, 233.0643266524159856, 9.188101187500095079 ) ) ;
#93860=CARTESIAN_POINT ( 'NONE',  ( 190.1052739022278217, 301.3750021449804990, -4.471918118598219749 ) ) ;
#93862=CARTESIAN_POINT ( 'NONE',  ( 154.8833801513861772, 262.3811116602312268, -17.49275566389638215 ) ) ;
#93865=CARTESIAN_POINT ( 'NONE',  ( 174.7971014982606448, 252.6639005122666219, 5.121287243991948124 ) ) ;
#93868=CARTESIAN_POINT ( 'NONE',  ( -8.762112762712645164, 154.2012482093457777, 0.000000000000000000 ) ) ;
#93869=CARTESIAN_POINT ( 'NONE',  ( 182.2804195259451774, 259.9783927104286363, 10.74157115564638154 ) ) ;
#93871=CARTESIAN_POINT ( 'NONE',  ( 136.7913381204293728, 237.5327760586659736, 1.948934522072302763E-15 ) ) ;
#93872=CARTESIAN_POINT ( 'NONE',  ( 150.9003228897357189, 269.2799692068659283, -14.30003212299500781 ) ) ;
#93874=CARTESIAN_POINT ( 'NONE',  ( 189.0720805967732758, 299.7343203868808246, 4.955419684386629164 ) ) ;
#93875=CARTESIAN_POINT ( 'NONE',  ( 196.3021893095863959, 290.6416298092292436, 17.45656988653421138 ) ) ;
#93877=CARTESIAN_POINT ( 'NONE',  ( 51.08127902204942927, 209.4869531367911009, 4.594050593750046652 ) ) ;
#93879=B_SPLINE_CURVE_WITH_KNOTS ( 'NONE', 3,
 ( #39973, #86656, #24787, #93743, #48608, #17187, #78515, #71913, #86162, #2515, #55178, #48089 ),
 .UNSPECIFIED., .F., .F.,
 ( 4, 2, 2, 2, 2, 4 ),
 ( 0.001243902885841379705, 0.001690362744074533916, 0.001913592673191032200, 0.002136822602307530700, 0.002583282460540394128, 0.003029742318773257122 ),
 .UNSPECIFIED. ) ;
#93881=CARTESIAN_POINT ( 'NONE',  ( 173.0837253472800796, 264.8280141993791972, 17.07053884509587860 ) ) ;
#93884=CARTESIAN_POINT ( 'NONE',  ( 175.0973281419315697, 261.2292456205797748, 14.95496001069501091 ) ) ;
#93888=CARTESIAN_POINT ( 'NONE',  ( 13.35530768973961457, 178.5177522451418497, -10.00000000000009592 ) ) ;
#93889=CARTESIAN_POINT ( 'NONE',  ( 126.3716228836089215, 233.7677522451417929, -5.000000000000041744 ) ) ;
#93890=CARTESIAN_POINT ( 'NONE',  ( 167.5469267500292574, 266.7168544022062520, -17.80679023418265672 ) ) ;
#93893=CARTESIAN_POINT ( 'NONE',  ( 163.2835940097493790, 247.8315144631017404, 11.08416305054517359 ) ) ;
#93894=DIRECTION ( 'NONE',  ( -0.8660254037844387076, -0.4999999999999998890, -0.000000000000000000 ) ) ;
#93895=CARTESIAN_POINT ( 'NONE',  ( 35.30381256655795852, 185.0643266524160140, 9.188101187500095079 ) ) ;
#93897=CARTESIAN_POINT ( 'NONE',  ( 192.2499099399883846, 272.0886754808119008, 15.43621497701505341 ) ) ;
#93898=CARTESIAN_POINT ( 'NONE',  ( 190.1693911629507738, 301.2639477917662703, -5.112716700269980485 ) ) ;
#93901=CARTESIAN_POINT ( 'NONE',  ( 60.19284827774796298, 218.8927522451419350, 2.944929066748280225E-16 ) ) ;
#93903=CARTESIAN_POINT ( 'NONE',  ( 163.0473843169341706, 256.3777160336861130, -15.36546227846566559 ) ) ;
#93905=CARTESIAN_POINT ( 'NONE',  ( 157.8696211474012330, 257.2087905314882619, -17.27527248276125604 ) ) ;
#93908=EDGE_CURVE ( 'NONE', #2785, #11457, #64350, .T. ) ;
#93909=CARTESIAN_POINT ( 'NONE',  ( 21.31191609055701974, 193.1115022471903160, -5.000000000000047962 ) ) ;
#93910=CARTESIAN_POINT ( 'NONE',  ( 32.38751264475774860, 201.0530062829863027, -4.648177544792955347E-16 ) ) ;
#93911=CARTESIAN_POINT ( 'NONE',  ( 181.1477013271936016, 287.8971774238942203, -14.15342935774602218 ) ) ;
#93912=CARTESIAN_POINT ( 'NONE',  ( -10.75808714510939090, 164.5958772461660544, -9.188101187500095079 ) ) ;
#93914=CARTESIAN_POINT ( 'NONE',  ( 164.1174636406832406, 260.3667033378403630, -16.13808382457397173 ) ) ;
#93915=CARTESIAN_POINT ( 'NONE',  ( 200.3843439899536634, 282.5246900502644962, 16.99942400046845492 ) ) ;
#93916=CARTESIAN_POINT ( 'NONE',  ( 185.2882774749097052, 260.3413492530625604, 6.861618744156088745 ) ) ;
#93918=CARTESIAN_POINT ( 'NONE',  ( 185.4079346854762207, 258.9246787615279572, -2.323817269112564254 ) ) ;
#93920=ORIENTED_EDGE ( 'NONE', *, *, #40480, .T. ) ;
#93923=CARTESIAN_POINT ( 'NONE',  ( 166.8963884910926936, 286.1636476361714472, 0.4999093504684499201 ) ) ;
#93926=CARTESIAN_POINT ( 'NONE',  ( 159.2102594322688844, 254.8867369075254885, -16.13039487917589199 ) ) ;
#93927=CARTESIAN_POINT ( 'NONE',  ( 152.6615646578087819, 266.2294089801508221, 16.94722993326405813 ) ) ;
#93928=CARTESIAN_POINT ( 'NONE',  ( 189.9900095322273046, 294.8206031209193725, 12.79687042303630840 ) ) ;
#93930=CARTESIAN_POINT ( 'NONE',  ( 163.4178923001155681, 247.5989030008181260, -10.38047187240561442 ) ) ;
#93932=VERTEX_POINT ( 'NONE', #32454 ) ;
#93934=EDGE_CURVE ( 'NONE', #100061, #58518, #98132, .T. ) ;
#93935=CARTESIAN_POINT ( 'NONE',  ( 129.8617249334801613, 257.3297689869269220, -2.679491924311252493 ) ) ;
#93937=ORIENTED_EDGE ( 'NONE', *, *, #4575, .F. ) ;
#93939=CARTESIAN_POINT ( 'NONE',  ( 203.8609927293776707, 267.9499622782657866, -0.9252015903767020211 ) ) ;
#93940=ORIENTED_EDGE ( 'NONE', *, *, #85891, .F. ) ;
#93944=EDGE_CURVE ( 'NONE', #39202, #81343, #53878, .T. ) ;
#93946=ORIENTED_EDGE ( 'NONE', *, *, #55161, .F. ) ;
#93947=CARTESIAN_POINT ( 'NONE',  ( 161.1990332043106946, 251.4420796895884394, 14.26998817770995487 ) ) ;
#93948=B_SPLINE_CURVE_WITH_KNOTS ( 'NONE', 3,
 ( #90261, #57804, #73043, #3636 ),
 .UNSPECIFIED., .F., .F.,
 ( 4, 4 ),
 ( 0.009422416152678910611, 0.01491714414824748224 ),
 .UNSPECIFIED. ) ;
#93949=CARTESIAN_POINT ( 'NONE',  ( 151.4159295687746294, 268.3869122420484814, 14.78076517566594106 ) ) ;
#93952=EDGE_CURVE ( 'NONE', #37817, #86137, #91112, .T. ) ;
#93956=ORIENTED_EDGE ( 'NONE', *, *, #53934, .T. ) ;
#93957=CARTESIAN_POINT ( 'NONE',  ( 180.3976227892601685, 269.7841510484220748, 17.25711389196291279 ) ) ;
#93959=VERTEX_POINT ( 'NONE', #94786 ) ;
#93960=CARTESIAN_POINT ( 'NONE',  ( 208.3135187673106543, 269.8373969220020285, 2.829653198597726682 ) ) ;
#93962=B_SPLINE_CURVE_WITH_KNOTS ( 'NONE', 3,
 ( #56226, #2052, #79083, #83819 ),
 .UNSPECIFIED., .F., .F.,
 ( 4, 4 ),
 ( 0.01139215366488464942, 0.01983881652011612248 ),
 .UNSPECIFIED. ) ;
#93966=CARTESIAN_POINT ( 'NONE',  ( 198.2505066714982149, 285.2670451491296149, 0.000000000000000000 ) ) ;
#93967=CARTESIAN_POINT ( 'NONE',  ( 167.1118283438475487, 246.8866125954127426, 1.959209920999884336 ) ) ;
#93970=CARTESIAN_POINT ( 'NONE',  ( 164.2545401858843945, 246.1497863546213978, 2.275217130759496609 ) ) ;
#93971=CARTESIAN_POINT ( 'NONE',  ( 159.2303255284352304, 254.8519814094557603, 16.39103317446447150 ) ) ;
#93973=CARTESIAN_POINT ( 'NONE',  ( -22.42236680055709641, 157.8615022471902591, 0.000000000000000000 ) ) ;
#93974=FACE_OUTER_BOUND ( 'NONE', #77589, .T. ) ;
#93975=CARTESIAN_POINT ( 'NONE',  ( 206.2809287719926488, 273.3579460648492159, -10.70911012174624588 ) ) ;
#93976=CARTESIAN_POINT ( 'NONE',  ( 157.6304115535352537, 270.8650229002738001, -16.00510772102553858 ) ) ;
#93978=CARTESIAN_POINT ( 'NONE',  ( 200.6449165581618956, 283.1198055712825976, 18.35107460171532523 ) ) ;
#93980=ORIENTED_EDGE ( 'NONE', *, *, #63283, .T. ) ;
#93981=CARTESIAN_POINT ( 'NONE',  ( 155.7698133297891729, 260.8457643577225440, -17.53298471631897826 ) ) ;
#93982=FACE_OUTER_BOUND ( 'NONE', #83356, .T. ) ;
#93983=B_SPLINE_CURVE_WITH_KNOTS ( 'NONE', 3,
 ( #10546, #44287, #90950, #18650, #28593, #18144 ),
 .UNSPECIFIED., .F., .F.,
 ( 4, 2, 4 ),
 ( 0.0009160183432510218956, 0.001204151881099926186, 0.001492285418948830584 ),
 .UNSPECIFIED. ) ;
#93986=CARTESIAN_POINT ( 'NONE',  ( 16.02555268474166539, 173.3927522451417929, -10.00000000000009059 ) ) ;
#93987=CARTESIAN_POINT ( 'NONE',  ( 81.20281187136818346, 223.8149278399160664, 9.188101187500093303 ) ) ;
#93989=CARTESIAN_POINT ( 'NONE',  ( 199.5820190223589066, 281.0610403850588455, -17.29246150691365358 ) ) ;
#93990=CARTESIAN_POINT ( 'NONE',  ( 170.3095142286849750, 280.6389898262832503, -13.87900323416883275 ) ) ;
#93991=B_SPLINE_CURVE_WITH_KNOTS ( 'NONE', 3,
 ( #53372, #6284, #44274, #14388 ),
 .UNSPECIFIED., .F., .F.,
 ( 4, 4 ),
 ( 0.001625297393536941689, 0.006935763186732861116 ),
 .UNSPECIFIED. ) ;
#93992=CARTESIAN_POINT ( 'NONE',  ( 3.802138503898990329, 166.8768266524160140, 9.188101187500098632 ) ) ;
#93994=CARTESIAN_POINT ( 'NONE',  ( 200.4116241316243645, 283.5238799070667142, 18.37703770054986663 ) ) ;
#93995=EDGE_LOOP ( 'NONE', ( #26291, #85748, #58730, #80789 ) ) ;
#93998=CARTESIAN_POINT ( 'NONE',  ( 197.8465159808518763, 265.0022582763427863, -3.002757407549030866 ) ) ;
#94001=CARTESIAN_POINT ( 'NONE',  ( 161.4143265314674522, 251.0691807084224365, -12.94469757303959234 ) ) ;
#94002=( BOUNDED_CURVE ( )  B_SPLINE_CURVE ( 2, ( #76382, #5968, #22164, #6472, #92117, #100181, #30766, #54035, #22669 ),
 .UNSPECIFIED., .F., .T. ) 
 B_SPLINE_CURVE_WITH_KNOTS ( ( 3, 2, 2, 2, 3 ),
 ( 0.6572580645161290036, 0.6586021505376343788, 0.6612903225806451291, 0.6639784946236558794, 0.6653225806451612545 ),
 .UNSPECIFIED. ) 
 CURVE ( )  GEOMETRIC_REPRESENTATION_ITEM ( )  RATIONAL_B_SPLINE_CURVE ( ( 0.9330127018922194093, 0.9330127018922194093, 1.000000000000000000, 0.8660254037844387076, 1.000000000000000000, 0.8660254037844387076, 1.000000000000000000, 0.9330127018922194093, 0.9330127018922194093 ) ) 
 REPRESENTATION_ITEM ( '' )  );
#94003=CARTESIAN_POINT ( 'NONE',  ( 185.3339445475077696, 286.4653616608484299, 16.08708905285897828 ) ) ;
#94004=CARTESIAN_POINT ( 'NONE',  ( 107.7317227740038987, 244.5530062829863311, -4.648177544792955347E-16 ) ) ;
#94005=CARTESIAN_POINT ( 'NONE',  ( 31.13589176296283156, 188.7833772461660544, -9.188101187500095079 ) ) ;
#94006=CARTESIAN_POINT ( 'NONE',  ( 198.8055222331880145, 277.1762050399552209, 15.17661964589477996 ) ) ;
#94008=CARTESIAN_POINT ( 'NONE',  ( 25.93867647934751730, 197.3297689869269220, -2.679491924311252493 ) ) ;
#94009=CARTESIAN_POINT ( 'NONE',  ( 175.3077253703091003, 281.1061267443325278, -14.92186143449572100 ) ) ;
#94011=CARTESIAN_POINT ( 'NONE',  ( 157.2168982216852555, 258.3393398020932636, 18.09635675623264106 ) ) ;
#94013=CARTESIAN_POINT ( 'NONE',  ( 169.5007657120409874, 248.2156828994837099, -1.963647642838588503 ) ) ;
#94014=CARTESIAN_POINT ( 'NONE',  ( 186.5421308631587465, 282.7087754812748130, 16.16777212897319771 ) ) ;
#94015=CARTESIAN_POINT ( 'NONE',  ( 194.6943296385021824, 293.4265244509877562, -16.10917128197217352 ) ) ;
#94016=CARTESIAN_POINT ( 'NONE',  ( 189.8346037648321101, 263.3851992863394571, 7.885794067937258234 ) ) ;
#94017=CARTESIAN_POINT ( 'NONE',  ( 204.3276935076901850, 276.7410487817560920, 13.46217427333259309 ) ) ;
#94018=CARTESIAN_POINT ( 'NONE',  ( 176.6943099527350682, 256.7931168052207340, -11.17617521364210731 ) ) ;
#94020=CARTESIAN_POINT ( 'NONE',  ( 146.5913834600193582, 276.7432712258716947, -0.4909717733184599253 ) ) ;
#94021=CARTESIAN_POINT ( 'NONE',  ( 190.2476911738421848, 301.1283281946692796, -1.360079143321618611 ) ) ;
#94023=CARTESIAN_POINT ( 'NONE',  ( 152.4638493392093608, 266.9524761909081576, -15.49024149966747466 ) ) ;
#94024=ADVANCED_FACE ( 'NONE', ( #89218 ), #75115, .F. ) ;
#94026=CARTESIAN_POINT ( 'NONE',  ( 14.88889434582250537, 172.7365022471902023, -10.00000000000009237 ) ) ;
#94027=CARTESIAN_POINT ( 'NONE',  ( 112.1907172202364080, 226.3923013555410080, 4.594050593750050204 ) ) ;
#94031=CARTESIAN_POINT ( 'NONE',  ( 196.3720681610792553, 290.5205960880691691, 16.18360420724715354 ) ) ;
#94032=CARTESIAN_POINT ( 'NONE',  ( 195.6526726375238070, 278.3487319424068573, 16.84146745586420479 ) ) ;
#94033=CARTESIAN_POINT ( 'NONE',  ( 151.0468907355330543, 269.0261062511888213, -14.45235335422399814 ) ) ;
#94035=CARTESIAN_POINT ( 'NONE',  ( 197.0313051377892748, 289.3787641501790517, -17.15509075150697882 ) ) ;
#94037=CARTESIAN_POINT ( 'NONE',  ( -27.42236680055714260, 166.5217562850347406, 1.224646799147364892E-15 ) ) ;
#94040=CARTESIAN_POINT ( 'NONE',  ( 189.4560346390393875, 265.8111423811684517, 10.75552142954006740 ) ) ;
#94041=CARTESIAN_POINT ( 'NONE',  ( 179.0021197982646584, 280.8427306710001403, 16.33118346667503928 ) ) ;
#94042=CARTESIAN_POINT ( 'NONE',  ( 200.5907457738537119, 269.0703187529413185, 9.184797546115563094 ) ) ;
#94043=ORIENTED_EDGE ( 'NONE', *, *, #30650, .F. ) ;
#94044=B_SPLINE_CURVE_WITH_KNOTS ( 'NONE', 3,
 ( #53021, #23108, #53999, #84960 ),
 .UNSPECIFIED., .F., .F.,
 ( 4, 4 ),
 ( 0.01212979347998805260, 0.02063677174155311225 ),
 .UNSPECIFIED. ) ;
#94046=CARTESIAN_POINT ( 'NONE',  ( 186.2588223522137696, 258.3231150775076230, 4.130381131686830187 ) ) ;
#94047=CARTESIAN_POINT ( 'NONE',  ( 170.9071956757241821, 261.0918318682022914, -16.28277954748680401 ) ) ;
#94049=CARTESIAN_POINT ( 'NONE',  ( 192.6470966816805230, 296.9724359471326807, 11.11268290051284424 ) ) ;
#94052=CARTESIAN_POINT ( 'NONE',  ( 191.2263287708686050, 280.2574088826832508, 17.09578982601275854 ) ) ;
#94056=CARTESIAN_POINT ( 'NONE',  ( 177.7342311040593756, 255.2532439957012684, -8.367404576774948310 ) ) ;
#94058=CARTESIAN_POINT ( 'NONE',  ( 201.5189872289815867, 266.7509884862435570, -2.318412474989284267 ) ) ;
#94059=ORIENTED_EDGE ( 'NONE', *, *, #62646, .T. ) ;
#94061=CARTESIAN_POINT ( 'NONE',  ( 188.8213496144733483, 293.6675690155782945, 12.81620811140911265 ) ) ;
#94062=CARTESIAN_POINT ( 'NONE',  ( 1.210598108517954685, 183.0530062829863596, 2.649461200531984646E-14 ) ) ;
#94070=CARTESIAN_POINT ( 'NONE',  ( 195.4899348203562965, 291.0385781265877085, 16.10920391193625179 ) ) ;
#94076=ORIENTED_EDGE ( 'NONE', *, *, #49866, .T. ) ;
#94077=CARTESIAN_POINT ( 'NONE',  ( 184.5471555646610682, 281.3800897130075782, -16.25044877093907658 ) ) ;
#94078=CARTESIAN_POINT ( 'NONE',  ( 164.3448606421738702, 245.9933467353647814, -1.273739175181084260 ) ) ;
#94079=CARTESIAN_POINT ( 'NONE',  ( 190.0367258288550829, 301.4937308908229170, 2.142183824395127445 ) ) ;
#94080=CARTESIAN_POINT ( 'NONE',  ( 196.1272880827983442, 284.4644126364685235, -17.48124770668370331 ) ) ;
#94082=CARTESIAN_POINT ( 'NONE',  ( 168.2785332225647323, 249.6087795265106593, -5.466131228726310631 ) ) ;
#94084=CARTESIAN_POINT ( 'NONE',  ( 157.9722338812990472, 280.9990382926234247, 2.257701763675134199 ) ) ;
#94085=CARTESIAN_POINT ( 'NONE',  ( 134.5719744753492364, 242.3768266524159856, -9.188101187500091527 ) ) ;
#94086=VERTEX_POINT ( 'NONE', #44018 ) ;
#94091=CARTESIAN_POINT ( 'NONE',  ( 152.6809499003229860, 273.9044486092186048, 12.24870461040242553 ) ) ;
#94093=CARTESIAN_POINT ( 'NONE',  ( 200.3208879218390450, 274.1164785610297372, 13.54232579234367506 ) ) ;
#94094=DIRECTION ( 'NONE',  ( -0.8660254037844387076, -0.4999999999999998890, -0.000000000000000000 ) ) ;
#94096=CARTESIAN_POINT ( 'NONE',  ( 147.4519858293454320, 275.2526641970844707, 3.572377003827207353 ) ) ;
#94099=CARTESIAN_POINT ( 'NONE',  ( 173.3818033105709446, 287.4306447483324405, -9.822949107308927452 ) ) ;
#94100=CARTESIAN_POINT ( 'NONE',  ( 174.7211242335244208, 282.3968719112178292, 14.74411924494472359 ) ) ;
#94101=AXIS2_PLACEMENT_3D ( 'NONE', #17493, #79344, #2313 ) ;
#94102=CARTESIAN_POINT ( 'NONE',  ( 176.0127109592394277, 252.6004560315867593, -4.768680066900455650 ) ) ;
#94104=CARTESIAN_POINT ( 'NONE',  ( 194.6782745185928434, 293.4543327343926080, -14.56555309295305634 ) ) ;
#94105=CARTESIAN_POINT ( 'NONE',  ( 152.7208596440031840, 273.9049655622842465, 12.23028915028310415 ) ) ;
#94107=CARTESIAN_POINT ( 'NONE',  ( 190.0162302916581893, 267.2141329825763023, -11.93996759466560853 ) ) ;
#94108=CARTESIAN_POINT ( 'NONE',  ( 190.9800885167487650, 283.3134609288387651, -16.57359780736571153 ) ) ;
#94109=CARTESIAN_POINT ( 'NONE',  ( 192.1932326858383249, 297.7585514476576236, -9.982766916270952251 ) ) ;
#94112=CARTESIAN_POINT ( 'NONE',  ( 161.4469300188632701, 281.4659579066204174, -6.636762326697274617 ) ) ;
#94113=CARTESIAN_POINT ( 'NONE',  ( 151.4960827286219001, 274.9315224285210206, -8.792788082167028563 ) ) ;
#94114=CARTESIAN_POINT ( 'NONE',  ( 164.9043417134678577, 286.5925546497160212, 0.04530247668140159611 ) ) ;
#94115=ORIENTED_EDGE ( 'NONE', *, *, #58313, .T. ) ;
#94116=CARTESIAN_POINT ( 'NONE',  ( 147.5492216329511166, 275.0842468449245644, 4.751613690710122739 ) ) ;
#94118=DIRECTION ( 'NONE',  ( 0.8660254037844395958, 0.4999999999999985567, 0.000000000000000000 ) ) ;
#94120=CARTESIAN_POINT ( 'NONE',  ( 3.808674319871268921, 184.5530062829863027, -4.648177544792955347E-16 ) ) ;
#94121=CARTESIAN_POINT ( 'NONE',  ( 152.6615646578087819, 266.2294089801508221, 16.94722993326405813 ) ) ;
#94125=CARTESIAN_POINT ( 'NONE',  ( -15.46727382606978374, 168.0024278399161233, -9.188101187500093303 ) ) ;
#94126=CARTESIAN_POINT ( 'NONE',  ( 84.07169456928664886, 219.3458772461660544, 9.188101187500095079 ) ) ;
#94127=CARTESIAN_POINT ( 'NONE',  ( 155.6066474290145720, 261.1283759879266881, -18.16552045242181279 ) ) ;
#94128=CARTESIAN_POINT ( 'NONE',  ( 146.8312060062178830, 276.3278863910550172, -4.807241325481028227 ) ) ;
#94129=CARTESIAN_POINT ( 'NONE',  ( 182.8446340216047474, 294.1739319776609705, -7.947300712334529393 ) ) ;
#94135=CARTESIAN_POINT ( 'NONE',  ( 178.4123150140798941, 290.7538431597592421, 9.991683058491686253 ) ) ;
#94136=CARTESIAN_POINT ( 'NONE',  ( -2.160980794731546695, 162.8927522451417929, -10.00000000000009237 ) ) ;
#94139=CARTESIAN_POINT ( 'NONE',  ( 157.1338510812060747, 258.4831816688264325, 17.88958125218800888 ) ) ;
#94143=CARTESIAN_POINT ( 'NONE',  ( 46.56214281575564939, 191.5643266524159856, -9.188101187500093303 ) ) ;
#94146=CARTESIAN_POINT ( 'NONE',  ( 72.70511114461589841, 212.7833772461660544, -9.188101187500095079 ) ) ;
#94147=CARTESIAN_POINT ( 'NONE',  ( 57.23161641937173982, 215.3967562850347122, -4.648177544792955347E-16 ) ) ;
#94149=CARTESIAN_POINT ( 'NONE',  ( 167.2874460902532689, 259.7876024158500741, 16.17904535958410150 ) ) ;
#94152=CARTESIAN_POINT ( 'NONE',  ( 196.5459883665041332, 268.9076809661281686, -10.53567312597886563 ) ) ;
#94154=CARTESIAN_POINT ( 'NONE',  ( 151.0801312611820890, 268.9685319718947198, -15.83903210480701240 ) ) ;
#94155=CARTESIAN_POINT ( 'NONE',  ( 149.2593905435863348, 272.1221474021800759, -12.98626158366800176 ) ) ;
#94157=CARTESIAN_POINT ( 'NONE',  ( 61.47358386746269332, 215.4869531367911009, 4.594050593750046652 ) ) ;
#94159=DIRECTION ( 'NONE',  ( 0.4999999999999992784, -0.8660254037844390407, 0.000000000000000000 ) ) ;
#94160=CARTESIAN_POINT ( 'NONE',  ( 159.4574711498080433, 254.4585536525209477, 16.86100557095418395 ) ) ;
#94162=CARTESIAN_POINT ( 'NONE',  ( 154.1156850538427250, 263.7107985738977618, 17.28418349447918700 ) ) ;
#94166=CARTESIAN_POINT ( 'NONE',  ( 101.8522786425098445, 239.6115022471902876, -5.000000000000047962 ) ) ;
#94168=CARTESIAN_POINT ( 'NONE',  ( 164.2578067403839555, 246.1441285162624126, -2.322300236470859591 ) ) ;
#94171=CARTESIAN_POINT ( 'NONE',  ( 188.1310009398110878, 273.3760639908985581, 15.63936761710383827 ) ) ;
#94172=EDGE_LOOP ( 'NONE', ( #93302, #823, #95337, #81955 ) ) ;
#94173=CARTESIAN_POINT ( 'NONE',  ( 159.5895502557670795, 254.2297859303815244, -16.92708575547316485 ) ) ;
#94174=B_SPLINE_CURVE_WITH_KNOTS ( 'NONE', 3,
 ( #53133, #91669, #30335, #61225 ),
 .UNSPECIFIED., .F., .F.,
 ( 4, 4 ),
 ( 0.02770447213199976264, 0.03690780161571044493 ),
 .UNSPECIFIED. ) ;
#94175=CARTESIAN_POINT ( 'NONE',  ( 190.3874097485314394, 278.8119828322884928, -16.52278601034964112 ) ) ;
#94178=CARTESIAN_POINT ( 'NONE',  ( 177.2494136933412108, 252.9521367768340383, -0.2656116247643500183 ) ) ;
#94181=CARTESIAN_POINT ( 'NONE',  ( 170.0689406639716879, 250.0722447876482875, 3.416113949011092110 ) ) ;
#94183=ORIENTED_EDGE ( 'NONE', *, *, #10962, .F. ) ;
#94191=CARTESIAN_POINT ( 'NONE',  ( 206.6268150440956504, 272.7588534679261443, -10.76664753678610609 ) ) ;
#94193=CARTESIAN_POINT ( 'NONE',  ( 171.8003058497035624, 285.7827424729591712, 11.35508565917934654 ) ) ;
#94197=CARTESIAN_POINT ( 'NONE',  ( 180.4218656208765310, 293.5880668416769481, 7.617716764297705723 ) ) ;
#94199=CARTESIAN_POINT ( 'NONE',  ( 157.8811243250769110, 257.1888664433053009, -17.39256699147873064 ) ) ;
#94200=CARTESIAN_POINT ( 'NONE',  ( 142.6909626358283560, 247.0643266524159856, -9.188101187500093303 ) ) ;
#94201=CARTESIAN_POINT ( 'NONE',  ( 205.7955998042208421, 270.2654991239114111, 2.441702357542676616 ) ) ;
#94203=CARTESIAN_POINT ( 'NONE',  ( 90.72909131299699936, 229.3149278399160949, -9.188101187500095079 ) ) ;
#94204=ORIENTED_EDGE ( 'NONE', *, *, #95871, .T. ) ;
#94205=CARTESIAN_POINT ( 'NONE',  ( 190.7851751463332164, 300.1973786460605425, 8.237717828100052486 ) ) ;
#94209=CARTESIAN_POINT ( 'NONE',  ( 157.4595529495266533, 257.9190494847748027, -17.35536051855973838 ) ) ;
#94210=ORIENTED_EDGE ( 'NONE', *, *, #22281, .F. ) ;
#94214=B_SPLINE_SURFACE_WITH_KNOTS ( 'NONE', 3, 1, ( 
 ( #25951, #56320 ),
 ( #33539, #79681 ),
 ( #10243, #54821 ),
 ( #41112, #72046 ),
 ( #71345, #24720 ),
 ( #1445, #77943 ),
 ( #38915, #63729 ),
 ( #77446, #55602 ),
 ( #70319, #933 ),
 ( #39901, #15610 ),
 ( #7519, #47026 ),
 ( #78447, #31319 ),
 ( #1936, #38412 ),
 ( #24232, #94168 ),
 ( #46508, #56110 ),
 ( #32822, #70833 ),
 ( #69820, #32325 ),
 ( #8532, #31809 ),
 ( #39404, #94665 ),
 ( #9029, #431 ),
 ( #69327, #93159 ),
 ( #62207, #23709 ),
 ( #63226, #100248 ),
 ( #86587, #87100 ),
 ( #62709, #85062 ),
 ( #17122, #25223 ),
 ( #46002, #61716 ),
 ( #8042, #54603 ),
 ( #48018, #30830 ),
 ( #93668, #54105 ),
 ( #76920, #92663 ),
 ( #78961, #9549 ),
 ( #55110, #85587 ),
 ( #16128, #16623 ) ),
 .UNSPECIFIED., .T., .F., .F.,
 ( 4, 2, 2, 2, 2, 2, 2, 2, 2, 2, 2, 2, 2, 2, 2, 2, 4 ),
 ( 2, 2 ),
 ( 0.000000000000000000, 0.06250000000000000000, 0.1250000000000000000, 0.1875000000000000000, 0.2500000000000000000, 0.3125000000000000000, 0.3750000000000000000, 0.4375000000000000000, 0.5000000000000000000, 0.5625000000000000000, 0.6250000000000000000, 0.6875000000000000000, 0.7500000000000000000, 0.8125000000000000000, 0.8750000000000000000, 0.9375000000000000000, 1.000000000000000000 ),
 ( 0.000000000000000000, 1.000000000000000000 ),
 .UNSPECIFIED. ) ;
#94217=CARTESIAN_POINT ( 'NONE',  ( 84.12564760914067108, 225.5024278399160664, 9.188101187500095079 ) ) ;
#94223=CARTESIAN_POINT ( 'NONE',  ( 200.3254990932456110, 283.6730528493424117, -17.74520030754218780 ) ) ;
#94225=EDGE_CURVE ( 'NONE', #96030, #76205, #47381, .T. ) ;
#94227=CARTESIAN_POINT ( 'NONE',  ( 163.1501015339556773, 284.1938231124877916, 0.5074629045209336775 ) ) ;
#94228=CARTESIAN_POINT ( 'NONE',  ( 109.2134945746776538, 223.8615022471902023, 5.000000000000051514 ) ) ;
#94232=CARTESIAN_POINT ( 'NONE',  ( 185.1813530213977685, 260.2351280040860502, 6.311033929732698944 ) ) ;
#94233=CARTESIAN_POINT ( 'NONE',  ( 159.9997000813754084, 253.5193855937126841, -16.28798248637880519 ) ) ;
#94234=CARTESIAN_POINT ( 'NONE',  ( -27.42236680055714260, 166.5217562850347406, 1.224646799147364892E-15 ) ) ;
#94235=CARTESIAN_POINT ( 'NONE',  ( 153.1983976505312626, 265.2995869615763809, -17.69657798691567763 ) ) ;
#94240=CARTESIAN_POINT ( 'NONE',  ( 200.2316334480823912, 283.8356329158505105, 17.02791935830326508 ) ) ;
#94242=CARTESIAN_POINT ( 'NONE',  ( 171.2441523153178480, 251.6414079514013338, 7.096601279279188823 ) ) ;
#94244=CARTESIAN_POINT ( 'NONE',  ( 174.9183164536166259, 290.4820404178226454, -6.477921979946556164 ) ) ;
#94245=CARTESIAN_POINT ( 'NONE',  ( 153.0416928436757189, 270.7721196883188099, 13.91023073786846531 ) ) ;
#94247=CARTESIAN_POINT ( 'NONE',  ( 181.0193311394079103, 261.5502185760933003, 13.24438261311760812 ) ) ;
#94250=CARTESIAN_POINT ( 'NONE',  ( 180.5685635681490737, 266.8160690160535182, -14.77224249148190971 ) ) ;
#94255=CARTESIAN_POINT ( 'NONE',  ( 183.4832052704994965, 274.8226554140247799, 16.36505719518536495 ) ) ;
#94256=CARTESIAN_POINT ( 'NONE',  ( 178.2338095707201262, 261.7061032656386601, -14.47991691129509206 ) ) ;
#94257=CARTESIAN_POINT ( 'NONE',  ( 191.5691986906763873, 262.2710266103114805, 2.934180375091335335 ) ) ;
#94258=CARTESIAN_POINT ( 'NONE',  ( 161.8926315922002743, 250.2407320417157166, -13.77020595223768495 ) ) ;
#94259=CARTESIAN_POINT ( 'NONE',  ( 3.071516343397128423, 163.3923013555410080, 4.594050593750050204 ) ) ;
#94263=CARTESIAN_POINT ( 'NONE',  ( 176.1749608394459301, 255.9580892509862906, 8.247052548410042760 ) ) ;
#94266=CARTESIAN_POINT ( 'NONE',  ( 21.98867198337220330, 177.3768266524160140, 9.188101187500096856 ) ) ;
#94270=CARTESIAN_POINT ( 'NONE',  ( 178.5328262458293693, 291.6488152232226980, 5.998782872725313631 ) ) ;
#94271=CARTESIAN_POINT ( 'NONE',  ( 147.3047606266276546, 275.5076657283461827, -0.02269072295920609994 ) ) ;
#94274=CARTESIAN_POINT ( 'NONE',  ( 186.7692638048808362, 295.9158464710309886, -8.508718364155994252 ) ) ;
#94275=AXIS2_PLACEMENT_3D ( 'NONE', #31772, #69785, #395 ) ;
#94276=CARTESIAN_POINT ( 'NONE',  ( 91.91334042722833431, 212.3262482093457493, 3.021315404115420679E-15 ) ) ;
#94277=CARTESIAN_POINT ( 'NONE',  ( 62.37595398666918101, 213.4865022471903160, 10.00000000000009237 ) ) ;
#94281=CARTESIAN_POINT ( 'NONE',  ( 30.29666933122289407, 197.4869531367911293, 4.594050593750046652 ) ) ;
#94282=DIRECTION ( 'NONE',  ( -0.8660254037844387076, -0.4999999999999998890, -0.000000000000000000 ) ) ;
#94284=CARTESIAN_POINT ( 'NONE',  ( 199.1867231605587278, 285.6454706231928071, -17.41989184023605475 ) ) ;
#94286=EDGE_LOOP ( 'NONE', ( #68614, #70842, #2449 ) ) ;
#94288=CARTESIAN_POINT ( 'NONE',  ( 78.01622611019826081, 227.3967562850346837, -4.648177544792955347E-16 ) ) ;
#94294=CARTESIAN_POINT ( 'NONE',  ( 163.3543347837650686, 247.7089878483399730, 10.92686688779373405 ) ) ;
#94295=CARTESIAN_POINT ( 'NONE',  ( 196.6317700900902139, 290.0707791521982131, -17.91116578096951883 ) ) ;
#94296=CARTESIAN_POINT ( 'NONE',  ( 185.8360495164496626, 267.6137447244977920, -14.93125900359994063 ) ) ;
#94297=ORIENTED_EDGE ( 'NONE', *, *, #64706, .F. ) ;
#94300=CARTESIAN_POINT ( 'NONE',  ( 198.0816276881963915, 264.5915495180347534, -1.723934393811154182E-14 ) ) ;
#94303=VERTEX_POINT ( 'NONE', #41936 ) ;
#94305=FACE_OUTER_BOUND ( 'NONE', #21870, .T. ) ;
#94306=CARTESIAN_POINT ( 'NONE',  ( 178.8278557635266566, 282.3355866844354409, 15.39618937652901742 ) ) ;
#94308=CARTESIAN_POINT ( 'NONE',  ( 181.1193550619148311, 257.2754919020080138, -7.706538992632681051 ) ) ;
#94309=CARTESIAN_POINT ( 'NONE',  ( 190.1751179328237242, 301.2540287353828035, 3.252640783176552475 ) ) ;
#94312=CARTESIAN_POINT ( 'NONE',  ( 207.8718670335145475, 270.6023601641878713, -6.322166851501095586 ) ) ;
#94318=CARTESIAN_POINT ( 'NONE',  ( 205.3465787480556344, 274.9762877783610406, -13.79319041940166279 ) ) ;
#94319=CARTESIAN_POINT ( 'NONE',  ( 104.8295012880686699, 222.1423013555409796, -4.594050593750043987 ) ) ;
#94320=CARTESIAN_POINT ( 'NONE',  ( 180.4037401415526460, 287.2066285221069961, -13.85796317411490719 ) ) ;
#94324=ORIENTED_EDGE ( 'NONE', *, *, #75314, .T. ) ;
#94326=CARTESIAN_POINT ( 'NONE',  ( 157.1285250363530679, 258.9546388635270091, 16.90635852484395940 ) ) ;
#94329=CARTESIAN_POINT ( 'NONE',  ( 55.81761577081934433, 203.0333772461660544, 9.188101187500095079 ) ) ;
#94331=CARTESIAN_POINT ( 'NONE',  ( 190.8443993347725325, 300.0947993426467519, 8.522468760355437212 ) ) ;
#94332=CARTESIAN_POINT ( 'NONE',  ( 150.2761558193201381, 270.3610582852369930, 14.81920478290713028 ) ) ;
#94333=CARTESIAN_POINT ( 'NONE',  ( 174.3168710180726464, 271.9212240863662373, 16.46052307220685762 ) ) ;
#94335=CARTESIAN_POINT ( 'NONE',  ( 190.8842374621117699, 299.6106664202726506, 5.533255903905391015 ) ) ;
#94339=CARTESIAN_POINT ( 'NONE',  ( 108.4196379545418978, 226.7365022471902591, -10.00000000000009237 ) ) ;
#94341=EDGE_CURVE ( 'NONE', #33367, #40898, #100190, .T. ) ;
#94342=CARTESIAN_POINT ( 'NONE',  ( 207.6129110656513035, 271.0508850574501025, -5.265106572941297358 ) ) ;
#94343=CARTESIAN_POINT ( 'NONE',  ( 146.9700173529739970, 276.0874580858064746, -5.099093031535578469 ) ) ;
#94350=DIRECTION ( 'NONE',  ( -0.8660254037844387076, -0.4999999999999998890, -0.000000000000000000 ) ) ;
#94351=CARTESIAN_POINT ( 'NONE',  ( 114.2743305262689404, 236.7833772461660544, -9.188101187500095079 ) ) ;
#94353=CARTESIAN_POINT ( 'NONE',  ( 147.1447476476323004, 275.7848163378367872, 0.6373001129109078233 ) ) ;
#94356=CARTESIAN_POINT ( 'NONE',  ( 203.5629025532486196, 278.0657055720176913, -15.85226727704602823 ) ) ;
#94360=CARTESIAN_POINT ( 'NONE',  ( 178.0841129145181583, 255.3396897122842688, 4.676894877019703856 ) ) ;
#94363=CARTESIAN_POINT ( 'NONE',  ( 156.8878975079533973, 274.1353535065238702, -12.64326179356356938 ) ) ;
#94364=CARTESIAN_POINT ( 'NONE',  ( 182.1031022951341640, 260.5023910914902103, 9.513370520185286949 ) ) ;
#94366=CARTESIAN_POINT ( 'NONE',  ( 130.0789470495699618, 258.1589784336661637, -6.496448406907676862E-16 ) ) ;
#94367=CARTESIAN_POINT ( 'NONE',  ( 190.2164219629064803, 294.6625793156072177, -12.31662424489765506 ) ) ;
#94369=CARTESIAN_POINT ( 'NONE',  ( 188.9209837766938733, 282.1233005308658903, -16.64026405500985106 ) ) ;
#94370=DIRECTION ( 'NONE',  ( 0.4999999999999992784, -0.8660254037844390407, 0.000000000000000000 ) ) ;
#94371=CARTESIAN_POINT ( 'NONE',  ( 38.09089796528284211, 201.9869531367911293, 4.594050593750046652 ) ) ;
#94375=CARTESIAN_POINT ( 'NONE',  ( 167.0847919564587585, 251.8796711988679533, 11.83011900582259557 ) ) ;
#94376=CARTESIAN_POINT ( 'NONE',  ( 173.4258591900324689, 261.5801875239348533, 14.40537091172031658 ) ) ;
#94377=CARTESIAN_POINT ( 'NONE',  ( 151.6587809176374719, 278.2529691159808749, -1.644010740688682581 ) ) ;
#94378=CARTESIAN_POINT ( 'NONE',  ( 178.8774314082362196, 291.7284028483271072, -6.329699548260768083 ) ) ;
#94379=CARTESIAN_POINT ( 'NONE',  ( 162.2336410148055279, 251.8862672885301492, -14.09881826716025799 ) ) ;
#94380=CARTESIAN_POINT ( 'NONE',  ( 178.6939486350811421, 261.2861450363681683, 12.21674390882607852 ) ) ;
#94385=CARTESIAN_POINT ( 'NONE',  ( 163.1484656051875106, 248.0655637253488806, 9.714247672444804138 ) ) ;
#94387=CARTESIAN_POINT ( 'NONE',  ( 32.08336737017582152, 180.1423013555409796, -4.594050593750043987 ) ) ;
#94389=CARTESIAN_POINT ( 'NONE',  ( 188.7278402105932003, 290.4693834276403095, -14.85022589635486590 ) ) ;
#94390=CARTESIAN_POINT ( 'NONE',  ( 190.2236813008869660, 301.1699145145108218, -5.401374690107298093 ) ) ;
#94392=EDGE_CURVE ( 'NONE', #74173, #30217, #83345, .T. ) ;
#94394=CARTESIAN_POINT ( 'NONE',  ( 54.85235828774393951, 209.1427522451419350, -10.00000000000009415 ) ) ;
#94396=CARTESIAN_POINT ( 'NONE',  ( 182.4242555483369586, 257.1454310557409144, 1.318756070452638429 ) ) ;
#94398=CARTESIAN_POINT ( 'NONE',  ( 162.0972708797375219, 251.7219848490821903, -12.96270428423550491 ) ) ;
#94400=CARTESIAN_POINT ( 'NONE',  ( 32.20940242151128530, 182.7365022471902307, 10.00000000000009592 ) ) ;
#94402=CARTESIAN_POINT ( 'NONE',  ( 202.4017613376760494, 280.0768611521521620, 15.73960524502980540 ) ) ;
#94403=CARTESIAN_POINT ( 'NONE',  ( 151.1618603905361624, 248.8923013555409796, 4.594050593750050204 ) ) ;
#94406=CARTESIAN_POINT ( 'NONE',  ( 169.1454910628425807, 262.9544248868517684, 15.90528355961972551 ) ) ;
#94409=CARTESIAN_POINT ( 'NONE',  ( 164.8537203408104972, 245.1119758834023230, 2.926011033004258355 ) ) ;
#94410=CARTESIAN_POINT ( 'NONE',  ( 183.5235222349306525, 257.1254191288140305, -1.613677778301620958 ) ) ;
#94412=ORIENTED_EDGE ( 'NONE', *, *, #33031, .F. ) ;
#94414=( NAMED_UNIT ( * ) SI_UNIT ( $, .STERADIAN. ) SOLID_ANGLE_UNIT ( ) );
#94415=CARTESIAN_POINT ( 'NONE',  ( 178.6224597485341974, 285.5496574381789401, 13.02649328767307502 ) ) ;
#94416=CARTESIAN_POINT ( 'NONE',  ( 152.9587330967189871, 278.2315804880608425, -6.245711854568786414 ) ) ;
#94418=CARTESIAN_POINT ( 'NONE',  ( 207.1057321044409605, 271.9293447867963209, 8.088836166795815075 ) ) ;
#94420=CARTESIAN_POINT ( 'NONE',  ( 206.8313602288537538, 272.4045708154811791, -9.607337080360906612 ) ) ;
#94423=CARTESIAN_POINT ( 'NONE',  ( 89.43128961965948065, 210.8932355074535678, -2.679491924311248496 ) ) ;
#94425=CARTESIAN_POINT ( 'NONE',  ( 162.7007457333762090, 248.8410372908842021, -10.94671474643812914 ) ) ;
#94426=CARTESIAN_POINT ( 'NONE',  ( 193.7706395672514645, 295.0264025848412075, 15.16938698680137065 ) ) ;
#94429=CARTESIAN_POINT ( 'NONE',  ( 138.2253456014563255, 240.6115022471902023, -5.000000000000041744 ) ) ;
#94432=ORIENTED_EDGE ( 'NONE', *, *, #25032, .T. ) ;
#94435=CARTESIAN_POINT ( 'NONE',  ( 146.5502055023624735, 276.8145935406849389, 0.3770461397900869427 ) ) ;
#94440=CARTESIAN_POINT ( 'NONE',  ( 161.6707029936031574, 250.6251236501384483, 14.45053103226186231 ) ) ;
#94442=CARTESIAN_POINT ( 'NONE',  ( 151.4025156491502742, 268.4101458323662541, 14.71049357081981235 ) ) ;
#94443=CARTESIAN_POINT ( 'NONE',  ( 150.4141202964276260, 274.4678425752150019, -8.669812683062808389 ) ) ;
#94444=B_SPLINE_SURFACE_WITH_KNOTS ( 'NONE', 3, 1, ( 
 ( #39289, #810 ),
 ( #55492, #17005 ),
 ( #31689, #1829 ),
 ( #32711, #63611 ),
 ( #27631, #65115 ),
 ( #33734, #71740 ),
 ( #95065, #87983 ),
 ( #81361, #96064 ),
 ( #64624, #2333 ),
 ( #96560, #72751 ),
 ( #95579, #26124 ),
 ( #10425, #66111 ),
 ( #41298, #18532 ),
 ( #41804, #3823 ),
 ( #72239, #80361 ),
 ( #19545, #56509 ),
 ( #97059, #50406 ),
 ( #49414, #50901 ),
 ( #81851, #64113 ),
 ( #19043, #25625 ),
 ( #10933, #34706 ),
 ( #3344, #57002 ),
 ( #65606, #87498 ),
 ( #11931, #80872 ),
 ( #58495, #34220 ),
 ( #2844, #18033 ),
 ( #42787, #89469 ),
 ( #26622, #12426 ),
 ( #73722, #20027 ),
 ( #27129, #57503 ),
 ( #4304, #88481 ),
 ( #49916, #33216 ),
 ( #35209, #48925 ),
 ( #79863, #11445 ) ),
 .UNSPECIFIED., .T., .F., .F.,
 ( 4, 2, 2, 2, 2, 2, 2, 2, 2, 2, 2, 2, 2, 2, 2, 2, 4 ),
 ( 2, 2 ),
 ( 0.000000000000000000, 0.06250000000000000000, 0.1250000000000000000, 0.1875000000000000000, 0.2500000000000000000, 0.3125000000000000000, 0.3750000000000000000, 0.4375000000000000000, 0.5000000000000000000, 0.5625000000000000000, 0.6250000000000000000, 0.6875000000000000000, 0.7500000000000000000, 0.8125000000000000000, 0.8750000000000000000, 0.9375000000000000000, 1.000000000000000000 ),
 ( 0.000000000000000000, 1.000000000000000000 ),
 .UNSPECIFIED. ) ;
#94446=CARTESIAN_POINT ( 'NONE',  ( 171.2499256315726939, 254.4673999717836352, -11.80878994424205963 ) ) ;
#94447=CARTESIAN_POINT ( 'NONE',  ( 163.2442700311756596, 247.8996255919473697, 11.14021925110252020 ) ) ;
#94448=VERTEX_POINT ( 'NONE', #53017 ) ;
#94449=ORIENTED_EDGE ( 'NONE', *, *, #3737, .F. ) ;
#94451=VERTEX_POINT ( 'NONE', #90074 ) ;
#94452=CARTESIAN_POINT ( 'NONE',  ( 161.0001838071895008, 271.1393494378992273, 16.41176471004197523 ) ) ;
#94455=CARTESIAN_POINT ( 'NONE',  ( 166.5798837419092706, 271.6578438917711082, 16.15769450769992233 ) ) ;
#94456=CARTESIAN_POINT ( 'NONE',  ( 165.8975677354378035, 271.5909624305264174, 17.28637137770206067 ) ) ;
#94457=CARTESIAN_POINT ( 'NONE',  ( 194.6782745185928434, 293.4543327343926080, -14.56555309295305634 ) ) ;
#94458=EDGE_CURVE ( 'NONE', #95964, #3105, #53427, .T. ) ;
#94459=CARTESIAN_POINT ( 'NONE',  ( 174.5497488978029423, 290.1244087063413417, 6.358272735726022695 ) ) ;
#94461=ORIENTED_EDGE ( 'NONE', *, *, #40719, .T. ) ;
#94462=CARTESIAN_POINT ( 'NONE',  ( 167.0271109968743417, 287.8086958075197686, 0.5416428030073258126 ) ) ;
#94464=CARTESIAN_POINT ( 'NONE',  ( 206.2520115784021471, 273.4080321133600933, 11.69992874350409018 ) ) ;
#94465=CARTESIAN_POINT ( 'NONE',  ( 205.8918578537579833, 274.0318366629789466, 11.52627491423194250 ) ) ;
#94466=CARTESIAN_POINT ( 'NONE',  ( 206.8877919403300041, 271.6698519413213830, 5.894673806612072298 ) ) ;
#94468=CARTESIAN_POINT ( 'NONE',  ( 190.4261619690305167, 300.8192077097357355, 5.480148282445501451 ) ) ;
#94469=DIRECTION ( 'NONE',  ( -0.4999999999999987232, 0.8660254037844394848, 0.000000000000000000 ) ) ;
#94470=CARTESIAN_POINT ( 'NONE',  ( 206.8851632406098702, 272.3113812655195716, -9.957011741946159233 ) ) ;
#94471=EDGE_CURVE ( 'NONE', #99635, #33095, #72389, .T. ) ;
#94474=CARTESIAN_POINT ( 'NONE',  ( 161.1884843536000744, 251.4603508349806873, 13.21272898143761942 ) ) ;
#94475=CARTESIAN_POINT ( 'NONE',  ( 191.1851897594308127, 262.2115044052416124, -0.7464089480405260435 ) ) ;
#94477=CARTESIAN_POINT ( 'NONE',  ( 194.2703023721977047, 294.1609612200219317, -15.68238946779285037 ) ) ;
#94478=CARTESIAN_POINT ( 'NONE',  ( -22.42236680055709641, 157.8615022471902591, 0.000000000000000000 ) ) ;
#94479=CARTESIAN_POINT ( 'NONE',  ( 207.6628070930962906, 270.9644626028195376, 7.378217122120054761 ) ) ;
#94480=CARTESIAN_POINT ( 'NONE',  ( 12.05626958406292104, 187.7677522451419065, -5.000000000000047962 ) ) ;
#94481=CARTESIAN_POINT ( 'NONE',  ( 91.86592320334659689, 223.8458772461660544, 9.188101187500095079 ) ) ;
#94485=CARTESIAN_POINT ( 'NONE',  ( -2.422939729449181012, 181.6589784336661637, -6.496448406907675876E-16 ) ) ;
#94488=CARTESIAN_POINT ( 'NONE',  ( 200.1102648775588193, 284.0458494464393198, 17.54251420653697835 ) ) ;
#94490=ORIENTED_EDGE ( 'NONE', *, *, #863, .T. ) ;
#94492=CARTESIAN_POINT ( 'NONE',  ( 189.0340129193126018, 261.4605574960352214, -6.057196126885922460 ) ) ;
#94497=CARTESIAN_POINT ( 'NONE',  ( 185.7830797826618721, 286.6111327835436100, 15.87653701371242931 ) ) ;
#94499=ADVANCED_FACE ( 'NONE', ( #98655 ), #13546, .T. ) ;
#94500=CARTESIAN_POINT ( 'NONE',  ( 34.76219959342767396, 197.0024278399161517, 9.188101187500095079 ) ) ;
#94501=CARTESIAN_POINT ( 'NONE',  ( 84.36939080006362701, 209.5177522451417929, 5.000000000000051514 ) ) ;
#94511=CARTESIAN_POINT ( 'NONE',  ( 155.5660013421004919, 261.1987770755905558, 17.28709111629370199 ) ) ;
#94512=CARTESIAN_POINT ( 'NONE',  ( 161.8750289368003621, 250.2712207352165592, -13.97436367953006098 ) ) ;
#94513=CARTESIAN_POINT ( 'NONE',  ( 186.1456503528468431, 283.3687638237425404, 16.57478981768027992 ) ) ;
#94514=CARTESIAN_POINT ( 'NONE',  ( 148.1632261683078013, 274.0207597936089883, -7.853210555358286271 ) ) ;
#94516=ADVANCED_FACE ( 'NONE', ( #20030 ), #48928, .T. ) ;
#94518=CARTESIAN_POINT ( 'NONE',  ( 204.3574891606595827, 276.6894411969685166, 13.41627538812899978 ) ) ;
#94519=CARTESIAN_POINT ( 'NONE',  ( 191.8000917695741805, 298.4394914891611847, -9.452573400474340914 ) ) ;
#94520=CARTESIAN_POINT ( 'NONE',  ( 190.1063449786324213, 301.3731469862293011, 0.2163967485516588019 ) ) ;
#94522=CARTESIAN_POINT ( 'NONE',  ( 181.3121490855964169, 267.9468540978079432, 15.06114782510337236 ) ) ;
#94523=CARTESIAN_POINT ( 'NONE',  ( 109.2403843188893831, 240.0024278399160949, -9.188101187500093303 ) ) ;
#94527=CARTESIAN_POINT ( 'NONE',  ( 178.6627340464712859, 256.9245264283825918, 10.00612643570717708 ) ) ;
#94529=CARTESIAN_POINT ( 'NONE',  ( 191.3737201945137656, 299.1779887200690951, -7.181879264107196903 ) ) ;
#94530=FACE_OUTER_BOUND ( 'NONE', #85598, .T. ) ;
#94531=CARTESIAN_POINT ( 'NONE',  ( 196.7491951525289835, 289.8673929779723721, -16.35352603081977207 ) ) ;
#94532=CARTESIAN_POINT ( 'NONE',  ( 80.73032772533602497, 228.9637435831425023, 2.679491924311251605 ) ) ;
#94533=CARTESIAN_POINT ( 'NONE',  ( 203.6458270900087655, 276.5680210061898947, 14.19527340636538959 ) ) ;
#94535=CARTESIAN_POINT ( 'NONE',  ( 135.4648896233454991, 249.0177522451418497, -10.00000000000009592 ) ) ;
#94536=CARTESIAN_POINT ( 'NONE',  ( 175.2191928923303124, 279.1726182442799313, 15.58576654816208062 ) ) ;
#94537=CARTESIAN_POINT ( 'NONE',  ( 165.6500576547331036, 269.1436911520689250, -17.16406264618244037 ) ) ;
#94543=CARTESIAN_POINT ( 'NONE',  ( 192.8010417052266234, 296.7057953447782097, 12.10593424093686643 ) ) ;
#94545=CARTESIAN_POINT ( 'NONE',  ( 165.3929592122126451, 286.2279243276498732, 4.432946431554212197 ) ) ;
#94547=CARTESIAN_POINT ( 'NONE',  ( 193.5255742412444420, 289.0164190174409100, -16.00935465151201598 ) ) ;
#94549=CARTESIAN_POINT ( 'NONE',  ( 167.7406742120077752, 280.9361443569400762, 11.73743621418454985 ) ) ;
#94552=CARTESIAN_POINT ( 'NONE',  ( 16.11576366785043746, 180.1115022471902591, 10.00000000000009592 ) ) ;
#94553=ORIENTED_EDGE ( 'NONE', *, *, #53326, .T. ) ;
#94560=CARTESIAN_POINT ( 'NONE',  ( 155.0619429961492983, 262.0718317407570339, -17.08853361476647592 ) ) ;
#94561=VERTEX_POINT ( 'NONE', #49418 ) ;
#94563=CARTESIAN_POINT ( 'NONE',  ( 178.4219847520450628, 261.0252761168330835, 12.14700762561149538 ) ) ;
#94564=ORIENTED_EDGE ( 'NONE', *, *, #70776, .T. ) ;
#94569=CARTESIAN_POINT ( 'NONE',  ( 155.6281496932864457, 261.0911329737299980, -18.07904265579665548 ) ) ;
#94571=CARTESIAN_POINT ( 'NONE',  ( 182.7167784989862014, 280.1855270853789079, -16.12831863832678536 ) ) ;
#94572=CARTESIAN_POINT ( 'NONE',  ( 164.6027939175806125, 245.5465931973980105, -2.481135897876769913 ) ) ;
#94573=CARTESIAN_POINT ( 'NONE',  ( 147.7773877150008559, 274.6890515982507281, -5.974666768616035739 ) ) ;
#94575=CARTESIAN_POINT ( 'NONE',  ( 147.5118896528469179, 275.1489077312122049, -3.975523961781759930 ) ) ;
#94579=EDGE_CURVE ( 'NONE', #41928, #88465, #50409, .T. ) ;
#94580=CARTESIAN_POINT ( 'NONE',  ( 183.5836227624010917, 284.2690207048559046, -15.88295186417738591 ) ) ;
#94581=CARTESIAN_POINT ( 'NONE',  ( 124.8827946268633298, 255.1589784336661069, -6.496448406907675876E-16 ) ) ;
#94583=CARTESIAN_POINT ( 'NONE',  ( 186.5849876461966801, 262.7207080590939654, -9.049355759300835800 ) ) ;
#94590=CARTESIAN_POINT ( 'NONE',  ( 192.8203422047577078, 296.6723658989791943, 12.07326395438877320 ) ) ;
#94593=CARTESIAN_POINT ( 'NONE',  ( 197.5405456899788419, 268.5419454055666506, 10.87215985704571963 ) ) ;
#94594=CARTESIAN_POINT ( 'NONE',  ( 176.4132951231468098, 288.3403858341706609, -9.320880473285331647 ) ) ;
#94595=CARTESIAN_POINT ( 'NONE',  ( 195.2684241838297510, 292.4321635301326978, 16.66903275019414465 ) ) ;
#94597=CARTESIAN_POINT ( 'NONE',  ( 194.6318672504471863, 291.7125382847361266, 16.11827429453959226 ) ) ;
#94598=( BOUNDED_CURVE ( )  B_SPLINE_CURVE ( 2, ( #6395, #51487, #21596, #13018, #75310, #73801, #67183, #59569, #52478 ),
 .UNSPECIFIED., .F., .T. ) 
 B_SPLINE_CURVE_WITH_KNOTS ( ( 3, 2, 2, 2, 3 ),
 ( 0.3991935483870967527, 0.4005376344086021279, 0.4032258064516128782, 0.4059139784946236285, 0.4072580645161290591 ),
 .UNSPECIFIED. ) 
 CURVE ( )  GEOMETRIC_REPRESENTATION_ITEM ( )  RATIONAL_B_SPLINE_CURVE ( ( 0.9330127018922194093, 0.9330127018922194093, 1.000000000000000000, 0.8660254037844387076, 1.000000000000000000, 0.8660254037844387076, 1.000000000000000000, 0.9330127018922179660, 0.9330127018922194093 ) ) 
 REPRESENTATION_ITEM ( '' )  );
#94600=CARTESIAN_POINT ( 'NONE',  ( 194.1789525331299728, 294.3191837825503967, -15.34533909744314961 ) ) ;
#94601=CARTESIAN_POINT ( 'NONE',  ( 152.8245645352945417, 273.6623100745259762, 11.98233510762519316 ) ) ;
#94606=CARTESIAN_POINT ( 'NONE',  ( 190.7222376050763444, 300.3063896652212179, 3.365789908110941475 ) ) ;
#94607=CARTESIAN_POINT ( 'NONE',  ( 202.2773826701151165, 280.2922913237452462, 16.62862787739668846 ) ) ;
#94608=CARTESIAN_POINT ( 'NONE',  ( 153.5300831522595502, 269.9241095255698610, 14.65767817066312517 ) ) ;
#94609=CARTESIAN_POINT ( 'NONE',  ( 151.5094854109957225, 274.9022664227586006, -9.147610560135673197 ) ) ;
#94610=CARTESIAN_POINT ( 'NONE',  ( 153.1983976505312626, 265.2995869615763809, -17.69657798691567763 ) ) ;
#94612=CARTESIAN_POINT ( 'NONE',  ( 167.8684523614047635, 281.9072385613080769, -10.90217489050904831 ) ) ;
#94613=CARTESIAN_POINT ( 'NONE',  ( 186.9162837453443728, 262.3935138041393884, -8.704777280997261002 ) ) ;
#94614=CARTESIAN_POINT ( 'NONE',  ( 193.5562164153924414, 276.1342835013242620, -16.47396278362798938 ) ) ;
#94615=CARTESIAN_POINT ( 'NONE',  ( 74.84311135843471163, 224.0177522451419350, 5.000000000000046185 ) ) ;
#94616=CARTESIAN_POINT ( 'NONE',  ( 188.4553964595242235, 298.4901091694543425, -4.262234365374711231 ) ) ;
#94617=CARTESIAN_POINT ( 'NONE',  ( 204.2071116102253256, 275.4331146181932013, 13.30069288008150430 ) ) ;
#94619=CARTESIAN_POINT ( 'NONE',  ( -4.215479392844351914, 156.8262482093458061, -4.415768667553307481E-15 ) ) ;
#94621=EDGE_CURVE ( 'NONE', #62092, #31573, #4735, .T. ) ;
#94622=CARTESIAN_POINT ( 'NONE',  ( -9.405095999578705346, 171.5024278399160949, 9.188101187500095079 ) ) ;
#94623=CARTESIAN_POINT ( 'NONE',  ( 92.62404252742298638, 212.0327760586659451, 1.948934522072303157E-15 ) ) ;
#94624=CARTESIAN_POINT ( 'NONE',  ( 5.270092192305422252, 185.3967562850347122, -4.648177544792955347E-16 ) ) ;
#94626=CARTESIAN_POINT ( 'NONE',  ( 147.7269857344357149, 275.1802626144117312, 4.082897581163150491 ) ) ;
#94632=CARTESIAN_POINT ( 'NONE',  ( 208.3764315856425640, 269.7284287242038658, -1.833640725398759441 ) ) ;
#94633=CARTESIAN_POINT ( 'NONE',  ( 162.0519062060177475, 249.9648603182279487, 13.45613752710952937 ) ) ;
#94638=CARTESIAN_POINT ( 'NONE',  ( -14.37785915960194494, 174.0530062829862743, 6.972266317189433612E-15 ) ) ;
#94641=CARTESIAN_POINT ( 'NONE',  ( 37.98264478980979675, 201.9244531367911293, -4.594050593750046652 ) ) ;
#94643=CARTESIAN_POINT ( 'NONE',  ( 57.65757265809627086, 216.3464784336661353, 1.353441290958777327E-15 ) ) ;
#94644=CARTESIAN_POINT ( 'NONE',  ( 164.0020300202577346, 247.0572029250454307, -5.999176618229816071 ) ) ;
#94647=CARTESIAN_POINT ( 'NONE',  ( 167.0980956493596921, 259.5690430767091925, 16.41267671096424863 ) ) ;
#94649=CARTESIAN_POINT ( 'NONE',  ( 151.9976068546241095, 267.3794176293484952, 15.44464033079018250 ) ) ;
#94650=ADVANCED_FACE ( 'NONE', ( #74245 ), #72638, .F. ) ;
#94657=CARTESIAN_POINT ( 'NONE',  ( 69.78227540684341079, 211.0958772461660544, -9.188101187500095079 ) ) ;
#94659=CARTESIAN_POINT ( 'NONE',  ( 179.0685761320505947, 258.5468394390073286, -11.57600102548048149 ) ) ;
#94661=CARTESIAN_POINT ( 'NONE',  ( 201.4964414552794949, 281.6449211855650674, 17.70651170561034249 ) ) ;
#94662=CARTESIAN_POINT ( 'NONE',  ( 189.8554816459523806, 286.6603570597984003, 16.85211268990574851 ) ) ;
#94663=CARTESIAN_POINT ( 'NONE',  ( 132.5961804768574837, 237.3615022471901739, 5.000000000000051514 ) ) ;
#94665=CARTESIAN_POINT ( 'NONE',  ( 164.3774690880109119, 245.9368672504194819, -2.805681983503304000 ) ) ;
#94668=CARTESIAN_POINT ( 'NONE',  ( 188.1508358339878839, 273.3824090696089115, 15.63829542113482418 ) ) ;
#94670=CARTESIAN_POINT ( 'NONE',  ( 202.4900219881211854, 279.9239892212719383, 15.63116161057562259 ) ) ;
#94671=CARTESIAN_POINT ( 'NONE',  ( 207.3553394910502163, 270.5667219550074947, -0.3217649823664716080 ) ) ;
#94674=CARTESIAN_POINT ( 'NONE',  ( 177.2644709662962725, 252.9866977164365096, -0.2652805781673223118 ) ) ;
#94677=CARTESIAN_POINT ( 'NONE',  ( 170.7247694180109931, 250.3410439623759487, 3.110155547565024214 ) ) ;
#94685=CARTESIAN_POINT ( 'NONE',  ( 75.53417530262939295, 225.9637435831425023, 2.679491924311251605 ) ) ;
#94688=CARTESIAN_POINT ( 'NONE',  ( 185.8761704939435049, 297.8286767897885738, 1.040812290680570795 ) ) ;
#94690=CARTESIAN_POINT ( 'NONE',  ( 159.0906380018002153, 259.2649656523443582, -17.57712761084927067 ) ) ;
#94692=CARTESIAN_POINT ( 'NONE',  ( 155.4917600441137324, 261.3273667757233056, 17.14261720787171939 ) ) ;
#94693=CARTESIAN_POINT ( 'NONE',  ( 157.6036818288543486, 257.6694109429415107, -16.73826488331764395 ) ) ;
#94694=CARTESIAN_POINT ( 'NONE',  ( 164.2953130194600817, 246.0791657352997959, 5.812963931023970687 ) ) ;
#94696=CARTESIAN_POINT ( 'NONE',  ( 170.9618134082231506, 249.0169227132842309, -1.633238342494487183 ) ) ;
#94697=CARTESIAN_POINT ( 'NONE',  ( 89.26784699199328088, 222.3458772461660544, 9.188101187500095079 ) ) ;
#94698=ORIENTED_EDGE ( 'NONE', *, *, #89791, .F. ) ;
#94699=CARTESIAN_POINT ( 'NONE',  ( 191.2729698983822288, 299.3524933518466469, 8.871011392605806734 ) ) ;
#94703=CARTESIAN_POINT ( 'NONE',  ( 196.0995493315176645, 290.9926125468888927, -16.21657796881217806 ) ) ;
#94704=EDGE_LOOP ( 'NONE', ( #30873, #67903, #27135, #61504 ) ) ;
#94707=CARTESIAN_POINT ( 'NONE',  ( 164.1785392759978492, 249.9733907654231473, 10.19594168643268084 ) ) ;
#94710=CARTESIAN_POINT ( 'NONE',  ( 207.5772549350081988, 271.1126432873252838, 2.658056670308439617 ) ) ;
#94711=CARTESIAN_POINT ( 'NONE',  ( 97.03527265400872182, 217.6423013555409796, -4.594050593750043987 ) ) ;
#94713=EDGE_CURVE ( 'NONE', #99270, #66266, #73631, .T. ) ;
#94714=ORIENTED_EDGE ( 'NONE', *, *, #90750, .T. ) ;
#94724=VERTEX_POINT ( 'NONE', #46800 ) ;
#94727=CARTESIAN_POINT ( 'NONE',  ( 206.2313482792274328, 273.4438219973828268, -9.403385562213845361 ) ) ;
#94729=CARTESIAN_POINT ( 'NONE',  ( 201.1060504099706350, 282.3210983108598384, -18.18000168485860257 ) ) ;
#94730=CARTESIAN_POINT ( 'NONE',  ( 102.9889369814289921, 240.2677522451419065, -5.000000000000047962 ) ) ;
#94731=DIRECTION ( 'NONE',  ( -0.8660254037844359321, -0.5000000000000051070, -0.000000000000000000 ) ) ;
#94733=CARTESIAN_POINT ( 'NONE',  ( 203.4917594071969518, 276.5501419217281409, -14.41400602080355675 ) ) ;
#94734=CARTESIAN_POINT ( 'NONE',  ( 161.2313178023453588, 251.3861611254901618, 13.12937145726518473 ) ) ;
#94736=CARTESIAN_POINT ( 'NONE',  ( 171.6188493331028440, 251.5817016751831829, 7.205359137630009236 ) ) ;
#94738=CARTESIAN_POINT ( 'NONE',  ( 175.1691724511426571, 290.1382956017840797, -6.308240513192195031 ) ) ;
#94739=CARTESIAN_POINT ( 'NONE',  ( 153.1064336331667732, 270.6633677442188173, 13.89254713196513258 ) ) ;
#94742=CARTESIAN_POINT ( 'NONE',  ( 206.9059968923335475, 272.2752963222270068, 6.902135944297345560 ) ) ;
#94743=CARTESIAN_POINT ( 'NONE',  ( 180.6430269190001354, 266.9122829459220725, -14.79710749879348342 ) ) ;
#94744=CARTESIAN_POINT ( 'NONE',  ( 183.6422324172568210, 264.5785696717482551, 14.31652553825990104 ) ) ;
#94745=CARTESIAN_POINT ( 'NONE',  ( 199.5820190223589066, 281.0610403850588455, -17.29246150691365358 ) ) ;
#94748=CARTESIAN_POINT ( 'NONE',  ( 172.2641683536514563, 275.0456089790841361, 16.51748826216277877 ) ) ;
#94750=CARTESIAN_POINT ( 'NONE',  ( 160.4237162281696953, 273.2376347127639633, -15.66572034412998882 ) ) ;
#94752=CARTESIAN_POINT ( 'NONE',  ( 188.6780514684627406, 261.0664558817952638, 2.867164000797742585 ) ) ;
#94753=CARTESIAN_POINT ( 'NONE',  ( 207.6129110656513035, 271.0508850574501025, -5.265106572941297358 ) ) ;
#94754=CARTESIAN_POINT ( 'NONE',  ( 8.267668766103758671, 166.3923013555410080, 4.594050593750050204 ) ) ;
#94756=VERTEX_POINT ( 'NONE', #53876 ) ;
#94757=CARTESIAN_POINT ( 'NONE',  ( 174.9036676751700838, 255.2839639389062256, 8.319262650324212416 ) ) ;
#94760=CARTESIAN_POINT ( 'NONE',  ( 21.36630299834339652, 173.9548013555409796, -4.594050593750042211 ) ) ;
#94764=CARTESIAN_POINT ( 'NONE',  ( 199.9961967999579713, 267.3157181498997375, -6.792282625736725699 ) ) ;
#94765=CARTESIAN_POINT ( 'NONE',  ( 107.0484310652165476, 222.6115022471901739, -5.000000000000041744 ) ) ;
#94767=CARTESIAN_POINT ( 'NONE',  ( 149.7656787950428736, 271.2452304273818413, 12.35216892413132328 ) ) ;
#94773=CARTESIAN_POINT ( 'NONE',  ( 192.8108164209771473, 295.4770219581381525, -13.03931828728948439 ) ) ;
#94774=CARTESIAN_POINT ( 'NONE',  ( 73.70645301951556405, 223.3615022471903160, 5.000000000000046185 ) ) ;
#94776=CARTESIAN_POINT ( 'NONE',  ( 184.6509992051337861, 277.2187774885003364, -17.79388780315141005 ) ) ;
#94778=CARTESIAN_POINT ( 'NONE',  ( 51.43353571204313823, 194.3768266524159856, -9.188101187500091527 ) ) ;
#94781=CARTESIAN_POINT ( 'NONE',  ( 203.0006266442389062, 270.0465963985643612, -6.413920096036100915 ) ) ;
#94782=CARTESIAN_POINT ( 'NONE',  ( 190.7569505155522904, 300.2462651405980978, -5.670926626284815697 ) ) ;
#94784=ORIENTED_EDGE ( 'NONE', *, *, #78318, .T. ) ;
#94786=CARTESIAN_POINT ( 'NONE',  ( 163.7166294601506991, 282.3380383384618995, 10.03031969300557513 ) ) ;
#94787=CARTESIAN_POINT ( 'NONE',  ( 147.1567732723861468, 275.7639873447703280, 6.815990338468913556 ) ) ;
#94790=CARTESIAN_POINT ( 'NONE',  ( 202.3421728196210552, 280.1800714929709670, 16.85915999540957344 ) ) ;
#94791=CARTESIAN_POINT ( 'NONE',  ( 149.2765980486851731, 272.0923431290771646, -11.40617906909507973 ) ) ;
#94792=CARTESIAN_POINT ( 'NONE',  ( 188.8661607138717216, 269.9864860826438644, -14.08757442533680937 ) ) ;
#94793=ORIENTED_EDGE ( 'NONE', *, *, #84447, .F. ) ;
#94798=VERTEX_POINT ( 'NONE', #70591 ) ;
#94800=B_SPLINE_CURVE_WITH_KNOTS ( 'NONE', 3,
 ( #60187, #59703, #15093, #84554, #38395, #44998, #36400 ),
 .UNSPECIFIED., .F., .F.,
 ( 4, 3, 4 ),
 ( 2.060279009607550184E-15, 0.001498044985907314363, 0.002185450007172562263 ),
 .UNSPECIFIED. ) ;
#94803=CARTESIAN_POINT ( 'NONE',  ( 149.4539134692060145, 271.7852238117696402, 12.95627816374690688 ) ) ;
#94806=CARTESIAN_POINT ( 'NONE',  ( 188.9222622718724836, 273.7787661784663555, -15.66217235147567344 ) ) ;
#94807=CARTESIAN_POINT ( 'NONE',  ( 163.2324542190761747, 279.0921727632539842, -13.03962765338508945 ) ) ;
#94813=CARTESIAN_POINT ( 'NONE',  ( 157.1965120183049578, 258.3746497421212780, -18.06591467563559306 ) ) ;
#94814=CARTESIAN_POINT ( 'NONE',  ( 99.22679203974934126, 240.3464784336661637, 1.353441290958777525E-15 ) ) ;
#94815=CARTESIAN_POINT ( 'NONE',  ( 182.9913983929653796, 288.1037905649602635, -13.18133572435033862 ) ) ;
#94817=ORIENTED_EDGE ( 'NONE', *, *, #17613, .F. ) ;
#94821=CARTESIAN_POINT ( 'NONE',  ( 157.1924206424350814, 259.3163744206771639, 17.17865936927501380 ) ) ;
#94823=CARTESIAN_POINT ( 'NONE',  ( 62.31280629920263436, 206.7833772461660828, -9.188101187500095079 ) ) ;
#94826=CARTESIAN_POINT ( 'NONE',  ( 198.3791677596651368, 287.0441976074670833, 16.95474403075850134 ) ) ;
#94832=CARTESIAN_POINT ( 'NONE',  ( 177.9680647294031246, 288.9635307193505582, 11.07995066775972326 ) ) ;
#94833=CARTESIAN_POINT ( 'NONE',  ( 189.9457600613112902, 301.6512882219586800, 0.04117870562599101891 ) ) ;
#94835=CARTESIAN_POINT ( 'NONE',  ( 174.8478238567398080, 261.1473787441764784, -14.11631832387472762 ) ) ;
#94836=CARTESIAN_POINT ( 'NONE',  ( 174.1347695310112158, 277.0700907782643299, -15.64018019512398361 ) ) ;
#94837=CARTESIAN_POINT ( 'NONE',  ( 161.1747502674735415, 251.4841389699472529, -13.25152330924089839 ) ) ;
#94838=ADVANCED_FACE ( 'NONE', ( #24496 ), #55375, .T. ) ;
#94839=CARTESIAN_POINT ( 'NONE',  ( 147.5118896528469179, 275.1489077312122049, -3.975523961781759930 ) ) ;
#94844=CARTESIAN_POINT ( 'NONE',  ( 167.5479283814150051, 256.4993515244221385, 13.68654468072246466 ) ) ;
#94846=CARTESIAN_POINT ( 'NONE',  ( 110.3772162092389948, 234.5333772461660828, 9.188101187500095079 ) ) ;
#94848=CARTESIAN_POINT ( 'NONE',  ( 147.1731211915891322, 275.7356719181125868, 0.5879280619134324981 ) ) ;
#94850=CARTESIAN_POINT ( 'NONE',  ( 154.9528145190857344, 262.2608478075840708, -17.26679351315302213 ) ) ;
#94852=CARTESIAN_POINT ( 'NONE',  ( 204.2129321040862919, 276.9398213635460024, 14.41515352680879758 ) ) ;
#94857=CARTESIAN_POINT ( 'NONE',  ( 154.8126376379091482, 273.3510647301234258, -13.05415025889605651 ) ) ;
#94858=CARTESIAN_POINT ( 'NONE',  ( 185.2040473238361074, 261.9552295311297598, 9.692790394095107231 ) ) ;
#94860=CARTESIAN_POINT ( 'NONE',  ( 135.2750994722765654, 261.1589784336661637, -6.496448406907676862E-16 ) ) ;
#94861=CARTESIAN_POINT ( 'NONE',  ( 190.6639305750654785, 294.8294108904519248, -12.23618567142708002 ) ) ;
#94862=CARTESIAN_POINT ( 'NONE',  ( 189.1009243799269939, 299.7219271834727010, 4.948171813933484486 ) ) ;
#94865=B_SPLINE_CURVE_WITH_KNOTS ( 'NONE', 3,
 ( #97850, #93128, #60301, #37509 ),
 .UNSPECIFIED., .F., .F.,
 ( 4, 4 ),
 ( 0.000000000000000000, 0.001113216594625077464 ),
 .UNSPECIFIED. ) ;
#94866=CARTESIAN_POINT ( 'NONE',  ( 66.15596757637857195, 202.8768266524160140, 9.188101187500098632 ) ) ;
#94868=CARTESIAN_POINT ( 'NONE',  ( 157.4211152037729562, 257.9856256133486454, -16.71526195140576831 ) ) ;
#94871=CARTESIAN_POINT ( 'NONE',  ( 174.5041736941544741, 262.1790157217919273, 14.33285218853700549 ) ) ;
#94873=CARTESIAN_POINT ( 'NONE',  ( 178.8774038177254226, 291.7538915902231906, -6.223713788846963801 ) ) ;
#94874=CARTESIAN_POINT ( 'NONE',  ( 203.5477091018662748, 278.0920214017542662, -16.09930363698006062 ) ) ;
#94875=CARTESIAN_POINT ( 'NONE',  ( 153.6323727466833873, 269.3172676078306154, -15.66543061290010641 ) ) ;
#94876=CARTESIAN_POINT ( 'NONE',  ( 122.4023397829301700, 248.1427522451419065, -10.00000000000009415 ) ) ;
#94879=CARTESIAN_POINT ( 'NONE',  ( 189.9925954911225290, 301.5701668779311717, 0.1154287172046158938 ) ) ;
#94883=CARTESIAN_POINT ( 'NONE',  ( 40.22915850269944116, 194.0333772461660544, 9.188101187500095079 ) ) ;
#94886=CARTESIAN_POINT ( 'NONE',  ( -27.42236680055714260, 166.5217562850347406, 1.224646799147364892E-15 ) ) ;
#94888=CARTESIAN_POINT ( 'NONE',  ( 147.0670278774466908, 275.9194309285509235, 3.666898409139099257 ) ) ;
#94890=CARTESIAN_POINT ( 'NONE',  ( 198.2531640016911467, 277.4683007453174355, -15.40479037756460912 ) ) ;
#94891=CARTESIAN_POINT ( 'NONE',  ( 57.59477206639465408, 217.3927522451419634, 2.944929066748280225E-16 ) ) ;
#94893=CARTESIAN_POINT ( 'NONE',  ( 181.6765490640407847, 256.7658362468879432, 1.316456346048687998 ) ) ;
#94894=CARTESIAN_POINT ( 'NONE',  ( 158.8270733235451075, 260.0119502166541565, 17.68969926203419618 ) ) ;
#94895=CARTESIAN_POINT ( 'NONE',  ( 162.2082684172974325, 251.9275946936870980, -13.07642668292197285 ) ) ;
#94896=( BOUNDED_CURVE ( )  B_SPLINE_CURVE ( 2, ( #10731, #64926, #58304, #3153, #95872, #57309, #49713, #80668, #88279 ),
 .UNSPECIFIED., .F., .T. ) 
 B_SPLINE_CURVE_WITH_KNOTS ( ( 3, 2, 2, 2, 3 ),
 ( 0.05241935483870967943, 0.05376344086021505458, 0.05645161290322580488, 0.05913978494623656212, 0.06048387096774193727 ),
 .UNSPECIFIED. ) 
 CURVE ( )  GEOMETRIC_REPRESENTATION_ITEM ( )  RATIONAL_B_SPLINE_CURVE ( ( 0.9330127018922194093, 0.9330127018922194093, 1.000000000000000000, 0.8660254037844387076, 1.000000000000000000, 0.8660254037844387076, 1.000000000000000000, 0.9330127018922194093, 0.9330127018922194093 ) ) 
 REPRESENTATION_ITEM ( '' )  );
#94897=ORIENTED_EDGE ( 'NONE', *, *, #62419, .F. ) ;
#94898=CARTESIAN_POINT ( 'NONE',  ( 26.50806851326374414, 176.1115022471901739, -5.000000000000041744 ) ) ;
#94899=CARTESIAN_POINT ( 'NONE',  ( 184.5457051153594534, 294.3635293766698169, 10.03055039675435367 ) ) ;
#94900=CARTESIAN_POINT ( 'NONE',  ( 162.6220573360242270, 248.9773295930640131, 10.49878733418918486 ) ) ;
#94901=CARTESIAN_POINT ( 'NONE',  ( -8.160010933756074891, 166.0958772461660544, -9.188101187500095079 ) ) ;
#94903=CARTESIAN_POINT ( 'NONE',  ( 163.5210672374943783, 252.3610180297824570, 13.14880157932337390 ) ) ;
#94904=CARTESIAN_POINT ( 'NONE',  ( 170.9231213378963616, 262.8267322446009757, 16.60664178200664409 ) ) ;
#94906=CARTESIAN_POINT ( 'NONE',  ( 152.9262073036446168, 265.7710344717137900, 16.19159804214501008 ) ) ;
#94908=CARTESIAN_POINT ( 'NONE',  ( 55.54027346828191725, 191.3262482093457777, 3.021315404115420679E-15 ) ) ;
#94909=CARTESIAN_POINT ( 'NONE',  ( 183.3631853222992163, 257.4081984927463509, -1.690945316791027109 ) ) ;
#94912=CARTESIAN_POINT ( 'NONE',  ( 148.9285945872975390, 272.6951028054104427, -12.01265727652413240 ) ) ;
#94915=CARTESIAN_POINT ( 'NONE',  ( 165.8902591964293549, 285.5389980135179258, 0.4923433930893942878 ) ) ;
#94919=CARTESIAN_POINT ( 'NONE',  ( 153.4678846701812915, 275.0478545690473879, 10.56604701146394376 ) ) ;
#94920=FACE_OUTER_BOUND ( 'NONE', #33400, .T. ) ;
#94921=CARTESIAN_POINT ( 'NONE',  ( 61.65426615018220957, 199.7365022471902023, -10.00000000000009237 ) ) ;
#94922=ORIENTED_EDGE ( 'NONE', *, *, #39328, .F. ) ;
#94924=CARTESIAN_POINT ( 'NONE',  ( 192.0645969571214096, 297.9813550654635605, 11.46542907566974812 ) ) ;
#94925=CARTESIAN_POINT ( 'NONE',  ( 207.5686001603237116, 271.1276337968068333, 7.659944433763431704 ) ) ;
#94927=CARTESIAN_POINT ( 'NONE',  ( 191.6219713859826186, 298.2580554142066376, 8.895068270853277781 ) ) ;
#94929=CARTESIAN_POINT ( 'NONE',  ( 193.8603219414924013, 294.8710681561126989, 15.36476279452078586 ) ) ;
#94931=CARTESIAN_POINT ( 'NONE',  ( 158.7920399039511494, 277.9748776850930767, -9.821990816589480033 ) ) ;
#94933=ORIENTED_EDGE ( 'NONE', *, *, #15028, .T. ) ;
#94935=CARTESIAN_POINT ( 'NONE',  ( 155.5995420464182644, 262.6346450740109617, -17.48312782858739567 ) ) ;
#94936=ORIENTED_EDGE ( 'NONE', *, *, #90945, .F. ) ;
#94939=B_SPLINE_CURVE_WITH_KNOTS ( 'NONE', 3,
 ( #98763, #35439, #91173, #66342 ),
 .UNSPECIFIED., .F., .F.,
 ( 4, 4 ),
 ( 0.006879015221108502644, 0.01190597477310000214 ),
 .UNSPECIFIED. ) ;
#94942=CARTESIAN_POINT ( 'NONE',  ( 200.9111546617170916, 282.6586676490145464, 17.66063511622358106 ) ) ;
#94943=CARTESIAN_POINT ( 'NONE',  ( 166.1691510717052154, 273.9072633124648632, -15.34805146679062382 ) ) ;
#94945=CARTESIAN_POINT ( 'NONE',  ( 151.3795629253287132, 275.1161925579037870, -8.452185327743000798 ) ) ;
#94946=VERTEX_POINT ( 'NONE', #49795 ) ;
#94949=CARTESIAN_POINT ( 'NONE',  ( 171.1327466086072207, 254.6685794175523938, -11.52810047878565669 ) ) ;
#94951=ORIENTED_EDGE ( 'NONE', *, *, #69760, .F. ) ;
#94952=ORIENTED_EDGE ( 'NONE', *, *, #19780, .F. ) ;
#94953=CARTESIAN_POINT ( 'NONE',  ( 160.0395937287001402, 268.6003992623327576, -16.49027686160719952 ) ) ;
#94955=CARTESIAN_POINT ( 'NONE',  ( 160.7841707400127405, 270.7800417481713566, 15.89061575048816444 ) ) ;
#94959=CARTESIAN_POINT ( 'NONE',  ( 147.7897704884714472, 274.6676040054608166, 7.256941229896001211 ) ) ;
#94960=CARTESIAN_POINT ( 'NONE',  ( 190.5526305594705434, 299.9695577504274979, -4.324655322867677398 ) ) ;
#94970=CARTESIAN_POINT ( 'NONE',  ( 205.8030308266901898, 274.1856895869457844, 10.55961490432110317 ) ) ;
#94971=CARTESIAN_POINT ( 'NONE',  ( 164.8537203408104972, 245.1119758834023230, 2.926011033004258355 ) ) ;
#94972=CARTESIAN_POINT ( 'NONE',  ( 159.5284711081640125, 254.3355781173132755, 15.34104435652608522 ) ) ;
#94977=CARTESIAN_POINT ( 'NONE',  ( 168.3758771850754670, 256.9182401831289440, -14.77350533378223219 ) ) ;
#94978=ADVANCED_FACE ( 'NONE', ( #64504 ), #4188, .T. ) ;
#94979=CARTESIAN_POINT ( 'NONE',  ( 159.5050723400634638, 254.3761059724978679, -15.34938048045353298 ) ) ;
#94982=B_SPLINE_CURVE_WITH_KNOTS ( 'NONE', 3,
 ( #5102, #66886, #43588, #52178 ),
 .UNSPECIFIED., .F., .F.,
 ( 4, 4 ),
 ( 0.0005619842127425911946, 0.0007738637477710976062 ),
 .UNSPECIFIED. ) ;
#94983=CARTESIAN_POINT ( 'NONE',  ( 200.2316334480823912, 283.8356329158505105, 17.02791935830326508 ) ) ;
#94986=CARTESIAN_POINT ( 'NONE',  ( 176.5337195050044556, 270.3037592414455048, -17.69951539620915071 ) ) ;
#94990=CARTESIAN_POINT ( 'NONE',  ( 13.42747647338826589, 191.8927522451419350, 2.944929066748280225E-16 ) ) ;
#94991=CARTESIAN_POINT ( 'NONE',  ( 97.33288211261837830, 220.8768266524160140, 9.188101187500096856 ) ) ;
#94994=CARTESIAN_POINT ( 'NONE',  ( 162.6684717218148251, 248.8969375186720754, 11.76041465758671833 ) ) ;
#94995=CARTESIAN_POINT ( 'NONE',  ( 28.72751893051112049, 178.2048013555409796, 4.594050593750051981 ) ) ;
#94996=CARTESIAN_POINT ( 'NONE',  ( 161.1027382213887336, 251.6088674925233022, 13.55451100897754557 ) ) ;
#94998=ORIENTED_EDGE ( 'NONE', *, *, #31635, .T. ) ;
#95002=CARTESIAN_POINT ( 'NONE',  ( 199.7522530777181089, 267.1256835885929490, -2.850022460144068237 ) ) ;
#95003=CARTESIAN_POINT ( 'NONE',  ( 186.0244278979135117, 262.8604796214907537, 11.87503556831948615 ) ) ;
#95011=CARTESIAN_POINT ( 'NONE',  ( 26.96797095936772237, 192.5024278399161233, 9.188101187500095079 ) ) ;
#95012=CARTESIAN_POINT ( 'NONE',  ( 86.96746701141694302, 211.0177522451417929, 5.000000000000051514 ) ) ;
#95013=CARTESIAN_POINT ( 'NONE',  ( 199.8909283227609990, 276.8366623509729152, 15.27167089021202351 ) ) ;
#95016=DIRECTION ( 'NONE',  ( 0.5000000000000144329, -0.8660254037844303809, -1.474271392894062072E-14 ) ) ;
#95018=CARTESIAN_POINT ( 'NONE',  ( -6.536213301660246167, 167.0333772461660828, 9.188101187500095079 ) ) ;
#95020=CARTESIAN_POINT ( 'NONE',  ( 207.7296438747196134, 270.8486979012336633, -6.692930657757584001 ) ) ;
#95021=CARTESIAN_POINT ( 'NONE',  ( 186.5316309442283114, 282.7232008768231140, 16.16643943244534398 ) ) ;
#95022=CARTESIAN_POINT ( 'NONE',  ( 148.4042165687623083, 273.6033521758856750, -8.709765892313745539 ) ) ;
#95025=CARTESIAN_POINT ( 'NONE',  ( 204.8284483594339065, 275.8737159363993214, 14.69997973035875383 ) ) ;
#95026=CARTESIAN_POINT ( 'NONE',  ( 191.8329718516215223, 298.3825415164982928, -8.871589506312979267 ) ) ;
#95027=CARTESIAN_POINT ( 'NONE',  ( 207.1122325394003951, 271.9180857031755636, 7.794245785756032774 ) ) ;
#95028=ORIENTED_EDGE ( 'NONE', *, *, #70725, .T. ) ;
#95029=CARTESIAN_POINT ( 'NONE',  ( 136.8541387121308617, 256.4865022471902876, -10.00000000000009592 ) ) ;
#95030=CARTESIAN_POINT ( 'NONE',  ( 118.9295641673753181, 227.2202760586659736, -5.415160957724236172E-17 ) ) ;
#95033=EDGE_CURVE ( 'NONE', #2343, #58518, #5197, .T. ) ;
#95037=CARTESIAN_POINT ( 'NONE',  ( 191.1107143855515176, 299.6335281438774700, -6.486502120340617239 ) ) ;
#95039=CARTESIAN_POINT ( 'NONE',  ( 189.6294122595523675, 261.2013800515091475, -4.514607050631846086 ) ) ;
#95040=CARTESIAN_POINT ( 'NONE',  ( 196.4170778717353585, 290.4426369823788718, -17.78762421190030452 ) ) ;
#95043=CARTESIAN_POINT ( 'NONE',  ( 173.5071485195266803, 289.9167268689076877, -1.068890946380929075 ) ) ;
#95044=CARTESIAN_POINT ( 'NONE',  ( 194.4178591205541409, 270.7991877699529937, -14.20622043910200460 ) ) ;
#95047=CARTESIAN_POINT ( 'NONE',  ( 175.5424091614122517, 278.6358477417585959, 15.42837206623358348 ) ) ;
#95049=CARTESIAN_POINT ( 'NONE',  ( 166.5715075414655360, 270.4169618060113862, -16.29706984472633735 ) ) ;
#95053=CARTESIAN_POINT ( 'NONE',  ( 200.2438720683531415, 272.4341333479218861, 12.65294705144797760 ) ) ;
#95056=CARTESIAN_POINT ( 'NONE',  ( 152.7153488183568300, 266.1362520814392951, 17.33540622643059237 ) ) ;
#95062=CARTESIAN_POINT ( 'NONE',  ( 192.2621181266863459, 288.2322237920654402, -15.87800504598256168 ) ) ;
#95064=CARTESIAN_POINT ( 'NONE',  ( 167.8294318762166029, 280.8099396157227829, 12.36612508801571231 ) ) ;
#95065=CARTESIAN_POINT ( 'NONE',  ( 194.6943296385021824, 293.4265244509877562, -16.10917128197217352 ) ) ;
#95066=CARTESIAN_POINT ( 'NONE',  ( 21.64925731690437516, 171.7592609112379876, 2.679491924311254714 ) ) ;
#95069=CARTESIAN_POINT ( 'NONE',  ( 188.6836721603714864, 293.3912136806342232, 12.63380796591361133 ) ) ;
#95074=CARTESIAN_POINT ( 'NONE',  ( 155.6328838216860220, 261.0829332228125850, -17.51014940606912518 ) ) ;
#95075=EDGE_LOOP ( 'NONE', ( #33227, #29140, #43343, #51306 ) ) ;
#95078=CARTESIAN_POINT ( 'NONE',  ( 175.6813301723168479, 259.2852654454819117, 12.45547364025740045 ) ) ;
#95079=ORIENTED_EDGE ( 'NONE', *, *, #95662, .T. ) ;
#95082=CARTESIAN_POINT ( 'NONE',  ( 173.2789054804935631, 270.6729449864580488, 16.65581685045554039 ) ) ;
#95083=CARTESIAN_POINT ( 'NONE',  ( 203.4696564630250464, 278.2272125378923988, -16.38980782817167636 ) ) ;
#95086=CARTESIAN_POINT ( 'NONE',  ( 186.0705390081322435, 282.4759132538421227, -17.12146972818776547 ) ) ;
#95087=CARTESIAN_POINT ( 'NONE',  ( 164.3883575065421496, 245.9180079563093955, -2.230252308397467687 ) ) ;
#95088=CARTESIAN_POINT ( 'NONE',  ( 147.8696095030242645, 274.5293187758293811, -6.165255295277477288 ) ) ;
#95089=CARTESIAN_POINT ( 'NONE',  ( 158.4485968073939546, 275.2084588272041401, -13.86993402366507944 ) ) ;
#95091=CARTESIAN_POINT ( 'NONE',  ( 200.8251833487811666, 282.8075743310126882, -16.74393672780000131 ) ) ;
#95093=CARTESIAN_POINT ( 'NONE',  ( 153.9280534239306917, 279.9716514717067639, 2.220587593257353554 ) ) ;
#95094=ADVANCED_FACE ( 'NONE', ( #83727 ), #37564, .T. ) ;
#95095=CARTESIAN_POINT ( 'NONE',  ( 135.2486435959970947, 239.7048013555409796, 4.594050593750051981 ) ) ;
#95098=ORIENTED_EDGE ( 'NONE', *, *, #41874, .T. ) ;
#95101=ORIENTED_EDGE ( 'NONE', *, *, #74601, .F. ) ;
#95102=CARTESIAN_POINT ( 'NONE',  ( 203.5034052210150719, 276.4946534009981178, 13.91832450903958751 ) ) ;
#95103=CARTESIAN_POINT ( 'NONE',  ( 177.5631567369229913, 253.5128631816587870, 1.374242336938259701 ) ) ;
#95105=CARTESIAN_POINT ( 'NONE',  ( 147.3869853863401715, 275.3652482668841230, 3.850002650366144419 ) ) ;
#95106=CARTESIAN_POINT ( 'NONE',  ( 157.4449103128602587, 280.3754508376611057, -7.050241416987695686 ) ) ;
#95107=CARTESIAN_POINT ( 'NONE',  ( 152.7729059155601021, 266.0365602647466972, -17.50667083025758686 ) ) ;
#95108=CARTESIAN_POINT ( 'NONE',  ( 176.9886338728968553, 288.6665034793379050, -9.311589415884686360 ) ) ;
#95109=CARTESIAN_POINT ( 'NONE',  ( 171.4101398265137846, 280.2079561268039924, 13.77150215915619214 ) ) ;
#95110=CARTESIAN_POINT ( 'NONE',  ( 177.6986938504743136, 255.3162907930642405, -8.390269233711947550 ) ) ;
#95111=ORIENTED_EDGE ( 'NONE', *, *, #56188, .T. ) ;
#95112=B_SPLINE_CURVE_WITH_KNOTS ( 'NONE', 3,
 ( #93057, #99152, #92096, #68730 ),
 .UNSPECIFIED., .F., .F.,
 ( 4, 4 ),
 ( 0.005695445479479283035, 0.01374854309124446533 ),
 .UNSPECIFIED. ) ;
#95117=CARTESIAN_POINT ( 'NONE',  ( 201.1778739778297052, 267.9238834610532081, -2.849212060748330888 ) ) ;
#95118=CARTESIAN_POINT ( 'NONE',  ( 152.5006243422696741, 266.5081657836506679, -15.99602084911275135 ) ) ;
#95119=CARTESIAN_POINT ( 'NONE',  ( 190.2318383114841254, 301.1557861577188078, 3.177919994438449525 ) ) ;
#95120=CARTESIAN_POINT ( 'NONE',  ( 162.9148248802443106, 248.4702413316674381, 9.709394404200100581 ) ) ;
#95121=CARTESIAN_POINT ( 'NONE',  ( 163.4970835327194436, 283.9977148944103078, -7.100329127627979631 ) ) ;
#95122=CARTESIAN_POINT ( 'NONE',  ( 160.9062962349007080, 281.5834788170423622, 5.946759227913918089 ) ) ;
#95123=CARTESIAN_POINT ( 'NONE',  ( -22.42236680055709641, 157.8615022471902591, 0.000000000000000000 ) ) ;
#95124=VERTEX_POINT ( 'NONE', #44663 ) ;
#95127=CARTESIAN_POINT ( 'NONE',  ( 192.9525843507564957, 275.9342408156254578, -16.09309137864095263 ) ) ;
#95129=CARTESIAN_POINT ( 'NONE',  ( 192.0331311261993790, 298.0358554833232461, 11.82583305898340953 ) ) ;
#95130=LINE ( 'NONE', #78908, #52677 ) ;
#95134=CARTESIAN_POINT ( 'NONE',  ( -8.782727014549898570, 174.9244531367911293, -4.594050593750046652 ) ) ;
#95135=CARTESIAN_POINT ( 'NONE',  ( 81.20281187136818346, 223.8149278399160664, 9.188101187500093303 ) ) ;
#95137=CARTESIAN_POINT ( 'NONE',  ( 193.8354046899084153, 268.4885937380259406, 12.87375928640720524 ) ) ;
#95138=CARTESIAN_POINT ( 'NONE',  ( -7.266922234329411978, 166.6115022471902591, 10.00000000000009592 ) ) ;
#95142=CARTESIAN_POINT ( 'NONE',  ( 160.8951580803594936, 281.6687235497548727, 5.528266179044310391 ) ) ;
#95144=B_SPLINE_CURVE_WITH_KNOTS ( 'NONE', 3,
 ( #52687, #98827, #13709, #53681 ),
 .UNSPECIFIED., .F., .F.,
 ( 4, 4 ),
 ( 0.000000000000000000, 0.004151113516842898886 ),
 .UNSPECIFIED. ) ;
#95146=CARTESIAN_POINT ( 'NONE',  ( 207.9138579432917879, 270.5296297749978294, 5.245628703246491220 ) ) ;
#95147=CARTESIAN_POINT ( 'NONE',  ( 175.7622132985686392, 274.0430017844784629, -17.75579533532145504 ) ) ;
#95148=CARTESIAN_POINT ( 'NONE',  ( 190.0370014622527322, 286.8089957100377205, 16.96978714573610247 ) ) ;
#95151=CARTESIAN_POINT ( 'NONE',  ( 49.16021902710897251, 193.0643266524159856, -9.188101187500093303 ) ) ;
#95154=CARTESIAN_POINT ( 'NONE',  ( 70.10703493326258240, 211.2833772461660544, -9.188101187500095079 ) ) ;
#95155=CARTESIAN_POINT ( 'NONE',  ( 161.8807657183444064, 250.2612843381103573, -13.52770735624900311 ) ) ;
#95156=FACE_OUTER_BOUND ( 'NONE', #55641, .T. ) ;
#95157=ADVANCED_FACE ( 'NONE', ( #51803 ), #79921, .F. ) ;
#95159=CARTESIAN_POINT ( 'NONE',  ( 192.9064638172013417, 270.9369261147751331, 14.92505667092759758 ) ) ;
#95160=CARTESIAN_POINT ( 'NONE',  ( 152.2331915504236690, 266.9713729667379880, 15.44938373281010158 ) ) ;
#95164=CARTESIAN_POINT ( 'NONE',  ( 196.2293283710122012, 290.7678286567270902, -17.07152402978540096 ) ) ;
#95165=ORIENTED_EDGE ( 'NONE', *, *, #21270, .F. ) ;
#95167=CARTESIAN_POINT ( 'NONE',  ( 73.95019621043851998, 207.3768266524160140, 9.188101187500096856 ) ) ;
#95169=CARTESIAN_POINT ( 'NONE',  ( 169.4535728852475813, 288.8904079931804745, -1.135962625816850480 ) ) ;
#95171=CARTESIAN_POINT ( 'NONE',  ( 153.6692166914362474, 264.4841044615581040, 18.11141839824787070 ) ) ;
#95172=EDGE_CURVE ( 'NONE', #30881, #22269, #24011, .T. ) ;
#95175=CARTESIAN_POINT ( 'NONE',  ( 124.7297830591487724, 249.4865022471903160, 10.00000000000009237 ) ) ;
#95176=CARTESIAN_POINT ( 'NONE',  ( 14.74455677852503932, 185.9865022471903160, -10.00000000000009592 ) ) ;
#95179=CARTESIAN_POINT ( 'NONE',  ( 185.0482011028098270, 271.4938003020888004, 15.97631097496702424 ) ) ;
#95181=CARTESIAN_POINT ( 'NONE',  ( 163.2835940097493790, 247.8315144631017404, 11.08416305054517359 ) ) ;
#95184=ORIENTED_EDGE ( 'NONE', *, *, #87124, .F. ) ;
#95185=CARTESIAN_POINT ( 'NONE',  ( 173.2975034251014392, 251.6701835053000593, -0.1618941120760299945 ) ) ;
#95188=CARTESIAN_POINT ( 'NONE',  ( 45.83126033165607538, 197.2677522451418781, 10.00000000000009592 ) ) ;
#95198=CARTESIAN_POINT ( 'NONE',  ( 48.59171630976688760, 198.8615022471902591, -10.00000000000009592 ) ) ;
#95200=ORIENTED_EDGE ( 'NONE', *, *, #8741, .T. ) ;
#95203=( BOUNDED_CURVE ( )  B_SPLINE_CURVE ( 2, ( #3162, #26933, #34048, #65424, #64937, #50221, #43611, #80680, #11255 ),
 .UNSPECIFIED., .F., .T. ) 
 B_SPLINE_CURVE_WITH_KNOTS ( ( 3, 2, 2, 2, 3 ),
 ( 0.2298387096774193450, 0.2311827956989247201, 0.2338709677419354704, 0.2365591397849462485, 0.2379032258064516236 ),
 .UNSPECIFIED. ) 
 CURVE ( )  GEOMETRIC_REPRESENTATION_ITEM ( )  RATIONAL_B_SPLINE_CURVE ( ( 0.9330127018922194093, 0.9330127018922194093, 1.000000000000000000, 0.8660254037844387076, 1.000000000000000000, 0.8660254037844387076, 1.000000000000000000, 0.9330127018922194093, 0.9330127018922194093 ) ) 
 REPRESENTATION_ITEM ( '' )  );
#95204=ADVANCED_FACE ( 'NONE', ( #48177 ), #36259, .F. ) ;
#95205=CARTESIAN_POINT ( 'NONE',  ( 204.8284483594339065, 275.8737159363993214, 14.69997973035875383 ) ) ;
#95206=CARTESIAN_POINT ( 'NONE',  ( 178.8794786194264930, 266.0179056750089899, -16.39995361575137167 ) ) ;
#95208=CARTESIAN_POINT ( 'NONE',  ( 154.8556227199321427, 262.4291889417971788, 17.77326384500479861 ) ) ;
#95211=CARTESIAN_POINT ( 'NONE',  ( 164.0022889252203129, 246.5866983543648701, 5.359592124775450550 ) ) ;
#95216=CARTESIAN_POINT ( 'NONE',  ( 79.66011734693590540, 225.9869531367911293, 4.594050593750046652 ) ) ;
#95217=ORIENTED_EDGE ( 'NONE', *, *, #83049, .F. ) ;
#95218=CARTESIAN_POINT ( 'NONE',  ( 150.2600589618944582, 271.4479585178293632, 12.50551682633786221 ) ) ;
#95221=B_SPLINE_CURVE_WITH_KNOTS ( 'NONE', 3,
 ( #18486, #49371, #18994, #10884, #41759, #72704, #65070, #49867, #80830, #76181, #21459, #99470, #52845, #36644, #38122, #74690, #68544, #89900, #91387, #84296, #29557, #28550, #75180, #83794, #59433, #14844, #98972, #37150, #60430, #90412, #12889, #90910, #30045, #5752, #97490, #36147, #6756, #67550, #37633, #60934, #98482, #44242, #52346, #82807, #13855, #14358, #51352, #45244 ),
 .UNSPECIFIED., .F., .F.,
 ( 4, 2, 2, 2, 2, 2, 2, 2, 2, 2, 2, 2, 2, 2, 2, 2, 2, 2, 2, 2, 2, 2, 2, 4 ),
 ( 0.002005250820186432748, 0.002448144949604836359, 0.002669592014314038381, 0.002891039079023239970, 0.003001762611377881314, 0.003112486143732522657, 0.003223209676087163134, 0.003333933208441804477, 0.003555380273151086297, 0.003776827337860368984, 0.004662615596697672338, 0.005548403855534974824, 0.006434192114372278178, 0.006877086243790892992, 0.007319980373209508673, 0.007430703905564181241, 0.007486065671741557424, 0.007541427437918933607, 0.007652150970273684238, 0.007762874502628435737, 0.008205768632047496375, 0.008427215696757027127, 0.008648662761466557880, 0.009091556890885619385 ),
 .UNSPECIFIED. ) ;
#95222=CARTESIAN_POINT ( 'NONE',  ( 168.3457246661429565, 267.1986757268145993, -17.36865887974328615 ) ) ;
#95223=ORIENTED_EDGE ( 'NONE', *, *, #24576, .F. ) ;
#95226=CARTESIAN_POINT ( 'NONE',  ( 156.6812872898450735, 261.2670451491295012, 0.000000000000000000 ) ) ;
#95228=FACE_OUTER_BOUND ( 'NONE', #21163, .T. ) ;
#95231=ORIENTED_EDGE ( 'NONE', *, *, #86416, .T. ) ;
#95234=CARTESIAN_POINT ( 'NONE',  ( 162.8480293090835005, 248.5859346546387769, -9.753154585358942086 ) ) ;
#95235=ORIENTED_EDGE ( 'NONE', *, *, #64637, .F. ) ;
#95239=CARTESIAN_POINT ( 'NONE',  ( -0.4289299871626708338, 163.8927522451418213, 10.00000000000009592 ) ) ;
#95241=B_SPLINE_CURVE_WITH_KNOTS ( 'NONE', 3,
 ( #17206, #71932, #64825, #48112, #59056, #2536, #82451, #33418, #26326, #20602, #71433, #90027, #25837, #55686, #79053, #18726, #74816, #36279, #9642, #56712, #87695, #49123, #13014, #32908, #3538, #63815, #43873, #88179, #5395, #94255, #40501, #49610, #2023, #90540, #5886, #52473, #75305, #98102, #14488, #75805, #21590, #45367, #67178, #92031, #14962, #67683, #36775, #22079, #37276, #6873, #83420, #22577 ),
 .UNSPECIFIED., .F., .F.,
 ( 4, 2, 2, 2, 2, 2, 2, 2, 2, 2, 2, 2, 2, 2, 2, 2, 2, 2, 2, 2, 2, 2, 2, 2, 2, 4 ),
 ( 0.0006380557224042569678, 0.001138346313157871745, 0.001638636903911486632, 0.001888782199288259380, 0.002138927494665032129, 0.002264000142353447126, 0.002389072790041862123, 0.002514145437730277120, 0.002639218085418692118, 0.002889363380795566781, 0.003139508676172441011, 0.003639799266926106204, 0.004640380448433350721, 0.005640961629940595239, 0.006141252220694258697, 0.006391397516071126855, 0.006641542811447994146, 0.006704079135292192321, 0.006766615459136391363, 0.006829151782980589537, 0.006891688106824788579, 0.007141833402201395661, 0.007642123992954569928, 0.008142414583707744194, 0.008392559879084330460, 0.008642705174460914991 ),
 .UNSPECIFIED. ) ;
#95243=FACE_OUTER_BOUND ( 'NONE', #64793, .T. ) ;
#95245=CARTESIAN_POINT ( 'NONE',  ( -22.42236680055709641, 157.8615022471902591, 0.000000000000000000 ) ) ;
#95246=CARTESIAN_POINT ( 'NONE',  ( 192.2047958520457200, 271.8935057982316721, 14.16859286990318978 ) ) ;
#95249=B_SPLINE_CURVE_WITH_KNOTS ( 'NONE', 3,
 ( #70248, #40833, #854, #48464, #7970, #71779, #8957, #2378, #85509, #47940, #94099, #64157, #71277, #31733, #93591, #16552, #47447, #78376, #24650, #78882, #56032, #1867, #9467, #40338, #32751, #63655, #87026, #94594, #25148, #17558, #79406, #95108, #56553, #15536, #46436, #77365, #69749, #360, #31247, #62134, #28021, #36109, #64669, #83249, #88025, #43711, #28513, #98938, #59395, #35625, #58896, #90372 ),
 .UNSPECIFIED., .F., .F.,
 ( 4, 2, 2, 2, 2, 2, 2, 2, 2, 2, 2, 2, 2, 2, 2, 2, 2, 2, 2, 2, 2, 2, 2, 2, 2, 4 ),
 ( 0.0007684721497847792765, 0.001259722117377088746, 0.001750972084969398216, 0.001996597068765640012, 0.002242222052561882242, 0.002365034544460022006, 0.002487847036358162203, 0.002610659528256302833, 0.002733472020154442596, 0.002979097003950728628, 0.003224721987747015094, 0.003715971955339622285, 0.004698471890524970676, 0.005680971825710319500, 0.006172221793303030342, 0.006417846777099385329, 0.006663471760895741183, 0.006724878006844846844, 0.006786284252793953371, 0.006847690498743059032, 0.006909096744692165559, 0.007154721728488628099, 0.007645971696081424809, 0.008137221663674221520, 0.008382846647470635487, 0.008628471631267047720 ),
 .UNSPECIFIED. ) ;
#95250=EDGE_CURVE ( 'NONE', #3137, #51575, #60131, .T. ) ;
#95253=CARTESIAN_POINT ( 'NONE',  ( 149.0417755939924405, 274.5147917236959643, 9.103005964151618556 ) ) ;
#95254=CARTESIAN_POINT ( 'NONE',  ( 161.4025183475459073, 251.0896330829197041, 14.50747140106038735 ) ) ;
#95260=CARTESIAN_POINT ( 'NONE',  ( 174.8794285395499344, 290.4103569552396493, -6.460613355744903252 ) ) ;
#95262=CYLINDRICAL_SURFACE ( 'NONE', #18751, 17.82106496071139645 ) ;
#95268=CARTESIAN_POINT ( 'NONE',  ( 164.2953672501826929, 246.0790718049323687, -2.576662677987826111 ) ) ;
#95269=CARTESIAN_POINT ( 'NONE',  ( 178.5610891250362045, 265.5608437732782363, -14.90458899103854051 ) ) ;
#95270=CARTESIAN_POINT ( 'NONE',  ( 194.6056312668138162, 268.3159250634341788, -12.34445183914189670 ) ) ;
#95274=CARTESIAN_POINT ( 'NONE',  ( 171.6149855087873561, 274.5829882844238341, 16.21406585132328004 ) ) ;
#95278=CARTESIAN_POINT ( 'NONE',  ( 207.8984236726843164, 270.5563627158673512, -6.084369154771423815 ) ) ;
#95280=CARTESIAN_POINT ( 'NONE',  ( 6.454167755106333892, 174.5333772461660828, 9.188101187500095079 ) ) ;
#95285=CARTESIAN_POINT ( 'NONE',  ( 164.4578252119609090, 245.7976863610386999, -6.211333091911165560 ) ) ;
#95287=CARTESIAN_POINT ( 'NONE',  ( 29.86365662933068066, 197.2369531367911293, -4.594050593750048428 ) ) ;
#95291=CARTESIAN_POINT ( 'NONE',  ( 181.7688266870327709, 294.4230621335508999, 6.401746037419756341 ) ) ;
#95292=B_SPLINE_CURVE_WITH_KNOTS ( 'NONE', 3,
 ( #56134, #95206, #34837, #80502 ),
 .UNSPECIFIED., .F., .F.,
 ( 4, 4 ),
 ( 0.008997718677290020978, 0.01512492955424769338 ),
 .UNSPECIFIED. ) ;
#95293=CARTESIAN_POINT ( 'NONE',  ( 191.0862225170008628, 299.6759493045793192, -9.402218231374108726 ) ) ;
#95294=CARTESIAN_POINT ( 'NONE',  ( 149.2197514927185580, 272.1908042522468349, 11.55035869369450197 ) ) ;
#95295=CARTESIAN_POINT ( 'NONE',  ( 181.7535138776731003, 279.7363418824564860, -16.10976311149228479 ) ) ;
#95297=B_SPLINE_SURFACE_WITH_KNOTS ( 'NONE', 3, 1, ( 
 ( #49331, #80270 ),
 ( #19458, #26537 ),
 ( #11839, #6711 ),
 ( #6207, #44195 ),
 ( #67503, #68499 ),
 ( #52302, #36101 ),
 ( #14311, #13808 ),
 ( #45683, #59898 ),
 ( #37589, #84743 ),
 ( #29026, #90865 ),
 ( #99423, #60883 ),
 ( #67004, #90361 ),
 ( #21417, #36599 ),
 ( #30000, #91845 ),
 ( #68007, #13331 ),
 ( #15284, #82765 ),
 ( #38080, #45197 ),
 ( #74646, #22895 ),
 ( #22407, #75133 ),
 ( #76609, #53300 ),
 ( #83241, #53780 ),
 ( #7195, #30504 ),
 ( #84253, #68993 ),
 ( #14801, #99919 ),
 ( #5710, #98435 ),
 ( #61394, #92346 ),
 ( #44689, #75619 ),
 ( #37102, #5222 ),
 ( #97929, #98931 ),
 ( #28504, #59385 ),
 ( #76137, #20942 ),
 ( #51823, #29509 ),
 ( #60387, #91342 ),
 ( #21903, #52791 ) ),
 .UNSPECIFIED., .T., .F., .F.,
 ( 4, 2, 2, 2, 2, 2, 2, 2, 2, 2, 2, 2, 2, 2, 2, 2, 4 ),
 ( 2, 2 ),
 ( 0.000000000000000000, 0.06250000000000000000, 0.1250000000000000000, 0.1875000000000000000, 0.2500000000000000000, 0.3125000000000000000, 0.3750000000000000000, 0.4375000000000000000, 0.5000000000000000000, 0.5625000000000000000, 0.6250000000000000000, 0.6875000000000000000, 0.7500000000000000000, 0.8125000000000000000, 0.8750000000000000000, 0.9375000000000000000, 1.000000000000000000 ),
 ( 0.000000000000000000, 1.000000000000000000 ),
 .UNSPECIFIED. ) ;
#95298=CARTESIAN_POINT ( 'NONE',  ( 190.1042286455896999, 298.6140004201554348, -8.058983885598134833 ) ) ;
#95299=CARTESIAN_POINT ( 'NONE',  ( 92.02936583101279666, 212.3932355074535678, -2.679491924311248496 ) ) ;
#95302=CARTESIAN_POINT ( 'NONE',  ( 84.89261448506465513, 206.4865022471901455, 1.119607411625061291E-15 ) ) ;
#95303=CARTESIAN_POINT ( 'NONE',  ( 165.5845016731641124, 245.8462254865437160, 0.7221155814038995313 ) ) ;
#95304=CARTESIAN_POINT ( 'NONE',  ( 161.9385560670746145, 267.8585340882163450, -16.83787897924083055 ) ) ;
#95306=CARTESIAN_POINT ( 'NONE',  ( 42.77328167419873495, 189.3768266524160140, 9.188101187500098632 ) ) ;
#95307=CARTESIAN_POINT ( 'NONE',  ( 159.4285914931787431, 254.5085746851079023, 15.41072477910873673 ) ) ;
#95312=VERTEX_POINT ( 'NONE', #91393 ) ;
#95313=CARTESIAN_POINT ( 'NONE',  ( 167.5137480047340830, 285.0270040894174031, 7.743640753283266953 ) ) ;
#95314=CARTESIAN_POINT ( 'NONE',  ( 168.0608149624495979, 281.9755942893786482, -10.94157658500136598 ) ) ;
#95316=CARTESIAN_POINT ( 'NONE',  ( 87.40047971330908183, 231.2677522451419065, -5.000000000000047962 ) ) ;
#95318=CARTESIAN_POINT ( 'NONE',  ( 163.4216610345155800, 247.5923753613567442, 10.58669027323842826 ) ) ;
#95319=CARTESIAN_POINT ( 'NONE',  ( 110.3501529135968013, 224.5177522451418213, 5.000000000000051514 ) ) ;
#95320=CARTESIAN_POINT ( 'NONE',  ( 157.0858749576330524, 258.5662787524049122, 18.43576942457294976 ) ) ;
#95323=CARTESIAN_POINT ( 'NONE',  ( 24.36335893204212155, 173.3262482093457777, 3.021315404115420679E-15 ) ) ;
#95333=EDGE_CURVE ( 'NONE', #41802, #94756, #61395, .T. ) ;
#95336=CARTESIAN_POINT ( 'NONE',  ( 196.9976074755333286, 289.4371302133026802, -16.79549473444794216 ) ) ;
#95337=ORIENTED_EDGE ( 'NONE', *, *, #93688, .T. ) ;
#95338=CARTESIAN_POINT ( 'NONE',  ( 152.6740002182599767, 266.2078699576288159, -17.16212636348624088 ) ) ;
#95340=CARTESIAN_POINT ( 'NONE',  ( 193.5005633302724277, 262.8551920378705518, -5.236817587991198231 ) ) ;
#95343=CARTESIAN_POINT ( 'NONE',  ( 204.8057697639265768, 275.9129964160624695, -12.68356524114230766 ) ) ;
#95344=CARTESIAN_POINT ( 'NONE',  ( 113.7598676209481994, 245.6744531367911293, 4.594050593750047540 ) ) ;
#95346=AXIS2_PLACEMENT_3D ( 'NONE', #63794, #42963, #33919 ) ;
#95347=CARTESIAN_POINT ( 'NONE',  ( 180.9150213778623879, 287.7115838886965093, -14.09538787175014996 ) ) ;
#95349=AXIS2_PLACEMENT_3D ( 'NONE', #95741, #64796, #26294 ) ;
#95350=CARTESIAN_POINT ( 'NONE',  ( 201.1403430031335517, 280.2617017971787732, 16.85780947333721613 ) ) ;
#95353=CARTESIAN_POINT ( 'NONE',  ( 157.1202548728886654, 259.0885287614115668, 16.98198004443705500 ) ) ;
#95355=CARTESIAN_POINT ( 'NONE',  ( 54.00411475982191689, 211.1744531367911293, 4.594050593750047540 ) ) ;
#95357=CARTESIAN_POINT ( 'NONE',  ( 151.3589047706063582, 268.4856820897672378, 14.56544807350869419 ) ) ;
#95358=CARTESIAN_POINT ( 'NONE',  ( 95.69988983291004558, 219.3927522451418213, 10.00000000000009948 ) ) ;
#95359=CARTESIAN_POINT ( 'NONE',  ( 173.1256968621561896, 271.2508009423272028, 16.42367957618433039 ) ) ;
#95360=ORIENTED_EDGE ( 'NONE', *, *, #79346, .F. ) ;
#95364=CARTESIAN_POINT ( 'NONE',  ( 177.6299345319881411, 288.9505342943081700, 11.21071512699488792 ) ) ;
#95365=CARTESIAN_POINT ( 'NONE',  ( 189.8171280724701546, 301.8740853621098950, -0.4360232994423257624 ) ) ;
#95367=CARTESIAN_POINT ( 'NONE',  ( 172.5074440713383979, 259.9802927986077066, -13.86797602670016438 ) ) ;
#95369=CARTESIAN_POINT ( 'NONE',  ( 207.1211793645798878, 271.9025893473983047, -6.294110402770905388 ) ) ;
#95371=CARTESIAN_POINT ( 'NONE',  ( 190.0707697440390689, 301.4347651000360884, 4.271360729158901748 ) ) ;
#95373=CARTESIAN_POINT ( 'NONE',  ( 177.5204303635850067, 269.6146312835412004, 16.09809966445594753 ) ) ;
#95374=CARTESIAN_POINT ( 'NONE',  ( 164.3090168944849836, 246.0554299274959931, 2.641760039552302430 ) ) ;
#95376=CARTESIAN_POINT ( 'NONE',  ( 167.0666417749207824, 256.2416655149617100, 13.72858796342581833 ) ) ;
#95377=DIRECTION ( 'NONE',  ( -0.8660254037844387076, -0.4999999999999998890, -0.000000000000000000 ) ) ;
#95378=CARTESIAN_POINT ( 'NONE',  ( 136.0064158243085046, 240.1423013555409796, -4.594050593750043987 ) ) ;
#95380=CARTESIAN_POINT ( 'NONE',  ( 146.6834825911944620, 276.5837508513432681, 0.6716460511724984261 ) ) ;
#95385=CARTESIAN_POINT ( 'NONE',  ( 177.9758113737784413, 255.3779581033551267, 4.856556020679135166 ) ) ;
#95386=ORIENTED_EDGE ( 'NONE', *, *, #21352, .T. ) ;
#95389=CARTESIAN_POINT ( 'NONE',  ( 147.6272135932435674, 275.4487879174903355, 2.980883776998032531 ) ) ;
#95390=CARTESIAN_POINT ( 'NONE',  ( 181.9635258183570841, 260.5293054935651753, 10.24091241681038689 ) ) ;
#95391=CARTESIAN_POINT ( 'NONE',  ( 206.2016707383607184, 271.6730508100820316, 8.149847062769225658 ) ) ;
#95393=CARTESIAN_POINT ( 'NONE',  ( 185.9155157935707905, 296.7526516983074316, 4.644333911091743872 ) ) ;
#95395=CARTESIAN_POINT ( 'NONE',  ( 60.41820218054165537, 211.8149278399160664, 9.188101187500093303 ) ) ;
#95397=CARTESIAN_POINT ( 'NONE',  ( 157.4068442735347446, 281.9945091197541274, 2.874377194828706905 ) ) ;
#95399=CARTESIAN_POINT ( 'NONE',  ( 171.1029346131852549, 259.8587293126610120, 14.99369131906140140 ) ) ;
#95402=CARTESIAN_POINT ( 'NONE',  ( 203.0498946958275326, 278.9542612457532869, -15.11479947333269003 ) ) ;
#95404=CARTESIAN_POINT ( 'NONE',  ( 132.7946446283434909, 234.1427522451417644, 1.119607411625061291E-15 ) ) ;
#95408=CARTESIAN_POINT ( 'NONE',  ( 159.7633413689523536, 257.8948702361064989, -17.25380331320266336 ) ) ;
#95409=CARTESIAN_POINT ( 'NONE',  ( -10.59588092978231266, 170.8149278399160949, -9.188101187500095079 ) ) ;
#95410=CARTESIAN_POINT ( 'NONE',  ( 42.55642822748761489, 201.5024278399160949, 9.188101187500095079 ) ) ;
#95413=CARTESIAN_POINT ( 'NONE',  ( 32.50353804854218964, 201.1199935810940929, 2.679491924311251605 ) ) ;
#95414=CARTESIAN_POINT ( 'NONE',  ( 181.2581408264541949, 265.9245715698776280, -15.25451850613310434 ) ) ;
#95416=CARTESIAN_POINT ( 'NONE',  ( 147.3023124603499809, 275.5119060767245287, 5.196938859334171212 ) ) ;
#95418=CARTESIAN_POINT ( 'NONE',  ( 205.7627300303947209, 272.2554926137148072, 9.584172220806708609 ) ) ;
#95419=CARTESIAN_POINT ( 'NONE',  ( 54.05850166760819775, 212.0177522451419065, 5.000000000000046185 ) ) ;
#95421=CARTESIAN_POINT ( 'NONE',  ( 163.0929729200167912, 256.2987166179328256, -15.18292651160261642 ) ) ;
#95422=CARTESIAN_POINT ( 'NONE',  ( 157.8820657059571033, 257.1872359237914338, -17.60412210594719440 ) ) ;
#95423=CARTESIAN_POINT ( 'NONE',  ( 165.5298684834693574, 269.3554679133272884, -17.63324793928101997 ) ) ;
#95427=CARTESIAN_POINT ( 'NONE',  ( 44.26158929084472504, 186.3615022471902023, 5.000000000000051514 ) ) ;
#95428=CARTESIAN_POINT ( 'NONE',  ( 151.2701135660092007, 248.9548013555409796, -4.594050593750042211 ) ) ;
#95430=CARTESIAN_POINT ( 'NONE',  ( 3.260525530768699998, 178.8149278399161233, 9.188101187500093303 ) ) ;
#95433=CARTESIAN_POINT ( 'NONE',  ( 170.7188017663200981, 263.1837195185569271, 15.88278987561155375 ) ) ;
#95434=EDGE_CURVE ( 'NONE', #74497, #69106, #37157, .T. ) ;
#95435=CARTESIAN_POINT ( 'NONE',  ( 24.54146915528859907, 191.6427522451419350, 10.00000000000009415 ) ) ;
#95437=CARTESIAN_POINT ( 'NONE',  ( 206.4695239676918845, 273.0312896038346366, 10.41704154450801667 ) ) ;
#95443=CARTESIAN_POINT ( 'NONE',  ( 168.5369495251266017, 288.2168004222731952, 0.5299370344187100956 ) ) ;
#95446=CARTESIAN_POINT ( 'NONE',  ( 160.2868107770284780, 253.0220952814450470, 14.63377360142983896 ) ) ;
#95448=CARTESIAN_POINT ( 'NONE',  ( 152.9666954755989821, 274.9684375997553047, 10.70794663735621910 ) ) ;
#95449=CARTESIAN_POINT ( 'NONE',  ( 206.2041691044954348, 273.4908977089264113, -9.455375957961031474 ) ) ;
#95451=CARTESIAN_POINT ( 'NONE',  ( 192.5049767439991513, 297.2185948999652965, 12.57567268027295881 ) ) ;
#95452=CARTESIAN_POINT ( 'NONE',  ( 164.3706594650489023, 245.9486618633701482, -1.665857659249071698 ) ) ;
#95458=CARTESIAN_POINT ( 'NONE',  ( 155.9203642860871071, 276.9606713036284873, -10.23193020684348653 ) ) ;
#95462=CARTESIAN_POINT ( 'NONE',  ( 188.6770513902144160, 297.7343742726931168, 7.725911427269801734 ) ) ;
#95463=ORIENTED_EDGE ( 'NONE', *, *, #79064, .T. ) ;
#95466=B_SPLINE_CURVE_WITH_KNOTS ( 'NONE', 3,
 ( #80648, #49214, #26410, #88262 ),
 .UNSPECIFIED., .F., .F.,
 ( 4, 4 ),
 ( 2.151919402719074343E-15, 0.001406589747191096295 ),
 .UNSPECIFIED. ) ;
#95469=CARTESIAN_POINT ( 'NONE',  ( 173.8153613617645590, 267.2422669803751205, 17.07281103384172383 ) ) ;
#95470=CARTESIAN_POINT ( 'NONE',  ( 164.8849641302980444, 245.0578600525887794, 2.884140591399200648 ) ) ;
#95473=CARTESIAN_POINT ( 'NONE',  ( 170.9300592470816014, 255.0224789877633214, -11.37166744830014586 ) ) ;
#95474=CARTESIAN_POINT ( 'NONE',  ( 163.4004183463084416, 247.6291687766210146, 10.19167732382099345 ) ) ;
#95475=ORIENTED_EDGE ( 'NONE', *, *, #95662, .F. ) ;
#95477=CARTESIAN_POINT ( 'NONE',  ( 158.0824493049356363, 267.3773279949191988, -16.20755095283232450 ) ) ;
#95478=ORIENTED_EDGE ( 'NONE', *, *, #13111, .F. ) ;
#95479=CARTESIAN_POINT ( 'NONE',  ( 160.6762863198379421, 270.7031352422249597, 15.85774362266417015 ) ) ;
#95482=CARTESIAN_POINT ( 'NONE',  ( 147.4174248404692094, 275.3125255857779052, 7.386196481672387293 ) ) ;
#95483=CARTESIAN_POINT ( 'NONE',  ( 180.0945261039350953, 290.8209287807282521, -9.536000357058787458 ) ) ;
#95484=CARTESIAN_POINT ( 'NONE',  ( 194.6820509838467785, 270.8910309865917156, -14.27696746312268239 ) ) ;
#95485=CARTESIAN_POINT ( 'NONE',  ( 192.1640094933931096, 297.8091675017319062, 12.36911124822534447 ) ) ;
#95487=CARTESIAN_POINT ( 'NONE',  ( 174.7134278764181659, 289.9860957709516924, 6.278215837728235549 ) ) ;
#95488=CARTESIAN_POINT ( 'NONE',  ( 158.3414723807261169, 256.3915202217551723, -16.63524069124627758 ) ) ;
#95493=CARTESIAN_POINT ( 'NONE',  ( 164.2545401858843945, 246.1497863546213978, 2.275217130759496609 ) ) ;
#95494=CARTESIAN_POINT ( 'NONE',  ( 206.1932826529868805, 273.5097535960530877, 11.72208607728249241 ) ) ;
#95495=CARTESIAN_POINT ( 'NONE',  ( 198.3075590527773784, 287.1682275260610027, 16.94807365630277118 ) ) ;
#95496=EDGE_LOOP ( 'NONE', ( #13926, #21046, #74750 ) ) ;
#95498=CARTESIAN_POINT ( 'NONE',  ( 190.3379505298266849, 300.9719944042457200, 6.192102975663287268 ) ) ;
#95504=CARTESIAN_POINT ( 'NONE',  ( 200.2690241097007799, 283.7708703901988656, 16.96680019208369927 ) ) ;
#95505=CARTESIAN_POINT ( 'NONE',  ( 190.9055496984007902, 261.7574849729193716, -0.1787456162138263693 ) ) ;
#95508=CARTESIAN_POINT ( 'NONE',  ( 161.2535912560966551, 263.0844709175967182, -17.80682751047658030 ) ) ;
#95510=CARTESIAN_POINT ( 'NONE',  ( 207.4826643481121664, 271.2764789897469768, 7.783310782367018454 ) ) ;
#95512=CARTESIAN_POINT ( 'NONE',  ( 22.44857442947622417, 183.7677522451418497, 10.00000000000009592 ) ) ;
#95513=CARTESIAN_POINT ( 'NONE',  ( 92.21748570181026139, 233.2369531367911009, -4.594050593750048428 ) ) ;
#95515=CARTESIAN_POINT ( 'NONE',  ( 92.09145065047479761, 230.6427522451419065, 10.00000000000009415 ) ) ;
#95516=CARTESIAN_POINT ( 'NONE',  ( 207.5573902749007971, 271.1470498879065190, 2.528158314636208548 ) ) ;
#95517=CARTESIAN_POINT ( 'NONE',  ( 20.58103360645747770, 188.8149278399161233, -9.188101187500095079 ) ) ;
#95519=CARTESIAN_POINT ( 'NONE',  ( 200.6449165581618956, 283.1198055712825976, 18.35107460171532523 ) ) ;
#95520=ORIENTED_EDGE ( 'NONE', *, *, #76421, .T. ) ;
#95522=CARTESIAN_POINT ( 'NONE',  ( 147.7487458879263897, 276.5474634960659728, -0.9591148040551028542 ) ) ;
#95523=( BOUNDED_CURVE ( )  B_SPLINE_CURVE ( 2, ( #837, #70232, #40321, #87011, #31718, #46423, #77348, #48447, #62622 ),
 .UNSPECIFIED., .F., .T. ) 
 B_SPLINE_CURVE_WITH_KNOTS ( ( 3, 2, 2, 2, 3 ),
 ( 0.3911290322580645018, 0.3924731182795698770, 0.3951612903225806273, 0.3978494623655913776, 0.3991935483870967527 ),
 .UNSPECIFIED. ) 
 CURVE ( )  GEOMETRIC_REPRESENTATION_ITEM ( )  RATIONAL_B_SPLINE_CURVE ( ( 0.9330127018922194093, 0.9330127018922194093, 1.000000000000000000, 0.8660254037844387076, 1.000000000000000000, 0.8660254037844387076, 1.000000000000000000, 0.9330127018922194093, 0.9330127018922194093 ) ) 
 REPRESENTATION_ITEM ( '' )  );
#95526=CARTESIAN_POINT ( 'NONE',  ( 193.6173108488650882, 262.6670938961573825, -4.018541380834022014 ) ) ;
#95527=CARTESIAN_POINT ( 'NONE',  ( 207.8996209429610360, 270.5542889829179103, -5.987818313449536411 ) ) ;
#95528=CARTESIAN_POINT ( 'NONE',  ( 185.8808357693771427, 286.5678490806189984, 15.69086117514267897 ) ) ;
#95529=CARTESIAN_POINT ( 'NONE',  ( 167.7347975179296498, 251.7814102707968118, 10.38933443070461138 ) ) ;
#95530=CARTESIAN_POINT ( 'NONE',  ( 41.01373370305532973, 203.6744531367911293, 4.594050593750047540 ) ) ;
#95531=CARTESIAN_POINT ( 'NONE',  ( 78.37938175722116796, 229.3927522451419350, 2.944929066748280225E-16 ) ) ;
#95533=CARTESIAN_POINT ( 'NONE',  ( 180.9257151590790897, 260.3651392059021532, -10.38670931792631968 ) ) ;
#95534=CARTESIAN_POINT ( 'NONE',  ( 7.212287079182728711, 162.7202760586659736, -5.415160957724236172E-17 ) ) ;
#95536=CARTESIAN_POINT ( 'NONE',  ( 199.0756812798354645, 285.8378008023734083, -18.45377816087746936 ) ) ;
#95537=CARTESIAN_POINT ( 'NONE',  ( 186.4273393382061386, 282.8874102186402411, 16.17533557276407308 ) ) ;
#95538=CARTESIAN_POINT ( 'NONE',  ( 147.2567621633200474, 275.5908015054806128, -3.647191014543873955 ) ) ;
#95539=B_SPLINE_CURVE_WITH_KNOTS ( 'NONE', 3,
 ( #78370, #24153, #85502, #9461, #86019, #70242, #17043, #39818, #16050, #46951, #63147, #16545, #77868, #94093, #79895, #86512, #64151, #56546, #8951, #56026, #47934, #8453, #70750, #39325, #78875, #40331, #71271, #87533, #9966, #847, #1861, #32745, #63649, #31727, #62629, #25142, #87020, #17551, #48458, #79400, #40827, #2372, #18064, #33250, #95102, #25666, #48961, #10460 ),
 .UNSPECIFIED., .F., .F.,
 ( 4, 2, 2, 2, 2, 2, 2, 2, 2, 2, 2, 2, 2, 2, 2, 2, 2, 2, 2, 2, 2, 2, 2, 4 ),
 ( 0.003452227750546106588, 0.003635194737864935396, 0.003726678231524355872, 0.003818161725183775914, 0.003909645218843195956, 0.004001128712502616432, 0.004184095699821572742, 0.004550029674459376075, 0.004915963649097178541, 0.005647831598372718420, 0.006379699547648259167, 0.007843435446199253924, 0.008026402433518126101, 0.008117885927177600353, 0.008163627674007377377, 0.008209369420837152667, 0.008232240294252041179, 0.008255111167666931427, 0.008300852914496736207, 0.008392336408156418626, 0.008575303395475786933, 0.008758270382795155240, 0.008941237370114523547, 0.009307171344753268835 ),
 .UNSPECIFIED. ) ;
#95540=CARTESIAN_POINT ( 'NONE',  ( 156.6812872898450735, 261.2670451491295012, 0.000000000000000000 ) ) ;
#95541=CARTESIAN_POINT ( 'NONE',  ( 204.8523313866422484, 275.8323493198358847, 14.65426965484541100 ) ) ;
#95542=CARTESIAN_POINT ( 'NONE',  ( 191.4082244002820516, 299.1182256826033949, -8.271837126846561361 ) ) ;
#95543=CARTESIAN_POINT ( 'NONE',  ( 164.6460902696047128, 245.4716017159096566, -3.036414139157908476 ) ) ;
#95545=CARTESIAN_POINT ( 'NONE',  ( 0.09429369783835704621, 160.8615022471902023, 5.000000000000051514 ) ) ;
#95546=CARTESIAN_POINT ( 'NONE',  ( 161.3754592430677235, 251.5660820581029782, -13.21728889732328582 ) ) ;
#95547=CARTESIAN_POINT ( 'NONE',  ( 117.9006383567337792, 245.0024278399160949, 9.188101187500095079 ) ) ;
#95556=CARTESIAN_POINT ( 'NONE',  ( 190.8353200730629737, 300.1105250852234008, -7.980428465987968067 ) ) ;
#95557=ORIENTED_EDGE ( 'NONE', *, *, #56772, .T. ) ;
#95558=CARTESIAN_POINT ( 'NONE',  ( 192.7873893855839071, 263.7602658877742670, -4.354176413973807058 ) ) ;
#95559=CARTESIAN_POINT ( 'NONE',  ( 149.6564118588553924, 271.4344863124460971, -11.76165597393390172 ) ) ;
#95564=CARTESIAN_POINT ( 'NONE',  ( 189.1046751719556482, 265.6539275885750158, 10.79115261866721198 ) ) ;
#95565=CARTESIAN_POINT ( 'NONE',  ( 193.1884577481565373, 273.3595093090821706, -16.04199635000458457 ) ) ;
#95566=CARTESIAN_POINT ( 'NONE',  ( 168.7265333031080843, 271.8518808229929959, -17.19668397201396814 ) ) ;
#95568=CARTESIAN_POINT ( 'NONE',  ( 200.1392393678551684, 272.4654854410964617, 12.57020546295501440 ) ) ;
#95572=CARTESIAN_POINT ( 'NONE',  ( 192.5049767439991513, 297.2185948999652965, 12.57567268027295881 ) ) ;
#95574=CARTESIAN_POINT ( 'NONE',  ( 159.6023402823087451, 258.6676503891110883, 17.43025742997651761 ) ) ;
#95576=CARTESIAN_POINT ( 'NONE',  ( 173.9832671538335660, 272.2600618968111235, -16.61040946315311473 ) ) ;
#95578=CARTESIAN_POINT ( 'NONE',  ( 167.2512865494106222, 280.7487606393313513, 11.65990675234894169 ) ) ;
#95579=CARTESIAN_POINT ( 'NONE',  ( 194.9636675848471441, 292.9600174435121289, -15.57898232594655319 ) ) ;
#95580=CARTESIAN_POINT ( 'NONE',  ( 164.8961913205752694, 246.0452500519421619, -1.096323744997464322 ) ) ;
#95582=DIRECTION ( 'NONE',  ( -0.8660254037844387076, -0.4999999999999998890, -0.000000000000000000 ) ) ;
#95583=CARTESIAN_POINT ( 'NONE',  ( 186.3725304700115544, 291.5966866658558843, 12.20655306884721369 ) ) ;
#95585=CARTESIAN_POINT ( 'NONE',  ( 191.2056514706806070, 299.4690922889112699, 7.290007621276087590 ) ) ;
#95588=CARTESIAN_POINT ( 'NONE',  ( 203.4357368910538355, 278.2859629599173559, -16.45855118664066197 ) ) ;
#95591=CARTESIAN_POINT ( 'NONE',  ( 178.1614477613976817, 260.9598035071301751, 12.21005518007415702 ) ) ;
#95593=CARTESIAN_POINT ( 'NONE',  ( 192.9863438995966760, 294.0432375156728995, 14.14043846130007331 ) ) ;
#95595=CARTESIAN_POINT ( 'NONE',  ( -22.42236680055709641, 157.8615022471902591, 0.000000000000000000 ) ) ;
#95596=CARTESIAN_POINT ( 'NONE',  ( 149.0237174825091415, 274.5263358477994871, 9.114370506038131481 ) ) ;
#95599=CARTESIAN_POINT ( 'NONE',  ( 160.2740869459746023, 254.0686150970925610, -15.36085255641610914 ) ) ;
#95600=CARTESIAN_POINT ( 'NONE',  ( 159.2487512388012476, 275.3823027008313034, -12.53260474664770463 ) ) ;
#95601=CARTESIAN_POINT ( 'NONE',  ( 146.8574506849497538, 276.2824292740633041, -4.888313306692038118 ) ) ;
#95602=FACE_OUTER_BOUND ( 'NONE', #53743, .T. ) ;
#95604=CARTESIAN_POINT ( 'NONE',  ( 157.9689631420808951, 280.9937072662406194, 2.205630096026304887 ) ) ;
#95605=CARTESIAN_POINT ( 'NONE',  ( 144.0982539169780523, 247.8768266524160140, 9.188101187500098632 ) ) ;
#95610=ORIENTED_EDGE ( 'NONE', *, *, #37502, .T. ) ;
#95612=CARTESIAN_POINT ( 'NONE',  ( 163.0683798854284703, 248.2042762609320903, 11.26611642476872710 ) ) ;
#95616=CARTESIAN_POINT ( 'NONE',  ( 153.3480993750124810, 276.8750838587924363, 7.125264275211442566 ) ) ;
#95617=CARTESIAN_POINT ( 'NONE',  ( 153.1983976505312626, 265.2995869615763809, -17.69657798691567763 ) ) ;
#95619=CARTESIAN_POINT ( 'NONE',  ( 171.6965468371157897, 280.0430691848860647, 13.87941070326743720 ) ) ;
#95626=CARTESIAN_POINT ( 'NONE',  ( 164.0769311498514753, 278.1829446335003126, 13.34093408993252439 ) ) ;
#95628=CARTESIAN_POINT ( 'NONE',  ( 201.0920123907623065, 267.8787980814687444, -2.846255320721498006 ) ) ;
#95629=CARTESIAN_POINT ( 'NONE',  ( 152.1077061761917832, 267.1887200105145439, -15.41283704233756247 ) ) ;
#95630=CARTESIAN_POINT ( 'NONE',  ( 190.0550686570564949, 301.4619601804237732, 4.203010638620038542 ) ) ;
#95631=CARTESIAN_POINT ( 'NONE',  ( 202.2603678735342214, 280.3217618159037556, 16.49712126737133744 ) ) ;
#95633=CARTESIAN_POINT ( 'NONE',  ( 154.1310696087535632, 276.6461666010558247, -8.687488248752188724 ) ) ;
#95634=CARTESIAN_POINT ( 'NONE',  ( 67.18526205639879834, 198.0494855054051868, -2.679491924311248496 ) ) ;
#95637=CARTESIAN_POINT ( 'NONE',  ( 193.2657730933340474, 276.0652844845805021, -16.22139663033825130 ) ) ;
#95645=CARTESIAN_POINT ( 'NONE',  ( -7.835251407336910390, 166.2833772461660828, -9.188101187500095079 ) ) ;
#95646=CARTESIAN_POINT ( 'NONE',  ( 82.25819355828922141, 227.4869531367911293, 4.594050593750046652 ) ) ;
#95647=CARTESIAN_POINT ( 'NONE',  ( 203.2187760522547819, 278.6617501559703101, -15.08675642319914978 ) ) ;
#95649=CARTESIAN_POINT ( 'NONE',  ( 184.1217943198085152, 275.8755882355715130, -17.79325935397197256 ) ) ;
#95650=B_SPLINE_CURVE_WITH_KNOTS ( 'NONE', 3,
 ( #45827, #76750, #61034, #92007, #7344, #22554, #99075, #29658, #61541, #76276 ),
 .UNSPECIFIED., .F., .F.,
 ( 4, 2, 2, 2, 4 ),
 ( 0.000000000000000000, 0.0004052285844863903752, 0.0008104571689727807504, 0.001215685753459171126, 0.001620914337945561501 ),
 .UNSPECIFIED. ) ;
#95651=CARTESIAN_POINT ( 'NONE',  ( 138.6787122315880367, 239.3262482093457493, 3.021315404115420679E-15 ) ) ;
#95653=CARTESIAN_POINT ( 'NONE',  ( 160.6263868137985753, 282.0864858795503096, 5.113129440300967943 ) ) ;
#95656=CARTESIAN_POINT ( 'NONE',  ( 178.0629634300817941, 289.8938732657310879, 9.603314252689274966 ) ) ;
#95662=EDGE_CURVE ( 'NONE', #25397, #98060, #98932, .T. ) ;
#95663=CARTESIAN_POINT ( 'NONE',  ( 56.08842225738448661, 197.0643266524160140, 9.188101187500095079 ) ) ;
#95665=CARTESIAN_POINT ( 'NONE',  ( 76.87303194821100760, 209.0643266524160424, 9.188101187500095079 ) ) ;
#95666=CARTESIAN_POINT ( 'NONE',  ( 161.8882824960653579, 250.2482648971885340, -13.83574485983625557 ) ) ;
#95668=CARTESIAN_POINT ( 'NONE',  ( 163.4612457243555923, 257.9110273980033980, 15.57507432676986703 ) ) ;
#95671=CARTESIAN_POINT ( 'NONE',  ( 174.6996461476103661, 269.1010435442095172, -16.34783327481654780 ) ) ;
#95676=ORIENTED_EDGE ( 'NONE', *, *, #72281, .T. ) ;
#95678=CARTESIAN_POINT ( 'NONE',  ( 76.62902843369037953, 224.2369531367911293, -4.594050593750048428 ) ) ;
#95680=CARTESIAN_POINT ( 'NONE',  ( 169.1474947851822321, 288.3004841199922339, -1.112798234388539198 ) ) ;
#95681=CARTESIAN_POINT ( 'NONE',  ( 192.5551423381268989, 297.1317055421444024, -13.20528585388119858 ) ) ;
#95684=EDGE_CURVE ( 'NONE', #3083, #11960, #75975, .T. ) ;
#95687=CARTESIAN_POINT ( 'NONE',  ( 189.8780818209742733, 286.5329341612866756, 16.47277920618313729 ) ) ;
#95689=CARTESIAN_POINT ( 'NONE',  ( 122.2038756314442054, 231.3615022471901739, 5.000000000000051514 ) ) ;
#95690=CARTESIAN_POINT ( 'NONE',  ( 205.2414727015710412, 275.1583367910551488, -12.71338796362297963 ) ) ;
#95693=CARTESIAN_POINT ( 'NONE',  ( 165.5692510255798027, 246.8512466342675395, -1.587510859644124750 ) ) ;
#95694=ORIENTED_EDGE ( 'NONE', *, *, #64382, .F. ) ;
#95695=CARTESIAN_POINT ( 'NONE',  ( 202.3421728196210552, 280.1800714929709670, 16.85915999540957344 ) ) ;
#95696=CARTESIAN_POINT ( 'NONE',  ( 207.4143922525829566, 270.9009812163183142, -1.235003168413449703 ) ) ;
#95698=ORIENTED_EDGE ( 'NONE', *, *, #20105, .F. ) ;
#95700=ORIENTED_EDGE ( 'NONE', *, *, #15710, .T. ) ;
#95702=CARTESIAN_POINT ( 'NONE',  ( 170.6386111665514989, 250.4289151046095299, 3.370994400240735711 ) ) ;
#95709=CYLINDRICAL_SURFACE ( 'NONE', #80514, 17.82106496071139645 ) ;
#95713=CARTESIAN_POINT ( 'NONE',  ( 198.2524512863544430, 286.8805590551967839, 16.95567094640148298 ) ) ;
#95714=CARTESIAN_POINT ( 'NONE',  ( 164.2059258710715994, 246.2339888178522926, 7.329631442356459914 ) ) ;
#95715=CARTESIAN_POINT ( 'NONE',  ( 194.5252985417586729, 293.7192948986070178, -14.54632727629426370 ) ) ;
#95717=CARTESIAN_POINT ( 'NONE',  ( 155.4812142336614329, 261.3456326552338282, 18.45193178807985745 ) ) ;
#95718=CARTESIAN_POINT ( 'NONE',  ( 147.7136411429809186, 276.4209930201117231, 0.9264851003149958686 ) ) ;
#95719=CARTESIAN_POINT ( 'NONE',  ( 205.0994677818405023, 275.4042965269534307, -14.14519517703424789 ) ) ;
#95720=CARTESIAN_POINT ( 'NONE',  ( 163.9711092878513341, 246.6407030704495185, 4.892543501721282162 ) ) ;
#95721=CARTESIAN_POINT ( 'NONE',  ( 166.1339902640533523, 265.4989097315049094, 16.56817675206516682 ) ) ;
#95723=CARTESIAN_POINT ( 'NONE',  ( 91.86592320334659689, 223.8458772461660544, 9.188101187500095079 ) ) ;
#95726=CARTESIAN_POINT ( 'NONE',  ( 119.0307608796806278, 227.9824982072973683, 3.021315404115420679E-15 ) ) ;
#95727=ORIENTED_EDGE ( 'NONE', *, *, #16674, .T. ) ;
#95730=CARTESIAN_POINT ( 'NONE',  ( 177.2071603091147836, 292.4572209928213624, -2.700943100067172420 ) ) ;
#95731=DIRECTION ( 'NONE',  ( 0.8660254037844395958, 0.4999999999999985567, 0.000000000000000000 ) ) ;
#95732=CARTESIAN_POINT ( 'NONE',  ( 206.1615484827472358, 273.5647187912443314, -9.556459874778100883 ) ) ;
#95733=CARTESIAN_POINT ( 'NONE',  ( 206.8716470161501491, 270.6909265943963874, -4.951756624771148196 ) ) ;
#95734=CARTESIAN_POINT ( 'NONE',  ( 95.92559083146868204, 220.0643266524159856, -9.188101187500093303 ) ) ;
#95735=VERTEX_POINT ( 'NONE', #6138 ) ;
#95736=ORIENTED_EDGE ( 'NONE', *, *, #46394, .T. ) ;
#95737=CARTESIAN_POINT ( 'NONE',  ( 207.6163508138795635, 271.0449272387537576, -1.385071889578343152 ) ) ;
#95739=EDGE_CURVE ( 'NONE', #4581, #82473, #43269, .T. ) ;
#95741=CARTESIAN_POINT ( 'NONE',  ( -22.42236680055709641, 157.8615022471902591, 0.000000000000000000 ) ) ;
#95742=CARTESIAN_POINT ( 'NONE',  ( 143.4758849319492526, 244.4548013555409796, -4.594050593750042211 ) ) ;
#95744=CARTESIAN_POINT ( 'NONE',  ( -3.027006198515987734, 162.3927522451418213, 10.00000000000009592 ) ) ;
#95746=ORIENTED_EDGE ( 'NONE', *, *, #91626, .F. ) ;
#95751=CARTESIAN_POINT ( 'NONE',  ( 175.8027662909930484, 284.8719843250962072, 14.11304877541382119 ) ) ;
#95753=B_SPLINE_CURVE_WITH_KNOTS ( 'NONE', 3,
 ( #60896, #58899, #89868, #31500 ),
 .UNSPECIFIED., .F., .F.,
 ( 4, 4 ),
 ( 0.004047834017227748896, 0.01202942932177893109 ),
 .UNSPECIFIED. ) ;
#95755=ADVANCED_FACE ( 'NONE', ( #51756 ), #60811, .T. ) ;
#95756=DIRECTION ( 'NONE',  ( 0.5000000000000048850, -0.8660254037844358210, 0.000000000000000000 ) ) ;
#95757=CARTESIAN_POINT ( 'NONE',  ( 7.888522331898304429, 165.3615022471902023, 5.000000000000051514 ) ) ;
#95758=CARTESIAN_POINT ( 'NONE',  ( 161.0952649348064938, 251.6218116045831437, 13.81854265722852482 ) ) ;
#95760=CARTESIAN_POINT ( 'NONE',  ( 167.7650414173376134, 249.6746511289063335, 7.938333554227506639 ) ) ;
#95762=CARTESIAN_POINT ( 'NONE',  ( 175.8212761817833893, 290.2801695444399002, -6.226935068522726269 ) ) ;
#95764=B_SPLINE_CURVE_WITH_KNOTS ( 'NONE', 3,
 ( #10465, #8956, #33256, #70755 ),
 .UNSPECIFIED., .F., .F.,
 ( 4, 4 ),
 ( 0.000000000000000000, 0.0008757035534864545051 ),
 .UNSPECIFIED. ) ;
#95766=CARTESIAN_POINT ( 'NONE',  ( 185.3869297780163095, 266.3934770207134193, 13.10756805561828742 ) ) ;
#95770=( LENGTH_UNIT ( ) NAMED_UNIT ( * ) SI_UNIT ( .MILLI., .METRE. ) );
#95771=CARTESIAN_POINT ( 'NONE',  ( 157.7295765003705696, 271.0796008204293912, -14.71699761758586256 ) ) ;
#95775=CARTESIAN_POINT ( 'NONE',  ( 12.78715206816254302, 172.0643266524160140, -9.188101187500093303 ) ) ;
#95780=ADVANCED_FACE ( 'NONE', ( #30932 ), #83684, .T. ) ;
#95781=CYLINDRICAL_SURFACE ( 'NONE', #69341, 10.00000000000010658 ) ;
#95783=CARTESIAN_POINT ( 'NONE',  ( 36.95476026646328194, 182.9548013555409796, -4.594050593750042211 ) ) ;
#95785=CARTESIAN_POINT ( 'NONE',  ( 147.5498377207569263, 275.0831797495432056, 4.097967709737811326 ) ) ;
#95787=CARTESIAN_POINT ( 'NONE',  ( 11.37297787527554327, 165.8262482093457777, 3.021315404115420679E-15 ) ) ;
#95788=CARTESIAN_POINT ( 'NONE',  ( 147.1731211915891322, 275.7356719181125868, 0.5879280619134324981 ) ) ;
#95789=CARTESIAN_POINT ( 'NONE',  ( 182.1788207689431829, 279.9818748238459420, -16.09985332685275594 ) ) ;
#95791=EDGE_CURVE ( 'NONE', #80984, #83021, #66453, .T. ) ;
#95792=CARTESIAN_POINT ( 'NONE',  ( 166.6772716030373260, 257.8718083500641001, -15.18422749061457466 ) ) ;
#95794=CARTESIAN_POINT ( 'NONE',  ( 83.66574516303663245, 229.1115022471903160, -5.000000000000047962 ) ) ;
#95795=CARTESIAN_POINT ( 'NONE',  ( 92.83118068642198750, 217.7365022471902023, -10.00000000000009059 ) ) ;
#95799=CARTESIAN_POINT ( 'NONE',  ( 43.63930707798317599, 189.8768266524159856, -9.188101187500091527 ) ) ;
#95803=CARTESIAN_POINT ( 'NONE',  ( 198.4427928769277969, 286.9339956717308837, -17.97122743692687763 ) ) ;
#95806=CARTESIAN_POINT ( 'NONE',  ( 171.2443217382905800, 286.5344483683264798, 7.485321208534859494 ) ) ;
#95807=CARTESIAN_POINT ( 'NONE',  ( 164.2578067403839555, 246.1441285162624126, -2.322300236470859591 ) ) ;
#95808=CARTESIAN_POINT ( 'NONE',  ( 193.3873874904946035, 295.6902146538902230, 13.58053800763477703 ) ) ;
#95811=CARTESIAN_POINT ( 'NONE',  ( 163.0171530587457767, 248.2930037274571191, 9.677214176418313940 ) ) ;
#95812=CARTESIAN_POINT ( 'NONE',  ( 197.0313051377892748, 289.3787641501790517, -17.15509075150697882 ) ) ;
#95813=CARTESIAN_POINT ( 'NONE',  ( 174.9413478015634098, 257.3571669544361384, 11.48782993742858771 ) ) ;
#95818=LINE ( 'NONE', #56249, #1977 ) ;
#95819=VERTEX_POINT ( 'NONE', #79074 ) ;
#95821=CARTESIAN_POINT ( 'NONE',  ( 167.0487131668929806, 261.4106595961994230, 16.87154839675361018 ) ) ;
#95824=ORIENTED_EDGE ( 'NONE', *, *, #63745, .F. ) ;
#95825=EDGE_LOOP ( 'NONE', ( #64879, #80299, #66522, #30108 ) ) ;
#95826=CARTESIAN_POINT ( 'NONE',  ( 207.1285138014047504, 271.8898857301724661, -5.752177443817618752 ) ) ;
#95828=CARTESIAN_POINT ( 'NONE',  ( 149.3253462891332219, 272.0079086998416074, -12.99539319630191336 ) ) ;
#95834=EDGE_CURVE ( 'NONE', #74117, #33600, #4320, .T. ) ;
#95835=CARTESIAN_POINT ( 'NONE',  ( 163.4341025207368716, 282.8476932499685859, 9.116081536633066307 ) ) ;
#95836=CARTESIAN_POINT ( 'NONE',  ( 109.2403843188893831, 240.0024278399160949, -9.188101187500093303 ) ) ;
#95839=CARTESIAN_POINT ( 'NONE',  ( 207.9622466093905189, 270.4458181468041289, 3.586592550214158681 ) ) ;
#95842=CARTESIAN_POINT ( 'NONE',  ( 159.8655504377736918, 253.7517395922482706, 15.51368179719542262 ) ) ;
#95844=CARTESIAN_POINT ( 'NONE',  ( 63.61184440487929947, 207.5333772461660544, 9.188101187500095079 ) ) ;
#95846=CARTESIAN_POINT ( 'NONE',  ( 191.5281967176683509, 298.9104275333885994, 7.715154960566919407 ) ) ;
#95851=CARTESIAN_POINT ( 'NONE',  ( 168.3557124657904467, 273.6222795104500278, 17.14480014634877136 ) ) ;
#95854=CARTESIAN_POINT ( 'NONE',  ( 173.8768829991239500, 278.0004084252144594, -16.03808046269689314 ) ) ;
#95855=CARTESIAN_POINT ( 'NONE',  ( 161.8153478334749877, 250.3745914384277285, -14.21120979595050215 ) ) ;
#95856=CARTESIAN_POINT ( 'NONE',  ( 146.8574506849497538, 276.2824292740633041, -4.888313306692038118 ) ) ;
#95858=CARTESIAN_POINT ( 'NONE',  ( 190.2935937139882299, 301.0488226629397559, 4.649863831023156813 ) ) ;
#95859=CARTESIAN_POINT ( 'NONE',  ( 36.90037335867696555, 192.1115022471902591, 10.00000000000009592 ) ) ;
#95860=CARTESIAN_POINT ( 'NONE',  ( 165.0565241268390366, 244.7607094220335568, 2.191926263411719589 ) ) ;
#95862=CARTESIAN_POINT ( 'NONE',  ( 164.3199246584869115, 254.2670161280514094, 14.21696250712841270 ) ) ;
#95863=CARTESIAN_POINT ( 'NONE',  ( 207.9622466093905189, 270.4458181468041289, 3.586592550214158681 ) ) ;
#95864=CARTESIAN_POINT ( 'NONE',  ( 117.0346129529493311, 244.5024278399160949, -9.188101187500093303 ) ) ;
#95865=ORIENTED_EDGE ( 'NONE', *, *, #59647, .T. ) ;
#95868=CARTESIAN_POINT ( 'NONE',  ( 155.4810912439522212, 261.3458456796594760, -18.44218279064527266 ) ) ;
#95870=CARTESIAN_POINT ( 'NONE',  ( 204.9432097630379417, 275.6749433546094679, 13.74700047688257776 ) ) ;
#95871=EDGE_CURVE ( 'NONE', #68457, #44895, #57278, .T. ) ;
#95872=CARTESIAN_POINT ( 'NONE',  ( -4.668846022976095966, 168.1115022471902591, 10.00000000000009592 ) ) ;
#95873=CARTESIAN_POINT ( 'NONE',  ( 175.8939073520130592, 252.7054158260212375, 5.280091837693253964 ) ) ;
#95874=ORIENTED_EDGE ( 'NONE', *, *, #62989, .T. ) ;
#95876=CARTESIAN_POINT ( 'NONE',  ( 155.1825101010379910, 273.4369430123585403, -12.92776615095295156 ) ) ;
#95877=CARTESIAN_POINT ( 'NONE',  ( 147.6472966492084140, 275.3178831392595498, 3.373654813989544365 ) ) ;
#95878=CARTESIAN_POINT ( 'NONE',  ( 184.9620068429786386, 260.8549389384861570, 10.28307718128925607 ) ) ;
#95879=CARTESIAN_POINT ( 'NONE',  ( 206.1142978005191821, 273.6465593735555899, -11.17423994621995753 ) ) ;
#95880=CARTESIAN_POINT ( 'NONE',  ( 138.9021014942714487, 244.8768266524160140, 9.188101187500096856 ) ) ;
#95883=CARTESIAN_POINT ( 'NONE',  ( 72.89481452351749624, 203.7048013555409796, 4.594050593750051981 ) ) ;
#95884=CIRCLE ( 'NONE', #52137, 17.82106496071138224 ) ;
#95885=CARTESIAN_POINT ( 'NONE',  ( 174.6446264865013802, 251.8031208292603083, 3.583545318800930080 ) ) ;
#95888=CARTESIAN_POINT ( 'NONE',  ( 190.6893905452545823, 300.3632824417117604, 3.294993852933539191 ) ) ;
#95890=CARTESIAN_POINT ( 'NONE',  ( 172.6334465443935358, 287.8136291912904312, -8.329514407067593496 ) ) ;
#95891=CARTESIAN_POINT ( 'NONE',  ( -22.42236680055709641, 157.8615022471902591, 0.000000000000000000 ) ) ;
#95892=CARTESIAN_POINT ( 'NONE',  ( 193.7773542058511680, 288.6392134509156335, 16.07539256311286024 ) ) ;
#95894=CARTESIAN_POINT ( 'NONE',  ( 110.7831656154889259, 244.7677522451419065, -5.000000000000047962 ) ) ;
#95896=ORIENTED_EDGE ( 'NONE', *, *, #28920, .F. ) ;
#95897=B_SPLINE_CURVE_WITH_KNOTS ( 'NONE', 3,
 ( #58797, #4118, #81662, #43610, #56820, #65913, #89289, #19837, #35520, #49238, #80173, #75527, #83149, #6619, #99822, #91246, #53688, #28409, #29418, #53209, #13717, #84645, #44592, #6112, #37984, #67917, #90267, #21810, #52695, #37493, #14215, #5615, #30406, #67410, #68896, #37007, #36006, #60287, #61298, #83657, #68401, #99328, #51732, #29908, #91744, #84162, #15186, #74548, #5126, #20840 ),
 .UNSPECIFIED., .F., .F.,
 ( 4, 2, 2, 2, 2, 2, 2, 2, 2, 2, 2, 2, 2, 2, 2, 2, 2, 2, 2, 2, 2, 2, 2, 2, 4 ),
 ( 0.001855169425541140348, 0.002306674773933914662, 0.002532427448130358198, 0.002758180122326801299, 0.002871056459425064267, 0.002983932796523326800, 0.003096809133621589334, 0.003209685470719852302, 0.003435438144916219943, 0.003661190819112586717, 0.004112696167505321132, 0.004564201515898056415, 0.005467212212683564276, 0.006370222909469071271, 0.006821728257861788339, 0.007273233606254505407, 0.007386109943352781385, 0.007442548111901956670, 0.007498986280451131956, 0.007611862617549461710, 0.007724738954647791464, 0.008176244303041004663, 0.008627749651434217862, 0.008853502325630750736, 0.009079254999827283609 ),
 .UNSPECIFIED. ) ;
#95899=CARTESIAN_POINT ( 'NONE',  ( 196.4994169513186364, 290.3000215130921902, 16.82935102260526961 ) ) ;
#95901=CARTESIAN_POINT ( 'NONE',  ( -3.126064726376516667, 162.8768266524159856, -9.188101187500093303 ) ) ;
#95902=CARTESIAN_POINT ( 'NONE',  ( 41.36599039304901737, 188.5643266524159571, -9.188101187500093303 ) ) ;
#95903=FACE_OUTER_BOUND ( 'NONE', #82223, .T. ) ;
#95906=CARTESIAN_POINT ( 'NONE',  ( 204.7764732025852084, 275.9637395487929439, -14.02287343454361412 ) ) ;
#95908=CARTESIAN_POINT ( 'NONE',  ( 190.4240181651484818, 300.8229208869809668, -4.214281362166949485 ) ) ;
#95910=CARTESIAN_POINT ( 'NONE',  ( 67.84273934451060484, 196.6427522451417644, 1.119607411625061291E-15 ) ) ;
#95911=CARTESIAN_POINT ( 'NONE',  ( 179.4717503424750191, 254.9888846402135698, -4.048912934998680768 ) ) ;
#95912=CARTESIAN_POINT ( 'NONE',  ( 205.4103625296683617, 274.8658110279089897, -13.38953657917851814 ) ) ;
#95914=CARTESIAN_POINT ( 'NONE',  ( 40.86965645935558911, 207.7365022471903444, 2.944929066748280225E-16 ) ) ;
#95916=CARTESIAN_POINT ( 'NONE',  ( 202.8167949821795446, 279.3580017930215149, 15.61966256214195070 ) ) ;
#95917=CARTESIAN_POINT ( 'NONE',  ( 7.590652549690899420, 181.3149278399161233, -9.188101187500095079 ) ) ;
#95919=CARTESIAN_POINT ( 'NONE',  ( 164.2249907514728591, 247.3163270870697374, 7.119847084444697494 ) ) ;
#95920=CARTESIAN_POINT ( 'NONE',  ( 153.2712411579340426, 265.1734183057532732, 16.26687330118495467 ) ) ;
#95923=CARTESIAN_POINT ( 'NONE',  ( 207.6477529416552557, 270.9905371579805546, 7.447146952410988341 ) ) ;
#95924=DIRECTION ( 'NONE',  ( 0.4999999999999998890, -0.8660254037844385966, 0.000000000000000000 ) ) ;
#95925=CARTESIAN_POINT ( 'NONE',  ( 148.9831146496684084, 272.6006712873522133, -12.63706091291043343 ) ) ;
#95926=CARTESIAN_POINT ( 'NONE',  ( 179.1373849174831605, 262.4190059985190828, -12.86234133925216661 ) ) ;
#95929=CARTESIAN_POINT ( 'NONE',  ( 168.8002605504911742, 287.8170950039586842, 0.5153475582423447943 ) ) ;
#95932=CARTESIAN_POINT ( 'NONE',  ( 193.8603219414924013, 294.8710681561126989, 15.36476279452078586 ) ) ;
#95934=CARTESIAN_POINT ( 'NONE',  ( 159.9997000813754084, 253.5193855937126841, -16.28798248637880519 ) ) ;
#95937=CARTESIAN_POINT ( 'NONE',  ( 153.4281311866982946, 266.9016768047333130, 16.59090889036721350 ) ) ;
#95938=CARTESIAN_POINT ( 'NONE',  ( 206.9258336080761183, 272.2409381227055292, 6.776000910836894597 ) ) ;
#95940=FACE_OUTER_BOUND ( 'NONE', #22373, .T. ) ;
#95941=ORIENTED_EDGE ( 'NONE', *, *, #17580, .F. ) ;
#95942=ORIENTED_EDGE ( 'NONE', *, *, #92076, .F. ) ;
#95943=CARTESIAN_POINT ( 'NONE',  ( 159.3707800328339772, 279.3010520915150892, -9.512535167852366413 ) ) ;
#95944=CYLINDRICAL_SURFACE ( 'NONE', #3864, 10.00000000000010658 ) ;
#95946=ORIENTED_EDGE ( 'NONE', *, *, #18900, .F. ) ;
#95948=CARTESIAN_POINT ( 'NONE',  ( 174.4609212082891645, 262.3652053495598011, 14.45053099647883421 ) ) ;
#95952=B_SPLINE_CURVE_WITH_KNOTS ( 'NONE', 3,
 ( #98945, #68517, #14326, #21920 ),
 .UNSPECIFIED., .F., .F.,
 ( 4, 4 ),
 ( 0.03783155665041418314, 0.04640911067165707365 ),
 .UNSPECIFIED. ) ;
#95956=CARTESIAN_POINT ( 'NONE',  ( 161.8948331661419218, 250.2369188037922356, 13.64419044796309777 ) ) ;
#95957=CARTESIAN_POINT ( 'NONE',  ( 166.2387117564082928, 273.7804834095634305, -15.53909978882808751 ) ) ;
#95963=CARTESIAN_POINT ( 'NONE',  ( 160.1909080944511174, 268.7107883851168140, -16.56060088188987223 ) ) ;
#95964=VERTEX_POINT ( 'NONE', #97766 ) ;
#95965=CARTESIAN_POINT ( 'NONE',  ( 159.6567935606206277, 270.0351555761940290, 15.68078944156235366 ) ) ;
#95967=CARTESIAN_POINT ( 'NONE',  ( 158.9454381233514653, 259.8133225073038375, 16.87078617150929460 ) ) ;
#95968=CARTESIAN_POINT ( 'NONE',  ( 168.1983705843401538, 272.5412240438793674, 15.99188398643980058 ) ) ;
#95969=CARTESIAN_POINT ( 'NONE',  ( 147.4780248038723869, 275.2075633702266941, 5.829684594924993135 ) ) ;
#95970=CARTESIAN_POINT ( 'NONE',  ( 177.2459596484374345, 288.9155558376918407, -10.33532049625327787 ) ) ;
#95973=CARTESIAN_POINT ( 'NONE',  ( 161.0515428782683500, 277.3244187559503189, -13.42420650014866368 ) ) ;
#95974=CARTESIAN_POINT ( 'NONE',  ( 197.2421906572374439, 289.0134997159141790, -18.24225164680234812 ) ) ;
#95979=CARTESIAN_POINT ( 'NONE',  ( 206.0041637419966776, 273.8373171585603814, 11.66586596407113596 ) ) ;
#95981=CARTESIAN_POINT ( 'NONE',  ( 159.5573297132660002, 254.2855935470410031, 16.91607698584599007 ) ) ;
#95984=CARTESIAN_POINT ( 'NONE',  ( 146.9058596572515114, 276.1985824744942875, -2.634658857186392922 ) ) ;
#95985=CARTESIAN_POINT ( 'NONE',  ( 171.5908562547398617, 259.5510650329395617, -15.12831101081834007 ) ) ;
#95987=CARTESIAN_POINT ( 'NONE',  ( 182.7190055043868142, 259.1992038300794547, 9.912833159430794794 ) ) ;
#95989=CARTESIAN_POINT ( 'NONE',  ( 160.2969203227064554, 253.0045850346894269, -16.23213669264525549 ) ) ;
#95990=EDGE_CURVE ( 'NONE', #48869, #55638, #55282, .T. ) ;
#95991=CARTESIAN_POINT ( 'NONE',  ( 190.4261963075636288, 300.8191482336517311, 0.009177945319502334165 ) ) ;
#95992=ORIENTED_EDGE ( 'NONE', *, *, #15181, .F. ) ;
#95996=CARTESIAN_POINT ( 'NONE',  ( 207.3062152119541679, 271.5820978585240368, 7.879821064966149535 ) ) ;
#95998=CARTESIAN_POINT ( 'NONE',  ( 36.73799359191946934, 192.0177522451418781, -10.00000000000009592 ) ) ;
#95999=CARTESIAN_POINT ( 'NONE',  ( 107.1028179730028285, 223.4548013555409796, -4.594050593750042211 ) ) ;
#96002=CARTESIAN_POINT ( 'NONE',  ( 162.9703553142854560, 248.3740597985417935, 10.27208824138328680 ) ) ;
#96003=CARTESIAN_POINT ( 'NONE',  ( 15.38488118375084390, 185.8149278399160949, -9.188101187500095079 ) ) ;
#96004=CARTESIAN_POINT ( 'NONE',  ( 161.6256441450323678, 250.7031678651938762, 14.48526717260977037 ) ) ;
#96007=CARTESIAN_POINT ( 'NONE',  ( 185.6735584039211346, 258.9728196454306612, -5.407965940105455616 ) ) ;
#96009=CARTESIAN_POINT ( 'NONE',  ( 190.1693911629507738, 301.2639477917662703, -5.112716700269980485 ) ) ;
#96010=CARTESIAN_POINT ( 'NONE',  ( 193.2375489934525774, 264.0021672994329833, -4.337961694823889047 ) ) ;
#96012=CARTESIAN_POINT ( 'NONE',  ( 182.2194435411068412, 284.5217316963779126, 14.88384173871227389 ) ) ;
#96013=CARTESIAN_POINT ( 'NONE',  ( 167.9188900012335353, 251.8113548967955069, 10.43936956030474406 ) ) ;
#96014=CARTESIAN_POINT ( 'NONE',  ( 45.77687342386973057, 206.4244531367911293, -4.594050593750046652 ) ) ;
#96015=CARTESIAN_POINT ( 'NONE',  ( 74.84311135843471163, 224.0177522451419350, 5.000000000000046185 ) ) ;
#96018=B_SPLINE_CURVE_WITH_KNOTS ( 'NONE', 3,
 ( #36192, #90461, #27128, #58010 ),
 .UNSPECIFIED., .F., .F.,
 ( 4, 4 ),
 ( 0.04590184937980493207, 0.04887066958154933499 ),
 .UNSPECIFIED. ) ;
#96020=CARTESIAN_POINT ( 'NONE',  ( 3.504529045289348055, 163.6423013555410080, -4.594050593750043987 ) ) ;
#96022=CARTESIAN_POINT ( 'NONE',  ( 198.7501991201633018, 286.4015524398827779, -18.58948563601804693 ) ) ;
#96024=CARTESIAN_POINT ( 'NONE',  ( 192.8011239859581849, 296.7056528303708660, -11.79847971295421694 ) ) ;
#96027=CARTESIAN_POINT ( 'NONE',  ( 204.9103773355753617, 275.7318107871104189, 13.62808820451859937 ) ) ;
#96028=CARTESIAN_POINT ( 'NONE',  ( 67.73994666856947333, 221.4637435831424739, 2.679491924311251605 ) ) ;
#96029=CARTESIAN_POINT ( 'NONE',  ( 164.2723164851102808, 246.1189969011916503, -1.993789335506892302 ) ) ;
#96030=VERTEX_POINT ( 'NONE', #98263 ) ;
#96031=CARTESIAN_POINT ( 'NONE',  ( 3.630564096624801174, 166.2365022471902307, 10.00000000000009592 ) ) ;
#96034=CARTESIAN_POINT ( 'NONE',  ( 117.4133255192225391, 250.8464784336661353, 1.353441290958777327E-15 ) ) ;
#96036=CARTESIAN_POINT ( 'NONE',  ( 3.578749241215597010, 161.3262482093458061, 3.021315404115420679E-15 ) ) ;
#96040=CARTESIAN_POINT ( 'NONE',  ( 185.2961235551778714, 291.2460235572835927, 13.48139818756336616 ) ) ;
#96043=FACE_OUTER_BOUND ( 'NONE', #46813, .T. ) ;
#96044=CARTESIAN_POINT ( 'NONE',  ( 149.2765980486851731, 272.0923431290771646, -11.40617906909507973 ) ) ;
#96047=CARTESIAN_POINT ( 'NONE',  ( 175.1157827236675359, 291.0147020075365276, -1.073647810211864728 ) ) ;
#96049=ORIENTED_EDGE ( 'NONE', *, *, #46180, .T. ) ;
#96051=DIRECTION ( 'NONE',  ( -0.8660254037844387076, -0.4999999999999998890, -0.000000000000000000 ) ) ;
#96052=CARTESIAN_POINT ( 'NONE',  ( 168.5384773887906817, 271.6194111364977175, -16.60815838436107228 ) ) ;
#96056=CARTESIAN_POINT ( 'NONE',  ( 148.3005007218871754, 275.7829932922234093, 6.053100225771809839 ) ) ;
#96057=ORIENTED_EDGE ( 'NONE', *, *, #25118, .T. ) ;
#96058=CARTESIAN_POINT ( 'NONE',  ( 190.9787802623316395, 280.6762851157768637, 16.68083368884855133 ) ) ;
#96060=CARTESIAN_POINT ( 'NONE',  ( 191.8304510568365515, 287.8979185100550922, -15.87805886543832301 ) ) ;
#96061=ORIENTED_EDGE ( 'NONE', *, *, #85468, .F. ) ;
#96064=CARTESIAN_POINT ( 'NONE',  ( 148.3253847707240141, 273.7398928553401447, -9.074433450356286457 ) ) ;
#96066=ORIENTED_EDGE ( 'NONE', *, *, #91497, .T. ) ;
#96068=CARTESIAN_POINT ( 'NONE',  ( 184.7981748744009565, 292.1161861115109559, 12.46270998733229440 ) ) ;
#96069=ORIENTED_EDGE ( 'NONE', *, *, #27951, .F. ) ;
#96073=ORIENTED_EDGE ( 'NONE', *, *, #97037, .F. ) ;
#96075=CARTESIAN_POINT ( 'NONE',  ( 177.7821213501779596, 260.7347052373945075, 12.22434273024177642 ) ) ;
#96078=VERTEX_POINT ( 'NONE', #14144 ) ;
#96079=CARTESIAN_POINT ( 'NONE',  ( 173.0521476969070420, 271.0393772927264422, 16.43803289686445623 ) ) ;
#96083=CARTESIAN_POINT ( 'NONE',  ( 186.0347410764376264, 282.3483404750993486, -16.68897569456403929 ) ) ;
#96085=CARTESIAN_POINT ( 'NONE',  ( 151.7906504039364677, 268.6165513190795764, 14.84293751212445756 ) ) ;
#96086=CARTESIAN_POINT ( 'NONE',  ( 158.6890521156693978, 274.7924871683402444, -13.35768562937069248 ) ) ;
#96087=CARTESIAN_POINT ( 'NONE',  ( 147.4271219180435253, 275.2957297547342819, -3.800519706258907782 ) ) ;
#96090=B_SPLINE_CURVE_WITH_KNOTS ( 'NONE', 3,
 ( #46806, #39674, #47297, #39178 ),
 .UNSPECIFIED., .F., .F.,
 ( 4, 4 ),
 ( 0.01347489213781506538, 0.01986238529349775711 ),
 .UNSPECIFIED. ) ;
#96092=CARTESIAN_POINT ( 'NONE',  ( 146.0739611433025686, 245.9548013555409796, -4.594050593750042211 ) ) ;
#96094=ORIENTED_EDGE ( 'NONE', *, *, #82293, .T. ) ;
#96096=CARTESIAN_POINT ( 'NONE',  ( 200.0667980463371407, 270.2277230917726456, 9.267277343170334802 ) ) ;
#96100=CARTESIAN_POINT ( 'NONE',  ( 157.4904714317286221, 280.4337344728688208, -7.062405996491910365 ) ) ;
#96101=CARTESIAN_POINT ( 'NONE',  ( 165.4809825843558144, 246.8843404400683426, -1.876936066672490133 ) ) ;
#96103=CARTESIAN_POINT ( 'NONE',  ( 173.1647931292061742, 280.9218488979392987, 13.94953713923030492 ) ) ;
#96107=ORIENTED_EDGE ( 'NONE', *, *, #16510, .T. ) ;
#96108=CARTESIAN_POINT ( 'NONE',  ( 196.9526636073363477, 287.5149752765084941, -17.63101726665603053 ) ) ;
#96109=B_SPLINE_CURVE_WITH_KNOTS ( 'NONE', 3,
 ( #90138, #75922, #68286, #20712, #99207, #5995 ),
 .UNSPECIFIED., .F., .F.,
 ( 4, 2, 4 ),
 ( 0.002220428187929036467, 0.002625085253351148312, 0.003029742318773260158 ),
 .UNSPECIFIED. ) ;
#96114=VECTOR ( 'NONE', #43682, 1000.000000000000000 ) ;
#96115=CARTESIAN_POINT ( 'NONE',  ( 156.8165751444726368, 276.6223283072765753, 10.15807613942431864 ) ) ;
#96118=CARTESIAN_POINT ( 'NONE',  ( 163.4216610345155800, 247.5923753613567442, 10.58669027323842826 ) ) ;
#96127=CARTESIAN_POINT ( 'NONE',  ( 153.1973045377566507, 265.3014802884401320, 17.70608187426261892 ) ) ;
#96130=CARTESIAN_POINT ( 'NONE',  ( 162.6774150396764469, 248.8814472377480911, 10.88033986792731689 ) ) ;
#96131=CARTESIAN_POINT ( 'NONE',  ( 7.915412076110063033, 181.5024278399160949, -9.188101187500093303 ) ) ;
#96132=CARTESIAN_POINT ( 'NONE',  ( 101.9874215621947258, 235.8149278399160664, 9.188101187500093303 ) ) ;
#96133=CARTESIAN_POINT ( 'NONE',  ( 155.6569868912636991, 261.0411854816857158, -17.75433477650897984 ) ) ;
#96135=CARTESIAN_POINT ( 'NONE',  ( 183.4063344672451024, 294.1939596807018233, -7.811441401943769236 ) ) ;
#96138=CARTESIAN_POINT ( 'NONE',  ( 160.2180067946362385, 282.7949301045907760, 5.350916848644969193 ) ) ;
#96139=CARTESIAN_POINT ( 'NONE',  ( 147.6264044922760377, 274.9505622111005323, -8.841872555777701592 ) ) ;
#96140=CARTESIAN_POINT ( 'NONE',  ( 181.4983227144077205, 291.4050983097472454, 9.327077225370901559 ) ) ;
#96141=CARTESIAN_POINT ( 'NONE',  ( 205.2888330531426959, 275.0763062558687579, -13.80886464497609722 ) ) ;
#96143=CARTESIAN_POINT ( 'NONE',  ( 166.2198113297622797, 253.6686547745754012, -13.40419981475687727 ) ) ;
#96144=CYLINDRICAL_SURFACE ( 'NONE', #88682, 17.82106496071139645 ) ;
#96145=CARTESIAN_POINT ( 'NONE',  ( 88.13136219740870558, 215.5643266524159571, -9.188101187500093303 ) ) ;
#96146=CARTESIAN_POINT ( 'NONE',  ( 207.7296438747196134, 270.8486979012336633, -6.692930657757584001 ) ) ;
#96150=CARTESIAN_POINT ( 'NONE',  ( 199.6559772518980651, 284.8326986953333630, 17.73582247532196021 ) ) ;
#96151=CARTESIAN_POINT ( 'NONE',  ( 12.48928228595513801, 188.0177522451419065, 5.000000000000046185 ) ) ;
#96158=CARTESIAN_POINT ( 'NONE',  ( 73.40858323730822121, 219.3149278399160664, 9.188101187500093303 ) ) ;
#96159=CARTESIAN_POINT ( 'NONE',  ( 169.3506085783429569, 288.1634877583111916, -1.098730409881071068 ) ) ;
#96160=CARTESIAN_POINT ( 'NONE',  ( 198.2505066714982149, 285.2670451491296149, 0.000000000000000000 ) ) ;
#96161=CARTESIAN_POINT ( 'NONE',  ( 191.7268773518517548, 288.0406801274909867, -15.82109936370516401 ) ) ;
#96165=CARTESIAN_POINT ( 'NONE',  ( 191.5191886079283279, 287.3386404407627879, 16.08985289718287959 ) ) ;
#96166=CARTESIAN_POINT ( 'NONE',  ( 191.6148588865760871, 296.7603242537468873, -11.89382487812838995 ) ) ;
#96167=CARTESIAN_POINT ( 'NONE',  ( 127.3278592705020742, 250.9865022471903160, 10.00000000000009237 ) ) ;
#96168=CARTESIAN_POINT ( 'NONE',  ( 205.4103625296683617, 274.8658110279089897, -13.38953657917851814 ) ) ;
#96171=CARTESIAN_POINT ( 'NONE',  ( 165.9356184270984613, 246.2207987049553424, -1.153993396985025566 ) ) ;
#96172=ORIENTED_EDGE ( 'NONE', *, *, #87841, .F. ) ;
#96173=CARTESIAN_POINT ( 'NONE',  ( 162.8037981520209314, 248.6625452659484381, 9.809699077002424161 ) ) ;
#96176=CARTESIAN_POINT ( 'NONE',  ( 153.4542976351440302, 264.8563551865710224, -17.11782692037292009 ) ) ;
#96177=ORIENTED_EDGE ( 'NONE', *, *, #34312, .T. ) ;
#96182=CARTESIAN_POINT ( 'NONE',  ( 171.4181495053564106, 290.1579472564245634, 2.469270419063871902 ) ) ;
#96183=CARTESIAN_POINT ( 'NONE',  ( 158.5653297872535177, 257.5252213299329469, -17.07718443373846640 ) ) ;
#96186=CARTESIAN_POINT ( 'NONE',  ( 107.0484310652165192, 232.6115022471902307, 10.00000000000009592 ) ) ;
#96191=CARTESIAN_POINT ( 'NONE',  ( 84.17092664857760553, 212.7365022471902023, 10.00000000000009948 ) ) ;
#96192=VERTEX_POINT ( 'NONE', #43020 ) ;
#96194=CARTESIAN_POINT ( 'NONE',  ( 198.3080508722109698, 286.5404284581068168, 17.10115148743064850 ) ) ;
#96195=CARTESIAN_POINT ( 'NONE',  ( 204.4325665793906524, 276.5594032932251594, 13.33817701435311598 ) ) ;
#96196=CARTESIAN_POINT ( 'NONE',  ( 194.9757425430702824, 292.9391030023704161, -15.21392314336593365 ) ) ;
#96198=CARTESIAN_POINT ( 'NONE',  ( 198.2505066714982149, 285.2670451491296149, 0.000000000000000000 ) ) ;
#96200=CARTESIAN_POINT ( 'NONE',  ( 187.6200950315515854, 291.3050749031608007, -13.78314674982586396 ) ) ;
#96201=CARTESIAN_POINT ( 'NONE',  ( 207.3663924633328577, 271.4778678016768936, -4.575037815448358636 ) ) ;
#96202=CARTESIAN_POINT ( 'NONE',  ( 169.8438327850726637, 267.4680064843133209, 17.16903572500528696 ) ) ;
#96204=CARTESIAN_POINT ( 'NONE',  ( 98.19890751640281223, 221.3768266524159856, -9.188101187500091527 ) ) ;
#96207=CARTESIAN_POINT ( 'NONE',  ( 163.7597937213045611, 277.3359689971894682, -14.45435855620203647 ) ) ;
#96208=ORIENTED_EDGE ( 'NONE', *, *, #28685, .F. ) ;
#96210=EDGE_CURVE ( 'NONE', #39719, #14532, #51734, .T. ) ;
#96212=CARTESIAN_POINT ( 'NONE',  ( 176.8004942653151943, 292.7834445522077544, -2.779440414855350650 ) ) ;
#96214=CARTESIAN_POINT ( 'NONE',  ( 206.8313602288537538, 272.4045708154811791, -9.607337080360906612 ) ) ;
#96216=CARTESIAN_POINT ( 'NONE',  ( 93.32751462011533761, 218.5643266524159856, -9.188101187500093303 ) ) ;
#96218=ADVANCED_FACE ( 'NONE', ( #67338 ), #48314, .F. ) ;
#96219=CARTESIAN_POINT ( 'NONE',  ( 207.5920568422024814, 271.0870056320159165, -1.586464549033245186 ) ) ;
#96221=EDGE_CURVE ( 'NONE', #39284, #74626, #10637, .T. ) ;
#96224=CARTESIAN_POINT ( 'NONE',  ( 165.0397143271508753, 286.3398299935479940, 1.252190257168839249 ) ) ;
#96225=CARTESIAN_POINT ( 'NONE',  ( 132.6770232609233062, 259.6589784336661637, -6.496448406907675876E-16 ) ) ;
#96227=CARTESIAN_POINT ( 'NONE',  ( -13.49147982757802389, 173.0177522451419350, 5.000000000000046185 ) ) ;
#96230=CARTESIAN_POINT ( 'NONE',  ( 204.4735667670548764, 276.4883888850707763, 14.55282211540290227 ) ) ;
#96231=EDGE_CURVE ( 'NONE', #83200, #55188, #1070, .T. ) ;
#96232=CARTESIAN_POINT ( 'NONE',  ( 160.7803790444903314, 275.4413384178728847, 13.47929685474721495 ) ) ;
#96234=EDGE_CURVE ( 'NONE', #7170, #35723, #96552, .T. ) ;
#96235=CARTESIAN_POINT ( 'NONE',  ( 189.1451319728309954, 269.5633631987243461, 15.00206811136211549 ) ) ;
#96236=CARTESIAN_POINT ( 'NONE',  ( 44.26158929084472504, 186.3615022471902023, 5.000000000000051514 ) ) ;
#96238=B_SPLINE_CURVE_WITH_KNOTS ( 'NONE', 3,
 ( #97682, #10572, #73373, #89132, #72387, #97197, #35854, #20174, #3961, #57646, #96202, #72894, #66747, #49555, #51041, #2997, #81999, #19683, #81501, #28248, #11580, #42927, #73866, #59123, #41958, #34843, #88622, #18169, #42438, #80003, #49070, #41447, #33887, #64773, #95721, #26270, #57145, #80508, #18674, #11082, #3485, #34360, #83995, #22650, #44440, #37337, #30247, #53535, #68738, #59635, #99163, #76369 ),
 .UNSPECIFIED., .F., .F.,
 ( 4, 2, 2, 2, 2, 2, 2, 2, 2, 2, 2, 2, 2, 2, 2, 2, 2, 2, 2, 2, 2, 2, 2, 2, 2, 4 ),
 ( 0.001642988356310917143, 0.002095883426664464384, 0.002548778497018011190, 0.002775226032194823625, 0.002888449799783281667, 0.003001673567371739276, 0.003228121102548607221, 0.003454568637725474733, 0.003907463708079213227, 0.004360358778432952588, 0.005266148919140437382, 0.006171939059847923043, 0.006624834130201743936, 0.007077729200555563961, 0.007190952968144056698, 0.007247564851938301765, 0.007304176735732547700, 0.007360788619526793634, 0.007417400503321038702, 0.007530624270909660675, 0.007757071806087032124, 0.007983519341264403574, 0.008209966876441775890, 0.008436414411619144738, 0.008662861946796517054, 0.008889309481973889371 ),
 .UNSPECIFIED. ) ;
#96239=CIRCLE ( 'NONE', #26636, 16.82106496071145685 ) ;
#96240=DIRECTION ( 'NONE',  ( -0.8660254037844387076, -0.4999999999999998890, -0.000000000000000000 ) ) ;
#96244=CARTESIAN_POINT ( 'NONE',  ( 167.6093229551651689, 249.9473136708200229, 7.507881343133518293 ) ) ;
#96246=CARTESIAN_POINT ( 'NONE',  ( 162.6262389125959373, 248.9700868899859074, -10.50380342094597808 ) ) ;
#96247=CARTESIAN_POINT ( 'NONE',  ( 163.1438579415164156, 248.0735444329312713, -11.47272517958888116 ) ) ;
#96250=CARTESIAN_POINT ( 'NONE',  ( 183.1835119402560963, 265.1834291825128389, 13.30006602047987130 ) ) ;
#96251=CARTESIAN_POINT ( 'NONE',  ( 68.76057960370418698, 222.0530062829863027, -4.648177544792955347E-16 ) ) ;
#96255=CARTESIAN_POINT ( 'NONE',  ( 158.2435942055431326, 271.3764418995982055, -14.70623264937866637 ) ) ;
#96257=CARTESIAN_POINT ( 'NONE',  ( 16.08835327644320401, 192.3464784336661637, 1.353441290958777327E-15 ) ) ;
#96259=ORIENTED_EDGE ( 'NONE', *, *, #52189, .T. ) ;
#96263=CARTESIAN_POINT ( 'NONE',  ( 35.49282175392953320, 200.4869531367911293, 4.594050593750046652 ) ) ;
#96264=CIRCLE ( 'NONE', #50959, 17.82106496071138935 ) ;
#96265=ADVANCED_FACE ( 'NONE', ( #41937 ), #72872, .T. ) ;
#96267=CARTESIAN_POINT ( 'NONE',  ( 147.5693121967435957, 275.0494489676833041, 4.210973343677100189 ) ) ;
#96269=CARTESIAN_POINT ( 'NONE',  ( 179.7950818681164833, 292.4219657804791836, 6.105251856334193761 ) ) ;
#96270=CARTESIAN_POINT ( 'NONE',  ( 147.0276296945837373, 275.9876705829954062, 0.7617065417431535534 ) ) ;
#96273=CARTESIAN_POINT ( 'NONE',  ( 166.9910584687719108, 257.7488603398688838, -15.68734378694487752 ) ) ;
#96276=CARTESIAN_POINT ( 'NONE',  ( 82.36670705735998865, 218.3615022471902591, -10.00000000000009592 ) ) ;
#96278=CARTESIAN_POINT ( 'NONE',  ( 187.1412927779018673, 261.9835105880691231, -10.20549468610707322 ) ) ;
#96279=CARTESIAN_POINT ( 'NONE',  ( 49.94514132322986910, 190.4548013555409796, -4.594050593750042211 ) ) ;
#96281=CARTESIAN_POINT ( 'NONE',  ( 162.7713784074331329, 263.3385562889519065, 17.72620173005347866 ) ) ;
#96282=FACE_OUTER_BOUND ( 'NONE', #97557, .T. ) ;
#96283=ADVANCED_FACE ( 'NONE', ( #66728 ), #20091, .F. ) ;
#96285=ORIENTED_EDGE ( 'NONE', *, *, #97417, .F. ) ;
#96286=CARTESIAN_POINT ( 'NONE',  ( 168.0515290973648632, 286.0491048284131921, 8.058232580181940108 ) ) ;
#96288=DIRECTION ( 'NONE',  ( -0.8660254037844387076, -0.4999999999999998890, -0.000000000000000000 ) ) ;
#96290=CARTESIAN_POINT ( 'NONE',  ( 186.1724765274662730, 262.9988875480885895, 11.43256481527857105 ) ) ;
#96291=CARTESIAN_POINT ( 'NONE',  ( 196.3507576896697344, 290.5575069072837664, -17.68249398312240928 ) ) ;
#96293=ORIENTED_EDGE ( 'NONE', *, *, #73411, .T. ) ;
#96296=CARTESIAN_POINT ( 'NONE',  ( 171.6600481915988041, 252.6781227079003997, 8.579917601003849370 ) ) ;
#96300=CARTESIAN_POINT ( 'NONE',  ( 150.6790040019602088, 269.6633047651677089, 15.38315204620803378 ) ) ;
#96302=CARTESIAN_POINT ( 'NONE',  ( 177.3188500945199166, 256.0766865477347665, -7.229946009214981650 ) ) ;
#96303=CARTESIAN_POINT ( 'NONE',  ( 167.9508935690271016, 247.1955620634513480, 0.2374292289661225908 ) ) ;
#96305=B_SPLINE_CURVE_WITH_KNOTS ( 'NONE', 3,
 ( #43951, #74890, #37844, #90622 ),
 .UNSPECIFIED., .F., .F.,
 ( 4, 4 ),
 ( 0.006895705269663468875, 0.01263911957245467989 ),
 .UNSPECIFIED. ) ;
#96308=CARTESIAN_POINT ( 'NONE',  ( 161.8882824960653579, 250.2482648971885340, -13.83574485983625557 ) ) ;
#96309=CARTESIAN_POINT ( 'NONE',  ( 150.9428143250784728, 269.7061216501884928, -13.70542669507604394 ) ) ;
#96310=CARTESIAN_POINT ( 'NONE',  ( 196.2293283710122012, 290.7678286567270902, -17.07152402978540096 ) ) ;
#96313=CARTESIAN_POINT ( 'NONE',  ( 169.5727729373952002, 284.0798650663272156, -11.84966624384599676 ) ) ;
#96316=CARTESIAN_POINT ( 'NONE',  ( 205.2941531242069857, 275.0670916224857478, -13.92605142593109058 ) ) ;
#96318=CARTESIAN_POINT ( 'NONE',  ( 110.6480226958041158, 228.5643266524160708, 9.188101187500095079 ) ) ;
#96319=B_SPLINE_CURVE_WITH_KNOTS ( 'NONE', 3,
 ( #82356, #60469, #98519, #14400 ),
 .UNSPECIFIED., .F., .F.,
 ( 4, 4 ),
 ( 7.881068500304280180E-17, 0.001344325176028971728 ),
 .UNSPECIFIED. ) ;
#96322=CARTESIAN_POINT ( 'NONE',  ( 163.7085541710205234, 247.0954618725873217, -6.713544974106887331 ) ) ;
#96323=VERTEX_POINT ( 'NONE', #85472 ) ;
#96327=CARTESIAN_POINT ( 'NONE',  ( 62.85372508080288867, 219.3464784336661637, 1.353441290958777525E-15 ) ) ;
#96329=CARTESIAN_POINT ( 'NONE',  ( 191.0900422946452011, 299.6693332556258724, 8.872191398975367349 ) ) ;
#96330=CARTESIAN_POINT ( 'NONE',  ( 151.0438343122359584, 269.0314001316289705, 14.41873139571475626 ) ) ;
#96331=CARTESIAN_POINT ( 'NONE',  ( 175.8442789310321928, 278.0726236853578257, 16.35466010686542404 ) ) ;
#96341=CARTESIAN_POINT ( 'NONE',  ( 74.57247842330004062, 213.8615022471902591, -10.00000000000009592 ) ) ;
#96342=EDGE_CURVE ( 'NONE', #24856, #5719, #70233, .T. ) ;
#96343=CARTESIAN_POINT ( 'NONE',  ( 190.7516742497373059, 300.2554039010641418, 4.342609251298632067 ) ) ;
#96344=CARTESIAN_POINT ( 'NONE',  ( 205.7668501412109663, 274.2483563724483133, 11.09689540819876896 ) ) ;
#96345=CARTESIAN_POINT ( 'NONE',  ( 206.4943150373521803, 272.9883502116088039, 11.34100825923693101 ) ) ;
#96346=DIRECTION ( 'NONE',  ( -0.8660254037844387076, -0.4999999999999998890, -0.000000000000000000 ) ) ;
#96347=CARTESIAN_POINT ( 'NONE',  ( 164.1280364607038393, 254.0203960612020921, 14.38687283228996350 ) ) ;
#96349=B_SPLINE_CURVE_WITH_KNOTS ( 'NONE', 3,
 ( #4852, #13450, #59507, #44315 ),
 .UNSPECIFIED., .F., .F.,
 ( 4, 4 ),
 ( 0.04668517186442352335, 0.04887066958154938356 ),
 .UNSPECIFIED. ) ;
#96350=EDGE_CURVE ( 'NONE', #44309, #85762, #23105, .T. ) ;
#96351=CARTESIAN_POINT ( 'NONE',  ( 120.0114017305758551, 252.3464784336661353, 1.353441290958777327E-15 ) ) ;
#96353=CARTESIAN_POINT ( 'NONE',  ( 146.5502055023624735, 276.8145935406849389, 0.3770461397900869427 ) ) ;
#96354=DIRECTION ( 'NONE',  ( 0.5000000000000048850, -0.8660254037844358210, 0.000000000000000000 ) ) ;
#96356=B_SPLINE_CURVE_WITH_KNOTS ( 'NONE', 3,
 ( #48378, #53949, #84905, #268 ),
 .UNSPECIFIED., .F., .F.,
 ( 4, 4 ),
 ( 0.01288686481989116672, 0.01922162384058315882 ),
 .UNSPECIFIED. ) ;
#96357=CARTESIAN_POINT ( 'NONE',  ( 164.4761815919938215, 245.7658921781788592, 6.833796894895563412 ) ) ;
#96361=CARTESIAN_POINT ( 'NONE',  ( 103.4423036115607601, 218.9824982072973967, 3.021315404115420679E-15 ) ) ;
#96362=CARTESIAN_POINT ( 'NONE',  ( 158.5080245674752177, 275.0720563644080130, -12.47040154529214817 ) ) ;
#96363=CARTESIAN_POINT ( 'NONE',  ( 147.8791740781505837, 276.5127524457575987, 2.771564245682613947 ) ) ;
#96364=CARTESIAN_POINT ( 'NONE',  ( 206.9960295002423436, 269.8401794964582905, 1.771342953264500197 ) ) ;
#96365=CARTESIAN_POINT ( 'NONE',  ( 164.2901811315512077, 246.0880544258967575, -1.801919852217561235 ) ) ;
#96366=CARTESIAN_POINT ( 'NONE',  ( 147.5623555321158165, 249.8768266524159856, -9.188101187500093303 ) ) ;
#96367=CARTESIAN_POINT ( 'NONE',  ( 146.9324727656309335, 276.1524872186338371, 3.813717745456558728 ) ) ;
#96368=CARTESIAN_POINT ( 'NONE',  ( 157.3305006125302441, 282.1378183958786963, 1.589776369934247979 ) ) ;
#96369=CARTESIAN_POINT ( 'NONE',  ( 191.2649737798357705, 297.3663430354321235, 11.06343876070684296 ) ) ;
#96371=CARTESIAN_POINT ( 'NONE',  ( 190.7705347155322499, 300.2227366160529414, 3.504769718465625239 ) ) ;
#96372=CARTESIAN_POINT ( 'NONE',  ( 155.2699163265236280, 279.6096657672135279, -1.575243086752120325 ) ) ;
#96373=CARTESIAN_POINT ( 'NONE',  ( 172.4925392983816153, 287.4467975273285560, -8.192266032599757608 ) ) ;
#96375=CARTESIAN_POINT ( 'NONE',  ( 203.3041373168503299, 278.5139001086923827, -16.61929732091214973 ) ) ;
#96376=CARTESIAN_POINT ( 'NONE',  ( 157.0827652098068654, 271.8075571977315121, -14.85186543366582335 ) ) ;
#96377=( BOUNDED_CURVE ( )  B_SPLINE_CURVE ( 2, ( #66555, #36638, #74685, #67044, #60424, #93248, #15701, #8125, #97968 ),
 .UNSPECIFIED., .F., .T. ) 
 B_SPLINE_CURVE_WITH_KNOTS ( ( 3, 2, 2, 2, 3 ),
 ( 0.4798387096774193727, 0.4811827956989247479, 0.4838709677419354982, 0.4865591397849462485, 0.4879032258064516236 ),
 .UNSPECIFIED. ) 
 CURVE ( )  GEOMETRIC_REPRESENTATION_ITEM ( )  RATIONAL_B_SPLINE_CURVE ( ( 0.9330127018922194093, 0.9330127018922194093, 1.000000000000000000, 0.8660254037844387076, 1.000000000000000000, 0.8660254037844387076, 1.000000000000000000, 0.9330127018922194093, 0.9330127018922194093 ) ) 
 REPRESENTATION_ITEM ( '' )  );
#96378=CARTESIAN_POINT ( 'NONE',  ( 127.5984922056368163, 251.1427522451419634, -10.00000000000009415 ) ) ;
#96383=CARTESIAN_POINT ( 'NONE',  ( 196.1573359623355088, 290.8925231663144473, 17.55680092534192482 ) ) ;
#96384=CARTESIAN_POINT ( 'NONE',  ( 148.0427192501136062, 274.2294838985851015, 9.385226820296049155 ) ) ;
#96385=CARTESIAN_POINT ( 'NONE',  ( 1.691375130056927301, 159.5327760586659451, 1.948934522072302763E-15 ) ) ;
#96386=CARTESIAN_POINT ( 'NONE',  ( 34.27488675591641965, 202.8464784336661353, 1.353441290958777327E-15 ) ) ;
#96387=CARTESIAN_POINT ( 'NONE',  ( 175.4807071158155054, 256.8036674190846043, -10.68012024109663827 ) ) ;
#96390=CARTESIAN_POINT ( 'NONE',  ( 157.8820657059571033, 257.1872359237914338, -17.60412210594719440 ) ) ;
#96391=CARTESIAN_POINT ( 'NONE',  ( 188.8632942670357693, 290.4480958481585731, -14.71172498564733644 ) ) ;
#96392=CARTESIAN_POINT ( 'NONE',  ( 190.1607982559816890, 301.2788311432216233, -4.972636536415983244 ) ) ;
#96393=B_SPLINE_CURVE_WITH_KNOTS ( 'NONE', 3,
 ( #40937, #71881, #9583, #56658 ),
 .UNSPECIFIED., .F., .F.,
 ( 4, 4 ),
 ( 0.01101634049414615402, 0.01680390332395608269 ),
 .UNSPECIFIED. ) ;
#96395=CARTESIAN_POINT ( 'NONE',  ( 171.2371238201655217, 258.3827728951262657, 14.06634987601701425 ) ) ;
#96396=CARTESIAN_POINT ( 'NONE',  ( 200.4906113350036776, 281.3870700576555919, -17.24871243658977704 ) ) ;
#96397=CARTESIAN_POINT ( 'NONE',  ( 205.0994677818405023, 275.4042965269534307, -14.14519517703424789 ) ) ;
#96398=CARTESIAN_POINT ( 'NONE',  ( 162.2030298726479884, 251.9395672944197315, -14.03258911121123553 ) ) ;
#96399=CARTESIAN_POINT ( 'NONE',  ( 34.30229714732359980, 200.6115022471903160, -5.000000000000047962 ) ) ;
#96402=CARTESIAN_POINT ( 'NONE',  ( 1.204062292545672097, 165.3768266524159856, 9.188101187500098632 ) ) ;
#96404=CARTESIAN_POINT ( 'NONE',  ( -22.42236680055709641, 157.8615022471902591, 0.000000000000000000 ) ) ;
#96405=CARTESIAN_POINT ( 'NONE',  ( 192.5254593562406171, 297.1831179748913314, 11.00703791256144015 ) ) ;
#96407=CARTESIAN_POINT ( 'NONE',  ( 75.30212449506053929, 225.8297689869268652, -2.679491924311252493 ) ) ;
#96409=CARTESIAN_POINT ( 'NONE',  ( 179.5755015609138354, 277.2059287606015801, 16.35061197133128275 ) ) ;
#96411=CARTESIAN_POINT ( 'NONE',  ( 67.57210640937580592, 216.4865022471902876, 10.00000000000009415 ) ) ;
#96417=CARTESIAN_POINT ( 'NONE',  ( 159.6023402823087451, 258.6676503891110883, 17.43025742997651761 ) ) ;
#96419=CARTESIAN_POINT ( 'NONE',  ( 154.8838596469624349, 262.3802811495310152, 18.07457254681616021 ) ) ;
#96421=CARTESIAN_POINT ( 'NONE',  ( 156.2426905888906958, 276.2173076510940177, 10.27655790510740985 ) ) ;
#96423=CARTESIAN_POINT ( 'NONE',  ( 158.8266160086023149, 257.5512268093053194, -17.29683829744028856 ) ) ;
#96424=CARTESIAN_POINT ( 'NONE',  ( -17.42236680055705023, 149.2012482093457777, 0.000000000000000000 ) ) ;
#96427=CARTESIAN_POINT ( 'NONE',  ( 192.4454213697443095, 297.3217478340386606, 12.58566886711101596 ) ) ;
#96428=CARTESIAN_POINT ( 'NONE',  ( 207.1059763530604698, 271.9289217357780899, 6.370907250589925575 ) ) ;
#96431=EDGE_CURVE ( 'NONE', #85237, #30618, #4638, .T. ) ;
#96432=CARTESIAN_POINT ( 'NONE',  ( 125.6883311748214425, 231.8262482093457493, 3.021315404115420679E-15 ) ) ;
#96433=ORIENTED_EDGE ( 'NONE', *, *, #37924, .T. ) ;
#96436=CARTESIAN_POINT ( 'NONE',  ( 204.8284483594339065, 275.8737159363993214, 14.69997973035875383 ) ) ;
#96440=CARTESIAN_POINT ( 'NONE',  ( 178.1946123598630720, 263.8186659389383522, 15.20355339309904963 ) ) ;
#96443=CARTESIAN_POINT ( 'NONE',  ( 84.80240350195585108, 209.7677522451417929, -5.000000000000041744 ) ) ;
#96445=EDGE_LOOP ( 'NONE', ( #12324, #19053, #88600, #32385 ) ) ;
#96446=CARTESIAN_POINT ( 'NONE',  ( 161.4469036912142599, 251.0127554125742222, 12.93933463576739307 ) ) ;
#96447=CARTESIAN_POINT ( 'NONE',  ( 166.7606102460582918, 274.5312062198365197, -15.18303354322240395 ) ) ;
#96452=CARTESIAN_POINT ( 'NONE',  ( 148.9230895364621574, 272.7046378331555161, 12.20434325797056019 ) ) ;
#96453=CARTESIAN_POINT ( 'NONE',  ( 202.9216520459657147, 279.1763840310111391, 15.75371595331685803 ) ) ;
#96454=VERTEX_POINT ( 'NONE', #72756 ) ;
#96457=VERTEX_POINT ( 'NONE', #32715 ) ;
#96458=CARTESIAN_POINT ( 'NONE',  ( 157.0284915711613678, 269.7273995439030045, 16.18108137139518732 ) ) ;
#96461=CARTESIAN_POINT ( 'NONE',  ( 147.8105987091051645, 274.6315284690918475, 6.028275121586289309 ) ) ;
#96462=CARTESIAN_POINT ( 'NONE',  ( 180.5415972302508010, 291.3317084335843674, -9.685907878306698748 ) ) ;
#96463=CARTESIAN_POINT ( 'NONE',  ( 133.4622058806418750, 257.8615022471902876, 5.000000000000046185 ) ) ;
#96464=CARTESIAN_POINT ( 'NONE',  ( 199.5820190223589066, 281.0610403850588455, -17.29246150691365358 ) ) ;
#96467=CARTESIAN_POINT ( 'NONE',  ( 128.5163324648304410, 256.5530062829863027, -4.648177544792955347E-16 ) ) ;
#96469=CARTESIAN_POINT ( 'NONE',  ( 156.9440562780969231, 274.4750137900673508, 13.77464823823377316 ) ) ;
#96471=CARTESIAN_POINT ( 'NONE',  ( 165.0087721269838710, 244.8434183119457543, 2.604344609212914108 ) ) ;
#96472=CARTESIAN_POINT ( 'NONE',  ( 159.9880386575927957, 253.5395837721924863, 15.85893018594752846 ) ) ;
#96474=ORIENTED_EDGE ( 'NONE', *, *, #4721, .F. ) ;
#96475=CARTESIAN_POINT ( 'NONE',  ( 187.6035355654556724, 277.1252990796724589, 17.06676580984018443 ) ) ;
#96480=CARTESIAN_POINT ( 'NONE',  ( 160.6603037333772761, 252.3751865047794070, -15.24058959229929222 ) ) ;
#96481=CARTESIAN_POINT ( 'NONE',  ( 147.9974455564266691, 274.3079002362971437, -10.09869768668086820 ) ) ;
#96482=VERTEX_POINT ( 'NONE', #1331 ) ;
#96483=DIRECTION ( 'NONE',  ( -0.8660254037844387076, -0.4999999999999998890, -0.000000000000000000 ) ) ;
#96485=CARTESIAN_POINT ( 'NONE',  ( 155.5582350408321588, 263.0053103591359900, 17.59663451232534825 ) ) ;
#96486=CARTESIAN_POINT ( 'NONE',  ( 26.34568874650619463, 186.0177522451418497, -10.00000000000009592 ) ) ;
#96487=CARTESIAN_POINT ( 'NONE',  ( 97.41363812451689341, 236.2369531367911009, -4.594050593750048428 ) ) ;
#96488=CARTESIAN_POINT ( 'NONE',  ( 183.9927074563704537, 296.7549153586903685, -2.755382768168008756 ) ) ;
#96489=CARTESIAN_POINT ( 'NONE',  ( 167.4702904630335070, 282.8281168849647997, -10.76115858899906108 ) ) ;
#96491=CARTESIAN_POINT ( 'NONE',  ( 207.7117873102786518, 270.8796263780940308, 1.712754233133884085 ) ) ;
#96492=CARTESIAN_POINT ( 'NONE',  ( 16.52171307410043255, 180.3458772461660544, 9.188101187500095079 ) ) ;
#96493=AXIS2_PLACEMENT_3D ( 'NONE', #20207, #50098, #81534 ) ;
#96497=CARTESIAN_POINT ( 'NONE',  ( 147.6461304576096438, 276.1816894454201474, -0.8296389602296602162 ) ) ;
#96500=FACE_OUTER_BOUND ( 'NONE', #42794, .T. ) ;
#96501=CARTESIAN_POINT ( 'NONE',  ( 193.4275275796228186, 262.9968912118912954, -3.779748889324304528 ) ) ;
#96503=CARTESIAN_POINT ( 'NONE',  ( 207.6357208050208101, 271.0113774299547913, -6.790259683043212036 ) ) ;
#96504=CARTESIAN_POINT ( 'NONE',  ( 185.7809047750413356, 286.4304272575490700, 15.54309313237488155 ) ) ;
#96506=CARTESIAN_POINT ( 'NONE',  ( 46.56214281575564939, 191.5643266524159856, -9.188101187500093303 ) ) ;
#96507=CARTESIAN_POINT ( 'NONE',  ( 89.99855592466239784, 232.7677522451419065, -5.000000000000047962 ) ) ;
#96508=ORIENTED_EDGE ( 'NONE', *, *, #39180, .F. ) ;
#96509=ADVANCED_FACE ( 'NONE', ( #78840 ), #56514, .T. ) ;
#96511=CARTESIAN_POINT ( 'NONE',  ( 178.7669947432931110, 259.1165679222901304, -10.20806745893763079 ) ) ;
#96512=CARTESIAN_POINT ( 'NONE',  ( 4.992923434102598534, 167.5643266524160140, -9.188101187500093303 ) ) ;
#96514=CARTESIAN_POINT ( 'NONE',  ( 150.6815632051821581, 269.6588720951601772, -14.68790257316217307 ) ) ;
#96517=CARTESIAN_POINT ( 'NONE',  ( 147.4271219180435253, 275.2957297547342819, -3.800519706258907782 ) ) ;
#96519=CARTESIAN_POINT ( 'NONE',  ( 204.8523313866422484, 275.8323493198358847, 14.65426965484541100 ) ) ;
#96521=CARTESIAN_POINT ( 'NONE',  ( 207.6007741873543750, 271.0719067473055475, 7.587922723682903658 ) ) ;
#96522=ORIENTED_EDGE ( 'NONE', *, *, #27585, .F. ) ;
#96524=CARTESIAN_POINT ( 'NONE',  ( 164.4414259850711915, 245.8260906552167171, -6.983224448873608381 ) ) ;
#96525=CARTESIAN_POINT ( 'NONE',  ( 7.094665711762558225, 168.2365022471901739, -10.00000000000009059 ) ) ;
#96527=CARTESIAN_POINT ( 'NONE',  ( 122.0685591603289026, 241.2833772461660544, -9.188101187500095079 ) ) ;
#96531=CARTESIAN_POINT ( 'NONE',  ( 157.3363371328520088, 258.1324655395517311, 18.24585617226787093 ) ) ;
#96535=CARTESIAN_POINT ( 'NONE',  ( 151.0778907302193943, 268.9724126853576536, 15.84769371787143832 ) ) ;
#96536=CARTESIAN_POINT ( 'NONE',  ( 207.6440815245055092, 270.9968962390196339, -0.7124146351304289082 ) ) ;
#96541=CARTESIAN_POINT ( 'NONE',  ( 138.1351346183475357, 243.8927522451417929, -10.00000000000009237 ) ) ;
#96544=EDGE_CURVE ( 'NONE', #3105, #13470, #55009, .T. ) ;
#96547=CARTESIAN_POINT ( 'NONE',  ( 156.6812872898450735, 261.2670451491295012, 0.000000000000000000 ) ) ;
#96550=CARTESIAN_POINT ( 'NONE',  ( 150.2135478535318782, 277.3480115108075097, -0.0001741048118424651735 ) ) ;
#96551=ORIENTED_EDGE ( 'NONE', *, *, #4528, .T. ) ;
#96552=B_SPLINE_CURVE_WITH_KNOTS ( 'NONE', 3,
 ( #57626, #10051, #88604, #80489, #65236, #9043, #41425, #17134, #72370, #70846, #87620, #40424, #25235, #63240, #3464, #34341, #49535, #1949, #88106, #94181, #79488, #48032, #2976, #32833, #49048, #9561, #64754, #63743, #95702, #87114, #56637, #2459, #17650, #10551, #94677, #71863, #56121, #48548, #79984, #33341, #26249, #11060 ),
 .UNSPECIFIED., .F., .F.,
 ( 4, 2, 2, 2, 2, 2, 2, 2, 2, 2, 2, 2, 2, 2, 2, 2, 2, 2, 2, 2, 4 ),
 ( 0.0009056366646472498085, 0.001003186449675941110, 0.001100736234704632411, 0.001198286019733323712, 0.001295835804762014796, 0.001490935374819419949, 0.001686034944876825103, 0.002466433225106563244, 0.004027229785566034323, 0.004807628065795770296, 0.005197827205910719381, 0.005392926775968194357, 0.005490476560996922738, 0.005588026346025650251, 0.005636801238540015309, 0.005685576131054379499, 0.005783125916083084461, 0.005978225486140473569, 0.006368424626255224895, 0.006758623766369976221, 0.007148822906484728415 ),
 .UNSPECIFIED. ) ;
#96557=ORIENTED_EDGE ( 'NONE', *, *, #29284, .T. ) ;
#96559=ADVANCED_FACE ( 'NONE', ( #18037 ), #63615, .T. ) ;
#96560=CARTESIAN_POINT ( 'NONE',  ( 194.9385458806846430, 293.0035295114944347, -15.70518692812489192 ) ) ;
#96561=CARTESIAN_POINT ( 'NONE',  ( 159.6649394982892716, 264.0993667363822510, -17.39019615698379795 ) ) ;
#96564=CARTESIAN_POINT ( 'NONE',  ( 204.7319642249719038, 272.9966618342774041, -9.756553772762273979 ) ) ;
#96566=AXIS2_PLACEMENT_3D ( 'NONE', #15934, #70123, #31124 ) ;
#96567=DIRECTION ( 'NONE',  ( -0.8660254037844387076, -0.4999999999999998890, -0.000000000000000000 ) ) ;
#96569=CARTESIAN_POINT ( 'NONE',  ( 89.94416901687610277, 231.9244531367911009, -4.594050593750046652 ) ) ;
#96574=CARTESIAN_POINT ( 'NONE',  ( 181.8938501633026874, 257.1921657151197564, -6.106366152575129824 ) ) ;
#96575=EDGE_LOOP ( 'NONE', ( #83214, #64622, #2209, #81775 ) ) ;
#96580=CARTESIAN_POINT ( 'NONE',  ( 144.9863040978925142, 263.1751974929321705, -1.822351119449947324E-15 ) ) ;
#96581=ORIENTED_EDGE ( 'NONE', *, *, #72896, .T. ) ;
#96582=CARTESIAN_POINT ( 'NONE',  ( 169.6747932974647028, 272.0074737424269529, -17.60367342859795059 ) ) ;
#96583=CARTESIAN_POINT ( 'NONE',  ( 154.9528145190857344, 262.2608478075840708, -17.26679351315302213 ) ) ;
#96584=ORIENTED_EDGE ( 'NONE', *, *, #85999, .F. ) ;
#96585=CARTESIAN_POINT ( 'NONE',  ( 182.9098479943871212, 279.8073795562751798, -16.44634284297093885 ) ) ;
#96587=CARTESIAN_POINT ( 'NONE',  ( 151.3074424083568204, 269.1194857459262266, 14.21895990402933307 ) ) ;
#96588=FACE_OUTER_BOUND ( 'NONE', #10823, .T. ) ;
#96589=CARTESIAN_POINT ( 'NONE',  ( 201.1388841337167435, 282.2642286331299601, -18.17233400608081340 ) ) ;
#96591=CARTESIAN_POINT ( 'NONE',  ( 157.4068442735347446, 281.9945091197541274, 2.874377194828706905 ) ) ;
#96592=CARTESIAN_POINT ( 'NONE',  ( 142.6906155400633622, 259.3149278399160380, -9.188101187500095079 ) ) ;
#96597=CARTESIAN_POINT ( 'NONE',  ( 200.0079957071587273, 270.2013779111154577, 9.272782244027494514 ) ) ;
#96602=CARTESIAN_POINT ( 'NONE',  ( 129.4230657250939203, 233.9824982072973683, 3.021315404115420679E-15 ) ) ;
#96603=CARTESIAN_POINT ( 'NONE',  ( 153.2255732592549009, 277.0430973404892825, 6.869329404264208350 ) ) ;
#96604=CARTESIAN_POINT ( 'NONE',  ( 165.5128516766338294, 246.9059456859405373, -1.886539856749224420 ) ) ;
#96605=VECTOR ( 'NONE', #65445, 1000.000000000000114 ) ;
#96606=CARTESIAN_POINT ( 'NONE',  ( 192.6480976257870452, 292.3694868334920329, -14.35794368392827636 ) ) ;
#96609=ORIENTED_EDGE ( 'NONE', *, *, #81456, .F. ) ;
#96610=CARTESIAN_POINT ( 'NONE',  ( 147.6264044922760377, 274.9505622111005323, -8.841872555777701592 ) ) ;
#96613=CARTESIAN_POINT ( 'NONE',  ( -18.11259370987442452, 171.8967562850347406, 9.296355089585912665E-16 ) ) ;
#96614=CARTESIAN_POINT ( 'NONE',  ( 201.0067457102312005, 267.8329504270425900, -2.840095696601848907 ) ) ;
#96615=CARTESIAN_POINT ( 'NONE',  ( 203.8401700684498792, 277.5854641484010585, -14.28809178781177636 ) ) ;
#96617=EDGE_CURVE ( 'NONE', #45450, #1077, #8229, .T. ) ;
#96618=CARTESIAN_POINT ( 'NONE',  ( 202.4900219881211854, 279.9239892212719383, 15.63116161057562259 ) ) ;
#96625=CARTESIAN_POINT ( 'NONE',  ( 153.0070714074088016, 265.6309737354857248, 17.74442213480098474 ) ) ;
#96626=CARTESIAN_POINT ( 'NONE',  ( -27.42236680055714260, 166.5217562850347406, 1.224646799147364892E-15 ) ) ;
#96628=CARTESIAN_POINT ( 'NONE',  ( 6.805730253569997501, 183.9244531367911293, -4.594050593750046652 ) ) ;
#96629=CARTESIAN_POINT ( 'NONE',  ( 107.1835739849013578, 238.8149278399160664, 9.188101187500093303 ) ) ;
#96631=CARTESIAN_POINT ( 'NONE',  ( 179.9070225497684419, 255.1121438720595620, -2.403939176287567037 ) ) ;
#96636=VECTOR ( 'NONE', #6684, 1000.000000000000000 ) ;
#96637=CARTESIAN_POINT ( 'NONE',  ( 160.7389373414059435, 281.8969065408946335, 5.212150423231117990 ) ) ;
#96638=CARTESIAN_POINT ( 'NONE',  ( 194.7576540903134799, 293.3168432830895540, -14.62421624641040196 ) ) ;
#96644=CARTESIAN_POINT ( 'NONE',  ( 173.3240139114783460, 264.2345359633658859, -15.45835341172655930 ) ) ;
#96645=CARTESIAN_POINT ( 'NONE',  ( 76.33141897508073725, 221.0024278399160949, 9.188101187500095079 ) ) ;
#96646=CARTESIAN_POINT ( 'NONE',  ( 161.0965315767822972, 251.6196177163260188, -13.76772246540905442 ) ) ;
#96648=CARTESIAN_POINT ( 'NONE',  ( 163.4477778843836404, 257.9215091531312396, 15.58283331752105738 ) ) ;
#96649=CARTESIAN_POINT ( 'NONE',  ( 196.4677102463732012, 290.3549391369982686, 16.45225250689336249 ) ) ;
#96650=CARTESIAN_POINT ( 'NONE',  ( 151.9413948867106683, 267.4767796137679170, 15.48523777917124100 ) ) ;
#96652=CARTESIAN_POINT ( 'NONE',  ( 176.5572900059099197, 270.1083417844832866, -16.76627801634431947 ) ) ;
#96658=CARTESIAN_POINT ( 'NONE',  ( 171.8195984572240889, 288.9771131316106789, -1.063263625893295483 ) ) ;
#96662=CARTESIAN_POINT ( 'NONE',  ( 189.7523420421647131, 286.5162620012252432, 16.62308081069983956 ) ) ;
#96665=CARTESIAN_POINT ( 'NONE',  ( 115.2756724011686202, 247.3615022471903160, 5.000000000000046185 ) ) ;
#96666=( BOUNDED_CURVE ( )  B_SPLINE_CURVE ( 2, ( #64124, #86486, #2854, #25637, #24126, #85993, #70723, #33744, #64636 ),
 .UNSPECIFIED., .F., .T. ) 
 B_SPLINE_CURVE_WITH_KNOTS ( ( 3, 2, 2, 2, 3 ),
 ( 0.2620967741935483764, 0.2634408602150537515, 0.2661290322580645018, 0.2688172043010752521, 0.2701612903225806273 ),
 .UNSPECIFIED. ) 
 CURVE ( )  GEOMETRIC_REPRESENTATION_ITEM ( )  RATIONAL_B_SPLINE_CURVE ( ( 0.9330127018922194093, 0.9330127018922194093, 1.000000000000000000, 0.8660254037844387076, 1.000000000000000000, 0.8660254037844387076, 1.000000000000000000, 0.9330127018922194093, 0.9330127018922194093 ) ) 
 REPRESENTATION_ITEM ( '' )  );
#96667=CARTESIAN_POINT ( 'NONE',  ( 157.8696211474012330, 257.2087905314882619, -17.27527248276125604 ) ) ;
#96669=AXIS2_PLACEMENT_3D ( 'NONE', #78535, #93763, #53220 ) ;
#96671=CARTESIAN_POINT ( 'NONE',  ( 169.5637984545885786, 248.3293919737242845, -1.956443885671045102 ) ) ;
#96672=ORIENTED_EDGE ( 'NONE', *, *, #5435, .F. ) ;
#96673=CARTESIAN_POINT ( 'NONE',  ( 203.0535368433499457, 278.9479528611958585, 16.46202213522710167 ) ) ;
#96674=CARTESIAN_POINT ( 'NONE',  ( 182.7674680796695554, 291.1753568628804487, -12.34959082582511058 ) ) ;
#96675=EDGE_CURVE ( 'NONE', #28264, #50323, #27624, .T. ) ;
#96678=ORIENTED_EDGE ( 'NONE', *, *, #44375, .T. ) ;
#96681=CARTESIAN_POINT ( 'NONE',  ( 141.9056932439424372, 261.9244531367911577, -4.594050593750046652 ) ) ;
#96682=CARTESIAN_POINT ( 'NONE',  ( 205.4925884257800988, 274.0740247280971857, 10.80283695292349222 ) ) ;
#96686=CARTESIAN_POINT ( 'NONE',  ( 164.6915199398825393, 274.4969406795170812, 14.73953457787395749 ) ) ;
#96687=( BOUNDED_CURVE ( )  B_SPLINE_CURVE ( 2, ( #84741, #61390, #62894, #9206, #38591, #8704, #7193, #39076, #603 ),
 .UNSPECIFIED., .F., .T. ) 
 B_SPLINE_CURVE_WITH_KNOTS ( ( 3, 2, 2, 2, 3 ),
 ( 0.9314516129032257563, 0.9327956989247311315, 0.9354838709677418818, 0.9381720430107527431, 0.9395161290322581182 ),
 .UNSPECIFIED. ) 
 CURVE ( )  GEOMETRIC_REPRESENTATION_ITEM ( )  RATIONAL_B_SPLINE_CURVE ( ( 0.9330127018922194093, 0.9330127018922194093, 1.000000000000000000, 0.8660254037844387076, 1.000000000000000000, 0.8660254037844387076, 1.000000000000000000, 0.9330127018922194093, 0.9330127018922194093 ) ) 
 REPRESENTATION_ITEM ( '' )  );
#96693=CARTESIAN_POINT ( 'NONE',  ( 194.9220242159064185, 293.0321458743159724, -14.92681063007793263 ) ) ;
#96696=CARTESIAN_POINT ( 'NONE',  ( 123.2683651867145898, 248.6427522451419350, 10.00000000000009415 ) ) ;
#96699=CARTESIAN_POINT ( 'NONE',  ( 208.1405733532425018, 270.1369471661045623, -4.189134151581175303 ) ) ;
#96702=CARTESIAN_POINT ( 'NONE',  ( 99.93095832397169431, 222.3768266524160140, 9.188101187500098632 ) ) ;
#96703=EDGE_LOOP ( 'NONE', ( #39299, #59354, #2660, #65126 ) ) ;
#96705=CARTESIAN_POINT ( 'NONE',  ( 163.7315607857516682, 276.6876062851454208, -13.69158268838586245 ) ) ;
#96707=ORIENTED_EDGE ( 'NONE', *, *, #79849, .T. ) ;
#96711=CARTESIAN_POINT ( 'NONE',  ( 177.1313973275757405, 292.4482777636210926, -2.705817427292956268 ) ) ;
#96713=CARTESIAN_POINT ( 'NONE',  ( 195.8627871995700502, 291.4026965887302936, 17.41145040657729481 ) ) ;
#96714=CARTESIAN_POINT ( 'NONE',  ( 159.9894443651313338, 253.5371490153152081, -16.36035038356864391 ) ) ;
#96715=CARTESIAN_POINT ( 'NONE',  ( 162.9703553142854560, 248.3740597985417935, 10.27208824138328680 ) ) ;
#96716=CARTESIAN_POINT ( 'NONE',  ( 92.94880205384217220, 212.2202760586659736, -5.415160957724236172E-17 ) ) ;
#96717=EDGE_LOOP ( 'NONE', ( #96172, #94793, #91551, #78834 ) ) ;
#96721=CARTESIAN_POINT ( 'NONE',  ( 162.6341128535665064, 248.9564488241690299, -10.63508949045170660 ) ) ;
#96724=CARTESIAN_POINT ( 'NONE',  ( 193.2053853833890287, 265.4515565053490604, -7.760948457033734371 ) ) ;
#96726=EDGE_CURVE ( 'NONE', #23023, #41212, #77116, .T. ) ;
#96728=CARTESIAN_POINT ( 'NONE',  ( 134.1932619090760568, 236.0327760586659736, 1.948934522072303157E-15 ) ) ;
#96730=CARTESIAN_POINT ( 'NONE',  ( 154.8782533782051871, 264.3899914918594050, -17.45241046926759765 ) ) ;
#96731=ORIENTED_EDGE ( 'NONE', *, *, #97659, .T. ) ;
#96733=CARTESIAN_POINT ( 'NONE',  ( 157.3812306876618266, 258.0547076216885785, 17.10114491953027027 ) ) ;
#96734=CARTESIAN_POINT ( 'NONE',  ( 157.8961455691572837, 274.3508122300142986, 13.06461853355700775 ) ) ;
#96737=CARTESIAN_POINT ( 'NONE',  ( 178.2793323077814591, 285.7144920781913697, 14.42518415939602683 ) ) ;
#96738=B_SPLINE_CURVE_WITH_KNOTS ( 'NONE', 3,
 ( #51951, #97577, #59523, #28148, #20565, #51444, #67143, #90502, #75263, #21075, #82891, #13465, #44331, #36733, #98572, #29155, #81715, #35573, #42168, #3214, #35066, #88344, #57870, #89339, #56869, #19891, #18394, #57369, #33590, #12796, #49779, #34575, #50763, #64486, #87853, #42655, #27493, #65972 ),
 .UNSPECIFIED., .F., .F.,
 ( 4, 2, 2, 2, 2, 2, 2, 2, 2, 2, 2, 2, 2, 2, 2, 2, 2, 2, 4 ),
 ( 0.0009333477296225796459, 0.001027619387414748084, 0.001121891045206916413, 0.001310434360791252638, 0.001687520991959938314, 0.002441694254297281912, 0.003950040778971889745, 0.004704214041309194745, 0.005081300672477920104, 0.005269843988062358243, 0.005364115645854540017, 0.005458387303646720923, 0.005505523132542770176, 0.005552658961438818562, 0.005646930619230842475, 0.005835473934814966630, 0.006212560565983246165, 0.006589647197151524832, 0.006966733828319804367 ),
 .UNSPECIFIED. ) ;
#96740=EDGE_CURVE ( 'NONE', #32549, #38232, #21037, .T. ) ;
#96741=CARTESIAN_POINT ( 'NONE',  ( 195.4525600527361746, 279.6603085545519320, -17.06130316034534999 ) ) ;
#96744=AXIS2_PLACEMENT_3D ( 'NONE', #49018, #42874, #33831 ) ;
#96745=CARTESIAN_POINT ( 'NONE',  ( 206.3512583665959994, 271.5101124371017818, 7.607313674450764118 ) ) ;
#96746=CARTESIAN_POINT ( 'NONE',  ( 167.7141816491835868, 249.9697211030261883, 6.963387598742469820 ) ) ;
#96748=CARTESIAN_POINT ( 'NONE',  ( 188.9122134955663910, 290.7695941481946988, -15.11888497690123678 ) ) ;
#96756=CARTESIAN_POINT ( 'NONE',  ( 160.5496179049985130, 273.2860930542701112, -15.62709310798295803 ) ) ;
#96758=CARTESIAN_POINT ( 'NONE',  ( 161.1750406344237661, 251.4836360396366501, -14.21198410781773802 ) ) ;
#96759=CARTESIAN_POINT ( 'NONE',  ( 10.35128207213630169, 176.7833772461660544, -9.188101187500095079 ) ) ;
#96760=CARTESIAN_POINT ( 'NONE',  ( 207.1433070480561014, 270.6377863507698294, 3.317773331146615323 ) ) ;
#96763=B_SPLINE_CURVE_WITH_KNOTS ( 'NONE', 3,
 ( #74608, #4687, #27968, #57372 ),
 .UNSPECIFIED., .F., .F.,
 ( 4, 4 ),
 ( 0.005575214141566578116, 0.01056667930948825516 ),
 .UNSPECIFIED. ) ;
#96765=CARTESIAN_POINT ( 'NONE',  ( 33.00325904164698443, 189.8615022471902591, -10.00000000000009592 ) ) ;
#96766=CARTESIAN_POINT ( 'NONE',  ( 207.6590484093196096, 270.9709728340903894, 3.402057849327809524 ) ) ;
#96768=CARTESIAN_POINT ( 'NONE',  ( 36.16949087457737733, 197.8149278399160949, -9.188101187500095079 ) ) ;
#96770=CARTESIAN_POINT ( 'NONE',  ( 200.9111546617170916, 282.6586676490145464, 17.66063511622358106 ) ) ;
#96771=CARTESIAN_POINT ( 'NONE',  ( 147.5813496936708020, 275.0285994114094592, 4.516581957185684004 ) ) ;
#96773=CARTESIAN_POINT ( 'NONE',  ( 183.7975612849717777, 256.6346208101135176, -2.981236333899912161 ) ) ;
#96774=CARTESIAN_POINT ( 'NONE',  ( 191.4082244002820516, 299.1182256826033949, -8.271837126846561361 ) ) ;
#96776=CARTESIAN_POINT ( 'NONE',  ( 179.7576857715609435, 278.6407688031329712, -16.34641460967070259 ) ) ;
#96778=B_SPLINE_CURVE_WITH_KNOTS ( 'NONE', 3,
 ( #75927, #30295, #82556, #28292, #44483, #76415, #45481, #83038, #90140, #98218, #5998, #29796, #68288, #22703, #99706, #6506 ),
 .UNSPECIFIED., .F., .F.,
 ( 4, 2, 2, 2, 2, 2, 2, 4 ),
 ( 3.469446951953614189E-18, 0.0003787177898466141516, 0.0007574355796932248338, 0.001136153369539835353, 0.001514871159386446198, 0.001893588949233056826, 0.002272306739079667237, 0.003029742318772781808 ),
 .UNSPECIFIED. ) ;
#96785=CARTESIAN_POINT ( 'NONE',  ( 86.26382137439000530, 210.6115022471902023, -5.000000000000041744 ) ) ;
#96789=CARTESIAN_POINT ( 'NONE',  ( 49.51212862133765213, 190.2048013555409796, 4.594050593750051981 ) ) ;
#96792=CARTESIAN_POINT ( 'NONE',  ( 150.7850480413316632, 269.4796311011364764, -14.43114374163211089 ) ) ;
#96795=ORIENTED_EDGE ( 'NONE', *, *, #99560, .T. ) ;
#96796=CARTESIAN_POINT ( 'NONE',  ( 171.3574066310837054, 286.5369029633047830, 8.062752042993464485 ) ) ;
#96797=CARTESIAN_POINT ( 'NONE',  ( 206.9377610035629118, 272.2202792677204002, 7.440532334334675646 ) ) ;
#96798=CARTESIAN_POINT ( 'NONE',  ( 192.7288556637334125, 292.1918731402626577, -15.52061534916644447 ) ) ;
#96800=CARTESIAN_POINT ( 'NONE',  ( 185.9360266901250043, 262.9690012174675076, 11.35307557420283686 ) ) ;
#96801=CARTESIAN_POINT ( 'NONE',  ( 196.3174919959537306, 290.6151247789487684, -17.61248417473235151 ) ) ;
#96802=CARTESIAN_POINT ( 'NONE',  ( 171.4894766845286540, 255.7030988890395236, 11.23559410916937296 ) ) ;
#96806=CARTESIAN_POINT ( 'NONE',  ( 174.8283672253976704, 255.1773154208834455, 8.220612995860930639 ) ) ;
#96808=EDGE_CURVE ( 'NONE', #47657, #8304, #6961, .T. ) ;
#96809=ORIENTED_EDGE ( 'NONE', *, *, #2279, .F. ) ;
#96810=CARTESIAN_POINT ( 'NONE',  ( 182.4154252063833894, 284.1042553539095366, 14.98678786608993185 ) ) ;
#96811=CARTESIAN_POINT ( 'NONE',  ( 151.4361976351029000, 268.3518069213970421, 15.15218985681980612 ) ) ;
#96812=CARTESIAN_POINT ( 'NONE',  ( 172.7371573690596449, 271.6299009131761864, 17.79590902495428040 ) ) ;
#96815=CARTESIAN_POINT ( 'NONE',  ( 161.8150574665248200, 250.3750943687383881, -13.25074899737357903 ) ) ;
#96816=CARTESIAN_POINT ( 'NONE',  ( 151.1237910559533475, 270.8929109891034841, -13.93008610078706688 ) ) ;
#96817=CARTESIAN_POINT ( 'NONE',  ( 149.0164813726494799, 272.5428784278667536, -11.67305721329070423 ) ) ;
#96819=CARTESIAN_POINT ( 'NONE',  ( 197.8822014719394531, 287.9049684674569676, 17.88172308374019792 ) ) ;
#96822=CARTESIAN_POINT ( 'NONE',  ( 198.0036776755666210, 286.8752984553728993, 16.94019974494662861 ) ) ;
#96823=CARTESIAN_POINT ( 'NONE',  ( 114.8152493078691947, 249.3464784336662206, 1.353441290958777525E-15 ) ) ;
#96824=CARTESIAN_POINT ( 'NONE',  ( 112.6775961898153184, 245.8615022471903160, 5.000000000000046185 ) ) ;
#96825=CARTESIAN_POINT ( 'NONE',  ( 27.64472685218281711, 196.7677522451419350, -5.000000000000047962 ) ) ;
#96827=CARTESIAN_POINT ( 'NONE',  ( 163.7587049410067266, 247.0085981909329576, -6.137518685179130351 ) ) ;
#96830=CARTESIAN_POINT ( 'NONE',  ( 159.5204760365350012, 254.3494259875849082, 16.90107507090185379 ) ) ;
#96832=CARTESIAN_POINT ( 'NONE',  ( 72.86731735994297310, 219.0024278399160949, -9.188101187500093303 ) ) ;
#96833=CARTESIAN_POINT ( 'NONE',  ( 172.1774115781176420, 284.2304136030405743, 13.05068545833847438 ) ) ;
#96834=CARTESIAN_POINT ( 'NONE',  ( 150.8888667059421209, 269.2998118992572927, 15.79021133717968617 ) ) ;
#96835=CARTESIAN_POINT ( 'NONE',  ( 193.8913555215501390, 294.8173164187117550, 15.40725395879721837 ) ) ;
#96836=CARTESIAN_POINT ( 'NONE',  ( -13.76211276271269668, 162.8615022471902591, -10.00000000000007816 ) ) ;
#96839=CARTESIAN_POINT ( 'NONE',  ( 203.4696564630250464, 278.2272125378923988, -16.38980782817167636 ) ) ;
#96842=CARTESIAN_POINT ( 'NONE',  ( 148.6255488361104540, 273.2199934434842703, 9.123621776406645623 ) ) ;
#96844=CARTESIAN_POINT ( 'NONE',  ( 163.9093945587947587, 260.4689496177562091, -16.17298052259348040 ) ) ;
#96845=CARTESIAN_POINT ( 'NONE',  ( 207.3589495855971450, 271.0586446502292119, 2.456771036675355457 ) ) ;
#96848=CARTESIAN_POINT ( 'NONE',  ( 206.3907062969896060, 273.1678058140250300, 11.56942460516550675 ) ) ;
#96849=EDGE_CURVE ( 'NONE', #28117, #100032, #58972, .T. ) ;
#96850=CARTESIAN_POINT ( 'NONE',  ( 206.5571822944673670, 272.8794609281530938, 10.95833005210827515 ) ) ;
#96855=CARTESIAN_POINT ( 'NONE',  ( 123.6384037525706958, 236.0643266524160140, 9.188101187500095079 ) ) ;
#96860=CARTESIAN_POINT ( 'NONE',  ( 172.2601350562971447, 284.0070134640075139, -13.26565049143300712 ) ) ;
#96864=EDGE_LOOP ( 'NONE', ( #75592, #20855, #25665, #31833 ) ) ;
#96868=CARTESIAN_POINT ( 'NONE',  ( 164.3284847670581144, 246.0217105830841433, -2.055838629128057704 ) ) ;
#96869=CARTESIAN_POINT ( 'NONE',  ( 139.4158702080621879, 260.4869531367911009, 4.594050593750046652 ) ) ;
#96871=CARTESIAN_POINT ( 'NONE',  ( 190.5653282632609091, 300.5781646174276602, -5.775635208185608604 ) ) ;
#96873=CARTESIAN_POINT ( 'NONE',  ( 157.0877926458200307, 258.5629572190321710, -17.40668770468195703 ) ) ;
#96874=CARTESIAN_POINT ( 'NONE',  ( 172.0768229479522518, 251.2702533327793049, 3.412387498982429879 ) ) ;
#96875=EDGE_CURVE ( 'NONE', #20065, #130, #17935, .T. ) ;
#96879=CARTESIAN_POINT ( 'NONE',  ( 155.4178462578491917, 279.7076410523796994, -1.474083510808620767 ) ) ;
#96880=CARTESIAN_POINT ( 'NONE',  ( 169.1881285547887899, 285.4409231072398256, -9.045257849526111116 ) ) ;
#96881=CARTESIAN_POINT ( 'NONE',  ( 163.7166294601506991, 282.3380383384618995, 10.03031969300557513 ) ) ;
#96882=CARTESIAN_POINT ( 'NONE',  ( 193.7377806475841737, 288.6157489428582039, 16.07307194723800947 ) ) ;
#96884=CARTESIAN_POINT ( 'NONE',  ( 134.1658515176688411, 248.2677522451418497, 10.00000000000009592 ) ) ;
#96885=CARTESIAN_POINT ( 'NONE',  ( 182.9478530203177797, 278.8618512465640720, 17.45115622927625409 ) ) ;
#96887=CARTESIAN_POINT ( 'NONE',  ( 157.7365441389748923, 257.4392866714015895, 18.13124212464487073 ) ) ;
#96888=CARTESIAN_POINT ( 'NONE',  ( 190.6036479972031259, 300.5117928913073797, -0.6824572005520307405 ) ) ;
#96889=CARTESIAN_POINT ( 'NONE',  ( -6.509410329615746171, 176.2369531367911293, -4.594050593750048428 ) ) ;
#96891=CARTESIAN_POINT ( 'NONE',  ( 42.47567221558909267, 186.1423013555410080, -4.594050593750043987 ) ) ;
#96892=CARTESIAN_POINT ( 'NONE',  ( 179.0685761320505947, 258.5468394390073286, -11.57600102548048149 ) ) ;
#96895=CARTESIAN_POINT ( 'NONE',  ( 205.2414727015710412, 275.1583367910551488, -12.71338796362297963 ) ) ;
#96896=CARTESIAN_POINT ( 'NONE',  ( 192.5408418301696827, 292.3122096881645575, -14.34927581417471032 ) ) ;
#96900=CARTESIAN_POINT ( 'NONE',  ( 170.2584372531675285, 258.0169095780440216, 13.81827105252718191 ) ) ;
#96902=CARTESIAN_POINT ( 'NONE',  ( 166.1251398123678769, 278.2158936690458972, 14.79076461835531831 ) ) ;
#96903=CARTESIAN_POINT ( 'NONE',  ( 162.1420711923595945, 252.0453937043351971, -13.78871268869485966 ) ) ;
#96905=CARTESIAN_POINT ( 'NONE',  ( 40.72531889205820477, 200.9865022471903160, -10.00000000000009415 ) ) ;
#96906=CARTESIAN_POINT ( 'NONE',  ( 182.3148671385995954, 291.9086626978152594, 9.339946855409639426 ) ) ;
#96907=CARTESIAN_POINT ( 'NONE',  ( 189.8147415777049218, 301.8782188922952514, -0.5019643756309712934 ) ) ;
#96908=CARTESIAN_POINT ( 'NONE',  ( -0.2035760843690503918, 176.8149278399160949, -9.188101187500095079 ) ) ;
#96909=CARTESIAN_POINT ( 'NONE',  ( 168.2775622310419976, 286.2832889018337141, 4.256419143223407531 ) ) ;
#96912=CARTESIAN_POINT ( 'NONE',  ( 164.9356397357043704, 244.9700873293209042, 2.799217332519396972 ) ) ;
#96914=CARTESIAN_POINT ( 'NONE',  ( 179.3501926571443335, 277.5838325412013887, 16.80239616393437885 ) ) ;
#96916=CARTESIAN_POINT ( 'NONE',  ( 193.7118145980225279, 295.1282904202991517, 14.61271143546694162 ) ) ;
#96917=CARTESIAN_POINT ( 'NONE',  ( 73.77862180316432728, 206.7365022471902023, 10.00000000000009948 ) ) ;
#96921=CARTESIAN_POINT ( 'NONE',  ( 165.6714170802892454, 285.4141558977842692, 0.4680648764968557973 ) ) ;
#96925=LINE ( 'NONE', #66471, #12810 ) ;
#96931=ORIENTED_EDGE ( 'NONE', *, *, #76717, .T. ) ;
#96932=DIRECTION ( 'NONE',  ( -0.8660254037844387076, -0.4999999999999998890, -0.000000000000000000 ) ) ;
#96933=CARTESIAN_POINT ( 'NONE',  ( 164.3138894970802824, 246.0469903322357368, -2.642126690130961020 ) ) ;
#96939=CARTESIAN_POINT ( 'NONE',  ( 165.2177353524737953, 246.3385600597696623, -4.395826225581572544 ) ) ;
#96941=CARTESIAN_POINT ( 'NONE',  ( 192.2431834237441706, 297.6720342317289578, 11.07782187406058938 ) ) ;
#96944=CARTESIAN_POINT ( 'NONE',  ( 176.9918222592760912, 263.5879201535869925, 14.48983262399754324 ) ) ;
#96945=ORIENTED_EDGE ( 'NONE', *, *, #72996, .F. ) ;
#96948=B_SPLINE_CURVE_WITH_KNOTS ( 'NONE', 3,
 ( #45459, #85003, #84511, #30777, #83515, #15055, #7981, #21680, #76863, #45946, #23154, #44460, #38352, #61658, #14076, #84022, #75392, #60151 ),
 .UNSPECIFIED., .F., .F.,
 ( 4, 2, 2, 2, 2, 2, 2, 2, 4 ),
 ( 0.003618221803335557821, 0.003736881880739065936, 0.003855541958142574051, 0.003974202035546082167, 0.004092862112949589848, 0.004330182267756606078, 0.004567502422563622308, 0.005516783041791769628, 0.007415344280248136258 ),
 .UNSPECIFIED. ) ;
#96950=CARTESIAN_POINT ( 'NONE',  ( 180.4139436811555299, 273.2462330171467215, 17.76112568380599654 ) ) ;
#96952=CARTESIAN_POINT ( 'NONE',  ( 203.0008710209992273, 267.9386651392713929, 2.532706327771747645 ) ) ;
#96953=CARTESIAN_POINT ( 'NONE',  ( 169.4554350835716150, 276.4675945671627915, -15.95358343529382950 ) ) ;
#96956=ORIENTED_EDGE ( 'NONE', *, *, #4337, .F. ) ;
#96957=CARTESIAN_POINT ( 'NONE',  ( 174.4395595858021579, 277.0650199303285035, -15.70439895477656123 ) ) ;
#96958=CARTESIAN_POINT ( 'NONE',  ( 170.3633989215723545, 262.4553760836484457, -15.63040615342705486 ) ) ;
#96960=FACE_OUTER_BOUND ( 'NONE', #90785, .T. ) ;
#96963=ORIENTED_EDGE ( 'NONE', *, *, #38847, .F. ) ;
#96965=CARTESIAN_POINT ( 'NONE',  ( 147.6079937265279511, 274.9824505927824134, 7.417156936634978770 ) ) ;
#96966=CARTESIAN_POINT ( 'NONE',  ( 188.9510948051018602, 298.8071002461200578, -4.271560164622560940 ) ) ;
#96968=CARTESIAN_POINT ( 'NONE',  ( 152.6656396574222754, 266.2223508737794759, 17.04346597795114349 ) ) ;
#96970=CARTESIAN_POINT ( 'NONE',  ( 28.76880349826970473, 198.9637435831425023, 2.679491924311251605 ) ) ;
#96971=CARTESIAN_POINT ( 'NONE',  ( 158.3286259501534232, 256.4137708922029333, -16.88280927543103616 ) ) ;
#96974=CARTESIAN_POINT ( 'NONE',  ( 206.5571822944673670, 272.8794609281530938, 10.95833005210827515 ) ) ;
#96975=CARTESIAN_POINT ( 'NONE',  ( 182.2991478702006134, 275.2734891516705034, -17.80812521087705846 ) ) ;
#96976=CARTESIAN_POINT ( 'NONE',  ( 159.9014600375868440, 253.6895423408921886, 15.57825579621527368 ) ) ;
#96977=ORIENTED_EDGE ( 'NONE', *, *, #63283, .F. ) ;
#96979=CARTESIAN_POINT ( 'NONE',  ( 147.3872053751516944, 275.3648672350856259, -2.900151178210554015 ) ) ;
#96980=CARTESIAN_POINT ( 'NONE',  ( 196.2350291401047571, 264.4780031501763347, 5.359379669934941859 ) ) ;
#96981=CARTESIAN_POINT ( 'NONE',  ( 163.5475621151755661, 247.8473668945463828, 8.020086546505606151 ) ) ;
#96983=CARTESIAN_POINT ( 'NONE',  ( 199.0447321067873361, 285.8914063425450536, -17.01815350566629448 ) ) ;
#96986=CARTESIAN_POINT ( 'NONE',  ( 167.2496274829885294, 252.8828136207999648, -12.23857971285498181 ) ) ;
#96989=AXIS2_PLACEMENT_3D ( 'NONE', #11189, #42056, #50648 ) ;
#96990=CARTESIAN_POINT ( 'NONE',  ( 206.8986117509267899, 272.2880877623646825, 6.975890063856878598 ) ) ;
#96991=CARTESIAN_POINT ( 'NONE',  ( 25.47966334272171807, 195.5177522451419350, 5.000000000000046185 ) ) ;
#96992=CARTESIAN_POINT ( 'NONE',  ( 111.1892885731693923, 228.8768266524159856, -9.188101187500093303 ) ) ;
#96994=CARTESIAN_POINT ( 'NONE',  ( 182.6307980359219982, 295.3544251836937065, -2.669455251163955101 ) ) ;
#96996=CARTESIAN_POINT ( 'NONE',  ( 162.7915066255068837, 249.6040781700690161, -11.20594800013087067 ) ) ;
#96999=CARTESIAN_POINT ( 'NONE',  ( 17.82075117977708700, 181.0958772461660544, -9.188101187500095079 ) ) ;
#97004=CARTESIAN_POINT ( 'NONE',  ( 147.4751173256875632, 275.5971820653270470, -0.1352375326296694491 ) ) ;
#97005=ADVANCED_FACE ( 'NONE', ( #78717 ), #87388, .T. ) ;
#97008=CARTESIAN_POINT ( 'NONE',  ( 193.3043481395981189, 264.0380534965367474, -4.339446791620638955 ) ) ;
#97010=CARTESIAN_POINT ( 'NONE',  ( 185.1858115004773140, 285.9426224659952140, 15.27411408704069729 ) ) ;
#97012=CARTESIAN_POINT ( 'NONE',  ( 46.20988612576196175, 206.6744531367911009, 4.594050593750047540 ) ) ;
#97013=CARTESIAN_POINT ( 'NONE',  ( 93.82350145804367969, 231.6427522451419065, -10.00000000000009415 ) ) ;
#97014=EDGE_LOOP ( 'NONE', ( #10185, #41550, #55014, #2029, #88398 ) ) ;
#97016=CARTESIAN_POINT ( 'NONE',  ( 181.6949246677837664, 260.6778951557793675, -10.47883949846568541 ) ) ;
#97018=CARTESIAN_POINT ( 'NONE',  ( -5.751638101304356709, 176.6744531367911293, 4.594050593750047540 ) ) ;
#97020=CARTESIAN_POINT ( 'NONE',  ( 199.1867231605587278, 285.6454706231928071, -17.41989184023605475 ) ) ;
#97022=CARTESIAN_POINT ( 'NONE',  ( 146.8312060062178830, 276.3278863910550172, -4.807241325481028227 ) ) ;
#97026=CARTESIAN_POINT ( 'NONE',  ( 164.5867587387928950, 245.5743669417666126, -3.022048486790635202 ) ) ;
#97027=ORIENTED_EDGE ( 'NONE', *, *, #28507, .T. ) ;
#97028=EDGE_CURVE ( 'NONE', #90758, #74996, #32123, .T. ) ;
#97029=CARTESIAN_POINT ( 'NONE',  ( -0.6995629222973920314, 163.7365022471902023, -10.00000000000009059 ) ) ;
#97031=CARTESIAN_POINT ( 'NONE',  ( 118.9560200436548314, 248.6744531367911293, 4.594050593750047540 ) ) ;
#97033=CARTESIAN_POINT ( 'NONE',  ( 186.3061762155872714, 258.1895346003614122, -3.525132546332560235 ) ) ;
#97037=EDGE_CURVE ( 'NONE', #91958, #7762, #49323, .T. ) ;
#97040=CARTESIAN_POINT ( 'NONE',  ( 157.3305006125302441, 282.1378183958786963, 1.589776369934247979 ) ) ;
#97041=CARTESIAN_POINT ( 'NONE',  ( 207.7670811201955701, 270.7838546899739640, -1.661274253000708079 ) ) ;
#97043=CARTESIAN_POINT ( 'NONE',  ( 172.8310867690399846, 268.0400968755592430, -16.30299140802141267 ) ) ;
#97051=CYLINDRICAL_SURFACE ( 'NONE', #70406, 10.00000000000010658 ) ;
#97054=CARTESIAN_POINT ( 'NONE',  ( 156.0045539464697981, 278.3546514767295434, -9.412258334191998088 ) ) ;
#97056=CARTESIAN_POINT ( 'NONE',  ( 124.2269133023872882, 230.9824982072973683, 3.021315404115420679E-15 ) ) ;
#97057=ORIENTED_EDGE ( 'NONE', *, *, #33240, .T. ) ;
#97059=CARTESIAN_POINT ( 'NONE',  ( 194.8432095198904221, 293.1686569321988145, -14.74101036184996616 ) ) ;
#97064=CARTESIAN_POINT ( 'NONE',  ( 184.7894305693181138, 292.1317680087225881, 12.52679022050396895 ) ) ;
#97065=CARTESIAN_POINT ( 'NONE',  ( -22.42236680055709641, 157.8615022471902591, 0.000000000000000000 ) ) ;
#97067=CARTESIAN_POINT ( 'NONE',  ( 91.05385083941617097, 229.5024278399160949, -9.188101187500093303 ) ) ;
#97080=CARTESIAN_POINT ( 'NONE',  ( 203.2732885619977026, 278.5673317194472247, -16.64305493556850024 ) ) ;
#97087=CARTESIAN_POINT ( 'NONE',  ( 157.4702324156611155, 281.8845292153815194, 2.929819485995689199 ) ) ;
#97088=CARTESIAN_POINT ( 'NONE',  ( 133.7867050834633460, 257.2369531367911009, -4.594050593750048428 ) ) ;
#97089=CARTESIAN_POINT ( 'NONE',  ( 157.1606728774482065, 258.4367249549846974, -18.41782236529479633 ) ) ;
#97095=CARTESIAN_POINT ( 'NONE',  ( 164.1096337185929315, 281.6968895742988934, 8.720925588203845891 ) ) ;
#97096=CARTESIAN_POINT ( 'NONE',  ( 203.7752293336776006, 271.7063540172214857, 9.638331677649306428 ) ) ;
#97098=CARTESIAN_POINT ( 'NONE',  ( 167.0546803224166297, 282.1702852132879684, 12.27869116404093752 ) ) ;
#97099=CARTESIAN_POINT ( 'NONE',  ( 181.3784564040530256, 255.2489373100174532, 0.6922490234118574559 ) ) ;
#97102=CARTESIAN_POINT ( 'NONE',  ( 156.5207620954022616, 279.5661031660920912, 7.531452285229264021 ) ) ;
#97103=CARTESIAN_POINT ( 'NONE',  ( 165.5301935577539609, 246.9158322381169057, -2.041142469049267660 ) ) ;
#97104=CARTESIAN_POINT ( 'NONE',  ( 194.3452430042056847, 293.4673175397701357, -14.50972866970454866 ) ) ;
#97108=CARTESIAN_POINT ( 'NONE',  ( 184.8382098728736480, 273.0595371315191073, -16.47964124523516460 ) ) ;
#97110=ORIENTED_EDGE ( 'NONE', *, *, #89795, .F. ) ;
#97111=CARTESIAN_POINT ( 'NONE',  ( 160.6282313088876492, 275.7627601117830523, 12.77581587744434088 ) ) ;
#97112=EDGE_CURVE ( 'NONE', #48299, #24507, #3410, .T. ) ;
#97113=CARTESIAN_POINT ( 'NONE',  ( 156.2170492467576821, 277.6398520454177969, 10.26798254968793600 ) ) ;
#97114=CARTESIAN_POINT ( 'NONE',  ( 175.3074307085254020, 254.5436327766159650, 9.407465564047683415 ) ) ;
#97116=CARTESIAN_POINT ( 'NONE',  ( 161.7595754908867605, 272.9535027612637350, 15.05830031582055817 ) ) ;
#97117=CARTESIAN_POINT ( 'NONE',  ( 159.1812762191934212, 274.8495840587517023, 14.39428968362149241 ) ) ;
#97119=CARTESIAN_POINT ( 'NONE',  ( 162.8839417982861448, 263.3994626277539055, 17.77684832337497767 ) ) ;
#97121=ORIENTED_EDGE ( 'NONE', *, *, #36803, .T. ) ;
#97126=B_SPLINE_CURVE_WITH_KNOTS ( 'NONE', 3,
 ( #61229, #45033, #75977, #17002, #44526, #22237, #21255, #63110, #99755, #53138, #45526, #98264, #78833, #15121, #22747, #76931, #28853, #52134, #83084, #13654, #75458, #6042, #18528, #11442, #3820, #49912, #40791, #80358, #57498, #27126, #50403, #9929, #48416, #42295, #41295, #19040, #10422, #88988, #81358, #95576, #87980, #88478, #79365, #71737, #11928, #73228 ),
 .UNSPECIFIED., .F., .F.,
 ( 4, 2, 2, 2, 2, 2, 2, 2, 2, 2, 2, 2, 2, 2, 2, 2, 2, 2, 2, 2, 2, 2, 4 ),
 ( 0.0002912000113238576810, 0.001310581117245713037, 0.001820271670206675789, 0.002075116946687189257, 0.002202539584927487408, 0.002329962223167785559, 0.002457384861408083276, 0.002584807499648380993, 0.002839652776129052321, 0.003349343329090460463, 0.004368724435013277181, 0.005388105540936094333, 0.005897796093897495970, 0.006152641370378155589, 0.006407486646858814340, 0.006471197965978995291, 0.006534909285099176242, 0.006598620604219358060, 0.006662331923339539011, 0.006917177199820049444, 0.007426867752781065105, 0.007936558305742080766, 0.008446248858703096427 ),
 .UNSPECIFIED. ) ;
#97128=CARTESIAN_POINT ( 'NONE',  ( 192.8010417052266234, 296.7057953447782097, 12.10593424093686643 ) ) ;
#97131=CARTESIAN_POINT ( 'NONE',  ( 157.9225728654248257, 276.1116997103654285, -12.95724163227552239 ) ) ;
#97132=CARTESIAN_POINT ( 'NONE',  ( 9.810363290536042058, 164.2202760586659451, -5.415160957724236172E-17 ) ) ;
#97133=CARTESIAN_POINT ( 'NONE',  ( 100.7969837277561282, 222.8768266524159856, -9.188101187500091527 ) ) ;
#97135=CARTESIAN_POINT ( 'NONE',  ( 183.0033326268229246, 294.1337744772658880, -7.888237667023935806 ) ) ;
#97136=CARTESIAN_POINT ( 'NONE',  ( -17.42236680055705023, 149.2012482093457777, 0.000000000000000000 ) ) ;
#97137=CARTESIAN_POINT ( 'NONE',  ( 194.4556067646799420, 282.9884635700969397, 17.82090350285937319 ) ) ;
#97138=CARTESIAN_POINT ( 'NONE',  ( 0.07393976959879319799, 182.3967562850347406, 2.649461200531984646E-14 ) ) ;
#97139=CARTESIAN_POINT ( 'NONE',  ( 148.4083960970861256, 273.5961130204771052, -8.574185186226726429 ) ) ;
#97141=CARTESIAN_POINT ( 'NONE',  ( 86.83321340830613622, 209.3932355074535678, -2.679491924311248496 ) ) ;
#97142=CARTESIAN_POINT ( 'NONE',  ( -27.42236680055714260, 166.5217562850347406, 1.224646799147364892E-15 ) ) ;
#97147=CARTESIAN_POINT ( 'NONE',  ( 79.47110815956433783, 210.5643266524160424, 9.188101187500095079 ) ) ;
#97148=CARTESIAN_POINT ( 'NONE',  ( 161.1492466472929266, 251.5283125358769212, -13.33353587056634915 ) ) ;
#97149=CARTESIAN_POINT ( 'NONE',  ( 163.4266023455967911, 257.9436588619666963, 15.59867604562648324 ) ) ;
#97150=CARTESIAN_POINT ( 'NONE',  ( 157.3988263959001870, 258.0242309610243865, 16.72376558639979294 ) ) ;
#97153=CARTESIAN_POINT ( 'NONE',  ( 203.9080669571095257, 275.9035274530119182, -13.79279311472316394 ) ) ;
#97156=CARTESIAN_POINT ( 'NONE',  ( 79.15288444911743682, 228.0530062829863027, -4.648177544792955347E-16 ) ) ;
#97161=CARTESIAN_POINT ( 'NONE',  ( 191.2622316156482043, 288.8574828335728171, -16.55244734589887656 ) ) ;
#97163=CARTESIAN_POINT ( 'NONE',  ( 153.6845034812979804, 266.9389077895647802, 16.46468584801201374 ) ) ;
#97165=CARTESIAN_POINT ( 'NONE',  ( 140.3182403272686543, 258.4865022471902876, 10.00000000000009237 ) ) ;
#97166=CARTESIAN_POINT ( 'NONE',  ( 205.3708847852691406, 274.9341884869767227, -13.70973585089674174 ) ) ;
#97167=B_SPLINE_CURVE_WITH_KNOTS ( 'NONE', 3,
 ( #87582, #33297, #41892, #79447 ),
 .UNSPECIFIED., .F., .F.,
 ( 4, 4 ),
 ( 0.01508109614910603871, 0.02383471597684285251 ),
 .UNSPECIFIED. ) ;
#97169=VERTEX_POINT ( 'NONE', #42430 ) ;
#97171=ORIENTED_EDGE ( 'NONE', *, *, #50036, .F. ) ;
#97174=ORIENTED_EDGE ( 'NONE', *, *, #7512, .T. ) ;
#97178=CARTESIAN_POINT ( 'NONE',  ( 205.9050707304272407, 274.0089512892737389, 12.32231322111777772 ) ) ;
#97179=CARTESIAN_POINT ( 'NONE',  ( 158.2778382039339533, 257.5751017963053187, -16.89175558457479198 ) ) ;
#97180=CARTESIAN_POINT ( 'NONE',  ( 204.0490764393590553, 272.8272845076828617, 11.09290516031127005 ) ) ;
#97181=CARTESIAN_POINT ( 'NONE',  ( 201.1388841337167435, 282.2642286331299601, -18.17233400608081340 ) ) ;
#97184=DIRECTION ( 'NONE',  ( -0.8660254037844387076, -0.4999999999999998890, -0.000000000000000000 ) ) ;
#97185=CARTESIAN_POINT ( 'NONE',  ( 165.0963061027407832, 274.7047549202629284, 14.74588534425331332 ) ) ;
#97186=CARTESIAN_POINT ( 'NONE',  ( 167.5469267500292574, 266.7168544022062520, -17.80679023418265672 ) ) ;
#97191=CARTESIAN_POINT ( 'NONE',  ( 147.7467138384290308, 274.7421803109381813, -9.190172068879620682 ) ) ;
#97193=CARTESIAN_POINT ( 'NONE',  ( 164.7364331287320738, 247.3151232938002693, -7.618980141130590411 ) ) ;
#97194=CARTESIAN_POINT ( 'NONE',  ( 147.4749560789897771, 275.5966042365595854, 0.1362648926203907929 ) ) ;
#97196=CARTESIAN_POINT ( 'NONE',  ( 170.8905786597765086, 288.0411465072718329, -4.155906328687864359 ) ) ;
#97197=CARTESIAN_POINT ( 'NONE',  ( 169.7144176936253359, 267.3710074754821449, 17.44705272466886115 ) ) ;
#97198=CARTESIAN_POINT ( 'NONE',  ( 181.6012535417948186, 256.1925639173799709, 5.230076733189143567 ) ) ;
#97199=CARTESIAN_POINT ( 'NONE',  ( 93.70588009062352342, 237.1589784336661637, -6.496448406907675876E-16 ) ) ;
#97200=B_SPLINE_CURVE_WITH_KNOTS ( 'NONE', 3,
 ( #40714, #41717, #72662, #34140, #41210, #25535, #1233, #55402, #55898, #85898, #16423, #9332, #56423, #9854, #71657, #33128, #17947, #71150 ),
 .UNSPECIFIED., .F., .F.,
 ( 4, 2, 2, 2, 2, 2, 2, 2, 4 ),
 ( 2.819365433277861356E-15, 0.0003786859679666404054, 0.0007573719359304614514, 0.001136057903894282552, 0.001514743871858103543, 0.001893429839821924535, 0.002272115807785745744, 0.002650801775749566519, 0.003029487743713387728 ),
 .UNSPECIFIED. ) ;
#97204=CARTESIAN_POINT ( 'NONE',  ( 112.0100349375168918, 242.1427522451419065, -10.00000000000009592 ) ) ;
#97205=ORIENTED_EDGE ( 'NONE', *, *, #73528, .F. ) ;
#97207=DIRECTION ( 'NONE',  ( 0.4999999999999998890, -0.8660254037844385966, 0.000000000000000000 ) ) ;
#97209=CARTESIAN_POINT ( 'NONE',  ( 164.5512980253735122, 249.3551712322193055, 9.899787939062008491 ) ) ;
#97210=CARTESIAN_POINT ( 'NONE',  ( 159.4491226731523454, 254.4730136382542582, -15.39140229921534520 ) ) ;
#97211=CARTESIAN_POINT ( 'NONE',  ( 189.3399741911424314, 300.7005401275983445, 2.182451016153226694E-15 ) ) ;
#97214=VERTEX_POINT ( 'NONE', #41950 ) ;
#97215=CARTESIAN_POINT ( 'NONE',  ( 162.6262389125959373, 248.9700868899859074, -10.50380342094597808 ) ) ;
#97217=CARTESIAN_POINT ( 'NONE',  ( 148.7305541605275607, 275.0381188865328568, -8.045727261058747359 ) ) ;
#97218=CARTESIAN_POINT ( 'NONE',  ( 15.61058218230948036, 186.4865022471903160, 10.00000000000009415 ) ) ;
#97220=CARTESIAN_POINT ( 'NONE',  ( 124.5040820605901217, 248.8149278399161233, -9.188101187500095079 ) ) ;
#97221=CARTESIAN_POINT ( 'NONE',  ( 199.3488497299964024, 284.5376415457495796, 17.19460419984376287 ) ) ;
#97222=CARTESIAN_POINT ( 'NONE',  ( 182.5686778644665083, 296.6873302901632314, 1.787712280751329708 ) ) ;
#97223=EDGE_LOOP ( 'NONE', ( #25575, #87117, #25797, #38845 ) ) ;
#97224=CARTESIAN_POINT ( 'NONE',  ( 204.5482460332032986, 276.3590406018296903, 14.63243279326650814 ) ) ;
#97225=CARTESIAN_POINT ( 'NONE',  ( 63.21847669855743135, 195.7592609112380160, 2.679491924311254714 ) ) ;
#97227=CARTESIAN_POINT ( 'NONE',  ( 192.3159699081281815, 271.9052417175213918, 14.14648652338713397 ) ) ;
#97228=CARTESIAN_POINT ( 'NONE',  ( 178.5440531547785952, 285.2457182098279986, 13.27232952186126802 ) ) ;
#97229=EDGE_CURVE ( 'NONE', #47888, #20349, #72308, .T. ) ;
#97231=CYLINDRICAL_SURFACE ( 'NONE', #8144, 10.00000000000010658 ) ;
#97232=EDGE_CURVE ( 'NONE', #77581, #26850, #84337, .T. ) ;
#97235=EDGE_CURVE ( 'NONE', #51575, #3137, #2136, .T. ) ;
#97236=CARTESIAN_POINT ( 'NONE',  ( 167.7939926630123182, 249.6251980485383513, 7.973689277210887383 ) ) ;
#97238=CARTESIAN_POINT ( 'NONE',  ( 207.6523394534040392, 270.9825930866021508, -2.115019688068903392 ) ) ;
#97245=FACE_OUTER_BOUND ( 'NONE', #13182, .T. ) ;
#97247=CARTESIAN_POINT ( 'NONE',  ( 157.7483529369466737, 270.6632484235471452, -15.17384122213293729 ) ) ;
#97249=CARTESIAN_POINT ( 'NONE',  ( 207.2707369601997982, 271.6435479931266173, -5.381413637561199614 ) ) ;
#97250=( BOUNDED_CURVE ( )  B_SPLINE_CURVE ( 2, ( #27865, #28870, #59746, #75474, #52149, #12689, #37440, #90208, #45050 ),
 .UNSPECIFIED., .F., .F. ) 
 B_SPLINE_CURVE_WITH_KNOTS ( ( 3, 2, 2, 2, 3 ),
 ( 0.4314516129032258118, 0.4327956989247311870, 0.4354838709677419373, 0.4381720430107526876, 0.4395161290322580627 ),
 .UNSPECIFIED. ) 
 CURVE ( )  GEOMETRIC_REPRESENTATION_ITEM ( )  RATIONAL_B_SPLINE_CURVE ( ( 0.9330127018922194093, 0.9330127018922194093, 1.000000000000000000, 0.8660254037844387076, 1.000000000000000000, 0.8660254037844387076, 1.000000000000000000, 0.9330127018922194093, 0.9330127018922194093 ) ) 
 REPRESENTATION_ITEM ( '' )  );
#97251=CARTESIAN_POINT ( 'NONE',  ( 16.06189740016370848, 170.8923013555409796, 4.594050593750050204 ) ) ;
#97252=CARTESIAN_POINT ( 'NONE',  ( 207.3589495855971450, 271.0586446502292119, 2.456771036675355457 ) ) ;
#97253=ORIENTED_EDGE ( 'NONE', *, *, #75168, .F. ) ;
#97256=CARTESIAN_POINT ( 'NONE',  ( 42.50247518763358556, 195.3458772461660544, 9.188101187500095079 ) ) ;
#97258=CARTESIAN_POINT ( 'NONE',  ( 199.1216527653377000, 285.7581758537840528, -18.37739894744384728 ) ) ;
#97259=CARTESIAN_POINT ( 'NONE',  ( 147.0538900202505488, 275.9421863647172017, 5.192507380313251986 ) ) ;
#97261=CARTESIAN_POINT ( 'NONE',  ( 173.3264126386846726, 289.1951097772950448, -8.140207440225699642 ) ) ;
#97262=CARTESIAN_POINT ( 'NONE',  ( 178.5991144655399410, 293.9124374319637809, 2.724545304837039605 ) ) ;
#97263=CARTESIAN_POINT ( 'NONE',  ( 198.2489255580726422, 287.2697837179150042, 18.53597557040773225 ) ) ;
#97264=CARTESIAN_POINT ( 'NONE',  ( 180.1848004237850205, 278.8644883139655235, -16.25315175759617148 ) ) ;
#97266=CARTESIAN_POINT ( 'NONE',  ( 166.9153220475343460, 257.9520600803688239, -15.27885173810403785 ) ) ;
#97268=CARTESIAN_POINT ( 'NONE',  ( 99.25420243115659957, 218.1115022471901739, -5.000000000000041744 ) ) ;
#97269=CARTESIAN_POINT ( 'NONE',  ( 10.41442975960284834, 183.4865022471903160, 10.00000000000009415 ) ) ;
#97270=CARTESIAN_POINT ( 'NONE',  ( 161.6733100514768466, 267.8128507344575837, -17.34687799797600860 ) ) ;
#97271=ORIENTED_EDGE ( 'NONE', *, *, #31318, .T. ) ;
#97272=CARTESIAN_POINT ( 'NONE',  ( 63.28708487846012076, 207.3458772461660544, 9.188101187500095079 ) ) ;
#97273=EDGE_LOOP ( 'NONE', ( #63389, #82021, #69707, #79366 ) ) ;
#97275=CARTESIAN_POINT ( 'NONE',  ( 161.7836053227420905, 250.9551966261522296, 12.65126904800779606 ) ) ;
#97278=CARTESIAN_POINT ( 'NONE',  ( 170.8453059873319830, 287.4268083147989614, 8.562683323710214012 ) ) ;
#97279=CARTESIAN_POINT ( 'NONE',  ( 207.0200405408487541, 272.0777669287182334, 6.494273599193515878 ) ) ;
#97282=CARTESIAN_POINT ( 'NONE',  ( 189.0171803163284494, 265.5415642084109891, 10.72429650996405215 ) ) ;
#97284=EDGE_CURVE ( 'NONE', #4619, #79225, #83263, .T. ) ;
#97286=VERTEX_POINT ( 'NONE', #98168 ) ;
#97289=CARTESIAN_POINT ( 'NONE',  ( 16.11576366785039127, 190.1115022471903160, -5.000000000000047962 ) ) ;
#97290=CARTESIAN_POINT ( 'NONE',  ( 5.386117596089862403, 185.4637435831425023, 2.679491924311251605 ) ) ;
#97293=CARTESIAN_POINT ( 'NONE',  ( 150.6571681785161445, 269.7011255207979730, 15.24894850018880454 ) ) ;
#97294=CYLINDRICAL_SURFACE ( 'NONE', #51231, 17.82106496071139645 ) ;
#97297=CARTESIAN_POINT ( 'NONE',  ( 207.2683629543511756, 271.6476598918739001, -6.694388351944108528 ) ) ;
#97301=CARTESIAN_POINT ( 'NONE',  ( 197.9002057575219453, 287.8737841300738296, 18.01270164875645818 ) ) ;
#97305=CARTESIAN_POINT ( 'NONE',  ( 116.8724067376222706, 238.2833772461660544, -9.188101187500095079 ) ) ;
#97306=CARTESIAN_POINT ( 'NONE',  ( 190.9907605556751093, 299.8412942717858414, 8.799173206188184437 ) ) ;
#97307=CARTESIAN_POINT ( 'NONE',  ( 31.54184116921283376, 189.0177522451418497, -10.00000000000009592 ) ) ;
#97308=ORIENTED_EDGE ( 'NONE', *, *, #54175, .F. ) ;
#97309=CARTESIAN_POINT ( 'NONE',  ( 208.2764314485352770, 269.9016340424377063, 2.433736665191914117 ) ) ;
#97310=ORIENTED_EDGE ( 'NONE', *, *, #3400, .T. ) ;
#97311=ORIENTED_EDGE ( 'NONE', *, *, #73436, .F. ) ;
#97313=CARTESIAN_POINT ( 'NONE',  ( 162.7006039569504594, 261.3497057169571463, 17.57720365097131676 ) ) ;
#97314=CARTESIAN_POINT ( 'NONE',  ( 75.14098114064213974, 208.0643266524159856, -9.188101187500093303 ) ) ;
#97317=CARTESIAN_POINT ( 'NONE',  ( 198.6701036545953230, 286.5402818557027445, 17.25253558010639310 ) ) ;
#97318=CARTESIAN_POINT ( 'NONE',  ( 175.8184439186038048, 278.1148561126908021, 16.51363926675430349 ) ) ;
#97320=CARTESIAN_POINT ( 'NONE',  ( 113.3812418268422562, 246.2677522451419065, -5.000000000000047962 ) ) ;
#97325=CARTESIAN_POINT ( 'NONE',  ( 206.4719461165055066, 270.6153493572695083, 2.407488219507921912 ) ) ;
#97326=CARTESIAN_POINT ( 'NONE',  ( 200.3687477146384310, 283.1577567649229650, -16.79529056473667126 ) ) ;
#97328=CARTESIAN_POINT ( 'NONE',  ( 196.3174919959537306, 290.6151247789487684, -17.61248417473235151 ) ) ;
#97329=CARTESIAN_POINT ( 'NONE',  ( 206.2456893945931142, 273.4189824569319285, 10.13882547285618152 ) ) ;
#97331=CARTESIAN_POINT ( 'NONE',  ( 164.3053959849042087, 246.0617015268593661, -7.251939739328854273 ) ) ;
#97332=CARTESIAN_POINT ( 'NONE',  ( 117.4133255192225391, 250.8464784336661353, 1.353441290958777327E-15 ) ) ;
#97334=CARTESIAN_POINT ( 'NONE',  ( 191.0481192767711036, 299.7419460525905492, -9.103377665618040737 ) ) ;
#97335=CARTESIAN_POINT ( 'NONE',  ( 184.4251457649926067, 259.7825290899927495, 6.334789828098508657 ) ) ;
#97337=CARTESIAN_POINT ( 'NONE',  ( 199.5442653985851962, 283.0261893010793415, -17.63221794778640117 ) ) ;
#97338=CARTESIAN_POINT ( 'NONE',  ( 204.2799274532736433, 276.8237820148827950, 13.55359442435934803 ) ) ;
#97341=DIRECTION ( 'NONE',  ( -0.8660254037844387076, -0.4999999999999998890, -0.000000000000000000 ) ) ;
#97345=B_SPLINE_CURVE_WITH_KNOTS ( 'NONE', 3,
 ( #91244, #60286, #60779, #58796, #98836, #76040, #97839, #67409, #27914, #74546, #90266, #90771, #21321, #13239, #52199, #28408, #67916, #5125, #59288, #20839, #89765, #83148, #29417, #21809, #91743, #52694, #83656, #22307, #53208, #84161, #74037, #4626, #35518, #20334, #51205, #85666, #86169, #7603, #69895, #9108, #54179, #16205, #99821, #507, #38990, #47097, #45592, #7102, #1524, #22809, #19, #16703 ),
 .UNSPECIFIED., .F., .F.,
 ( 4, 2, 2, 2, 2, 2, 2, 2, 2, 2, 2, 2, 2, 2, 2, 2, 2, 2, 2, 2, 2, 2, 2, 2, 2, 4 ),
 ( 0.0007713298675087345126, 0.0009758712993485446586, 0.001078142015268449732, 0.001180412731188354696, 0.001282683447108259878, 0.001384954163028164842, 0.001589495594868055653, 0.001998578458547837274, 0.002407661322227618896, 0.003225827049587262369, 0.004043992776946906710, 0.004862158504306550617, 0.005271241367986409000, 0.005475782799826377223, 0.005578053515746398197, 0.005629188873706406950, 0.005680324231666414835, 0.005731459589626423587, 0.005782594947586431472, 0.005884865663506446375, 0.006089407095346483986, 0.006293948527186521598, 0.006498489959026559210, 0.006703031390866596821, 0.006907572822706634433, 0.007316655686386753024 ),
 .UNSPECIFIED. ) ;
#97346=LINE ( 'NONE', #90264, #72179 ) ;
#97347=CARTESIAN_POINT ( 'NONE',  ( 164.3448606421738702, 245.9933467353647814, -1.273739175181084260 ) ) ;
#97351=CARTESIAN_POINT ( 'NONE',  ( 146.8358616138309571, 276.3198226421291679, 4.054088818585255716 ) ) ;
#97353=CARTESIAN_POINT ( 'NONE',  ( 157.1458804504438831, 258.4623461901232417, -17.08829597948888335 ) ) ;
#97354=CARTESIAN_POINT ( 'NONE',  ( 171.0793476467304970, 250.7099474803164298, 3.411557086744808398 ) ) ;
#97356=CARTESIAN_POINT ( 'NONE',  ( 190.0274641710971082, 301.5097725526222803, 3.738976720635653450 ) ) ;
#97357=DIRECTION ( 'NONE',  ( 0.4999999999999992784, -0.8660254037844390407, 0.000000000000000000 ) ) ;
#97359=CARTESIAN_POINT ( 'NONE',  ( 197.8822014719394531, 287.9049684674569676, 17.88172308374019792 ) ) ;
#97360=CARTESIAN_POINT ( 'NONE',  ( 157.5034794998415180, 271.0532920065124358, -14.68140584649887614 ) ) ;
#97361=CARTESIAN_POINT ( 'NONE',  ( 134.1658515176688411, 238.2677522451417929, -5.000000000000041744 ) ) ;
#97362=CARTESIAN_POINT ( 'NONE',  ( 175.7752474544214465, 285.2040480104212179, -12.03434417915003607 ) ) ;
#97363=ORIENTED_EDGE ( 'NONE', *, *, #35562, .T. ) ;
#97364=CARTESIAN_POINT ( 'NONE',  ( 157.3363371328520088, 258.1324655395517311, 18.24585617226787093 ) ) ;
#97365=CARTESIAN_POINT ( 'NONE',  ( 198.9369963555428740, 286.0780101374919013, -18.58432392708837710 ) ) ;
#97366=B_SPLINE_CURVE_WITH_KNOTS ( 'NONE', 3,
 ( #88703, #50139, #41529, #81092 ),
 .UNSPECIFIED., .F., .F.,
 ( 4, 4 ),
 ( 0.01180967855186642636, 0.01789565966245129647 ),
 .UNSPECIFIED. ) ;
#97367=CARTESIAN_POINT ( 'NONE',  ( -3.478321416370212305, 177.9869531367911293, 4.594050593750046652 ) ) ;
#97368=B_SPLINE_CURVE_WITH_KNOTS ( 'NONE', 3,
 ( #6444, #100151, #17400, #83474 ),
 .UNSPECIFIED., .F., .F.,
 ( 4, 4 ),
 ( 0.005778719348092632713, 0.01383577470342770011 ),
 .UNSPECIFIED. ) ;
#97369=CARTESIAN_POINT ( 'NONE',  ( 61.01376819352597636, 206.0333772461660544, 9.188101187500095079 ) ) ;
#97373=CARTESIAN_POINT ( 'NONE',  ( 157.8811243250769110, 257.1888664433053009, -17.39256699147873064 ) ) ;
#97374=CARTESIAN_POINT ( 'NONE',  ( 189.4518811391805855, 290.6466329671102926, -14.51581993625191025 ) ) ;
#97376=CARTESIAN_POINT ( 'NONE',  ( 168.2274955120613811, 256.9427370946946780, 13.69819450224870572 ) ) ;
#97377=CARTESIAN_POINT ( 'NONE',  ( 179.3779096336606642, 254.7328586665793466, -4.090843683719358026 ) ) ;
#97378=CARTESIAN_POINT ( 'NONE',  ( 150.5355989389948093, 269.9116896202863245, 15.28294032643914768 ) ) ;
#97379=CARTESIAN_POINT ( 'NONE',  ( 36.90037335867692292, 202.1115022471903160, -5.000000000000047962 ) ) ;
#97380=CARTESIAN_POINT ( 'NONE',  ( 181.1156277128715431, 292.7914473640799997, 9.490545386343454126 ) ) ;
#97381=CARTESIAN_POINT ( 'NONE',  ( 147.6300909839706321, 274.9441770201837585, 8.328755691084779755 ) ) ;
#97382=CARTESIAN_POINT ( 'NONE',  ( 10.97399815293012892, 167.9548013555409796, -4.594050593750042211 ) ) ;
#97387=CARTESIAN_POINT ( 'NONE',  ( 206.9676408587583296, 272.1685258403992975, 7.544050792475608169 ) ) ;
#97388=CARTESIAN_POINT ( 'NONE',  ( 193.9204722154232741, 294.7668848255750049, 15.43855698596013859 ) ) ;
#97390=CARTESIAN_POINT ( 'NONE',  ( 176.7575342647435832, 260.2821926596799926, -13.68860621714789083 ) ) ;
#97398=CARTESIAN_POINT ( 'NONE',  ( 154.4564265542881287, 275.3778590288120540, 10.40416966185339653 ) ) ;
#97402=CARTESIAN_POINT ( 'NONE',  ( 153.4289928607825573, 264.9001843414388873, 17.27358709529985958 ) ) ;
#97405=CARTESIAN_POINT ( 'NONE',  ( 155.1601726304954809, 261.9016930232608615, -18.56587418422714464 ) ) ;
#97408=B_SPLINE_CURVE_WITH_KNOTS ( 'NONE', 3,
 ( #11041, #57105, #41918, #86094, #16618, #47514, #39895 ),
 .UNSPECIFIED., .F., .F.,
 ( 4, 3, 4 ),
 ( 0.000000000000000000, 0.001498044977021790319, 0.001501190957620832577 ),
 .UNSPECIFIED. ) ;
#97409=CARTESIAN_POINT ( 'NONE',  ( 159.1615944546315689, 279.6649321670822133, -9.874806447338704274 ) ) ;
#97410=CARTESIAN_POINT ( 'NONE',  ( 163.8040269124969939, 246.9300982336122559, 6.025552750865228013 ) ) ;
#97411=CARTESIAN_POINT ( 'NONE',  ( 192.7507137768506880, 296.7929658737652971, 11.30364540927242345 ) ) ;
#97413=CARTESIAN_POINT ( 'NONE',  ( 124.7815979145579632, 254.3967562850346553, -4.648177544792955347E-16 ) ) ;
#97415=CARTESIAN_POINT ( 'NONE',  ( 178.3247016823351601, 264.0066948325919043, 15.02962100587847871 ) ) ;
#97417=EDGE_CURVE ( 'NONE', #81475, #21873, #50564, .T. ) ;
#97418=CARTESIAN_POINT ( 'NONE',  ( -22.42236680055709641, 157.8615022471902591, 0.000000000000000000 ) ) ;
#97419=CARTESIAN_POINT ( 'NONE',  ( 83.57553417992789946, 212.3927522451417929, -10.00000000000009237 ) ) ;
#97423=CARTESIAN_POINT ( 'NONE',  ( 164.8537203408104972, 245.1119758834023230, 2.926011033004258355 ) ) ;
#97426=CARTESIAN_POINT ( 'NONE',  ( 190.0226014859668453, 301.5181949703289774, 3.835066345245774500 ) ) ;
#97427=CARTESIAN_POINT ( 'NONE',  ( 172.0812938429579617, 263.5228582765859642, -15.46802600247669801 ) ) ;
#97430=CARTESIAN_POINT ( 'NONE',  ( 94.51141663858166453, 213.8262482093457493, 3.021315404115420679E-15 ) ) ;
#97431=EDGE_LOOP ( 'NONE', ( #28771, #45655, #3855, #87250 ) ) ;
#97434=CARTESIAN_POINT ( 'NONE',  ( 154.1866580352537142, 265.2320175785073388, -16.52215184523099012 ) ) ;
#97439=CARTESIAN_POINT ( 'NONE',  ( 157.0986688504555957, 258.9827579613123589, -16.89964245493843009 ) ) ;
#97440=CARTESIAN_POINT ( 'NONE',  ( 178.5510943472214080, 291.5559069241597285, 6.267371293791870634 ) ) ;
#97441=CARTESIAN_POINT ( 'NONE',  ( 197.5889545809544927, 288.4128869818045473, -18.07878478781679732 ) ) ;
#97444=CARTESIAN_POINT ( 'NONE',  ( 206.5318754762992910, 272.9232936229979032, 10.63244694018452741 ) ) ;
#97446=EDGE_CURVE ( 'NONE', #89517, #98021, #95112, .T. ) ;
#97447=CARTESIAN_POINT ( 'NONE',  ( 164.5348324038273518, 245.6643059921780718, 1.473102934610569958 ) ) ;
#97450=CARTESIAN_POINT ( 'NONE',  ( 190.3920422363981118, 300.2250452325370134, 3.000504360528113423 ) ) ;
#97452=ORIENTED_EDGE ( 'NONE', *, *, #20682, .F. ) ;
#97453=CARTESIAN_POINT ( 'NONE',  ( 190.9657205613840176, 299.8846648141192190, 6.643422157963062347 ) ) ;
#97454=EDGE_CURVE ( 'NONE', #60835, #47928, #19006, .T. ) ;
#97456=CARTESIAN_POINT ( 'NONE',  ( 196.0051728737935832, 265.8263463907475170, 8.406970388261065352 ) ) ;
#97458=CARTESIAN_POINT ( 'NONE',  ( 199.1664853598643958, 285.6805235222289525, -17.06967930939392986 ) ) ;
#97459=CARTESIAN_POINT ( 'NONE',  ( 148.7148527636650783, 273.0653145036440606, -9.755595106506282477 ) ) ;
#97461=FACE_OUTER_BOUND ( 'NONE', #26997, .T. ) ;
#97462=EDGE_CURVE ( 'NONE', #91470, #59759, #35846, .T. ) ;
#97463=CARTESIAN_POINT ( 'NONE',  ( 205.6722311478874019, 272.8858671130868743, 10.04445090448162325 ) ) ;
#97464=CARTESIAN_POINT ( 'NONE',  ( -22.42236680055709641, 157.8615022471902591, 0.000000000000000000 ) ) ;
#97465=CARTESIAN_POINT ( 'NONE',  ( 165.0156970625405108, 244.8314239717225007, -1.890480716182876719 ) ) ;
#97466=CARTESIAN_POINT ( 'NONE',  ( 28.94376495785951775, 187.5177522451418497, -10.00000000000009592 ) ) ;
#97467=CARTESIAN_POINT ( 'NONE',  ( 104.5854977735480560, 237.3149278399160949, 9.188101187500093303 ) ) ;
#97468=CARTESIAN_POINT ( 'NONE',  ( 183.9376067633702405, 297.0345910832352843, -2.798678428840943866 ) ) ;
#97470=CARTESIAN_POINT ( 'NONE',  ( 162.6526018557966324, 249.3110776357280542, -10.56149055985843077 ) ) ;
#97472=CARTESIAN_POINT ( 'NONE',  ( 162.5705829494080490, 249.0664858459717550, 10.39261705965051341 ) ) ;
#97473=CARTESIAN_POINT ( 'NONE',  ( 42.15091268916992817, 185.9548013555409796, -4.594050593750042211 ) ) ;
#97474=CARTESIAN_POINT ( 'NONE',  ( 200.8828793852583203, 282.7076418644388696, 17.90302398138411633 ) ) ;
#97477=CARTESIAN_POINT ( 'NONE',  ( 191.2475944631368918, 298.9070266337688508, 7.531767195273644688 ) ) ;
#97478=ADVANCED_FACE ( 'NONE', ( #1845 ), #9948, .T. ) ;
#97481=DIRECTION ( 'NONE',  ( -0.8660254037844387076, -0.4999999999999998890, -0.000000000000000000 ) ) ;
#97483=CARTESIAN_POINT ( 'NONE',  ( 207.3874697692679945, 271.4413608369101780, -6.809237722377445401 ) ) ;
#97484=CARTESIAN_POINT ( 'NONE',  ( 179.1577515201028348, 287.5192237336674452, -12.38474070812784156 ) ) ;
#97486=CARTESIAN_POINT ( 'NONE',  ( 56.57573509489573382, 191.2202760586659451, -5.415160957724236172E-17 ) ) ;
#97487=CARTESIAN_POINT ( 'NONE',  ( 91.36976281398784749, 216.8927522451417929, -10.00000000000009059 ) ) ;
#97490=CARTESIAN_POINT ( 'NONE',  ( 155.4606602694522337, 279.7057978631885931, -1.662051915602662966 ) ) ;
#97491=CARTESIAN_POINT ( 'NONE',  ( 162.6262389125959373, 248.9700868899859074, -10.50380342094597808 ) ) ;
#97492=CARTESIAN_POINT ( 'NONE',  ( 17.11727908708474288, 174.5643266524160424, 9.188101187500095079 ) ) ;
#97493=CARTESIAN_POINT ( 'NONE',  ( 150.6916211261701619, 269.6414512649903941, -15.44346024757110847 ) ) ;
#97496=CARTESIAN_POINT ( 'NONE',  ( 45.77687342386973057, 206.4244531367911293, -4.594050593750046652 ) ) ;
#97497=CARTESIAN_POINT ( 'NONE',  ( 163.7587049410067266, 247.0085981909329576, -6.137518685179130351 ) ) ;
#97500=CARTESIAN_POINT ( 'NONE',  ( 165.0437781805843258, 244.7827860485373606, -2.050141714668513693 ) ) ;
#97502=CARTESIAN_POINT ( 'NONE',  ( 10.48659854325162222, 166.8615022471902023, 5.000000000000051514 ) ) ;
#97504=CARTESIAN_POINT ( 'NONE',  ( 130.8102634016018442, 237.1423013555409796, -4.594050593750043987 ) ) ;
#97506=CARTESIAN_POINT ( 'NONE',  ( 182.4308498937394347, 262.1046043556927430, 13.04123466523721753 ) ) ;
#97507=CARTESIAN_POINT ( 'NONE',  ( 188.1018771210319471, 260.4230313274653099, 6.875771660441075461 ) ) ;
#97508=CARTESIAN_POINT ( 'NONE',  ( 98.82118972926437550, 217.8615022471902023, 5.000000000000051514 ) ) ;
#97512=ORIENTED_EDGE ( 'NONE', *, *, #68581, .T. ) ;
#97513=CARTESIAN_POINT ( 'NONE',  ( 190.7779368023172708, 300.2099158256590385, 8.142228434510803581 ) ) ;
#97514=CARTESIAN_POINT ( 'NONE',  ( 163.9771286558119527, 246.6302772193120916, 8.800578722892527850 ) ) ;
#97517=CARTESIAN_POINT ( 'NONE',  ( 193.9623890821095245, 270.7088843966109266, -14.00671964082007293 ) ) ;
#97518=ORIENTED_EDGE ( 'NONE', *, *, #62081, .T. ) ;
#97521=CARTESIAN_POINT ( 'NONE',  ( 171.1428126037558286, 284.1639577662504621, -11.21521392563669828 ) ) ;
#97527=CARTESIAN_POINT ( 'NONE',  ( 185.4705698274941597, 296.4713422579150119, 4.661272572182228124 ) ) ;
#97529=CARTESIAN_POINT ( 'NONE',  ( 148.5539059455934137, 274.4840833604166619, -7.867015923118076515 ) ) ;
#97532=CARTESIAN_POINT ( 'NONE',  ( 84.46506227560851698, 231.1199935810940929, 2.679491924311251605 ) ) ;
#97536=CARTESIAN_POINT ( 'NONE',  ( 156.2331364254156085, 261.5399799853009313, -17.15694452653591640 ) ) ;
#97539=CARTESIAN_POINT ( 'NONE',  ( 146.9456733906991417, 276.1296230653242105, -0.7988785540157754550 ) ) ;
#97542=CARTESIAN_POINT ( 'NONE',  ( 164.0777181605478745, 246.4560510864015441, 5.763760713451748785 ) ) ;
#97546=CARTESIAN_POINT ( 'NONE',  ( 77.38680066200176100, 224.6744531367911293, 4.594050593750047540 ) ) ;
#97547=CARTESIAN_POINT ( 'NONE',  ( 198.6706607409806793, 282.8345047477174035, 17.53097579465153899 ) ) ;
#97549=CARTESIAN_POINT ( 'NONE',  ( 181.9149013745693821, 257.5326720783834844, -5.998799190420378125 ) ) ;
#97550=ORIENTED_EDGE ( 'NONE', *, *, #41974, .F. ) ;
#97552=ORIENTED_EDGE ( 'NONE', *, *, #60522, .F. ) ;
#97557=EDGE_LOOP ( 'NONE', ( #37241, #25641, #56744, #69611 ) ) ;
#97559=CARTESIAN_POINT ( 'NONE',  ( 203.2369479875374623, 278.6302754407888074, -16.66242713208754367 ) ) ;
#97560=ORIENTED_EDGE ( 'NONE', *, *, #8996, .T. ) ;
#97561=CARTESIAN_POINT ( 'NONE',  ( 158.4485968073939546, 275.2084588272041401, -13.86993402366507944 ) ) ;
#97563=CARTESIAN_POINT ( 'NONE',  ( 176.2806738015978567, 292.0729657887243889, -5.728603416521778513 ) ) ;
#97564=CARTESIAN_POINT ( 'NONE',  ( 148.0346525705264469, 274.2434557974783615, -9.381294579651672905 ) ) ;
#97566=CARTESIAN_POINT ( 'NONE',  ( 168.3608126884537342, 267.2090580166349696, -17.33422820738878301 ) ) ;
#97568=B_SPLINE_CURVE_WITH_KNOTS ( 'NONE', 3,
 ( #23839, #70448, #1573, #31936, #78571, #9677, #93796, #24357, #86211, #55228, #71472, #17767, #32456, #54732 ),
 .UNSPECIFIED., .F., .F.,
 ( 4, 2, 2, 2, 2, 2, 4 ),
 ( 0.002656117551711010150, 0.002819458382855290820, 0.002982799213999571923, 0.003146140045143852593, 0.003309480876288133262, 0.003962844200865130173, 0.005269570850019082361 ),
 .UNSPECIFIED. ) ;
#97571=CARTESIAN_POINT ( 'NONE',  ( 167.3679022544422423, 283.9162485395274302, 9.094197141742041524 ) ) ;
#97572=CARTESIAN_POINT ( 'NONE',  ( 200.5676506042510141, 270.4838747193165887, 9.277400309797105393 ) ) ;
#97573=ORIENTED_EDGE ( 'NONE', *, *, #29360, .F. ) ;
#97574=CARTESIAN_POINT ( 'NONE',  ( 1.898513289055925979, 165.2365022471902023, -10.00000000000009237 ) ) ;
#97575=DIRECTION ( 'NONE',  ( -0.4999999999999987788, 0.8660254037844392627, 0.000000000000000000 ) ) ;
#97577=CARTESIAN_POINT ( 'NONE',  ( 149.0751598600045611, 276.4070164360279591, -5.531358103402955528 ) ) ;
#97578=CARTESIAN_POINT ( 'NONE',  ( -22.42236680055709641, 157.8615022471902591, 0.000000000000000000 ) ) ;
#97580=CARTESIAN_POINT ( 'NONE',  ( 168.3515070634022948, 252.8892669010618306, 12.01402775453702709 ) ) ;
#97581=CARTESIAN_POINT ( 'NONE',  ( 194.9222774061866232, 292.5393265380751586, 15.09658607083830439 ) ) ;
#97585=EDGE_LOOP ( 'NONE', ( #21287, #52404, #9307, #3697 ) ) ;
#97586=CARTESIAN_POINT ( 'NONE',  ( 10.91961124514384274, 167.1115022471901739, -5.000000000000041744 ) ) ;
#97589=CARTESIAN_POINT ( 'NONE',  ( 175.0183846948854125, 281.5670661755301580, -14.11114436949414674 ) ) ;
#97590=CARTESIAN_POINT ( 'NONE',  ( 196.1252721995043942, 284.4712197134549001, -17.81715240067734030 ) ) ;
#97591=CARTESIAN_POINT ( 'NONE',  ( 149.0802055316563326, 272.4325049467973940, 12.84384348890831085 ) ) ;
#97597=B_SPLINE_CURVE_WITH_KNOTS ( 'NONE', 3,
 ( #12806, #5186, #42176, #20902 ),
 .UNSPECIFIED., .F., .F.,
 ( 4, 4 ),
 ( 0.04303599427739471933, 0.04887120950165264183 ),
 .UNSPECIFIED. ) ;
#97600=DIRECTION ( 'NONE',  ( -0.4999999999999987788, 0.8660254037844392627, 0.000000000000000000 ) ) ;
#97601=EDGE_CURVE ( 'NONE', #41192, #87863, #43315, .T. ) ;
#97606=CARTESIAN_POINT ( 'NONE',  ( 175.6309865724497001, 290.9702953720650385, 2.692108822669778245 ) ) ;
#97607=CARTESIAN_POINT ( 'NONE',  ( 192.3401793061076717, 297.5040324353506094, 12.56432540404525611 ) ) ;
#97609=CARTESIAN_POINT ( 'NONE',  ( 6.454167755106333892, 174.5333772461660828, 9.188101187500095079 ) ) ;
#97610=CARTESIAN_POINT ( 'NONE',  ( 101.4736528484039724, 220.2048013555409796, 4.594050593750051981 ) ) ;
#97612=CARTESIAN_POINT ( 'NONE',  ( 186.3706575779193599, 296.6012036956348652, -7.271390144495396335 ) ) ;
#97616=CARTESIAN_POINT ( 'NONE',  ( 163.3740049908953438, 249.6749180501957710, -11.76522313559978627 ) ) ;
#97618=CARTESIAN_POINT ( 'NONE',  ( 147.7467138384290308, 274.7421803109381813, -9.190172068879620682 ) ) ;
#97620=CARTESIAN_POINT ( 'NONE',  ( 196.3986213162682759, 266.7212399403405243, 8.097488202709509864 ) ) ;
#97621=CARTESIAN_POINT ( 'NONE',  ( 77.90020070641381267, 227.3297689869269504, -2.679491924311252493 ) ) ;
#97622=CARTESIAN_POINT ( 'NONE',  ( 56.65657787896151376, 213.5177522451419065, 5.000000000000046185 ) ) ;
#97623=CARTESIAN_POINT ( 'NONE',  ( 54.07885559584777013, 190.4824982072973967, 3.021315404115420679E-15 ) ) ;
#97624=CARTESIAN_POINT ( 'NONE',  ( 152.8894687064977234, 278.3516875449029158, -6.243347624783317507 ) ) ;
#97625=B_SPLINE_CURVE_WITH_KNOTS ( 'NONE', 3,
 ( #89528, #20089, #49978, #97119 ),
 .UNSPECIFIED., .F., .F.,
 ( 4, 4 ),
 ( 0.001250264319432415911, 0.006536272345052643665 ),
 .UNSPECIFIED. ) ;
#97627=CARTESIAN_POINT ( 'NONE',  ( 90.72943840876202160, 217.0643266524159571, -9.188101187500093303 ) ) ;
#97629=CARTESIAN_POINT ( 'NONE',  ( 163.2245414155497087, 258.2687556262928297, 16.54154467503536452 ) ) ;
#97630=FACE_OUTER_BOUND ( 'NONE', #2738, .T. ) ;
#97631=CARTESIAN_POINT ( 'NONE',  ( 199.9055245033136714, 284.4004701769926555, 18.46055504797378077 ) ) ;
#97632=FACE_OUTER_BOUND ( 'NONE', #36941, .T. ) ;
#97636=CARTESIAN_POINT ( 'NONE',  ( 193.0761489135300906, 296.2292956824684893, -11.99675185248219655 ) ) ;
#97637=CARTESIAN_POINT ( 'NONE',  ( 127.8330407560429904, 254.6115022471903160, -5.000000000000047962 ) ) ;
#97641=CARTESIAN_POINT ( 'NONE',  ( 193.2140586456748679, 295.9904290195353269, -12.67640480829088823 ) ) ;
#97642=CARTESIAN_POINT ( 'NONE',  ( 190.4205601722502479, 287.1571841927307673, -15.84311712791906857 ) ) ;
#97643=B_SPLINE_CURVE_WITH_KNOTS ( 'NONE', 3,
 ( #93018, #54464, #14982, #30701, #786, #1302, #33193, #64094, #10908, #56490, #55470, #86456, #56978, #95039, #87477, #33711, #80341, #48398, #64603, #41784, #87964, #40769, #25603, #18011, #93532, #16489, #10405, #32186, #31672, #8890, #86957, #95558, #71721, #85963, #62568, #49394, #48904, #79839, #39759, #41275, #72217, #47385, #18508, #24088, #2821, #9397 ),
 .UNSPECIFIED., .F., .F.,
 ( 4, 2, 2, 2, 2, 2, 2, 2, 2, 2, 2, 2, 2, 2, 2, 2, 2, 2, 2, 2, 2, 2, 4 ),
 ( 0.0009098864418214376668, 0.001395788648591240848, 0.001881690855361043812, 0.002124641958745928597, 0.002367593062130813383, 0.002489068613823246234, 0.002610544165515678652, 0.002732019717208111504, 0.002853495268900544356, 0.003096446372285409192, 0.003339397475670274895, 0.003825299682440005435, 0.004797104095979466513, 0.005768908509518927592, 0.006254810716288658132, 0.006740712923058388671, 0.006862188474750856651, 0.006922926250597124034, 0.006983664026443391418, 0.007226615129828508656, 0.007712517336598743133, 0.008198419543368978477, 0.008684321750139212953 ),
 .UNSPECIFIED. ) ;
#97644=ORIENTED_EDGE ( 'NONE', *, *, #89156, .T. ) ;
#97646=CARTESIAN_POINT ( 'NONE',  ( 198.6587626159274294, 286.5599251108861267, 17.99840276545888784 ) ) ;
#97647=CARTESIAN_POINT ( 'NONE',  ( 178.3542226995226940, 255.3138203415698513, 7.881446944319069559 ) ) ;
#97648=CARTESIAN_POINT ( 'NONE',  ( 201.5189872289815867, 266.7509884862435570, -2.318412474989284267 ) ) ;
#97649=CARTESIAN_POINT ( 'NONE',  ( 130.4311169673963207, 256.1115022471902876, -5.000000000000047962 ) ) ;
#97651=ORIENTED_EDGE ( 'NONE', *, *, #3349, .T. ) ;
#97654=CARTESIAN_POINT ( 'NONE',  ( 196.6801871783479498, 265.3273392373002366, -4.500484501757973099 ) ) ;
#97659=EDGE_CURVE ( 'NONE', #71349, #64147, #53940, .T. ) ;
#97661=CARTESIAN_POINT ( 'NONE',  ( 205.9877610862153858, 273.8657273917527846, 10.74600286489862988 ) ) ;
#97662=CARTESIAN_POINT ( 'NONE',  ( 150.4851912698882757, 251.5643266524160424, -9.188101187500093303 ) ) ;
#97663=CARTESIAN_POINT ( 'NONE',  ( 193.0139627561028988, 296.3370052666596735, -13.53354153023428275 ) ) ;
#97664=CARTESIAN_POINT ( 'NONE',  ( 196.3249884498792994, 275.2518087180711177, 16.06659936265807431 ) ) ;
#97667=CARTESIAN_POINT ( 'NONE',  ( 167.4994950215155427, 276.2173684559796243, 14.96917790999040321 ) ) ;
#97668=EDGE_CURVE ( 'NONE', #17163, #27033, #10564, .T. ) ;
#97674=CARTESIAN_POINT ( 'NONE',  ( 173.9599451638853509, 256.5427416416744677, -12.41841015343009680 ) ) ;
#97675=CARTESIAN_POINT ( 'NONE',  ( 162.3916291218297943, 272.3095098889435235, -15.78716446736534351 ) ) ;
#97677=CARTESIAN_POINT ( 'NONE',  ( 168.2235428883953432, 249.7409626584020543, -8.343714295448053875 ) ) ;
#97679=CARTESIAN_POINT ( 'NONE',  ( 147.6130046165826570, 276.0663062336524263, 0.7645130601501862744 ) ) ;
#97680=CARTESIAN_POINT ( 'NONE',  ( 189.8147415777049218, 301.8782188922952514, -0.5019643756309712934 ) ) ;
#97682=CARTESIAN_POINT ( 'NONE',  ( 168.9285091408607684, 266.8905904589466900, 17.77692745299157195 ) ) ;
#97684=CARTESIAN_POINT ( 'NONE',  ( 178.7706546344515743, 255.8485219706211353, 4.885452066709516039 ) ) ;
#97685=CARTESIAN_POINT ( 'NONE',  ( 97.84665082640911749, 236.4869531367911293, 4.594050593750046652 ) ) ;
#97687=CARTESIAN_POINT ( 'NONE',  ( 192.0122679602540643, 293.3270677385487488, -14.68313672456705810 ) ) ;
#97691=CARTESIAN_POINT ( 'NONE',  ( 195.0951974243075142, 285.7261168938122751, -17.71149292247018181 ) ) ;
#97692=CARTESIAN_POINT ( 'NONE',  ( 195.8248271798537417, 291.4684452715354155, 17.35175160929494709 ) ) ;
#97693=CARTESIAN_POINT ( 'NONE',  ( 159.7132918459648181, 254.0154592091499239, -16.90058287995827158 ) ) ;
#97694=CARTESIAN_POINT ( 'NONE',  ( 208.3210024379012282, 269.8244348243121635, 2.045688540111487264 ) ) ;
#97695=VERTEX_POINT ( 'NONE', #58516 ) ;
#97698=CARTESIAN_POINT ( 'NONE',  ( 163.2000388741132895, 247.9762362032568035, -11.19676374274550312 ) ) ;
#97701=CARTESIAN_POINT ( 'NONE',  ( 99.09182266439904652, 228.0177522451418781, -10.00000000000009592 ) ) ;
#97703=CARTESIAN_POINT ( 'NONE',  ( 141.9874905431360332, 240.5327760586659451, 1.948934522072303157E-15 ) ) ;
#97704=CARTESIAN_POINT ( 'NONE',  ( 199.9134407114337364, 283.6250491837689651, 17.05367660732407842 ) ) ;
#97707=CARTESIAN_POINT ( 'NONE',  ( 190.8545714895799392, 300.0771806536980648, -5.516553996882049837 ) ) ;
#97709=CARTESIAN_POINT ( 'NONE',  ( 190.0760587457662325, 263.4785607165754868, -9.739317369409583591 ) ) ;
#97710=EDGE_CURVE ( 'NONE', #15038, #21882, #49126, .T. ) ;
#97711=CARTESIAN_POINT ( 'NONE',  ( 173.2675837151294900, 251.6514125879787969, -0.3741643316691787846 ) ) ;
#97712=CARTESIAN_POINT ( 'NONE',  ( 178.3763904113375247, 285.3699055491184140, 13.04576391269180746 ) ) ;
#97714=CARTESIAN_POINT ( 'NONE',  ( 197.9956738476683711, 281.2438040225179634, -16.56933298855467740 ) ) ;
#97718=CARTESIAN_POINT ( 'NONE',  ( 61.82584055745639517, 200.3768266524159856, -9.188101187500091527 ) ) ;
#97719=CARTESIAN_POINT ( 'NONE',  ( 159.3586121662929713, 254.6297824347537642, -15.50090345830412630 ) ) ;
#97721=CARTESIAN_POINT ( 'NONE',  ( 162.7070706717508699, 248.8300821762643693, -9.986337079333621247 ) ) ;
#97722=EDGE_CURVE ( 'NONE', #79294, #9648, #60053, .T. ) ;
#97732=CARTESIAN_POINT ( 'NONE',  ( 17.98330449086917682, 175.0643266524160140, -9.188101187500093303 ) ) ;
#97734=VERTEX_POINT ( 'NONE', #61507 ) ;
#97737=CARTESIAN_POINT ( 'NONE',  ( 201.7504478526379899, 278.7391314730009526, 15.42661883977095805 ) ) ;
#97738=CARTESIAN_POINT ( 'NONE',  ( 178.3142739445455618, 279.4967965441328488, 17.12304257816909825 ) ) ;
#97739=CARTESIAN_POINT ( 'NONE',  ( 208.0287371622045782, 270.3306531311065442, 3.558879245883286746 ) ) ;
#97741=CARTESIAN_POINT ( 'NONE',  ( 61.44712799118319424, 194.0327760586659451, 1.948934522072302763E-15 ) ) ;
#97743=CARTESIAN_POINT ( 'NONE',  ( 171.1378123370926971, 286.9384401993552842, 7.092917925564754533 ) ) ;
#97744=CARTESIAN_POINT ( 'NONE',  ( 146.8000281410530192, 276.3818880375922049, 4.652863924796177386 ) ) ;
#97746=CARTESIAN_POINT ( 'NONE',  ( 197.8517725239618699, 287.3315203694608044, 17.01882341879843707 ) ) ;
#97747=CARTESIAN_POINT ( 'NONE',  ( 178.4307736886035229, 293.0376200449680368, 2.618413240329335867 ) ) ;
#97748=CARTESIAN_POINT ( 'NONE',  ( 178.4481950008050433, 276.1063989467955935, 16.34093626456154524 ) ) ;
#97752=CARTESIAN_POINT ( 'NONE',  ( 118.1443815476567352, 229.0177522451417929, 5.000000000000051514 ) ) ;
#97754=CARTESIAN_POINT ( 'NONE',  ( 96.65612621980318409, 236.6115022471902876, -5.000000000000047962 ) ) ;
#97756=CARTESIAN_POINT ( 'NONE',  ( 194.7041213697769422, 285.5929353680269855, -17.62016002267809256 ) ) ;
#97758=CARTESIAN_POINT ( 'NONE',  ( 56.27743144475606130, 212.4869531367911009, 4.594050593750046652 ) ) ;
#97760=CARTESIAN_POINT ( 'NONE',  ( 165.8605944207784262, 265.2106218463247274, 16.56633027260685864 ) ) ;
#97761=CARTESIAN_POINT ( 'NONE',  ( 161.5266078408477597, 251.3399204103630211, 13.01505764280997468 ) ) ;
#97765=CARTESIAN_POINT ( 'NONE',  ( 207.3062152119541679, 271.5820978585240368, 7.879821064966149535 ) ) ;
#97766=CARTESIAN_POINT ( 'NONE',  ( 39.04508293989853485, 204.8967562850347122, -4.648177544792955347E-16 ) ) ;
#97768=CARTESIAN_POINT ( 'NONE',  ( 189.5731351232621762, 264.7541819150383162, 10.55408932226666785 ) ) ;
#97770=CARTESIAN_POINT ( 'NONE',  ( 156.8993174718108605, 258.8894057963813680, 16.93179113901802069 ) ) ;
#97775=CARTESIAN_POINT ( 'NONE',  ( 175.1307738592725798, 254.8361248832076740, 7.862726238744712326 ) ) ;
#97777=ORIENTED_EDGE ( 'NONE', *, *, #69711, .F. ) ;
#97780=CARTESIAN_POINT ( 'NONE',  ( 150.8359915840788688, 269.3913942967808453, 15.73449616766854575 ) ) ;
#97781=CARTESIAN_POINT ( 'NONE',  ( 206.8659638600981623, 272.3446355680395641, -10.26115277030573125 ) ) ;
#97784=CARTESIAN_POINT ( 'NONE',  ( 207.7666684749232786, 270.7845694125510931, -6.630926507062123498 ) ) ;
#97785=CARTESIAN_POINT ( 'NONE',  ( 196.1245817477023650, 288.9492551302209336, 17.30641872853625074 ) ) ;
#97786=CARTESIAN_POINT ( 'NONE',  ( 196.3174919959537306, 290.6151247789487684, -17.61248417473235151 ) ) ;
#97788=EDGE_CURVE ( 'NONE', #7026, #85624, #80566, .T. ) ;
#97789=CARTESIAN_POINT ( 'NONE',  ( 198.2040940955416488, 287.3474340887963763, 16.95806375232200480 ) ) ;
#97790=DIRECTION ( 'NONE',  ( 0.4999999999999992784, -0.8660254037844390407, 0.000000000000000000 ) ) ;
#97793=CARTESIAN_POINT ( 'NONE',  ( 124.1521724663614492, 251.6744531367911577, 4.594050593750047540 ) ) ;
#97794=DIRECTION ( 'NONE',  ( -0.8660254037844387076, -0.4999999999999998890, -0.000000000000000000 ) ) ;
#97795=ORIENTED_EDGE ( 'NONE', *, *, #42615, .T. ) ;
#97798=CARTESIAN_POINT ( 'NONE',  ( 106.5950644350847369, 243.8967562850346837, -4.648177544792955347E-16 ) ) ;
#97799=ORIENTED_EDGE ( 'NONE', *, *, #86527, .F. ) ;
#97800=CARTESIAN_POINT ( 'NONE',  ( 166.2800977938260019, 260.3313707980180993, -16.91817955569885257 ) ) ;
#97803=CARTESIAN_POINT ( 'NONE',  ( 198.4706398937704819, 286.8857632237200619, 17.04020736381253798 ) ) ;
#97805=CARTESIAN_POINT ( 'NONE',  ( 83.61187889534991768, 209.8923013555409796, 4.594050593750050204 ) ) ;
#97807=CARTESIAN_POINT ( 'NONE',  ( 24.61363793893735874, 175.0177522451417929, 5.000000000000051514 ) ) ;
#97808=CARTESIAN_POINT ( 'NONE',  ( 179.7389585068036979, 283.2694176073634935, 16.15404047216739514 ) ) ;
#97809=CARTESIAN_POINT ( 'NONE',  ( 150.3996455637841621, 270.1471677736116703, 15.13740740754872327 ) ) ;
#97810=CARTESIAN_POINT ( 'NONE',  ( -16.43235775771475105, 167.9865022471903160, -10.00000000000009592 ) ) ;
#97811=ORIENTED_EDGE ( 'NONE', *, *, #13609, .F. ) ;
#97814=CARTESIAN_POINT ( 'NONE',  ( 153.3939648708017387, 264.9608545997728015, -16.49556533540763681 ) ) ;
#97815=B_SPLINE_SURFACE_WITH_KNOTS ( 'NONE', 3, 1, ( 
 ( #8180, #60851 ),
 ( #38052, #7675 ),
 ( #53754, #78086 ),
 ( #38560, #30967 ),
 ( #61856, #23358 ),
 ( #29974, #85216 ),
 ( #15761, #91815 ),
 ( #93306, #62351 ),
 ( #23863, #54754 ),
 ( #53273, #85741 ),
 ( #39545, #47162 ),
 ( #21874, #83722 ),
 ( #70467, #91314 ),
 ( #14279, #84227 ),
 ( #14774, #76581 ),
 ( #45171, #49667 ),
 ( #26383, #80623 ),
 ( #24868, #25370 ),
 ( #70992, #17270 ),
 ( #62862, #79623 ),
 ( #86733, #64376 ),
 ( #56768, #80121 ),
 ( #40052, #87254 ),
 ( #71988, #48173 ),
 ( #2593, #95338 ),
 ( #1596, #2087 ),
 ( #33479, #32965 ),
 ( #93819, #10186 ),
 ( #10683, #3111 ),
 ( #55250, #33999 ),
 ( #17788, #32479 ),
 ( #71494, #41561 ),
 ( #63375, #48688 ),
 ( #41052, #25896 ) ),
 .UNSPECIFIED., .T., .F., .F.,
 ( 4, 2, 2, 2, 2, 2, 2, 2, 2, 2, 2, 2, 2, 2, 2, 2, 4 ),
 ( 2, 2 ),
 ( 0.000000000000000000, 0.06250000000000000000, 0.1250000000000000000, 0.1875000000000000000, 0.2500000000000000000, 0.3125000000000000000, 0.3750000000000000000, 0.4375000000000000000, 0.5000000000000000000, 0.5625000000000000000, 0.6250000000000000000, 0.6875000000000000000, 0.7500000000000000000, 0.8125000000000000000, 0.8750000000000000000, 0.9375000000000000000, 1.000000000000000000 ),
 ( 0.000000000000000000, 1.000000000000000000 ),
 .UNSPECIFIED. ) ;
#97817=ORIENTED_EDGE ( 'NONE', *, *, #85842, .F. ) ;
#97823=CARTESIAN_POINT ( 'NONE',  ( 196.1197415632541379, 279.6791495332669797, 16.37442619035736158 ) ) ;
#97825=CARTESIAN_POINT ( 'NONE',  ( 130.8910194135003735, 252.5024278399160949, 9.188101187500095079 ) ) ;
#97827=CARTESIAN_POINT ( 'NONE',  ( 148.6500818154487433, 275.1775010768142238, 7.719411301773694944 ) ) ;
#97830=CARTESIAN_POINT ( 'NONE',  ( 203.5517807763935991, 276.4131063546051337, 14.32831804246049678 ) ) ;
#97831=CARTESIAN_POINT ( 'NONE',  ( 153.2819058590468160, 274.2512448977743134, -12.24885634829186287 ) ) ;
#97835=( BOUNDED_CURVE ( )  B_SPLINE_CURVE ( 2, ( #50807, #96970, #81265, #36100, #81757, #89856, #12842, #97928, #28503 ),
 .UNSPECIFIED., .F., .T. ) 
 B_SPLINE_CURVE_WITH_KNOTS ( ( 3, 2, 2, 2, 3 ),
 ( 0.2943548387096774355, 0.2956989247311828106, 0.2983870967741935609, 0.3010752688172043112, 0.3024193548387096864 ),
 .UNSPECIFIED. ) 
 CURVE ( )  GEOMETRIC_REPRESENTATION_ITEM ( )  RATIONAL_B_SPLINE_CURVE ( ( 0.9330127018922194093, 0.9330127018922194093, 1.000000000000000000, 0.8660254037844387076, 1.000000000000000000, 0.8660254037844387076, 1.000000000000000000, 0.9330127018922194093, 0.9330127018922194093 ) ) 
 REPRESENTATION_ITEM ( '' )  );
#97836=CARTESIAN_POINT ( 'NONE',  ( 185.5156133380430390, 277.7268379766968565, -17.03516142629836594 ) ) ;
#97838=CARTESIAN_POINT ( 'NONE',  ( 205.9281787291064347, 273.9689270615001533, -10.62323193457751458 ) ) ;
#97839=CARTESIAN_POINT ( 'NONE',  ( 202.6577094508454024, 267.5156926251955838, 0.8710555158424478917 ) ) ;
#97840=EDGE_CURVE ( 'NONE', #312, #8895, #8321, .T. ) ;
#97846=CARTESIAN_POINT ( 'NONE',  ( 148.9266665119372703, 272.6984423298952152, 12.06339424062075061 ) ) ;
#97847=DIRECTION ( 'NONE',  ( -0.8660254037844387076, -0.4999999999999998890, -0.000000000000000000 ) ) ;
#97849=CARTESIAN_POINT ( 'NONE',  ( 159.3169041484411537, 254.7020228407560580, 16.67170756419672628 ) ) ;
#97850=CARTESIAN_POINT ( 'NONE',  ( 193.6523268064705974, 293.2313262976975352, 15.26490498002906193 ) ) ;
#97851=CARTESIAN_POINT ( 'NONE',  ( 137.2691092145631160, 243.3927522451418213, 10.00000000000009592 ) ) ;
#97855=CARTESIAN_POINT ( 'NONE',  ( 178.0315741628076012, 287.5935043698759728, -13.06113257055532451 ) ) ;
#97856=CARTESIAN_POINT ( 'NONE',  ( 198.4522155198218059, 286.9176751754968109, -17.57438352224490075 ) ) ;
#97857=CARTESIAN_POINT ( 'NONE',  ( 4.992576338337582520, 179.8149278399160949, -9.188101187500095079 ) ) ;
#97858=CARTESIAN_POINT ( 'NONE',  ( 175.6766631755835419, 257.0359803582177847, -10.59688122334902793 ) ) ;
#97861=CARTESIAN_POINT ( 'NONE',  ( -22.42236680055709641, 157.8615022471902591, 0.000000000000000000 ) ) ;
#97863=CARTESIAN_POINT ( 'NONE',  ( 150.1195797453556793, 276.5050416553082755, 3.721351720276065755 ) ) ;
#97864=CARTESIAN_POINT ( 'NONE',  ( 171.3734714223081426, 258.1936803860005512, 14.40034214095746989 ) ) ;
#97865=CARTESIAN_POINT ( 'NONE',  ( 70.58515312316129098, 204.8927522451418213, -10.00000000000009059 ) ) ;
#97866=CARTESIAN_POINT ( 'NONE',  ( 173.2798715285074991, 281.8114527337138497, 15.08241540710736750 ) ) ;
#97867=CARTESIAN_POINT ( 'NONE',  ( 198.0827002274358222, 287.5576944360828975, 17.17879237213074006 ) ) ;
#97869=CARTESIAN_POINT ( 'NONE',  ( 53.71569994882479193, 208.4865022471902876, -10.00000000000009415 ) ) ;
#97870=CARTESIAN_POINT ( 'NONE',  ( 181.8674585300132378, 291.6431133160953664, 9.312409377393402465 ) ) ;
#97871=CARTESIAN_POINT ( 'NONE',  ( 189.9052851100924215, 301.7213928939034986, -1.077181946533001256 ) ) ;
#97872=CARTESIAN_POINT ( 'NONE',  ( 13.92363686274711299, 178.8458772461660544, 9.188101187500095079 ) ) ;
#97873=CARTESIAN_POINT ( 'NONE',  ( 168.2127584262427149, 286.2670693736010890, 4.111954200343466148 ) ) ;
#97874=CARTESIAN_POINT ( 'NONE',  ( 5.218277336896219865, 180.4865022471903160, 10.00000000000009415 ) ) ;
#97876=CARTESIAN_POINT ( 'NONE',  ( 201.6018788519649831, 280.5407822744489863, -16.29061894498408947 ) ) ;
#97878=CARTESIAN_POINT ( 'NONE',  ( 180.9785907350442926, 277.5730618892402504, 16.35545640519342925 ) ) ;
#97880=CARTESIAN_POINT ( 'NONE',  ( 153.4409967745565666, 266.3578157004054106, -16.49295564300695460 ) ) ;
#97881=CARTESIAN_POINT ( 'NONE',  ( 176.4956094263426110, 260.4465060475594100, -13.34520323348970194 ) ) ;
#97884=CARTESIAN_POINT ( 'NONE',  ( 165.6285009359904734, 285.3942701294749327, 0.4263846489270779472 ) ) ;
#97885=CARTESIAN_POINT ( 'NONE',  ( -22.42236680055709641, 157.8615022471902591, 0.000000000000000000 ) ) ;
#97886=CARTESIAN_POINT ( 'NONE',  ( 159.1005818787057819, 259.4300168470162475, 16.69242165874631567 ) ) ;
#97887=CARTESIAN_POINT ( 'NONE',  ( 193.9401685343300699, 294.7327698005063326, 14.01047396938887069 ) ) ;
#97890=CARTESIAN_POINT ( 'NONE',  ( 156.5356202806696615, 276.3685272183531083, 10.26723329993582112 ) ) ;
#97891=CARTESIAN_POINT ( 'NONE',  ( 206.6703863510205679, 272.6833857505801006, -10.72500664779635393 ) ) ;
#97896=CARTESIAN_POINT ( 'NONE',  ( 155.6535436963908694, 261.0471492701456668, -17.87366571046205976 ) ) ;
#97897=ORIENTED_EDGE ( 'NONE', *, *, #10351, .T. ) ;
#97898=ORIENTED_EDGE ( 'NONE', *, *, #64448, .F. ) ;
#97900=CARTESIAN_POINT ( 'NONE',  ( 164.3853877993040840, 245.9231516401292197, 5.995325337583643943 ) ) ;
#97901=CARTESIAN_POINT ( 'NONE',  ( 192.8325075361489382, 296.6512949269187516, 11.74553025762331515 ) ) ;
#97903=CARTESIAN_POINT ( 'NONE',  ( 150.6453220160077251, 269.7216436761371483, 14.94145576020818034 ) ) ;
#97906=VERTEX_POINT ( 'NONE', #16906 ) ;
#97909=AXIS2_PLACEMENT_3D ( 'NONE', #96547, #66103, #5795 ) ;
#97911=CARTESIAN_POINT ( 'NONE',  ( 165.0087721269838710, 244.8434183119457543, 2.604344609212914108 ) ) ;
#97913=ORIENTED_EDGE ( 'NONE', *, *, #7315, .T. ) ;
#97914=CARTESIAN_POINT ( 'NONE',  ( 174.8404000400799703, 277.4648157049296628, -15.64849645087200791 ) ) ;
#97915=CYLINDRICAL_SURFACE ( 'NONE', #2978, 10.00000000000010658 ) ;
#97917=CARTESIAN_POINT ( 'NONE',  ( 75.41814989884494480, 225.8967562850346837, -4.648177544792955347E-16 ) ) ;
#97918=CARTESIAN_POINT ( 'NONE',  ( 147.5381343315788172, 275.1034506142203782, -4.056595942992749393 ) ) ;
#97920=CARTESIAN_POINT ( 'NONE',  ( 157.0239713899953244, 269.7369771206523978, 16.31777668093047851 ) ) ;
#97922=CARTESIAN_POINT ( 'NONE',  ( 156.2277803658613777, 266.3225699999913445, -16.24938540415413613 ) ) ;
#97923=CARTESIAN_POINT ( 'NONE',  ( 168.8785100482814698, 272.6966330010931756, 17.41127854651366391 ) ) ;
#97924=CARTESIAN_POINT ( 'NONE',  ( 147.4811722709131914, 275.2021117973970377, 3.890385073228495916 ) ) ;
#97927=CARTESIAN_POINT ( 'NONE',  ( 192.5712965840290849, 297.1037255674836501, 11.03742858512898906 ) ) ;
#97928=CARTESIAN_POINT ( 'NONE',  ( 39.83579079637758014, 182.2592609112380160, 2.679491924311254714 ) ) ;
#97929=CARTESIAN_POINT ( 'NONE',  ( 191.0702043019150835, 299.7036936669546776, -8.800021049343948576 ) ) ;
#97932=B_SPLINE_CURVE_WITH_KNOTS ( 'NONE', 3,
 ( #62621, #68737, #32236, #61628 ),
 .UNSPECIFIED., .F., .F.,
 ( 4, 4 ),
 ( 0.008172245353423012934, 0.01420657290482196973 ),
 .UNSPECIFIED. ) ;
#97934=CARTESIAN_POINT ( 'NONE',  ( 149.4171629335945681, 271.8488776066536730, -11.42564036194071520 ) ) ;
#97936=CARTESIAN_POINT ( 'NONE',  ( 198.6755293322981117, 286.5308843062557571, 17.86676876308990103 ) ) ;
#97939=CARTESIAN_POINT ( 'NONE',  ( 51.48077938449444702, 188.9824982072973967, 3.021315404115420679E-15 ) ) ;
#97940=ORIENTED_EDGE ( 'NONE', *, *, #98038, .F. ) ;
#97941=CARTESIAN_POINT ( 'NONE',  ( 149.5090996232239036, 271.6896385891362797, -11.55286514765376005 ) ) ;
#97946=CARTESIAN_POINT ( 'NONE',  ( 160.1964060607056979, 253.1786808433599845, -14.64952422815191113 ) ) ;
#97947=CARTESIAN_POINT ( 'NONE',  ( 148.0419010042100751, 274.2309011420633169, -10.20829995470312568 ) ) ;
#97949=CARTESIAN_POINT ( 'NONE',  ( 170.1313062173066726, 255.2739091071986479, -11.62815245866028313 ) ) ;
#97951=CARTESIAN_POINT ( 'NONE',  ( 153.4495116231415750, 264.8646448025247082, -16.73555355292144498 ) ) ;
#97952=CARTESIAN_POINT ( 'NONE',  ( 206.9258336080761183, 272.2409381227055292, 6.776000910836894597 ) ) ;
#97953=CARTESIAN_POINT ( 'NONE',  ( 30.67581576542834654, 198.5177522451419350, 5.000000000000046185 ) ) ;
#97954=CARTESIAN_POINT ( 'NONE',  ( 117.0885659928033817, 250.6589784336661069, -6.496448406907676862E-16 ) ) ;
#97955=CARTESIAN_POINT ( 'NONE',  ( 180.8000599349354900, 294.0875826803771247, -2.709611528315936102 ) ) ;
#97956=CARTESIAN_POINT ( 'NONE',  ( 167.7145385494464165, 281.8102352406253317, -10.91421457602037925 ) ) ;
#97957=CARTESIAN_POINT ( 'NONE',  ( 208.3379394461497895, 269.7950990654974817, 2.541397148058371691 ) ) ;
#97960=B_SPLINE_CURVE_WITH_KNOTS ( 'NONE', 3,
 ( #84483, #45431, #37827, #59631 ),
 .UNSPECIFIED., .F., .F.,
 ( 4, 4 ),
 ( 0.002796930759027657122, 0.003029742318773366843 ),
 .UNSPECIFIED. ) ;
#97962=CARTESIAN_POINT ( 'NONE',  ( 7.365298646897277202, 168.3927522451418213, 10.00000000000009948 ) ) ;
#97963=CARTESIAN_POINT ( 'NONE',  ( 180.5010753389648812, 267.3347324538273710, 15.01776452798817374 ) ) ;
#97966=EDGE_CURVE ( 'NONE', #59762, #6045, #5701, .T. ) ;
#97967=CARTESIAN_POINT ( 'NONE',  ( 207.1007598919583472, 271.9379569114424271, -6.086525981869248092 ) ) ;
#97968=CARTESIAN_POINT ( 'NONE',  ( 59.82969263072505584, 216.8967562850347122, -4.648177544792955347E-16 ) ) ;
#97970=CARTESIAN_POINT ( 'NONE',  ( 99.95784806818352308, 218.5177522451417929, 5.000000000000051514 ) ) ;
#97971=EDGE_LOOP ( 'NONE', ( #88392, #19758, #56778 ) ) ;
#97972=ADVANCED_FACE ( 'NONE', ( #32101 ), #10329, .T. ) ;
#97974=CARTESIAN_POINT ( 'NONE',  ( 162.6774150396764469, 248.8814472377480911, 10.88033986792731689 ) ) ;
#97975=CARTESIAN_POINT ( 'NONE',  ( 162.7007457333762090, 248.8410372908842021, -10.94671474643812914 ) ) ;
#97977=CARTESIAN_POINT ( 'NONE',  ( 6.454167755106333892, 174.5333772461660828, 9.188101187500095079 ) ) ;
#97982=CARTESIAN_POINT ( 'NONE',  ( 53.97765888354242492, 189.7202760586659736, -5.415160957724236172E-17 ) ) ;
#97983=CARTESIAN_POINT ( 'NONE',  ( 164.4405316900629259, 245.8276396196081350, -6.144538123479245328 ) ) ;
#97984=CARTESIAN_POINT ( 'NONE',  ( 203.7313627084707832, 276.2715032248725038, 13.33488798586162360 ) ) ;
#97987=ORIENTED_EDGE ( 'NONE', *, *, #53326, .F. ) ;
#97989=CARTESIAN_POINT ( 'NONE',  ( 14.74455677852503932, 185.9865022471903444, -10.00000000000009415 ) ) ;
#97991=CARTESIAN_POINT ( 'NONE',  ( 130.0249940097159254, 252.0024278399160949, -9.188101187500093303 ) ) ;
#97996=CARTESIAN_POINT ( 'NONE',  ( 196.0034224882197975, 291.1591091234520263, 17.53794140922627776 ) ) ;
#97997=CARTESIAN_POINT ( 'NONE',  ( 189.4804681487932783, 289.7638976020832047, 15.63394399629991582 ) ) ;
#98000=CARTESIAN_POINT ( 'NONE',  ( 190.8604783348975502, 300.0669496974951471, 7.597731640149610222 ) ) ;
#98002=CARTESIAN_POINT ( 'NONE',  ( 151.6041069312964567, 268.5621543234237834, -14.59499063436561528 ) ) ;
#98003=CARTESIAN_POINT ( 'NONE',  ( 173.0384568215392562, 268.2350346299093644, -16.30935032955606445 ) ) ;
#98004=CARTESIAN_POINT ( 'NONE',  ( 193.8643712729062543, 270.7948579697045943, -13.84106480611635526 ) ) ;
#98011=CARTESIAN_POINT ( 'NONE',  ( 196.1975761016102808, 270.9518507311354369, 12.17928950200870020 ) ) ;
#98013=CARTESIAN_POINT ( 'NONE',  ( 185.7675376949824795, 296.6512829522437187, 4.668071064500018963 ) ) ;
#98014=CARTESIAN_POINT ( 'NONE',  ( 140.3182403272686258, 258.4865022471902876, 10.00000000000009415 ) ) ;
#98016=CARTESIAN_POINT ( 'NONE',  ( 153.2583947049096764, 265.1956690150883560, -17.64103123457563882 ) ) ;
#98017=EDGE_CURVE ( 'NONE', #79399, #86304, #64931, .T. ) ;
#98021=VERTEX_POINT ( 'NONE', #40193 ) ;
#98026=CARTESIAN_POINT ( 'NONE',  ( 161.5631100156346633, 265.8146362027571854, -17.76550717985403693 ) ) ;
#98027=EDGE_CURVE ( 'NONE', #77732, #53564, #22567, .T. ) ;
#98028=CARTESIAN_POINT ( 'NONE',  ( 204.6941148245495583, 272.9778480757090620, -9.756815831893453250 ) ) ;
#98029=CARTESIAN_POINT ( 'NONE',  ( 204.2799274532736433, 276.8237820148827950, 13.55359442435934803 ) ) ;
#98031=ORIENTED_EDGE ( 'NONE', *, *, #27670, .F. ) ;
#98032=CARTESIAN_POINT ( 'NONE',  ( 88.13136219740870558, 215.5643266524159856, -9.188101187500093303 ) ) ;
#98033=CARTESIAN_POINT ( 'NONE',  ( 203.0984285455635074, 278.8701981521235211, 16.46020897279243300 ) ) ;
#98034=CARTESIAN_POINT ( 'NONE',  ( 179.1756939090309402, 269.5685363826416960, -17.30465729557930388 ) ) ;
#98035=CARTESIAN_POINT ( 'NONE',  ( -22.42236680055709641, 157.8615022471902591, 0.000000000000000000 ) ) ;
#98038=EDGE_CURVE ( 'NONE', #20654, #26223, #37096, .T. ) ;
#98039=CARTESIAN_POINT ( 'NONE',  ( -14.26183375581750568, 174.1199935810940644, 2.679491924311255158 ) ) ;
#98040=ORIENTED_EDGE ( 'NONE', *, *, #82849, .F. ) ;
#98044=CARTESIAN_POINT ( 'NONE',  ( 155.5211745099813356, 261.2764194263634749, -17.18163098020766810 ) ) ;
#98045=ORIENTED_EDGE ( 'NONE', *, *, #74575, .T. ) ;
#98046=CARTESIAN_POINT ( 'NONE',  ( 182.8487395599695731, 279.9155653989188295, -17.44888926691034925 ) ) ;
#98048=CYLINDRICAL_SURFACE ( 'NONE', #46237, 10.00000000000010658 ) ;
#98051=CARTESIAN_POINT ( 'NONE',  ( 156.9594519734722269, 258.7852497842161483, -18.40072354977459312 ) ) ;
#98052=ORIENTED_EDGE ( 'NONE', *, *, #69067, .F. ) ;
#98053=B_SPLINE_CURVE_WITH_KNOTS ( 'NONE', 3,
 ( #72282, #63654, #94593, #25147 ),
 .UNSPECIFIED., .F., .F.,
 ( 4, 4 ),
 ( 0.03384845726238354391, 0.04271176938863220640 ),
 .UNSPECIFIED. ) ;
#98058=CARTESIAN_POINT ( 'NONE',  ( 166.9003224155486294, 284.2591062721578510, 9.432497891095570353 ) ) ;
#98059=CARTESIAN_POINT ( 'NONE',  ( 199.8975600284485097, 270.2813002518563508, 9.754130713005407571 ) ) ;
#98060=VERTEX_POINT ( 'NONE', #28002 ) ;
#98062=CARTESIAN_POINT ( 'NONE',  ( 162.7644741734472120, 248.7306563947940958, 9.865755277559742353 ) ) ;
#98063=CARTESIAN_POINT ( 'NONE',  ( 159.9894443651313338, 253.5371490153152081, -16.36035038356864391 ) ) ;
#98064=CARTESIAN_POINT ( 'NONE',  ( 157.5297984379545255, 279.9475811940735639, -6.869905029983002898 ) ) ;
#98067=CARTESIAN_POINT ( 'NONE',  ( 159.3291946290163992, 279.0199804063916531, 10.96233109238993109 ) ) ;
#98071=CARTESIAN_POINT ( 'NONE',  ( 181.4968897611953480, 271.1066667875069243, -15.95701483517411567 ) ) ;
#98072=ORIENTED_EDGE ( 'NONE', *, *, #93908, .T. ) ;
#98073=CARTESIAN_POINT ( 'NONE',  ( 193.3401853099748564, 294.2072595941227178, -14.34885575185585260 ) ) ;
#98074=CARTESIAN_POINT ( 'NONE',  ( 171.4019447439835915, 279.6636507153484672, -14.71532880965975565 ) ) ;
#98077=CARTESIAN_POINT ( 'NONE',  ( 164.6388426154193780, 274.3663210464239341, 14.78880850689299997 ) ) ;
#98078=CARTESIAN_POINT ( 'NONE',  ( -6.076397627723526540, 176.4869531367911293, 4.594050593750046652 ) ) ;
#98081=CARTESIAN_POINT ( 'NONE',  ( 189.0710311799717829, 297.0389175199307488, 8.160305977522897436 ) ) ;
#98087=ADVANCED_FACE ( 'NONE', ( #73137 ), #3731, .T. ) ;
#98093=CARTESIAN_POINT ( 'NONE',  ( 11.29875767934929520, 168.1423013555409796, -4.594050593750043987 ) ) ;
#98094=CARTESIAN_POINT ( 'NONE',  ( 110.4040191812834735, 243.7369531367911009, -4.594050593750048428 ) ) ;
#98096=CARTESIAN_POINT ( 'NONE',  ( 186.4048238715421917, 296.5436351738768508, -7.262416587777808630 ) ) ;
#98099=CARTESIAN_POINT ( 'NONE',  ( 175.9236718092338663, 281.9243915816493313, -14.20169403765913430 ) ) ;
#98101=CARTESIAN_POINT ( 'NONE',  ( 193.7275870247597425, 295.1009717758319084, 14.48058678254265885 ) ) ;
#98102=CARTESIAN_POINT ( 'NONE',  ( 183.9879157655500705, 275.0531484184239162, 16.36130672943231801 ) ) ;
#98103=CARTESIAN_POINT ( 'NONE',  ( 147.8308140999695866, 274.5965143850199865, -7.866624397492971710 ) ) ;
#98106=CARTESIAN_POINT ( 'NONE',  ( 192.7546399067283858, 265.3065417519427456, 7.788706340340938006 ) ) ;
#98108=CARTESIAN_POINT ( 'NONE',  ( 184.0492996101627341, 268.5858911698572342, -15.15661456208596114 ) ) ;
#98112=CARTESIAN_POINT ( 'NONE',  ( 105.9391831106087380, 219.7202760586659736, -5.415160957724236172E-17 ) ) ;
#98114=CARTESIAN_POINT ( 'NONE',  ( 150.6431064791187850, 269.7254810985950257, 15.11064854015152470 ) ) ;
#98115=CARTESIAN_POINT ( 'NONE',  ( 157.5215017335775940, 258.4853116787141971, -16.92298772477023761 ) ) ;
#98116=CARTESIAN_POINT ( 'NONE',  ( 195.7291534503633272, 291.6341570319625021, 16.44925029361851543 ) ) ;
#98117=CARTESIAN_POINT ( 'NONE',  ( 200.1153681990099074, 284.0370102343983376, 18.51598427690537108 ) ) ;
#98118=CARTESIAN_POINT ( 'NONE',  ( 197.0696450891457516, 289.3123574064699710, 17.43500942416782706 ) ) ;
#98120=CARTESIAN_POINT ( 'NONE',  ( 173.2732189505960037, 267.9125929267007677, -16.31862377501282779 ) ) ;
#98123=CARTESIAN_POINT ( 'NONE',  ( 192.4259603496955719, 297.3554553095298729, -12.40738485318142814 ) ) ;
#98127=CYLINDRICAL_SURFACE ( 'NONE', #18393, 17.82106496071139645 ) ;
#98130=CARTESIAN_POINT ( 'NONE',  ( 191.5300323225266368, 288.3933188615314975, -15.83635432281777611 ) ) ;
#98132=( BOUNDED_CURVE ( )  B_SPLINE_CURVE ( 2, ( #63351, #63847, #7277, #60971, #100004, #17242, #84822, #79599, #87728 ),
 .UNSPECIFIED., .F., .T. ) 
 B_SPLINE_CURVE_WITH_KNOTS ( ( 3, 2, 2, 2, 3 ),
 ( 0.004032258064516129788, 0.005376344086021505805, 0.008064516129032257841, 0.01075268817204301161, 0.01209677419354838676 ),
 .UNSPECIFIED. ) 
 CURVE ( )  GEOMETRIC_REPRESENTATION_ITEM ( )  RATIONAL_B_SPLINE_CURVE ( ( 0.9330127018922194093, 0.9330127018922194093, 1.000000000000000000, 0.8660254037844387076, 1.000000000000000000, 0.8660254037844387076, 1.000000000000000000, 0.9330127018922192983, 0.9330127018922194093 ) ) 
 REPRESENTATION_ITEM ( '' )  );
#98135=CARTESIAN_POINT ( 'NONE',  ( 198.4706398937704819, 286.8857632237200619, 17.04020736381253798 ) ) ;
#98136=CARTESIAN_POINT ( 'NONE',  ( -27.42236680055714260, 166.5217562850347406, 1.224646799147364892E-15 ) ) ;
#98137=CARTESIAN_POINT ( 'NONE',  ( 171.4736130609155680, 253.3145436162068052, -8.798943912126190980 ) ) ;
#98138=CARTESIAN_POINT ( 'NONE',  ( 147.3907811248416522, 249.2365022471902023, -10.00000000000009059 ) ) ;
#98139=CARTESIAN_POINT ( 'NONE',  ( 204.7242223814549504, 276.0542406257275161, -13.93608974681376189 ) ) ;
#98144=CARTESIAN_POINT ( 'NONE',  ( 196.6049509491368781, 265.3221703615579941, -4.491441117979137587 ) ) ;
#98146=ORIENTED_EDGE ( 'NONE', *, *, #16841, .F. ) ;
#98148=ADVANCED_FACE ( 'NONE', ( #80584 ), #78551, .T. ) ;
#98149=ORIENTED_EDGE ( 'NONE', *, *, #23194, .F. ) ;
#98150=CARTESIAN_POINT ( 'NONE',  ( 47.79785968963117426, 191.7365022471902023, 10.00000000000009948 ) ) ;
#98151=EDGE_CURVE ( 'NONE', #64147, #69624, #858, .T. ) ;
#98152=CARTESIAN_POINT ( 'NONE',  ( 205.5867850959394900, 274.5602381795258111, 12.00218932530894378 ) ) ;
#98153=CARTESIAN_POINT ( 'NONE',  ( 192.3746808059117654, 279.8490869531318026, -16.68648498102840350 ) ) ;
#98154=CARTESIAN_POINT ( 'NONE',  ( 204.1006587545853677, 272.9409856097431657, 11.03402274723170606 ) ) ;
#98162=CARTESIAN_POINT ( 'NONE',  ( 167.8678039839016662, 276.4972622578981145, 15.08462999136594718 ) ) ;
#98163=B_SPLINE_CURVE_WITH_KNOTS ( 'NONE', 3,
 ( #34217, #33212, #18029, #19542, #17511, #48922, #63607, #71233, #10929, #79859, #64621, #1825, #94547, #86980, #64110, #41801, #95062, #25622, #56506, #87495, #72235, #2841, #49411, #72748, #3341, #65112, #96060, #26619, #29115, #99017, #21995, #81848, #20024, #13901, #12932, #90953, #82363, #89944 ),
 .UNSPECIFIED., .F., .F.,
 ( 4, 2, 2, 2, 2, 2, 2, 2, 2, 2, 2, 2, 2, 2, 2, 2, 2, 2, 4 ),
 ( 0.0009759269190796634021, 0.001069240376951313210, 0.001162553834822963126, 0.001349180750566163645, 0.001722434582052570105, 0.002468942245025379772, 0.003961957570971087576, 0.004708465233943942563, 0.005081719065430376561, 0.005268345981173551060, 0.005361659439045146983, 0.005454972896916742038, 0.005501629625852569490, 0.005548286354788396074, 0.005641599812660188888, 0.005828226728403780588, 0.006201480559890833882, 0.006574734391377886310, 0.006947988222864938737 ),
 .UNSPECIFIED. ) ;
#98167=EDGE_LOOP ( 'NONE', ( #34741, #6720, #4887, #64161 ) ) ;
#98168=CARTESIAN_POINT ( 'NONE',  ( 197.4075646047015482, 273.1427705089788560, -14.69744958829762815 ) ) ;
#98170=CARTESIAN_POINT ( 'NONE',  ( 162.2256012757624433, 272.3419497268096734, -16.04947957637165956 ) ) ;
#98171=CARTESIAN_POINT ( 'NONE',  ( 165.0807124393095364, 244.7188140358855151, -1.586079993046279446 ) ) ;
#98175=CARTESIAN_POINT ( 'NONE',  ( 171.0137737332507584, 287.8132002576012383, -4.438399254829208829 ) ) ;
#98177=CARTESIAN_POINT ( 'NONE',  ( 178.2715496052864523, 255.5664410081183746, 4.888700057109781838 ) ) ;
#98178=CARTESIAN_POINT ( 'NONE',  ( 106.6698052711106186, 223.2048013555410080, 4.594050593750051981 ) ) ;
#98180=CARTESIAN_POINT ( 'NONE',  ( 188.4925541850777506, 273.6131829772801325, 15.65818043819186478 ) ) ;
#98181=VERTEX_POINT ( 'NONE', #63332 ) ;
#98182=ORIENTED_EDGE ( 'NONE', *, *, #39884, .T. ) ;
#98185=CARTESIAN_POINT ( 'NONE',  ( 157.8740713127050981, 257.2010826190796706, 17.31862062017425075 ) ) ;
#98186=CARTESIAN_POINT ( 'NONE',  ( 206.1798448551755598, 273.5330285446045195, -10.53862763475382813 ) ) ;
#98188=B_SPLINE_CURVE_WITH_KNOTS ( 'NONE', 3,
 ( #69950, #567, #24369, #85731 ),
 .UNSPECIFIED., .F., .F.,
 ( 4, 4 ),
 ( 0.009256042836502432342, 0.01507217474330474830 ),
 .UNSPECIFIED. ) ;
#98191=CARTESIAN_POINT ( 'NONE',  ( 163.1369207721744772, 248.0855599626920593, -11.24692769914530110 ) ) ;
#98193=B_SPLINE_CURVE_WITH_KNOTS ( 'NONE', 3,
 ( #3568, #26855, #96286, #50147, #33975, #72977, #57236, #58237, #56745, #11176, #12156, #87727, #88711, #95313, #43018, #2569, #42043, #82094, #34449, #42529, #3084, #18265, #64349, #49159, #80095, #10661, #57731, #65347, #73462, #81100, #41537, #19280, #95806, #50634, #11667, #34935, #65830, #88211, #19765, #51132, #73957, #96796, #27355, #64859, #72482, #4542, #89217, #27845, #18762, #81587, #97278, #49640 ),
 .UNSPECIFIED., .F., .F.,
 ( 4, 2, 2, 2, 2, 2, 2, 2, 2, 2, 2, 2, 2, 2, 2, 2, 2, 2, 2, 2, 2, 2, 2, 2, 2, 4 ),
 ( 0.0001991101052095526139, 0.001225461298171744411, 0.001738636894652840310, 0.001866930793773159550, 0.001995224692893479007, 0.002123518592013798247, 0.002251812491134116186, 0.002380106390254435426, 0.002508400289374754667, 0.002764988087615294268, 0.003278163684096418139, 0.004304514877058586951, 0.005330866070020754896, 0.005844041666501914763, 0.006100629464742417934, 0.006357217262982921106, 0.006421364212543102627, 0.006485511162103285016, 0.006549658111663465669, 0.006613805061223648057, 0.006870392859464352457, 0.007383568455945755185, 0.007640156254186507290, 0.007896744052427259394, 0.008153331850668011499, 0.008409919648908761869 ),
 .UNSPECIFIED. ) ;
#98195=CARTESIAN_POINT ( 'NONE',  ( 103.5583290153452083, 219.0494855054051868, -2.679491924311248496 ) ) ;
#98198=CARTESIAN_POINT ( 'NONE',  ( 184.1873351008822226, 288.8905979614012836, -14.49962578542382907 ) ) ;
#98202=CARTESIAN_POINT ( 'NONE',  ( 59.25465409031482977, 215.0177522451419065, 5.000000000000046185 ) ) ;
#98205=CARTESIAN_POINT ( 'NONE',  ( 170.2455760408510912, 248.6530624101944511, -0.2700544060848846795 ) ) ;
#98206=CARTESIAN_POINT ( 'NONE',  ( 178.3183837364390172, 285.6435033645693125, 14.40467033256238949 ) ) ;
#98208=CARTESIAN_POINT ( 'NONE',  ( 196.4434894085402163, 280.3196924634482912, -16.68800359730008864 ) ) ;
#98210=VECTOR ( 'NONE', #93465, 1000.000000000000000 ) ;
#98213=CARTESIAN_POINT ( 'NONE',  ( 61.47358386746269332, 215.4869531367911009, 4.594050593750046652 ) ) ;
#98214=CARTESIAN_POINT ( 'NONE',  ( 159.2651917302844993, 254.7915913763855258, -16.53922207549818424 ) ) ;
#98216=CARTESIAN_POINT ( 'NONE',  ( 208.3764315856425640, 269.7284287242038658, -1.833640725398759441 ) ) ;
#98217=EDGE_CURVE ( 'NONE', #29718, #23380, #86678, .T. ) ;
#98218=CARTESIAN_POINT ( 'NONE',  ( 197.3443028699994954, 288.4215049135930826, -16.72861298487629256 ) ) ;
#98220=CARTESIAN_POINT ( 'NONE',  ( 161.7767236248226084, 250.4414905302161287, -13.15904643207033153 ) ) ;
#98221=CARTESIAN_POINT ( 'NONE',  ( 195.3506579275178581, 288.6704280282520472, 17.27067453383686768 ) ) ;
#98222=AXIS2_PLACEMENT_3D ( 'NONE', #80912, #66153, #11484 ) ;
#98230=CARTESIAN_POINT ( 'NONE',  ( 28.37560933628243731, 181.0643266524159856, -9.188101187500093303 ) ) ;
#98231=CARTESIAN_POINT ( 'NONE',  ( 196.4390255720217908, 290.4046224503736653, 16.34739044515864848 ) ) ;
#98233=B_SPLINE_CURVE_WITH_KNOTS ( 'NONE', 3,
 ( #16773, #79629, #95347, #63381, #32487, #54764, #94320, #85747, #63880, #8681, #41059, #16275, #25903, #47170, #1088, #55750, #47666, #71503, #10194, #39551, #71001, #2600, #1604, #33487, #94815, #49193, #86742, #10690, #64384, #78598, #56775, #87758, #86238, #41569, #48181, #72512, #79126, #34006, #62870, #2095, #93827, #32973, #55255, #9184, #44051, #51163, #35472, #49673 ),
 .UNSPECIFIED., .F., .F.,
 ( 4, 2, 2, 2, 2, 2, 2, 2, 2, 2, 2, 2, 2, 2, 2, 2, 2, 2, 2, 2, 2, 2, 2, 4 ),
 ( 0.001675801244915591480, 0.002130441261090271210, 0.002585081277264950940, 0.002812401285352291239, 0.002926061289395960954, 0.003039721293439630670, 0.003153381297483300819, 0.003267041301526970969, 0.003494361309614205449, 0.003949001325788674410, 0.004403641341963143371, 0.005312921374312083028, 0.006222201406661022685, 0.006676841422835528943, 0.007131481439010035200, 0.007245141443053576547, 0.007301971445075379312, 0.007358801447097183812, 0.007472461451140789343, 0.007586121455184395741, 0.008040761471358938428, 0.008495401487533481982, 0.008722721495620708657, 0.008950041503707935331 ),
 .UNSPECIFIED. ) ;
#98236=CARTESIAN_POINT ( 'NONE',  ( 58.36173894231862391, 198.3768266524160140, 9.188101187500096856 ) ) ;
#98237=B_SPLINE_CURVE_WITH_KNOTS ( 'NONE', 3,
 ( #67906, #44084, #44582, #15174 ),
 .UNSPECIFIED., .F., .F.,
 ( 4, 4 ),
 ( 0.008175067078588206526, 0.01423883080510260878 ),
 .UNSPECIFIED. ) ;
#98239=CARTESIAN_POINT ( 'NONE',  ( 151.3898985249405200, 268.4319993325432847, -14.65018536945715510 ) ) ;
#98240=CARTESIAN_POINT ( 'NONE',  ( -6.929581007982106300, 155.2592609112379876, 2.679491924311252937 ) ) ;
#98242=CARTESIAN_POINT ( 'NONE',  ( 200.9253810108797893, 268.8241845523467646, -6.444322578389119371 ) ) ;
#98243=CARTESIAN_POINT ( 'NONE',  ( 175.5883609201405022, 291.0961144979737014, 2.242416747171071645 ) ) ;
#98244=CARTESIAN_POINT ( 'NONE',  ( 180.1079967660572265, 276.2603422707981622, 17.03935691071084335 ) ) ;
#98247=CARTESIAN_POINT ( 'NONE',  ( 191.4207474145670460, 266.7759722589373723, 10.87581393504784444 ) ) ;
#98249=CARTESIAN_POINT ( 'NONE',  ( 90.23310447506860044, 236.2365022471903444, 2.944929066748280225E-16 ) ) ;
#98250=CARTESIAN_POINT ( 'NONE',  ( 161.4396252346964218, 251.0253620690641299, 14.51972485405798885 ) ) ;
#98252=CARTESIAN_POINT ( 'NONE',  ( 165.1203120823259098, 270.0476859643460443, -16.31784969181675748 ) ) ;
#98253=VERTEX_POINT ( 'NONE', #71952 ) ;
#98254=CARTESIAN_POINT ( 'NONE',  ( 59.55217677675723564, 211.3149278399160949, -9.188101187500095079 ) ) ;
#98255=ORIENTED_EDGE ( 'NONE', *, *, #69275, .F. ) ;
#98256=CARTESIAN_POINT ( 'NONE',  ( 166.0902180206555556, 265.3285796677840267, 16.55597451408016596 ) ) ;
#98257=CARTESIAN_POINT ( 'NONE',  ( 162.3203620077491962, 250.6751068356387577, 12.61930170232072435 ) ) ;
#98259=ORIENTED_EDGE ( 'NONE', *, *, #56472, .F. ) ;
#98260=CARTESIAN_POINT ( 'NONE',  ( 177.8194257969418288, 292.8449071177858514, 6.006967295066290013 ) ) ;
#98262=EDGE_CURVE ( 'NONE', #39107, #45874, #69561, .T. ) ;
#98263=CARTESIAN_POINT ( 'NONE',  ( 150.5780525126727980, 271.8381578737140103, 12.98431582152410968 ) ) ;
#98264=CARTESIAN_POINT ( 'NONE',  ( 177.2352494820021889, 274.8154387795073603, -16.96091352554584475 ) ) ;
#98267=CARTESIAN_POINT ( 'NONE',  ( 204.4814917997891541, 276.4746623257233296, 13.21872368206963877 ) ) ;
#98272=CARTESIAN_POINT ( 'NONE',  ( 174.9188381007038799, 255.1700493696978356, 8.143286963564044356 ) ) ;
#98275=ORIENTED_EDGE ( 'NONE', *, *, #91175, .T. ) ;
#98277=CARTESIAN_POINT ( 'NONE',  ( 167.0235062565406565, 261.5460872093962053, 16.43802016297843238 ) ) ;
#98278=CARTESIAN_POINT ( 'NONE',  ( 206.8313602288537538, 272.4045708154811791, -9.607337080360906612 ) ) ;
#98281=CARTESIAN_POINT ( 'NONE',  ( 162.7117101085248407, 283.4291563370742892, -3.114432215248377211 ) ) ;
#98282=CARTESIAN_POINT ( 'NONE',  ( 149.2678550509543811, 265.6471520882315076, -1.519623991172851672E-15 ) ) ;
#98283=CARTESIAN_POINT ( 'NONE',  ( 162.6425574510925003, 248.9418223522047526, -10.70838742014210077 ) ) ;
#98287=CARTESIAN_POINT ( 'NONE',  ( 205.1786601861764723, 272.2841766866060311, 10.06407076913277088 ) ) ;
#98288=CARTESIAN_POINT ( 'NONE',  ( 127.7791744883563183, 235.3923013555409796, 4.594050593750050204 ) ) ;
#98291=CARTESIAN_POINT ( 'NONE',  ( 170.4674085893365714, 263.7776824676311662, 15.83595988821661571 ) ) ;
#98296=ORIENTED_EDGE ( 'NONE', *, *, #10202, .T. ) ;
#98297=ORIENTED_EDGE ( 'NONE', *, *, #26633, .F. ) ;
#98300=CARTESIAN_POINT ( 'NONE',  ( 194.1740526473003001, 284.7360119068420090, 17.59213183599199937 ) ) ;
#98303=CARTESIAN_POINT ( 'NONE',  ( 194.2199708651012600, 294.2481379475345875, 15.50834247347371253 ) ) ;
#98304=CARTESIAN_POINT ( 'NONE',  ( 172.0455612308954869, 276.6794935234722743, 15.97629919534607268 ) ) ;
#98309=CARTESIAN_POINT ( 'NONE',  ( 153.3859906278383676, 264.9746663937372091, -17.41799046551451013 ) ) ;
#98311=ORIENTED_EDGE ( 'NONE', *, *, #9042, .F. ) ;
#98318=CARTESIAN_POINT ( 'NONE',  ( 191.0907015319009474, 260.9773198129059324, -3.629663310244437557 ) ) ;
#98319=CARTESIAN_POINT ( 'NONE',  ( 195.3647503060396957, 279.2613744222268792, 16.32278432642107902 ) ) ;
#98320=CARTESIAN_POINT ( 'NONE',  ( 207.6932907333322191, 270.9116633891313199, 2.120963121341169710 ) ) ;
#98321=CARTESIAN_POINT ( 'NONE',  ( 129.3483248890680954, 254.6744531367911577, 4.594050593750047540 ) ) ;
#98322=EDGE_LOOP ( 'NONE', ( #98542, #4192, #8697, #24460 ) ) ;
#98324=CARTESIAN_POINT ( 'NONE',  ( 182.1029699310405761, 257.8865440850851769, 6.538144971207902501 ) ) ;
#98325=CARTESIAN_POINT ( 'NONE',  ( 155.9473334272112197, 262.0296148265339298, -16.96532868042320885 ) ) ;
#98330=CARTESIAN_POINT ( 'NONE',  ( 182.1025678104670646, 275.6566577031950374, -16.43659905335109173 ) ) ;
#98331=CARTESIAN_POINT ( 'NONE',  ( 164.8584712946003776, 247.1261223207595492, -5.618710548772211766 ) ) ;
#98335=CARTESIAN_POINT ( 'NONE',  ( 184.5457051153594534, 294.3635293766698169, 10.03055039675435367 ) ) ;
#98336=CARTESIAN_POINT ( 'NONE',  ( 183.8274263638271577, 281.3324037098167310, 17.41033114534894111 ) ) ;
#98339=CARTESIAN_POINT ( 'NONE',  ( 192.9333490033828298, 268.2698727311234848, 12.60046548449609283 ) ) ;
#98343=CARTESIAN_POINT ( 'NONE',  ( 190.0707697440390689, 301.4347651000360884, 4.271360729158901748 ) ) ;
#98345=DIRECTION ( 'NONE',  ( -0.8660254037844387076, -0.4999999999999998890, -0.000000000000000000 ) ) ;
#98346=CARTESIAN_POINT ( 'NONE',  ( 159.2511875226268216, 254.8158473755685520, 15.75855490706745599 ) ) ;
#98347=EDGE_CURVE ( 'NONE', #69911, #38470, #24888, .T. ) ;
#98348=CARTESIAN_POINT ( 'NONE',  ( 161.2538201723544944, 251.3471858773438328, 13.36125779146621362 ) ) ;
#98350=CARTESIAN_POINT ( 'NONE',  ( 141.9600801517287607, 252.7677522451418497, 10.00000000000009592 ) ) ;
#98352=CARTESIAN_POINT ( 'NONE',  ( 172.9104462670787257, 284.5517195599988440, -12.97937505523477064 ) ) ;
#98356=CARTESIAN_POINT ( 'NONE',  ( 198.8533049117289977, 286.2229679703367538, -18.60939981449148561 ) ) ;
#98357=CARTESIAN_POINT ( 'NONE',  ( 12.46239254174337852, 171.8768266524159856, -9.188101187500093303 ) ) ;
#98358=CARTESIAN_POINT ( 'NONE',  ( 178.6255663458269112, 259.3103340517776587, -10.56300147729930927 ) ) ;
#98361=CARTESIAN_POINT ( 'NONE',  ( 63.56442718099752653, 219.0530062829863027, -4.648177544792955347E-16 ) ) ;
#98364=B_SPLINE_SURFACE_WITH_KNOTS ( 'NONE', 3, 1, ( 
 ( #16576, #79926 ),
 ( #1892, #87048 ),
 ( #46981, #24675 ),
 ( #63177, #72305 ),
 ( #71803, #94121 ),
 ( #95129, #55557 ),
 ( #48488, #79429 ),
 ( #47963, #86542 ),
 ( #33279, #87561 ),
 ( #18092, #41366 ),
 ( #62160, #23661 ),
 ( #54552, #16078 ),
 ( #70270, #881 ),
 ( #31759, #17073 ),
 ( #47474, #78398 ),
 ( #9494, #40361 ),
 ( #34282, #43861 ),
 ( #27694, #34769 ),
 ( #20589, #82439 ),
 ( #11508, #49475 ),
 ( #19611, #35776 ),
 ( #66183, #51471 ),
 ( #65179, #19106 ),
 ( #97128, #13002 ),
 ( #74312, #2913 ),
 ( #4377, #96127 ),
 ( #33806, #58565 ),
 ( #66671, #96625 ),
 ( #12496, #81423 ),
 ( #97607, #89536 ),
 ( #27190, #4894 ),
 ( #41878, #28174 ),
 ( #42852, #64689 ),
 ( #65670, #35276 ) ),
 .UNSPECIFIED., .T., .F., .F.,
 ( 4, 2, 2, 2, 2, 2, 2, 2, 2, 2, 2, 2, 2, 2, 2, 2, 4 ),
 ( 2, 2 ),
 ( 0.000000000000000000, 0.06250000000000000000, 0.1250000000000000000, 0.1875000000000000000, 0.2500000000000000000, 0.3125000000000000000, 0.3750000000000000000, 0.4375000000000000000, 0.5000000000000000000, 0.5625000000000000000, 0.6250000000000000000, 0.6875000000000000000, 0.7500000000000000000, 0.8125000000000000000, 0.8750000000000000000, 0.9375000000000000000, 1.000000000000000000 ),
 ( 0.000000000000000000, 1.000000000000000000 ),
 .UNSPECIFIED. ) ;
#98365=CARTESIAN_POINT ( 'NONE',  ( 199.4209461648062529, 270.9799452176341674, -11.09900091224045582 ) ) ;
#98366=CARTESIAN_POINT ( 'NONE',  ( 77.00817486789590305, 205.2677522451417929, -5.000000000000041744 ) ) ;
#98368=CARTESIAN_POINT ( 'NONE',  ( 150.2982063762752603, 270.3228656002555681, 14.90512853129094495 ) ) ;
#98369=CARTESIAN_POINT ( 'NONE',  ( 45.12761469462908792, 206.8615022471902876, 5.000000000000046185 ) ) ;
#98370=FACE_OUTER_BOUND ( 'NONE', #75119, .T. ) ;
#98373=CARTESIAN_POINT ( 'NONE',  ( 148.3930300673291640, 273.6227277647267897, 8.375036249079425232 ) ) ;
#98374=CARTESIAN_POINT ( 'NONE',  ( 12.78680497239753144, 184.3149278399160949, -9.188101187500095079 ) ) ;
#98375=CARTESIAN_POINT ( 'NONE',  ( 164.4110119407497734, 285.3093287471372719, 4.354449836773983229 ) ) ;
#98378=CARTESIAN_POINT ( 'NONE',  ( 202.1480882124455718, 280.0251659497182004, -15.78546128548377681 ) ) ;
#98379=CARTESIAN_POINT ( 'NONE',  ( 206.8986117509267899, 272.2880877623646825, 6.975890063856878598 ) ) ;
#98380=CARTESIAN_POINT ( 'NONE',  ( 186.0194694746173241, 266.9068538997193514, 13.20651731842044718 ) ) ;
#98382=CARTESIAN_POINT ( 'NONE',  ( 160.2301616673542242, 280.0696522150809074, 9.247322956015198159 ) ) ;
#98388=CARTESIAN_POINT ( 'NONE',  ( 193.9495889092963807, 294.7164532324382549, 15.46986001312306058 ) ) ;
#98389=ORIENTED_EDGE ( 'NONE', *, *, #54975, .F. ) ;
#98390=CARTESIAN_POINT ( 'NONE',  ( 182.6812089762738651, 289.5349527171500199, 12.27369044368959905 ) ) ;
#98393=CARTESIAN_POINT ( 'NONE',  ( 182.8075329105516289, 285.5996758505444291, -15.91971760981349071 ) ) ;
#98394=ORIENTED_EDGE ( 'NONE', *, *, #46881, .F. ) ;
#98398=CARTESIAN_POINT ( 'NONE',  ( 203.5080190724872011, 278.1607665491929993, -15.47044080916498743 ) ) ;
#98399=EDGE_LOOP ( 'NONE', ( #26825, #3097, #14927, #39227, #61846, #11491, #79804, #44431, #57753, #64782, #99928, #62990, #37702, #23310, #81188, #96069, #58530, #75052, #22229, #78366, #44033, #72972 ) ) ;
#98402=CARTESIAN_POINT ( 'NONE',  ( 153.1164404339926080, 265.4415410246681972, 16.15325778160653414 ) ) ;
#98403=EDGE_LOOP ( 'NONE', ( #77454, #2740, #16789, #6704 ) ) ;
#98404=CARTESIAN_POINT ( 'NONE',  ( 190.8094645593471341, 300.1553081486349015, 8.399847186519689757 ) ) ;
#98407=CARTESIAN_POINT ( 'NONE',  ( 45.83126033165601854, 207.2677522451419350, -5.000000000000047962 ) ) ;
#98410=CARTESIAN_POINT ( 'NONE',  ( 149.3629284598386278, 271.9428144707212027, -12.99253781774931049 ) ) ;
#98412=EDGE_CURVE ( 'NONE', #32891, #20583, #45335, .T. ) ;
#98415=CARTESIAN_POINT ( 'NONE',  ( 165.0297293518065658, 244.8071193337670195, 2.517333243890161665 ) ) ;
#98416=CARTESIAN_POINT ( 'NONE',  ( 149.4378998887816294, 275.3713422307953351, -8.174376149720645301 ) ) ;
#98418=CARTESIAN_POINT ( 'NONE',  ( 174.5168695141670696, 276.9147204147473076, -15.82766731710391284 ) ) ;
#98419=CARTESIAN_POINT ( 'NONE',  ( 172.2673562241199363, 264.0187931579786778, -15.69345930386550947 ) ) ;
#98420=ORIENTED_EDGE ( 'NONE', *, *, #80960, .T. ) ;
#98421=CARTESIAN_POINT ( 'NONE',  ( 158.7066903866863754, 275.0672323892235340, -12.54353524617913074 ) ) ;
#98422=CARTESIAN_POINT ( 'NONE',  ( 91.96515528263753936, 217.2365022471902876, 10.00000000000009948 ) ) ;
#98423=CARTESIAN_POINT ( 'NONE',  ( 162.7006039569504594, 261.3497057169571463, 17.57720365097131676 ) ) ;
#98425=ORIENTED_EDGE ( 'NONE', *, *, #43374, .F. ) ;
#98428=( BOUNDED_CURVE ( )  B_SPLINE_CURVE ( 2, ( #13686, #46052, #60748, #99296, #67884, #90735, #45071, #44559, #75494 ),
 .UNSPECIFIED., .F., .T. ) 
 B_SPLINE_CURVE_WITH_KNOTS ( ( 3, 2, 2, 2, 3 ),
 ( 0.06048387096774193727, 0.06182795698924731242, 0.06451612903225806273, 0.06720430107526881303, 0.06854838709677418818 ),
 .UNSPECIFIED. ) 
 CURVE ( )  GEOMETRIC_REPRESENTATION_ITEM ( )  RATIONAL_B_SPLINE_CURVE ( ( 0.9330127018922194093, 0.9330127018922194093, 1.000000000000000000, 0.8660254037844387076, 1.000000000000000000, 0.8660254037844387076, 1.000000000000000000, 0.9330127018922194093, 0.9330127018922194093 ) ) 
 REPRESENTATION_ITEM ( '' )  );
#98430=CARTESIAN_POINT ( 'NONE',  ( 147.5634954182374372, 275.0595239235922236, 4.682022975662822439 ) ) ;
#98432=CARTESIAN_POINT ( 'NONE',  ( 190.0274641710971082, 301.5097725526222803, 3.738976720635653450 ) ) ;
#98433=CARTESIAN_POINT ( 'NONE',  ( 152.7314557461996571, 266.1083540640618708, 17.39314074348802208 ) ) ;
#98434=CARTESIAN_POINT ( 'NONE',  ( 147.2428775945425912, 275.6148502840442234, 0.4280630669697413349 ) ) ;
#98435=CARTESIAN_POINT ( 'NONE',  ( 146.6834825911944620, 276.5837508513432681, 0.6716460511724984261 ) ) ;
#98436=CIRCLE ( 'NONE', #19191, 17.82106496071138935 ) ;
#98439=CARTESIAN_POINT ( 'NONE',  ( 149.9885642792388865, 274.4180868986143196, -10.02378587638088092 ) ) ;
#98442=CARTESIAN_POINT ( 'NONE',  ( 171.1714030391351855, 288.3798238850056919, 4.167722100051413747 ) ) ;
#98443=CARTESIAN_POINT ( 'NONE',  ( 165.4826352078684408, 255.7221904534726775, -15.26429383359580960 ) ) ;
#98444=ORIENTED_EDGE ( 'NONE', *, *, #25704, .F. ) ;
#98445=CARTESIAN_POINT ( 'NONE',  ( 190.6416006417717597, 300.4460569826327969, -3.339060657009423672 ) ) ;
#98447=CARTESIAN_POINT ( 'NONE',  ( 202.5155473443252561, 279.0643611876510022, 15.50872832146021807 ) ) ;
#98449=CARTESIAN_POINT ( 'NONE',  ( 171.2741013746033332, 249.3936815359432728, 2.927055546763141169 ) ) ;
#98451=ORIENTED_EDGE ( 'NONE', *, *, #77743, .F. ) ;
#98452=CARTESIAN_POINT ( 'NONE',  ( 170.7628550155183973, 255.3019951891120058, -12.90626094114390909 ) ) ;
#98455=CARTESIAN_POINT ( 'NONE',  ( 155.5311623832600958, 261.6886619413561448, 17.00987194985870943 ) ) ;
#98456=CARTESIAN_POINT ( 'NONE',  ( 44.60439100962805981, 209.8927522451419350, 2.944929066748280225E-16 ) ) ;
#98457=CARTESIAN_POINT ( 'NONE',  ( 111.8924135700967497, 247.6589784336661069, -6.496448406907676862E-16 ) ) ;
#98458=CARTESIAN_POINT ( 'NONE',  ( 180.5928094756065434, 294.4055607231725844, -3.443643769660447163 ) ) ;
#98460=CARTESIAN_POINT ( 'NONE',  ( 157.1338510812060747, 258.4831816688264325, 17.88958125218800888 ) ) ;
#98462=CARTESIAN_POINT ( 'NONE',  ( 33.57141466322406131, 196.3149278399160949, -9.188101187500095079 ) ) ;
#98464=CARTESIAN_POINT ( 'NONE',  ( 147.6166281148981625, 275.4172840431396594, -2.962624894996066960 ) ) ;
#98465=ORIENTED_EDGE ( 'NONE', *, *, #33774, .T. ) ;
#98466=CARTESIAN_POINT ( 'NONE',  ( 94.74134171723733289, 237.0530062829862743, -4.648177544792955347E-16 ) ) ;
#98467=CARTESIAN_POINT ( 'NONE',  ( 178.0159405646096218, 265.6579100072215169, 15.49631030714943414 ) ) ;
#98468=ADVANCED_FACE ( 'NONE', ( #30826 ), #57222, .F. ) ;
#98470=CARTESIAN_POINT ( 'NONE',  ( 146.7879906441258129, 276.4027375938661635, 4.347255311287614887 ) ) ;
#98474=CARTESIAN_POINT ( 'NONE',  ( 176.4155233639579876, 285.5687499269977252, -12.04987988516876385 ) ) ;
#98475=CARTESIAN_POINT ( 'NONE',  ( 182.0096190830649618, 262.8089543526228340, 12.58302938569931939 ) ) ;
#98476=B_SPLINE_CURVE_WITH_KNOTS ( 'NONE', 3,
 ( #83439, #12022, #37293, #50994 ),
 .UNSPECIFIED., .F., .F.,
 ( 4, 4 ),
 ( 0.02524082176100830507, 0.03448714665262276463 ),
 .UNSPECIFIED. ) ;
#98477=CARTESIAN_POINT ( 'NONE',  ( 102.9889369814290632, 220.2677522451417929, -5.000000000000041744 ) ) ;
#98480=CARTESIAN_POINT ( 'NONE',  ( 171.6154833087297789, 255.2606305366970503, 12.53362356821959978 ) ) ;
#98482=CARTESIAN_POINT ( 'NONE',  ( 155.3653809515997750, 279.8371988227073643, -2.156620399925142539 ) ) ;
#98483=CARTESIAN_POINT ( 'NONE',  ( 163.4084407101100851, 247.6152736349200438, -10.68829614238923931 ) ) ;
#98484=CARTESIAN_POINT ( 'NONE',  ( 7.915412076110063033, 181.5024278399160664, -9.188101187500093303 ) ) ;
#98485=AXIS2_PLACEMENT_3D ( 'NONE', #65372, #32481, #59237 ) ;
#98487=CARTESIAN_POINT ( 'NONE',  ( 192.8217334130199276, 272.2506572471322670, 14.19735341291291064 ) ) ;
#98490=CARTESIAN_POINT ( 'NONE',  ( 61.28457468009112574, 200.0643266524160424, 9.188101187500095079 ) ) ;
#98491=CARTESIAN_POINT ( 'NONE',  ( 163.8455942243524248, 246.8581015375447691, -7.178103170949780676 ) ) ;
#98492=CARTESIAN_POINT ( 'NONE',  ( 164.4990934228277411, 245.7262077230798809, 6.470820838822735510 ) ) ;
#98494=CARTESIAN_POINT ( 'NONE',  ( 164.8329445879545290, 245.1479605429143760, -2.955380775890217304 ) ) ;
#98495=ORIENTED_EDGE ( 'NONE', *, *, #12126, .F. ) ;
#98497=CARTESIAN_POINT ( 'NONE',  ( 165.2263101757220909, 269.2500600554935772, 17.42067060345640073 ) ) ;
#98498=CARTESIAN_POINT ( 'NONE',  ( 22.68312297988245518, 177.2365022471902023, -10.00000000000009059 ) ) ;
#98499=CARTESIAN_POINT ( 'NONE',  ( 208.2764314485352770, 269.9016340424377063, 2.433736665191914117 ) ) ;
#98500=CARTESIAN_POINT ( 'NONE',  ( 135.5734031224162663, 239.8923013555409796, 4.594050593750050204 ) ) ;
#98504=CARTESIAN_POINT ( 'NONE',  ( 63.68045258478197468, 219.1199935810940644, 2.679491924311251605 ) ) ;
#98506=CARTESIAN_POINT ( 'NONE',  ( 189.0837441151423377, 289.7671154662007780, 14.43762572592019211 ) ) ;
#98508=ORIENTED_EDGE ( 'NONE', *, *, #29598, .F. ) ;
#98509=CARTESIAN_POINT ( 'NONE',  ( 167.6010540021560189, 247.4270797612363708, 3.638657435017179864 ) ) ;
#98510=CARTESIAN_POINT ( 'NONE',  ( 163.9926361355883273, 246.6034174764422175, 7.548074001043944214 ) ) ;
#98512=CARTESIAN_POINT ( 'NONE',  ( 169.6866200653663270, 266.0524855449860979, -17.34380911347102483 ) ) ;
#98513=CARTESIAN_POINT ( 'NONE',  ( 194.5288312044114889, 271.4546633457422331, -13.52122573599391764 ) ) ;
#98516=CARTESIAN_POINT ( 'NONE',  ( 144.9899443387551798, 254.5170451491295296, 0.000000000000000000 ) ) ;
#98519=CARTESIAN_POINT ( 'NONE',  ( 192.4071554788542926, 293.6259026860700487, -14.64098184119582591 ) ) ;
#98524=CARTESIAN_POINT ( 'NONE',  ( 194.5423442527744271, 283.0110300053098058, 17.49863978369591422 ) ) ;
#98526=CARTESIAN_POINT ( 'NONE',  ( 172.3604664900529428, 278.3133719434953264, 16.43090493882906244 ) ) ;
#98531=EDGE_LOOP ( 'NONE', ( #94183, #63160, #69053, #44418 ) ) ;
#98532=CARTESIAN_POINT ( 'NONE',  ( 147.2229325088103735, 275.6493961858936927, -0.4918294119671829390 ) ) ;
#98534=CARTESIAN_POINT ( 'NONE',  ( 204.1780753366177237, 277.0001950557890495, 14.05599973203924158 ) ) ;
#98536=CARTESIAN_POINT ( 'NONE',  ( 49.43738778531180600, 210.8967562850346837, -4.648177544792955347E-16 ) ) ;
#98538=CARTESIAN_POINT ( 'NONE',  ( 90.89164462408909628, 223.2833772461660260, -9.188101187500095079 ) ) ;
#98539=CARTESIAN_POINT ( 'NONE',  ( 171.9473113485260285, 253.3425154589238275, -10.37853918848434809 ) ) ;
#98540=CARTESIAN_POINT ( 'NONE',  ( 181.3431098572050644, 271.2290024631702750, -15.98888968998948812 ) ) ;
#98542=ORIENTED_EDGE ( 'NONE', *, *, #5709, .F. ) ;
#98546=DIRECTION ( 'NONE',  ( -0.8660254037844387076, -0.4999999999999998890, -0.000000000000000000 ) ) ;
#98548=EDGE_CURVE ( 'NONE', #75611, #104, #97408, .T. ) ;
#98552=CARTESIAN_POINT ( 'NONE',  ( 207.2631600302859738, 271.6566716207027525, -6.785208696633175940 ) ) ;
#98555=DIRECTION ( 'NONE',  ( -0.8660254037844387076, -0.4999999999999998890, -0.000000000000000000 ) ) ;
#98557=CARTESIAN_POINT ( 'NONE',  ( 199.4720805209845196, 266.1420231043892954, 4.760232788326643316 ) ) ;
#98560=CARTESIAN_POINT ( 'NONE',  ( 195.6062856355109432, 291.8469703299019216, -17.24264465766131593 ) ) ;
#98561=ORIENTED_EDGE ( 'NONE', *, *, #85203, .T. ) ;
#98562=CYLINDRICAL_SURFACE ( 'NONE', #14016, 10.00000000000010658 ) ;
#98566=CARTESIAN_POINT ( 'NONE',  ( 167.0583404026868948, 284.2888315039880354, 9.398654938006481885 ) ) ;
#98568=CARTESIAN_POINT ( 'NONE',  ( 206.7927593038066618, 270.4714295788825780, 5.070506503021109168 ) ) ;
#98570=CARTESIAN_POINT ( 'NONE',  ( 202.2576150004249200, 280.3265299319959354, 16.24828394350762295 ) ) ;
#98571=CARTESIAN_POINT ( 'NONE',  ( 188.4457029989130490, 260.4214235001608131, 2.263077359424293444 ) ) ;
#98572=CARTESIAN_POINT ( 'NONE',  ( 152.2916497645251184, 277.1968680821945554, -5.228018422121015973 ) ) ;
#98576=CARTESIAN_POINT ( 'NONE',  ( 194.4679394788272475, 262.6816651586079843, -0.8071362648469233569 ) ) ;
#98577=AXIS2_PLACEMENT_3D ( 'NONE', #39331, #17047, #8457 ) ;
#98579=CARTESIAN_POINT ( 'NONE',  ( 155.4639880231617042, 261.3754693270417420, -18.58538060562953120 ) ) ;
#98582=CARTESIAN_POINT ( 'NONE',  ( 4.352251933111777049, 179.9865022471903160, -10.00000000000009592 ) ) ;
#98583=CARTESIAN_POINT ( 'NONE',  ( -8.728340106763610606, 175.7677522451419350, -5.000000000000047962 ) ) ;
#98584=CARTESIAN_POINT ( 'NONE',  ( 194.9646308670422172, 268.7998031773939260, -10.80984512674310416 ) ) ;
#98585=CARTESIAN_POINT ( 'NONE',  ( 171.5476497511431830, 279.6901843683210132, -14.62984903706609963 ) ) ;
#98586=CARTESIAN_POINT ( 'NONE',  ( 203.5086680611402983, 278.1596424678725157, -14.69722159556002872 ) ) ;
#98587=CARTESIAN_POINT ( 'NONE',  ( 167.2900023830132170, 283.1360949131732809, -11.47530909209802275 ) ) ;
#98588=CARTESIAN_POINT ( 'NONE',  ( 162.8049643890749962, 273.4538889149586680, 14.88131869267027874 ) ) ;
#98589=CARTESIAN_POINT ( 'NONE',  ( 1.204062292545672097, 165.3768266524159856, 9.188101187500098632 ) ) ;
#98591=CARTESIAN_POINT ( 'NONE',  ( 185.0690397135245746, 295.5174023956343490, 8.503999811686171029 ) ) ;
#98592=EDGE_LOOP ( 'NONE', ( #56119, #6371, #60996, #9316 ) ) ;
#98593=B_SPLINE_SURFACE_WITH_KNOTS ( 'NONE', 3, 1, ( 
 ( #34633, #96481 ),
 ( #59403, #4748 ),
 ( #3754, #97947 ),
 ( #35631, #82285 ),
 ( #58421, #12858 ),
 ( #49345, #89397 ),
 ( #19948, #81281 ),
 ( #88405, #41728 ),
 ( #88913, #27049 ),
 ( #80285, #10853 ),
 ( #72673, #50824 ),
 ( #57426, #74156 ),
 ( #66533, #97459 ),
 ( #34150, #11855 ),
 ( #51317, #18961 ),
 ( #49839, #11373 ),
 ( #42224, #65042 ),
 ( #95991, #26552 ),
 ( #35127, #89872 ),
 ( #28027, #73162 ),
 ( #19473, #73647 ),
 ( #42712, #4227 ),
 ( #66037, #81774 ),
 ( #12348, #43213 ),
 ( #46196, #99439 ),
 ( #36613, #38609 ),
 ( #60901, #53312 ),
 ( #61901, #60400 ),
 ( #29528, #20957 ),
 ( #91864, #91356 ),
 ( #92361, #6221 ),
 ( #84267, #31011 ),
 ( #75635, #37117 ),
 ( #14814, #7211 ) ),
 .UNSPECIFIED., .T., .F., .F.,
 ( 4, 2, 2, 2, 2, 2, 2, 2, 2, 2, 2, 2, 2, 2, 2, 2, 4 ),
 ( 2, 2 ),
 ( 0.000000000000000000, 0.06250000000000000000, 0.1250000000000000000, 0.1875000000000000000, 0.2500000000000000000, 0.3125000000000000000, 0.3750000000000000000, 0.4375000000000000000, 0.5000000000000000000, 0.5625000000000000000, 0.6250000000000000000, 0.6875000000000000000, 0.7500000000000000000, 0.8125000000000000000, 0.8750000000000000000, 0.9375000000000000000, 1.000000000000000000 ),
 ( 0.000000000000000000, 1.000000000000000000 ),
 .UNSPECIFIED. ) ;
#98598=CARTESIAN_POINT ( 'NONE',  ( 171.6388997907716316, 289.6077812978417683, 2.686983444171377577 ) ) ;
#98600=DIRECTION ( 'NONE',  ( -0.8660254037844387076, -0.4999999999999998890, -0.000000000000000000 ) ) ;
#98601=CARTESIAN_POINT ( 'NONE',  ( 152.1649379268514792, 277.7140263207647308, 3.704665498480741004 ) ) ;
#98602=B_SPLINE_CURVE_WITH_KNOTS ( 'NONE', 3,
 ( #94744, #11135, #87691, #11627, #4009, #88671, #72440, #12115, #3046, #34893, #10117, #79560, #81064, #33933, #56708, #25832, #40982, #73917, #96250, #2531, #80557, #33413, #18223, #49117, #80054, #50595, #26813, #42487, #58202, #73422, #57695, #89180, #64819, #42978, #95766, #81545, #10621, #32902, #63811, #59690, #20218, #67296, #75417, #35898, #51088, #90659, #6510, #44487 ),
 .UNSPECIFIED., .F., .F.,
 ( 4, 2, 2, 2, 2, 2, 2, 2, 2, 2, 2, 2, 2, 2, 2, 2, 2, 2, 2, 2, 2, 2, 2, 4 ),
 ( 0.0003268706731840239797, 0.001346441947956916827, 0.001856227585343372954, 0.002111120404036600801, 0.002238566813383220146, 0.002366013222729838623, 0.002620906041422961519, 0.002875798860116085282, 0.003385584497502390922, 0.004405155772275003503, 0.005424727047047616518, 0.005934512684433878790, 0.006189405503127002987, 0.006444298321820127184, 0.006508021526493336026, 0.006571744731166544000, 0.006635467935839751974, 0.006699191140512959948, 0.006954083959205918479, 0.007463869596591793040, 0.007718762415284729887, 0.007973655233977666734, 0.008228548052670604449, 0.008483440871363540428 ),
 .UNSPECIFIED. ) ;
#98603=CARTESIAN_POINT ( 'NONE',  ( 26.45420224557697608, 176.8923013555409796, 4.594050593750050204 ) ) ;
#98604=CARTESIAN_POINT ( 'NONE',  ( 117.8466853168797428, 238.8458772461660544, 9.188101187500095079 ) ) ;
#98606=LINE ( 'NONE', #61556, #60862 ) ;
#98608=CARTESIAN_POINT ( 'NONE',  ( 206.2998527406910512, 271.9071720711702369, -8.006848967205936418 ) ) ;
#98609=EDGE_CURVE ( 'NONE', #84087, #11048, #82897, .T. ) ;
#98610=CARTESIAN_POINT ( 'NONE',  ( 175.3896052792100306, 281.5987068202503565, -14.18719490586176235 ) ) ;
#98613=CARTESIAN_POINT ( 'NONE',  ( -17.42236680055705023, 149.2012482093457777, 0.000000000000000000 ) ) ;
#98617=CARTESIAN_POINT ( 'NONE',  ( 187.4789422952534892, 298.9514069382850039, -0.5906970195174623406 ) ) ;
#98619=CARTESIAN_POINT ( 'NONE',  ( 164.7195526368693947, 253.2027545570438178, -12.99489340351435551 ) ) ;
#98620=B_SPLINE_CURVE_WITH_KNOTS ( 'NONE', 3,
 ( #1619, #93331, #32504, #24889 ),
 .UNSPECIFIED., .F., .F.,
 ( 4, 4 ),
 ( 0.02660023401806649312, 0.03583121442840941917 ),
 .UNSPECIFIED. ) ;
#98623=CARTESIAN_POINT ( 'NONE',  ( 101.1217432541752856, 223.0643266524159571, -9.188101187500093303 ) ) ;
#98627=DIRECTION ( 'NONE',  ( -0.8660254037844387076, -0.4999999999999998890, -0.000000000000000000 ) ) ;
#98628=CARTESIAN_POINT ( 'NONE',  ( 157.7529601300917363, 257.4108533407307959, 16.91445305439664892 ) ) ;
#98629=CARTESIAN_POINT ( 'NONE',  ( 200.4404104491965768, 283.4740205424688497, 17.49842356273781263 ) ) ;
#98630=CARTESIAN_POINT ( 'NONE',  ( 203.7909709648339458, 272.4802963485253713, -9.740038563755955892 ) ) ;
#98632=CARTESIAN_POINT ( 'NONE',  ( 173.5499876061905979, 267.4222840943004940, -16.96674921312246198 ) ) ;
#98634=CARTESIAN_POINT ( 'NONE',  ( 147.3715240516018810, 275.3920280842035595, -3.728968767617475866 ) ) ;
#98639=CARTESIAN_POINT ( 'NONE',  ( 192.4867975473904949, 297.2500821921321972, -13.04960750009181325 ) ) ;
#98643=CARTESIAN_POINT ( 'NONE',  ( 157.5879965179223916, 268.7330653384368588, 15.67728094257759786 ) ) ;
#98646=CARTESIAN_POINT ( 'NONE',  ( 142.0502911348375221, 259.4865022471902876, -10.00000000000009415 ) ) ;
#98650=CARTESIAN_POINT ( 'NONE',  ( 163.1008115941903895, 248.1481028935802442, 11.25332017433677834 ) ) ;
#98652=ORIENTED_EDGE ( 'NONE', *, *, #80993, .T. ) ;
#98654=ORIENTED_EDGE ( 'NONE', *, *, #61510, .F. ) ;
#98655=FACE_OUTER_BOUND ( 'NONE', #34420, .T. ) ;
#98656=CARTESIAN_POINT ( 'NONE',  ( 158.4451082418582359, 256.2120176447879203, 16.27803009664086176 ) ) ;
#98657=CARTESIAN_POINT ( 'NONE',  ( 190.5362692644993672, 278.6201753252890967, -16.51120110810393982 ) ) ;
#98659=CARTESIAN_POINT ( 'NONE',  ( 200.7484899876179441, 282.9404111291507888, -16.88964748465601673 ) ) ;
#98662=EDGE_CURVE ( 'NONE', #40485, #52219, #56692, .T. ) ;
#98666=CARTESIAN_POINT ( 'NONE',  ( 165.3709094149136263, 274.8634007614296593, 14.74939627246788554 ) ) ;
#98669=ORIENTED_EDGE ( 'NONE', *, *, #69275, .T. ) ;
#98672=CARTESIAN_POINT ( 'NONE',  ( 174.2444115436975665, 257.3183303361469143, -11.90217922001411743 ) ) ;
#98673=CARTESIAN_POINT ( 'NONE',  ( 165.9041802389429563, 274.0587237628353137, -15.17960966916681365 ) ) ;
#98674=CARTESIAN_POINT ( 'NONE',  ( 206.4738852556816369, 273.0237356314501085, -9.746110091792012042 ) ) ;
#98675=CARTESIAN_POINT ( 'NONE',  ( 197.4417221320944122, 273.1026795264489238, -13.30033383848224204 ) ) ;
#98682=CARTESIAN_POINT ( 'NONE',  ( 118.6048046409561465, 227.0327760586659451, 1.948934522072303157E-15 ) ) ;
#98686=CARTESIAN_POINT ( 'NONE',  ( 191.9871034619986574, 275.2958097524751224, 16.51095949440587418 ) ) ;
#98688=CARTESIAN_POINT ( 'NONE',  ( 164.0123586716512705, 248.3359725020313533, -9.617851509444742319 ) ) ;
#98691=CARTESIAN_POINT ( 'NONE',  ( 157.7861133721078772, 257.3534302411229646, 18.03837896619386783 ) ) ;
#98692=CARTESIAN_POINT ( 'NONE',  ( 206.5237403681858552, 272.9373840435757188, -10.81420335655575116 ) ) ;
#98694=ADVANCED_FACE ( 'NONE', ( #99126 ), #73448, .F. ) ;
#98695=ORIENTED_EDGE ( 'NONE', *, *, #78407, .T. ) ;
#98696=CARTESIAN_POINT ( 'NONE',  ( 195.2812657889309662, 292.4099212176463425, 15.19213940613456337 ) ) ;
#98699=EDGE_LOOP ( 'NONE', ( #76459, #79250, #17438, #62726, #64903, #66232, #12919, #49913, #84639, #93940, #20683, #52270, #20925, #27688, #54295, #11733, #51350, #94461, #48004, #21514 ) ) ;
#98702=CARTESIAN_POINT ( 'NONE',  ( 186.1263547150109900, 286.8862237501084564, -16.18252752151998308 ) ) ;
#98705=CARTESIAN_POINT ( 'NONE',  ( -22.42236680055709641, 157.8615022471902591, 0.000000000000000000 ) ) ;
#98706=CARTESIAN_POINT ( 'NONE',  ( 201.1679199471075492, 282.2139371290980989, -16.62385308864941535 ) ) ;
#98708=CARTESIAN_POINT ( 'NONE',  ( 157.4243923570103050, 257.9799494174374104, 18.06359219958597606 ) ) ;
#98711=CARTESIAN_POINT ( 'NONE',  ( 189.5599828453989346, 263.0657735508838186, -9.804501003715218488 ) ) ;
#98712=CARTESIAN_POINT ( 'NONE',  ( 173.5113001039477751, 251.2546712883042517, -0.9897563821454024025 ) ) ;
#98713=CARTESIAN_POINT ( 'NONE',  ( 189.0912321849916111, 270.0745130361697193, -14.07025751438627381 ) ) ;
#98716=CARTESIAN_POINT ( 'NONE',  ( 147.6095992045671323, 244.4824982072973967, 3.021315404115420679E-15 ) ) ;
#98718=CARTESIAN_POINT ( 'NONE',  ( 194.3252252352508265, 294.0658320307167628, 14.07225870721148731 ) ) ;
#98719=CARTESIAN_POINT ( 'NONE',  ( 191.4382082719228322, 282.7680930013282250, -17.46921905594915003 ) ) ;
#98721=CARTESIAN_POINT ( 'NONE',  ( 83.28711936893076029, 209.7048013555409796, 4.594050593750051981 ) ) ;
#98722=CARTESIAN_POINT ( 'NONE',  ( 159.8597520197352537, 253.7617827468940277, -16.74905990210778839 ) ) ;
#98725=EDGE_CURVE ( 'NONE', #82418, #91683, #1681, .T. ) ;
#98728=EDGE_CURVE ( 'NONE', #94724, #81988, #11636, .T. ) ;
#98729=CARTESIAN_POINT ( 'NONE',  ( 161.1747502674735415, 251.4841389699472529, -13.25152330924089839 ) ) ;
#98735=CARTESIAN_POINT ( 'NONE',  ( 149.7247407264208618, 272.0633196944937140, -11.44969454563192279 ) ) ;
#98737=CARTESIAN_POINT ( 'NONE',  ( 157.2464636617698375, 258.2881309577184652, 18.14284729738657731 ) ) ;
#98739=CARTESIAN_POINT ( 'NONE',  ( 168.0185004389765595, 274.8492260674121326, -16.75068961788599609 ) ) ;
#98740=CARTESIAN_POINT ( 'NONE',  ( 199.2580273620699813, 277.9411595627967699, 16.03392482410259845 ) ) ;
#98741=CARTESIAN_POINT ( 'NONE',  ( 147.8163551302855296, 274.6215580551378821, -9.286329195885331345 ) ) ;
#98743=CARTESIAN_POINT ( 'NONE',  ( 49.53858449761714411, 211.6589784336661637, -6.496448406907676862E-16 ) ) ;
#98745=CARTESIAN_POINT ( 'NONE',  ( 171.3554945684980453, 286.6428740666748354, 7.414102809553750006 ) ) ;
#98748=CARTESIAN_POINT ( 'NONE',  ( 157.6921299354026189, 257.5162143285667753, -18.18720974599499840 ) ) ;
#98749=CARTESIAN_POINT ( 'NONE',  ( 180.9962514683335257, 255.6518059654043782, 5.281628127585873855 ) ) ;
#98751=CARTESIAN_POINT ( 'NONE',  ( 176.1626442602351403, 274.9078016565098892, 17.19964070129887546 ) ) ;
#98754=CARTESIAN_POINT ( 'NONE',  ( 163.5147782259477083, 255.5762155980353896, -14.85420212278641117 ) ) ;
#98756=CARTESIAN_POINT ( 'NONE',  ( 88.35671610020233402, 228.4865022471903160, 10.00000000000009237 ) ) ;
#98757=CARTESIAN_POINT ( 'NONE',  ( 161.1089126327036354, 251.5981730984191529, 13.95161017039218976 ) ) ;
#98758=CARTESIAN_POINT ( 'NONE',  ( 165.2395056520857111, 269.6740676042253995, -16.28644685873352671 ) ) ;
#98760=CARTESIAN_POINT ( 'NONE',  ( 55.84441874286383722, 212.2369531367911293, -4.594050593750048428 ) ) ;
#98762=CARTESIAN_POINT ( 'NONE',  ( 163.2151044353641680, 263.6560547264549541, 16.97092589136012108 ) ) ;
#98763=CARTESIAN_POINT ( 'NONE',  ( 182.5291792280718823, 296.7636338796572204, 0.3805386115670883473 ) ) ;
#98765=CARTESIAN_POINT ( 'NONE',  ( 204.9574235042572923, 272.8759434632493708, -10.91876598039351265 ) ) ;
#98768=FACE_OUTER_BOUND ( 'NONE', #57552, .T. ) ;
#98773=CARTESIAN_POINT ( 'NONE',  ( 116.5487100721118026, 226.5494855054051584, -2.679491924311248496 ) ) ;
#98778=DIRECTION ( 'NONE',  ( -0.8660254037844387076, -0.4999999999999998890, -0.000000000000000000 ) ) ;
#98780=CARTESIAN_POINT ( 'NONE',  ( 182.2841300395537871, 284.0799011696702223, 14.96127849592191161 ) ) ;
#98781=CARTESIAN_POINT ( 'NONE',  ( 159.9788992190088948, 253.5554137441726255, -15.81862932303382330 ) ) ;
#98787=CARTESIAN_POINT ( 'NONE',  ( 207.7625791259561652, 270.7916523727319031, -1.015623356719550063 ) ) ;
#98788=CARTESIAN_POINT ( 'NONE',  ( 204.3276935076901850, 276.7410487817560920, 13.46217427333259309 ) ) ;
#98791=CARTESIAN_POINT ( 'NONE',  ( 161.1500805419174469, 263.0475797279946164, -17.31870440403353228 ) ) ;
#98792=CARTESIAN_POINT ( 'NONE',  ( 122.6094779419291712, 253.8464784336661353, 1.353441290958777525E-15 ) ) ;
#98793=EDGE_CURVE ( 'NONE', #32891, #89364, #78015, .T. ) ;
#98794=CARTESIAN_POINT ( 'NONE',  ( 76.27746593522670082, 214.8458772461660544, 9.188101187500095079 ) ) ;
#98796=CARTESIAN_POINT ( 'NONE',  ( 170.3407533412963915, 263.8712159389925205, 15.90218549753505428 ) ) ;
#98797=CARTESIAN_POINT ( 'NONE',  ( 128.2864073861747727, 233.3262482093457493, 3.021315404115420679E-15 ) ) ;
#98799=B_SPLINE_CURVE_WITH_KNOTS ( 'NONE', 3,
 ( #75535, #6120, #37506, #37016, #98847, #52705, #60298, #67924, #29424, #21820, #74558, #83665, #14228, #36016, #66917, #76049 ),
 .UNSPECIFIED., .F., .F.,
 ( 4, 2, 2, 2, 2, 2, 2, 4 ),
 ( 0.001006769657979127586, 0.001259641240578331274, 0.001512512823177534962, 0.001765384405776738433, 0.002018255988375941903, 0.002271127570975146025, 0.002523999153574349279, 0.003029742318772843390 ),
 .UNSPECIFIED. ) ;
#98800=CARTESIAN_POINT ( 'NONE',  ( 169.3971321688942169, 259.0209908423287288, 15.77637843574870224 ) ) ;
#98801=VERTEX_POINT ( 'NONE', #21855 ) ;
#98803=CARTESIAN_POINT ( 'NONE',  ( 89.56554322277027325, 212.5177522451417929, 5.000000000000051514 ) ) ;
#98805=CARTESIAN_POINT ( 'NONE',  ( 72.93609909127609114, 224.4637435831424739, 2.679491924311251605 ) ) ;
#98806=ADVANCED_FACE ( 'NONE', ( #43141 ), #83699, .T. ) ;
#98808=CARTESIAN_POINT ( 'NONE',  ( 109.3091660502225011, 245.4637435831425023, 2.679491924311251605 ) ) ;
#98809=CARTESIAN_POINT ( 'NONE',  ( 194.1493756275458793, 294.3704124857528655, 13.94613522129020744 ) ) ;
#98812=CARTESIAN_POINT ( 'NONE',  ( 182.9932251654942945, 257.3252772383810338, -6.270752636691518056 ) ) ;
#98813=ORIENTED_EDGE ( 'NONE', *, *, #8161, .F. ) ;
#98814=B_SPLINE_CURVE_WITH_KNOTS ( 'NONE', 3,
 ( #18686, #19696, #95733, #3974, #28263, #57159, #57659, #73880, #88639, #11097, #42941, #89626, #88140, #90108, #49569, #50073 ),
 .UNSPECIFIED., .F., .F.,
 ( 4, 2, 2, 2, 2, 2, 2, 4 ),
 ( 1.156196775494863067E-16, 0.0003787177898467221381, 0.0007574355796933285919, 0.001136153369539935317, 0.001514871159386541608, 0.001893588949233148116, 0.002272306739079755274, 0.003029742318773115308 ),
 .UNSPECIFIED. ) ;
#98815=CARTESIAN_POINT ( 'NONE',  ( 161.8900357011995652, 250.2452282568197859, -12.82231662042267217 ) ) ;
#98818=CARTESIAN_POINT ( 'NONE',  ( 163.7258651212256382, 261.0251292819381774, -16.78914756408816089 ) ) ;
#98820=CARTESIAN_POINT ( 'NONE',  ( 206.4943150373521803, 272.9883502116088039, 11.34100825923693101 ) ) ;
#98821=CARTESIAN_POINT ( 'NONE',  ( 157.6304115535352537, 270.8650229002738001, -16.00510772102553858 ) ) ;
#98822=CARTESIAN_POINT ( 'NONE',  ( 142.6909626358283560, 247.0643266524159856, -9.188101187500093303 ) ) ;
#98823=ORIENTED_EDGE ( 'NONE', *, *, #78443, .F. ) ;
#98827=CARTESIAN_POINT ( 'NONE',  ( 148.9701624811553984, 277.3468434241520981, -1.218048504557616152 ) ) ;
#98829=ORIENTED_EDGE ( 'NONE', *, *, #67909, .F. ) ;
#98830=CARTESIAN_POINT ( 'NONE',  ( 206.7325995683429767, 270.5756292972641859, -5.459556455514786855 ) ) ;
#98831=CARTESIAN_POINT ( 'NONE',  ( 185.4538201292061785, 277.6915352341014227, -16.99660624438589451 ) ) ;
#98836=CARTESIAN_POINT ( 'NONE',  ( 202.6452040468594475, 267.4133178899479049, 0.8753174002111273611 ) ) ;
#98838=CARTESIAN_POINT ( 'NONE',  ( 190.9559560067148425, 299.9015775189195665, -4.895152914295826108 ) ) ;
#98839=EDGE_CURVE ( 'NONE', #31470, #82130, #83953, .T. ) ;
#98841=CARTESIAN_POINT ( 'NONE',  ( 205.1793861064249711, 275.2658739283173759, -14.08953480709093675 ) ) ;
#98842=CARTESIAN_POINT ( 'NONE',  ( 196.3021051436114135, 270.7336484030830093, 11.92689920574754581 ) ) ;
#98843=EDGE_CURVE ( 'NONE', #30467, #60494, #57549, .T. ) ;
#98844=EDGE_CURVE ( 'NONE', #1717, #23755, #33329, .T. ) ;
#98847=CARTESIAN_POINT ( 'NONE',  ( 205.4355683657304326, 274.4353959702803536, 11.00905889885928879 ) ) ;
#98849=CARTESIAN_POINT ( 'NONE',  ( 159.9671766634011192, 253.5757178060795809, 16.49140845334465411 ) ) ;
#98852=CARTESIAN_POINT ( 'NONE',  ( 148.4552706801120507, 256.5177522451418213, -10.00000000000009592 ) ) ;
#98853=CARTESIAN_POINT ( 'NONE',  ( 174.7421405500457752, 284.6308697351560681, -12.06511137246073417 ) ) ;
#98857=CARTESIAN_POINT ( 'NONE',  ( 202.5051313019488646, 273.9765361377286581, -13.12135839583134000 ) ) ;
#98858=CARTESIAN_POINT ( 'NONE',  ( 151.3681950933278983, 268.4695907787949523, -15.50699599486383917 ) ) ;
#98859=CARTESIAN_POINT ( 'NONE',  ( 9.864316330390064280, 170.3768266524159856, -9.188101187500093303 ) ) ;
#98862=CARTESIAN_POINT ( 'NONE',  ( 204.8878784573704195, 275.7707799872745795, -14.13380496213581594 ) ) ;
#98865=DIRECTION ( 'NONE',  ( -0.8660254037844359321, -0.5000000000000051070, -0.000000000000000000 ) ) ;
#98866=CARTESIAN_POINT ( 'NONE',  ( 150.7576929667484080, 269.5270114801595582, 13.75028158740543205 ) ) ;
#98867=CARTESIAN_POINT ( 'NONE',  ( 57.68498304950349365, 204.1115022471902591, 10.00000000000009592 ) ) ;
#98869=CARTESIAN_POINT ( 'NONE',  ( 190.1063449786324213, 301.3731469862293011, 0.2163967485516588019 ) ) ;
#98870=CARTESIAN_POINT ( 'NONE',  ( 7.969365115964081703, 187.6589784336661637, -6.496448406907675876E-16 ) ) ;
#98871=CARTESIAN_POINT ( 'NONE',  ( 164.5437530064905332, 284.7883962438557433, 4.221428904827313033 ) ) ;
#98873=CARTESIAN_POINT ( 'NONE',  ( 152.9489295551198893, 265.7316783776963121, 17.71675637597311237 ) ) ;
#98878=CARTESIAN_POINT ( 'NONE',  ( 173.2106840999569215, 256.4575935151219710, 12.77520126633179487 ) ) ;
#98879=CARTESIAN_POINT ( 'NONE',  ( 163.5517623707881398, 281.2794412073851049, 8.859983951043487238 ) ) ;
#98881=CARTESIAN_POINT ( 'NONE',  ( 189.8480911035503880, 301.8204558191226283, -0.8992086515915015399 ) ) ;
#98883=CARTESIAN_POINT ( 'NONE',  ( 155.3017250444513024, 261.6565170503553190, 18.58368563027307374 ) ) ;
#98884=VERTEX_POINT ( 'NONE', #52251 ) ;
#98885=CARTESIAN_POINT ( 'NONE',  ( 185.4369573720926496, 290.9562819449305380, 12.20735569394162923 ) ) ;
#98886=CARTESIAN_POINT ( 'NONE',  ( 179.0484917649878298, 259.9789987921100192, 12.89662402083353854 ) ) ;
#98887=B_SPLINE_CURVE_WITH_KNOTS ( 'NONE', 3,
 ( #50184, #11704, #90734, #58277, #83115, #75493, #8571, #22770, #93193, #85619, #14670, #85099, #15141, #84119, #6576, #61249, #31844, #46543, #38447, #53164 ),
 .UNSPECIFIED., .F., .F.,
 ( 4, 2, 2, 2, 2, 2, 2, 2, 2, 4 ),
 ( 1.040834085586084257E-17, 0.0003687798516324237216, 0.0007375597032648370348, 0.001106339554897250348, 0.001475119406529663661, 0.001659509332345890376, 0.001843899258162117307, 0.002212679109794577891, 0.002581458961427039126, 0.002950238813059499494 ),
 .UNSPECIFIED. ) ;
#98888=B_SPLINE_CURVE_WITH_KNOTS ( 'NONE', 3,
 ( #60848, #90833, #46147, #83212, #6175, #13777, #37073, #67977, #98897, #29479, #60352, #21871, #99393, #29971, #2084, #40556, #69958, #93303, #87251, #78083, #87746, #24375, #63869, #2591, #18287, #94806, #573, #55739, #8672, #77590, #17267, #32962, #63372, #17785, #86730, #62859, #41049, #71491, #56259, #1593, #79619, #8177, #16266, #10183, #93816, #48170, #39046, #62349 ),
 .UNSPECIFIED., .F., .F.,
 ( 4, 2, 2, 2, 2, 2, 2, 2, 2, 2, 2, 2, 2, 2, 2, 2, 2, 2, 2, 2, 2, 2, 2, 4 ),
 ( 0.001274896852544186261, 0.001747937982023140945, 0.002220979111502095846, 0.002457499676241543807, 0.002575759958611299229, 0.002694020240981054651, 0.002812280523350810073, 0.002930540805720565495, 0.003167061370460208612, 0.003640102499939553392, 0.004113143629418897738, 0.005059225888377677505, 0.006005308147336457271, 0.006478349276815923916, 0.006714869841555615171, 0.006951390406295307293, 0.007010520547480196714, 0.007069650688665086134, 0.007128780829849976422, 0.007187910971034865842, 0.007424431535774564037, 0.007897472665253960425, 0.008370513794733356813, 0.008843554924212754936 ),
 .UNSPECIFIED. ) ;
#98890=VERTEX_POINT ( 'NONE', #13282 ) ;
#98891=CARTESIAN_POINT ( 'NONE',  ( 196.4843898260797914, 289.9262166352153258, -16.29546860276009212 ) ) ;
#98894=CARTESIAN_POINT ( 'NONE',  ( 155.3250150347760723, 261.6161776038049425, -18.57420904020362684 ) ) ;
#98897=CARTESIAN_POINT ( 'NONE',  ( 186.3734546673078682, 271.9784816327500607, -16.50000383220312372 ) ) ;
#98898=CARTESIAN_POINT ( 'NONE',  ( 163.8670932201372352, 246.8208641845333773, 5.912697114930636211 ) ) ;
#98899=ORIENTED_EDGE ( 'NONE', *, *, #43309, .F. ) ;
#98900=CARTESIAN_POINT ( 'NONE',  ( 151.0715479399129606, 268.9833987204304435, 14.24612252017116987 ) ) ;
#98904=ORIENTED_EDGE ( 'NONE', *, *, #37707, .F. ) ;
#98908=CARTESIAN_POINT ( 'NONE',  ( 164.5813345449211624, 245.5837619211427523, 1.447064457712487373 ) ) ;
#98911=CARTESIAN_POINT ( 'NONE',  ( 190.8072577185990610, 300.1591305089344814, 3.698484652594827171 ) ) ;
#98916=CARTESIAN_POINT ( 'NONE',  ( 184.7894305693181138, 292.1317680087225881, 12.52679022050396895 ) ) ;
#98917=CARTESIAN_POINT ( 'NONE',  ( 186.1370921618058674, 283.3846817430978149, 17.26256540491417368 ) ) ;
#98919=ORIENTED_EDGE ( 'NONE', *, *, #28439, .T. ) ;
#98920=EDGE_CURVE ( 'NONE', #76357, #81989, #99720, .T. ) ;
#98922=ORIENTED_EDGE ( 'NONE', *, *, #96231, .F. ) ;
#98924=CARTESIAN_POINT ( 'NONE',  ( 156.6880320546838448, 266.5988282340034061, -16.21688391091432280 ) ) ;
#98926=CARTESIAN_POINT ( 'NONE',  ( 147.4963928429778264, 275.1757489932608109, 4.929816573182678852 ) ) ;
#98927=CARTESIAN_POINT ( 'NONE',  ( 190.4744901378711290, 300.7355008658671522, 0.04566709859947504224 ) ) ;
#98928=CARTESIAN_POINT ( 'NONE',  ( 174.7951948700959406, 260.5428239264330728, -14.87950749134391515 ) ) ;
#98929=CARTESIAN_POINT ( 'NONE',  ( 192.2431834237441706, 297.6720342317289578, 11.07782187406058938 ) ) ;
#98930=CARTESIAN_POINT ( 'NONE',  ( 191.0825225312146927, 299.6823578679484967, 9.402918570603322479 ) ) ;
#98931=CARTESIAN_POINT ( 'NONE',  ( 146.5046981847821428, 276.8934145268504494, 0.02269072295920678689 ) ) ;
#98932=B_SPLINE_CURVE_WITH_KNOTS ( 'NONE', 3,
 ( #12770, #73561, #43635, #65945, #81690, #4653, #74574, #36033, #66933, #97863, #91273, #21348, #38010, #37035, #91772, #21838, #68428, #7127, #75554, #52723, #76070, #90795, #29934, #20865 ),
 .UNSPECIFIED., .F., .F.,
 ( 4, 2, 2, 2, 2, 2, 2, 2, 2, 2, 2, 4 ),
 ( 0.0003514956339727903431, 0.002330141894556584173, 0.002824803459702569276, 0.002886636155345798874, 0.002948468850989028906, 0.002979385198810643055, 0.003010301546632258071, 0.003072134242275503715, 0.003319465024848496700, 0.003814126589994490477, 0.004061457372567502111, 0.004308788155140514178 ),
 .UNSPECIFIED. ) ;
#98937=CARTESIAN_POINT ( 'NONE',  ( 190.1365087082723448, 300.4060458655738444, 1.955324997898008732 ) ) ;
#98938=CARTESIAN_POINT ( 'NONE',  ( 176.6582871775508465, 289.9246802630469233, -9.262345648488825134 ) ) ;
#98940=CYLINDRICAL_SURFACE ( 'NONE', #41617, 17.82106496071139645 ) ;
#98945=CARTESIAN_POINT ( 'NONE',  ( 185.0684497205900527, 286.3477220876792444, 16.15350733335134237 ) ) ;
#98949=EDGE_CURVE ( 'NONE', #17524, #32720, #81632, .T. ) ;
#98951=CARTESIAN_POINT ( 'NONE',  ( 45.83126033165601854, 207.2677522451419350, -5.000000000000047962 ) ) ;
#98952=CARTESIAN_POINT ( 'NONE',  ( 116.5476472112030990, 238.0958772461660544, -9.188101187500095079 ) ) ;
#98956=CARTESIAN_POINT ( 'NONE',  ( 175.9814757996596200, 252.6576015325999833, -4.798176622748077769 ) ) ;
#98957=CARTESIAN_POINT ( 'NONE',  ( 26.64321143294855077, 192.3149278399161233, 9.188101187500093303 ) ) ;
#98959=ORIENTED_EDGE ( 'NONE', *, *, #77280, .T. ) ;
#98960=CARTESIAN_POINT ( 'NONE',  ( 191.3524005040257236, 298.6585226206977950, 8.123788837531561668 ) ) ;
#98962=B_SPLINE_SURFACE_WITH_KNOTS ( 'NONE', 3, 1, ( 
 ( #29508, #111 ),
 ( #59384, #13330 ),
 ( #36598, #22405 ),
 ( #38593, #21902 ),
 ( #14310, #76136 ),
 ( #76608, #5708 ),
 ( #6206, #82764 ),
 ( #52301, #53299 ),
 ( #45196, #7700 ),
 ( #61392, #15283 ),
 ( #69498, #14800 ),
 ( #6710, #37588 ),
 ( #99422, #67502 ),
 ( #20941, #60386 ),
 ( #84252, #68498 ),
 ( #59897, #91341 ),
 ( #90360, #77098 ),
 ( #90864, #51822 ),
 ( #44194, #45682 ),
 ( #7194, #92345 ),
 ( #75132, #98434 ),
 ( #38079, #29999 ),
 ( #83240, #60882 ),
 ( #29025, #21416 ),
 ( #91844, #68992 ),
 ( #13807, #44687 ),
 ( #75618, #37101 ),
 ( #68006, #99918 ),
 ( #98930, #30503 ),
 ( #22894, #61881 ),
 ( #41081, #93850 ),
 ( #39573, #9731 ),
 ( #31488, #1625 ),
 ( #604, #23387 ) ),
 .UNSPECIFIED., .T., .F., .F.,
 ( 4, 2, 2, 2, 2, 2, 2, 2, 2, 2, 2, 2, 2, 2, 2, 2, 4 ),
 ( 2, 2 ),
 ( 0.000000000000000000, 0.06250000000000000000, 0.1250000000000000000, 0.1875000000000000000, 0.2500000000000000000, 0.3125000000000000000, 0.3750000000000000000, 0.4375000000000000000, 0.5000000000000000000, 0.5625000000000000000, 0.6250000000000000000, 0.6875000000000000000, 0.7500000000000000000, 0.8125000000000000000, 0.8750000000000000000, 0.9375000000000000000, 1.000000000000000000 ),
 ( 0.000000000000000000, 1.000000000000000000 ),
 .UNSPECIFIED. ) ;
#98964=CARTESIAN_POINT ( 'NONE',  ( 146.8881680668833951, 276.2292252078784145, 4.973452195244782104 ) ) ;
#98967=CARTESIAN_POINT ( 'NONE',  ( 178.8036298231600654, 287.2060828167640238, -12.28353354550265841 ) ) ;
#98969=CARTESIAN_POINT ( 'NONE',  ( 110.7831656154889970, 234.7677522451418497, 10.00000000000009592 ) ) ;
#98971=CARTESIAN_POINT ( 'NONE',  ( 194.7982713327389774, 266.3824398888097562, -7.721487577295030214 ) ) ;
#98972=CARTESIAN_POINT ( 'NONE',  ( 156.1210910306064932, 280.0783503266571302, -1.584537544745406201 ) ) ;
#98973=CARTESIAN_POINT ( 'NONE',  ( 163.0056347026689707, 248.3129541054019569, -11.27842346302751508 ) ) ;
#98975=CARTESIAN_POINT ( 'NONE',  ( 15.00651571324267763, 167.2202760586659736, -5.415160957724236172E-17 ) ) ;
#98977=CARTESIAN_POINT ( 'NONE',  ( 192.6343007834967693, 272.1501977007545179, 14.19046712901153739 ) ) ;
#98980=CARTESIAN_POINT ( 'NONE',  ( 174.8448227160035913, 286.3557171739080900, 10.48088963969321519 ) ) ;
#98981=CARTESIAN_POINT ( 'NONE',  ( 59.71473008784930414, 205.2833772461660828, -9.188101187500095079 ) ) ;
#98988=CARTESIAN_POINT ( 'NONE',  ( 13.51768745649706993, 188.6115022471903160, -5.000000000000047962 ) ) ;
#98989=CARTESIAN_POINT ( 'NONE',  ( 207.5230514910949182, 271.2065264061283756, 2.678931747975364708 ) ) ;
#98990=CARTESIAN_POINT ( 'NONE',  ( 131.1618259000655371, 246.5333772461660544, 9.188101187500095079 ) ) ;
#98992=CARTESIAN_POINT ( 'NONE',  ( 186.6441056357332116, 263.8218773865065714, 12.43495875309242571 ) ) ;
#99000=CARTESIAN_POINT ( 'NONE',  ( 181.8774662184618194, 285.1120569720015965, 15.89814067624403116 ) ) ;
#99005=CARTESIAN_POINT ( 'NONE',  ( 182.7190055043868142, 259.1992038300794547, 9.912833159430794794 ) ) ;
#99006=CARTESIAN_POINT ( 'NONE',  ( 171.2938040444012131, 284.3570267106589426, -11.29644022524450619 ) ) ;
#99011=CARTESIAN_POINT ( 'NONE',  ( 35.43895548624280423, 191.2677522451418781, 10.00000000000009592 ) ) ;
#99012=CARTESIAN_POINT ( 'NONE',  ( 163.3473224498206093, 247.7211335670114352, -10.00320358166632850 ) ) ;
#99013=CARTESIAN_POINT ( 'NONE',  ( 200.6680263064462792, 283.0797783131037022, -17.21821073473145347 ) ) ;
#99014=( BOUNDED_CURVE ( )  B_SPLINE_CURVE ( 2, ( #55467, #99614, #30191, #92049, #22595, #53483, #84435, #14980, #80336 ),
 .UNSPECIFIED., .F., .T. ) 
 B_SPLINE_CURVE_WITH_KNOTS ( ( 3, 2, 2, 2, 3 ),
 ( 0.7459677419354838745, 0.7473118279569892497, 0.7500000000000000000, 0.7526881720430107503, 0.7540322580645161255 ),
 .UNSPECIFIED. ) 
 CURVE ( )  GEOMETRIC_REPRESENTATION_ITEM ( )  RATIONAL_B_SPLINE_CURVE ( ( 0.9330127018922194093, 0.9330127018922194093, 1.000000000000000000, 0.8660254037844387076, 1.000000000000000000, 0.8660254037844387076, 1.000000000000000000, 0.9330127018922194093, 0.9330127018922194093 ) ) 
 REPRESENTATION_ITEM ( '' )  );
#99015=DIRECTION ( 'NONE',  ( 0.4999999999999997780, -0.8660254037844388186, 0.000000000000000000 ) ) ;
#99017=CARTESIAN_POINT ( 'NONE',  ( 191.8988907218820827, 287.7686841597946454, -15.96143006346140858 ) ) ;
#99019=CARTESIAN_POINT ( 'NONE',  ( 190.2935937139882299, 301.0488226629397559, 4.649863831023156813 ) ) ;
#99020=CYLINDRICAL_SURFACE ( 'NONE', #87186, 17.82106496071139645 ) ;
#99023=CARTESIAN_POINT ( 'NONE',  ( 159.5606259118165724, 264.0648208006689401, -17.79391822139266566 ) ) ;
#99025=CARTESIAN_POINT ( 'NONE',  ( 204.9768178125733016, 275.6167325052707611, 13.98665089523138505 ) ) ;
#99027=CIRCLE ( 'NONE', #73150, 17.82106496071138935 ) ;
#99029=CARTESIAN_POINT ( 'NONE',  ( 94.03063961704269502, 237.3464784336661637, 1.353441290958777525E-15 ) ) ;
#99030=CARTESIAN_POINT ( 'NONE',  ( 202.8929259191885990, 279.2261391420940413, 15.95194794840659824 ) ) ;
#99031=B_SPLINE_CURVE_WITH_KNOTS ( 'NONE', 3,
 ( #1551, #84672, #77023, #18246, #87210, #56213, #24825, #41006, #18741, #95291, #34914, #17745, #71449, #72960, #71948, #10141, #48645, #79580, #32924, #65330, #49625, #96269, #2550, #63828, #33435, #26341, #42026, #79071, #17220, #19263, #3552, #4028, #64332, #73444, #94270, #9656, #80579, #55700, #33953, #34430, #88693, #86688, #11159, #41518, #26835, #64840, #3067, #40514 ),
 .UNSPECIFIED., .F., .F.,
 ( 4, 2, 2, 2, 2, 2, 2, 2, 2, 2, 2, 2, 2, 2, 2, 2, 2, 2, 2, 2, 2, 2, 2, 4 ),
 ( 0.0004917448815929795127, 0.0009375404226552196867, 0.001160438193186298953, 0.001271887078451796899, 0.001383335963717294628, 0.001494784848982792357, 0.001606233734248289869, 0.001829131504779285327, 0.002274927045841276460, 0.003166518127965259159, 0.004058109210089241858, 0.004949700292213225425, 0.005395495833275181646, 0.005618393603806124195, 0.005729842489071552969, 0.005785566931704267356, 0.005841291374336981743, 0.005897015816969696130, 0.005952740259602410516, 0.006064189144867911281, 0.006287086915398848626, 0.006732882456460760612, 0.007178677997522671730, 0.007624473538584582849 ),
 .UNSPECIFIED. ) ;
#99033=CARTESIAN_POINT ( 'NONE',  ( 178.1909066280907155, 269.2453967466507265, -16.39845926520222719 ) ) ;
#99044=CARTESIAN_POINT ( 'NONE',  ( 164.4414259850711915, 245.8260906552167171, -6.983224448873608381 ) ) ;
#99047=CARTESIAN_POINT ( 'NONE',  ( 153.2283961777204695, 265.2476279883323400, -17.66880461074566000 ) ) ;
#99048=EDGE_CURVE ( 'NONE', #4844, #83200, #64861, .T. ) ;
#99051=CARTESIAN_POINT ( 'NONE',  ( 165.0375907685516665, 264.5099736516525581, -16.99518358851781485 ) ) ;
#99055=ORIENTED_EDGE ( 'NONE', *, *, #32161, .T. ) ;
#99058=CARTESIAN_POINT ( 'NONE',  ( 124.2269133023873025, 230.9824982072973683, 3.021315404115420679E-15 ) ) ;
#99060=CARTESIAN_POINT ( 'NONE',  ( 162.6626107288841467, 248.9070890562113902, 10.12509462564867313 ) ) ;
#99061=CARTESIAN_POINT ( 'NONE',  ( 188.5695376368248617, 260.2104469467469698, 2.212583216593476898 ) ) ;
#99062=CARTESIAN_POINT ( 'NONE',  ( 161.2972242823068711, 281.6108077277488633, -6.333146725496678897 ) ) ;
#99064=CARTESIAN_POINT ( 'NONE',  ( 158.2221939799978543, 257.7339154173171778, 16.96189593371927984 ) ) ;
#99065=CARTESIAN_POINT ( 'NONE',  ( 171.9391425390357142, 254.6921945179661009, 11.15667454778956369 ) ) ;
#99066=CARTESIAN_POINT ( 'NONE',  ( 194.8270828572394180, 263.2003066260025435, -0.7951096159142986286 ) ) ;
#99067=ORIENTED_EDGE ( 'NONE', *, *, #96726, .T. ) ;
#99068=CARTESIAN_POINT ( 'NONE',  ( 181.8960946995764232, 270.3917867799183341, -16.61744280869827861 ) ) ;
#99070=CARTESIAN_POINT ( 'NONE',  ( 193.5443425788056402, 294.1820684295764750, -14.23539291189358558 ) ) ;
#99071=CARTESIAN_POINT ( 'NONE',  ( -7.357133217438262207, 179.8927522451419350, 2.944929066748280225E-16 ) ) ;
#99073=CARTESIAN_POINT ( 'NONE',  ( 204.1031112175353996, 277.1300367187844813, -15.72043984417398299 ) ) ;
#99075=CARTESIAN_POINT ( 'NONE',  ( 161.7796304268777305, 250.9944936524672414, -12.70549294170103849 ) ) ;
#99076=CARTESIAN_POINT ( 'NONE',  ( -5.021015940802497468, 180.1589784336661637, -6.496448406907675876E-16 ) ) ;
#99077=CARTESIAN_POINT ( 'NONE',  ( 181.2440676231241241, 294.5520841294345473, -6.623935519155441654 ) ) ;
#99078=CARTESIAN_POINT ( 'NONE',  ( 162.8185578269781502, 249.0392105293238956, 10.15993992013319236 ) ) ;
#99080=B_SPLINE_CURVE_WITH_KNOTS ( 'NONE', 3,
 ( #61639, #98688, #14063, #68747, #99671, #6467, #37346, #68248, #92113, #84495, #15039, #45930 ),
 .UNSPECIFIED., .F., .F.,
 ( 4, 2, 2, 2, 2, 4 ),
 ( 0.000000000000000000, 0.0004890028609250972628, 0.0009780057218501945256, 0.001467008582775291680, 0.001711510013237798949, 0.001956011443700306218 ),
 .UNSPECIFIED. ) ;
#99083=CARTESIAN_POINT ( 'NONE',  ( 195.4436462626574667, 265.1414692012189676, -7.795071168451356058 ) ) ;
#99084=CARTESIAN_POINT ( 'NONE',  ( 175.5914919541931738, 291.0691946881663625, 3.106523132310328617 ) ) ;
#99086=CARTESIAN_POINT ( 'NONE',  ( 202.6926917162147674, 279.5729549550576962, -16.99192271786972697 ) ) ;
#99088=CARTESIAN_POINT ( 'NONE',  ( 149.8701220700901331, 277.0052374769863377, 3.110135497610186039 ) ) ;
#99089=CARTESIAN_POINT ( 'NONE',  ( 23.17945691357580529, 178.0643266524160140, -9.188101187500093303 ) ) ;
#99090=CARTESIAN_POINT ( 'NONE',  ( 115.5194155920915620, 231.3768266524159856, 9.188101187500098632 ) ) ;
#99091=CARTESIAN_POINT ( 'NONE',  ( 181.7851089240506042, 293.9661549358203843, -6.312394866988652709 ) ) ;
#99092=CARTESIAN_POINT ( 'NONE',  ( 167.0546803224166297, 282.1702852132879684, 12.27869116404093752 ) ) ;
#99093=CARTESIAN_POINT ( 'NONE',  ( 206.6389649419900536, 271.5030152196637800, -6.665702415263554670 ) ) ;
#99094=CARTESIAN_POINT ( 'NONE',  ( 175.2840916747148583, 281.5314111190519952, -14.18821149970558793 ) ) ;
#99095=EDGE_CURVE ( 'NONE', #93932, #87229, #72979, .T. ) ;
#99098=CARTESIAN_POINT ( 'NONE',  ( 155.2098048002210930, 261.8157275836062468, 16.98811268941991059 ) ) ;
#99099=CARTESIAN_POINT ( 'NONE',  ( 161.6127771116929921, 250.7254542206800352, -12.96229604595372464 ) ) ;
#99100=CARTESIAN_POINT ( 'NONE',  ( 190.0718788718888561, 284.8848510743849829, 17.19586970428585460 ) ) ;
#99102=CARTESIAN_POINT ( 'NONE',  ( 169.9825419676943454, 279.0846337363201997, 13.95515977481708880 ) ) ;
#99103=CARTESIAN_POINT ( 'NONE',  ( 194.7543982349976943, 266.2713905260540059, 7.866109266362086849 ) ) ;
#99106=DIRECTION ( 'NONE',  ( 0.5000000000000001110, -0.8660254037844387076, 0.000000000000000000 ) ) ;
#99107=CARTESIAN_POINT ( 'NONE',  ( 189.2799346409867098, 299.6783261569402157, -5.455465579895408368 ) ) ;
#99108=ADVANCED_FACE ( 'NONE', ( #79600 ), #81102, .T. ) ;
#99109=CARTESIAN_POINT ( 'NONE',  ( 89.32180003184730310, 228.5024278399160949, 9.188101187500095079 ) ) ;
#99111=CARTESIAN_POINT ( 'NONE',  ( 191.0816511748900268, 299.6838671013740623, 7.311127128005925790 ) ) ;
#99112=CARTESIAN_POINT ( 'NONE',  ( 159.1262782119615622, 259.2998576110095996, -17.50214152247988864 ) ) ;
#99115=CARTESIAN_POINT ( 'NONE',  ( 200.0556816868432009, 284.1403903059980394, 18.52209780479840973 ) ) ;
#99116=CARTESIAN_POINT ( 'NONE',  ( 193.8212943487757514, 292.9386659295947197, 15.46346239154970625 ) ) ;
#99118=CARTESIAN_POINT ( 'NONE',  ( 173.4448748457378144, 267.6069952321146275, -16.52737671724458224 ) ) ;
#99120=CARTESIAN_POINT ( 'NONE',  ( 193.2053309019613891, 296.0055459150826778, -12.79465285318189061 ) ) ;
#99121=CARTESIAN_POINT ( 'NONE',  ( 74.86346528667428402, 202.4824982072973967, 3.021315404115420679E-15 ) ) ;
#99125=CARTESIAN_POINT ( 'NONE',  ( 147.4323331177958494, 275.2867036919951147, -5.064030047414062707 ) ) ;
#99126=FACE_OUTER_BOUND ( 'NONE', #35072, .T. ) ;
#99130=CARTESIAN_POINT ( 'NONE',  ( 181.4567237428606745, 263.7202305692823074, -12.89642589240160930 ) ) ;
#99131=CARTESIAN_POINT ( 'NONE',  ( 169.3297900994355416, 252.0805612567175729, -8.701650770669226986 ) ) ;
#99132=CARTESIAN_POINT ( 'NONE',  ( 139.4522149234843198, 237.9865022471901455, 1.119607411625061291E-15 ) ) ;
#99134=CARTESIAN_POINT ( 'NONE',  ( 187.8790403671745821, 279.1610126101560923, 17.78295330846802358 ) ) ;
#99135=VERTEX_POINT ( 'NONE', #18765 ) ;
#99137=CARTESIAN_POINT ( 'NONE',  ( 185.2989352822014553, 292.6601518327293547, -10.61375395971920987 ) ) ;
#99141=CARTESIAN_POINT ( 'NONE',  ( 193.0800879007482251, 280.2392748681166381, -16.82455177969006854 ) ) ;
#99142=CARTESIAN_POINT ( 'NONE',  ( 153.3865286338695739, 264.9737345399563537, -17.77729132017696756 ) ) ;
#99143=CARTESIAN_POINT ( 'NONE',  ( 153.0308080659177392, 265.5898606369461277, -17.74682723936668438 ) ) ;
#99152=CARTESIAN_POINT ( 'NONE',  ( 159.0487832953843679, 273.6111705420391900, 15.08300900083998464 ) ) ;
#99154=CARTESIAN_POINT ( 'NONE',  ( 204.9608076533459950, 275.6444629144898499, 14.31488288944633069 ) ) ;
#99156=CARTESIAN_POINT ( 'NONE',  ( 201.1403430031335517, 280.2617017971787732, 16.85780947333721613 ) ) ;
#99157=B_SPLINE_CURVE_WITH_KNOTS ( 'NONE', 3,
 ( #55606, #1448, #41416, #32328, #32825, #86100, #47029, #70322, #17125, #77946, #79973, #93162, #86590, #936, #8535, #39407, #31812, #62713, #10542, #95179, #25225, #63229, #93671, #23712, #24235, #47522, #55113, #16626, #33332, #24723, #10042, #63733, #78450, #9032, #39904, #94171, #94668, #78965, #25749, #9552, #72360, #2966, #40414, #56112, #87103, #40905, #71853, #20144, #51015, #73835 ),
 .UNSPECIFIED., .F., .F.,
 ( 4, 2, 2, 2, 2, 2, 2, 2, 2, 2, 2, 2, 2, 2, 2, 2, 2, 2, 2, 2, 2, 2, 2, 2, 4 ),
 ( 0.001009582141182736046, 0.001495460752160263432, 0.001981339363137791035, 0.002224278668626549632, 0.002467217974115308663, 0.002588687626859688395, 0.002710157279604067694, 0.002831626932348446993, 0.002953096585092826291, 0.003196035890581580552, 0.003438975196070333945, 0.003924853807047937009, 0.004896611029003164819, 0.005868368250958392630, 0.006354246861935971408, 0.006597186167424759495, 0.006840125472913548450, 0.006900860299285765422, 0.006961595125657983260, 0.007022329952030199364, 0.007083064778402416335, 0.007326004083891550500, 0.007811882694869918577, 0.008297761305848286653, 0.008783639916826653862 ),
 .UNSPECIFIED. ) ;
#99158=CARTESIAN_POINT ( 'NONE',  ( 200.6588745812038610, 274.7719103742660991, -13.77739516878223291 ) ) ;
#99160=CARTESIAN_POINT ( 'NONE',  ( 189.9925954911225290, 301.5701668779311717, 0.1154287172046158938 ) ) ;
#99161=CARTESIAN_POINT ( 'NONE',  ( 167.2553560077112422, 286.2123104937505786, -4.790173979167302143 ) ) ;
#99163=CARTESIAN_POINT ( 'NONE',  ( 165.8632497677002675, 265.9352524487321148, 17.74980745403146187 ) ) ;
#99164=CARTESIAN_POINT ( 'NONE',  ( 183.8772343404243088, 284.9676589712560713, -15.02407609951014145 ) ) ;
#99165=CARTESIAN_POINT ( 'NONE',  ( 108.9156247924702114, 239.8149278399160949, -9.188101187500095079 ) ) ;
#99169=CARTESIAN_POINT ( 'NONE',  ( 188.5580838624726709, 273.6491553406668800, 15.66046095124196214 ) ) ;
#99170=ORIENTED_EDGE ( 'NONE', *, *, #15196, .T. ) ;
#99174=CARTESIAN_POINT ( 'NONE',  ( 180.7379841144351076, 294.0691683996430470, -2.595035569306750389 ) ) ;
#99175=B_SPLINE_SURFACE_WITH_KNOTS ( 'NONE', 3, 1, ( 
 ( #55320, #63444 ),
 ( #40624, #48756 ),
 ( #55808, #71560 ),
 ( #93378, #86801 ),
 ( #39612, #17335 ),
 ( #39115, #86300 ),
 ( #94874, #2157 ),
 ( #41120, #33036 ),
 ( #47723, #78658 ),
 ( #9245, #48240 ),
 ( #79186, #79688 ),
 ( #63936, #25436 ),
 ( #10249, #72053 ),
 ( #2656, #18353 ),
 ( #54828, #33547 ),
 ( #25957, #64443 ),
 ( #95402, #56829 ),
 ( #87815, #77662 ),
 ( #8250, #643 ),
 ( #31525, #62417 ),
 ( #23930, #85811 ),
 ( #70533, #16340 ),
 ( #47236, #8742 ),
 ( #88300, #88803 ),
 ( #89771, #3653 ),
 ( #34056, #80689 ),
 ( #72567, #4636 ),
 ( #35022, #27925 ),
 ( #18855, #64946 ),
 ( #58808, #50719 ),
 ( #3171, #65925 ),
 ( #20343, #49736 ),
 ( #80184, #81672 ),
 ( #96375, #51215 ) ),
 .UNSPECIFIED., .T., .F., .F.,
 ( 4, 2, 2, 2, 2, 2, 2, 2, 2, 2, 2, 2, 2, 2, 2, 2, 4 ),
 ( 2, 2 ),
 ( 0.000000000000000000, 0.06250000000000000000, 0.1250000000000000000, 0.1875000000000000000, 0.2500000000000000000, 0.3125000000000000000, 0.3750000000000000000, 0.4375000000000000000, 0.5000000000000000000, 0.5625000000000000000, 0.6250000000000000000, 0.6875000000000000000, 0.7500000000000000000, 0.8125000000000000000, 0.8750000000000000000, 0.9375000000000000000, 1.000000000000000000 ),
 ( 0.000000000000000000, 1.000000000000000000 ),
 .UNSPECIFIED. ) ;
#99176=CARTESIAN_POINT ( 'NONE',  ( 192.2058537381976464, 297.7366911437259773, 11.16662451037985981 ) ) ;
#99178=DIRECTION ( 'NONE',  ( 0.4999999999999998890, -0.8660254037844385966, 0.000000000000000000 ) ) ;
#99182=CARTESIAN_POINT ( 'NONE',  ( 44.60439100962815218, 189.8927522451418213, -10.00000000000009237 ) ) ;
#99184=CARTESIAN_POINT ( 'NONE',  ( 206.5280879940269756, 272.9298537347264642, 11.21709153681466731 ) ) ;
#99188=CARTESIAN_POINT ( 'NONE',  ( 189.5477897539192611, 288.2056741401361819, -16.43566040691730024 ) ) ;
#99189=CARTESIAN_POINT ( 'NONE',  ( -22.42236680055709641, 157.8615022471902591, 0.000000000000000000 ) ) ;
#99191=CARTESIAN_POINT ( 'NONE',  ( 158.7400172634752664, 280.5852593085238027, 5.670427242979651616 ) ) ;
#99192=CARTESIAN_POINT ( 'NONE',  ( 153.4361244163197000, 264.8878321249116539, -17.23169627811277493 ) ) ;
#99195=B_SPLINE_SURFACE_WITH_KNOTS ( 'NONE', 3, 1, ( 
 ( #92593, #76852 ),
 ( #92115, #14571 ),
 ( #76380, #31244 ),
 ( #15533, #62131 ),
 ( #7448, #46954 ),
 ( #99176, #84988 ),
 ( #93588, #93077 ),
 ( #47444, #68749 ),
 ( #24156, #70245 ),
 ( #54032, #55041 ),
 ( #38342, #86022 ),
 ( #16548, #37348 ),
 ( #30763, #68251 ),
 ( #29762, #60635 ),
 ( #91590, #99673 ),
 ( #22667, #15042 ),
 ( #69249, #80404 ),
 ( #17555, #79403 ),
 ( #94590, #70753 ),
 ( #48461, #94096 ),
 ( #63652, #39822 ),
 ( #2375, #95105 ),
 ( #66523, #78879 ),
 ( #1864, #72279 ),
 ( #26163, #87536 ),
 ( #79898, #86515 ),
 ( #1366, #25145 ),
 ( #88022, #33253 ),
 ( #40335, #8954 ),
 ( #2884, #9969 ),
 ( #71274, #32748 ),
 ( #17046, #72794 ),
 ( #47937, #56029 ),
 ( #40830, #10463 ) ),
 .UNSPECIFIED., .T., .F., .F.,
 ( 4, 2, 2, 2, 2, 2, 2, 2, 2, 2, 2, 2, 2, 2, 2, 2, 4 ),
 ( 2, 2 ),
 ( 0.000000000000000000, 0.06250000000000000000, 0.1250000000000000000, 0.1875000000000000000, 0.2500000000000000000, 0.3125000000000000000, 0.3750000000000000000, 0.4375000000000000000, 0.5000000000000000000, 0.5625000000000000000, 0.6250000000000000000, 0.6875000000000000000, 0.7500000000000000000, 0.8125000000000000000, 0.8750000000000000000, 0.9375000000000000000, 1.000000000000000000 ),
 ( 0.000000000000000000, 1.000000000000000000 ),
 .UNSPECIFIED. ) ;
#99198=CARTESIAN_POINT ( 'NONE',  ( 189.0471581402334209, 270.0386385729072458, -14.06369957967176809 ) ) ;
#99201=CARTESIAN_POINT ( 'NONE',  ( 51.02741275436266477, 210.2677522451419350, -5.000000000000047962 ) ) ;
#99202=CARTESIAN_POINT ( 'NONE',  ( 155.5888570658010508, 261.1591898008976500, 17.34682632352454945 ) ) ;
#99205=CARTESIAN_POINT ( 'NONE',  ( 79.22710464504368133, 225.7369531367911293, -4.594050593750048428 ) ) ;
#99207=CARTESIAN_POINT ( 'NONE',  ( 197.1070472075671489, 287.4405515990786739, 17.55387095912554329 ) ) ;
#99208=CARTESIAN_POINT ( 'NONE',  ( 49.43738778531180600, 210.8967562850346837, -4.648177544792955347E-16 ) ) ;
#99210=ADVANCED_FACE ( 'NONE', ( #40537 ), #4716, .F. ) ;
#99211=CARTESIAN_POINT ( 'NONE',  ( 161.4143265314674522, 251.0691807084224365, -12.94469757303959234 ) ) ;
#99218=DIRECTION ( 'NONE',  ( 0.4999999999999998890, -0.8660254037844385966, 0.000000000000000000 ) ) ;
#99222=CARTESIAN_POINT ( 'NONE',  ( 57.11665387649598813, 203.7833772461660828, -9.188101187500095079 ) ) ;
#99223=CARTESIAN_POINT ( 'NONE',  ( 157.8092552871339365, 257.3133472685137235, 17.04082256169242626 ) ) ;
#99226=CARTESIAN_POINT ( 'NONE',  ( 140.0925393287100178, 257.8149278399160949, -9.188101187500095079 ) ) ;
#99227=CARTESIAN_POINT ( 'NONE',  ( 49.94514132322986910, 190.4548013555409796, -4.594050593750042211 ) ) ;
#99228=CONICAL_SURFACE ( 'NONE', #55523, 17.82106496071138935, 0.7853981633974672638 ) ;
#99230=CARTESIAN_POINT ( 'NONE',  ( 198.9369963555428740, 286.0780101374919013, -18.58432392708837710 ) ) ;
#99231=CARTESIAN_POINT ( 'NONE',  ( 196.9431415128477170, 289.5314680279574304, -16.61413060656005669 ) ) ;
#99235=CARTESIAN_POINT ( 'NONE',  ( 175.1821364343245477, 291.7930096221122085, 1.896737885627243436 ) ) ;
#99236=CARTESIAN_POINT ( 'NONE',  ( 176.2722938307433367, 274.9184840992016916, 16.82248187572799125 ) ) ;
#99237=CARTESIAN_POINT ( 'NONE',  ( 182.1765326276830592, 281.0659326347872593, -16.99519206479797973 ) ) ;
#99238=CARTESIAN_POINT ( 'NONE',  ( 153.2535461983702021, 276.7944624501984663, 7.180768696100536808 ) ) ;
#99239=AXIS2_PLACEMENT_3D ( 'NONE', #37527, #60816, #29942 ) ;
#99240=B_SPLINE_CURVE_WITH_KNOTS ( 'NONE', 3,
 ( #94899, #56350, #17880, #48778, #41143, #2682, #39635, #33572, #87837, #18376, #80208, #3198, #34082, #90302, #20872, #73085, #65458, #51763, #35048, #66455, #12777, #43131, #18882, #81698, #88830, #43643, #96906, #19875, #89321, #19395, #74581, #44134, #66940, #97870, #5160, #36039, #50744, #12271, #65954, #74072, #27477, #4662, #82705, #42150, #28442, #50254, #26475, #57351, #89793, #73569, #35554, #97380 ),
 .UNSPECIFIED., .F., .F.,
 ( 4, 2, 2, 2, 2, 2, 2, 2, 2, 2, 2, 2, 2, 2, 2, 2, 2, 2, 2, 2, 2, 2, 2, 2, 2, 4 ),
 ( 0.0006742088093967555989, 0.0008834669511509028999, 0.001092725092905050092, 0.001197354163782128351, 0.001301983234659206609, 0.001406612305536284867, 0.001511241376413363126, 0.001720499518167624593, 0.001929757659921886061, 0.002348273943430352617, 0.003185306510447285296, 0.004022339077464217975, 0.004859371644481151088, 0.005277887927989698309, 0.005487146069744016155, 0.005591775140621175512, 0.005644089676059718327, 0.005696404211498261143, 0.005748718746936803958, 0.005801033282375345906, 0.005905662353252520008, 0.006114920495006899437, 0.006324178636761279733, 0.006533436778515659162, 0.006951953062024276639, 0.007370469345532895851 ),
 .UNSPECIFIED. ) ;
#99243=CARTESIAN_POINT ( 'NONE',  ( 100.5532405368332007, 228.8615022471902591, -10.00000000000009592 ) ) ;
#99244=CARTESIAN_POINT ( 'NONE',  ( 200.1662314894802819, 283.9489124310637180, 17.19420058542677054 ) ) ;
#99245=CARTESIAN_POINT ( 'NONE',  ( 194.6164141854688694, 285.4975589841284318, -17.28892555162024181 ) ) ;
#99248=CARTESIAN_POINT ( 'NONE',  ( 58.36173894231861681, 198.3768266524159856, 9.188101187500098632 ) ) ;
#99250=CARTESIAN_POINT ( 'NONE',  ( 166.5849221621933225, 264.6761944418691996, 17.19226874345410394 ) ) ;
#99251=CARTESIAN_POINT ( 'NONE',  ( 190.7403173041394950, 300.2750747078583800, -4.254144485856557800 ) ) ;
#99254=AXIS2_PLACEMENT_3D ( 'NONE', #36531, #37523, #29441 ) ;
#99257=CARTESIAN_POINT ( 'NONE',  ( 194.4666154385731431, 293.8209370148700827, -14.56896502715340702 ) ) ;
#99260=CARTESIAN_POINT ( 'NONE',  ( 156.9781162866021589, 258.7529222455866034, 16.87007551417546480 ) ) ;
#99261=ORIENTED_EDGE ( 'NONE', *, *, #73429, .F. ) ;
#99267=EDGE_LOOP ( 'NONE', ( #85083, #20774, #83759, #82688, #60525 ) ) ;
#99269=CARTESIAN_POINT ( 'NONE',  ( 206.2041691044954348, 273.4908977089264113, -9.455375957961031474 ) ) ;
#99270=VERTEX_POINT ( 'NONE', #76132 ) ;
#99274=CARTESIAN_POINT ( 'NONE',  ( 162.9186055433422382, 283.5390355093646804, -3.110742804078471924 ) ) ;
#99275=FACE_OUTER_BOUND ( 'NONE', #67021, .T. ) ;
#99276=CARTESIAN_POINT ( 'NONE',  ( 189.7094295309238419, 300.0606247079692253, 5.078421157105148076 ) ) ;
#99277=CARTESIAN_POINT ( 'NONE',  ( 164.2712161151136172, 246.1209027979328710, 7.276091357954241445 ) ) ;
#99278=CARTESIAN_POINT ( 'NONE',  ( 198.5966822647444587, 286.6674514332866579, 17.25284514431582750 ) ) ;
#99279=CARTESIAN_POINT ( 'NONE',  ( 182.1983635332545646, 295.7656116556308916, 4.955917269626422872 ) ) ;
#99280=CARTESIAN_POINT ( 'NONE',  ( 122.2307653756559773, 247.5024278399160949, -9.188101187500093303 ) ) ;
#99282=CARTESIAN_POINT ( 'NONE',  ( 203.2651555929824383, 267.8361268713933327, 2.564698397200394719 ) ) ;
#99283=CARTESIAN_POINT ( 'NONE',  ( 182.7190055043868142, 259.1992038300794547, 9.912833159430794794 ) ) ;
#99284=CARTESIAN_POINT ( 'NONE',  ( 69.62006919151632189, 204.8768266524160140, -9.188101187500091527 ) ) ;
#99287=CARTESIAN_POINT ( 'NONE',  ( 181.3346534254663140, 271.3440730695800767, -17.45372068697093226 ) ) ;
#99288=VERTEX_POINT ( 'NONE', #66997 ) ;
#99289=CARTESIAN_POINT ( 'NONE',  ( 164.5139018292655919, 259.6662038739244736, -17.01387605652571366 ) ) ;
#99290=VERTEX_POINT ( 'NONE', #74135 ) ;
#99292=ADVANCED_FACE ( 'NONE', ( #44682 ), #50792, .F. ) ;
#99293=CARTESIAN_POINT ( 'NONE',  ( 79.26890985290187075, 228.1199935810940929, 2.679491924311251605 ) ) ;
#99296=CARTESIAN_POINT ( 'NONE',  ( 0.4370954166217684844, 164.3927522451417644, -10.00000000000009237 ) ) ;
#99298=CARTESIAN_POINT ( 'NONE',  ( 114.8426596992764388, 237.1115022471902307, 10.00000000000009592 ) ) ;
#99301=B_SPLINE_CURVE_WITH_KNOTS ( 'NONE', 3,
 ( #88237, #57262, #58262, #96313 ),
 .UNSPECIFIED., .F., .F.,
 ( 4, 4 ),
 ( 0.008596905824991037462, 0.01496866495574719277 ),
 .UNSPECIFIED. ) ;
#99309=CARTESIAN_POINT ( 'NONE',  ( 183.9632230134671715, 275.2220319246098938, 16.38282608893444703 ) ) ;
#99310=AXIS2_PLACEMENT_3D ( 'NONE', #41791, #96051, #86965 ) ;
#99311=CARTESIAN_POINT ( 'NONE',  ( 198.9782417033094930, 281.1264296331257810, 17.13350274969746323 ) ) ;
#99312=CARTESIAN_POINT ( 'NONE',  ( 147.4771086736140262, 275.6046378290653251, -0.0003692388140982706527 ) ) ;
#99313=CARTESIAN_POINT ( 'NONE',  ( 138.6044920356617922, 241.6423013555409796, -4.594050593750043987 ) ) ;
#99314=ORIENTED_EDGE ( 'NONE', *, *, #7604, .T. ) ;
#99315=CARTESIAN_POINT ( 'NONE',  ( 0.9806730298622799991, 159.8262482093458061, 3.021315404115420679E-15 ) ) ;
#99318=( BOUNDED_CURVE ( )  B_SPLINE_CURVE ( 2, ( #44919, #44429, #51541, #67233, #73854, #22135, #60115, #66735, #5940 ),
 .UNSPECIFIED., .F., .T. ) 
 B_SPLINE_CURVE_WITH_KNOTS ( ( 3, 2, 2, 2, 3 ),
 ( 0.5040322580645161255, 0.5053763440860215006, 0.5080645161290322509, 0.5107526881720430012, 0.5120967741935483764 ),
 .UNSPECIFIED. ) 
 CURVE ( )  GEOMETRIC_REPRESENTATION_ITEM ( )  RATIONAL_B_SPLINE_CURVE ( ( 0.9330127018922194093, 0.9330127018922194093, 1.000000000000000000, 0.8660254037844387076, 1.000000000000000000, 0.8660254037844387076, 1.000000000000000000, 0.9330127018922194093, 0.9330127018922194093 ) ) 
 REPRESENTATION_ITEM ( '' )  );
#99323=CARTESIAN_POINT ( 'NONE',  ( 195.7165112625155530, 265.4114503779815664, 4.502320798389543022 ) ) ;
#99326=CARTESIAN_POINT ( 'NONE',  ( 185.0302441327199290, 263.6005475928211581, -12.60236960991709232 ) ) ;
#99327=CARTESIAN_POINT ( 'NONE',  ( 184.3405100053359149, 263.3003275659135625, -13.11914462798110748 ) ) ;
#99328=CARTESIAN_POINT ( 'NONE',  ( 198.5696159774462615, 266.1063467524069779, 0.3741886566019196891 ) ) ;
#99331=CARTESIAN_POINT ( 'NONE',  ( 146.7879906441258129, 276.4027375938661635, 4.347255311287614887 ) ) ;
#99332=CARTESIAN_POINT ( 'NONE',  ( 186.8085655849630200, 282.2086298501483839, 17.42445011646567110 ) ) ;
#99334=CARTESIAN_POINT ( 'NONE',  ( 164.3274319858398087, 246.0235340536434592, -1.770631424362269168 ) ) ;
#99339=CARTESIAN_POINT ( 'NONE',  ( 148.9275518150011806, 272.6969089400084272, 12.34519124974546500 ) ) ;
#99342=CARTESIAN_POINT ( 'NONE',  ( 19.39713158799116499, 193.5530062829863311, -4.648177544792955347E-16 ) ) ;
#99343=CARTESIAN_POINT ( 'NONE',  ( 140.5888732624033821, 258.6427522451418781, -10.00000000000009415 ) ) ;
#99344=CARTESIAN_POINT ( 'NONE',  ( -22.42236680055709641, 157.8615022471902591, 0.000000000000000000 ) ) ;
#99346=EDGE_CURVE ( 'NONE', #51044, #941, #42987, .T. ) ;
#99349=CARTESIAN_POINT ( 'NONE',  ( 199.2299651681423143, 285.5705732690366858, -17.65328173313980642 ) ) ;
#99350=CARTESIAN_POINT ( 'NONE',  ( 3.260525530768699998, 178.8149278399161233, 9.188101187500093303 ) ) ;
#99351=CARTESIAN_POINT ( 'NONE',  ( 178.7807591103801315, 273.8421904428736866, -16.83327263018412978 ) ) ;
#99354=CARTESIAN_POINT ( 'NONE',  ( 205.2391015854675516, 275.1624436846170738, -14.01434138479280911 ) ) ;
#99356=CARTESIAN_POINT ( 'NONE',  ( 123.0699010352285825, 251.8615022471902876, 5.000000000000046185 ) ) ;
#99357=CARTESIAN_POINT ( 'NONE',  ( 178.3085564311570295, 254.9668335614806551, -3.913436853880700728 ) ) ;
#99358=EDGE_CURVE ( 'NONE', #98253, #86118, #63792, .T. ) ;
#99359=CARTESIAN_POINT ( 'NONE',  ( 198.1857676047573307, 287.3791765019590798, 18.47549341984830562 ) ) ;
#99361=CARTESIAN_POINT ( 'NONE',  ( 51.18979252112020362, 200.3615022471902307, -10.00000000000009592 ) ) ;
#99363=CARTESIAN_POINT ( 'NONE',  ( 147.6121581866023007, 274.9752375363476631, 8.700660424766859080 ) ) ;
#99364=CARTESIAN_POINT ( 'NONE',  ( 10.56744132731740216, 189.1589784336661637, -6.496448406907675876E-16 ) ) ;
#99366=CARTESIAN_POINT ( 'NONE',  ( 152.7153488183568300, 266.1362520814392951, 17.33540622643059237 ) ) ;
#99368=B_SPLINE_CURVE_WITH_KNOTS ( 'NONE', 3,
 ( #48811, #25495, #57888, #4185 ),
 .UNSPECIFIED., .F., .F.,
 ( 4, 4 ),
 ( 0.04775794113389541379, 0.04887120950165265570 ),
 .UNSPECIFIED. ) ;
#99370=CARTESIAN_POINT ( 'NONE',  ( 164.4858674010174298, 245.7491158648375347, -2.958464974013825355 ) ) ;
#99371=CARTESIAN_POINT ( 'NONE',  ( 188.9070770133223505, 267.7838735664225851, 14.12628498767583629 ) ) ;
#99373=CARTESIAN_POINT ( 'NONE',  ( 160.6500289177108129, 280.8499340018469752, 9.543921644910932756 ) ) ;
#99376=CARTESIAN_POINT ( 'NONE',  ( 190.1158090214649405, 301.3567547831981983, -1.340987185199551845 ) ) ;
#99378=CARTESIAN_POINT ( 'NONE',  ( 155.3738696901333469, 261.5315588585399951, 17.02116401938635804 ) ) ;
#99380=CARTESIAN_POINT ( 'NONE',  ( 185.4471464075789982, 290.9481437133458144, 12.22111610210481381 ) ) ;
#99381=CARTESIAN_POINT ( 'NONE',  ( 160.9155581428462085, 282.2930683307629920, -7.657675304491033508 ) ) ;
#99382=DIRECTION ( 'NONE',  ( -0.8660254037844387076, -0.4999999999999998890, -0.000000000000000000 ) ) ;
#99386=CARTESIAN_POINT ( 'NONE',  ( 166.8965953329662568, 259.4083194189263963, 16.50658842888446642 ) ) ;
#99387=CARTESIAN_POINT ( 'NONE',  ( 195.6914848190668863, 279.7035040353765680, -17.46620344769279853 ) ) ;
#99388=CARTESIAN_POINT ( 'NONE',  ( 155.5587153255869453, 261.2113968263770971, -18.30500480654006878 ) ) ;
#99390=VERTEX_POINT ( 'NONE', #70491 ) ;
#99393=CARTESIAN_POINT ( 'NONE',  ( 186.2308893754327244, 271.9687482497705560, -16.31403051770207213 ) ) ;
#99396=CARTESIAN_POINT ( 'NONE',  ( 150.6571681785161445, 269.7011255207979730, 15.24894850018880454 ) ) ;
#99399=CARTESIAN_POINT ( 'NONE',  ( 188.9516232634142909, 259.5449388965931234, 2.625812016075142807 ) ) ;
#99401=CARTESIAN_POINT ( 'NONE',  ( 190.5893431400089923, 300.5365696307625853, -0.3099240395267599535 ) ) ;
#99404=CARTESIAN_POINT ( 'NONE',  ( 164.4261001824251878, 245.8526357240660900, 1.583002802772015549 ) ) ;
#99405=EDGE_CURVE ( 'NONE', #6345, #17132, #93640, .T. ) ;
#99407=VERTEX_POINT ( 'NONE', #8203 ) ;
#99408=CARTESIAN_POINT ( 'NONE',  ( 148.9230895364621574, 272.7046378331555161, 12.20434325797056019 ) ) ;
#99410=ORIENTED_EDGE ( 'NONE', *, *, #61202, .F. ) ;
#99411=CARTESIAN_POINT ( 'NONE',  ( 177.2105452297388979, 293.7001946432246768, 0.5067388932645889854 ) ) ;
#99418=CARTESIAN_POINT ( 'NONE',  ( 190.3791419447713906, 300.9006487807255326, -5.688668718458480988 ) ) ;
#99419=CARTESIAN_POINT ( 'NONE',  ( 190.1063449786324213, 301.3731469862293011, 0.2163967485516588019 ) ) ;
#99420=CARTESIAN_POINT ( 'NONE',  ( 149.6877696051026305, 271.3801731027346591, 11.89134584187677390 ) ) ;
#99421=CARTESIAN_POINT ( 'NONE',  ( 153.3616370783189211, 265.0168479788495688, 17.48287904751960653 ) ) ;
#99422=CARTESIAN_POINT ( 'NONE',  ( 191.8109306323408134, 298.4207180281530896, 8.739483817295738532 ) ) ;
#99423=CARTESIAN_POINT ( 'NONE',  ( 191.7247331938518187, 298.5700163710982338, -9.650650827884682315 ) ) ;
#99424=CARTESIAN_POINT ( 'NONE',  ( 190.1751179328237242, 301.2540287353828035, 3.252640783176552475 ) ) ;
#99426=CARTESIAN_POINT ( 'NONE',  ( 196.9728329903666122, 289.4800408803428695, -17.53478045286815856 ) ) ;
#99429=CARTESIAN_POINT ( 'NONE',  ( 170.8130694511098682, 289.0930926786006125, 4.372098042472422286 ) ) ;
#99431=CARTESIAN_POINT ( 'NONE',  ( 97.73839765093606502, 236.4244531367911009, -4.594050593750046652 ) ) ;
#99435=CARTESIAN_POINT ( 'NONE',  ( 185.1491161497484370, 292.9437783688060222, -11.97406807593424993 ) ) ;
#99437=B_SPLINE_CURVE_WITH_KNOTS ( 'NONE', 3,
 ( #51902, #83833, #5792, #22974, #7789, #38675, #14399, #13414, #7281, #75710, #38161, #69081 ),
 .UNSPECIFIED., .F., .F.,
 ( 4, 2, 2, 2, 2, 4 ),
 ( 0.001256110456608531753, 0.001699454778389175797, 0.001921126939279406420, 0.002142799100169636827, 0.002586143421950230347, 0.003029487743730823867 ),
 .UNSPECIFIED. ) ;
#99438=CARTESIAN_POINT ( 'NONE',  ( 191.2247497985414668, 298.1499797848484832, -9.475781189105788371 ) ) ;
#99439=CARTESIAN_POINT ( 'NONE',  ( 148.1409269118794327, 274.0593832387140765, -8.913879232967422794 ) ) ;
#99440=CARTESIAN_POINT ( 'NONE',  ( 165.7154513341344568, 284.2511262621020478, -8.535179277079183890 ) ) ;
#99441=ORIENTED_EDGE ( 'NONE', *, *, #92503, .T. ) ;
#99442=CARTESIAN_POINT ( 'NONE',  ( 167.5494526128936741, 253.3644281013700663, -11.97820646762932384 ) ) ;
#99443=CARTESIAN_POINT ( 'NONE',  ( 160.0061168334508750, 253.5082714530983026, -16.02306982074888708 ) ) ;
#99446=CARTESIAN_POINT ( 'NONE',  ( 41.86197723097736656, 201.6427522451419350, -10.00000000000009415 ) ) ;
#99447=CARTESIAN_POINT ( 'NONE',  ( 115.2486091055264410, 237.3458772461660544, 9.188101187500095079 ) ) ;
#99448=B_SPLINE_CURVE_WITH_KNOTS ( 'NONE', 3,
 ( #57940, #35640, #57435, #65050 ),
 .UNSPECIFIED., .F., .F.,
 ( 4, 4 ),
 ( 0.009420313403532103169, 0.01473026445887711325 ),
 .UNSPECIFIED. ) ;
#99449=CARTESIAN_POINT ( 'NONE',  ( 199.1216527653377000, 285.7581758537840528, -18.37739894744384728 ) ) ;
#99452=CARTESIAN_POINT ( 'NONE',  ( 175.6350414609877362, 253.2567788339581512, -4.713150756204576908 ) ) ;
#99453=CARTESIAN_POINT ( 'NONE',  ( 27.69859311986958872, 195.9869531367911293, 4.594050593750046652 ) ) ;
#99455=VERTEX_POINT ( 'NONE', #24891 ) ;
#99456=CARTESIAN_POINT ( 'NONE',  ( 197.2717555009968464, 267.1836181950307605, -9.366199491810448308 ) ) ;
#99457=CARTESIAN_POINT ( 'NONE',  ( 177.9286246128441462, 265.4632741294796006, 15.77837218392110685 ) ) ;
#99459=CARTESIAN_POINT ( 'NONE',  ( 190.2287563641723978, 301.1611242470490311, -4.521471513871881953 ) ) ;
#99464=CARTESIAN_POINT ( 'NONE',  ( 106.0200258946745322, 242.0177522451419350, 5.000000000000046185 ) ) ;
#99465=B_SPLINE_SURFACE_WITH_KNOTS ( 'NONE', 3, 1, ( 
 ( #16961, #78789 ),
 ( #47850, #40255 ),
 ( #48885, #32670 ),
 ( #25583, #71195 ),
 ( #79819, #63569 ),
 ( #95536, #50364 ),
 ( #33690, #88437 ),
 ( #2803, #43250 ),
 ( #66567, #10888 ),
 ( #35665, #87945 ),
 ( #34179, #72196 ),
 ( #97020, #51355 ),
 ( #81318, #35163 ),
 ( #18998, #18489 ),
 ( #64584, #49873 ),
 ( #66073, #56958 ),
 ( #10386, #11402 ),
 ( #26084, #57458 ),
 ( #12384, #81809 ),
 ( #42256, #49374 ),
 ( #41255, #27590 ),
 ( #41764, #74195 ),
 ( #57967, #96514 ),
 ( #28060, #80834 ),
 ( #19507, #88952 ),
 ( #11889, #73190 ),
 ( #42747, #97493 ),
 ( #89427, #4784 ),
 ( #73681, #58933 ),
 ( #80317, #72710 ),
 ( #58454, #3784 ),
 ( #3300, #65073 ),
 ( #96022, #26585 ),
 ( #34666, #89903 ) ),
 .UNSPECIFIED., .T., .F., .F.,
 ( 4, 2, 2, 2, 2, 2, 2, 2, 2, 2, 2, 2, 2, 2, 2, 2, 4 ),
 ( 2, 2 ),
 ( 0.000000000000000000, 0.06250000000000000000, 0.1250000000000000000, 0.1875000000000000000, 0.2500000000000000000, 0.3125000000000000000, 0.3750000000000000000, 0.4375000000000000000, 0.5000000000000000000, 0.5625000000000000000, 0.6250000000000000000, 0.6875000000000000000, 0.7500000000000000000, 0.8125000000000000000, 0.8750000000000000000, 0.9375000000000000000, 1.000000000000000000 ),
 ( 0.000000000000000000, 1.000000000000000000 ),
 .UNSPECIFIED. ) ;
#99470=CARTESIAN_POINT ( 'NONE',  ( 158.8128131472595328, 282.3092851352909634, -1.638803179544075617 ) ) ;
#99471=CARTESIAN_POINT ( 'NONE',  ( 163.3020905273760093, 247.7994775548095845, -11.05431316445765155 ) ) ;
#99472=CARTESIAN_POINT ( 'NONE',  ( 6.805730253569997501, 183.9244531367911293, -4.594050593750046652 ) ) ;
#99474=CARTESIAN_POINT ( 'NONE',  ( 192.4454877273399802, 272.0519467580534752, 14.18723452604855417 ) ) ;
#99476=CARTESIAN_POINT ( 'NONE',  ( 183.8274263638271577, 281.3324037098167310, 17.41033114534894111 ) ) ;
#99477=CARTESIAN_POINT ( 'NONE',  ( 176.9957387850661519, 287.7651793544013685, 10.62179850618674770 ) ) ;
#99478=CARTESIAN_POINT ( 'NONE',  ( 72.16419236301562989, 200.2202760586659736, -5.415160957724236172E-17 ) ) ;
#99481=EDGE_CURVE ( 'NONE', #59744, #12032, #74263, .T. ) ;
#99484=VERTEX_POINT ( 'NONE', #14851 ) ;
#99485=EDGE_CURVE ( 'NONE', #86658, #4092, #39214, .T. ) ;
#99486=CARTESIAN_POINT ( 'NONE',  ( 20.87890338866488804, 172.8615022471901739, 5.000000000000051514 ) ) ;
#99487=CARTESIAN_POINT ( 'NONE',  ( 164.3545367017254364, 245.9765873086048487, -5.942639963102972267 ) ) ;
#99488=CARTESIAN_POINT ( 'NONE',  ( 137.1160976468485444, 237.7202760586660020, -5.415160957724236172E-17 ) ) ;
#99490=CARTESIAN_POINT ( 'NONE',  ( 167.7835675164443217, 262.4791022244722853, -16.86277329496921240 ) ) ;
#99494=CARTESIAN_POINT ( 'NONE',  ( 174.0063104898480901, 290.5518564105048540, -6.237772892647018175 ) ) ;
#99499=DIRECTION ( 'NONE',  ( 0.4999999999999992784, -0.8660254037844390407, 0.000000000000000000 ) ) ;
#99500=CARTESIAN_POINT ( 'NONE',  ( 172.8007671839257284, 268.7064279019212449, -17.42650422937455090 ) ) ;
#99501=CARTESIAN_POINT ( 'NONE',  ( 183.8043731368310603, 268.5938253857621589, 16.29461355553033997 ) ) ;
#99502=ORIENTED_EDGE ( 'NONE', *, *, #54181, .T. ) ;
#99503=CARTESIAN_POINT ( 'NONE',  ( 206.4772459337023349, 273.0179147663701542, 8.756720646268034258 ) ) ;
#99504=DIRECTION ( 'NONE',  ( -0.4999999999999987788, 0.8660254037844392627, 0.000000000000000000 ) ) ;
#99507=CARTESIAN_POINT ( 'NONE',  ( 196.1406707052842648, 271.0373771141688053, 12.72512690933628754 ) ) ;
#99508=CARTESIAN_POINT ( 'NONE',  ( 149.7139371938020247, 271.7509892204764128, 11.49682272138129413 ) ) ;
#99509=CARTESIAN_POINT ( 'NONE',  ( 208.3682389855799499, 269.7426187237583690, -1.431169231381201890 ) ) ;
#99510=CARTESIAN_POINT ( 'NONE',  ( 152.9607371460978129, 265.7112270302071124, -16.17698032818104537 ) ) ;
#99512=CARTESIAN_POINT ( 'NONE',  ( 191.3384774259032781, 281.1688466949726717, 16.66770346665126823 ) ) ;
#99515=ORIENTED_EDGE ( 'NONE', *, *, #52956, .T. ) ;
#99516=CARTESIAN_POINT ( 'NONE',  ( -22.42236680055709641, 157.8615022471902591, 0.000000000000000000 ) ) ;
#99520=CARTESIAN_POINT ( 'NONE',  ( 147.0660117096331874, 275.9211909828330249, -0.7354350123930680772 ) ) ;
#99522=CARTESIAN_POINT ( 'NONE',  ( 163.7239493340838123, 247.0687966679708438, 6.286946239157660266 ) ) ;
#99525=EDGE_LOOP ( 'NONE', ( #49447, #94998, #62852, #99679 ) ) ;
#99526=CARTESIAN_POINT ( 'NONE',  ( 99.20033616346982797, 218.8923013555410080, 4.594050593750050204 ) ) ;
#99527=CARTESIAN_POINT ( 'NONE',  ( 198.6773861772114458, 282.8274967129041784, 17.60335148736512068 ) ) ;
#99528=CARTESIAN_POINT ( 'NONE',  ( 180.6861897690432102, 270.7994373234269574, -15.98932744349104773 ) ) ;
#99531=EDGE_CURVE ( 'NONE', #54122, #54506, #64546, .T. ) ;
#99532=ORIENTED_EDGE ( 'NONE', *, *, #50380, .T. ) ;
#99538=VERTEX_POINT ( 'NONE', #79702 ) ;
#99539=CARTESIAN_POINT ( 'NONE',  ( 164.0854748117396582, 246.4426161724408928, -5.757837433625331514 ) ) ;
#99540=CARTESIAN_POINT ( 'NONE',  ( 170.5211436381359533, 282.8630515260593938, 11.84943660316123015 ) ) ;
#99543=CARTESIAN_POINT ( 'NONE',  ( 166.9519864817992527, 247.0838024313254664, 1.931440104004218394 ) ) ;
#99545=CARTESIAN_POINT ( 'NONE',  ( 198.8589187919461949, 276.4374630719800621, -15.82469577996627130 ) ) ;
#99546=CYLINDRICAL_SURFACE ( 'NONE', #35393, 10.00000000000010658 ) ;
#99547=CYLINDRICAL_SURFACE ( 'NONE', #13693, 10.00000000000010658 ) ;
#99549=CARTESIAN_POINT ( 'NONE',  ( 53.28814773936871774, 213.1199935810940929, 2.679491924311251605 ) ) ;
#99550=CARTESIAN_POINT ( 'NONE',  ( 188.2270213252132862, 260.7737771934913553, 2.725760956200675267 ) ) ;
#99552=CARTESIAN_POINT ( 'NONE',  ( 159.5180972751518595, 279.0588588540967976, -11.03979334413982016 ) ) ;
#99554=CARTESIAN_POINT ( 'NONE',  ( 171.5550945788819774, 255.3501946510080529, 11.01174055729725509 ) ) ;
#99555=CARTESIAN_POINT ( 'NONE',  ( 194.5772998931005588, 262.7959408956480729, -0.8050316457746058418 ) ) ;
#99556=VERTEX_POINT ( 'NONE', #55823 ) ;
#99557=CARTESIAN_POINT ( 'NONE',  ( 181.8940748684893833, 270.3951945721110519, -16.94533521498305717 ) ) ;
#99560=EDGE_CURVE ( 'NONE', #79145, #8119, #18618, .T. ) ;
#99561=CARTESIAN_POINT ( 'NONE',  ( 0.2927578493243047641, 177.6427522451419350, -10.00000000000009415 ) ) ;
#99563=CARTESIAN_POINT ( 'NONE',  ( 175.0012011881278511, 281.4042580864821161, -14.16808929002857731 ) ) ;
#99564=CARTESIAN_POINT ( 'NONE',  ( 163.6464964730003544, 247.2029489585592330, -7.382887685002309297 ) ) ;
#99567=CARTESIAN_POINT ( 'NONE',  ( -7.131779314644562717, 172.8149278399161233, 9.188101187500093303 ) ) ;
#99568=CARTESIAN_POINT ( 'NONE',  ( 107.0484310652164481, 242.6115022471903160, -5.000000000000047962 ) ) ;
#99569=AXIS2_PLACEMENT_3D ( 'NONE', #84744, #30998, #8210 ) ;
#99570=CARTESIAN_POINT ( 'NONE',  ( 163.1187975016007385, 248.7328182447493532, 9.764213595475625951 ) ) ;
#99571=VERTEX_POINT ( 'NONE', #17349 ) ;
#99574=CARTESIAN_POINT ( 'NONE',  ( 165.8206990081297931, 283.8978799598649516, 9.576760697357309837 ) ) ;
#99575=CARTESIAN_POINT ( 'NONE',  ( 149.7671394830648239, 276.5111046941532322, 6.337641867686506281 ) ) ;
#99577=CARTESIAN_POINT ( 'NONE',  ( 195.7212628913762842, 264.3281170330985219, -5.774310659065233331 ) ) ;
#99578=CARTESIAN_POINT ( 'NONE',  ( 162.8324615148077044, 248.6128988652861551, -11.81889183148518363 ) ) ;
#99580=CARTESIAN_POINT ( 'NONE',  ( 165.1399196574946018, 246.6162641258139843, 5.603258891903981187 ) ) ;
#99581=CARTESIAN_POINT ( 'NONE',  ( 20.20266813594930611, 170.2202760586659736, -5.415160957724236172E-17 ) ) ;
#99582=CARTESIAN_POINT ( 'NONE',  ( 109.2943373587434053, 246.1589784336661069, -6.496448406907675876E-16 ) ) ;
#99583=CARTESIAN_POINT ( 'NONE',  ( 179.0238627954208539, 291.8726898088843313, -6.149396189656547662 ) ) ;
#99585=CARTESIAN_POINT ( 'NONE',  ( 206.6283329956240209, 272.3565576962875525, -7.313808307417591692 ) ) ;
#99588=CARTESIAN_POINT ( 'NONE',  ( 157.1837449796689725, 258.3967629017010381, 16.97243084443542216 ) ) ;
#99589=CARTESIAN_POINT ( 'NONE',  ( 154.9683083969241011, 262.2340116239618055, 18.33261662430134109 ) ) ;
#99590=CARTESIAN_POINT ( 'NONE',  ( 207.7836085030675690, 270.7552284231231852, -5.468305433308493058 ) ) ;
#99592=CARTESIAN_POINT ( 'NONE',  ( 190.0437544431386812, 284.7811193207209612, 16.84871526811737397 ) ) ;
#99593=CARTESIAN_POINT ( 'NONE',  ( 164.4161324736616905, 249.7809132986213569, -10.44438623667713628 ) ) ;
#99594=CARTESIAN_POINT ( 'NONE',  ( 196.5611414140106774, 266.4300535012234832, 8.275873407104286983 ) ) ;
#99597=CARTESIAN_POINT ( 'NONE',  ( 207.2958410051070359, 271.0543211874339136, 2.987874948847863976 ) ) ;
#99602=CARTESIAN_POINT ( 'NONE',  ( 53.19247626382384908, 191.5177522451418213, 5.000000000000051514 ) ) ;
#99604=( BOUNDED_CURVE ( )  B_SPLINE_CURVE ( 2, ( #39369, #85551, #24688, #85028, #8012, #38379, #70283, #397, #30802 ),
 .UNSPECIFIED., .F., .T. ) 
 B_SPLINE_CURVE_WITH_KNOTS ( ( 3, 2, 2, 2, 3 ),
 ( 0.3427419354838709964, 0.3440860215053763715, 0.3467741935483871218, 0.3494623655913978721, 0.3508064516129032473 ),
 .UNSPECIFIED. ) 
 CURVE ( )  GEOMETRIC_REPRESENTATION_ITEM ( )  RATIONAL_B_SPLINE_CURVE ( ( 0.9330127018922194093, 0.9330127018922207416, 1.000000000000000000, 0.8660254037844387076, 1.000000000000000000, 0.8660254037844387076, 1.000000000000000000, 0.9330127018922194093, 0.9330127018922194093 ) ) 
 REPRESENTATION_ITEM ( '' )  );
#99605=CARTESIAN_POINT ( 'NONE',  ( 181.4357933614753051, 267.9132554559569712, 15.01118169234261224 ) ) ;
#99608=CARTESIAN_POINT ( 'NONE',  ( 96.62871582839601103, 238.8464784336661637, 1.353441290958777327E-15 ) ) ;
#99611=CARTESIAN_POINT ( 'NONE',  ( 151.3284628043366524, 268.5384091220288383, 14.49047510809488237 ) ) ;
#99614=CARTESIAN_POINT ( 'NONE',  ( 102.6515957550817291, 241.6199935810941213, 2.679491924311251605 ) ) ;
#99615=CARTESIAN_POINT ( 'NONE',  ( 201.5269734158617325, 270.9427678591820268, -9.880288512841804760 ) ) ;
#99616=CARTESIAN_POINT ( 'NONE',  ( 198.7501991201633018, 286.4015524398827779, -18.58948563601804693 ) ) ;
#99624=CARTESIAN_POINT ( 'NONE',  ( 193.0065576635309412, 296.3498312632291913, -11.90044991639595295 ) ) ;
#99626=ORIENTED_EDGE ( 'NONE', *, *, #97966, .T. ) ;
#99627=CARTESIAN_POINT ( 'NONE',  ( 152.7751718343799325, 275.0649094835816300, 10.84773788932874794 ) ) ;
#99628=CARTESIAN_POINT ( 'NONE',  ( 160.0072461633487535, 253.5063153963366744, 16.23938890643736244 ) ) ;
#99630=CARTESIAN_POINT ( 'NONE',  ( 169.3468526685033737, 252.1302625595957636, -8.748020535966752220 ) ) ;
#99632=VERTEX_POINT ( 'NONE', #95418 ) ;
#99633=CARTESIAN_POINT ( 'NONE',  ( 187.8932624934218723, 279.1755607875103351, 16.84974327597278076 ) ) ;
#99635=VERTEX_POINT ( 'NONE', #34551 ) ;
#99636=CARTESIAN_POINT ( 'NONE',  ( 167.8545683410104061, 249.5148966473869621, 6.528852040077621766 ) ) ;
#99637=CARTESIAN_POINT ( 'NONE',  ( 181.7466027418385579, 291.4440130176707839, -11.38303403918490275 ) ) ;
#99641=CARTESIAN_POINT ( 'NONE',  ( 190.8728624356520811, 278.0230195662924189, -17.10495516205424238 ) ) ;
#99642=CARTESIAN_POINT ( 'NONE',  ( 154.1115650569507807, 263.7179346178419905, -17.19893844996447996 ) ) ;
#99643=CARTESIAN_POINT ( 'NONE',  ( 152.6873874250818517, 266.1846826352417565, -16.66598363829485763 ) ) ;
#99648=CARTESIAN_POINT ( 'NONE',  ( 164.3417294400100275, 285.2078986128140627, 5.660908321736507709 ) ) ;
#99649=AXIS2_PLACEMENT_3D ( 'NONE', #95226, #2489, #31856 ) ;
#99653=CARTESIAN_POINT ( 'NONE',  ( 169.5131043871994621, 269.1741712775740325, 17.46952269320804874 ) ) ;
#99654=CARTESIAN_POINT ( 'NONE',  ( 174.4761736470610458, 257.0948179687508173, -12.20380311476513491 ) ) ;
#99655=CARTESIAN_POINT ( 'NONE',  ( 190.6804423821413934, 299.9894766172849359, -4.019216027313348150 ) ) ;
#99656=FACE_OUTER_BOUND ( 'NONE', #72361, .T. ) ;
#99657=CARTESIAN_POINT ( 'NONE',  ( 197.7762623205388195, 272.5093575422661729, -13.29982618913853365 ) ) ;
#99658=CARTESIAN_POINT ( 'NONE',  ( 200.9170142906816352, 276.9211817098563984, 15.63114281021921137 ) ) ;
#99659=CARTESIAN_POINT ( 'NONE',  ( 147.6207754342248961, 274.9603120256437592, 8.795690793376332195 ) ) ;
#99662=CARTESIAN_POINT ( 'NONE',  ( 186.7880454944370570, 286.9919446152004525, -15.66394447814424851 ) ) ;
#99663=CARTESIAN_POINT ( 'NONE',  ( 104.0981849360367875, 243.1589784336661921, -6.496448406907675876E-16 ) ) ;
#99664=ORIENTED_EDGE ( 'NONE', *, *, #5473, .T. ) ;
#99666=CARTESIAN_POINT ( 'NONE',  ( 160.6137493263213685, 283.7672525351333661, 2.212664548855189040 ) ) ;
#99667=CARTESIAN_POINT ( 'NONE',  ( 188.0359106206746276, 273.7439271439645267, 15.87289339216772355 ) ) ;
#99670=AXIS2_PLACEMENT_3D ( 'NONE', #49356, #12364, #66052 ) ;
#99671=CARTESIAN_POINT ( 'NONE',  ( 163.3967530586554062, 248.5504513908809372, -9.594069682937940158 ) ) ;
#99672=CARTESIAN_POINT ( 'NONE',  ( 173.4505375608857491, 284.9503170016366198, -13.05978560202663452 ) ) ;
#99673=CARTESIAN_POINT ( 'NONE',  ( 147.4105367463733955, 275.3244561147192826, 2.971302497651425512 ) ) ;
#99674=CARTESIAN_POINT ( 'NONE',  ( 176.1640045926653499, 252.3529155287689321, -3.563159428949892682 ) ) ;
#99678=CARTESIAN_POINT ( 'NONE',  ( 148.3703817814266017, 273.6619557466142965, 8.838269745973029501 ) ) ;
#99679=ORIENTED_EDGE ( 'NONE', *, *, #48309, .T. ) ;
#99682=CARTESIAN_POINT ( 'NONE',  ( 188.0206444253974496, 266.1040571081818484, -11.77042872245799288 ) ) ;
#99683=B_SPLINE_CURVE_WITH_KNOTS ( 'NONE', 3,
 ( #87245, #17778, #33988, #18777, #80611, #63366, #64363, #33469, #25884, #81113, #56758, #87740, #26869, #88724, #17259, #32469, #94306, #24858, #18280, #49175, #80110, #20775, #81601, #83592, #82109, #5556, #51145, #89230, #27859, #59226, #75467, #98780, #12681, #19779, #13178, #29362, #96810, #43549, #4557, #42543, #35949, #13664, #65846, #60229, #36442, #74489, #50647, #12169 ),
 .UNSPECIFIED., .F., .F.,
 ( 4, 2, 2, 2, 2, 2, 2, 2, 2, 2, 2, 2, 2, 2, 2, 2, 2, 2, 2, 2, 2, 2, 2, 4 ),
 ( 0.001060904700683941307, 0.001544591180662389235, 0.002028277660640836946, 0.002270120900630112192, 0.002511964140619387439, 0.002632885760614010317, 0.002753807380608632761, 0.002874729000603255639, 0.002995650620597878518, 0.003479337100576584269, 0.003963023580555290019, 0.004930396540512700654, 0.005897769500470112156, 0.006381455980448894234, 0.006623299220438249278, 0.006865142460427603455, 0.006925603270424942649, 0.006986064080422280977, 0.007046524890419620171, 0.007106985700416958499, 0.007348828940406565945, 0.007832515420385781704, 0.008316201900365007005, 0.008799888380344232305 ),
 .UNSPECIFIED. ) ;
#99684=CARTESIAN_POINT ( 'NONE',  ( 195.6634864761266499, 265.3502972643460680, 4.386002604212382749 ) ) ;
#99685=CARTESIAN_POINT ( 'NONE',  ( -3.532187684056895538, 158.7677522451418213, -5.000000000000041744 ) ) ;
#99686=CARTESIAN_POINT ( 'NONE',  ( 204.6620543660203282, 273.0012950431568584, -9.812076529084375665 ) ) ;
#99687=CARTESIAN_POINT ( 'NONE',  ( 187.0714549478603317, 290.7469772780716539, -13.50987823813239608 ) ) ;
#99689=CARTESIAN_POINT ( 'NONE',  ( 153.3859906278383676, 264.9746663937372091, -17.41799046551451013 ) ) ;
#99691=CARTESIAN_POINT ( 'NONE',  ( 147.5693121967435957, 275.0494489676833041, 4.210973343677100189 ) ) ;
#99693=CARTESIAN_POINT ( 'NONE',  ( 190.4592742923115622, 264.3484275416739706, -9.369623864591236639 ) ) ;
#99694=CARTESIAN_POINT ( 'NONE',  ( 170.2764733827664259, 249.3178093264847632, -0.2615362982353570676 ) ) ;
#99695=CARTESIAN_POINT ( 'NONE',  ( 191.1572877534573252, 271.1716867410561349, -14.23756759126275107 ) ) ;
#99698=CARTESIAN_POINT ( 'NONE',  ( 54.92452707139267432, 202.5177522451418497, -10.00000000000009592 ) ) ;
#99699=CARTESIAN_POINT ( 'NONE',  ( 194.4459411895494725, 293.8567458645873103, 14.31012567920753042 ) ) ;
#99702=CARTESIAN_POINT ( 'NONE',  ( 74.81622161422296813, 207.8768266524159856, -9.188101187500091527 ) ) ;
#99703=CARTESIAN_POINT ( 'NONE',  ( 159.2289198208967775, 254.8544161663325838, -15.88961297684315888 ) ) ;
#99705=CARTESIAN_POINT ( 'NONE',  ( 208.3194307158603067, 269.8271571267425770, -2.120200867047394855 ) ) ;
#99706=CARTESIAN_POINT ( 'NONE',  ( 197.1135888508448204, 287.5974573846697240, -17.44979364819638334 ) ) ;
#99708=CARTESIAN_POINT ( 'NONE',  ( 161.6923300915171922, 250.5876644177310482, -14.43081872899884566 ) ) ;
#99715=CARTESIAN_POINT ( 'NONE',  ( 161.4806224016576266, 251.9447911281216932, 13.79057941382466090 ) ) ;
#99716=CARTESIAN_POINT ( 'NONE',  ( 195.8627871995700502, 291.4026965887302936, 17.41145040657729481 ) ) ;
#99719=EDGE_CURVE ( 'NONE', #26183, #98253, #52832, .T. ) ;
#99720=B_SPLINE_CURVE_WITH_KNOTS ( 'NONE', 3,
 ( #86210, #14751, #1056, #93795, #24356, #61834, #55227, #85714, #78570, #15231, #61339, #16748, #38539, #62330, #32455, #7141 ),
 .UNSPECIFIED., .F., .F.,
 ( 4, 2, 2, 2, 2, 2, 2, 4 ),
 ( 0.0003828982427913507776, 0.0007137219304090731964, 0.001044545618026795561, 0.001375369305644518142, 0.001706192993262240507, 0.002037016680879963088, 0.002367840368497685453, 0.003029487743733128013 ),
 .UNSPECIFIED. ) ;
#99721=CARTESIAN_POINT ( 'NONE',  ( 28.70002176693659379, 193.5024278399160949, -9.188101187500093303 ) ) ;
#99722=EDGE_CURVE ( 'NONE', #82234, #45423, #77828, .T. ) ;
#99723=CARTESIAN_POINT ( 'NONE',  ( 58.68649846873780263, 198.5643266524160140, 9.188101187500095079 ) ) ;
#99727=CARTESIAN_POINT ( 'NONE',  ( -12.46307465703608841, 173.6115022471903160, -5.000000000000047962 ) ) ;
#99728=CARTESIAN_POINT ( 'NONE',  ( 40.68897417663616523, 203.4869531367911293, 4.594050593750046652 ) ) ;
#99730=CARTESIAN_POINT ( 'NONE',  ( -15.51451749852110495, 173.3967562850347406, 6.972266317189433612E-15 ) ) ;
#99731=CARTESIAN_POINT ( 'NONE',  ( 149.4171629335945681, 271.8488776066536730, -11.42564036194071520 ) ) ;
#99734=CARTESIAN_POINT ( 'NONE',  ( 159.1311797733062861, 257.0237068946943282, -17.13424826516079946 ) ) ;
#99736=VECTOR ( 'NONE', #60375, 1000.000000000000000 ) ;
#99737=CARTESIAN_POINT ( 'NONE',  ( 198.4772197948566372, 286.8743665007300478, 18.43646439804394532 ) ) ;
#99738=FACE_OUTER_BOUND ( 'NONE', #64083, .T. ) ;
#99739=CARTESIAN_POINT ( 'NONE',  ( 150.9920758754981591, 275.7439016202259836, 7.274739978851465061 ) ) ;
#99740=VECTOR ( 'NONE', #30808, 1000.000000000000000 ) ;
#99742=CARTESIAN_POINT ( 'NONE',  ( 110.0795199784619882, 244.3615022471903160, 5.000000000000046185 ) ) ;
#99743=CARTESIAN_POINT ( 'NONE',  ( 170.9951952409888918, 289.7831227640691054, 3.187764637984034088 ) ) ;
#99744=CARTESIAN_POINT ( 'NONE',  ( 193.5734017704282621, 284.8397916126203882, -16.87703258719347232 ) ) ;
#99745=ORIENTED_EDGE ( 'NONE', *, *, #74431, .T. ) ;
#99747=ORIENTED_EDGE ( 'NONE', *, *, #59772, .F. ) ;
#99749=CARTESIAN_POINT ( 'NONE',  ( 190.0204217048978137, 278.5168619470970839, -16.50316915822402208 ) ) ;
#99751=ORIENTED_EDGE ( 'NONE', *, *, #87389, .F. ) ;
#99753=CARTESIAN_POINT ( 'NONE',  ( 165.0156970625405108, 244.8314239717225007, -1.890480716182876719 ) ) ;
#99754=CARTESIAN_POINT ( 'NONE',  ( 147.6054094044680198, 274.9869267698931594, -8.596541856229405809 ) ) ;
#99755=CARTESIAN_POINT ( 'NONE',  ( 177.2889782269291743, 274.8653421391169900, -17.15541123409079205 ) ) ;
#99756=VERTEX_POINT ( 'NONE', #42143 ) ;
#99762=CARTESIAN_POINT ( 'NONE',  ( 159.9770824720811220, 253.5585604421560788, -16.42166711341322483 ) ) ;
#99767=CARTESIAN_POINT ( 'NONE',  ( 162.7070706717508699, 248.8300821762643693, -9.986337079333621247 ) ) ;
#99768=CARTESIAN_POINT ( 'NONE',  ( 164.2851776226980860, 246.0967207574460929, 5.847738044744511754 ) ) ;
#99769=CARTESIAN_POINT ( 'NONE',  ( 188.7077645169274547, 295.3037981044213893, -11.26831191883383276 ) ) ;
#99770=CARTESIAN_POINT ( 'NONE',  ( 162.8135989904577059, 264.0325098608973349, -16.79570218761738687 ) ) ;
#99771=CARTESIAN_POINT ( 'NONE',  ( 132.6230702210692698, 253.5024278399161517, -9.188101187500093303 ) ) ;
#99772=CARTESIAN_POINT ( 'NONE',  ( 177.6377870308529339, 268.6994379071560388, 17.24334423480850731 ) ) ;
#99773=CARTESIAN_POINT ( 'NONE',  ( 178.7646095310575447, 257.7369032172456969, 9.998786432605333729 ) ) ;
#99774=CARTESIAN_POINT ( 'NONE',  ( 70.29673831216418023, 202.2048013555409796, 4.594050593750051981 ) ) ;
#99780=EDGE_CURVE ( 'NONE', #61039, #20047, #53750, .T. ) ;
#99783=AXIS2_PLACEMENT_3D ( 'NONE', #99516, #81116, #18780 ) ;
#99784=ORIENTED_EDGE ( 'NONE', *, *, #88991, .T. ) ;
#99787=CARTESIAN_POINT ( 'NONE',  ( 194.8739650922309750, 285.0886630353519990, 17.09777351973150061 ) ) ;
#99788=CARTESIAN_POINT ( 'NONE',  ( 191.3610003135137276, 299.2000202002271294, -9.855749861282104618 ) ) ;
#99791=CARTESIAN_POINT ( 'NONE',  ( 155.4812142336614329, 261.3456326552338282, 18.45193178807985745 ) ) ;
#99794=CARTESIAN_POINT ( 'NONE',  ( 183.6215648671697522, 257.5753772875778509, -6.308267261209747012 ) ) ;
#99795=VERTEX_POINT ( 'NONE', #20867 ) ;
#99796=EDGE_CURVE ( 'NONE', #56872, #16138, #46926, .T. ) ;
#99798=CARTESIAN_POINT ( 'NONE',  ( 161.9737235729598979, 250.1002766109539550, -13.93568599556967236 ) ) ;
#99801=CARTESIAN_POINT ( 'NONE',  ( 163.8012378421705364, 260.8922434983789458, -16.44114888586377887 ) ) ;
#99803=CARTESIAN_POINT ( 'NONE',  ( 162.0267809142322619, 284.7786981385619356, 0.5395386606957954800 ) ) ;
#99805=CARTESIAN_POINT ( 'NONE',  ( 198.3520206420438967, 280.8587880883060279, 16.77949005266407312 ) ) ;
#99806=DIRECTION ( 'NONE',  ( -0.8660254037844359321, -0.5000000000000051070, -0.000000000000000000 ) ) ;
#99809=CARTESIAN_POINT ( 'NONE',  ( 184.5672510228033616, 259.8720230735002019, 6.331763823368266486 ) ) ;
#99811=CARTESIAN_POINT ( 'NONE',  ( 152.7375212135632125, 266.0978483664162582, -16.47968945089317572 ) ) ;
#99817=CARTESIAN_POINT ( 'NONE',  ( 195.7010779147650510, 265.4079040883964922, 4.749425292133099497 ) ) ;
#99818=CARTESIAN_POINT ( 'NONE',  ( 79.10106959370823176, 223.1427522451419065, 10.00000000000009415 ) ) ;
#99821=CARTESIAN_POINT ( 'NONE',  ( 198.5902130130228045, 266.0844563504680877, 1.367436427555045908 ) ) ;
#99822=CARTESIAN_POINT ( 'NONE',  ( 195.1469348180016254, 263.6870364683385901, 0.8484810161304255915 ) ) ;
#99823=ORIENTED_EDGE ( 'NONE', *, *, #57502, .T. ) ;
#99826=CARTESIAN_POINT ( 'NONE',  ( 186.2853797466665924, 282.4387328436498024, 16.17679748871792356 ) ) ;
#99829=CARTESIAN_POINT ( 'NONE',  ( 192.9288088394134490, 268.5874188557070852, 12.31072070184183609 ) ) ;
#99831=EDGE_CURVE ( 'NONE', #56545, #73834, #24697, .T. ) ;
#99833=CARTESIAN_POINT ( 'NONE',  ( 23.74761253515288217, 184.5177522451418497, -10.00000000000009592 ) ) ;
#99834=CARTESIAN_POINT ( 'NONE',  ( 166.2154959952744662, 286.5665612494071866, -3.304685761217393658 ) ) ;
#99836=CARTESIAN_POINT ( 'NONE',  ( 198.2819808855875863, 287.2125302111982705, 18.53535247371401695 ) ) ;
#99837=CARTESIAN_POINT ( 'NONE',  ( -13.54586673536430830, 172.1744531367911293, 4.594050593750047540 ) ) ;
#99838=CARTESIAN_POINT ( 'NONE',  ( 82.65769392073423205, 206.9824982072973683, 3.021315404115420679E-15 ) ) ;
#99839=VERTEX_POINT ( 'NONE', #17103 ) ;
#99844=CARTESIAN_POINT ( 'NONE',  ( 13.13906166239122619, 169.2048013555410080, 4.594050593750051981 ) ) ;
#99845=AXIS2_PLACEMENT_3D ( 'NONE', #7728, #37616, #31019 ) ;
#99848=CARTESIAN_POINT ( 'NONE',  ( 172.8784199730727948, 272.2467176060330871, -16.38460412274964639 ) ) ;
#99849=CARTESIAN_POINT ( 'NONE',  ( 180.6988097879044517, 288.8653027392896320, 13.27852155705168435 ) ) ;
#99850=CARTESIAN_POINT ( 'NONE',  ( 175.6666422034487596, 253.2183536273479660, -3.362340235260868226 ) ) ;
#99851=CARTESIAN_POINT ( 'NONE',  ( 191.3785584962284361, 260.9239486072202681, -1.442731442779735751 ) ) ;
#99853=CARTESIAN_POINT ( 'NONE',  ( 46.78749671854927783, 204.4865022471903444, 10.00000000000009237 ) ) ;
#99854=CARTESIAN_POINT ( 'NONE',  ( 72.82007368749162879, 224.3967562850346837, -4.648177544792955347E-16 ) ) ;
#99855=CARTESIAN_POINT ( 'NONE',  ( 189.9462859318020946, 301.6503773875500087, -1.164147598593831656 ) ) ;
#99856=CARTESIAN_POINT ( 'NONE',  ( 27.26558041797736465, 195.7369531367911293, -4.594050593750048428 ) ) ;
#99862=CARTESIAN_POINT ( 'NONE',  ( 165.0532575723395041, 244.7663672603923715, -2.144843157699870773 ) ) ;
#99864=B_SPLINE_CURVE_WITH_KNOTS ( 'NONE', 3,
 ( #2768, #2259, #33141, #26055 ),
 .UNSPECIFIED., .F., .F.,
 ( 4, 4 ),
 ( 0.001589885323195327788, 0.003217162196932791228 ),
 .UNSPECIFIED. ) ;
#99865=CARTESIAN_POINT ( 'NONE',  ( 163.0755220416274085, 280.7677949813287341, -10.02769325734202788 ) ) ;
#99866=CARTESIAN_POINT ( 'NONE',  ( 160.1410856478538562, 280.1664495048587469, 9.328772672254729059 ) ) ;
#99870=CARTESIAN_POINT ( 'NONE',  ( 194.2764122224708103, 294.1503786489221284, 15.46903869661980835 ) ) ;
#99873=CARTESIAN_POINT ( 'NONE',  ( 182.0038524954867114, 289.2836466150820343, 12.40290735734220462 ) ) ;
#99874=CARTESIAN_POINT ( 'NONE',  ( 170.8805640699686990, 257.7213711969266114, 14.63406020945912367 ) ) ;
#99875=CARTESIAN_POINT ( 'NONE',  ( -22.42236680055709641, 157.8615022471902591, 0.000000000000000000 ) ) ;
#99876=CARTESIAN_POINT ( 'NONE',  ( 3.035171627975086217, 165.8927522451417929, -10.00000000000009237 ) ) ;
#99883=( BOUNDED_CURVE ( )  B_SPLINE_CURVE ( 2, ( #25852, #87711, #94765, #79072, #93266, #70430, #78549, #33436, #64333 ),
 .UNSPECIFIED., .F., .T. ) 
 B_SPLINE_CURVE_WITH_KNOTS ( ( 3, 2, 2, 2, 3 ),
 ( 0.7217741935483871218, 0.7231182795698924970, 0.7258064516129032473, 0.7284946236559139976, 0.7298387096774193727 ),
 .UNSPECIFIED. ) 
 CURVE ( )  GEOMETRIC_REPRESENTATION_ITEM ( )  RATIONAL_B_SPLINE_CURVE ( ( 0.9330127018922194093, 0.9330127018922194093, 1.000000000000000000, 0.8660254037844387076, 1.000000000000000000, 0.8660254037844387076, 1.000000000000000000, 0.9330127018922194093, 0.9330127018922194093 ) ) 
 REPRESENTATION_ITEM ( '' )  );
#99884=ORIENTED_EDGE ( 'NONE', *, *, #40719, .F. ) ;
#99886=CARTESIAN_POINT ( 'NONE',  ( 202.4560076411394220, 279.0611292670678267, 15.58065739802832717 ) ) ;
#99887=ORIENTED_EDGE ( 'NONE', *, *, #80799, .T. ) ;
#99888=CARTESIAN_POINT ( 'NONE',  ( 151.0778907302193943, 268.9724126853576536, 15.84769371787143832 ) ) ;
#99892=EDGE_LOOP ( 'NONE', ( #62599, #75116, #4038, #67484 ) ) ;
#99893=CARTESIAN_POINT ( 'NONE',  ( 190.1730848958311810, 301.2575500587478814, 0.2415986433272204748 ) ) ;
#99894=CARTESIAN_POINT ( 'NONE',  ( 196.7130436017243653, 289.9300093007386749, -16.33278734947153765 ) ) ;
#99896=VERTEX_POINT ( 'NONE', #64210 ) ;
#99900=CARTESIAN_POINT ( 'NONE',  ( 149.6700657135140489, 271.4108371424580355, 12.58635654151485284 ) ) ;
#99902=EDGE_CURVE ( 'NONE', #45796, #56872, #35385, .T. ) ;
#99906=( BOUNDED_CURVE ( )  B_SPLINE_CURVE ( 2, ( #59329, #37047, #60822, #83696, #12784, #14256, #43649, #74588, #20880 ),
 .UNSPECIFIED., .F., .T. ) 
 B_SPLINE_CURVE_WITH_KNOTS ( ( 3, 2, 2, 2, 3 ),
 ( 0.9395161290322581182, 0.9408602150537634934, 0.9435483870967742437, 0.9462365591397849940, 0.9475806451612903691 ),
 .UNSPECIFIED. ) 
 CURVE ( )  GEOMETRIC_REPRESENTATION_ITEM ( )  RATIONAL_B_SPLINE_CURVE ( ( 0.9330127018922194093, 0.9330127018922194093, 1.000000000000000000, 0.8660254037844387076, 1.000000000000000000, 0.8660254037844387076, 1.000000000000000000, 0.9330127018922194093, 0.9330127018922194093 ) ) 
 REPRESENTATION_ITEM ( '' )  );
#99907=CARTESIAN_POINT ( 'NONE',  ( 182.1983635332545646, 295.7656116556308916, 4.955917269626422872 ) ) ;
#99913=CARTESIAN_POINT ( 'NONE',  ( 190.2287563641723978, 301.1611242470490311, -4.521471513871881953 ) ) ;
#99914=CARTESIAN_POINT ( 'NONE',  ( 189.8123550829396891, 301.8823524224806647, -0.5679054518196169354 ) ) ;
#99915=CARTESIAN_POINT ( 'NONE',  ( 190.8072577185990610, 300.1591305089344814, 3.698484652594827171 ) ) ;
#99916=CARTESIAN_POINT ( 'NONE',  ( 44.24123536260515976, 207.8967562850346837, -4.648177544792955347E-16 ) ) ;
#99918=CARTESIAN_POINT ( 'NONE',  ( 146.6463933050551134, 276.6479913793529590, 0.6147864833414898866 ) ) ;
#99919=CARTESIAN_POINT ( 'NONE',  ( 146.7434471017767521, 276.4798892723637209, 0.7354350123930684102 ) ) ;
#99920=CARTESIAN_POINT ( 'NONE',  ( 163.1897601067718711, 257.7021624904846249, 15.57231341026512794 ) ) ;
#99923=CARTESIAN_POINT ( 'NONE',  ( 196.4242782546697015, 290.4301655533025155, -16.42402868779123537 ) ) ;
#99925=CARTESIAN_POINT ( 'NONE',  ( 167.7815509137003289, 287.1807699922843540, 3.524367436705626577 ) ) ;
#99928=ORIENTED_EDGE ( 'NONE', *, *, #16463, .T. ) ;
#99929=CARTESIAN_POINT ( 'NONE',  ( 190.2594329105515101, 301.1079909101196108, -4.731131889240534960 ) ) ;
#99931=CARTESIAN_POINT ( 'NONE',  ( 186.0400780920065529, 271.7087950812899066, 16.90619359840448510 ) ) ;
#99932=EDGE_CURVE ( 'NONE', #24384, #13304, #83960, .T. ) ;
#99935=CARTESIAN_POINT ( 'NONE',  ( 191.9609695629217185, 297.7799465995823880, -9.691856174275585545 ) ) ;
#99937=CARTESIAN_POINT ( 'NONE',  ( 168.6718440011762823, 286.3164514504627505, -7.916576175921965941 ) ) ;
#99939=CARTESIAN_POINT ( 'NONE',  ( 207.8446715390582540, 270.6494641423232679, -2.429516028743652800 ) ) ;
#99940=CARTESIAN_POINT ( 'NONE',  ( 159.9770824720811220, 253.5585604421560788, -16.42166711341322483 ) ) ;
#99941=B_SPLINE_CURVE_WITH_KNOTS ( 'NONE', 3,
 ( #12001, #28674, #19619, #65677, #3894, #89543, #4900, #73303, #58087, #51478, #11012, #34776, #81926, #12502, #96631, #59051, #28180, #3416, #34290, #89067, #90023, #42859, #82445, #90534, #43868, #74810, #41885, #26689, #57577, #88550, #29189, #92991, #75300, #46343, #15444, #29676, #30676, #77266, #69657, #60551, #266, #5881, #7877, #60057, #13983, #61052, #31147, #91508, #91020, #67677 ),
 .UNSPECIFIED., .F., .F.,
 ( 4, 2, 2, 2, 2, 2, 2, 2, 2, 2, 2, 2, 2, 2, 2, 2, 2, 2, 2, 2, 2, 2, 2, 2, 4 ),
 ( 0.0001506307258450928651, 0.0006494207944938545484, 0.001148210863142616178, 0.001397605897466997101, 0.001647000931791377807, 0.001771698448953568268, 0.001896395966115758730, 0.002021093483277948757, 0.002145791000440139436, 0.002395186034764520359, 0.002644581069088901282, 0.003143371137737662694, 0.004140951275035124370, 0.005138531412332585611, 0.005637321480981316232, 0.005886716515305681977, 0.006011414032467863981, 0.006136111549630046853, 0.006198460308211138289, 0.006260809066792229725, 0.006385506583954454231, 0.006634901618278900640, 0.007133691686927773508, 0.007632481755576647243, 0.008131271824225520112 ),
 .UNSPECIFIED. ) ;
#99943=CARTESIAN_POINT ( 'NONE',  ( 46.33644181719702715, 190.8927522451418213, 10.00000000000009592 ) ) ;
#99944=CARTESIAN_POINT ( 'NONE',  ( 104.0981849360367875, 243.1589784336661921, -6.496448406907676862E-16 ) ) ;
#99945=CARTESIAN_POINT ( 'NONE',  ( 50.57404612423096069, 211.5530062829863027, -4.648177544792955347E-16 ) ) ;
#99947=CARTESIAN_POINT ( 'NONE',  ( 179.4404154152157105, 291.3709498135804097, -10.08759257512885199 ) ) ;
#99948=CARTESIAN_POINT ( 'NONE',  ( 196.4994169513186364, 290.3000215130921902, 16.82935102260526961 ) ) ;
#99949=CARTESIAN_POINT ( 'NONE',  ( 172.3026122979113097, 250.6309043013457654, -4.095500398866238179 ) ) ;
#99950=CARTESIAN_POINT ( 'NONE',  ( 46.56179571999062716, 203.8149278399160949, -9.188101187500095079 ) ) ;
#99952=AXIS2_PLACEMENT_3D ( 'NONE', #78235, #47799, #19571 ) ;
#99954=EDGE_LOOP ( 'NONE', ( #4052, #82966, #5834 ) ) ;
#99956=CARTESIAN_POINT ( 'NONE',  ( 178.5191218520901941, 266.0570017862503391, 15.28294881942528605 ) ) ;
#99961=DIRECTION ( 'NONE',  ( -0.8660254037844387076, -0.4999999999999998890, -0.000000000000000000 ) ) ;
#99962=CARTESIAN_POINT ( 'NONE',  ( 182.1820416944426029, 262.5410710835092800, 12.93635752035984687 ) ) ;
#99963=EDGE_CURVE ( 'NONE', #74797, #37080, #98476, .T. ) ;
#99965=CARTESIAN_POINT ( 'NONE',  ( 112.0822037211656266, 235.5177522451418781, -10.00000000000009592 ) ) ;
#99968=EDGE_CURVE ( 'NONE', #2866, #53306, #79112, .T. ) ;
#99969=CARTESIAN_POINT ( 'NONE',  ( 163.1332433029523372, 248.0919295262283981, 11.24052392390482957 ) ) ;
#99970=CARTESIAN_POINT ( 'NONE',  ( 208.2124092825819162, 270.0125236866795149, -2.339659020816897694 ) ) ;
#99972=CARTESIAN_POINT ( 'NONE',  ( 31.13589176296283156, 188.7833772461660544, -9.188101187500095079 ) ) ;
#99978=CARTESIAN_POINT ( 'NONE',  ( 194.8339595175698378, 275.1781515239682676, -15.70821246309850672 ) ) ;
#99979=CARTESIAN_POINT ( 'NONE',  ( 58.76725448063633195, 213.9244531367911577, -4.594050593750046652 ) ) ;
#99980=CARTESIAN_POINT ( 'NONE',  ( 161.4025183475459073, 251.0896330829197041, 14.50747140106038735 ) ) ;
#99984=VERTEX_POINT ( 'NONE', #68188 ) ;
#99985=CARTESIAN_POINT ( 'NONE',  ( 8.321535033790441460, 185.6115022471903160, -5.000000000000047962 ) ) ;
#99986=CARTESIAN_POINT ( 'NONE',  ( 208.1876422586379647, 270.0554214305024630, 3.377638779759113863 ) ) ;
#99988=CARTESIAN_POINT ( 'NONE',  ( 142.3122500695552048, 240.7202760586659736, -5.415160957724236172E-17 ) ) ;
#99990=CARTESIAN_POINT ( 'NONE',  ( 167.4707736170151406, 262.2158691502890520, -17.12968171664879691 ) ) ;
#99994=CARTESIAN_POINT ( 'NONE',  ( 184.5123196318015459, 277.1383014161853566, -17.82024832176989904 ) ) ;
#99997=CARTESIAN_POINT ( 'NONE',  ( 150.6571681785161445, 269.7011255207979730, 15.24894850018880454 ) ) ;
#99998=CARTESIAN_POINT ( 'NONE',  ( 181.6560639069089405, 287.6780009453752882, 13.46709141213204219 ) ) ;
#100001=ORIENTED_EDGE ( 'NONE', *, *, #41012, .T. ) ;
#100002=CARTESIAN_POINT ( 'NONE',  ( 159.8726974749943679, 253.7393605606583264, 15.54228686887359956 ) ) ;
#100004=CARTESIAN_POINT ( 'NONE',  ( -11.32641631811688221, 164.2677522451418781, 10.00000000000009592 ) ) ;
#100005=CARTESIAN_POINT ( 'NONE',  ( 204.6235849755581455, 276.2285497258825444, -13.59355699282649432 ) ) ;
#100008=CYLINDRICAL_SURFACE ( 'NONE', #52546, 10.00000000000010658 ) ;
#100009=CARTESIAN_POINT ( 'NONE',  ( 163.2742264920156572, 247.8477394797576778, -9.850275379362519956 ) ) ;
#100010=CARTESIAN_POINT ( 'NONE',  ( 201.4463813434794019, 281.7316278426353620, -17.16864527463587820 ) ) ;
#100015=CARTESIAN_POINT ( 'NONE',  ( 190.2318383114841254, 301.1557861577188078, 3.177919994438449525 ) ) ;
#100016=CARTESIAN_POINT ( 'NONE',  ( 12.05626958406296367, 177.7677522451418497, 10.00000000000009592 ) ) ;
#100022=CARTESIAN_POINT ( 'NONE',  ( 164.3010377730689981, 246.0692501711882869, 7.247566249275159578 ) ) ;
#100025=CARTESIAN_POINT ( 'NONE',  ( 108.0499464844507997, 227.0643266524160140, 9.188101187500095079 ) ) ;
#100026=CARTESIAN_POINT ( 'NONE',  ( 203.6508973255666035, 277.9132941555627667, 15.44333727097066422 ) ) ;
#100027=B_SPLINE_CURVE_WITH_KNOTS ( 'NONE', 3,
 ( #62663, #94617, #63680, #39356, #24183, #77900, #85536, #31272, #25695, #32274 ),
 .UNSPECIFIED., .F., .F.,
 ( 4, 2, 2, 2, 4 ),
 ( 0.0002305552267270035902, 0.0005655946974594315644, 0.0009006341681918596199, 0.001235673638924287675, 0.001570713109656715623 ),
 .UNSPECIFIED. ) ;
#100028=CARTESIAN_POINT ( 'NONE',  ( 190.8604783348975502, 300.0669496974951471, 7.597731640149610222 ) ) ;
#100029=CARTESIAN_POINT ( 'NONE',  ( 133.6606700321278822, 254.6427522451419350, 10.00000000000009415 ) ) ;
#100032=VERTEX_POINT ( 'NONE', #75324 ) ;
#100035=ORIENTED_EDGE ( 'NONE', *, *, #21958, .T. ) ;
#100037=VERTEX_POINT ( 'NONE', #90558 ) ;
#100038=CARTESIAN_POINT ( 'NONE',  ( 164.3890147726454813, 245.9168695380243435, -6.010262808998044548 ) ) ;
#100041=CARTESIAN_POINT ( 'NONE',  ( 165.0577600008269883, 270.9917206407381514, 16.89019733054558969 ) ) ;
#100042=CARTESIAN_POINT ( 'NONE',  ( 170.4487297494370068, 283.5218045407765999, 12.45913950463387643 ) ) ;
#100043=CARTESIAN_POINT ( 'NONE',  ( 194.9757425430702824, 292.9391030023704161, -15.21392314336593365 ) ) ;
#100046=CARTESIAN_POINT ( 'NONE',  ( 160.3361140697378175, 267.4248822269044581, -17.47555075248032708 ) ) ;
#100048=CARTESIAN_POINT ( 'NONE',  ( 198.3719234351756029, 277.2891842173528403, -15.30621120788534917 ) ) ;
#100050=CARTESIAN_POINT ( 'NONE',  ( 184.6894110187365641, 293.7322318964822330, -10.88359728165448814 ) ) ;
#100052=CARTESIAN_POINT ( 'NONE',  ( 202.8167949821795446, 279.3580017930215149, 15.61966256214195070 ) ) ;
#100053=CARTESIAN_POINT ( 'NONE',  ( 185.2624990347796938, 257.9745213621091011, 3.033248750312471653 ) ) ;
#100059=CARTESIAN_POINT ( 'NONE',  ( 161.4726291907278721, 250.9681975403669867, 14.52346149734912117 ) ) ;
#100060=CARTESIAN_POINT ( 'NONE',  ( 160.5742256730731583, 282.6976774816733382, 2.097923326525145793 ) ) ;
#100061=VERTEX_POINT ( 'NONE', #53972 ) ;
#100062=CARTESIAN_POINT ( 'NONE',  ( 154.9942266892510361, 262.1891198248060846, -17.67321467605961871 ) ) ;
#100065=CARTESIAN_POINT ( 'NONE',  ( 3.756859464462060760, 179.6427522451419065, 10.00000000000009237 ) ) ;
#100069=CARTESIAN_POINT ( 'NONE',  ( 163.3870428549289784, 247.6523358072665815, -7.780367076891364420 ) ) ;
#100072=CARTESIAN_POINT ( 'NONE',  ( -5.724140937729833567, 161.3768266524159856, -9.188101187500091527 ) ) ;
#100074=CARTESIAN_POINT ( 'NONE',  ( 185.0750477229287867, 295.3417862086006380, 8.418566005137394725 ) ) ;
#100077=ORIENTED_EDGE ( 'NONE', *, *, #39277, .T. ) ;
#100080=CARTESIAN_POINT ( 'NONE',  ( 200.1294354126899009, 267.3366221627135246, -6.812218948514619399 ) ) ;
#100081=CARTESIAN_POINT ( 'NONE',  ( 162.0682692095595883, 276.6943036601504105, -14.28009534788524526 ) ) ;
#100084=CARTESIAN_POINT ( 'NONE',  ( 150.1307102130038231, 276.5622851665610824, 3.568617551434344559 ) ) ;
#100086=CARTESIAN_POINT ( 'NONE',  ( 19.79611131033658111, 191.4244531367911293, -4.594050593750046652 ) ) ;
#100087=CARTESIAN_POINT ( 'NONE',  ( 118.9835172072293403, 233.3768266524159856, -9.188101187500091527 ) ) ;
#100088=CARTESIAN_POINT ( 'NONE',  ( 182.0098606054055210, 294.2529630713442543, -6.366687197579980584 ) ) ;
#100089=CARTESIAN_POINT ( 'NONE',  ( 195.9586221255882776, 275.1547539371241555, 15.85971286464221741 ) ) ;
#100090=CARTESIAN_POINT ( 'NONE',  ( 149.9971034782919901, 271.5943028541292961, -11.77181595469703801 ) ) ;
#100092=CARTESIAN_POINT ( 'NONE',  ( -22.42236680055709641, 157.8615022471902591, 0.000000000000000000 ) ) ;
#100093=CARTESIAN_POINT ( 'NONE',  ( 190.3905927289960971, 299.7902959769909899, -5.393858292934030629 ) ) ;
#100094=CARTESIAN_POINT ( 'NONE',  ( -3.985554314188680003, 180.0530062829863311, 2.649461200531984646E-14 ) ) ;
#100095=B_SPLINE_CURVE_WITH_KNOTS ( 'NONE', 3,
 ( #56260, #33477, #49182, #87252 ),
 .UNSPECIFIED., .F., .F.,
 ( 4, 4 ),
 ( 0.02312224046294886898, 0.03234813536990691768 ),
 .UNSPECIFIED. ) ;
#100096=CARTESIAN_POINT ( 'NONE',  ( 194.4904290197884507, 293.7796906822950973, 14.50206953321744940 ) ) ;
#100098=CARTESIAN_POINT ( 'NONE',  ( 147.8163551302855296, 274.6215580551378821, -9.286329195885331345 ) ) ;
#100099=EDGE_CURVE ( 'NONE', #34618, #79381, #51238, .T. ) ;
#100100=CARTESIAN_POINT ( 'NONE',  ( 192.9863139185010823, 264.4497099342635806, 7.363406893430973099 ) ) ;
#100102=CARTESIAN_POINT ( 'NONE',  ( 192.5288239906588501, 265.2667636152285695, 7.994842260408330681 ) ) ;
#100105=CARTESIAN_POINT ( 'NONE',  ( 180.7712245451587023, 266.8564272240600417, -14.74105925231339675 ) ) ;
#100107=CARTESIAN_POINT ( 'NONE',  ( 152.3600061869313151, 268.0394768385043562, -15.51231027857158296 ) ) ;
#100109=CARTESIAN_POINT ( 'NONE',  ( 93.32751462011533761, 218.5643266524159856, -9.188101187500093303 ) ) ;
#100114=CARTESIAN_POINT ( 'NONE',  ( 194.8910033813863549, 278.9852380238355636, 16.30296749755410701 ) ) ;
#100115=CARTESIAN_POINT ( 'NONE',  ( 201.2627494921372318, 270.3193672810561452, -10.16707981755825507 ) ) ;
#100117=CARTESIAN_POINT ( 'NONE',  ( 149.9316386813282236, 271.7027146890849281, -11.63601498884044894 ) ) ;
#100121=ORIENTED_EDGE ( 'NONE', *, *, #80960, .F. ) ;
#100124=CARTESIAN_POINT ( 'NONE',  ( 198.0865539926831786, 269.0539714184355944, 9.273410383773954990 ) ) ;
#100127=CARTESIAN_POINT ( 'NONE',  ( 178.3110643035489886, 275.2106633751148479, 17.78055932151059793 ) ) ;
#100128=CARTESIAN_POINT ( 'NONE',  ( 183.4588407225135427, 264.5390380599170044, -13.26433237259526621 ) ) ;
#100129=CARTESIAN_POINT ( 'NONE',  ( 169.6418323749134345, 251.5059543197026812, -8.381711355332001290 ) ) ;
#100131=ORIENTED_EDGE ( 'NONE', *, *, #91967, .T. ) ;
#100132=CARTESIAN_POINT ( 'NONE',  ( 187.2079099222287937, 278.7762914448292122, 17.37045700181085550 ) ) ;
#100136=CARTESIAN_POINT ( 'NONE',  ( 164.5318270625157595, 247.4890712181827155, 7.205085160949176171 ) ) ;
#100137=ADVANCED_FACE ( 'NONE', ( #83943 ), #60577, .T. ) ;
#100138=CARTESIAN_POINT ( 'NONE',  ( 162.8384627734353387, 250.8402808221231624, -13.07578932517241732 ) ) ;
#100142=CARTESIAN_POINT ( 'NONE',  ( 158.8847951277724917, 256.6110959850601603, 16.62687674433572127 ) ) ;
#100144=CARTESIAN_POINT ( 'NONE',  ( 153.3367249302040705, 265.0599970851101830, -17.04307279798755559 ) ) ;
#100145=CARTESIAN_POINT ( 'NONE',  ( 184.5457051153594534, 294.3635293766698169, 10.03055039675435367 ) ) ;
#100150=B_SPLINE_CURVE_WITH_KNOTS ( 'NONE', 3,
 ( #82255, #52774, #58392, #11827 ),
 .UNSPECIFIED., .F., .F.,
 ( 4, 4 ),
 ( 0.002886184705558822276, 0.005727001040976496295 ),
 .UNSPECIFIED. ) ;
#100151=CARTESIAN_POINT ( 'NONE',  ( 182.5031894693219670, 295.9323099816722333, -5.011938148712897778 ) ) ;
#100152=EDGE_LOOP ( 'NONE', ( #3260, #91567, #35646, #74615 ) ) ;
#100153=CARTESIAN_POINT ( 'NONE',  ( 162.7890279636430364, 249.1383057319267493, 10.33273309180607491 ) ) ;
#100154=ORIENTED_EDGE ( 'NONE', *, *, #31281, .F. ) ;
#100156=CARTESIAN_POINT ( 'NONE',  ( 172.7281400051620039, 270.9921178062206195, 16.43065513605655070 ) ) ;
#100159=CARTESIAN_POINT ( 'NONE',  ( 152.6969771497951172, 279.2759573534439710, -2.920195053487867121 ) ) ;
#100160=CARTESIAN_POINT ( 'NONE',  ( 185.5235952014877512, 282.2194209058775414, -17.36127342983063215 ) ) ;
#100161=CARTESIAN_POINT ( 'NONE',  ( 164.7680996532798474, 245.2602752643843189, -0.9068639473870550027 ) ) ;
#100164=CARTESIAN_POINT ( 'NONE',  ( 192.5551423381268989, 297.1317055421444024, -13.20528585388119858 ) ) ;
#100165=CARTESIAN_POINT ( 'NONE',  ( 167.7051095246463319, 249.2567869413913684, -5.463550535418292498 ) ) ;
#100168=CARTESIAN_POINT ( 'NONE',  ( 178.0611136682076676, 255.4120370626262684, 5.423495861868194545 ) ) ;
#100169=CARTESIAN_POINT ( 'NONE',  ( 110.8370318831756975, 243.9869531367911009, 4.594050593750046652 ) ) ;
#100170=CARTESIAN_POINT ( 'NONE',  ( 186.8172687208401044, 262.5460427968739623, -10.14177788183279993 ) ) ;
#100172=CARTESIAN_POINT ( 'NONE',  ( 189.1495590004746532, 292.1788078851117234, -14.37282464736753163 ) ) ;
#100177=CARTESIAN_POINT ( 'NONE',  ( 204.6280226557913977, 269.5216201328459533, -5.879895947628904551 ) ) ;
#100181=CARTESIAN_POINT ( 'NONE',  ( 90.08876690777121610, 229.4865022471902876, -10.00000000000009592 ) ) ;
#100182=ORIENTED_EDGE ( 'NONE', *, *, #60897, .T. ) ;
#100183=CARTESIAN_POINT ( 'NONE',  ( 194.8996939547756426, 293.0708230211409386, 16.59726544114578672 ) ) ;
#100184=EDGE_CURVE ( 'NONE', #96457, #92439, #15243, .T. ) ;
#100185=EDGE_LOOP ( 'NONE', ( #89398, #92922, #39959, #77187 ) ) ;
#100189=CARTESIAN_POINT ( 'NONE',  ( 191.8581106210131679, 267.6082157204258465, -12.54179644138010552 ) ) ;
#100190=B_SPLINE_CURVE_WITH_KNOTS ( 'NONE', 3,
 ( #89588, #50523, #43423, #49534, #26248, #20152, #72871, #27247, #35831, #41424, #88603, #81476, #51021, #3939, #74369, #72369, #34822, #57122, #80994, #80488, #73843, #66727, #26740, #3462, #34340, #87619, #4952, #4432, #25757, #35330, #56636, #49047, #57625, #50041, #19167, #11559, #79983, #42417, #73351, #36322 ),
 .UNSPECIFIED., .F., .F.,
 ( 4, 2, 2, 2, 2, 2, 2, 2, 2, 2, 2, 2, 2, 2, 2, 2, 2, 2, 2, 4 ),
 ( 0.0008994082332149132882, 0.0009941114596324087359, 0.001088814686049904184, 0.001278221138884895079, 0.001657034044554877086, 0.002414659855894735717, 0.003929911478574387926, 0.004687537289914170228, 0.005066350195584095641, 0.005255756648419022785, 0.005350459874836527990, 0.005445163101254034063, 0.005492514714462768018, 0.005539866327671501972, 0.005634569554088842379, 0.005823976006923523192, 0.006013382459758203138, 0.006202788912592883952, 0.006581601818262287212, 0.006960414723931690473 ),
 .UNSPECIFIED. ) ;
#100192=CARTESIAN_POINT ( 'NONE',  ( 172.9311764467664716, 268.4779053881692334, -17.72160738022306603 ) ) ;
#100193=CARTESIAN_POINT ( 'NONE',  ( 204.6442892731280949, 273.0279791680289918, -9.871948230970470917 ) ) ;
#100195=CARTESIAN_POINT ( 'NONE',  ( 156.8490694893153261, 280.4450466293991440, 5.967606550010729372 ) ) ;
#100196=CARTESIAN_POINT ( 'NONE',  ( 153.4613150239306094, 264.8442007126561748, -16.86932470306368259 ) ) ;
#100197=VERTEX_POINT ( 'NONE', #62071 ) ;
#100198=CARTESIAN_POINT ( 'NONE',  ( 146.7879906441258129, 276.4027375938661635, 4.347255311287614887 ) ) ;
#100200=CARTESIAN_POINT ( 'NONE',  ( 163.6904632199346281, 247.9665650504956034, -8.459347815224287359 ) ) ;
#100201=CARTESIAN_POINT ( 'NONE',  ( 173.8053086200644088, 250.7437096766582556, -1.005346080584223811 ) ) ;
#100203=CARTESIAN_POINT ( 'NONE',  ( 185.4902135326318842, 296.9785454517182188, -4.308934458819135394 ) ) ;
#100206=CARTESIAN_POINT ( 'NONE',  ( 191.1373190028791953, 283.3211107657666616, -16.58886392611601224 ) ) ;
#100207=ADVANCED_FACE ( 'NONE', ( #93019 ), #11162, .F. ) ;
#100209=CARTESIAN_POINT ( 'NONE',  ( 82.23173768200972233, 206.0327760586659451, 1.948934522072303157E-15 ) ) ;
#100211=CARTESIAN_POINT ( 'NONE',  ( 193.1569697810063531, 296.0893098336876506, -13.02398914535779539 ) ) ;
#100212=CARTESIAN_POINT ( 'NONE',  ( 208.0421103033489771, 270.3074901711881353, -2.473242163239977476 ) ) ;
#100214=CARTESIAN_POINT ( 'NONE',  ( 155.0619429961492983, 262.0718317407570339, -17.08853361476647592 ) ) ;
#100215=CARTESIAN_POINT ( 'NONE',  ( 161.8750289368003621, 250.2712207352165592, -13.97436367953006098 ) ) ;
#100217=CARTESIAN_POINT ( 'NONE',  ( 162.7020145476934090, 284.0983276010327359, 6.051621772638641872 ) ) ;
#100220=CARTESIAN_POINT ( 'NONE',  ( 168.7012044067234910, 251.7376076084256624, -8.789497580350094097 ) ) ;
#100221=CARTESIAN_POINT ( 'NONE',  ( 164.5803890871363819, 245.5853995020621028, -4.343210071565205332 ) ) ;
#100222=CARTESIAN_POINT ( 'NONE',  ( 157.8092552871339365, 257.3133472685137235, 17.04082256169242626 ) ) ;
#100224=CARTESIAN_POINT ( 'NONE',  ( 22.82720022358212120, 193.1744531367911293, 4.594050593750047540 ) ) ;
#100225=CARTESIAN_POINT ( 'NONE',  ( 54.68078388046974680, 208.5024278399160664, -9.188101187500093303 ) ) ;
#100226=CARTESIAN_POINT ( 'NONE',  ( 163.8858323887012034, 247.1950272763415626, -6.367529170130759475 ) ) ;
#100229=CARTESIAN_POINT ( 'NONE',  ( 137.8731756836298814, 262.6589784336661069, -6.496448406907675876E-16 ) ) ;
#100232=CARTESIAN_POINT ( 'NONE',  ( 199.6771794652913457, 271.0505596696440307, -11.15657419087213320 ) ) ;
#100235=CARTESIAN_POINT ( 'NONE',  ( -9.864998445682726214, 165.1115022471902591, 10.00000000000009592 ) ) ;
#100236=CARTESIAN_POINT ( 'NONE',  ( 149.2923684163597784, 272.0650280510108701, -12.99082738998495756 ) ) ;
#100238=CARTESIAN_POINT ( 'NONE',  ( 71.83943283659647250, 200.0327760586659451, 1.948934522072302763E-15 ) ) ;
#100241=CARTESIAN_POINT ( 'NONE',  ( 159.5204760365350012, 254.3494259875849082, 16.90107507090185379 ) ) ;
#100243=CARTESIAN_POINT ( 'NONE',  ( 152.9995685277916380, 276.6655034792656807, 7.180448585384231919 ) ) ;
#100246=CARTESIAN_POINT ( 'NONE',  ( 114.3374782137354941, 243.4865022471903160, 10.00000000000009237 ) ) ;
#100247=CARTESIAN_POINT ( 'NONE',  ( 161.4844649541891499, 250.9476973967054789, 12.93553496455142415 ) ) ;
#100248=CARTESIAN_POINT ( 'NONE',  ( 164.6460902696047128, 245.4716017159096566, -3.036414139157908476 ) ) ;
#100253=CARTESIAN_POINT ( 'NONE',  ( 206.1798448551755598, 273.5330285446045195, -10.53862763475382813 ) ) ;
#100254=CARTESIAN_POINT ( 'NONE',  ( 190.3891352057751192, 278.7747448885224912, -16.51623031618344939 ) ) ;
#100259=CARTESIAN_POINT ( 'NONE',  ( 194.6782745185928434, 293.4543327343926080, -14.56555309295305634 ) ) ;
#100260=B_SPLINE_CURVE_WITH_KNOTS ( 'NONE', 3,
 ( #7317, #69616, #16414, #100042, #69115, #76723, #30628, #77222, #38197, #61513, #47310, #78236, #54911, #14911, #23006, #83872, #99540, #14435, #37708, #61004, #53900, #46817, #45316, #70612, #84858, #77740, #76250, #8325, #1226, #15401, #46293, #39190, #68617, #61994, #85890, #38708, #70105, #92945, #221, #22524, #31599, #31106, #23499, #62492 ),
 .UNSPECIFIED., .F., .F.,
 ( 4, 2, 2, 2, 2, 2, 2, 2, 2, 2, 2, 2, 2, 2, 2, 2, 2, 2, 2, 2, 2, 4 ),
 ( 0.0003810264101704981731, 0.001396625271846183014, 0.001904424702684024730, 0.002158324418102970741, 0.002285274275812445265, 0.002412224133521920222, 0.002666123848940999373, 0.002920023564360078091, 0.003427822995198067692, 0.004443421856874149242, 0.005459020718550229925, 0.005966820149388226899, 0.006220719864807147323, 0.006474619580226067747, 0.006538094509080816068, 0.006601569437935564388, 0.006665044366790312709, 0.006728519295645061030, 0.006982419011064167069, 0.007490218441902337515, 0.007998017872740507961, 0.008505817303578678407 ),
 .UNSPECIFIED. ) ;
#100266=ORIENTED_EDGE ( 'NONE', *, *, #70795, .T. ) ;
#100270=CARTESIAN_POINT ( 'NONE',  ( 174.4336096923461525, 286.7838703873537156, 11.78196039751662028 ) ) ;
#100271=CARTESIAN_POINT ( 'NONE',  ( 163.2660837978642689, 283.7406608692818963, -3.062460295508294905 ) ) ;
#100273=CARTESIAN_POINT ( 'NONE',  ( 163.3473224498206093, 247.7211335670114352, -10.00320358166632850 ) ) ;
#100274=CARTESIAN_POINT ( 'NONE',  ( 204.9780665305064531, 275.6145696623662502, 14.10615427165218883 ) ) ;
#100275=CARTESIAN_POINT ( 'NONE',  ( 188.5443543987748853, 294.9864749104084467, -11.10675611966633802 ) ) ;
#100276=CARTESIAN_POINT ( 'NONE',  ( 204.8057697639265768, 275.9129964160624695, -12.68356524114230766 ) ) ;
#100277=CARTESIAN_POINT ( 'NONE',  ( 137.6570164284488271, 250.2833772461660544, -9.188101187500095079 ) ) ;
#100279=CARTESIAN_POINT ( 'NONE',  ( 177.6153776630306140, 268.7380174264160928, 17.31615970785065173 ) ) ;
#100280=CARTESIAN_POINT ( 'NONE',  ( 178.8130962031900992, 258.0706443509022279, 9.810816441170940649 ) ) ;
#100281=CARTESIAN_POINT ( 'NONE',  ( 67.18419919549008057, 209.5958772461660544, -9.188101187500095079 ) ) ;
#100283=CARTESIAN_POINT ( 'NONE',  ( 191.5766842709549280, 298.8264446275616137, 8.039910086100929831 ) ) ;
#100285=DIRECTION ( 'NONE',  ( -0.4999999999999987788, 0.8660254037844392627, 0.000000000000000000 ) ) ;
#100287=CARTESIAN_POINT ( 'NONE',  ( 157.1930958003661090, 258.3805668051609814, -18.40493736487525211 ) ) ;
#100288=ORIENTED_EDGE ( 'NONE', *, *, #20789, .F. ) ;
#100291=CARTESIAN_POINT ( 'NONE',  ( 197.8448660367628520, 287.0410319951262181, 16.94590693131541315 ) ) ;
#100292=CARTESIAN_POINT ( 'NONE',  ( 147.1259762202154207, 275.8173294038533641, -0.6716460511724978710 ) ) ;
#100294=CARTESIAN_POINT ( 'NONE',  ( 155.5660013421004919, 261.1987770755905558, 17.28709111629370199 ) ) ;
#100332=COLOUR_RGB('Black',0.12,0.14,0.17);
#100333=FILL_AREA_STYLE_COLOUR('',#100332);
#100334=FILL_AREA_STYLE('',(#100333));
#100335=SURFACE_STYLE_FILL_AREA(#100334);
#100336=SURFACE_SIDE_STYLE('',(#100335));
#100337=SURFACE_STYLE_USAGE(.BOTH.,#100336);
#100338=PRESENTATION_STYLE_ASSIGNMENT((#100337));
ENDSEC;
END-ISO-10303-21;
